#87411=DIRECTION('ref_axis',(0.666102343611793,-0.0042812889172255,-0.745848066565896));
#87412=DIRECTION('',(-0.998646620316722,0.,-0.0520089197156425));
#87413=DIRECTION('center_axis',(-0.113998684179924,-0.987363722714415,-0.110078058998048));
#87414=DIRECTION('ref_axis',(0.807888800879984,-0.0276461771046428,-0.588686142442813));
#87415=DIRECTION('center_axis',(0.110880275037949,-0.987366232725912,0.113196674333434));
#87416=DIRECTION('ref_axis',(0.84938348857533,0.035011289492792,-0.526613614468572));
#87417=DIRECTION('',(0.26547247756443,0.,-0.964118438603786));
#87418=DIRECTION('center_axis',(2.40783168670246E-14,-1.,-1.73734121000225E-14));
#87419=DIRECTION('ref_axis',(1.,2.40783168670246E-14,4.08008794519545E-31));
#87420=DIRECTION('center_axis',(-0.0728831555136991,0.987363722760243,-0.140715758248324));
#87421=DIRECTION('ref_axis',(0.767503369580905,-0.0345726406209256,-0.640111951304187));
#87422=DIRECTION('center_axis',(0.0961353783662722,0.987363722591744,0.12597963460872));
#87423=DIRECTION('ref_axis',(0.81086452814338,-0.0042812878077453,-0.585218239269352));
#87424=DIRECTION('',(-0.964118437085268,0.,-0.265472483079246));
#87425=DIRECTION('center_axis',(-0.0876699255670326,-0.987363722825506,
-0.132010844248598));
#87426=DIRECTION('ref_axis',(0.915550928733872,-0.0276461726499358,-0.401250776986605));
#87427=DIRECTION('center_axis',(0.0839540246621183,-0.98736623247613,0.134386177521815));
#87428=DIRECTION('ref_axis',(0.942731734454702,0.0350112977016713,-0.331709339460428));
#87429=DIRECTION('',(0.466522844039702,0.,-0.884509149748666));
#87430=DIRECTION('center_axis',(-1.6350089538668E-13,-1.,7.07466299821404E-14));
#87431=DIRECTION('ref_axis',(1.,-1.6350089538668E-13,-1.81849133261287E-30));
#87432=DIRECTION('center_axis',(-0.0409294619248677,0.987363722825902,-0.153093624929051));
#87433=DIRECTION('ref_axis',(0.887164714821792,-0.0345726379632342,-0.460155953432563));
#87434=DIRECTION('center_axis',(0.0668058915489451,0.987363722561016,0.143700564455411));
#87435=DIRECTION('ref_axis',(0.91771158853251,-0.00428129039750786,-0.397224257599745));
#87436=DIRECTION('',(-0.88450914743618,0.,-0.466522848424086));
#87437=DIRECTION('center_axis',(-0.0572418275556243,-0.987363722669453,
-0.147770945501514));
#87438=DIRECTION('ref_axis',(0.980402912820427,-0.0276461782575986,-0.195053370545015));
#87439=DIRECTION('center_axis',(0.053102164630045,-0.987366232647523,0.149291937957282));
#87440=DIRECTION('ref_axis',(0.99199889342554,0.0350112918481292,-0.121294702628058));
#87441=DIRECTION('',(0.64575912037299,0.,-0.763541196305152));
#87442=DIRECTION('center_axis',(-2.91477949413467E-14,-1.,5.65745894311796E-15));
#87443=DIRECTION('ref_axis',(1.,-2.91477949413467E-14,2.51222006692366E-32));
#87444=DIRECTION('center_axis',(-0.00706194962947178,0.987363722828334,
-0.158313005498612));
#87445=DIRECTION('ref_axis',(0.9653432251743,-0.0345726379281121,-0.258683571795296));
#87446=DIRECTION('center_axis',(0.0343526394950947,0.987363722496506,0.154702216071917));
#87447=DIRECTION('ref_axis',(0.981647474883865,-0.00428129655811406,-0.190656511963041));
#87448=DIRECTION('',(-0.763541191686731,0.,-0.645759125833779));
#87449=DIRECTION('',(0.794800418951332,0.,-0.606870903928329));
#87450=DIRECTION('',(-0.606870901804627,0.,-0.794800420572888));
#87451=DIRECTION('center_axis',(0.0100961397169233,-0.98736372283294,-0.158148496029187));
#87452=DIRECTION('ref_axis',(0.971690369534208,-0.0276461723068847,0.234634854425451));
#87453=DIRECTION('center_axis',(-0.0144918387531781,-0.987366232640024,
0.15779071345234));
#87454=DIRECTION('ref_axis',(0.951244135720145,0.0350112914715787,0.306445433523697));
#87455=DIRECTION('',(0.906677731515565,0.,-0.421824004975759));
#87456=DIRECTION('center_axis',(2.88293275590696E-14,-1.,7.10427075007399E-15));
#87457=DIRECTION('ref_axis',(1.,2.88293275590696E-14,-2.33857374721434E-31));
#87458=DIRECTION('center_axis',(0.0600646558953371,0.987363722772028,-0.146646227588495));
#87459=DIRECTION('ref_axis',(0.984740195112118,-0.0345726400867478,0.170562248718703));
#87460=DIRECTION('center_axis',(-0.0337801645468462,0.987363722504648,0.154828227287382));
#87461=DIRECTION('ref_axis',(0.970973710277041,-0.00428129541679956,0.239147913351531));
#87462=DIRECTION('',(-0.421824000481472,0.,-0.906677733606493));
#87463=DIRECTION('center_axis',(0.0438573487855876,-0.987363722845839,-0.15228070056808));
#87464=DIRECTION('ref_axis',(0.898533230833495,-0.0276461728542834,0.438033928154466));
#87465=DIRECTION('center_axis',(-0.0480733690119884,-0.987366232709415,
0.150986336127));
#87466=DIRECTION('ref_axis',(0.863127866602312,0.0350112889476249,0.503770280525527));
#87467=DIRECTION('',(0.976159801597288,0.,-0.217053085086444));
#87468=DIRECTION('center_axis',(1.06512422773008E-13,-1.,5.25425203349921E-14));
#87469=DIRECTION('ref_axis',(1.,1.06512422773008E-13,-2.10878361398876E-32));
#87470=DIRECTION('center_axis',(0.0901849798539102,0.987363722846681,-0.130305595486506));
#87471=DIRECTION('ref_axis',(0.925051675281031,-0.0345726381980344,0.37826463057995));
#87472=DIRECTION('center_axis',(-0.0662738964295295,0.987363722501191,0.143946692010062));
#87473=DIRECTION('ref_axis',(0.896863152081214,-0.00428129419318685,0.442287414425258));
#87474=DIRECTION('',(-0.217053076899258,0.,-0.976159803417742));
#87475=DIRECTION('center_axis',(0.0755678353822223,-0.987363722751612,-0.13929243069788));
#87476=DIRECTION('ref_axis',(0.783361677221614,-0.0276461756599869,0.620951021926784));
#87477=DIRECTION('center_axis',(-0.0794070357866266,-0.987366232591193,
0.137122009197124));
#87478=DIRECTION('ref_axis',(0.734652698085276,0.0350112936683274,0.677539388162558));
#87479=DIRECTION('',(0.999997725152046,0.,-0.00213300040646513));
#87480=DIRECTION('center_axis',(9.27271328152013E-14,-1.,7.42111278501564E-14));
#87481=DIRECTION('ref_axis',(1.,9.27271328152013E-14,1.68823144866391E-30));
#87482=DIRECTION('center_axis',(0.116088355864864,0.987363722833873,-0.107872018912356));
#87483=DIRECTION('ref_axis',(0.822108766551035,-0.0345726372684886,0.568279780312688));
#87484=DIRECTION('center_axis',(-0.0956687346786959,0.987363722549271,0.126334368240095));
#87485=DIRECTION('ref_axis',(0.780816270242319,-0.00428129210391877,0.624746046536347));
#87486=DIRECTION('',(-0.00213299544913877,0.,-0.99999772516262));
#87487=DIRECTION('center_axis',(0.103744855571448,-0.98736372273247,-0.11979100122437));
#87488=DIRECTION('ref_axis',(0.631561003133862,-0.0276461768120529,0.774833135731963));
#87489=DIRECTION('center_axis',(-0.107027725080779,-0.987366232739294,0.116846003398692));
#87490=DIRECTION('ref_axis',(0.571825985200744,0.0350112887521891,0.819627508267694));
#87491=DIRECTION('',(0.977076865850012,0.,0.212886820213741));
#87492=DIRECTION('center_axis',(5.59545188505727E-14,-1.,6.930727908743E-14));
#87493=DIRECTION('ref_axis',(1.90179785867072E-30,-6.930727908743E-14,-1.));
#87494=DIRECTION('center_axis',(0.136563569902686,0.987363722841023,-0.0803944661836259));
#87495=DIRECTION('ref_axis',(0.68072496630421,-0.0345726372125825,0.731722797927125));
#87496=DIRECTION('center_axis',(-0.120590206989186,0.987363722543446,0.10281479165691));
#87497=DIRECTION('ref_axis',(0.628259286757571,-0.00428129314207606,0.777992248760809));
#87498=DIRECTION('',(0.212886825057003,0.,-0.977076864794756));
#87499=DIRECTION('center_axis',(0.127070884961093,-0.987363722842759,-0.0946882728181883));
#87500=DIRECTION('ref_axis',(0.450229235832201,-0.0276461724272758,0.892484915475928));
#87501=DIRECTION('center_axis',(-0.129643916496959,-0.987366232921069,0.0911064048384507));
#87502=DIRECTION('ref_axis',(0.382261324293031,0.0350112812986391,0.923390757010035));
#87503=DIRECTION('',(0.90846897872148,0.,0.417952287588848));
#87504=DIRECTION('center_axis',(-3.97473170466724E-14,-1.,-7.97154810525488E-14));
#87505=DIRECTION('ref_axis',(1.34542241016887E-30,7.97154810525487E-14,
-1.));
#87506=DIRECTION('center_axis',(0.150653221823406,0.987363722937457,-0.0491577601331854));
#87507=DIRECTION('ref_axis',(0.507511223892755,-0.0345726343239725,0.860951270734168));
#87508=DIRECTION('center_axis',(-0.139873017737147,0.987363722559245,0.0744877055832257));
#87509=DIRECTION('ref_axis',(0.446325598059899,-0.00428128909263173,0.894860397537057));
#87510=DIRECTION('',(0.417952293183605,0.,-0.908468976147544));
#87511=DIRECTION('center_axis',(0.144455217576619,-0.98736372279966,-0.0651580310789709));
#87512=DIRECTION('ref_axis',(0.247845252571248,-0.0276461738326995,0.968405090780871));
#87513=DIRECTION('center_axis',(-0.146198094728699,-0.987366232569038,0.061106790785668));
#87514=DIRECTION('ref_axis',(0.174822551263119,0.035011294342318,0.983977278618937));
#87515=DIRECTION('',(0.797382090536838,0.,0.603474773036207));
#87516=DIRECTION('center_axis',(-7.22719159625212E-15,-1.,-2.8798758529663E-14));
#87517=DIRECTION('ref_axis',(1.69754332887121E-32,2.8798758529663E-14,-1.));
#87518=DIRECTION('center_axis',(0.157698499589171,0.987363722825349,-0.0156224862231097));
#87519=DIRECTION('ref_axis',(0.310566820979779,-0.03457263809742,0.949922619165108));
#87520=DIRECTION('center_axis',(-0.152615518808298,0.987363722561227,0.0426776614742487));
#87521=DIRECTION('ref_axis',(0.243522219297542,-0.00428129052954995,0.969885869192763));
#87522=DIRECTION('',(0.60347477560539,0.,-0.797382088592429));
#87523=DIRECTION('center_axis',(0.155084985266925,-0.98736372273477,-0.0325810738327332));
#87524=DIRECTION('ref_axis',(0.0338722990281305,-0.0276461769946432,0.9990437208932));
#87525=DIRECTION('center_axis',(-0.155916218266008,-0.987366232783829,0.0282498715023055));
#87526=DIRECTION('ref_axis',(-0.0407907327075091,0.0350112867431234,0.998554117675039));
#87527=DIRECTION('',(0.649010505773103,0.,0.760779444646174));
#87528=DIRECTION('center_axis',(0.,-1.,0.));
#87529=DIRECTION('ref_axis',(0.0292115385192369,0.,0.999573251951721));
#87530=DIRECTION('center_axis',(0.157369968982369,0.987363722822651,0.0186432753636022));
#87531=DIRECTION('ref_axis',(0.0991006546873935,-0.0345726382874032,0.994476642723387));
#87532=DIRECTION('center_axis',(-0.158221888564979,0.987363722509714,0.00887206011545954));
#87533=DIRECTION('ref_axis',(0.0293320137080374,-0.00428129435385591,0.999560555189373));
#87534=DIRECTION('center_axis',(-0.16378581394621,-0.986495109396061,0.00126739403137102));
#87535=DIRECTION('ref_axis',(0.0279022377807928,-0.00334831589290775,0.999605048960591));
#87536=DIRECTION('center_axis',(0.162023731906375,-0.986495109491454,-0.0239939419140432));
#87537=DIRECTION('ref_axis',(0.13673669353806,-0.00163604997374152,0.990606077096624));
#87538=DIRECTION('center_axis',(-0.159684138304561,-0.986495109470319,0.0364468786739426));
#87539=DIRECTION('ref_axis',(0.242135436420398,-0.00334830841955299,0.970236682083414));
#87540=DIRECTION('center_axis',(0.153077721675863,-0.986495109421554,-0.0582632835830904));
#87541=DIRECTION('ref_axis',(0.346490890519673,-0.00163604293581091,0.938051910157639));
#87542=DIRECTION('center_axis',(-0.148115812598509,-0.986495109422795,0.0699221362888171));
#87543=DIRECTION('ref_axis',(0.445046649327853,-0.00334831284885684,0.895501127147876));
#87544=DIRECTION('center_axis',(0.13697396453894,-0.986495109434819,-0.089808307520348));
#87545=DIRECTION('ref_axis',(0.540043558052671,-0.00163604532087848,0.841635478554415));
#87546=DIRECTION('center_axis',(-0.129621748464855,-0.986495109530296,0.100127924165659));
#87547=DIRECTION('ref_axis',(0.627147978031225,-0.00334830330694471,0.778892933923726));
#87548=DIRECTION('center_axis',(0.114465459146429,-0.986495109423811,-0.117153991589281));
#87549=DIRECTION('ref_axis',(0.708344388266892,-0.00163604390614199,0.705865108197834));
#87550=DIRECTION('center_axis',(-0.105066725885366,-0.986495109424266,0.125651829249456));
#87551=DIRECTION('ref_axis',(0.779924561865009,-0.00334830996305795,0.625864575303687));
#87552=DIRECTION('center_axis',(0.0866046722159151,-0.986495109483246,-0.13902168793398));
#87553=DIRECTION('ref_axis',(0.843523823647868,-0.00163604705472412,0.537089268454058));
#87554=DIRECTION('center_axis',(-0.0755988969195904,-0.98649510943077,0.145300398670181));
#87555=DIRECTION('ref_axis',(0.896232743138345,-0.00334831229899437,0.443571481197186));
#87556=DIRECTION('center_axis',(0.0546943551485009,-0.986495109420496,-0.154388881090361));
#87557=DIRECTION('ref_axis',(0.939261021775134,-0.00163604133811556,0.343199732433856));
#87558=DIRECTION('center_axis',(-0.0425961438623839,-0.986495109459446,
0.158154884656308));
#87559=DIRECTION('ref_axis',(0.970634076275854,-0.00334831006889112,0.240537478975321));
#87560=DIRECTION('center_axis',(0.0202265784150031,-0.986495109504033,-0.162537024859717));
#87561=DIRECTION('ref_axis',(0.991079418779179,-0.00163604856804703,0.133262556696951));
#87562=DIRECTION('center_axis',(-0.00760164204240845,-0.986495109429919,
0.163614223431558));
#87563=DIRECTION('ref_axis',(0.99964963868433,-0.00334830736092119,0.0262562129048713));
#87564=DIRECTION('center_axis',(-0.0151869653104653,-0.986495109510341,
-0.163085115804104));
#87565=DIRECTION('ref_axis',(0.996556043201398,-0.00163605039412049,-0.0829058266823295));
#87566=DIRECTION('center_axis',(0.0277482981921578,-0.986495109405202,0.161423142910355));
#87567=DIRECTION('ref_axis',(0.981922695164601,-0.0033483111612951,-0.189252766249411));
#87568=DIRECTION('center_axis',(-0.0498903778715741,-0.98649510947419,-0.15600752923926));
#87569=DIRECTION('ref_axis',(0.955434815240343,-0.00163604664715935,-0.295197623936948));
#87570=DIRECTION('center_axis',(0.0618007641807002,-0.986495109440824,0.151684094736456));
#87571=DIRECTION('ref_axis',(0.918282137943364,-0.00334830913939569,-0.395912495332078));
#87572=DIRECTION('center_axis',(-0.0822609769858708,-0.98649510948161,-0.141635202665852));
#87573=DIRECTION('ref_axis',(0.869638516258114,-0.00163604780339735,-0.49368631172838));
#87574=DIRECTION('center_axis',(0.0929634947864884,-0.986495109470967,0.134852466150781));
#87575=DIRECTION('ref_axis',(0.81170372863756,-0.003348307097733,-0.584059796386861));
#87576=DIRECTION('center_axis',(-0.110785141534113,-0.986495109446713,-0.120640173462175));
#87577=DIRECTION('ref_axis',(0.743178886612869,-0.00163604553725314,-0.66909077549153));
#87578=DIRECTION('center_axis',(0.119779353350238,-0.986495109452289,0.111715287842424));
#87579=DIRECTION('ref_axis',(0.667170953063073,-0.0033483085449882,-0.744897112505344));
#87580=DIRECTION('center_axis',(-0.134129119919762,-0.986495109493058,-0.0940041389292526));
#87581=DIRECTION('ref_axis',(0.581969039393171,-0.00163605002861843,-0.813209296877559));
#87582=DIRECTION('center_axis',(0.140994461083604,-0.986495109424135,0.0833544301522559));
#87583=DIRECTION('ref_axis',(0.491442007146395,-0.00334831305064004,-0.870903865195027));
#87584=DIRECTION('center_axis',(-0.151201364943228,-0.986495109443453,-0.0629725835856714));
#87585=DIRECTION('ref_axis',(0.393546966780992,-0.00163604463201623,-0.919303055741382));
#87586=DIRECTION('center_axis',(0.155616827764946,-0.986495109435589,0.0510960074373685));
#87587=DIRECTION('ref_axis',(0.292733778957593,-0.00334831188603403,-0.956188121378174));
#87588=DIRECTION('center_axis',(-0.161203605678199,-0.986495109504632,-0.0289964901288311));
#87589=DIRECTION('ref_axis',(0.186723073336949,-0.00163604993960994,-0.982411226128956));
#87590=DIRECTION('center_axis',(0.16296272405839,-0.986495109424208,0.0164483935260796));
#87591=DIRECTION('ref_axis',(0.0803376455401133,-0.00334831203061902,-0.996762083706848));
#87592=DIRECTION('center_axis',(-0.163668143673876,-0.986495109448053,0.00633543853423027));
#87593=DIRECTION('ref_axis',(-0.028831781957428,-0.0016360466685548,-0.99958293888024));
#87594=DIRECTION('center_axis',(0.162688663305374,-0.986495109493919,-0.0189683361550779));
#87595=DIRECTION('ref_axis',(-0.135814987330012,-0.00334830488654736,-0.990728559228478));
#87596=DIRECTION('center_axis',(-0.158479742471285,-0.986495109454043,0.0413711282114918));
#87597=DIRECTION('ref_axis',(-0.24303849268562,-0.00163604274440781,-0.970015265053721));
#87598=DIRECTION('center_axis',(0.154807463282918,-0.98649510940734,-0.0534981161098913));
#87599=DIRECTION('ref_axis',(-0.345617063849709,-0.00334831002481114,-0.938369668092423));
#87600=DIRECTION('center_axis',(-0.145881002803882,-0.986495109476937,0.0744723572812044));
#87601=DIRECTION('ref_axis',(-0.445880998647102,-0.00163604585829139,-0.895090754281046));
#87602=DIRECTION('center_axis',(0.139687636995712,-0.98649510943774,-0.08552638847733));
#87603=DIRECTION('ref_axis',(-0.539258470200199,-0.0033483099529629,-0.842133653963431));
#87604=DIRECTION('center_axis',(-0.12646103108995,-0.98649510948253,0.104091337693001));
#87605=DIRECTION('ref_axis',(-0.627874600291905,-0.0016360454288523,-0.778312796800641));
#87606=DIRECTION('center_axis',(0.118036173957979,-0.986495109402125,-0.113555540433086));
#87607=DIRECTION('ref_axis',(-0.707684749028207,-0.00334831214599302,-0.706520406498395));
#87608=DIRECTION('center_axis',(-0.101127883902599,-0.986495109422555,0.128843122372763));
#87609=DIRECTION('ref_axis',(-0.780509485663125,-0.00163604296041615,-0.625141796837578));
#87610=DIRECTION('center_axis',(0.0908654643575122,-0.986495109472117,-0.136274966060128));
#87611=DIRECTION('ref_axis',(-0.843020475033029,-0.0033483062137657,-0.537871051015562));
#87612=DIRECTION('center_axis',(-0.071066104503773,-0.986495109454203,0.147570348693763));
#87613=DIRECTION('ref_axis',(-0.89664861531436,-0.00163604600655692,-0.442739860424047));
#87614=DIRECTION('center_axis',(0.0594459877428719,-0.986495109509029,-0.152622322928339));
#87615=DIRECTION('ref_axis',(-0.938937501589155,-0.00334830299426047,-0.34407144167538));
#87616=DIRECTION('center_axis',(-0.0376813513430268,-0.986495109508868,
0.159397348397173));
#87617=DIRECTION('ref_axis',(-0.970861451591853,-0.00163605045407286,-0.239635901216558));
#87618=DIRECTION('center_axis',(0.0252468968154617,-0.986495109386897,-0.161833226986684));
#87619=DIRECTION('ref_axis',(-0.990950853825989,-0.00334831436270505,-0.134183434493504));
#87620=DIRECTION('center_axis',(-0.00253466500971984,-0.986495109498837,
0.163771103703207));
#87621=DIRECTION('ref_axis',(-0.999677885568108,-0.00163604943518171,-0.0253268325757907));
#87622=DIRECTION('center_axis',(-0.010132729717057,-0.986495109483762,-0.163476991509819));
#87623=DIRECTION('ref_axis',(-0.996628445590177,-0.00334830604890707,0.081978840484062));
#87624=DIRECTION('center_axis',(0.0327305358517654,-0.986495109457993,0.160487105520406));
#87625=DIRECTION('ref_axis',(-0.981750492616112,-0.00163604488853,0.190166489174997));
#87626=DIRECTION('center_axis',(-0.0450385505003737,-0.986495109440284,
-0.157476753901098));
#87627=DIRECTION('ref_axis',(-0.955704798411601,-0.00334830901293553,0.294307878113712));
#87628=DIRECTION('center_axis',(0.0664652997818561,-0.986495109455715,0.149698907627493));
#87629=DIRECTION('ref_axis',(-0.917917538204367,-0.00163604722328872,0.396767836910097));
#87630=DIRECTION('center_axis',(-0.0778384232825467,-0.986495109488177,
-0.144113076494802));
#87631=DIRECTION('ref_axis',(-0.870093457590691,-0.0033483064689008,0.492875404033988));
#87632=DIRECTION('center_axis',(0.0970922171638184,-0.986495109489498,0.131910956025336));
#87633=DIRECTION('ref_axis',(-0.811163778570785,-0.00163604589998996,0.584816764199334));
#87634=DIRECTION('center_axis',(-0.106998645562323,-0.986495109310941,-0.12401084288651));
#87635=DIRECTION('ref_axis',(-0.743797514851689,-0.00334832064433674,0.66839662300861));
#87636=DIRECTION('center_axis',(0.123179209311741,-0.986495109425282,0.107954997444934));
#87637=DIRECTION('ref_axis',(-0.666480903457418,-0.00163604240632611,0.745520307363809));
#87638=DIRECTION('center_axis',(-0.13115574995207,-0.986495109501473,-0.0981099800437549));
#87639=DIRECTION('ref_axis',(-0.582722423500651,-0.00334830642559605,0.812664362448365));
#87640=DIRECTION('center_axis',(0.143506484117382,-0.986495109477908,0.0789511747375405));
#87641=DIRECTION('ref_axis',(-0.49063412094358,-0.00163604904476048,0.871364150461472));
#87642=DIRECTION('center_axis',(-0.149180147807827,-0.986495109495363,-0.0676216122387367));
#87643=DIRECTION('ref_axis',(-0.394399880085478,-0.00334830475442072,0.918932817698787));
#87644=DIRECTION('center_axis',(0.157123550617762,-0.986495109493207,0.046255689242015));
#87645=DIRECTION('ref_axis',(-0.291845832604245,-0.00163604775031448,0.956463973884691));
#87646=DIRECTION('center_axis',(-0.160229045095317,-0.986495109390512,-0.0339713446369772));
#87647=DIRECTION('ref_axis',(-0.187635640680993,-0.00334831465490897,0.982232994322225));
#87648=DIRECTION('center_axis',(0.163393695261222,-0.986495109401722,0.0113973451016927));
#87649=DIRECTION('ref_axis',(-0.0794111591883371,-0.00163604091525733,0.996840604693894));
#87650=DIRECTION('center_axis',(0.156388912663533,0.986495110500922,0.048681669586124));
#87651=DIRECTION('ref_axis',(-0.0847582830594673,-0.0357022416614575,0.995761710146136));
#87652=DIRECTION('center_axis',(-0.160735557249259,0.986495110220615,-0.0314877459750204));
#87653=DIRECTION('ref_axis',(-0.18718085442266,0.000856146315673481,0.982325096264515));
#87654=DIRECTION('center_axis',(0.142267507527056,0.986495108892049,0.0811625309739932));
#87655=DIRECTION('ref_axis',(-0.296836013366402,-0.0357022594544976,0.954260829039202));
#87656=DIRECTION('center_axis',(-0.150208717742484,0.986495110197419,-0.0653049666621294));
#87657=DIRECTION('ref_axis',(-0.393975526808956,0.000856139022975812,0.919120531432945));
#87658=DIRECTION('center_axis',(0.121493832547411,0.986495110620511,0.109848283440242));
#87659=DIRECTION('ref_axis',(-0.495034021429636,-0.0357022382722387,0.868139774350626));
#87660=DIRECTION('center_axis',(-0.132658279393524,0.986495110257214,-0.09606861270445));
#87661=DIRECTION('ref_axis',(-0.582348345137894,0.000856146012755316,0.812938910330389));
#87662=DIRECTION('center_axis',(0.0950392389665278,0.986495110605003,0.133397675426094));
#87663=DIRECTION('ref_axis',(-0.670084790738196,-0.0357022400622654,0.741425467107709));
#87664=DIRECTION('center_axis',(-0.108904892632645,0.986495110251071,-0.122340188864495));
#87665=DIRECTION('ref_axis',(-0.743491199728451,0.00085614329103587,0.668745170408739));
#87666=DIRECTION('center_axis',(0.0641407206135473,0.986495110682393,0.150709537053595));
#87667=DIRECTION('ref_axis',(-0.813803139234317,-0.0357022364465081,0.580042930208694));
#87668=DIRECTION('center_axis',(-0.0800592318971177,0.986495110224998,-0.142891276466454));
#87669=DIRECTION('ref_axis',(-0.869869231963275,0.000856144207940989,0.493281650075002));
#87670=DIRECTION('center_axis',(0.0302430480138401,0.986495110576137,0.160974391926818));
#87671=DIRECTION('ref_axis',(-0.919468959214345,-0.0357022389103626,0.391538226969062));
#87672=DIRECTION('center_axis',(-0.0474700944979826,0.986495110139844,-0.156760925611356));
#87673=DIRECTION('ref_axis',(-0.955573145865708,0.000856140779035256,0.294752828524647));
#87674=DIRECTION('center_axis',(-0.00506877555079224,0.986495108775113,
0.16371227161454));
#87675=DIRECTION('ref_axis',(-0.982141430286934,-0.0357022625894564,0.184725632655374));
#87676=DIRECTION('center_axis',(-0.0126613009637376,0.98649511023473,-0.16330060912585));
#87677=DIRECTION('ref_axis',(-0.996595522149375,0.000856144484601801,0.0824416899901725));
#87678=DIRECTION('center_axis',(-0.0401435441044833,0.986495110627201,0.158795127681416));
#87679=DIRECTION('ref_axis',(-0.998890061000584,-0.0357022375529674,-0.0307245222576411));
#87680=DIRECTION('center_axis',(0.0227395142084494,0.986495110181865,-0.162204537793593));
#87681=DIRECTION('ref_axis',(-0.991018199204409,0.000856141725757606,-0.13372432788014));
#87682=DIRECTION('center_axis',(-0.0733412699600103,0.986495110625005,0.146452909952692));
#87683=DIRECTION('ref_axis',(-0.968931701865205,-0.0357022384448084,-0.244738038095078));
#87684=DIRECTION('center_axis',(0.0570770554642903,0.986495110139408,-0.153523963636179));
#87685=DIRECTION('ref_axis',(-0.939101966597582,0.000856138904126028,-0.343637546491547));
#87686=DIRECTION('center_axis',(-0.103109656079224,0.986495108998291,0.127262715457723));
#87687=DIRECTION('ref_axis',(-0.893667172076722,-0.0357022550788138,-0.447307874438492));
#87688=DIRECTION('center_axis',(0.0887457420158007,0.98649511016544,-0.137664777244365));
#87689=DIRECTION('ref_axis',(-0.843274368614031,0.000856141453340625,-0.537482656706633));
#87690=DIRECTION('center_axis',(-0.128056731448259,0.986495108989023,0.102121855993337));
#87691=DIRECTION('ref_axis',(-0.776615760027788,-0.0357022549333386,-0.62896208969153));
#87692=DIRECTION('center_axis',(0.116264778148262,0.986495110253181,-0.115368534742798));
#87693=DIRECTION('ref_axis',(-0.708016200426445,0.000856148759243582,-0.706195671852358));
#87694=DIRECTION('center_axis',(-0.14701601859467,0.986495108895636,0.0722058889673023));
#87695=DIRECTION('ref_axis',(-0.623250656744172,-0.0357022582606523,-0.781206738080931));
#87696=DIRECTION('center_axis',(0.138347393324671,0.986495110212549,-0.0876777981418294));
#87697=DIRECTION('ref_axis',(-0.539651979497943,0.000856141284190815,-0.841887764518557));
#87698=DIRECTION('center_axis',(-0.159100984330672,0.986495110516033,0.038913670001308));
#87699=DIRECTION('ref_axis',(-0.440743048472606,-0.0357022410037261,-0.89692302635755));
#87700=DIRECTION('center_axis',(0.153961042610626,0.986495110180795,-0.0558873415688195));
#87701=DIRECTION('ref_axis',(-0.346054235065791,0.000856139963462675,-0.938214119173972));
#87702=DIRECTION('center_axis',(-0.163746580379322,0.98649511053951,0.00380188055029804));
#87703=DIRECTION('ref_axis',(-0.237626784347645,-0.0357022419978828,-0.970700191241829));
#87704=DIRECTION('center_axis',(0.162375645555585,0.986495110193823,-0.0214836517865166));
#87705=DIRECTION('ref_axis',(-0.136275375117657,0.000856141339044354,-0.990670625969373));
#87706=DIRECTION('center_axis',(-0.160735568247923,0.986495110466998,-0.0314876821110047));
#87707=DIRECTION('ref_axis',(-0.0233993533168982,-0.0357022441336381,-0.999088494593033));
#87708=DIRECTION('center_axis',(0.163197743665279,0.986495110172426,0.0139245850371073));
#87709=DIRECTION('ref_axis',(0.0798755669367271,0.000856138430815477,-0.996804474725873));
#87710=DIRECTION('center_axis',(-0.150208740918371,0.986495110672989,-0.0653049061710207));
#87711=DIRECTION('ref_axis',(0.191922203698308,-0.0357022365974855,-0.980760530419899));
#87712=DIRECTION('center_axis',(0.156388896590614,0.986495110143671,0.0486817284594198));
#87713=DIRECTION('ref_axis',(0.292291616845161,0.000856140246125589,-0.956328854393676));
#87714=DIRECTION('center_axis',(-0.132658318227324,0.986495110593608,-0.0960685556256756));
#87715=DIRECTION('ref_axis',(0.398269690649453,-0.0357022399347559,-0.916573294163446));
#87716=DIRECTION('center_axis',(0.142267476719927,0.986495110210636,0.0811625689480725));
#87717=DIRECTION('ref_axis',(0.491040435894112,0.000856143201521635,-0.871136359782864));
#87718=DIRECTION('center_axis',(-0.108904939865473,0.98649511054227,-0.122340144470624));
#87719=DIRECTION('ref_axis',(0.585994532833131,-0.0357022411327852,-0.809528107892356));
#87720=DIRECTION('center_axis',(0.121493790101187,0.986495110177345,0.109848334366241));
#87721=DIRECTION('ref_axis',(0.666828750295423,0.000856141722682205,-0.745210496974375));
#87722=DIRECTION('center_axis',(-0.0800592794798436,0.986495108881712,-0.142891259080559));
#87723=DIRECTION('ref_axis',(0.746318920951353,-0.0357022584185192,-0.66463028592882));
#87724=DIRECTION('center_axis',(0.0950391876824411,0.986495110247087,0.133397714610294));
#87725=DIRECTION('ref_axis',(0.81143689427034,0.000856141536668781,-0.584439418279238));
#87726=DIRECTION('center_axis',(-0.0474701529820085,0.986495110541533,-0.156760905373482));
#87727=DIRECTION('ref_axis',(0.871746264002991,-0.0357022413027112,-0.488655094276924));
#87728=DIRECTION('center_axis',(0.0641406633761717,0.986495110174397,0.150709564738503));
#87729=DIRECTION('ref_axis',(0.918103148850275,0.00085613707607792,-0.396340604910116));
#87730=DIRECTION('center_axis',(-0.0126613729171963,0.986495110734072,-0.163300600530505));
#87731=DIRECTION('ref_axis',(0.956411720781313,-0.0357022349766519,-0.289830934804756));
#87732=DIRECTION('center_axis',(0.0302429834584108,0.986495110181741,0.160974406472113));
#87733=DIRECTION('ref_axis',(0.981839921951651,0.000856142423214422,-0.189709342632688));
#87734=DIRECTION('center_axis',(0.022739465422101,0.986495108959912,-0.162204552064631));
#87735=DIRECTION('ref_axis',(0.996356429529177,-0.0357022555345247,-0.0774545949935659));
#87736=DIRECTION('center_axis',(-0.00506882451442394,0.98649511023803,0.163712261283324));
#87737=DIRECTION('ref_axis',(0.999666951069067,0.000856147178261841,0.0257925173700458));
#87738=DIRECTION('center_axis',(0.0570769958324413,0.986495110611179,-0.153523982774619));
#87739=DIRECTION('ref_axis',(0.989712619250393,-0.0357022389867386,0.138543427949004));
#87740=DIRECTION('center_axis',(-0.040143616149589,0.986495110223746,0.158795111974751));
#87741=DIRECTION('ref_axis',(0.970750664504711,0.000856148292627332,0.240088347017847));
#87742=DIRECTION('center_axis',(0.0887456881072519,0.98649511049776,-0.137664809615175));
#87743=DIRECTION('ref_axis',(0.936790945359738,-0.0357022412121723,0.348063319906647));
#87744=DIRECTION('center_axis',(-0.0733413333034938,0.986495110181623,0.146452881217863));
#87745=DIRECTION('ref_axis',(0.896443156372571,0.000856145515749334,0.443157911367537));
#87746=DIRECTION('center_axis',(0.116264744835295,0.986495108930328,-0.115368579626017));
#87747=DIRECTION('ref_axis',(0.840065968072642,-0.0357022576022493,0.541308154463128));
#87748=DIRECTION('center_axis',(-0.103109690306789,0.986495110153459,0.127262678771715));
#87749=DIRECTION('ref_axis',(0.780218961813407,0.000856140399447746,0.6255059061675));
#87750=DIRECTION('center_axis',(0.138347353699895,0.986495110711692,-0.087677855049969));
#87751=DIRECTION('ref_axis',(0.704060443534308,-0.0357022349542924,0.709242019531797));
#87752=DIRECTION('center_axis',(-0.128056758497583,0.986495110176505,0.102121810603498));
#87753=DIRECTION('ref_axis',(0.627512595764402,0.000856142745096334,0.778605939597575));
#87754=DIRECTION('center_axis',(0.153961016969757,0.986495110699521,-0.0558874030491539));
#87755=DIRECTION('ref_axis',(0.535133832406667,-0.0357022359846592,0.844012518721997));
#87756=DIRECTION('center_axis',(-0.147016033672443,0.986495110214052,0.0722058402553995));
#87757=DIRECTION('ref_axis',(0.44546443861938,0.000856144275045226,0.895299224249916));
#87758=DIRECTION('center_axis',(0.162375647399458,0.98649510885926,-0.021483699131286));
#87759=DIRECTION('ref_axis',(0.341184955381354,-0.0357022593273061,0.939317930681805));
#87760=DIRECTION('center_axis',(-0.159101001719445,0.986495110234289,0.0389136060486129));
#87761=DIRECTION('ref_axis',(0.242586858202287,0.000856144391280358,0.970129312640498));
#87762=DIRECTION('center_axis',(0.163197746490851,0.986495110577267,0.0139245232397132));
#87763=DIRECTION('ref_axis',(0.131282652802152,-0.0357022392364338,0.990701880076309));
#87764=DIRECTION('center_axis',(-0.16374658378085,0.986495110232372,0.00380181374105046));
#87765=DIRECTION('ref_axis',(0.0283661888251914,0.000856146182459187,0.999597232061618));
#87766=DIRECTION('center_axis',(0.158420667740754,0.98736372234608,0.00397137601677981));
#87767=DIRECTION('ref_axis',(0.100692121386749,-0.0201568010854275,0.994713426098511));
#87768=DIRECTION('',(-0.603992234724004,0.,0.796990200939199));
#87769=DIRECTION('center_axis',(-0.155915203883767,0.987363722011716,0.028343070635579));
#87770=DIRECTION('ref_axis',(0.241038780754158,0.0102046916675105,0.970461833582609));
#87771=DIRECTION('',(-0.796990199392668,0.,-0.603992236764708));
#87772=DIRECTION('center_axis',(5.40637229578749E-15,-1.,2.16025825271405E-14));
#87773=DIRECTION('ref_axis',(2.85199720979946E-32,-2.16025825271405E-14,
-1.));
#87774=DIRECTION('center_axis',(-0.158340230226139,-0.987363723437772,0.00642254863998973));
#87775=DIRECTION('ref_axis',(0.165682556882615,-0.020156456391398,0.985973127225373));
#87776=DIRECTION('center_axis',(0.149874468456674,-0.987363722435678,-0.0514832334142992));
#87777=DIRECTION('ref_axis',(0.245294997189495,-0.0133103743988677,0.969357105656717));
#87778=DIRECTION('center_axis',(0.155570608715075,0.987363722361946,-0.0301772342600132));
#87779=DIRECTION('ref_axis',(0.312171979328333,-0.0201568001148959,0.949811749101557));
#87780=DIRECTION('',(-0.418541898467443,0.,0.908197489110859));
#87781=DIRECTION('center_axis',(-0.146177069397483,0.987363722011113,0.0611975885041637));
#87782=DIRECTION('ref_axis',(0.444024037449279,0.0102046886099544,0.895956761511187));
#87783=DIRECTION('',(-0.908197487535576,0.,-0.418541901885662));
#87784=DIRECTION('center_axis',(9.9238909863824E-15,-1.,1.99353159073878E-14));
#87785=DIRECTION('ref_axis',(-1.38974827776255E-31,-1.99353159073878E-14,
-1.));
#87786=DIRECTION('center_axis',(-0.153257664657612,-0.987363723478468,0.0403108643225515));
#87787=DIRECTION('ref_axis',(0.373764067895711,-0.0201564538811349,0.927304771322238));
#87788=DIRECTION('center_axis',(0.13530311636008,-0.987363722522325,-0.0824981584649473));
#87789=DIRECTION('ref_axis',(0.447943259549841,-0.013310367689315,0.893962902102676));
#87790=DIRECTION('center_axis',(0.145446240991836,0.987363722371625,-0.0629147894043416));
#87791=DIRECTION('ref_axis',(0.509055019458456,-0.0201567997961947,0.8604979317733));
#87792=DIRECTION('',(-0.21352100493591,0.,0.976938473216793));
#87793=DIRECTION('center_axis',(-0.129603856677957,0.987363722010123,0.091190574033264));
#87794=DIRECTION('ref_axis',(0.626247222002202,0.0102046859892758,0.779557747263399));
#87795=DIRECTION('',(-0.976938472070386,0.,-0.21352101018115));
#87796=DIRECTION('center_axis',(-1.86365060963677E-14,-1.,-2.31145281227288E-14));
#87797=DIRECTION('ref_axis',(2.57068877191084E-31,2.31145281227288E-14,
-1.));
#87798=DIRECTION('center_axis',(-0.141008943747592,-0.987363723371414,0.0723142831902936));
#87799=DIRECTION('ref_axis',(0.564368787726565,-0.0201564581084856,0.82527667399277));
#87800=DIRECTION('center_axis',(0.11440513999799,-0.987363722521747,-0.109655567072713));
#87801=DIRECTION('ref_axis',(0.629646193568477,-0.0133103666202319,0.776767986637686));
#87802=DIRECTION('center_axis',(0.128520967516312,0.987363722411292,-0.0927105203026545));
#87803=DIRECTION('ref_axis',(0.682135215609266,-0.0201567981133334,0.73094818634122));
#87804=DIRECTION('',(0.00148388924556568,0.,0.999998899035747));
#87805=DIRECTION('center_axis',(-0.10697051813911,0.987363721991061,0.116919582384686));
#87806=DIRECTION('ref_axis',(0.779187780646539,0.0102046930062637,0.626707480992344));
#87807=DIRECTION('',(-0.999998899039541,0.,0.00148388668928533));
#87808=DIRECTION('center_axis',(-2.89621690381482E-14,-1.,-2.32097817301061E-14));
#87809=DIRECTION('ref_axis',(1.,-2.89621690381482E-14,1.79017293909041E-31));
#87810=DIRECTION('center_axis',(-0.122166803468733,-0.987363723230526,0.100936366977346));
#87811=DIRECTION('ref_axis',(0.728584246530449,-0.0201564625201907,0.684659559727556));
#87812=DIRECTION('center_axis',(0.0881577081516817,-0.987363722547253,-0.131685602444131));
#87813=DIRECTION('ref_axis',(0.781907570454382,-0.0133103640089616,0.623252264717966));
#87814=DIRECTION('center_axis',(0.105586199074021,0.987363722361599,-0.118171207700302));
#87815=DIRECTION('ref_axis',(0.823319527157923,-0.0201568003226023,0.567220115652829));
#87816=DIRECTION('',(0.216419402668491,0.,0.976300487631043));
#87817=DIRECTION('center_axis',(-0.0793353484309201,0.987363722023703,0.137181569173284));
#87818=DIRECTION('ref_axis',(0.895694387222186,0.0102046883173652,0.444553066612996));
#87819=DIRECTION('',(-0.976300488927256,0.,0.21641939682108));
#87820=DIRECTION('center_axis',(-1.33097866516519E-14,-1.,-6.57645588484366E-15));
#87821=DIRECTION('ref_axis',(1.,-1.33097866516519E-14,-6.73429246899876E-32));
#87822=DIRECTION('center_axis',(-0.0976122735306192,-0.987363723326527,
0.124838783697059));
#87823=DIRECTION('ref_axis',(0.858731920403179,-0.0201564599673544,0.512028520692209));
#87824=DIRECTION('center_axis',(0.0577881148582087,-0.987363722518273,-0.147558168991057));
#87825=DIRECTION('ref_axis',(0.897607820319684,-0.0133103672525045,0.440593957090368));
#87826=DIRECTION('center_axis',(0.0777143295770213,0.987363722455775,-0.138106345099239));
#87827=DIRECTION('ref_axis',(0.926006332830839,-0.0201567935764935,0.376969461932788));
#87828=DIRECTION('',(0.421235379219816,0.,0.906951352219918));
#87829=DIRECTION('center_axis',(-0.0479905531030168,0.987363722018253,0.151029094068421));
#87830=DIRECTION('ref_axis',(0.970319318195053,0.0102046915939821,0.241611847819925));
#87831=DIRECTION('',(-0.90695135278839,0.,0.421235377995853));
#87832=DIRECTION('center_axis',(-5.76494193762726E-14,-1.,-1.42459652129957E-14));
#87833=DIRECTION('ref_axis',(1.,-5.76494193762726E-14,1.74390848177407E-32));
#87834=DIRECTION('center_axis',(-0.0684934961056325,-0.987363723561827,
0.14290387813265));
#87835=DIRECTION('ref_axis',(0.948726241396025,-0.0201564508034618,0.315455601277865));
#87836=DIRECTION('center_axis',(0.0247164153401507,-0.987363722501066,-0.156531077749984));
#87837=DIRECTION('ref_axis',(0.971336925194111,-0.0133103682563698,0.237333966914409));
#87838=DIRECTION('center_axis',(0.0462086345200734,0.987363722388363,-0.151583778179547));
#87839=DIRECTION('ref_axis',(0.985394110347962,-0.0201567982226793,0.169092136945984));
#87840=DIRECTION('',(0.606354862831809,0.,0.795194177745422));
#87841=DIRECTION('',(-0.795194177911868,0.,0.606354862613527));
#87842=DIRECTION('',(0.763121866258984,0.,0.646254607130507));
#87843=DIRECTION('center_axis',(0.019860431055013,0.987363722013889,0.157221002824649));
#87844=DIRECTION('ref_axis',(0.982088143785789,0.0102046850143543,-0.188145534730805));
#87845=DIRECTION('',(-0.646254610502266,0.,0.763121863403588));
#87846=DIRECTION('center_axis',(7.28786518901112E-15,-1.,-1.40963438107777E-15));
#87847=DIRECTION('ref_axis',(1.,7.28786518901112E-15,2.85675081165747E-33));
#87848=DIRECTION('center_axis',(-0.00215923198134159,-0.98736372357585,
0.158455719630701));
#87849=DIRECTION('ref_axis',(0.993496985649308,-0.0201564503692403,-0.112060059852969));
#87850=DIRECTION('center_axis',(-0.0432936835167879,-0.987363722495348,
-0.15244191178176));
#87851=DIRECTION('ref_axis',(0.981215463559103,-0.013310369158375,-0.192455314671647));
#87852=DIRECTION('center_axis',(-0.0217105580192843,0.987363722442619,-0.156976212448723));
#87853=DIRECTION('ref_axis',(0.965319418559905,-0.0201567957597029,-0.260292381248219));
#87854=DIRECTION('',(0.884206138072509,0.,0.467096890799863));
#87855=DIRECTION('center_axis',(0.0531939704811207,0.987363722010318,0.14927585860542));
#87856=DIRECTION('ref_axis',(0.918681740755121,0.0102046879671231,-0.394866716179819));
#87857=DIRECTION('',(-0.467096893063886,0.,0.884206136876501));
#87858=DIRECTION('center_axis',(6.8144492270499E-15,-1.,-2.94335350051688E-15));
#87859=DIRECTION('ref_axis',(1.,6.8144492270499E-15,-2.58910475522156E-32));
#87860=DIRECTION('center_axis',(0.0319545399416091,-0.987363723398425,0.155215286276574));
#87861=DIRECTION('ref_axis',(0.946179978578477,-0.0201564559808906,-0.323012639720991));
#87862=DIRECTION('center_axis',(-0.075052005512317,-0.987363722501073,-0.139571042689389));
#87863=DIRECTION('ref_axis',(0.916902987768194,-0.0133103685324798,-0.398888136087411));
#87864=DIRECTION('center_axis',(-0.0549482178462372,0.98736372235751,-0.148639069991186));
#87865=DIRECTION('ref_axis',(0.886795619052634,-0.0201568012751914,-0.461722030437587));
#87866=DIRECTION('',(0.96394591401818,0.,0.266098242849622));
#87867=DIRECTION('center_axis',(0.0840402245882483,0.987363722020711,0.134350739069664));
#87868=DIRECTION('ref_axis',(0.812318799598595,0.0102046851148157,-0.583124371142559));
#87869=DIRECTION('',(-0.266098244580434,0.,0.963945913540387));
#87870=DIRECTION('center_axis',(-1.20447943868174E-14,-1.,8.67888936384583E-15));
#87871=DIRECTION('ref_axis',(1.,-1.20447943868174E-14,-1.00100324375465E-31));
#87872=DIRECTION('center_axis',(0.0645741589563264,-0.987363723387579,0.144717157701843));
#87873=DIRECTION('ref_axis',(0.85462064542993,-0.020156456556257,-0.51886151299169));
#87874=DIRECTION('center_axis',(-0.103300975920256,-0.987363722552581,-0.120173989536141));
#87875=DIRECTION('ref_axis',(0.809717148348452,-0.0133103638859008,-0.586669390614233));
#87876=DIRECTION('center_axis',(-0.0856165659527258,0.987363722399913,-0.133351727859263));
#87877=DIRECTION('ref_axis',(0.766806244018913,-0.0201567998990961,-0.641562068354602));
#87878=DIRECTION('',(0.99861265071478,0.,0.0526571346770876));
#87879=DIRECTION('center_axis',(0.110956844469907,0.987363721975615,0.113143533583412));
#87880=DIRECTION('ref_axis',(0.667972736265682,0.0102046905761982,-0.744115775868233));
#87881=DIRECTION('',(-0.0526571372340356,0.,0.998612650579951));
#87882=DIRECTION('center_axis',(0.,-1.,0.));
#87883=DIRECTION('ref_axis',(0.,0.,-1.));
#87884=DIRECTION('center_axis',(0.0941743618905338,-0.987363723370125,0.127452215889697));
#87885=DIRECTION('ref_axis',(0.72310020247839,-0.0201564567588206,-0.69044899480457));
#87886=DIRECTION('center_axis',(-0.126719716985301,-0.9873637224691,-0.0951577263238632));
#87887=DIRECTION('ref_axis',(0.664669831879971,-0.0133103712189968,-0.747018640066406));
#87888=DIRECTION('center_axis',(-0.112281578563455,0.987363722364124,-0.111829007303832));
#87889=DIRECTION('ref_axis',(0.61096185800018,-0.0201567995340252,-0.791403381027345));
#87890=DIRECTION('',(0.986585369800577,0.,-0.1632461579807));
#87891=DIRECTION('center_axis',(0.132685249336737,0.987363721998344,0.0866458602013091));
#87892=DIRECTION('ref_axis',(0.492393009084558,0.0102046921590675,-0.870313155629968));
#87893=DIRECTION('',(0.16324615825273,0.,0.986585369755565));
#87894=DIRECTION('center_axis',(-2.91495530570904E-14,-1.,5.1736898213001E-14));
#87895=DIRECTION('ref_axis',(-3.85548631941165E-31,-5.1736898213001E-14,
-1.));
#87896=DIRECTION('center_axis',(0.11937107525839,-0.987363723316579,0.104227751918948));
#87897=DIRECTION('ref_axis',(0.557768397564044,-0.0201564591618209,-0.829751849550753));
#87898=DIRECTION('center_axis',(-0.144213177987697,-0.9873637224976,-0.0656919994395904));
#87899=DIRECTION('ref_axis',(0.488543295503504,-0.0133103699190332,-0.872438125296685));
#87900=DIRECTION('center_axis',(-0.133696428325244,0.987363722375555,-0.0850772871556274));
#87901=DIRECTION('ref_axis',(0.426549576840701,-0.0201567997556429,-0.904239548969536));
#87902=DIRECTION('',(0.928426452468147,0.,-0.37151624777042));
#87903=DIRECTION('center_axis',(0.148209440985322,0.987363721996551,0.056096720830506));
#87904=DIRECTION('ref_axis',(0.293789531228519,0.0102046913623145,-0.955815659850123));
#87905=DIRECTION('',(0.371516244401546,0.,0.928426453816225));
#87906=DIRECTION('center_axis',(-4.33653723296519E-15,-1.,1.41984026416763E-14));
#87907=DIRECTION('ref_axis',(-1.11977916956078E-32,-1.41984026416763E-14,
-1.));
#87908=DIRECTION('center_axis',(0.138986131053651,-0.987363723276318,0.0761297138617028));
#87909=DIRECTION('ref_axis',(0.366355960441036,-0.0201564609952252,-0.930256430953032));
#87910=DIRECTION('center_axis',(-0.154963392508389,-0.987363722477634,-0.0331545851640646));
#87911=DIRECTION('ref_axis',(0.289573017145001,-0.0133103715252556,-0.957063373947306));
#87912=DIRECTION('center_axis',(-0.14885978163699,0.987363722346439,-0.0543474489297465));
#87913=DIRECTION('ref_axis',(0.222192310197494,-0.0201568014481594,-0.974794481234111));
#87914=DIRECTION('',(0.826855347492317,0.,-0.562414646256087));
#87915=DIRECTION('center_axis',(0.156803523203429,0.987363721998679,0.0229245630690647));
#87916=DIRECTION('ref_axis',(0.0814487825518928,0.0102046924843558,-0.996625285687712));
#87917=DIRECTION('',(0.562414644138879,0.,0.82685534893241));
#87918=DIRECTION('center_axis',(1.1829145367693E-15,-1.,-1.47986791925367E-14));
#87919=DIRECTION('ref_axis',(5.07998996178402E-33,1.47986791925367E-14,
-1.));
#87920=DIRECTION('center_axis',(0.152102351271975,-0.987363723473821,0.0444719271614001));
#87921=DIRECTION('ref_axis',(0.157813128528872,-0.0201564541640345,-0.987263254567627));
#87922=DIRECTION('center_axis',(-0.158467690465378,-0.987363722444021,0.000933102381670069));
#87923=DIRECTION('ref_axis',(0.0770626253115131,-0.0133103745061621,-0.996937403105432));
#87924=DIRECTION('center_axis',(-0.157062618092258,0.987363722440241,-0.0210763755649886));
#87925=DIRECTION('ref_axis',(0.00744557762538648,-0.0201567941043528,-0.999769106856808));
#87926=DIRECTION('',(0.686621405562476,0.,-0.727015161756211));
#87927=DIRECTION('center_axis',(0.158065647204977,0.987363722018725,-0.0113195236208035));
#87928=DIRECTION('ref_axis',(-0.13470042036027,0.0102046916006389,-0.990833821094184));
#87929=DIRECTION('',(0.727015160077817,0.,0.686621407339609));
#87930=DIRECTION('center_axis',(4.05203985556794E-15,-1.,2.94139719068973E-14));
#87931=DIRECTION('ref_axis',(4.21776386687562E-32,-2.94139719068973E-14,
-1.));
#87932=DIRECTION('center_axis',(0.158106432646324,-0.987363723454409,0.0107346896601449));
#87933=DIRECTION('ref_axis',(-0.0581088698147696,-0.020156454815659,-0.998106746083862));
#87934=DIRECTION('center_axis',(-0.154562215242167,-0.987363722455789,0.0349771525096206));
#87935=DIRECTION('ref_axis',(-0.139051128634763,-0.0133103707271488,-0.990195747141193));
#87936=DIRECTION('center_axis',(-0.1579213804655,0.987363722325964,0.0131801906847718));
#87937=DIRECTION('ref_axis',(-0.207649299429248,-0.0201568019413548,-0.977995639960649));
#87938=DIRECTION('',(0.514281808963848,0.,-0.857621257297691));
#87939=DIRECTION('center_axis',(0.151936795015725,0.987363722024644,-0.0450343285726719));
#87940=DIRECTION('ref_axis',(-0.344551184645105,0.0102046842600743,-0.93871206745136));
#87941=DIRECTION('',(0.85762125598085,0.,0.514281811159825));
#87942=DIRECTION('center_axis',(2.57010997481761E-15,-1.,6.9638051943949E-15));
#87943=DIRECTION('ref_axis',(-1.02824123169305E-32,-6.9638051943949E-15,
-1.));
#87944=DIRECTION('center_axis',(0.156717633007204,-0.987363723457172,-0.0235044911752826));
#87945=DIRECTION('ref_axis',(-0.271313764309302,-0.0201564546398896,-0.962279875417057));
#87946=DIRECTION('center_axis',(-0.143429583031234,-0.98736372249374,0.067385712245179));
#87947=DIRECTION('ref_axis',(-0.348663004676317,-0.0133103695970175,-0.937153639074871));
#87948=DIRECTION('center_axis',(-0.151395913459791,0.987363722414849,0.0468204767892139));
#87949=DIRECTION('ref_axis',(-0.413034727711651,-0.0201567986262182,-0.910492184026477));
#87950=DIRECTION('',(0.317894965895107,0.,-0.948125936075239));
#87951=DIRECTION('center_axis',(0.138703549433781,0.987363722008433,-0.0766433678547938));
#87952=DIRECTION('ref_axis',(-0.538291114974621,0.0102046874629256,-0.842697181609838));
#87953=DIRECTION('',(0.948125934970735,0.,0.317894969189305));
#87954=DIRECTION('center_axis',(-8.01406900089253E-15,-1.,-1.24969952536102E-14));
#87955=DIRECTION('ref_axis',(5.5988101841633E-32,1.24969952536102E-14,-1.));
#87956=DIRECTION('center_axis',(0.148000890389814,-0.98736372348648,-0.0566446289310448));
#87957=DIRECTION('ref_axis',(-0.471832327136548,-0.0201564532152196,-0.881457867661689));
#87958=DIRECTION('center_axis',(-0.125590341172455,-0.987363722487913,0.096643394595795));
#87959=DIRECTION('ref_axis',(-0.541971788445821,-0.0133103722979742,-0.840291267667425));
#87960=DIRECTION('center_axis',(-0.137791343910941,0.987363722360094,0.0782714846571654));
#87961=DIRECTION('ref_axis',(-0.59910710905729,-0.0201568003086184,-0.800415126842525));
#87962=DIRECTION('',(0.106643708884049,0.,-0.994297299279976));
#87963=DIRECTION('center_axis',(0.118984681183102,0.987363722010516,-0.104668649085082));
#87964=DIRECTION('ref_axis',(-0.706861150377732,0.0102046904694457,-0.707278713364889));
#87965=DIRECTION('',(0.99429729897422,0.,0.106643711734782));
#87966=DIRECTION('center_axis',(3.67961618320588E-14,-1.,3.6687120789681E-14));
#87967=DIRECTION('ref_axis',(1.,3.67961618320588E-14,3.26072068933872E-31));
#87968=DIRECTION('center_axis',(0.132363795311791,-0.987363723319243,-0.0871361208903633));
#87969=DIRECTION('ref_axis',(-0.650288534780861,-0.020156459527977,-0.759419869816335));
#87970=DIRECTION('center_axis',(-0.101878638104898,-0.987363722508935,0.12138213448111));
#87971=DIRECTION('ref_axis',(-0.70993857336524,-0.0133103689258311,-0.704137810465527));
#87972=DIRECTION('center_axis',(-0.117743803763562,0.987363722339622,0.106062606430982));
#87973=DIRECTION('ref_axis',(-0.757165912618984,-0.0201568014598007,-0.652911543873112));
#87974=DIRECTION('',(-0.109594089288496,0.,-0.993976426075098));
#87975=DIRECTION('center_axis',(0.0937022149624435,0.987363721983078,-0.127799747350516));
#87976=DIRECTION('ref_axis',(-0.842379146931304,0.0102046844862637,-0.538788675855223));
#87977=DIRECTION('',(0.993976426077082,0.,-0.109594089270505));
#87978=DIRECTION('center_axis',(-0.0921906923785673,0.987363722375303,0.128894359752262));
#87979=DIRECTION('ref_axis',(-0.879820474071797,-0.0201567989720614,-0.4748785495885));
#87980=DIRECTION('',(-0.32070739268036,0.,-0.947178319156517));
#87981=DIRECTION('center_axis',(1.87810864945458E-14,-1.,1.19654184080002E-14));
#87982=DIRECTION('ref_axis',(1.,1.87810864945458E-14,1.40607568508052E-31));
#87983=DIRECTION('center_axis',(0.1105375112111,-0.987363723357273,-0.113553231628687));
#87984=DIRECTION('ref_axis',(-0.798337974541286,-0.0201564572799021,-0.60187224195442));
#87985=DIRECTION('center_axis',(-0.0734032001647778,-0.987363722506507,
0.140445183910534));
#87986=DIRECTION('ref_axis',(-0.844709418820668,-0.0133103702887437,-0.535059652560746));
#87987=DIRECTION('',(0.947178320273384,0.,-0.320707389381802));
#87988=DIRECTION('center_axis',(0.0640383463728579,0.98736372199852,-0.144955064330502));
#87989=DIRECTION('ref_axis',(-0.938508429326151,0.0102046901058309,-0.345105480083415));
#87990=DIRECTION('center_axis',(2.0914206087111E-14,-1.,7.64829502003661E-15));
#87991=DIRECTION('ref_axis',(1.,2.0914206087111E-14,-8.25113485215167E-32));
#87992=DIRECTION('center_axis',(-0.0623268462666147,0.987363722417612,0.145699155413112));
#87993=DIRECTION('ref_axis',(-0.961335611757529,-0.0201567975226239,-0.274640756408094));
#87994=DIRECTION('center_axis',(0.083542615329035,-0.987363723423162,-0.134660718444295));
#87995=DIRECTION('ref_axis',(-0.909058017628497,-0.0201564551633859,-0.416181736625472));
#87996=DIRECTION('center_axis',(-0.0414955103318477,-0.987363722492924,
0.152941172112732));
#87997=DIRECTION('ref_axis',(-0.939982590838262,-0.0133103712526337,-0.340962700215295));
#87998=DIRECTION('',(-0.516824771977019,0.,-0.856091207215039));
#87999=DIRECTION('center_axis',(0.031380114436834,0.987363721969213,-0.155332446568753));
#88000=DIRECTION('ref_axis',(-0.990754100555664,0.0102046929717233,-0.135285536823009));
#88001=DIRECTION('',(0.856091208538387,0.,-0.516824769784967));
#88002=DIRECTION('center_axis',(0.,-1.,0.));
#88003=DIRECTION('ref_axis',(0.,0.,-1.));
#88004=DIRECTION('center_axis',(0.0526413608956559,-0.987363723435698,-0.149471618597803));
#88005=DIRECTION('ref_axis',(-0.977271517149688,-0.0201564542919456,-0.211031038281868));
#88006=DIRECTION('center_axis',(-0.00764753659104346,-0.987363722466829,
0.158285800817808));
#88007=DIRECTION('ref_axis',(-0.991303222019907,-0.0133103718993134,-0.130922710072981));
#88008=DIRECTION('center_axis',(-0.0295486682057246,0.987363722391953,0.15569121976391));
#88009=DIRECTION('ref_axis',(-0.997899763805172,-0.0201567984337628,-0.0615610662227575));
#88010=DIRECTION('',(-0.688775998780597,0.,-0.724974222647806));
#88011=DIRECTION('center_axis',(-0.00274542668702897,0.98736372204418,-0.158446656712502));
#88012=DIRECTION('ref_axis',(-0.996673211614824,0.0102046860210861,0.0808602104412514));
#88013=DIRECTION('',(0.72497422441144,0.,-0.688775996924277));
#88014=DIRECTION('center_axis',(-4.43853102088631E-14,-1.,3.68048528203422E-15));
#88015=DIRECTION('ref_axis',(1.,-4.43853102088631E-14,1.95112896246476E-32));
#88016=DIRECTION('center_axis',(0.0192786622826518,-0.987363723284348,-0.157293391859486));
#88017=DIRECTION('ref_axis',(-0.999788887210023,-0.0201564613367866,0.00398723936106009));
#88018=DIRECTION('center_axis',(0.0265580251024745,-0.987363722489466,0.156229161216469));
#88019=DIRECTION('ref_axis',(-0.996271616158001,-0.0133103700314487,0.08523908075261));
#88020=DIRECTION('center_axis',(0.00461116960966125,0.987363722328054,0.158403336282166));
#88021=DIRECTION('ref_axis',(-0.987803231645009,-0.0201568018434885,0.154397146641767));
#88022=DIRECTION('',(-0.828520826199668,0.,-0.559958248937739));
#88023=DIRECTION('center_axis',(-0.0367425811626304,0.987363721979082,-0.154152078315933));
#88024=DIRECTION('ref_axis',(-0.955988990855962,0.0102046928250184,0.293225022135811));
#88025=DIRECTION('',(0.559958251059167,0.,-0.828520824765895));
#88026=DIRECTION('center_axis',(2.83709405267036E-14,-1.,-8.75731150790327E-15));
#88027=DIRECTION('ref_axis',(1.,2.83709405267036E-14,7.1912366624173E-32));
#88028=DIRECTION('center_axis',(-0.0149854919521789,-0.98736372325921,-0.157760302429548));
#88029=DIRECTION('ref_axis',(-0.975557240018475,-0.0201564612391877,0.218819077134168));
#88030=DIRECTION('center_axis',(0.0595217627739908,-0.987363722497261,0.146867420664453));
#88031=DIRECTION('ref_axis',(-0.954655456726566,-0.0133103678476456,0.297415186313596));
#88032=DIRECTION('center_axis',(0.0385553986902689,0.987363722351512,0.153708688811013));
#88033=DIRECTION('ref_axis',(-0.931518118380999,-0.0201568010621421,0.363135922897837));
#88034=DIRECTION('',(-0.929524940202268,0.,-0.368759251466278));
#88035=DIRECTION('center_axis',(-0.0690217051008174,0.987363722050075,-0.142649516663741));
#88036=DIRECTION('ref_axis',(-0.870603787481898,0.0102046870362355,0.491878958265819));
#88037=DIRECTION('',(0.368759251362441,0.,-0.929524940243462));
#88038=DIRECTION('center_axis',(-1.29125402862554E-14,-1.,7.32574199636004E-15));
#88039=DIRECTION('ref_axis',(1.,-1.29125402862554E-14,-8.16791645553628E-32));
#88040=DIRECTION('center_axis',(-0.0485489464021499,-0.98736372345918,-0.150850513423275));
#88041=DIRECTION('ref_axis',(-0.905709621322346,-0.0201564548701381,0.423419176669174));
#88042=DIRECTION('center_axis',(0.0897023316329448,-0.987363722499683,0.130638322062027));
#88043=DIRECTION('ref_axis',(-0.868400668737379,-0.0133103683712337,0.495684488995061));
#88044=DIRECTION('center_axis',(0.070696815366875,0.987363722280158,0.141826796558527));
#88045=DIRECTION('ref_axis',(-0.831676253499289,-0.020156805758294,0.554894866210716));
#88046=DIRECTION('',(-0.987065502661801,0.,-0.160317477072854));
#88047=DIRECTION('center_axis',(-0.0980734470899598,0.987363722027219,-0.124476822744034));
#88048=DIRECTION('ref_axis',(-0.744510117580016,0.0102046851999408,0.667533182112291));
#88049=DIRECTION('',(0.160317479600262,0.,-0.987065502251304));
#88050=DIRECTION('center_axis',(5.51791714416026E-15,-1.,-4.96514234470038E-15));
#88051=DIRECTION('ref_axis',(1.,5.51791714416026E-15,-2.12802080022765E-32));
#88052=DIRECTION('center_axis',(-0.0798423016345343,-0.987363723490078,
-0.136887122862264));
#88053=DIRECTION('ref_axis',(-0.793512025280663,-0.020156453595699,0.60822066975188));
#88054=DIRECTION('center_axis',(0.115688518554701,-0.987363722502104,0.10830072096439));
#88055=DIRECTION('ref_axis',(-0.741540431297166,-0.0133103684642173,0.6707761346701));
#88056=DIRECTION('center_axis',(0.0995325357866225,0.987363722369425,0.123313235577846));
#88057=DIRECTION('ref_axis',(-0.692946129975743,-0.0201568006358742,0.720707544250625));
#88058=DIRECTION('',(-0.998451978423991,0.,0.0556205607776269));
#88059=DIRECTION('center_axis',(-0.122539379018189,0.987363722035633,-0.100483734991179));
#88060=DIRECTION('ref_axis',(-0.583603983803612,0.0102046893186796,0.811974294177138));
#88061=DIRECTION('',(-0.0556205582211081,0.,-0.998451978566407));
#88062=DIRECTION('center_axis',(-1.72862098727961E-14,-1.,2.41409965901936E-14));
#88063=DIRECTION('ref_axis',(9.88397516767577E-33,-2.41409965901936E-14,
-1.));
#88064=DIRECTION('center_axis',(-0.107402317354723,-0.987363723483623,-0.116523043967242));
#88065=DIRECTION('ref_axis',(-0.644210689681965,-0.0201564546481271,0.764582438089906));
#88066=DIRECTION('center_axis',(0.136265238378703,-0.987363722512312,0.0808990993536073));
#88067=DIRECTION('ref_axis',(-0.580006587686311,-0.0133103675608265,0.814503033975858));
#88068=DIRECTION('center_axis',(0.123714219117736,0.987363722312337,0.0990336904776107));
#88069=DIRECTION('ref_axis',(-0.521814617623308,-0.0201568038489919,0.852820736200307));
#88070=DIRECTION('',(-0.963151949602078,0.,0.268957844239047));
#88071=DIRECTION('center_axis',(-0.141275510311441,0.987363722055667,-0.0717921343506458));
#88072=DIRECTION('ref_axis',(-0.395409175669361,0.0102046865097965,0.918448391674629));
#88073=DIRECTION('',(-0.268957842517579,0.,-0.963151950082794));
#88074=DIRECTION('center_axis',(-2.92311680908922E-15,-1.,6.8231544174374E-15));
#88075=DIRECTION('ref_axis',(2.66748257699467E-34,-6.8231544174374E-15,
-1.));
#88076=DIRECTION('center_axis',(-0.129940323516781,-0.987363723620263,-0.0907104712978803));
#88077=DIRECTION('ref_axis',(-0.464786779218364,-0.020156448623246,0.885193180860945));
#88078=DIRECTION('center_axis',(0.15047034847597,-0.987363722496393,0.0497147234487595));
#88079=DIRECTION('ref_axis',(-0.391352279647315,-0.0133103692467653,0.920144677366209));
#88080=DIRECTION('center_axis',(0.142111168500603,0.987363722413081,0.0701234301070469));
#88081=DIRECTION('ref_axis',(-0.326283630981388,-0.0201567959017054,0.945056980151238));
#88082=DIRECTION('',(-0.882816006173181,0.,0.469718957723056));
#88083=DIRECTION('center_axis',(-0.153405753362529,0.987363721980081,-0.0397436202794466));
#88084=DIRECTION('ref_axis',(-0.188725472417248,0.0102046916293933,0.981976863439071));
#88085=DIRECTION('',(-0.469718957703103,0.,-0.882816006183797));
#88086=DIRECTION('center_axis',(-5.55199781974273E-15,-1.,2.91680662988243E-14));
#88087=DIRECTION('ref_axis',(2.33192543151121E-32,-2.91680662988243E-14,
-1.));
#88088=DIRECTION('center_axis',(-0.146402458494853,-0.98736372329281,-0.0606563934966637));
#88089=DIRECTION('ref_axis',(-0.263629954398167,-0.0201564602306307,0.964413274615707));
#88090=DIRECTION('center_axis',(0.157639630785437,-0.987363722515614,0.0162057479290574));
#88091=DIRECTION('ref_axis',(-0.184398776981366,-0.013310365432533,0.982761377558067));
#88092=DIRECTION('center_axis',(0.153863152643811,0.987363722405411,0.0379342844434553));
#88093=DIRECTION('ref_axis',(-0.115495988358612,-0.0201567971821641,0.993103408613838));
#88094=DIRECTION('',(-0.761200566737353,0.,0.648516535794372));
#88095=DIRECTION('center_axis',(4.24038427100572E-16,-1.,1.48398242449089E-14));
#88096=DIRECTION('ref_axis',(0.0285626985677906,1.48458813213445E-14,0.999592002894444));
#88097=DIRECTION('center_axis',(-0.156018981952462,-0.987363723488661,-0.027766072987104));
#88098=DIRECTION('ref_axis',(-0.0501460873759626,-0.020156453209744,0.998538475630702));
#88099=DIRECTION('center_axis',(0.157437859804754,-0.987363722525233,-0.0180610005596111));
#88100=DIRECTION('ref_axis',(0.0311770128597521,-0.0133103713432087,0.999425248772438));
#88101=DIRECTION('center_axis',(-0.15836291534669,0.987363722037061,-0.00583673264922174));
#88102=DIRECTION('ref_axis',(0.0267828210981455,0.0102046897763596,0.999589188017054));
#88103=DIRECTION('',(-0.648516533598721,0.,-0.761200568607971));
#88104=DIRECTION('center_axis',(-0.152772347587519,-0.987363722802381,-0.0421128092914994));
#88105=DIRECTION('ref_axis',(-0.157501995156474,-0.0177427248486509,0.98735926452162));
#88106=DIRECTION('',(0.562367402337263,0.,0.826887480125585));
#88107=DIRECTION('',(0.826887478900179,0.,-0.562367404139061));
#88108=DIRECTION('center_axis',(0.154431764554222,-0.987363722245923,0.0355487002483153));
#88109=DIRECTION('ref_axis',(-0.290069428666578,-0.0109157762395627,0.956943348575104));
#88110=DIRECTION('center_axis',(-0.140147600738479,-0.987363722297262,-0.073969790445442));
#88111=DIRECTION('ref_axis',(-0.366072744817863,-0.017742741678619,0.930417078851867));
#88112=DIRECTION('',(0.371463198744195,1.74545579967425E-14,0.928447678643622));
#88113=DIRECTION('center_axis',(-6.93975744812286E-14,-1.,2.27170476996506E-13));
#88114=DIRECTION('ref_axis',(-2.59199074825716E-30,-2.27170476996506E-13,
-1.));
#88115=DIRECTION('center_axis',(0.149682997529586,0.98736372254829,0.0520372909185504));
#88116=DIRECTION('ref_axis',(-0.221888126663152,-0.0177430369618895,0.974910685081093));
#88117=DIRECTION('center_axis',(-0.147323592067659,0.987363722382119,-0.0583835502860794));
#88118=DIRECTION('ref_axis',(-0.294137870802051,0.0126220186732162,0.955679652187201));
#88119=DIRECTION('',(0.928447676446041,0.,-0.371463204236903));
#88120=DIRECTION('center_axis',(0.14317931371119,-0.987363722302444,0.0679158597549498));
#88121=DIRECTION('ref_axis',(-0.489002301735146,-0.0109157720263509,0.872214190906567));
#88122=DIRECTION('center_axis',(-0.120969709374198,-0.987363722292978,-0.102368009229828));
#88123=DIRECTION('ref_axis',(-0.557526335016047,-0.0177427418820099,0.829969626476827));
#88124=DIRECTION('',(0.163189789191805,1.74545580137922E-14,0.986594695254102));
#88125=DIRECTION('center_axis',(1.45762543762546E-14,-1.,-2.58676162557461E-14));
#88126=DIRECTION('ref_axis',(5.47887179583638E-31,2.58676162557461E-14,
-1.));
#88127=DIRECTION('center_axis',(0.134997009526047,0.987363722493814,0.0829981139676269));
#88128=DIRECTION('ref_axis',(-0.426277486400253,-0.0177430437136482,0.904418425834004));
#88129=DIRECTION('center_axis',(-0.131328509014908,0.987363722362473,-0.0886887956984518));
#88130=DIRECTION('ref_axis',(-0.492703966323166,0.0126220221773717,0.87010544540623));
#88131=DIRECTION('',(0.986594694898509,0.,-0.16318979134161));
#88132=DIRECTION('center_axis',(0.125231962048202,-0.987363722236187,0.0971073410894351));
#88133=DIRECTION('ref_axis',(-0.665069967527274,-0.0109157769681648,0.746701268317158));
#88134=DIRECTION('center_axis',(-0.0961354101537728,-0.98736372234748,-0.125979612266014));
#88135=DIRECTION('ref_axis',(-0.72291061702561,-0.0177427394115162,0.690713714204247));
#88136=DIRECTION('',(-0.0527141905833193,1.74545580647872E-14,0.998609640505811));
#88137=DIRECTION('center_axis',(0.,-1.,0.));
#88138=DIRECTION('ref_axis',(0.,0.,-1.));
#88139=DIRECTION('center_axis',(0.113998717626461,0.987363722533795,0.110078025980343));
#88140=DIRECTION('ref_axis',(-0.610734581675629,-0.0177430374931817,0.791636567729163));
#88141=DIRECTION('center_axis',(-0.109192650142314,0.987363722346366,-0.114847050241731));
#88142=DIRECTION('ref_axis',(-0.668231773767008,0.0126220244917432,0.743846073476179));
#88143=DIRECTION('',(0.998609640477331,0.,0.0527141911228425));
#88144=DIRECTION('center_axis',(0.10142890137495,-0.987363722244127,0.121758194640415));
#88145=DIRECTION('ref_axis',(-0.810039701366378,-0.0109157780792778,0.586273424264817));
#88146=DIRECTION('center_axis',(-0.0668059229653221,-0.98736372227003,-0.143700551849403));
#88147=DIRECTION('ref_axis',(-0.854492399176007,-0.0177427420873099,0.519160798648795));
#88148=DIRECTION('',(-0.266153317126965,1.74545580075932E-14,0.963930709015079));
#88149=DIRECTION('center_axis',(-7.22717411294479E-14,-1.,5.20692070645034E-14));
#88150=DIRECTION('ref_axis',(1.,-7.22717411294479E-14,-4.37574147480012E-31));
#88151=DIRECTION('center_axis',(0.0876699694622647,0.987363722548048,0.132010817172483));
#88152=DIRECTION('ref_axis',(-0.766634408653477,-0.0177430370136917,0.641838662053062));
#88153=DIRECTION('center_axis',(-0.0819510665657728,0.987363722349466,-0.135635181560458));
#88154=DIRECTION('ref_axis',(-0.812513804304486,0.0126220234218375,0.582805286814893));
#88155=DIRECTION('',(0.963930709595031,0.,0.266153315026547));
#88156=DIRECTION('center_axis',(0.072883141041351,-0.987363722228438,0.140715769475741));
#88157=DIRECTION('ref_axis',(-0.917132878973961,-0.0109157821110874,0.398432087068595));
#88158=DIRECTION('center_axis',(-0.034352670340833,-0.987363722390964,-0.154702209896024));
#88159=DIRECTION('ref_axis',(-0.946119067924401,-0.0177427377607601,0.323332498469633));
#88160=DIRECTION('',(-0.467147409756163,0.,0.884179448730917));
#88161=DIRECTION('center_axis',(-1.90809286004832E-13,-1.,8.24029964450493E-14));
#88162=DIRECTION('ref_axis',(1.,-1.90809286004832E-13,-8.4845030837726E-31));
#88163=DIRECTION('center_axis',(0.0572418717109346,0.987363722545232,0.147770929227133));
#88164=DIRECTION('ref_axis',(-0.886687261996754,-0.0177430360388344,0.462029094413786));
#88165=DIRECTION('center_axis',(-0.0508775416265985,0.987363722375924,-0.150081163021854));
#88166=DIRECTION('ref_axis',(-0.918803591807643,0.0126220233357556,0.394513173681547));
#88167=DIRECTION('',(0.884179450376195,0.,0.467147406642111));
#88168=DIRECTION('center_axis',(0.0409294380513989,-0.987363722261476,0.153093634951816));
#88169=DIRECTION('ref_axis',(-0.981341943275492,-0.0109157773140059,0.191960506807813));
#88170=DIRECTION('center_axis',(-0.000293123762934843,-0.98736372243561,
-0.15847016658209));
#88171=DIRECTION('ref_axis',(-0.99350625910852,-0.0177427362610183,0.112385534754992));
#88172=DIRECTION('',(-0.646298209424309,0.,0.763084939240012));
#88173=DIRECTION('center_axis',(-5.83035654598321E-14,-1.,1.12737439807136E-14));
#88174=DIRECTION('ref_axis',(1.,-5.83035654598321E-14,1.9003774831539E-31));
#88175=DIRECTION('center_axis',(0.0241372029392072,0.987363722544784,0.156621437985924));
#88176=DIRECTION('ref_axis',(-0.96527960424997,-0.017743040055254,0.260615560066199));
#88177=DIRECTION('center_axis',(-0.0174250414748936,0.987363722392953,-0.157509516004368));
#88178=DIRECTION('ref_axis',(-0.982131145014957,0.0126220211409558,0.187774062569692));
#88179=DIRECTION('',(0.763084941849124,0.,0.646298206343728));
#88180=DIRECTION('center_axis',(0.0070619211713651,-0.987363722269307,0.158313010254586));
#88181=DIRECTION('ref_axis',(-0.999664548667799,-0.0109157740318901,-0.0234869328370264));
#88182=DIRECTION('center_axis',(0.0337801346917581,-0.987363722339333,-0.154828234855351));
#88183=DIRECTION('ref_axis',(-0.994438202640106,-0.0177427401627641,-0.103816454868353));
#88184=DIRECTION('',(-0.795228820662645,0.,0.606309428252191));
#88185=DIRECTION('center_axis',(-1.48409955798332E-13,-1.,-3.80843256108542E-15));
#88186=DIRECTION('ref_axis',(-0.999670904433375,1.48458812936906E-13,-0.0256531251382206));
#88187=DIRECTION('center_axis',(-0.0100960892824427,0.987363722538594,0.158148501086578));
#88188=DIRECTION('ref_axis',(-0.998736545245237,-0.0177430383254438,0.0470159311573217));
#88189=DIRECTION('center_axis',(0.0168422419368752,0.987363722326255,-0.157572899702271));
#88190=DIRECTION('ref_axis',(-0.999535337432634,0.0126220267804277,-0.0277451556741776));
#88191=DIRECTION('',(0.606309431371119,0.,0.795228818284669));
#88192=DIRECTION('center_axis',(-0.0271357980096675,-0.987363722266527,
0.156129844739459));
#88193=DIRECTION('ref_axis',(-0.971243950925299,-0.0109157760761481,-0.237836148689955));
#88194=DIRECTION('center_axis',(0.0662738680381684,-0.987363722346358,-0.143946706143641));
#88195=DIRECTION('ref_axis',(-0.948871320917237,-0.017742740453389,-0.315164102495797));
#88196=DIRECTION('',(-0.906975416896829,0.,0.421183562291816));
#88197=DIRECTION('center_axis',(-5.76486051496427E-14,-1.,-1.4249258802016E-14));
#88198=DIRECTION('ref_axis',(1.,-5.76486051496427E-14,-7.94905549468724E-31));
#88199=DIRECTION('center_axis',(-0.0438573035860945,0.987363722504216,0.152280715800702));
#88200=DIRECTION('ref_axis',(-0.98549367499417,-0.0177430405640933,-0.168782111190805));
#88201=DIRECTION('center_axis',(0.0503219900885229,0.987363722369066,-0.150268350170727));
#88202=DIRECTION('ref_axis',(-0.970202368722082,0.0126220214997916,-0.241967039696155));
#88203=DIRECTION('',(0.421183564268127,0.,0.906975415979064));
#88204=DIRECTION('center_axis',(-0.0600646816443866,-0.98736372228547,0.146646220317949));
#88205=DIRECTION('ref_axis',(-0.897409065200425,-0.0109157738880786,-0.441064412049447));
#88206=DIRECTION('center_axis',(0.0956687123460396,-0.987363722218188,-0.126334387739427));
#88207=DIRECTION('ref_axis',(-0.858936270142699,-0.017742744429567,-0.511775027578971));
#88208=DIRECTION('',(-0.976312851284768,0.,0.216363620824314));
#88209=DIRECTION('center_axis',(-5.32376433741381E-14,-1.,-2.63088650808751E-14));
#88210=DIRECTION('ref_axis',(1.,-5.32376433741381E-14,-1.03806303605968E-30));
#88211=DIRECTION('center_axis',(-0.0755677974580308,0.987363722503259,0.139292453032636));
#88212=DIRECTION('ref_axis',(-0.926170215653369,-0.0177430413683588,-0.376688088635137));
#88213=DIRECTION('center_axis',(0.0814487424077611,0.987363722364132,-0.13593741986458));
#88214=DIRECTION('ref_axis',(-0.895503815254515,0.0126220203453105,-0.444874815500957));
#88215=DIRECTION('',(0.216363620211501,0.,0.976312851420575));
#88216=DIRECTION('center_axis',(-0.0901850061830041,-0.987363722271896,
0.130305581619351));
#88217=DIRECTION('ref_axis',(-0.781612328340454,-0.0109157730780283,-0.623668994005893));
#88218=DIRECTION('center_axis',(0.120590189003312,-0.987363722259253,-0.102814815481514));
#88219=DIRECTION('ref_axis',(-0.728838316062047,-0.0177427435776927,-0.684455918295822));
#88220=DIRECTION('',(-0.999998982187443,0.,0.0014267529843288));
#88221=DIRECTION('center_axis',(2.31686742770819E-14,-1.,1.85691490357775E-14));
#88222=DIRECTION('ref_axis',(1.,2.31686742770819E-14,-7.24715462217508E-31));
#88223=DIRECTION('center_axis',(-0.103744820256812,0.987363722562306,0.119791033211119));
#88224=DIRECTION('ref_axis',(-0.823540068225522,-0.0177430367518507,-0.5669805469978));
#88225=DIRECTION('center_axis',(0.108767043471548,0.98736372236086,-0.11525020616105));
#88226=DIRECTION('ref_axis',(-0.778932498628811,0.0126220208625128,-0.626980739073556));
#88227=DIRECTION('',(0.00142675803820793,0.,0.999998982180232));
#88228=DIRECTION('center_axis',(-0.116088374672241,-0.987363722232209,0.107872004179562));
#88229=DIRECTION('ref_axis',(-0.629268269566731,-0.0109157796553593,-0.777111504657477));
#88230=DIRECTION('center_axis',(0.139873000841585,-0.987363722359222,-0.0744877399610901));
#88231=DIRECTION('ref_axis',(-0.564660688619854,-0.0177427383955641,-0.825132414804786));
#88232=DIRECTION('',(-0.976926272040803,0.,-0.213576822236072));
#88233=DIRECTION('center_axis',(3.72703708254283E-14,-1.,4.62311855372118E-14));
#88234=DIRECTION('ref_axis',(-1.04756410853878E-30,-4.62311855372118E-14,
-1.));
#88235=DIRECTION('center_axis',(-0.127070855555912,0.987363722556134,0.0946883152684742));
#88236=DIRECTION('ref_axis',(-0.682402100079866,-0.0177430371157247,-0.730761629014892));
#88237=DIRECTION('center_axis',(0.130999521498712,0.987363722324349,-0.0891740164224692));
#88238=DIRECTION('ref_axis',(-0.625939163365759,0.0126220266765779,-0.779769740505201));
#88239=DIRECTION('',(-0.213576822851012,0.,0.976926271906364));
#88240=DIRECTION('center_axis',(-0.13656358601598,-0.987363722260568,0.0803944459413213));
#88241=DIRECTION('ref_axis',(-0.447500324708907,-0.0109157777619702,-0.894217146548462));
#88242=DIRECTION('center_axis',(0.15261550972507,-0.987363722385411,-0.0426776980234713));
#88243=DIRECTION('ref_axis',(-0.374080159221782,-0.0177427380813195,-0.927226633419243));
#88244=DIRECTION('',(-0.908173574914686,0.,-0.418593786177817));
#88245=DIRECTION('center_axis',(-3.96910079242655E-14,-1.,-7.97435311668676E-14));
#88246=DIRECTION('ref_axis',(-2.13334119177811E-30,7.97435311668676E-14,
-1.));
#88247=DIRECTION('center_axis',(-0.144455199096664,0.987363722535034,0.065158076058957));
#88248=DIRECTION('ref_axis',(-0.509355770290959,-0.0177430388022161,-0.860373107346671));
#88249=DIRECTION('center_axis',(0.147106601607187,0.987363722352517,-0.0589281557981135));
#88250=DIRECTION('ref_axis',(-0.443677609396436,0.0126220232229998,-0.896097574737272));
#88251=DIRECTION('',(-0.418593784198901,0.,0.908173575826804));
#88252=DIRECTION('center_axis',(-0.15065323545887,-0.987363722271498,0.0491577317209224));
#88253=DIRECTION('ref_axis',(-0.244807760987597,-0.0109157752669287,-0.969510188709));
#88254=DIRECTION('center_axis',(0.158221887782401,-0.987363722345595,-0.00887209233635914));
#88255=DIRECTION('ref_axis',(-0.166008055151417,-0.0177427396082325,-0.98596476651858));
#88256=DIRECTION('',(-0.796955690039799,0.,-0.604037770435913));
#88257=DIRECTION('center_axis',(-2.16205522115258E-14,-1.,-8.64115651514208E-14));
#88258=DIRECTION('ref_axis',(4.82917687363763E-31,8.64115651514208E-14,
-1.));
#88259=DIRECTION('center_axis',(-0.155084977231928,0.987363722540378,0.0325811179700883));
#88260=DIRECTION('ref_axis',(-0.312492527935681,-0.0177430392379542,-0.949754496984862));
#88261=DIRECTION('center_axis',(0.156335143187237,0.987363722338763,-0.0259268743578526));
#88262=DIRECTION('ref_axis',(-0.24067018291622,0.0126220262462275,-0.970524882477782));
#88263=DIRECTION('',(-0.604037768699346,0.,0.796955691355997));
#88264=DIRECTION('',(-0.648473045044079,0.,-0.761237617207177));
#88265=DIRECTION('',(-0.761237617213291,0.,0.648473045036901));
#88266=DIRECTION('center_axis',(-0.157369969703018,-0.987363722263388,-0.0186432988995479));
#88267=DIRECTION('ref_axis',(0.184905254470325,-0.0109157789351342,-0.98269572739455));
#88268=DIRECTION('center_axis',(0.147323590960846,-0.987363722315772,0.0583835542010283));
#88269=DIRECTION('ref_axis',(0.263331029590432,-0.0177427404521949,-0.964542359886848));
#88270=DIRECTION('',(-0.469668516573739,0.,-0.882842842492039));
#88271=DIRECTION('center_axis',(2.77683211871253E-14,-1.,-1.45838744591726E-13));
#88272=DIRECTION('ref_axis',(-1.75617357726029E-31,1.45838744591726E-13,
-1.));
#88273=DIRECTION('center_axis',(-0.154431769535767,0.987363722528783,-0.0355486707508934));
#88274=DIRECTION('ref_axis',(0.115181024600642,-0.0177430401713234,-0.993186043044013));
#88275=DIRECTION('center_axis',(0.152772346306646,0.987363722381786,0.0421128237992417));
#88276=DIRECTION('ref_axis',(0.189086477475989,0.0126220211157706,-0.981879314691309));
#88277=DIRECTION('',(-0.882842840276596,0.,0.46966852073814));
#88278=DIRECTION('center_axis',(-0.149682990353858,-0.98736372222389,-0.0520373177144283));
#88279=DIRECTION('ref_axis',(0.39183280570531,-0.0109157821600972,-0.919971683299512));
#88280=DIRECTION('center_axis',(0.131328508972608,-0.987363722350935,0.0886887958895417));
#88281=DIRECTION('ref_axis',(0.464522591751889,-0.017742740090601,-0.885383508388419));
#88282=DIRECTION('',(-0.268902815661671,0.,-0.963167314504196));
#88283=DIRECTION('center_axis',(-1.16940264748932E-14,-1.,2.72919495009907E-14));
#88284=DIRECTION('ref_axis',(1.20821244774943E-32,-2.72919495009907E-14,
-1.));
#88285=DIRECTION('center_axis',(-0.143179326462339,0.987363722500805,-0.0679158299893592));
#88286=DIRECTION('ref_axis',(0.325993798533084,-0.0177430420158487,-0.945205389202788));
#88287=DIRECTION('center_axis',(0.140147601725461,0.987363722386407,0.0739697873855303));
#88288=DIRECTION('ref_axis',(0.395740769282578,0.0126220205100963,-0.918275518635816));
#88289=DIRECTION('',(-0.963167313918257,0.,0.268902817760414));
#88290=DIRECTION('center_axis',(-0.134996993412494,-0.987363722305443,-0.0829981424173244));
#88291=DIRECTION('ref_axis',(0.58043869111259,-0.0109157701802117,-0.814230785355649));
#88292=DIRECTION('center_axis',(0.10919265044991,-0.987363722260612,0.114847050686525));
#88293=DIRECTION('ref_axis',(0.643993593304886,-0.0177427429237519,-0.764825108672436));
#88294=DIRECTION('',(-0.0555635134513151,0.,-0.998455154712992));
#88295=DIRECTION('center_axis',(8.64379451953179E-14,-1.,-1.2070004440453E-13));
#88296=DIRECTION('ref_axis',(3.17309577792907E-30,1.2070004440453E-13,-1.));
#88297=DIRECTION('center_axis',(-0.125231977120001,0.987363722511643,-0.0971073188517023));
#88298=DIRECTION('ref_axis',(0.52156346317154,-0.0177430425746461,-0.853027982146368));
#88299=DIRECTION('center_axis',(0.120969709501029,0.987363722336303,0.102368008662062));
#88300=DIRECTION('ref_axis',(0.5838906615892,0.012622023301845,-0.811734180527526));
#88301=DIRECTION('',(-0.99845515443243,0.,0.0555635184929094));
#88302=DIRECTION('center_axis',(-0.113998700166117,-0.987363722223595,-0.11007804684497));
#88303=DIRECTION('ref_axis',(0.741903905967849,-0.0109157819403093,-0.670417362554313));
#88304=DIRECTION('center_axis',(0.0819510669257577,-0.987363722306909,0.135635181652755));
#88305=DIRECTION('ref_axis',(0.793352172628083,-0.0177427411803675,-0.608504334677828));
#88306=DIRECTION('',(0.160373871797992,0.,-0.987056341474245));
#88307=DIRECTION('center_axis',(8.82912126861344E-14,-1.,-7.94372331205514E-14));
#88308=DIRECTION('ref_axis',(1.,8.82912126861344E-14,4.09990452814717E-30));
#88309=DIRECTION('center_axis',(-0.101428922427798,0.987363722514867,-0.121758174907153));
#88310=DIRECTION('ref_axis',(0.692745400016714,-0.017743039406182,-0.720963934818042));
#88311=DIRECTION('center_axis',(0.0961354074716145,0.98736372232858,0.125979614460904));
#88312=DIRECTION('ref_axis',(0.744738477174182,0.0126220251617332,-0.6672370531506));
#88313=DIRECTION('',(-0.987056341368623,0.,-0.160373872448067));
#88314=DIRECTION('center_axis',(-0.0876699454717902,-0.987363722241175,
-0.132010835400075));
#88315=DIRECTION('ref_axis',(0.868678520543038,-0.0109157792923925,-0.495255967868736));
#88316=DIRECTION('center_axis',(0.0508775419888311,-0.987363722325599,0.150081163230142));
#88317=DIRECTION('ref_axis',(0.905614485029377,-0.0177427407083583,-0.423730574371417));
#88318=DIRECTION('',(0.36881235729421,0.,-0.929503870409956));
#88319=DIRECTION('center_axis',(-1.2912958762935E-13,-1.,7.32500423227334E-14));
#88320=DIRECTION('ref_axis',(1.,-1.2912958762935E-13,-3.62494059594665E-30));
#88321=DIRECTION('center_axis',(-0.0728831642249594,0.987363722545768,-0.140715755241269));
#88322=DIRECTION('ref_axis',(0.831535330186537,-0.0177430374288357,-0.555188417813597));
#88323=DIRECTION('center_axis',(0.0668059227393821,0.987363722362798,0.143700551317036));
#88324=DIRECTION('ref_axis',(0.870763148538878,0.0126220240826978,-0.491540663276922));
#88325=DIRECTION('',(-0.929503871604648,0.,-0.368812354283272));
#88326=DIRECTION('center_axis',(-0.0572418399771415,-0.987363722286597,
-0.147770943247942));
#88327=DIRECTION('ref_axis',(0.954834693482862,-0.010915775899325,-0.296936952833434));
#88328=DIRECTION('center_axis',(0.017425041224431,-0.987363722356895,0.157509516258108));
#88329=DIRECTION('ref_axis',(0.975531269058269,-0.0177427395283381,-0.219143647600366));
#88330=DIRECTION('',(0.560005585107136,0.,-0.828488831939704));
#88331=DIRECTION('center_axis',(-1.13485762705073E-13,-1.,3.50227621756936E-14));
#88332=DIRECTION('ref_axis',(1.,-1.13485762705073E-13,1.22045136905081E-30));
#88333=DIRECTION('center_axis',(-0.0409294637811914,0.987363722509901,-0.153093626470785));
#88334=DIRECTION('ref_axis',(0.931443595764125,-0.0177430419875243,-0.363452902548632));
#88335=DIRECTION('center_axis',(0.0343526699419355,0.987363722367053,0.154702210137208));
#88336=DIRECTION('ref_axis',(0.956071902701323,0.0126220207023251,-0.292860378778798));
#88337=DIRECTION('',(-0.828488832258417,0.,-0.560005584635622));
#88338=DIRECTION('center_axis',(-0.0241371697553315,-0.987363722282063,
-0.156621444756176));
#88339=DIRECTION('ref_axis',(0.996343856436258,-0.0109157726890224,-0.0847334977935284));
#88340=DIRECTION('center_axis',(-0.0168422380496672,-0.987363722328066,
0.157572900106406));
#88341=DIRECTION('ref_axis',(0.999833296486313,-0.0177427405920249,-0.0043098020368813));
#88342=DIRECTION('',(0.725013574350737,0.,-0.688734576602023));
#88343=DIRECTION('center_axis',(-1.77542081017899E-13,-1.,1.47117976467656E-14));
#88344=DIRECTION('ref_axis',(1.,-1.77542081017899E-13,3.24326134236472E-31));
#88345=DIRECTION('center_axis',(-0.00706195171111479,0.987363722497818,
-0.158313007467113));
#88346=DIRECTION('ref_axis',(0.987798592454597,-0.0177430417900404,-0.154722736573373));
#88347=DIRECTION('center_axis',(0.000293118801652807,0.987363722357134,
0.158470167080217));
#88348=DIRECTION('ref_axis',(0.996675797480111,0.0126220232240424,-0.0804862674443004));
#88349=DIRECTION('',(-0.68873457818185,0.,-0.725013572849964));
#88350=DIRECTION('center_axis',(0.0100961238614255,-0.9873637222979,-0.158148500381796));
#88351=DIRECTION('ref_axis',(0.991265088020046,-0.0109157736626055,0.131432002031304));
#88352=DIRECTION('center_axis',(-0.0503219922735293,-0.987363722301029,
0.150268349886061));
#88353=DIRECTION('ref_axis',(0.977384229993961,-0.0177427415408041,0.210725561054484));
#88354=DIRECTION('',(0.856120735019485,0.,-0.51677585766916));
#88355=DIRECTION('center_axis',(-5.88512824280692E-14,-1.,-7.93281843200647E-15));
#88356=DIRECTION('ref_axis',(1.,-5.88512824280692E-14,1.0842198170146E-31));
#88357=DIRECTION('center_axis',(0.0271357676639449,0.987363722543269,-0.156129848263511));
#88358=DIRECTION('ref_axis',(0.997965225106375,-0.0177430396859387,0.0612420935393733));
#88359=DIRECTION('center_axis',(-0.033780134470556,0.987363722380125,0.154828234643471));
#88360=DIRECTION('ref_axis',(0.990676239571682,0.0126220219592833,0.135651291589024));
#88361=DIRECTION('',(-0.516775860806531,0.,-0.85612073312569));
#88362=DIRECTION('center_axis',(0.0438573361251434,-0.987363722295469,-0.152280707782841));
#88363=DIRECTION('ref_axis',(0.939835865763662,-0.0109157723346735,0.341451887296887));
#88364=DIRECTION('center_axis',(-0.0814487486910026,-0.98736372219626,0.135937417319212));
#88365=DIRECTION('ref_axis',(0.909233762600149,-0.0177427448865258,0.41590763391872));
#88366=DIRECTION('',(0.947196641515208,0.,-0.32065327427349));
#88367=DIRECTION('center_axis',(-5.5770050700255E-14,-1.,-2.03986396420233E-14));
#88368=DIRECTION('ref_axis',(1.,-5.5770050700255E-14,-5.63063762659705E-31));
#88369=DIRECTION('center_axis',(0.0600646471800081,0.987363722582821,-0.146646232432119));
#88370=DIRECTION('ref_axis',(0.961468112966299,-0.0177430359170283,0.274343311246094));
#88371=DIRECTION('center_axis',(-0.0662738702393048,0.987363722336531,0.143946705197631));
#88372=DIRECTION('ref_axis',(0.938353761907754,0.0126220250365005,0.345445946564067));
#88373=DIRECTION('',(-0.32065327633744,0.,-0.947196640816502));
#88374=DIRECTION('center_axis',(0.0755678252582836,-0.987363722276059,-0.139292439561156));
#88375=DIRECTION('ref_axis',(0.844460963137086,-0.0109157740894685,0.535505861418541));
#88376=DIRECTION('center_axis',(-0.108767043096074,-0.987363722378186,0.115250206366968));
#88377=DIRECTION('ref_axis',(0.79856853679574,-0.0177427385073159,0.601642325032217));
#88378=DIRECTION('',(0.993982686191135,0.,-0.109537297539496));
#88379=DIRECTION('center_axis',(-5.00810733926824E-14,-1.,-3.1910643155052E-14));
#88380=DIRECTION('ref_axis',(1.,-5.00810733926824E-14,-1.71968141652445E-31));
#88381=DIRECTION('center_axis',(0.0901849763727487,0.987363722522623,-0.130305600351315));
#88382=DIRECTION('ref_axis',(0.88001382101897,-0.0177430385210899,0.474616539323728));
#88383=DIRECTION('center_axis',(-0.095668707141692,0.98736372237429,0.126334390460485));
#88384=DIRECTION('ref_axis',(0.842154904786648,0.0126220207242787,0.539087934326699));
#88385=DIRECTION('',(-0.109537302858737,0.,-0.993982685604952));
#88386=DIRECTION('center_axis',(0.103744844987445,-0.987363722267051,-0.119791014226798));
#88387=DIRECTION('ref_axis',(0.709600004588852,-0.0109157788340079,0.704520176616645));
#88388=DIRECTION('center_axis',(-0.130999520459926,-0.987363722265585,0.0891740185991351));
#88389=DIRECTION('ref_axis',(0.650563131571766,-0.0177427423106625,0.759244892597134));
#88390=DIRECTION('',(0.994291204618493,1.7454558011431E-14,0.106700517422864));
#88391=DIRECTION('center_axis',(4.20503607033623E-14,-1.,4.19305404221689E-14));
#88392=DIRECTION('ref_axis',(1.,4.20503607033623E-14,1.91185012013183E-30));
#88393=DIRECTION('center_axis',(0.116088354229398,0.987363722546353,-0.107872023304093));
#88394=DIRECTION('ref_axis',(0.757411060199225,-0.017743038907888,0.652697227248744));
#88395=DIRECTION('center_axis',(-0.120590188318903,0.987363722333388,0.102814815572313));
#88396=DIRECTION('ref_axis',(0.706577820236583,0.0126220248222844,0.70752276884854));
#88397=DIRECTION('',(0.106700515256271,0.,-0.994291204850996));
#88398=DIRECTION('center_axis',(0.12707087651531,-0.9873637222525,-0.0946882903072925));
#88399=DIRECTION('ref_axis',(0.541558938450353,-0.0109157767576206,0.840591911692174));
#88400=DIRECTION('center_axis',(-0.147106602631027,-0.98736372225952,0.0589281548004195));
#88401=DIRECTION('ref_axis',(0.472138117688431,-0.0177427424578752,0.881346012026887));
#88402=DIRECTION('',(0.948107771776315,0.,0.317949136022339));
#88403=DIRECTION('center_axis',(-4.80801298667729E-14,-1.,-7.49847183820041E-14));
#88404=DIRECTION('ref_axis',(2.14746148769039E-30,7.49847183820041E-14,
-1.));
#88405=DIRECTION('center_axis',(0.136563571728994,0.987363722495015,-0.0803944673308284));
#88406=DIRECTION('ref_axis',(0.599392599870526,-0.0177430430396784,0.800258518007864));
#88407=DIRECTION('center_axis',(-0.139873001359505,0.987363722361872,0.0744877389534123));
#88408=DIRECTION('ref_axis',(0.537961943656821,0.012622022091116,0.842874623971624));
#88409=DIRECTION('',(0.317949136540617,0.,-0.948107771602509));
#88410=DIRECTION('center_axis',(0.144455213172839,-0.987363722247192,-0.0651580492138836));
#88411=DIRECTION('ref_axis',(0.348195179853326,-0.0109157773107122,0.937358502672597));
#88412=DIRECTION('center_axis',(-0.15633514206494,-0.98736372237218,0.0259268798525389));
#88413=DIRECTION('ref_axis',(0.271636452700257,-0.0177427388279761,0.962236370536524));
#88414=DIRECTION('',(0.857591872604232,1.74545580696915E-14,0.514330807985645));
#88415=DIRECTION('center_axis',(0.,-1.,0.));
#88416=DIRECTION('ref_axis',(0.,0.,-1.));
#88417=DIRECTION('center_axis',(0.150653225068599,0.987363722493285,-0.0491577591091539));
#88418=DIRECTION('ref_axis',(0.413347208971823,-0.0177430422692839,0.910400609229934));
#88419=DIRECTION('center_axis',(-0.15261550883066,0.987363722410109,0.0426777006504942));
#88420=DIRECTION('ref_axis',(0.344191563648143,0.0126220174954829,0.938814599475205));
#88421=DIRECTION('',(0.514330808231272,0.,-0.85759187245692));
#88422=DIRECTION('center_axis',(0.155084985394089,-0.987363722264602,-0.0325810874757932));
#88423=DIRECTION('ref_axis',(0.138550198822444,-0.0109157754770187,0.990295253069506));
#88424=DIRECTION('center_axis',(-0.158253626581311,-0.98736372226607,-0.00828671386947175));
#88425=DIRECTION('ref_axis',(0.0584333675298601,-0.0177427423121442,0.998133626652446));
#88426=DIRECTION('',(0.726975930476597,0.,0.686662942430772));
#88427=DIRECTION('center_axis',(2.4302156024229E-14,-1.,1.76485219614137E-13));
#88428=DIRECTION('ref_axis',(1.46250166471626E-31,-1.76485219614137E-13,
-1.));
#88429=DIRECTION('center_axis',(0.157698501290677,0.987363722511173,-0.0156224889039468));
#88430=DIRECTION('ref_axis',(0.207974160398467,-0.0177430411066726,0.97797338056761));
#88431=DIRECTION('center_axis',(-0.158221887463882,0.987363722382384,0.00887209392241986));
#88432=DIRECTION('ref_axis',(0.13432716864759,0.0126220202709485,0.990856647738411));
#88433=DIRECTION('center_axis',(-1.18376001797387E-14,-1.,1.47986115205468E-13));
#88434=DIRECTION('ref_axis',(5.1637282516317E-31,-1.47986115205468E-13,
-1.));
#88435=DIRECTION('center_axis',(0.158463155145865,-0.987363722292628,0.00151932934686073));
#88436=DIRECTION('ref_axis',(-0.0775732331348036,-0.0109157737333195,0.996926897713577));
#88437=DIRECTION('center_axis',(0.157369971174573,0.987363722509919,0.018643273421546));
#88438=DIRECTION('ref_axis',(-0.00712352888697095,-0.0177430419567505,0.999817203191822));
#88439=DIRECTION('center_axis',(-0.156429985687579,0.987363722414907,-0.0253483576738535));
#88440=DIRECTION('ref_axis',(-0.0818182158823528,0.0126220183822201,0.996567340525359));
#88441=DIRECTION('',(0.686662939327361,0.,-0.726975933407915));
#88442=DIRECTION('center_axis',(0.162023728744164,-0.986495108954454,-0.0239939853458685));
#88443=DIRECTION('ref_axis',(0.0324773729665821,-0.0189711050413171,0.99929240836639));
#88444=DIRECTION('center_axis',(0.153077706971466,-0.986495108938772,-0.058263330390891));
#88445=DIRECTION('ref_axis',(0.246536396631873,-0.018971104116629,0.968947832622772));
#88446=DIRECTION('center_axis',(0.13697394371636,-0.986495108875294,-0.0898083454246302));
#88447=DIRECTION('ref_axis',(0.44906765042969,-0.0189711014311051,0.893296335293081));
#88448=DIRECTION('center_axis',(0.114465436194755,-0.986495109078521,-0.117154016921752));
#88449=DIRECTION('ref_axis',(0.630601004724684,-0.0189710906652105,0.775875293174871));
#88450=DIRECTION('center_axis',(0.0866046342375456,-0.986495108953145,-0.139021715354488));
#88451=DIRECTION('ref_axis',(0.782648160233291,-0.0189711058178337,0.622175179854913));
#88452=DIRECTION('center_axis',(0.0546943161535251,-0.986495108922816,-0.154388898084867));
#88453=DIRECTION('ref_axis',(0.898099551017545,-0.0189710967552618,0.439382855776128));
#88454=DIRECTION('center_axis',(0.0202265331475369,-0.986495108893428,-0.162537034198902));
#88455=DIRECTION('ref_axis',(0.971556809872428,-0.0189711067873972,0.236045466590173));
#88456=DIRECTION('center_axis',(-0.0151870056510711,-0.986495108979521,
-0.163085115258372));
#88457=DIRECTION('ref_axis',(0.999585149477771,-0.0189711027994199,0.0216708606676361));
#88458=DIRECTION('center_axis',(-0.0498904087762942,-0.986495109002119,
-0.156007522341176));
#88459=DIRECTION('ref_axis',(0.980873999808598,-0.018971090818931,-0.1937170467786));
#88460=DIRECTION('center_axis',(-0.0822610132790794,-0.986495109022473,
-0.141635184784849));
#88461=DIRECTION('ref_axis',(0.916298269164019,-0.018971100014056,-0.400046971356214));
#88462=DIRECTION('center_axis',(-0.110785172696402,-0.986495108908185,-0.120640149249146));
#88463=DIRECTION('ref_axis',(0.808877454441714,-0.0189710978365288,-0.587671133494551));
#88464=DIRECTION('center_axis',(-0.134129138216128,-0.986495109061941,-0.0940041173474185));
#88465=DIRECTION('ref_axis',(0.663634428213268,-0.0189710911115877,-0.747816450335298));
#88466=DIRECTION('center_axis',(-0.151201382438819,-0.986495108951864,-0.062972549278554));
#88467=DIRECTION('ref_axis',(0.487360592554928,-0.018971096011209,-0.872994702355428));
#88468=DIRECTION('center_axis',(-0.16120361374351,-0.986495109028429,-0.0289964614913726));
#88469=DIRECTION('ref_axis',(0.288298316451173,-0.0189710924938625,-0.957352692784122));
#88470=DIRECTION('center_axis',(-0.163668145749564,-0.986495108828605,0.00633548136598124));
#88471=DIRECTION('ref_axis',(0.0757555315809696,-0.0189711024502777,-0.996945934695912));
#88472=DIRECTION('center_axis',(-0.158479734362203,-0.986495108855783,0.0413711735403188));
#88473=DIRECTION('ref_axis',(-0.140329497611904,-0.0189711012108083,-0.98992309267884));
#88474=DIRECTION('center_axis',(-0.145880991273112,-0.986495109095868,0.0744723849161958));
#88475=DIRECTION('ref_axis',(-0.349852873668116,-0.01897108864457,-0.936612547738819));
#88476=DIRECTION('center_axis',(-0.126461011979806,-0.986495109024855,0.104091365247475));
#88477=DIRECTION('ref_axis',(-0.543017521318959,-0.0189710911169627,-0.839507039423998));
#88478=DIRECTION('center_axis',(-0.101127849063559,-0.986495108878455,0.128843153883565));
#88479=DIRECTION('ref_axis',(-0.710791271527493,-0.0189711022124235,-0.703147115190823));
#88480=DIRECTION('center_axis',(-0.0710660688100426,-0.986495108919276,
0.147570369458886));
#88481=DIRECTION('ref_axis',(-0.845329211087288,-0.0189710997746033,-0.533908814551591));
#88482=DIRECTION('center_axis',(-0.0376813248201236,-0.986495109040278,
0.159397357567215));
#88483=DIRECTION('ref_axis',(-0.940340495999881,-0.0189710911884959,-0.339705533192815));
#88484=DIRECTION('center_axis',(-0.00253463197808244,-0.986495108968311,
0.163771107410113));
#88485=DIRECTION('ref_axis',(-0.991382506037285,-0.0189710951273427,-0.129617993630908));
#88486=DIRECTION('center_axis',(0.0327305710932476,-0.986495108991966,0.160487101197692));
#88487=DIRECTION('ref_axis',(-0.996068571300047,-0.0189710930823987,0.0865303351174733));
#88488=DIRECTION('center_axis',(0.0664653398970494,-0.986495109036314,0.149698892580411));
#88489=DIRECTION('ref_axis',(-0.954179575331009,-0.0189711015572081,0.298632609282444));
#88490=DIRECTION('center_axis',(0.0970922492532798,-0.986495108967022,0.131910936313417));
#88491=DIRECTION('ref_axis',(-0.86767420750609,-0.018971096596724,0.496771141596003));
#88492=DIRECTION('center_axis',(0.123179242181962,-0.986495108881639,0.107954964907041));
#88493=DIRECTION('ref_axis',(-0.740597354552622,-0.0189711014686376,0.67168121585967));
#88494=DIRECTION('center_axis',(0.143506499163671,-0.986495109075195,0.0789511524203817));
#88495=DIRECTION('ref_axis',(-0.578890995779445,-0.018971089074444,0.815184220151993));
#88496=DIRECTION('center_axis',(0.157123563074936,-0.986495109019346,0.0462556570329008));
#88497=DIRECTION('ref_axis',(-0.390116332765927,-0.0189710950778334,0.920570119252636));
#88498=DIRECTION('center_axis',(0.163393702153687,-0.986495108818127,0.0113972968033836));
#88499=DIRECTION('ref_axis',(-0.183100264679772,-0.0189711023189716,0.982911181313449));
#88500=DIRECTION('center_axis',(-0.160735574475915,0.986495108729145,-0.03148770476503));
#88501=DIRECTION('ref_axis',(-0.0827414017722213,0.0183223861287446,0.996402604673089));
#88502=DIRECTION('center_axis',(0.156388933187229,0.986495109513922,0.0486816236548836));
#88503=DIRECTION('ref_axis',(-0.189986493512465,-0.0183223028001626,0.981615721911043));
#88504=DIRECTION('center_axis',(-0.150208708155227,0.986495107965014,-0.0653050224365125));
#88505=DIRECTION('ref_axis',(-0.295004101909852,0.0183224712765873,0.955320295452096));
#88506=DIRECTION('center_axis',(0.142267533730559,0.986495109449251,0.0811624782700377));
#88507=DIRECTION('ref_axis',(-0.39656307898551,-0.018322309651865,0.917824611434316));
#88508=DIRECTION('center_axis',(-0.132658262707296,0.986495107927723,-0.0960686596666776));
#88509=DIRECTION('ref_axis',(-0.493472694787282,0.0183224713738039,0.869568275952));
#88510=DIRECTION('center_axis',(0.121493864981184,0.986495109445291,0.109848258122087));
#88511=DIRECTION('ref_axis',(-0.584596816960018,-0.0183223081336044,0.811117041261539));
#88512=DIRECTION('center_axis',(-0.108904868035384,0.986495107974999,-0.122340229113693));
#88513=DIRECTION('ref_axis',(-0.668867050422418,0.0183224663674009,0.743156212438158));
#88514=DIRECTION('center_axis',(0.0950392813517184,0.986495109507679,0.133397653343611));
#88515=DIRECTION('ref_axis',(-0.745295455580775,-0.0183223031322053,0.666482540730495));
#88516=DIRECTION('center_axis',(-0.0800591980640834,0.986495108016897,-0.142891310666767));
#88517=DIRECTION('ref_axis',(-0.812985930735701,0.0183224676300055,0.581994985893997));
#88518=DIRECTION('center_axis',(0.0641407625183083,0.98649510951366,0.150709526869412));
#88519=DIRECTION('ref_axis',(-0.871144905238391,-0.0183223048337039,0.490684060493894));
#88520=DIRECTION('center_axis',(-0.0474700514394284,0.986495108004734,-0.156760952086502));
#88521=DIRECTION('ref_axis',(-0.919090489904261,0.0183224666752224,0.393620322877872));
#88522=DIRECTION('center_axis',(0.030243094789543,0.986495109526178,0.160974389573263));
#88523=DIRECTION('ref_axis',(-0.956260590131882,-0.0183223037027041,0.291941735535794));
#88524=DIRECTION('center_axis',(-0.0126612612175189,0.98649510803266,-0.16330062551017));
#88525=DIRECTION('ref_axis',(-0.982219398720206,0.0183224629032323,0.186840413537536));
#88526=DIRECTION('center_axis',(-0.00506870820519181,0.986495109499761,
0.163712269333076));
#88527=DIRECTION('ref_axis',(-0.996662592361594,-0.0183223045077197,0.0795485395503481));
#88528=DIRECTION('center_axis',(0.0227395578527785,0.986495108067057,-0.162204544536908));
#88529=DIRECTION('ref_axis',(-0.99942082101588,0.0183224615593546,-0.0286759467559414));
#88530=DIRECTION('center_axis',(-0.0401435017313524,0.986495109510236,0.158795145332385));
#88531=DIRECTION('ref_axis',(-0.99046175944326,-0.0183223030114974,-0.13656425701082));
#88532=DIRECTION('center_axis',(0.05707710669577,0.986495108026889,-0.153523958163722));
#88533=DIRECTION('ref_axis',(-0.969890436299754,0.0183224663519494,-0.242851454187645));
#88534=DIRECTION('center_axis',(-0.0733412334055878,0.986495109495549,0.146452935866481));
#88535=DIRECTION('ref_axis',(-0.937948035034169,-0.0183223051985068,-0.346291462077474));
#88536=DIRECTION('center_axis',(0.0887457784509185,0.986495108087939,-0.137664768643635));
#88537=DIRECTION('ref_axis',(-0.895009054991074,0.01832245519328,-0.445671492379392));
#88538=DIRECTION('center_axis',(-0.103109611601752,0.986495109457591,0.127262747933526));
#88539=DIRECTION('ref_axis',(-0.841576901967371,-0.0183223090775577,-0.539826463842844));
#88540=DIRECTION('center_axis',(0.116264815017321,0.986495107985349,-0.115368516979126));
#88541=DIRECTION('ref_axis',(-0.77827804080034,0.018322464811729,-0.627652434466088));
#88542=DIRECTION('center_axis',(-0.12805669118874,0.9864951095139,0.102121901406854));
#88543=DIRECTION('ref_axis',(-0.705854571165698,-0.0183223035697561,-0.708119776278269));
#88544=DIRECTION('center_axis',(0.138347433593088,0.986495107922349,-0.0876777603698864));
#88545=DIRECTION('ref_axis',(-0.625155611021741,0.0183224723337327,-0.780285043439648));
#88546=DIRECTION('center_axis',(-0.147015987202331,0.986495109509443,0.072205944498196));
#88547=DIRECTION('ref_axis',(-0.537127260541591,-0.0183223033714437,-0.843302199203969));
#88548=DIRECTION('center_axis',(0.153961071525636,0.986495108040822,-0.0558872996861048));
#88549=DIRECTION('ref_axis',(-0.442801601435135,0.0183224663569708,-0.896432389526995));
#88550=DIRECTION('center_axis',(-0.159100978613269,0.986495109517672,0.038913718686559));
#88551=DIRECTION('ref_axis',(-0.343284481816298,-0.0183223033521734,-0.939052744921172));
#88552=DIRECTION('center_axis',(0.162375666691975,0.986495107908977,-0.0214835969519158));
#88553=DIRECTION('ref_axis',(-0.239742676781274,0.0183224754522504,-0.970663554391042));
#88554=DIRECTION('center_axis',(-0.163746585579862,0.986495109490697,0.00380192870451849));
#88555=DIRECTION('ref_axis',(-0.133390098075001,-0.0183223046117274,-0.990894229920256));
#88556=DIRECTION('center_axis',(0.163197752322382,0.986495107979212,0.0139246389541917));
#88557=DIRECTION('ref_axis',(-0.0254736615879604,0.0183224693088499,-0.999507568597521));
#88558=DIRECTION('center_axis',(-0.16073558406174,0.986495109510974,-0.0314876313377507));
#88559=DIRECTION('ref_axis',(0.0827414566412087,-0.018322302109249,-0.996402601661752));
#88560=DIRECTION('center_axis',(0.156388895407881,0.986495108044351,0.0486817747998856));
#88561=DIRECTION('ref_axis',(0.189986480495769,0.0183224625414125,-0.981615721448699));
#88562=DIRECTION('center_axis',(-0.150208763039716,0.986495109468233,-0.0653048734884087));
#88563=DIRECTION('ref_axis',(0.295004112724699,-0.0183223089330748,-0.955320295226096));
#88564=DIRECTION('center_axis',(0.142267467124047,0.986495108042642,0.0811626121194061));
#88565=DIRECTION('ref_axis',(0.396563065841762,0.0183224630960468,-0.917824614050133));
#88566=DIRECTION('center_axis',(-0.132658350585122,0.986495109509682,-0.096068522074175));
#88567=DIRECTION('ref_axis',(0.493472703917656,-0.0183223047110463,-0.869568274282286));
#88568=DIRECTION('center_axis',(0.121493764696758,0.986495107991744,0.109848382091712));
#88569=DIRECTION('ref_axis',(0.584596805976639,0.0183224713431901,-0.81111704549084));
#88570=DIRECTION('center_axis',(-0.108904979399665,0.98649510950515,-0.122340117640862));
#88571=DIRECTION('ref_axis',(0.668867060361115,-0.0183223051419811,-0.743156207467962));
#88572=DIRECTION('center_axis',(0.0950391544766888,0.986495107995122,0.133397754921323));
#88573=DIRECTION('ref_axis',(0.745295445944788,0.0183224694080519,-0.66648254693484));
#88574=DIRECTION('center_axis',(-0.080059332910558,0.986495109481381,-0.142891225004316));
#88575=DIRECTION('ref_axis',(0.812985939220982,-0.0183223042755116,-0.581994979183681));
#88576=DIRECTION('center_axis',(0.0641406167314776,0.98649510794872,0.150709599158611));
#88577=DIRECTION('ref_axis',(0.871144897914193,0.0183224710739945,-0.490684067289547));
#88578=DIRECTION('center_axis',(-0.0474702014876177,0.986495109526955,-0.15676089706979));
#88579=DIRECTION('ref_axis',(0.919090496426534,-0.0183223033730333,-0.393620315250032));
#88580=DIRECTION('center_axis',(0.0302429388491882,0.986495108017902,0.160974428113639));
#88581=DIRECTION('ref_axis',(0.956260584933476,0.0183224675571459,-0.291941742279695));
#88582=DIRECTION('center_axis',(-0.0126614162704048,0.986495109510479,-0.163300604560837));
#88583=DIRECTION('ref_axis',(0.982219403911675,-0.0183223025459124,-0.186840401971333));
#88584=DIRECTION('center_axis',(-0.00506887179982308,0.986495107936615,
0.163712273687112));
#88585=DIRECTION('ref_axis',(0.996662588632331,0.018322471519566,-0.0795485478064573));
#88586=DIRECTION('center_axis',(0.0227394049424628,0.986495109493483,-0.162204557298197));
#88587=DIRECTION('ref_axis',(0.999420823519324,-0.0183223041105813,0.0286759601066141));
#88588=DIRECTION('center_axis',(-0.0401436445413463,0.986495108156152,0.158795117641948));
#88589=DIRECTION('ref_axis',(0.990461758653599,0.0183224525292182,0.136564242677704));
#88590=DIRECTION('center_axis',(0.0570769529460997,0.9864951095419,-0.153524005589694));
#88591=DIRECTION('ref_axis',(0.969890437076523,-0.0183223020859195,0.242851463478775));
#88592=DIRECTION('center_axis',(-0.0733413793153341,0.986495108018749,0.14645287274479));
#88593=DIRECTION('ref_axis',(0.937948035288988,0.0183224675093107,0.34629145279937));
#88594=DIRECTION('center_axis',(0.0887456490514789,0.986495109536923,-0.137664841677775));
#88595=DIRECTION('ref_axis',(0.895009051824839,-0.018322302725518,0.445671505006139));
#88596=DIRECTION('center_axis',(-0.103109737085043,0.986495108050338,0.12726265717407));
#88597=DIRECTION('ref_axis',(0.841576906157068,0.0183224677937832,0.539826451924174));
#88598=DIRECTION('center_axis',(0.116264699940127,0.986495109476491,-0.115368620199771));
#88599=DIRECTION('ref_axis',(0.778278035980726,-0.0183223065149454,0.627652445063314));
#88600=DIRECTION('center_axis',(-0.128056799605045,0.986495107974527,0.102121780327414));
#88601=DIRECTION('ref_axis',(0.705854575921104,0.0183224696374283,0.708119767241124));
#88602=DIRECTION('center_axis',(0.138347337245002,0.986495109509675,-0.0876778945385417));
#88603=DIRECTION('ref_axis',(0.625155606942879,-0.0183223039101845,0.78028505066245));
#88604=DIRECTION('center_axis',(-0.147016064077881,0.986495108038024,0.0722058080772992));
#88605=DIRECTION('ref_axis',(0.537127269546356,0.0183224638920168,0.843302189980912));
#88606=DIRECTION('center_axis',(0.153961009504263,0.98649510950004,-0.0558874447880148));
#88607=DIRECTION('ref_axis',(0.4428015927046,-0.0183223048421035,0.896432397140768));
#88608=DIRECTION('center_axis',(-0.159101026864052,0.986495107934884,0.0389135615351019));
#88609=DIRECTION('ref_axis',(0.34328448898429,0.0183224711543863,0.939052739026724));
#88610=DIRECTION('center_axis',(0.162375635431742,0.986495109483945,-0.0214837608997327));
#88611=DIRECTION('ref_axis',(0.239742670287193,-0.0183223053354739,0.970663559206155));
#88612=DIRECTION('center_axis',(-0.16374659742247,0.986495108103312,0.00380177863617757));
#88613=DIRECTION('ref_axis',(0.133390110991654,0.0183224591380823,0.99089422532416));
#88614=DIRECTION('center_axis',(0.163197756721024,0.986495109467979,0.0139244819288294));
#88615=DIRECTION('ref_axis',(0.0254736527193002,-0.0183223088757047,0.999507571764516));
#88616=DIRECTION('center_axis',(-0.155915195591883,0.987363722014138,0.0283431161648219));
#88617=DIRECTION('ref_axis',(0.137699079904333,-0.00668761038376333,0.99045153301959));
#88618=DIRECTION('',(-0.727555834386232,0.,-0.686048473397146));
#88619=DIRECTION('center_axis',(5.09401252609433E-15,-1.,3.67634634867259E-14));
#88620=DIRECTION('ref_axis',(-6.45625538871542E-32,-3.67634634867259E-14,
-1.));
#88621=DIRECTION('center_axis',(-0.152615513946062,-0.987363722125795,0.0426776889355044));
#88622=DIRECTION('ref_axis',(0.0672126608260175,0.032713973952949,0.997202213261128));
#88623=DIRECTION('center_axis',(0.149874467494489,-0.987363722004544,-0.0514832444837739));
#88624=DIRECTION('ref_axis',(0.141986603508105,-0.0300375739723024,0.989412729134859));
#88625=DIRECTION('',(-0.513606044697416,0.,0.858026124806393));
#88626=DIRECTION('center_axis',(-0.14617705138698,0.987363722010122,0.0611976315401775));
#88627=DIRECTION('ref_axis',(0.347397555335768,-0.00668761392715165,0.937694094236864));
#88628=DIRECTION('',(-0.858026123626375,0.,-0.513606046668745));
#88629=DIRECTION('center_axis',(-5.15119010035186E-15,-1.,-1.39235567883145E-14));
#88630=DIRECTION('ref_axis',(-6.20982939421556E-32,1.39235567883145E-14,
-1.));
#88631=DIRECTION('center_axis',(-0.139873004476777,-0.987363722032271,0.0744877374688009));
#88632=DIRECTION('ref_axis',(0.280010267064326,0.0327139789846414,0.959439443590661));
#88633=DIRECTION('center_axis',(0.135303109889243,-0.987363721994079,-0.082498175399821));
#88634=DIRECTION('ref_axis',(0.351361525093086,-0.0300375743814345,0.935757886854041));
#88635=DIRECTION('',(-0.317147963824608,0.,0.948376069416508));
#88636=DIRECTION('center_axis',(-0.129603829678582,0.987363721969541,0.0911906128452898));
#88637=DIRECTION('ref_axis',(0.540852105342674,-0.00668761734633794,0.841091122245756));
#88638=DIRECTION('',(-0.948376068001928,0.,-0.317147968054664));
#88639=DIRECTION('center_axis',(-4.01195563274949E-15,-1.,-6.24533907804427E-15));
#88640=DIRECTION('ref_axis',(1.34225804296661E-33,6.24533907804427E-15,
-1.));
#88641=DIRECTION('center_axis',(-0.120590190541021,-0.987363722095157,0.102814815253828));
#88642=DIRECTION('ref_axis',(0.479714901796952,0.0327139771544658,0.876814352467315));
#88643=DIRECTION('center_axis',(0.11440513091871,-0.987363722064315,-0.109655580664077));
#88644=DIRECTION('ref_axis',(0.544307172996746,-0.0300375714644054,0.838348045697496));
#88645=DIRECTION('',(-0.105860401342829,0.,0.994381001139671));
#88646=DIRECTION('center_axis',(-0.106970483025467,0.987363722064335,0.116919613891604));
#88647=DIRECTION('ref_axis',(0.709017011728858,-0.00668761002897997,0.705159664864051));
#88648=DIRECTION('',(-0.994381001052798,0.,-0.105860402158854));
#88649=DIRECTION('center_axis',(-2.10428865491674E-14,-1.,-2.0947498637656E-14));
#88650=DIRECTION('ref_axis',(1.,-2.10428865491674E-14,1.06656828981155E-31));
#88651=DIRECTION('center_axis',(-0.0956687124477457,-0.987363722032615,
0.126334389112749));
#88652=DIRECTION('ref_axis',(0.656988601142513,0.0327139780022003,0.753190396654177));
#88653=DIRECTION('center_axis',(0.0881576982976218,-0.987363722201013,-0.131685611637061));
#88654=DIRECTION('ref_axis',(0.711801621142929,-0.0300375659622816,0.701737982988921));
#88655=DIRECTION('',(0.110377077686696,0.,0.993889782984685));
#88656=DIRECTION('center_axis',(-0.0793353121724068,0.987363722060234,0.1371815898795));
#88657=DIRECTION('ref_axis',(0.844029071912828,-0.00668760940451682,0.536255724115299));
#88658=DIRECTION('',(-0.993889783075357,0.,0.110377076870243));
#88659=DIRECTION('center_axis',(-2.50540085574457E-14,-1.,-1.59341591747121E-14));
#88660=DIRECTION('ref_axis',(1.,-2.50540085574457E-14,2.03091541231879E-31));
#88661=DIRECTION('center_axis',(-0.0662738725216956,-0.987363722042481,
0.143946706163761));
#88662=DIRECTION('ref_axis',(0.803542242785219,0.0327139775453649,0.594348096432437));
#88663=DIRECTION('center_axis',(0.0577880969639443,-0.987363721938116,-0.147558179881013));
#88664=DIRECTION('ref_axis',(0.84601301874443,-0.0300375766578798,0.532315429142777));
#88665=DIRECTION('',(0.321453447978035,0.,0.946925382901437));
#88666=DIRECTION('center_axis',(-0.0479905089208821,0.987363722033518,0.151029108007807));
#88667=DIRECTION('ref_axis',(0.939575270352825,-0.00668761048465775,0.342277062052691));
#88668=DIRECTION('',(-0.946925383165727,0.,0.321453447199499));
#88669=DIRECTION('center_axis',(-1.39468164794721E-14,-1.,-5.08787806647015E-15));
#88670=DIRECTION('ref_axis',(1.,-1.39468164794721E-14,-5.70074136491531E-32));
#88671=DIRECTION('center_axis',(-0.0337801382797952,-0.987363722000072,
0.154828236236041));
#88672=DIRECTION('ref_axis',(0.912523143460641,0.0327139788577966,0.407714738801532));
#88673=DIRECTION('center_axis',(0.0247164010991849,-0.987363722070208,-0.156531082716402));
#88674=DIRECTION('ref_axis',(0.940665786847186,-0.0300375716952866,0.338002399017841));
#88675=DIRECTION('',(0.517499010316405,0.,0.855683805106501));
#88676=DIRECTION('center_axis',(-0.0144017231991955,0.987363722024748,0.157814672316391));
#88677=DIRECTION('ref_axis',(0.991187973412547,-0.0066876108997449,0.132293904707591));
#88678=DIRECTION('',(-0.855683805531977,0.,0.517499009612883));
#88679=DIRECTION('center_axis',(-2.20717365751389E-14,-1.,-2.95615954106558E-15));
#88680=DIRECTION('ref_axis',(1.,-2.20717365751389E-14,-3.49902049063999E-32));
#88681=DIRECTION('center_axis',(0.00029311340816282,-0.987363722109961,
0.158470168630232));
#88682=DIRECTION('ref_axis',(0.978835476575937,0.0327139753810231,0.202017092373709));
#88683=DIRECTION('center_axis',(-0.0095110066128146,-0.987363722136431,
-0.158184768426366));
#88684=DIRECTION('ref_axis',(0.991334067966758,-0.0300375680597071,0.127884753561701));
#88685=DIRECTION('',(0.689346896451424,0.,0.724431402102911));
#88686=DIRECTION('center_axis',(0.0198604748347696,0.98736372197993,0.157220997507575));
#88687=DIRECTION('ref_axis',(0.996453828388622,-0.00668761527781448,-0.0838751673116389));
#88688=DIRECTION('',(-0.724431404105314,0.,0.689346894347108));
#88689=DIRECTION('center_axis',(7.3970661933122E-15,-1.,-6.19241585272321E-16));
#88690=DIRECTION('ref_axis',(1.,7.3970661933122E-15,-2.73744258678365E-33));
#88691=DIRECTION('center_axis',(0.0343526630103307,-0.987363722117046,0.154702213272049));
#88692=DIRECTION('ref_axis',(0.999378550340755,0.0327139758686177,-0.0131266485318631));
#88693=DIRECTION('center_axis',(-0.0432936985350912,-0.987363722000109,
-0.152441910724197));
#88694=DIRECTION('ref_axis',(0.995648669933615,-0.030037572720232,-0.088212642430092));
#88695=DIRECTION('',(0.828961684948636,0.,0.559305395009845));
#88696=DIRECTION('center_axis',(0.0531940151561749,0.987363721983716,0.149275842861553));
#88697=DIRECTION('ref_axis',(0.955126609739221,-0.00668761530697499,-0.296122331426671));
#88698=DIRECTION('',(-0.559305393715893,0.,0.828961685821673));
#88699=DIRECTION('center_axis',(-2.12730247814828E-14,-1.,6.58474391108148E-15));
#88700=DIRECTION('ref_axis',(1.,-2.12730247814828E-14,-4.11537089026276E-32));
#88701=DIRECTION('center_axis',(0.066805920029825,-0.987363722085958,0.143700554478858));
#88702=DIRECTION('ref_axis',(0.973191793942822,0.0327139762673729,-0.22765660095664));
#88703=DIRECTION('center_axis',(-0.0750520182188506,-0.987363722081671,
-0.139571038823626));
#88704=DIRECTION('ref_axis',(0.95340784703351,-0.0300375703472505,-0.300185312069997));
#88705=DIRECTION('',(0.929815148606726,0.,0.368026886818684));
#88706=DIRECTION('center_axis',(0.0840402591504759,0.987363722035372,0.134350717342248));
#88707=DIRECTION('ref_axis',(0.869138731961614,-0.00668761158347473,-0.494523144509402));
#88708=DIRECTION('',(-0.368026888566917,0.,0.929815147914764));
#88709=DIRECTION('center_axis',(6.45338266227362E-15,-1.,-3.66795591991993E-15));
#88710=DIRECTION('ref_axis',(1.,6.45338266227362E-15,2.19847859555268E-32));
#88711=DIRECTION('center_axis',(0.0961354053430143,-0.987363722113789,0.125979617768667));
#88712=DIRECTION('ref_axis',(0.901499670081164,0.0327139749884623,-0.431541586274148));
#88713=DIRECTION('center_axis',(-0.103300989414795,-0.987363722147405,-0.120173981265271));
#88714=DIRECTION('ref_axis',(0.86658673311804,-0.0300375681323686,-0.498121650286851));
#88715=DIRECTION('',(0.987191489212963,0.,0.15953984964733));
#88716=DIRECTION('center_axis',(0.110956879962712,0.98736372196159,0.113143498898947));
#88717=DIRECTION('ref_axis',(0.742510893754301,-0.00668761482372817,-0.669800603511342));
#88718=DIRECTION('',(-0.159539850458518,0.,0.987191489081867));
#88719=DIRECTION('center_axis',(1.65420121889355E-14,-1.,-1.49084629836801E-14));
#88720=DIRECTION('ref_axis',(1.,1.65420121889355E-14,6.43307823203382E-32));
#88721=DIRECTION('center_axis',(0.120969707670699,-0.987363722086591,0.102368013233525));
#88722=DIRECTION('ref_axis',(0.787654424115901,0.0327139760771574,-0.615248164515646));
#88723=DIRECTION('center_axis',(-0.126719727503591,-0.987363722008549,-0.0951577170955746));
#88724=DIRECTION('ref_axis',(0.739244985382749,-0.0300375738261793,-0.672766375308023));
#88725=DIRECTION('',(0.998407852567291,0.,-0.0564070911496949));
#88726=DIRECTION('center_axis',(0.132685278204196,0.98736372199092,0.0866458160796747));
#88727=DIRECTION('ref_axis',(0.58116407064798,-0.00668761625283787,-0.813758931611029));
#88728=DIRECTION('',(0.0564070903287917,0.,0.99840785261367));
#88729=DIRECTION('center_axis',(-3.02175773341056E-14,-1.,4.22705617652681E-14));
#88730=DIRECTION('ref_axis',(-3.42385489395757E-32,-4.22705617652681E-14,
-1.));
#88731=DIRECTION('center_axis',(0.140147600521612,-0.987363722064494,0.0739697939633669));
#88732=DIRECTION('ref_axis',(0.636979333125905,0.0327139770656922,-0.770186422157014));
#88733=DIRECTION('center_axis',(-0.144213188971448,-0.987363721901816,-0.0656919842817939));
#88734=DIRECTION('ref_axis',(0.577336963336558,-0.0300375769362138,-0.815953292007038));
#88735=DIRECTION('',(0.962939774722175,0.,-0.269716499788217));
#88736=DIRECTION('center_axis',(0.148209458094694,0.987363721996652,0.0560966756251662));
#88737=DIRECTION('ref_axis',(0.392642662313079,-0.00668761280541487,-0.919666795946587));
#88738=DIRECTION('',(0.269716499743162,0.,0.962939774734794));
#88739=DIRECTION('center_axis',(2.91774084025479E-15,-1.,-6.82545505654051E-15));
#88740=DIRECTION('ref_axis',(-6.44641099708178E-33,6.82545505654051E-15,
-1.));
#88741=DIRECTION('center_axis',(0.152772347138366,-0.987363722035567,0.042112828899362));
#88742=DIRECTION('ref_axis',(0.456519795472252,0.0327139780841959,-0.889111619528099));
#88743=DIRECTION('center_axis',(-0.154963396046347,-0.987363722152358,-0.0331545783146796));
#88744=DIRECTION('ref_axis',(0.388433310595543,-0.0300375678177878,-0.92098713766229));
#88745=DIRECTION('',(0.882445701968546,0.,-0.470414267510287));
#88746=DIRECTION('center_axis',(0.156803530198347,0.987363722024449,0.022924514114007));
#88747=DIRECTION('ref_axis',(0.18576171983432,-0.00668761285105647,-0.982572063147813));
#88748=DIRECTION('',(0.470414265591377,0.,0.882445702991479));
#88749=DIRECTION('center_axis',(2.76450920575637E-15,-1.,-1.45862154872855E-14));
#88750=DIRECTION('ref_axis',(3.9736416322651E-32,1.45862154872855E-14,-1.));
#88751=DIRECTION('center_axis',(0.158253627833745,-0.987363722044687,0.00828671632925747));
#88752=DIRECTION('ref_axis',(0.254713900192221,0.0327139774057854,-0.966462945348222));
#88753=DIRECTION('center_axis',(-0.158467693352313,-0.987363721969011,0.000933114730172718));
#88754=DIRECTION('ref_axis',(0.181366942943162,-0.0300375755843955,-0.982956650143059));
#88755=DIRECTION('',(0.760689450324145,0.,-0.649115983600427));
#88756=DIRECTION('',(0.649115982975009,0.,0.760689450857831));
#88757=DIRECTION('',(0.603364203507011,0.,-0.797465759720347));
#88758=DIRECTION('center_axis',(0.15193678307463,0.987363721986491,-0.0450343696959965));
#88759=DIRECTION('ref_axis',(-0.243978531110299,-0.00668761449916178,-0.969757573917096));
#88760=DIRECTION('',(0.797465757841021,0.,0.603364205990914));
#88761=DIRECTION('center_axis',(3.61559231045529E-15,-1.,1.43988779150332E-14));
#88762=DIRECTION('ref_axis',(2.43352655744764E-33,-1.43988779150332E-14,
-1.));
#88763=DIRECTION('center_axis',(0.147106605238035,-0.987363722139964,-0.0589281502955677));
#88764=DIRECTION('ref_axis',(-0.174635182534135,0.0327139741043342,-0.984089604111115));
#88765=DIRECTION('center_axis',(-0.14342958100638,-0.98736372219215,0.0673857209740856));
#88766=DIRECTION('ref_axis',(-0.248128604798918,-0.0300375668343596,-0.968261297408511));
#88767=DIRECTION('',(0.417826320448815,0.,-0.908526920867073));
#88768=DIRECTION('center_axis',(0.138703528025338,0.9873637219984,-0.0766434067274603));
#88769=DIRECTION('ref_axis',(-0.446743660603705,-0.0066876128263548,-0.894637008817032));
#88770=DIRECTION('',(0.908526921025422,0.,0.417826320104499));
#88771=DIRECTION('center_axis',(-3.31319745013849E-15,-1.,-6.64249734523797E-15));
#88772=DIRECTION('ref_axis',(-2.41067561919743E-32,6.64249734523797E-15,
-1.));
#88773=DIRECTION('center_axis',(0.130999522255125,-0.987363722009175,-0.0891740188009809));
#88774=DIRECTION('ref_axis',(-0.382102486511712,0.032713978423544,-0.923540732949701));
#88775=DIRECTION('center_axis',(-0.125590338476149,-0.987363722138999,0.0966434016644088));
#88776=DIRECTION('ref_axis',(-0.450475053156877,-0.0300375682025106,-0.8922835709458));
#88777=DIRECTION('',(0.212751341222145,0.,-0.977106374356538));
#88778=DIRECTION('center_axis',(0.118984649782232,0.987363722013483,-0.104668684752799));
#88779=DIRECTION('ref_axis',(-0.628619553791156,-0.00668761262270496,-0.777684211250824));
#88780=DIRECTION('',(0.97710637405149,0.,0.212751342623141));
#88781=DIRECTION('center_axis',(0.,-1.,0.));
#88782=DIRECTION('ref_axis',(0.,0.,-1.));
#88783=DIRECTION('center_axis',(0.108767048291564,-0.987363722066022,-0.115250204138089));
#88784=DIRECTION('ref_axis',(-0.571703099871005,0.0327139779658703,-0.819808124650843));
#88785=DIRECTION('center_axis',(-0.101878629407447,-0.987363722040434,0.121382145592017));
#88786=DIRECTION('ref_axis',(-0.631757788857494,-0.0300375715922423,-0.774583656237808));
#88787=DIRECTION('',(-0.00227165580984505,0.,-0.999997419786612));
#88788=DIRECTION('center_axis',(0.0937021788006043,0.9873637219845,-0.127799773853223));
#88789=DIRECTION('ref_axis',(-0.781101895149244,-0.00668761622474827,-0.624367764369277));
#88790=DIRECTION('',(0.99999741978848,0.,-0.00227165498764559));
#88791=DIRECTION('',(-0.217188431596517,0.,-0.976129696905409));
#88792=DIRECTION('center_axis',(4.0572621615691E-14,-1.,3.24617426702296E-14));
#88793=DIRECTION('ref_axis',(1.,4.0572621615691E-14,-2.92296430474148E-31));
#88794=DIRECTION('center_axis',(0.0814487487035971,-0.987363722049272,-0.135937418379291));
#88795=DIRECTION('ref_axis',(-0.734571511907989,0.032713977419385,-0.677742199936388));
#88796=DIRECTION('center_axis',(-0.0734031935085418,-0.987363722173652,
0.140445189729441));
#88797=DIRECTION('ref_axis',(-0.783500232034526,-0.0300375676236387,-0.620665071462136));
#88798=DIRECTION('',(0.97612969721957,0.,-0.217188430184553));
#88799=DIRECTION('center_axis',(0.0640383051982778,0.987363722029317,-0.144955082310855));
#88800=DIRECTION('ref_axis',(-0.897060779917043,-0.00668761072181317,-0.441856575143406));
#88801=DIRECTION('center_axis',(1.33149632604712E-14,-1.,6.56596881425884E-15));
#88802=DIRECTION('ref_axis',(1.,1.33149632604712E-14,8.86106816052588E-32));
#88803=DIRECTION('center_axis',(0.0503219999089623,-0.987363722182468,-0.150268348108123));
#88804=DIRECTION('ref_axis',(-0.863092177279706,0.0327139724496799,-0.503985802900377));
#88805=DIRECTION('center_axis',(-0.0414955038933948,-0.987363722188286,
0.152941175826287));
#88806=DIRECTION('ref_axis',(-0.898607075736631,-0.0300375670188769,-0.437724877067374));
#88807=DIRECTION('',(-0.42194971744984,0.,-0.906619234267617));
#88808=DIRECTION('center_axis',(0.0313800657302326,0.987363722003927,-0.155332456187748));
#88809=DIRECTION('ref_axis',(-0.971074099998923,-0.00668761233512322,-0.238684662583368));
#88810=DIRECTION('',(0.906619235714275,0.,-0.421949714341488));
#88811=DIRECTION('center_axis',(7.20757801078152E-15,-1.,1.77506829913838E-15));
#88812=DIRECTION('ref_axis',(1.,7.20757801078152E-15,-1.50447430979086E-32));
#88813=DIRECTION('center_axis',(0.0168422433773957,-0.987363722095952,-0.157572900991399));
#88814=DIRECTION('ref_axis',(-0.951255611113478,0.0327139760516595,-0.306663591083151));
#88815=DIRECTION('center_axis',(-0.00764752809376302,-0.987363722126041,
0.158285803354138));
#88816=DIRECTION('ref_axis',(-0.97169605093596,-0.0300375693087569,-0.234317154782747));
#88817=DIRECTION('',(-0.606981102892634,0.,-0.794716264292635));
#88818=DIRECTION('center_axis',(-0.00274546710291745,0.98736372205532,-0.158446655942785));
#88819=DIRECTION('ref_axis',(-0.999681074168654,-0.00668761021136266,-0.0243521214407966));
#88820=DIRECTION('',(0.794716264791645,0.,-0.606981102239283));
#88821=DIRECTION('center_axis',(5.9365248500426E-14,-1.,1.4732157731511E-15));
#88822=DIRECTION('ref_axis',(-0.999692221970019,-5.9383525444618E-14,-0.0248084931554796));
#88823=DIRECTION('center_axis',(-0.0174250350984094,-0.987363722096869,
-0.157509518565821));
#88824=DIRECTION('ref_axis',(-0.99493939068009,0.0327139763908477,-0.0950021295647155));
#88825=DIRECTION('center_axis',(0.0265580391453566,-0.98736372202936,0.15622916173712));
#88826=DIRECTION('ref_axis',(-0.999349599106874,-0.0300375724690615,-0.0199530199492971));
#88827=DIRECTION('',(-0.763630725504658,0.,-0.645653246770455));
#88828=DIRECTION('center_axis',(-0.0367426341140373,0.987363721963562,-0.154152065794214));
#88829=DIRECTION('ref_axis',(-0.981544072352426,-0.00668761746811693,0.191119098476359));
#88830=DIRECTION('',(0.645653245721824,0.,-0.76363072639128));
#88831=DIRECTION('center_axis',(2.18602574241031E-14,-1.,-4.24612529797942E-15));
#88832=DIRECTION('ref_axis',(1.,2.18602574241031E-14,1.16412908801297E-32));
#88833=DIRECTION('center_axis',(-0.0508775382972576,-0.987363722076295,
-0.150081166121724));
#88834=DIRECTION('ref_axis',(-0.992100910024825,0.0327139764061875,0.121101527965626));
#88835=DIRECTION('center_axis',(0.0595217788630251,-0.987363722020241,0.14686741735088));
#88836=DIRECTION('ref_axis',(-0.980274670496925,-0.0300375728765124,0.1953440928153));
#88837=DIRECTION('',(-0.884573827309064,0.,-0.466400197298193));
#88838=DIRECTION('center_axis',(-0.0690217385068017,0.987363722098133,-0.142649500167436));
#88839=DIRECTION('ref_axis',(-0.917511161069893,-0.00668760596951243,0.397653800734475));
#88840=DIRECTION('',(0.466400199211432,0.,-0.884573826300291));
#88841=DIRECTION('center_axis',(-4.08727706304602E-14,-1.,1.7692324809619E-14));
#88842=DIRECTION('ref_axis',(1.,-4.08727706304603E-14,-1.5709522500068E-31));
#88843=DIRECTION('center_axis',(-0.0819510664810077,-0.987363722021505,
-0.135635183999088));
#88844=DIRECTION('ref_axis',(-0.942872892860092,0.0327139788905535,0.331542611883886));
#88845=DIRECTION('center_axis',(0.0897023381954629,-0.987363722254225,0.130638319411068));
#88846=DIRECTION('ref_axis',(-0.915363188590782,-0.0300375642560458,0.401507132821424));
#88847=DIRECTION('',(-0.964155239073704,0.,-0.265338792804085));
#88848=DIRECTION('center_axis',(-0.0980734823229331,0.987363721984803,-0.124476795320935));
#88849=DIRECTION('ref_axis',(-0.810576446806066,-0.00668761541326269,0.585594654759875));
#88850=DIRECTION('',(0.265338796269035,0.,-0.964155238120138));
#88851=DIRECTION('center_axis',(-3.61138611426735E-14,-1.,2.60651256016803E-14));
#88852=DIRECTION('ref_axis',(1.,-3.61138611426735E-14,7.03962851519167E-32));
#88853=DIRECTION('center_axis',(-0.10919264797883,-0.987363722125025,-0.114847054201611));
#88854=DIRECTION('ref_axis',(-0.849557187882663,0.0327139749465049,0.526481130108288));
#88855=DIRECTION('center_axis',(0.115688529444972,-0.98736372208904,0.108300713097081));
#88856=DIRECTION('ref_axis',(-0.807650340411127,-0.0300375706146091,0.588896147028798));
#88857=DIRECTION('',(-0.998653822462692,0.,-0.0518704432278601));
#88858=DIRECTION('center_axis',(-0.122539409041195,0.987363721996483,-0.100483698762969));
#88859=DIRECTION('ref_axis',(-0.665740079912513,-0.00668761365265042,0.746153752132705));
#88860=DIRECTION('',(0.0518704469159844,0.,-0.998653822271129));
#88861=DIRECTION('center_axis',(-9.88876920374125E-15,-1.,1.10730500259122E-14));
#88862=DIRECTION('ref_axis',(2.65179613550382E-33,-1.10730500259122E-14,
-1.));
#88863=DIRECTION('center_axis',(-0.131328506916138,-0.987363722072865,-0.0886888020304502));
#88864=DIRECTION('ref_axis',(-0.716517133417842,0.0327139757254959,0.69680197567954));
#88865=DIRECTION('center_axis',(0.13626524791609,-0.987363722104922,0.0808990882611246));
#88866=DIRECTION('ref_axis',(-0.662172659358769,-0.0300375706213195,0.748749032419344));
#88867=DIRECTION('',(-0.986456463077436,0.,0.164023310699287));
#88868=DIRECTION('center_axis',(-0.141275529117461,0.987363722015998,-0.0717920978889472));
#88869=DIRECTION('ref_axis',(-0.489774445357342,-0.00668761016490139,0.871823530621416));
#88870=DIRECTION('',(-0.164023306625657,0.,-0.98645646375478));
#88871=DIRECTION('center_axis',(3.63859842182505E-15,-1.,-6.46998067506677E-15));
#88872=DIRECTION('ref_axis',(2.29970405697103E-32,6.46998067506677E-15,
-1.));
#88873=DIRECTION('center_axis',(-0.147323591451942,-0.987363722036411,-0.058383557686263));
#88874=DIRECTION('ref_axis',(-0.549973531153307,0.0327139780733239,0.834541137793327));
#88875=DIRECTION('center_axis',(0.150470353914617,-0.987363722120249,0.0497147144581797));
#88876=DIRECTION('ref_axis',(-0.485732522241045,-0.0300375683489521,0.873591243846362));
#88877=DIRECTION('',(-0.928133496571451,0.,0.372247515159002));
#88878=DIRECTION('center_axis',(-0.153405764587397,0.987363722018912,-0.039743575988041));
#88879=DIRECTION('ref_axis',(-0.290907503589963,-0.00668761014234149,0.95672780884933));
#88880=DIRECTION('',(-0.372247514395924,0.,-0.9281334968775));
#88881=DIRECTION('center_axis',(1.08133770958267E-14,-1.,-3.55045361378079E-14));
#88882=DIRECTION('ref_axis',(-5.72023480965401E-33,3.55045361378079E-14,
-1.));
#88883=DIRECTION('center_axis',(-0.156429986999111,-0.987363722017236,-0.0253483650701108));
#88884=DIRECTION('ref_axis',(-0.357713779802522,0.0327139782837103,0.933258081863878));
#88885=DIRECTION('center_axis',(0.157639635047916,-0.987363722095111,0.0162057320861793));
#88886=DIRECTION('ref_axis',(-0.286580070934241,-0.0300375700506857,0.957585300288583));
#88887=DIRECTION('',(-0.82641203914066,0.,0.563065841232956));
#88888=DIRECTION('center_axis',(-0.158362916897451,0.987363722042217,-0.00583668970149514));
#88889=DIRECTION('ref_axis',(-0.0784380504043121,-0.00668760906902361,0.996896558391948));
#88890=DIRECTION('',(-0.563065840553765,0.,-0.826412039603419));
#88891=DIRECTION('center_axis',(1.17125623364526E-15,-1.,-1.47996064969821E-14));
#88892=DIRECTION('ref_axis',(3.94381262549887E-33,1.47996064969821E-14,
-1.));
#88893=DIRECTION('center_axis',(-0.15822188942635,-0.98736372216291,0.00887208334943327));
#88894=DIRECTION('ref_axis',(-0.14872773252229,0.0327139731913081,0.988336914992462));
#88895=DIRECTION('center_axis',(0.157437861539007,-0.987363721967107,-0.0180610159538643));
#88896=DIRECTION('ref_axis',(-0.0740274533496773,-0.0300375752097382,0.996803732048632));
#88897=DIRECTION('',(-0.686048471277773,0.,0.727555836384694));
#88898=DIRECTION('',(0.761237618626307,0.,-0.648473043378173));
#88899=DIRECTION('center_axis',(0.154431769357297,-0.987363722514828,0.0355486719138206));
#88900=DIRECTION('ref_axis',(-0.188052377251641,0.00594770337842175,0.982140992034509));
#88901=DIRECTION('center_axis',(9.79631271996063E-14,-1.,-5.15165042619057E-13));
#88902=DIRECTION('ref_axis',(-2.51994924462431E-30,5.15165042619057E-13,
-1.));
#88903=DIRECTION('center_axis',(-0.179949042279907,0.983673454101297,0.00220859207834743));
#88904=DIRECTION('ref_axis',(-0.00321947738172968,-0.00283418610278911,
0.999990801134952));
#88905=DIRECTION('center_axis',(0.,1.,-4.27898457407613E-15));
#88906=DIRECTION('ref_axis',(0.,-4.27898457407613E-15,-1.));
#88907=DIRECTION('center_axis',(0.15853152106945,0.98256963623183,0.0970807230229386));
#88908=DIRECTION('ref_axis',(-0.347991529212697,-0.0364113180679517,0.936790324198944));
#88909=DIRECTION('center_axis',(-0.1527723673653,-0.987363723844037,-0.0421127131213217));
#88910=DIRECTION('ref_axis',(-0.260766127816424,-0.000828290449268767,0.965401647252873));
#88911=DIRECTION('',(0.469668518497478,0.,0.882842841468619));
#88912=DIRECTION('center_axis',(5.55366423743563E-15,-1.,-2.91677489184056E-14));
#88913=DIRECTION('ref_axis',(-1.35478984408908E-31,2.91677489184056E-14,
-1.));
#88914=DIRECTION('center_axis',(-0.14732530161365,0.987363878712072,-0.0583765922189797));
#88915=DIRECTION('ref_axis',(-0.215660138228666,0.0255338646749638,0.976134584232089));
#88916=DIRECTION('center_axis',(0.157369919791754,0.987363724405155,0.0186436067733055));
#88917=DIRECTION('ref_axis',(-0.160618010575024,0.00696334191558068,0.986992080286508));
#88918=DIRECTION('',(0.882842841300013,0.,-0.469668518814407));
#88919=DIRECTION('center_axis',(0.143179326239305,-0.987363722493451,0.0679158305664762));
#88920=DIRECTION('ref_axis',(-0.394787099410106,0.0059477047491631,0.918753378740765));
#88921=DIRECTION('center_axis',(-2.06418061594693E-13,-1.,4.8206159791424E-13));
#88922=DIRECTION('ref_axis',(-8.43588309106855E-30,-4.8206159791424E-13,
-1.));
#88923=DIRECTION('center_axis',(-0.176216739608827,0.983673453678242,-0.0365266643748751));
#88924=DIRECTION('ref_axis',(-0.218112650942901,-0.00283429096832737,0.975919483509458));
#88925=DIRECTION('center_axis',(0.,1.,-4.27898457407613E-15));
#88926=DIRECTION('ref_axis',(0.,-4.27898457407613E-15,-1.));
#88927=DIRECTION('center_axis',(0.133955657112767,0.982569636300036,0.12889061932003));
#88928=DIRECTION('ref_axis',(-0.541237908795975,-0.0364113167100376,0.840080794982007));
#88929=DIRECTION('center_axis',(-0.140147645931868,-0.98736372384866,-0.0739696841108766));
#88930=DIRECTION('ref_axis',(-0.462202379579607,-0.000828289852944301,0.886774082981042));
#88931=DIRECTION('',(0.268902817760427,0.,0.963167313918253));
#88932=DIRECTION('center_axis',(3.50820794247826E-14,-1.,-8.18758485032203E-14));
#88933=DIRECTION('ref_axis',(1.0873911167328E-31,8.18758485032203E-14,-1.));
#88934=DIRECTION('center_axis',(-0.131331675171813,0.987363878709653,-0.0886823664320867));
#88935=DIRECTION('ref_axis',(-0.42045820551751,0.0255338665054303,0.906952545106015));
#88936=DIRECTION('center_axis',(0.149682873117739,0.987363724365384,0.052037614304822));
#88937=DIRECTION('ref_axis',(-0.369036976815383,0.00696333868578459,0.929388627893256));
#88938=DIRECTION('',(0.9631673145042,0.,-0.268902815661658));
#88939=DIRECTION('center_axis',(0.125231976535853,-0.987363722499094,0.0971073197326294));
#88940=DIRECTION('ref_axis',(-0.583062014846573,0.0059477057068179,0.812405878634491));
#88941=DIRECTION('center_axis',(1.52610558579865E-13,-1.,-2.13208742943039E-13));
#88942=DIRECTION('ref_axis',(4.34777305341731E-30,2.13208742943039E-13,
-1.));
#88943=DIRECTION('center_axis',(-0.164244673331451,0.983673454241399,-0.0735542160792886));
#88944=DIRECTION('ref_axis',(-0.422807164527357,-0.00283414450632821,0.906215244436582));
#88945=DIRECTION('center_axis',(0.,1.,-4.27898457407613E-15));
#88946=DIRECTION('ref_axis',(0.,-4.27898457407613E-15,-1.));
#88947=DIRECTION('center_axis',(0.10311615443596,0.982569635229474,0.154673755431737));
#88948=DIRECTION('ref_axis',(-0.709176608070518,-0.036411345534319,0.70409001731453));
#88949=DIRECTION('center_axis',(-0.120969775086762,-0.987363723798551,-0.102367917054697));
#88950=DIRECTION('ref_axis',(-0.642026559594874,-0.000828292162798994,0.76668194885941));
#88951=DIRECTION('',(0.0555635156269576,0.,0.998455154591919));
#88952=DIRECTION('center_axis',(8.64379451955931E-14,-1.,-1.2070004440492E-13));
#88953=DIRECTION('ref_axis',(3.17309574127229E-30,1.2070004440492E-13,-1.));
#88954=DIRECTION('center_axis',(-0.109197112976554,0.987363878298483,-0.114841466156457));
#88955=DIRECTION('ref_axis',(-0.605596116332949,0.0255338871524541,0.795362410784753));
#88956=DIRECTION('center_axis',(0.134996817658912,0.987363724450577,0.08299840276205));
#88957=DIRECTION('ref_axis',(-0.560200179129411,0.00696333125741769,0.82832799742685));
#88958=DIRECTION('',(0.998455154553505,1.49610497004341E-14,-0.055563516317241));
#88959=DIRECTION('center_axis',(0.10142892175727,-0.987363722503769,0.121758175555722));
#88960=DIRECTION('ref_axis',(-0.74407359701472,0.00594770268880726,0.668071184125092));
#88961=DIRECTION('center_axis',(-7.79504734952084E-13,-1.,7.01669120585349E-13));
#88962=DIRECTION('ref_axis',(1.,-7.79504734952084E-13,-1.59279744026798E-30));
#88963=DIRECTION('center_axis',(-0.14459285205623,0.983673453495816,-0.107142167337888));
#88964=DIRECTION('ref_axis',(-0.607731631042885,-0.00283432086000192,0.794137413332994));
#88965=DIRECTION('center_axis',(0.,1.,-4.27898457407613E-15));
#88966=DIRECTION('ref_axis',(0.,-4.27898457407613E-15,-1.));
#88967=DIRECTION('center_axis',(0.0674551032578653,0.982569636602003,0.173224473652768));
#88968=DIRECTION('ref_axis',(-0.843954992283683,-0.036411307495574,0.535176781714146));
#88969=DIRECTION('center_axis',(-0.0961354912201982,-0.987363723790838,
-0.125979539091637));
#88970=DIRECTION('ref_axis',(-0.791830292288917,-0.000828293965008936,0.610740617727981));
#88971=DIRECTION('',(-0.160373869647189,0.,0.987056341823701));
#88972=DIRECTION('center_axis',(1.10364015858298E-13,-1.,-9.92965414012673E-14));
#88973=DIRECTION('ref_axis',(1.,1.10364015858298E-13,3.53523353257534E-30));
#88974=DIRECTION('center_axis',(-0.0819566430429945,0.98736387872903,-0.135630673677782));
#88975=DIRECTION('ref_axis',(-0.762417021447238,0.025533864141092,0.646582018919137));
#88976=DIRECTION('center_axis',(0.113998471850588,0.987363724368407,0.110078264053714));
#88977=DIRECTION('ref_axis',(-0.725169043306024,0.00696334205636933,0.688535671187798));
#88978=DIRECTION('',(0.987056341019167,0.,0.160373874598871));
#88979=DIRECTION('center_axis',(0.0728831631304263,-0.987363722530532,0.140715755915086));
#88980=DIRECTION('ref_axis',(-0.870293126478398,0.00594770050821674,0.492498222192852));
#88981=DIRECTION('center_axis',(1.8242369488553E-12,-1.,-1.03538802890571E-12));
#88982=DIRECTION('ref_axis',(1.,1.8242369488553E-12,4.32938170593567E-29));
#88983=DIRECTION('center_axis',(-0.118179854965378,0.983673454033135,-0.135720513228048));
#88984=DIRECTION('ref_axis',(-0.764239288201414,-0.00283419611140209,0.644926567681778));
#88985=DIRECTION('center_axis',(0.,1.,-4.27898457407613E-15));
#88986=DIRECTION('ref_axis',(0.,-4.27898457407613E-15,-1.));
#88987=DIRECTION('center_axis',(0.0286398862805303,0.982569636100756,0.183675439639233));
#88988=DIRECTION('ref_axis',(-0.939270981848649,-0.0364113211302585,0.341239268476863));
#88989=DIRECTION('center_axis',(-0.0668060207260926,-0.987363723825072,
-0.143700495716029));
#88990=DIRECTION('ref_axis',(-0.904608919750942,-0.000828292839112309,0.426241734509898));
#88991=DIRECTION('',(-0.368812355268781,0.,0.929503871213614));
#88992=DIRECTION('center_axis',(0.,-1.,0.));
#88993=DIRECTION('ref_axis',(0.,0.,-1.));
#88994=DIRECTION('center_axis',(-0.0508839561738066,0.987363878729922,-0.150077959685978));
#88995=DIRECTION('ref_axis',(-0.883588156432343,0.0255338646246355,0.467568167832054));
#88996=DIRECTION('center_axis',(0.0876696764382493,0.987363724373119,0.132010998122337));
#88997=DIRECTION('ref_axis',(-0.856229809932433,0.00696333997322604,0.516548182147114));
#88998=DIRECTION('',(0.929503870800998,-1.49610497208486E-14,0.36881235630868));
#88999=DIRECTION('center_axis',(0.040929462489895,-0.987363722493695,0.153093626920526));
#89000=DIRECTION('ref_axis',(-0.955818717023452,0.0059477052689164,0.293896588938483));
#89001=DIRECTION('center_axis',(1.25260320433439E-12,-1.,-3.86890133542238E-13));
#89002=DIRECTION('ref_axis',(1.,1.25260320433439E-12,9.01406401442751E-30));
#89003=DIRECTION('center_axis',(-0.0862408680956417,0.983673454504075,-0.157952675109125));
#89004=DIRECTION('ref_axis',(-0.885011957399521,-0.00283407536007535,0.465559666720305));
#89005=DIRECTION('center_axis',(0.,1.,-4.27898457407613E-15));
#89006=DIRECTION('ref_axis',(0.,-4.27898457407613E-15,-1.));
#89007=DIRECTION('center_axis',(-0.0115145015438457,0.982569635704634,0.185537940177905));
#89008=DIRECTION('ref_axis',(-0.990667703801824,-0.0364113341316314,0.131345785584377));
#89009=DIRECTION('center_axis',(-0.0343527775896078,-0.987363723829323,
-0.15470217690056));
#89010=DIRECTION('ref_axis',(-0.975089038524001,-0.000828289881604484,0.221812264958932));
#89011=DIRECTION('',(-0.560005583301831,0.,0.828488833159975));
#89012=DIRECTION('center_axis',(-2.55342966086297E-13,-1.,7.88012148952781E-14));
#89013=DIRECTION('ref_axis',(1.,-2.55342966086297E-13,-6.56380829255718E-31));
#89014=DIRECTION('center_axis',(-0.0174319786951678,0.987363878487336,-0.157507769894744));
#89015=DIRECTION('ref_axis',(-0.963443691424393,0.025533878586369,0.26669134687664));
#89016=DIRECTION('center_axis',(0.0572415384935087,0.987363724423093,0.147771045757462));
#89017=DIRECTION('ref_axis',(-0.94725422437822,0.00696333293275186,0.320407469313818));
#89018=DIRECTION('',(0.828488831038156,0.,0.560005586440912));
#89019=DIRECTION('center_axis',(0.00706195074453439,-0.98736372248627,0.158313007582248));
#89020=DIRECTION('ref_axis',(-0.996651285552064,0.00594770480154678,0.081552681225151));
#89021=DIRECTION('center_axis',(-5.22595194025683E-13,-1.,4.34288782212213E-14));
#89022=DIRECTION('ref_axis',(1.,-5.22595194025683E-13,8.12900788325336E-31));
#89023=DIRECTION('center_axis',(-0.0502692615742574,0.983673455286747,-0.172799116621036));
#89024=DIRECTION('ref_axis',(-0.964402445769318,-0.00283388505453427,0.26442369729216));
#89025=DIRECTION('center_axis',(0.,1.,-4.27898457407613E-15));
#89026=DIRECTION('ref_axis',(0.,-4.27898457407613E-15,-1.));
#89027=DIRECTION('center_axis',(-0.0511301072340958,0.982569648595428,0.178724922138149));
#89028=DIRECTION('ref_axis',(-0.995741923384931,-0.0364109742150284,-0.0846892140144853));
#89029=DIRECTION('center_axis',(-0.000293231080172163,-0.987363723819408,
-0.158470157761663));
#89030=DIRECTION('ref_axis',(-0.99997507892601,-0.000828292153617314,0.00701109542287292));
#89031=DIRECTION('',(-0.725013572849968,0.,0.688734578181845));
#89032=DIRECTION('center_axis',(8.87710405090975E-14,-1.,-7.35589882339766E-15));
#89033=DIRECTION('ref_axis',(1.,8.87710405090975E-14,-3.44266811200455E-31));
#89034=DIRECTION('center_axis',(0.0168351068554852,0.987363878107483,-0.157572686039542));
#89035=DIRECTION('ref_axis',(-0.998249669190184,0.0255338992760699,0.0533443338082583));
#89036=DIRECTION('center_axis',(0.0241368608849463,0.987363724418675,0.156621478886847));
#89037=DIRECTION('ref_axis',(-0.99398608115497,0.00696333673097982,0.109284868173762));
#89038=DIRECTION('',(0.688734576602033,0.,0.725013574350727));
#89039=DIRECTION('center_axis',(-0.0271357688700418,-0.987363722528924,
0.156129848144604));
#89040=DIRECTION('ref_axis',(-0.990881548149455,0.00594770300098519,-0.134604540658744));
#89041=DIRECTION('center_axis',(-2.33870895678053E-12,-1.,-3.14680407007958E-13));
#89042=DIRECTION('ref_axis',(1.,-2.33870895678053E-12,1.39936086943571E-29));
#89043=DIRECTION('center_axis',(-0.0119474158641637,0.983673454794409,-0.179565569046522));
#89044=DIRECTION('ref_axis',(-0.998698529282127,-0.00283400570072031,0.0509236293031502));
#89045=DIRECTION('center_axis',(0.,1.,-1.15648231693495E-15));
#89046=DIRECTION('ref_axis',(0.,-1.15648231693495E-15,-1.));
#89047=DIRECTION('center_axis',(-0.0883556907948313,0.982569633847177,0.163554842623486));
#89048=DIRECTION('ref_axis',(-0.954256320475309,-0.0364113920932505,-0.29676435998744));
#89049=DIRECTION('center_axis',(0.0337800228186421,-0.987363723842413,-0.1548282496782));
#89050=DIRECTION('ref_axis',(-0.978103395941278,-0.000828291187283654,-0.20811790115665));
#89051=DIRECTION('',(-0.856120733893417,0.,0.51677585953467));
#89052=DIRECTION('center_axis',(2.94256412139621E-14,-1.,3.96640921599374E-15));
#89053=DIRECTION('ref_axis',(1.,2.94256412139621E-14,-2.02248610404404E-31));
#89054=DIRECTION('center_axis',(0.0503150650657662,0.987363876577224,-0.15026965581189));
#89055=DIRECTION('ref_axis',(-0.986378597171141,0.0255339838968591,-0.162497011384971));
#89056=DIRECTION('center_axis',(-0.0100964402476896,0.987363724433846,0.158148466848242));
#89057=DIRECTION('ref_axis',(-0.994240255523169,0.00696332969227714,-0.106947773875007));
#89058=DIRECTION('',(0.516775858941039,0.,0.856120734251748));
#89059=DIRECTION('center_axis',(-0.060064648265057,-0.987363722569294,0.14664623207877));
#89060=DIRECTION('ref_axis',(-0.938779290848018,0.00594769916006849,-0.3444678039376));
#89061=DIRECTION('center_axis',(2.46264932681847E-13,-1.,9.00085221191213E-14));
#89062=DIRECTION('ref_axis',(1.,2.46264932681847E-13,-2.27872523730751E-30));
#89063=DIRECTION('center_axis',(0.026932910420601,0.98367345360326,-0.177935817115363));
#89064=DIRECTION('ref_axis',(-0.986296594519741,-0.00283429344636968,-0.164957553386989));
#89065=DIRECTION('center_axis',(0.,1.,6.24500451401115E-15));
#89066=DIRECTION('ref_axis',(0.,6.24500451401115E-15,-1.));
#89067=DIRECTION('center_axis',(-0.121449392028066,0.982569635669132,0.140737188536086));
#89068=DIRECTION('ref_axis',(-0.868150771829313,-0.036411333705666,-0.494963081603004));
#89069=DIRECTION('center_axis',(0.066273764426829,-0.987363723798804,-0.143946743884176));
#89070=DIRECTION('ref_axis',(-0.910496684258415,-0.000828293773487352,-0.413515540075408));
#89071=DIRECTION('',(-0.947196640816497,0.,0.320653276337453));
#89072=DIRECTION('center_axis',(-1.39425126750654E-13,-1.,-5.09965991050609E-14));
#89073=DIRECTION('ref_axis',(1.,-1.39425126750654E-13,2.37851799223888E-30));
#89074=DIRECTION('center_axis',(0.0814421546484781,0.987363878604472,-0.135940231989459));
#89075=DIRECTION('ref_axis',(-0.928385569322247,0.0255338686512898,-0.370740146498738));
#89076=DIRECTION('center_axis',(-0.0438576377861118,0.987363724437607,0.152280607013892));
#89077=DIRECTION('ref_axis',(-0.948004858277966,0.00696332974445473,-0.318179667358307));
#89078=DIRECTION('',(0.320653274273476,0.,0.947196641515213));
#89079=DIRECTION('center_axis',(-0.0901849776072001,-0.98736372250566,0.13030559962548));
#89080=DIRECTION('ref_axis',(-0.842780756740556,0.00594770166763986,-0.538224136315614));
#89081=DIRECTION('center_axis',(1.76926578827669E-12,-1.,1.12675082955071E-12));
#89082=DIRECTION('ref_axis',(1.,1.76926578827669E-12,-4.04402725272487E-29));
#89083=DIRECTION('center_axis',(0.0645545535556254,0.983673455265295,-0.167985841729802));
#89084=DIRECTION('ref_axis',(-0.927776503494073,-0.00283389108700792,-0.373125620435824));
#89085=DIRECTION('center_axis',(-7.60100351384829E-30,1.,-4.27898457407613E-15));
#89086=DIRECTION('ref_axis',(-1.77635683940025E-15,-4.27898457407613E-15,
-1.));
#89087=DIRECTION('center_axis',(-0.148864294762263,0.982569636291619,0.111338814358196));
#89088=DIRECTION('ref_axis',(-0.741451459750958,-0.0364113156534541,-0.670017872094139));
#89089=DIRECTION('center_axis',(0.0956686121200815,-0.987363723836582,-0.126334450988536));
#89090=DIRECTION('ref_axis',(-0.800316162506508,-0.000828290255901962,-0.599577646319564));
#89091=DIRECTION('',(-0.993982685952451,0.,0.109537299705404));
#89092=DIRECTION('center_axis',(0.,-1.,0.));
#89093=DIRECTION('ref_axis',(0.,0.,-1.));
#89094=DIRECTION('center_axis',(0.108761234480361,0.987363878205077,-0.115254353020345));
#89095=DIRECTION('ref_axis',(-0.826982255347822,0.0255338944294636,-0.561647905342034));
#89096=DIRECTION('center_axis',(-0.0755680941385575,0.987363724415618,0.139292278523919));
#89097=DIRECTION('ref_axis',(-0.857441809996997,0.00696333571685899,-0.514533822430332));
#89098=DIRECTION('',(0.109537300692827,0.,0.993982685843636));
#89099=DIRECTION('center_axis',(-0.116088355286957,-0.987363722529239,0.107872022322625));
#89100=DIRECTION('ref_axis',(-0.707374732400917,0.00594770236913799,-0.706813704449241));
#89101=DIRECTION('center_axis',(1.11426240627337E-12,-1.,1.11056089515527E-12));
#89102=DIRECTION('ref_axis',(1.,1.11426240627337E-12,3.64970774101204E-29));
#89103=DIRECTION('center_axis',(0.0991569279023106,0.983673453428792,-0.150181359257569));
#89104=DIRECTION('ref_axis',(-0.825874670625604,-0.00283432932651998,-0.563846605910082));
#89105=DIRECTION('center_axis',(0.,1.,-4.27898457407613E-15));
#89106=DIRECTION('ref_axis',(0.,-4.27898457407613E-15,-1.));
#89107=DIRECTION('center_axis',(-0.169318486318183,0.982569636205712,0.0767343482248568));
#89108=DIRECTION('ref_axis',(-0.580082699670365,-0.0364113198382961,-0.813743373140927));
#89109=DIRECTION('center_axis',(0.120590108538849,-0.987363723795561,-0.102814895103539));
#89110=DIRECTION('ref_axis',(-0.652713741417794,-0.000828293707041192,-0.75760417481289));
#89111=DIRECTION('',(-0.994291204850995,0.,-0.106700515256288));
#89112=DIRECTION('center_axis',(-1.47176262462041E-13,-1.,-1.46756891477855E-13));
#89113=DIRECTION('ref_axis',(1.,-1.47176262462041E-13,6.44798894018817E-30));
#89114=DIRECTION('center_axis',(0.130994717001781,0.987363878694593,-0.0891793427133922));
#89115=DIRECTION('ref_axis',(-0.686910176005267,0.0255338649006621,-0.726293626464978));
#89116=DIRECTION('center_axis',(-0.103745077874136,0.987363724403459,0.119790794926074));
#89117=DIRECTION('ref_axis',(-0.726785732907313,0.00696333438935478,-0.686828952808894));
#89118=DIRECTION('',(-0.106700517422838,0.,0.994291204618495));
#89119=DIRECTION('center_axis',(-0.136563572302587,-0.987363722483103,0.0803944665027728));
#89120=DIRECTION('ref_axis',(-0.538892649528834,0.00594770583704457,-0.842353451396187));
#89121=DIRECTION('center_axis',(-4.24736902889226E-13,-1.,-6.62065039069767E-13));
#89122=DIRECTION('ref_axis',(1.77844195838957E-29,6.62065039069767E-13,
-1.));
#89123=DIRECTION('center_axis',(0.129123319223923,0.983673453902652,-0.125354315920209));
#89124=DIRECTION('ref_axis',(-0.685355812260115,-0.00283422476887034,-0.728202841089787));
#89125=DIRECTION('center_axis',(0.,1.,-4.27898457407613E-15));
#89126=DIRECTION('ref_axis',(0.,-4.27898457407613E-15,-1.));
#89127=DIRECTION('center_axis',(-0.181855534063347,0.982569635880059,0.038541865251469));
#89128=DIRECTION('ref_axis',(-0.391589916338328,-0.0364113275118482,-0.919419138723448));
#89129=DIRECTION('center_axis',(0.139872940537657,-0.987363723824141,-0.0744878337815988));
#89130=DIRECTION('ref_axis',(-0.474591153553507,-0.000828290669261229,-0.88020597072692));
#89131=DIRECTION('',(-0.948107772469134,0.,-0.317949133956387));
#89132=DIRECTION('center_axis',(4.80801298666205E-14,-1.,7.49847183817704E-14));
#89133=DIRECTION('ref_axis',(2.14746147750984E-30,-7.49847183817705E-14,
-1.));
#89134=DIRECTION('center_axis',(0.147103062861328,0.987363878429286,-0.0589343742640444));
#89135=DIRECTION('ref_axis',(-0.514718935115872,0.0255338794681674,-0.856978668831663));
#89136=DIRECTION('center_axis',(-0.127071055085179,0.987363724395657,0.0946880283197176));
#89137=DIRECTION('ref_axis',(-0.562145965376946,0.0069633349371206,-0.827008721584588));
#89138=DIRECTION('',(-0.317949138606538,-1.49610497417568E-14,0.9481077709097));
#89139=DIRECTION('center_axis',(-0.150653225448128,-0.987363722481458,0.049157758183571));
#89140=DIRECTION('ref_axis',(-0.345212548031876,0.00594770514329176,-0.938505685376955));
#89141=DIRECTION('center_axis',(-1.8165491871178E-13,-1.,-4.91928138225692E-13));
#89142=DIRECTION('ref_axis',(5.43771059840649E-30,4.91928138225691E-13,
-1.));
#89143=DIRECTION('center_axis',(0.153052046561606,0.983673454582958,-0.0946657582874232));
#89144=DIRECTION('ref_axis',(-0.512790461815737,-0.00283405764388026,-0.858509120736684));
#89145=DIRECTION('center_axis',(0.,1.,-4.27898457407613E-15));
#89146=DIRECTION('ref_axis',(0.,-4.27898457407613E-15,-1.));
#89147=DIRECTION('center_axis',(-0.185889211649551,0.982569636439812,-0.00145276937064705));
#89148=DIRECTION('ref_axis',(-0.184786826538217,-0.0364113103312805,-0.982103887181949));
#89149=DIRECTION('center_axis',(0.152615469816189,-0.987363723872379,-0.0426778063359844));
#89150=DIRECTION('ref_axis',(-0.274277213979071,-0.000828286521980904,-0.961650312657005));
#89151=DIRECTION('',(-0.85759187372498,0.,-0.514330806116917));
#89152=DIRECTION('center_axis',(3.08365452100123E-14,-1.,8.35674239769942E-14));
#89153=DIRECTION('ref_axis',(-1.42611513161612E-30,-8.35674239769942E-14,
-1.));
#89154=DIRECTION('center_axis',(0.156333027251661,0.987363878204671,-0.0259336963613628));
#89155=DIRECTION('ref_axis',(-0.318460008541339,0.0255338945707047,-0.947592340190602));
#89156=DIRECTION('center_axis',(-0.144455329569359,0.987363724393657,0.0651577586362149));
#89157=DIRECTION('ref_axis',(-0.371220879538658,0.00696333928487479,-0.928518481507261));
#89158=DIRECTION('',(-0.514330810099968,0.,0.857591871336191));
#89159=DIRECTION('center_axis',(-0.157698501364659,-0.987363722506079,0.0156224884790626));
#89160=DIRECTION('ref_axis',(-0.135390689940926,0.00594770349990451,-0.990774437447998));
#89161=DIRECTION('center_axis',(1.07486897960175E-13,-1.,7.79216493293677E-13));
#89162=DIRECTION('ref_axis',(-6.24504444031443E-30,-7.79216493293677E-13,
-1.));
#89163=DIRECTION('center_axis',(0.169824166749787,0.983673455248736,-0.059550699632786));
#89164=DIRECTION('ref_axis',(-0.316247594399455,-0.00283389191344847,-0.948672455641662));
#89165=DIRECTION('center_axis',(0.,1.,-6.93889390918615E-16));
#89166=DIRECTION('ref_axis',(0.,-6.93889390918615E-16,-1.));
#89167=DIRECTION('center_axis',(-0.181230923707162,0.982569636964586,-0.0413794732630985));
#89168=DIRECTION('ref_axis',(0.0306566983224309,-0.0364112919812353,-0.998866549977636));
#89169=DIRECTION('center_axis',(0.158221872134797,-0.987363723844001,-0.00887220463401044));
#89170=DIRECTION('ref_axis',(-0.0611383729137627,-0.000828289971577882,
-0.998128956244222));
#89171=DIRECTION('',(-0.726975931972861,0.,-0.686662940846665));
#89172=DIRECTION('center_axis',(8.10071867472569E-15,-1.,5.8828406537924E-14));
#89173=DIRECTION('ref_axis',(-2.96027912643716E-31,-5.8828406537924E-14,
-1.));
#89174=DIRECTION('center_axis',(0.158253025172948,0.987363878522611,0.00827957803249001));
#89175=DIRECTION('ref_axis',(-0.107310253376575,0.0255338744852763,-0.993897646024995));
#89176=DIRECTION('center_axis',(-0.155085035730741,0.987363724409335,0.0325807828776812));
#89177=DIRECTION('ref_axis',(-0.162937899276276,0.00696334414091573,-0.986611753841302));
#89178=DIRECTION('',(-0.686662940911435,-1.49610497356062E-14,0.726975931911682));
#89179=DIRECTION('center_axis',(-0.157369971134395,-0.987363722499165,-0.0186432743302372));
#89180=DIRECTION('ref_axis',(0.0807618870172637,0.00594770483092212,-0.996715677820237));
#89181=DIRECTION('center_axis',(-1.45914037233135E-13,-1.,1.82957882068821E-12));
#89182=DIRECTION('ref_axis',(-5.57821049776919E-30,-1.82957882068821E-12,
-1.));
#89183=DIRECTION('center_axis',(0.178655370734987,0.983673453557913,-0.021651680604346));
#89184=DIRECTION('ref_axis',(-0.104917442185756,-0.0028343060231339,-0.994476896179376));
#89185=DIRECTION('center_axis',(-1.17815554464648E-28,1.,-4.27898457407613E-15));
#89186=DIRECTION('ref_axis',(-2.75335310107039E-14,-4.27898457407613E-15,
-1.));
#89187=DIRECTION('center_axis',(-0.168098470378799,0.982569635535979,-0.0793713775803403));
#89188=DIRECTION('ref_axis',(0.244666740213606,-0.0364113367971972,-0.968923320384998));
#89189=DIRECTION('center_axis',(0.156429994655349,-0.987363723877192,0.0253482453730552));
#89190=DIRECTION('ref_axis',(0.154859228584172,-0.000828287352707057,-0.987936198983708));
#89191=DIRECTION('',(-0.56236740413906,0.,-0.82688747890018));
#89192=DIRECTION('center_axis',(-7.1025601078218E-15,-1.,8.87916691229752E-14));
#89193=DIRECTION('ref_axis',(1.85894219214295E-31,-8.87916691229752E-14,
-1.));
#89194=DIRECTION('center_axis',(0.152773294212726,0.987363878745721,0.0421057184192046));
#89195=DIRECTION('ref_axis',(0.108857216014725,0.0255338639803358,-0.993729403968584));
#89196=DIRECTION('center_axis',(-0.158463138768053,0.987363724435778,-0.00151964472347802));
#89197=DIRECTION('ref_axis',(0.0529638481076019,0.00696333330908011,-0.998572152016499));
#89198=DIRECTION('',(-0.826887480125574,0.,0.562367402337279));
#89199=DIRECTION('center_axis',(-0.149682997251398,-0.987363722535522,-0.0520372919610015));
#89200=DIRECTION('ref_axis',(0.293138125971869,0.00594769977683875,-0.956051601101669));
#89201=DIRECTION('center_axis',(-1.53087973129973E-13,-1.,5.01553352378593E-13));
#89202=DIRECTION('ref_axis',(-1.5439867913458E-30,-5.01553352378593E-13,
-1.));
#89203=DIRECTION('center_axis',(0.179132969840175,0.983673453912093,0.017260219723152));
#89204=DIRECTION('ref_axis',(0.111318599148628,-0.00283423072957411,-0.993780728641766));
#89205=DIRECTION('center_axis',(5.42341871852767E-29,1.,1.3877787795361E-15));
#89206=DIRECTION('ref_axis',(-3.90798504668055E-14,1.3877787795361E-15,
-1.));
#89207=DIRECTION('center_axis',(-0.147105795085869,0.982569626528976,-0.113652162649302));
#89208=DIRECTION('ref_axis',(0.447236418309252,-0.0364116177255003,-0.893674314407953));
#89209=DIRECTION('center_axis',(0.147323624967262,-0.987363723844384,0.0583834425385917));
#89210=DIRECTION('ref_axis',(0.36361578510832,-0.000828287599040628,-0.931548643260089));
#89211=DIRECTION('',(-0.371463200767281,0.,-0.928447677834204));
#89212=DIRECTION('center_axis',(-7.80722712912228E-14,-1.,2.55566786620522E-13));
#89213=DIRECTION('ref_axis',(1.23397180528547E-30,-2.55566786620522E-13,
-1.));
#89214=DIRECTION('center_axis',(0.140149924152897,0.987363872412991,0.0739633842760113));
#89215=DIRECTION('ref_axis',(0.319934693632977,0.025534215437582,-0.947095452239087));
#89216=DIRECTION('center_axis',(-0.154431681661387,0.987363724384509,-0.0355490009534356));
#89217=DIRECTION('ref_axis',(0.266389055963699,0.0069633360032921,-0.96384043431186));
#89218=DIRECTION('',(-0.928447677255466,0.,0.3714632022138));
#89219=DIRECTION('center_axis',(-0.134997009578242,-0.987363722498697,-0.0829981138246456));
#89220=DIRECTION('ref_axis',(0.491807553744111,0.00594770547493303,-0.870683613535833));
#89221=DIRECTION('center_axis',(3.85992086760888E-13,-1.,-6.85377023961864E-13));
#89222=DIRECTION('ref_axis',(1.33719385355037E-30,6.85377023961864E-13,
-1.));
#89223=DIRECTION('center_axis',(0.171234423252512,0.983673454841072,0.0553652105063214));
#89224=DIRECTION('ref_axis',(0.322349575412552,-0.00283399345383913,-0.946616458610588));
#89225=DIRECTION('center_axis',(-1.06414049193876E-28,1.,-4.27898457407613E-15));
#89226=DIRECTION('ref_axis',(-2.48689957516035E-14,-4.27898457407613E-15,
-1.));
#89227=DIRECTION('center_axis',(-0.119234878010352,0.982569636402058,-0.142618208818457));
#89228=DIRECTION('ref_axis',(0.628893860402292,-0.0364113135319287,-0.776638093705931));
#89229=DIRECTION('center_axis',(0.131328564306877,-0.98736372382475,0.0886886975438091));
#89230=DIRECTION('ref_axis',(0.555370071831342,-0.00082829114203254,-0.831602908393083));
#89231=DIRECTION('',(-0.163189791341605,0.,-0.98659469489851));
#89232=DIRECTION('center_axis',(5.83050175047892E-14,-1.,-1.03470465022567E-13));
#89233=DIRECTION('ref_axis',(2.02332272046579E-30,1.03470465022567E-13,
-1.));
#89234=DIRECTION('center_axis',(0.120973533980727,0.987363878077678,0.102361986809662));
#89235=DIRECTION('ref_axis',(0.516052284274361,0.0255339002001935,-0.856176418640329));
#89236=DIRECTION('center_axis',(-0.143179166359676,0.987363724446293,-0.0679161392313565));
#89237=DIRECTION('ref_axis',(0.467358252587167,0.0069633313518086,-0.884040596214424));
#89238=DIRECTION('',(-0.986594695254103,0.,0.163189789191801));
#89239=DIRECTION('center_axis',(-0.113998716707124,-0.98736372251679,-0.110078027084955));
#89240=DIRECTION('ref_axis',(0.667480605241743,0.00594770079844067,-0.74460342900186));
#89241=DIRECTION('center_axis',(-8.73839331637463E-13,-1.,9.77293987086083E-13));
#89242=DIRECTION('ref_axis',(-4.44913230794167E-30,-9.77293987086083E-13,
-1.));
#89243=DIRECTION('center_axis',(0.155329156822049,0.983673454978525,0.0908811697303888));
#89244=DIRECTION('ref_axis',(0.518307778400948,-0.0028339603480268,-0.855189461767286));
#89245=DIRECTION('center_axis',(1.52533651582418E-28,1.,-6.36065274470406E-15));
#89246=DIRECTION('ref_axis',(2.39808173319034E-14,-6.36065274470406E-15,
-1.));
#89247=DIRECTION('center_axis',(-0.0857885343236945,0.982569636375351,-0.164915848394877));
#89248=DIRECTION('ref_axis',(0.781144903269328,-0.0364113132365839,-0.623287137974738));
#89249=DIRECTION('center_axis',(0.109192725242245,-0.987363723808637,0.114846966267784));
#89250=DIRECTION('ref_axis',(0.721155873171584,-0.000828293443733472,-0.692772343934212));
#89251=DIRECTION('',(0.0527141884073562,0.,-0.998609640620675));
#89252=DIRECTION('center_axis',(3.95924850534664E-14,-1.,-4.42587639328991E-14));
#89253=DIRECTION('ref_axis',(1.36628995448307E-30,4.42587639328991E-14,
-1.));
#89254=DIRECTION('center_axis',(0.0961404457214033,0.987363878266434,0.12597454739413));
#89255=DIRECTION('ref_axis',(0.68803988955902,0.0255338903723136,-0.725223504044143));
#89256=DIRECTION('center_axis',(-0.125231756383122,0.987363724377778,-0.0971075845443635));
#89257=DIRECTION('ref_axis',(0.646474270713916,0.00696333327397,-0.762904010537778));
#89258=DIRECTION('',(-0.998609640362467,0.,-0.0527141932988016));
#89259=DIRECTION('center_axis',(-0.0876699683262286,-0.987363722531034,
-0.132010818054195));
#89260=DIRECTION('ref_axis',(0.811943006995923,0.00594770035885419,-0.58370641443354));
#89261=DIRECTION('center_axis',(-1.4888983012459E-12,-1.,1.0732340937512E-12));
#89262=DIRECTION('ref_axis',(1.,-1.4888983012459E-12,-4.69499685681978E-29));
#89263=DIRECTION('center_axis',(0.132160981848279,0.983673454392736,0.122147492810783));
#89264=DIRECTION('ref_axis',(0.690030470301091,-0.00283410202124129,-0.723774770161125));
#89265=DIRECTION('center_axis',(-2.4703261420007E-28,1.,-4.27898457407613E-15));
#89266=DIRECTION('ref_axis',(-5.77315972805081E-14,-4.27898457407613E-15,
-1.));
#89267=DIRECTION('center_axis',(-0.048330800738981,0.982569635885247,-0.179502212622192));
#89268=DIRECTION('ref_axis',(0.896870480711448,-0.0364113271556149,-0.440791964630915));
#89269=DIRECTION('center_axis',(0.0819511579642553,-0.987363723811783,0.135635115692239));
#89270=DIRECTION('ref_axis',(0.853221223833652,-0.000828292888265932,-0.52154851848193));
#89271=DIRECTION('',(0.266153315026551,0.,-0.96393070959503));
#89272=DIRECTION('center_axis',(0.,-1.,0.));
#89273=DIRECTION('ref_axis',(0.,0.,-1.));
#89274=DIRECTION('center_axis',(0.0668119404962166,0.987363878416488,0.143696681261193));
#89275=DIRECTION('ref_axis',(0.827855514450642,0.0255338802774692,-0.560359945170637));
#89276=DIRECTION('center_axis',(-0.101428648131142,0.987363724383358,-0.121758388253595));
#89277=DIRECTION('ref_axis',(0.795361873886099,0.00696333474618824,-0.606094878329793));
#89278=DIRECTION('',(-0.963930709015073,0.,-0.266153317126987));
#89279=DIRECTION('center_axis',(-0.0572418717027848,-0.987363722547846,
-0.147770929212829));
#89280=DIRECTION('ref_axis',(0.918439855202016,0.00594769809152563,-0.395515938065601));
#89281=DIRECTION('center_axis',(2.40686042267118E-13,-1.,-1.04010479394898E-13));
#89282=DIRECTION('ref_axis',(1.,2.40686042267118E-13,2.52683201209334E-30));
#89283=DIRECTION('center_axis',(0.102812939313603,0.983673454849758,0.147702517695669));
#89284=DIRECTION('ref_axis',(0.829488134170337,-0.00283399370384824,-0.558517147230324));
#89285=DIRECTION('center_axis',(3.80050175692414E-28,1.,-4.27898457407613E-15));
#89286=DIRECTION('ref_axis',(8.88178419700125E-14,-4.27898457407613E-15,
-1.));
#89287=DIRECTION('center_axis',(-0.00861320750497983,0.982569636773598,
-0.185695238353267));
#89288=DIRECTION('ref_axis',(0.970659390064181,-0.0364113029242347,-0.237685854647665));
#89289=DIRECTION('center_axis',(0.0508776450489319,-0.987363723838188,0.150081118341584));
#89290=DIRECTION('ref_axis',(0.945390901075399,-0.000828292330195558,-0.325937659830314));
#89291=DIRECTION('',(0.467147407829532,0.,-0.884179449748833));
#89292=DIRECTION('center_axis',(1.63550816575494E-13,-1.,-7.06311398100092E-14));
#89293=DIRECTION('ref_axis',(1.,1.63550816575494E-13,1.71046772606188E-30));
#89294=DIRECTION('center_axis',(0.0343593611981407,0.987363878193159,0.154699729597115));
#89295=DIRECTION('ref_axis',(0.928961537110486,0.0255338952362097,-0.369294574511176));
#89296=DIRECTION('center_axis',(-0.0728828540416005,0.987363724372173,-0.140715903083703));
#89297=DIRECTION('ref_axis',(0.907059237206504,0.00696334084921954,-0.420945426489672));
#89298=DIRECTION('',(-0.884179449358273,0.,-0.467147408568753));
#89299=DIRECTION('center_axis',(-0.0241372016724106,-0.987363722529379,
-0.156621438278268));
#89300=DIRECTION('ref_axis',(0.981991477421219,0.00594770310859909,-0.188831573365852));
#89301=DIRECTION('center_axis',(0.,-1.,0.));
#89302=DIRECTION('ref_axis',(0.,0.,-1.));
#89303=DIRECTION('center_axis',(0.0686577849377437,0.983673453837433,0.166350968686623));
#89304=DIRECTION('ref_axis',(0.930159821925432,-0.00283423621027203,-0.367143940138951));
#89305=DIRECTION('center_axis',(1.82424084332359E-28,1.,-4.27898457407613E-15));
#89306=DIRECTION('ref_axis',(4.2632564145606E-14,-4.27898457407613E-15,
-1.));
#89307=DIRECTION('center_axis',(0.031507168033603,0.982569636191183,-0.183205372185503));
#89308=DIRECTION('ref_axis',(0.999061345195437,-0.0364113191898648,-0.0234658128164505));
#89309=DIRECTION('center_axis',(0.0174251520844417,-0.987363723855214,0.15750949460143));
#89310=DIRECTION('ref_axis',(0.993355149241018,-0.00082829030093904,-0.115086321565737));
#89311=DIRECTION('',(0.646298207761542,0.,-0.763084940648299));
#89312=DIRECTION('center_axis',(5.83035654598128E-14,-1.,-1.12737439807098E-14));
#89313=DIRECTION('ref_axis',(1.,5.83035654598128E-14,1.90037748068761E-31));
#89314=DIRECTION('center_axis',(0.000300225257138507,0.98736387884835,0.158469178739384));
#89315=DIRECTION('ref_axis',(0.98663034989482,0.0255338596358639,-0.160961407419668));
#89316=DIRECTION('center_axis',(-0.0409291257697323,0.987363724396822,-0.153093704667965));
#89317=DIRECTION('ref_axis',(0.976343520524065,0.0069633328823719,-0.21611303043973));
#89318=DIRECTION('',(-0.763084940440831,0.,-0.646298208006501));
#89319=DIRECTION('',(0.795228819341496,0.,-0.606309429984995));
#89320=DIRECTION('',(-0.606309429638273,0.,-0.795228819605849));
#89321=DIRECTION('center_axis',(0.0438573042826761,-0.987363722495775,-0.152280715654819));
#89322=DIRECTION('ref_axis',(0.970519647114226,0.00594770341361158,0.240948623962417));
#89323=DIRECTION('center_axis',(-5.09105898905421E-13,-1.,-1.25709930644235E-13));
#89324=DIRECTION('ref_axis',(1.,-5.09105898905421E-13,-1.1652925221308E-30));
#89325=DIRECTION('center_axis',(-0.00753699341927212,0.983673454470314,
0.179804695991614));
#89326=DIRECTION('ref_axis',(0.998349928692214,-0.00283408599568885,0.0573531850625539));
#89327=DIRECTION('center_axis',(2.50833115956993E-28,1.,-4.27898457407613E-15));
#89328=DIRECTION('ref_axis',(5.86197757002083E-14,-4.27898457407613E-15,
-1.));
#89329=DIRECTION('center_axis',(0.105521068239957,0.982569636245178,-0.153043177196886));
#89330=DIRECTION('ref_axis',(0.916576558659195,-0.0364113166791358,0.398197976054825));
#89331=DIRECTION('center_axis',(-0.0503218807322454,-0.987363723831604,
0.150268377182156));
#89332=DIRECTION('ref_axis',(0.949868207862548,-0.000828290154810337,0.312649486849749));
#89333=DIRECTION('',(0.906975415979067,0.,-0.421183564268121));
#89334=DIRECTION('center_axis',(0.,-1.,0.));
#89335=DIRECTION('ref_axis',(0.,0.,-1.));
#89336=DIRECTION('center_axis',(-0.0662670360058364,0.987363878238492,0.14394878217215));
#89337=DIRECTION('ref_axis',(0.963027392457796,0.025533892898744,0.268190718872546));
#89338=DIRECTION('center_axis',(0.0271361056266256,0.987363724411646,-0.156129777708749));
#89339=DIRECTION('ref_axis',(0.976848887222061,0.00696333644544283,0.213817126251775));
#89340=DIRECTION('',(-0.421183562291818,0.,-0.906975416896828));
#89341=DIRECTION('center_axis',(0.0755677988040467,-0.987363722485756,-0.139292452426475));
#89342=DIRECTION('ref_axis',(0.896032605267977,0.0059477050242739,0.443948414910591));
#89343=DIRECTION('center_axis',(-1.41053807967382E-12,-1.,-6.9664085453623E-13));
#89344=DIRECTION('ref_axis',(1.,-1.41053807967382E-12,-2.42403792294253E-29));
#89345=DIRECTION('center_axis',(-0.0460132468312074,0.983673453550403,0.173980797492924));
#89346=DIRECTION('ref_axis',(0.962679834130023,-0.00283432164793642,0.270627980039365));
#89347=DIRECTION('center_axis',(1.5582057203389E-28,1.,-4.27898457407613E-15));
#89348=DIRECTION('ref_axis',(3.64153152077052E-14,-4.27898457407613E-15,
-1.));
#89349=DIRECTION('center_axis',(0.135953811406594,0.982569635914727,-0.126781196328247));
#89350=DIRECTION('ref_axis',(0.809546713012962,-0.0364113265778112,0.585925195521368));
#89351=DIRECTION('center_axis',(-0.0814486413983933,-0.987363723826403,
0.135937469764647));
#89352=DIRECTION('ref_axis',(0.860450419908865,-0.000828289274779208,0.509533501170958));
#89353=DIRECTION('',(0.976312850813305,0.,-0.216363622951729));
#89354=DIRECTION('center_axis',(-1.33094108435448E-13,-1.,-6.57721627022386E-14));
#89355=DIRECTION('ref_axis',(1.,-1.33094108435448E-13,1.11854033061799E-30));
#89356=DIRECTION('center_axis',(-0.0956624610075087,0.98736387863115,0.126337899018621));
#89357=DIRECTION('ref_axis',(0.882859272566599,0.0255338678676378,0.468942988469701));
#89358=DIRECTION('center_axis',(0.0600649648957384,0.987363724432964,-0.146646089841971));
#89359=DIRECTION('ref_axis',(0.908046341563117,0.00696333706420843,0.418811835447339));
#89360=DIRECTION('',(-0.21636361808406,0.,-0.976312851892043));
#89361=DIRECTION('center_axis',(0.103744821263164,-0.987363722547432,-0.119791032462169));
#89362=DIRECTION('ref_axis',(0.779648074778519,0.00594769971540888,0.626189671235676));
#89363=DIRECTION('center_axis',(4.09267768806296E-13,-1.,3.27859260674821E-13));
#89364=DIRECTION('ref_axis',(1.,4.09267768806296E-13,2.71155125619176E-30));
#89365=DIRECTION('center_axis',(0.16002949161871,0.982569636160366,-0.0945910773167529));
#89366=DIRECTION('ref_axis',(0.664663364509743,-0.0364113192768025,0.746255202800699));
#89367=DIRECTION('center_axis',(-0.0823382876057148,0.983673453893709,0.160021693838619));
#89368=DIRECTION('ref_axis',(0.881995891203354,-0.00283423637138487,0.471248570294481));
#89369=DIRECTION('center_axis',(-1.56128720824992E-28,1.,-4.39463280580791E-15));
#89370=DIRECTION('ref_axis',(-3.5527136788005E-14,-4.39463280580791E-15,
-1.));
#89371=DIRECTION('center_axis',(-0.108766955552993,-0.987363723823093,0.115250276606735));
#89372=DIRECTION('ref_axis',(0.73079892771557,-0.000828290184863653,0.682592294993976));
#89373=DIRECTION('',(0.999998982184334,0.,-0.00142675516336331));
#89374=DIRECTION('center_axis',(2.31686742770906E-14,-1.,1.85691490357841E-14));
#89375=DIRECTION('ref_axis',(1.,2.31686742770906E-14,-7.24715462277955E-31));
#89376=DIRECTION('center_axis',(-0.120584843313759,0.987363878562272,0.102819584094973));
#89377=DIRECTION('ref_axis',(0.761409632159749,0.0255338730448354,0.647768008921162));
#89378=DIRECTION('center_axis',(0.0901852594295258,0.987363724414169,-0.130305390113422));
#89379=DIRECTION('ref_axis',(0.796784555967793,0.00696333089617327,0.604223372101773));
#89380=DIRECTION('',(-0.00142675585914351,0.,-0.999998982183341));
#89381=DIRECTION('center_axis',(0.127070856507359,-0.987363722538901,-0.0946883141713354));
#89382=DIRECTION('ref_axis',(0.626808067237821,0.0059477006431547,0.779150994161367));
#89383=DIRECTION('center_axis',(-1.15226743321196E-12,-1.,-1.42861098163512E-12));
#89384=DIRECTION('ref_axis',(-2.34737927052863E-29,1.42861098163512E-12,
-1.));
#89385=DIRECTION('center_axis',(-0.114813363762878,0.983673454762913,0.13858003426269));
#89386=DIRECTION('ref_axis',(0.76007077865168,-0.00283402119491597,0.649834117112741));
#89387=DIRECTION('center_axis',(0.,1.,-4.27898457407613E-15));
#89388=DIRECTION('ref_axis',(0.,-4.27898457407613E-15,-1.));
#89389=DIRECTION('center_axis',(0.17662236999008,0.982569636655051,-0.0579779918818218));
#89390=DIRECTION('ref_axis',(0.488701096710683,-0.0364113059965099,0.871691146490203));
#89391=DIRECTION('center_axis',(-0.130999450776611,-0.987363723786601,0.0891741041249308));
#89392=DIRECTION('ref_axis',(0.566976085211815,-0.000828295465522612,0.82373383609301));
#89393=DIRECTION('',(0.976926272506191,0.,0.213576820107329));
#89394=DIRECTION('center_axis',(3.72703708255265E-14,-1.,4.6231185537332E-14));
#89395=DIRECTION('ref_axis',(-1.04756410394469E-30,-4.6231185537332E-14,
-1.));
#89396=DIRECTION('center_axis',(-0.139868816840048,0.987363878289649,0.0744935294142248));
#89397=DIRECTION('ref_axis',(0.60435732197669,0.0255338886823933,0.796304117722568));
#89398=DIRECTION('center_axis',(0.116088579768143,0.987363724373446,-0.107871763862534));
#89399=DIRECTION('ref_axis',(0.648266013062696,0.00696333901246309,0.761382090817478));
#89400=DIRECTION('',(0.213576824979769,0.,-0.976926271440973));
#89401=DIRECTION('center_axis',(0.144455199395496,-0.987363722528263,-0.065158075499038));
#89402=DIRECTION('ref_axis',(0.444659211184389,0.00594770136013063,0.895680082818306));
#89403=DIRECTION('center_axis',(-1.16888399219326E-13,-1.,-2.34702002391639E-13));
#89404=DIRECTION('ref_axis',(-3.88788071104734E-30,2.34702002391639E-13,
-1.));
#89405=DIRECTION('center_axis',(-0.14191956762245,0.983673453820766,0.110658811552366));
#89406=DIRECTION('ref_axis',(0.602605669735964,-0.00283423879207645,0.798034068127759));
#89407=DIRECTION('center_axis',(0.,1.,-1.61907524309175E-15));
#89408=DIRECTION('ref_axis',(0.,-1.61907524309175E-15,-1.));
#89409=DIRECTION('center_axis',(0.184956653255885,0.982569629181649,-0.018653692026481));
#89410=DIRECTION('ref_axis',(0.289887718521787,-0.0364115390294351,0.956367769467239));
#89411=DIRECTION('center_axis',(-0.14710655139176,-0.987363723814766,0.0589282566538495));
#89412=DIRECTION('ref_axis',(0.376642076271981,-0.000828292363707701,0.926358494489737));
#89413=DIRECTION('',(0.90817357582681,0.,0.418593784198889));
#89414=DIRECTION('center_axis',(6.61516798739843E-14,-1.,1.32905885278519E-13));
#89415=DIRECTION('ref_axis',(1.72437707524548E-30,-1.32905885278519E-13,
-1.));
#89416=DIRECTION('center_axis',(-0.152612751853645,0.987363874356831,0.042684043701661));
#89417=DIRECTION('ref_axis',(0.419045901386645,0.0255341087752613,0.9076059397228));
#89418=DIRECTION('center_axis',(0.136563732792872,0.987363724405006,-0.0803941702784063));
#89419=DIRECTION('ref_axis',(0.469435287154992,0.00696333778263528,0.882939422101332));
#89420=DIRECTION('',(0.418593786177838,0.,-0.908173574914676));
#89421=DIRECTION('center_axis',(0.155084977486587,-0.987363722529484,-0.0325811170880482));
#89422=DIRECTION('ref_axis',(0.241718583101083,0.00594770221519151,0.970328166870345));
#89423=DIRECTION('center_axis',(3.18508154599476E-13,-1.,1.27171196046668E-12));
#89424=DIRECTION('ref_axis',(-1.33343971397308E-29,-1.27171196046668E-12,
-1.));
#89425=DIRECTION('center_axis',(-0.162389976522538,0.983673454176114,0.0775630780348588));
#89426=DIRECTION('ref_axis',(0.416963315730168,-0.00283415624667476,0.908918896763443));
#89427=DIRECTION('center_axis',(0.,1.,-4.27898457407613E-15));
#89428=DIRECTION('ref_axis',(0.,-4.27898457407613E-15,-1.));
#89429=DIRECTION('center_axis',(0.184642449885204,0.982569635942888,0.021542428448301));
#89430=DIRECTION('ref_axis',(0.0775194882547595,-0.036411326478108,0.996325721962865));
#89431=DIRECTION('center_axis',(-0.156335115827123,-0.987363723801012,0.0259269836486918));
#89432=DIRECTION('ref_axis',(0.168696700721925,-0.000828295499094795,0.985667660569273));
#89433=DIRECTION('',(0.796955691356011,0.,0.604037768699328));
#89434=DIRECTION('center_axis',(3.60342536859394E-14,-1.,1.44019275252605E-13));
#89435=DIRECTION('ref_axis',(1.34143802813749E-30,-1.44019275252605E-13,
-1.));
#89436=DIRECTION('center_axis',(-0.158220517681057,0.987363878676579,0.00887912549075674));
#89437=DIRECTION('ref_axis',(0.214140432742777,0.0255338675260978,0.97646909663025));
#89438=DIRECTION('center_axis',(0.150653321523514,0.987363724405075,-0.0491574251041693));
#89439=DIRECTION('ref_axis',(0.268654254564643,0.00696333221351926,0.963211505074976));
#89440=DIRECTION('',(0.604037770435926,0.,-0.796955690039789));
#89441=DIRECTION('center_axis',(0.158463153889849,-0.98736372254709,0.0015192949799761));
#89442=DIRECTION('ref_axis',(0.0274754649281728,0.00594770014627042,0.999604783747032));
#89443=DIRECTION('center_axis',(3.01449049754687E-14,-1.,1.04835990607084E-12));
#89444=DIRECTION('ref_axis',(-1.4108466334676E-30,-1.04835990607084E-12,
-1.));
#89445=DIRECTION('center_axis',(-0.175267182846845,0.983673454681373,0.0408405334458729));
#89446=DIRECTION('ref_axis',(0.211824227594113,-0.00283403766675145,0.977303670736307));
#89447=DIRECTION('center_axis',(0.,1.,-4.27898457407613E-15));
#89448=DIRECTION('ref_axis',(0.,-4.27898457407613E-15,-1.));
#89449=DIRECTION('center_axis',(0.175694629832079,0.982569636637783,0.0607314268370501));
#89450=DIRECTION('ref_axis',(-0.138473451533026,-0.0364113059094351,0.989696579777105));
#89451=DIRECTION('center_axis',(-0.158253622888124,-0.987363723835983,-0.00828659734288716));
#89452=DIRECTION('ref_axis',(-0.04713674460817,-0.000828289383721378,0.998888102464155));
#89453=DIRECTION('',(0.64847304670282,0.,0.76123761579415));
#89454=DIRECTION('center_axis',(3.38552468895019E-15,-1.,1.18718787206932E-13));
#89455=DIRECTION('ref_axis',(0.0285055878552679,1.187670502004E-13,0.99959363316351));
#89456=DIRECTION('center_axis',(-0.156430158416636,0.987363878238024,-0.0253412211330566));
#89457=DIRECTION('ref_axis',(-0.000778046602915284,0.0255338905306592,0.999673654288164));
#89458=DIRECTION('center_axis',(0.157698523550761,0.98736372441666,-0.015622143770062));
#89459=DIRECTION('ref_axis',(0.0553112685315642,0.00696333467226083,0.998444878570505));
#89460=DIRECTION('center_axis',(-0.15910099913347,-0.986495109064463,0.0389136462776974));
#89461=DIRECTION('ref_axis',(0.0348288484460351,0.0337827392776246,0.998822145250506));
#89462=DIRECTION('center_axis',(0.153085996405273,-0.986495981700291,-0.0582267618349548));
#89463=DIRECTION('ref_axis',(0.142839315879286,-0.0362134380952001,0.989083169779196));
#89464=DIRECTION('center_axis',(-0.147016025755211,-0.986495109314144,0.0722058686702008));
#89465=DIRECTION('ref_axis',(0.248731805575957,0.0337827286644027,0.967983066039335));
#89466=DIRECTION('center_axis',(0.136989899164217,-0.986495981735127,-0.0897744147707253));
#89467=DIRECTION('ref_axis',(0.352123454896517,-0.0362134363722373,0.935252724956123));
#89468=DIRECTION('center_axis',(-0.12805674336805,-0.986495109232666,0.102121838692806));
#89469=DIRECTION('ref_axis',(0.451004340964367,0.0337827324183721,0.891882173508164));
#89470=DIRECTION('center_axis',(0.114488302547269,-0.986495981577749,-0.117124322456091));
#89471=DIRECTION('ref_axis',(0.544942693575336,-0.036213442345283,0.837690902011215));
#89472=DIRECTION('center_axis',(-0.10310967042645,-0.986495109194319,0.127262702313903));
#89473=DIRECTION('ref_axis',(0.632188414504733,0.0337827335010053,0.774077861382944));
#89474=DIRECTION('center_axis',(0.086633361464682,-0.986495981838967,-0.13899762047209));
#89475=DIRECTION('ref_axis',(0.712281020862011,-0.0362134416118077,0.700959580836441));
#89476=DIRECTION('center_axis',(-0.073341303578005,-0.986495109199416,0.146452902719994));
#89477=DIRECTION('ref_axis',(0.783812058775744,0.0337827346231783,0.62007852999367));
#89478=DIRECTION('center_axis',(0.0547275474985977,-0.986495981988411,-0.154371542278719));
#89479=DIRECTION('ref_axis',(0.846313876508417,-0.0362134352149882,0.531452170509469));
#89480=DIRECTION('center_axis',(-0.040143577861672,-0.986495109147448,0.158795128340351));
#89481=DIRECTION('ref_axis',(0.898785522715291,0.0337827367069714,0.437085015595352));
#89482=DIRECTION('center_axis',(0.0202627271776249,-0.986495981683972,-0.1625272285148));
#89483=DIRECTION('ref_axis',(0.9407740341983,-0.0362134386515169,0.337094650564627));
#89484=DIRECTION('center_axis',(-0.00506879005578622,-0.986495109267344,
0.163712268199367));
#89485=DIRECTION('ref_axis',(0.971732775009283,0.0337827312287656,0.23365389156503));
#89486=DIRECTION('center_axis',(-0.0151495567526714,-0.986495981610252,
-0.163083319800101));
#89487=DIRECTION('ref_axis',(0.991244645617973,-0.0362134411919114,0.126974955053111));
#89488=DIRECTION('center_axis',(0.0302430200186485,-0.986495109092999,0.160974406275479));
#89489=DIRECTION('ref_axis',(0.999242882453265,0.0337827374707905,0.0192973706880221));
#89490=DIRECTION('center_axis',(-0.0498534591473214,-0.986495981670541,
-0.156013815923214));
#89491=DIRECTION('ref_axis',(0.99536575872004,-0.0362134386964945,-0.0890819466864886));
#89492=DIRECTION('center_axis',(0.0641406912897081,-0.986495109175036,0.150709559400234));
#89493=DIRECTION('ref_axis',(0.980029503274231,0.0337827344540997,-0.195961474695582));
#89494=DIRECTION('center_axis',(-0.0822262684116405,-0.986495981776016,
-0.141649280700155));
#89495=DIRECTION('ref_axis',(0.952944675122492,-0.0362134351371844,-0.300973476026134));
#89496=DIRECTION('center_axis',(0.0950392159144675,-0.98649510921924,0.133397702097462));
#89497=DIRECTION('ref_axis',(0.914991035274494,0.0337827328184258,-0.402057374426374));
#89498=DIRECTION('center_axis',(-0.110754276086024,-0.986495981633421,-0.120661379694472));
#89499=DIRECTION('ref_axis',(0.865964958740324,-0.0362134402304153,-0.498791817275051));
#89500=DIRECTION('center_axis',(0.121493814933346,-0.986495109215181,0.109848315542248));
#89501=DIRECTION('ref_axis',(0.807168602240863,0.0337827331963323,-0.589353522509468));
#89502=DIRECTION('center_axis',(-0.134103531952518,-0.986495981849886,-0.0940314868110145));
#89503=DIRECTION('ref_axis',(0.738493679513785,-0.0362134399459039,-0.673287213665516));
#89504=DIRECTION('center_axis',(0.142267496094858,-0.986495109287407,0.0811625462077628));
#89505=DIRECTION('ref_axis',(0.661603860893941,0.0337827300359943,-0.74909215614739));
#89506=DIRECTION('center_axis',(-0.151182255928033,-0.986495981692509,-0.0630047902706147));
#89507=DIRECTION('ref_axis',(0.576491261957089,-0.0362134382866778,-0.816300442101179));
#89508=DIRECTION('center_axis',(0.156388911180492,-0.986495109171287,0.0486817012943271));
#89509=DIRECTION('ref_axis',(0.48510326018357,0.0337827340495557,-0.873804070624192));
#89510=DIRECTION('center_axis',(-0.161191868028005,-0.986495981537598,-0.0290320528349762));
#89511=DIRECTION('ref_axis',(0.387532750534317,-0.0362134429097134,-0.92114437186357));
#89512=DIRECTION('center_axis',(0.163197752494024,-0.986495109143777,0.0139245544383681));
#89513=DIRECTION('ref_axis',(0.285919770480985,0.0337827368528131,-0.957657878127066));
#89514=DIRECTION('center_axis',(-0.16366432424346,-0.986495981676962,0.00629818268533493));
#89515=DIRECTION('ref_axis',(0.180453638313151,-0.0362134381069366,-0.982916614632198));
#89516=DIRECTION('center_axis',(0.16237564746021,-0.98649510913597,-0.021483685966046));
#89517=DIRECTION('ref_axis',(0.0733669880836664,0.0337827359901104,-0.996732668175652));
#89518=DIRECTION('center_axis',(-0.158484018513546,-0.9864959819173,0.0413339271884475));
#89519=DIRECTION('ref_axis',(-0.0350632868139038,-0.0362134385253087,-0.998728768379073));
#89520=DIRECTION('center_axis',(0.153961037350102,-0.986495109136799,-0.0558873744888276));
#89521=DIRECTION('ref_axis',(-0.142616351467159,0.0337827368293704,-0.989201346029469));
#89522=DIRECTION('center_axis',(-0.145893179781864,-0.986495981719679,0.0744369407220874));
#89523=DIRECTION('ref_axis',(-0.248940685134136,-0.0362134373496924,-0.967841475780134));
#89524=DIRECTION('center_axis',(0.138347381237093,-0.986495109182415,-0.087677828805308));
#89525=DIRECTION('ref_axis',(-0.351931111039965,0.0337827344076185,-0.935416067821224));
#89526=DIRECTION('center_axis',(-0.126480538531204,-0.986495981840687,0.104059363754717));
#89527=DIRECTION('ref_axis',(-0.451177899420923,-0.0362134328151596,-0.89169899089203));
#89528=DIRECTION('center_axis',(0.116264754633397,-0.986495109150601,-0.115368567868286));
#89529=DIRECTION('ref_axis',(-0.544789961245158,0.0337827349730038,-0.837891774004402));
#89530=DIRECTION('center_axis',(-0.101153799865448,-0.986495981532177,0.128816098348177));
#89531=DIRECTION('ref_axis',(-0.63231853649629,-0.0362134428581971,-0.773861651045939));
#89532=DIRECTION('center_axis',(0.0887457169003776,-0.986495109151898,-0.137664800698008));
#89533=DIRECTION('ref_axis',(-0.712175035857152,0.0337827361605426,-0.701188594487511));
#89534=DIRECTION('center_axis',(-0.0710972307886002,-0.986495981675317,
0.147549523593419));
#89535=DIRECTION('ref_axis',(-0.783892659372715,-0.0362134382290662,-0.61983940296919));
#89536=DIRECTION('center_axis',(0.0570770288023917,-0.986495109144716,-0.15352397994009));
#89537=DIRECTION('ref_axis',(-0.84625960139423,0.0337827355307125,-0.531698611835822));
#89538=DIRECTION('center_axis',(-0.037716230030684,-0.986495981658015,0.159383701064012));
#89539=DIRECTION('ref_axis',(-0.89881283339374,-0.0362134394467856,-0.436834153117806));
#89540=DIRECTION('center_axis',(0.0227394843068792,-0.98649510919204,-0.162204548005417));
#89541=DIRECTION('ref_axis',(-0.940774006315102,0.033782733441347,-0.337346996374748));
#89542=DIRECTION('center_axis',(-0.00257165909992377,-0.986495981600037,
0.163765273658531));
#89543=DIRECTION('ref_axis',(-0.971705519356601,-0.036213441281663,-0.233403021236782));
#89544=DIRECTION('center_axis',(-0.0126613353093978,-0.986495109225122,
-0.163300612561919));
#89545=DIRECTION('ref_axis',(-0.991298865155135,0.0337827334408555,-0.127221408824948));
#89546=DIRECTION('center_axis',(0.0326931560685295,-0.986495981648445,0.160489363316543));
#89547=DIRECTION('ref_axis',(-0.999162334596164,-0.0362134394397524,-0.0190582246887204));
#89548=DIRECTION('center_axis',(-0.0474701296012096,-0.986495109081729,
-0.156760921640161));
#89549=DIRECTION('ref_axis',(-0.99547169045246,0.0337827378314939,0.0888529129085293));
#89550=DIRECTION('center_axis',(0.0664292714792586,-0.986495981820537,0.149709150497458));
#89551=DIRECTION('ref_axis',(-0.979899429874397,-0.0362134335515134,0.196177711685712));
#89552=DIRECTION('center_axis',(-0.0800592635377692,-0.986495109206595,
-0.142891265769669));
#89553=DIRECTION('ref_axis',(-0.953097367008042,0.0337827328533723,0.300772565177237));
#89554=DIRECTION('center_axis',(0.0970592346613633,-0.986495982026382,0.131928702005114));
#89555=DIRECTION('ref_axis',(-0.914817516009326,-0.0362134347011463,0.402240599081785));
#89556=DIRECTION('center_axis',(-0.108904925617401,-0.986495109062015,-0.122340169090091));
#89557=DIRECTION('ref_axis',(-0.866157268702823,0.0337827385282152,0.498628431249964));
#89558=DIRECTION('center_axis',(0.123150817142994,-0.986495981721548,0.107979416021075));
#89559=DIRECTION('ref_axis',(-0.806959753962968,-0.0362134370030227,0.589495158983052));
#89560=DIRECTION('center_axis',(-0.132658304626744,-0.986495109226923,-0.0960685884403372));
#89561=DIRECTION('ref_axis',(-0.73871662136084,0.0337827326810044,0.673168983463906));
#89562=DIRECTION('center_axis',(0.14348400268928,-0.986495981690008,0.0789811311752993));
#89563=DIRECTION('ref_axis',(-0.661369448832978,-0.0362134378285858,0.749185583864905));
#89564=DIRECTION('center_axis',(-0.150208734751247,-0.986495109188334,-0.0653049427832723));
#89565=DIRECTION('ref_axis',(-0.576734403862306,0.0337827341053085,0.816232904432283));
#89566=DIRECTION('center_axis',(0.157108035070394,-0.98649598169556,0.0462897765692665));
#89567=DIRECTION('ref_axis',(-0.484854242613642,-0.0362134380174296,0.873844923499879));
#89568=DIRECTION('center_axis',(-0.160735569747072,-0.986495109243657,-0.03148771278498));
#89569=DIRECTION('ref_axis',(-0.387784725587891,0.0337827325626061,0.921130682140883));
#89570=DIRECTION('center_axis',(0.163385869707142,-0.986495981745934,0.0114339660295916));
#89571=DIRECTION('ref_axis',(-0.285667791249065,-0.036213435650009,0.957644245072931));
#89572=DIRECTION('center_axis',(-0.163746589113287,-0.986495109212928,0.00380184859480349));
#89573=DIRECTION('ref_axis',(-0.180702665110739,0.0337827324230032,0.982957412003141));
#89574=DIRECTION('center_axis',(0.162023961952625,-0.986495981990144,-0.0239564870228622));
#89575=DIRECTION('ref_axis',(-0.0731238305327095,-0.0362134362190338,0.996665185729608));
#89576=DIRECTION('center_axis',(0.16319774342888,0.986495109427954,0.0139246405501089));
#89577=DIRECTION('ref_axis',(-0.0798755533746233,-0.000856196801981241,
0.996804475762491));
#89578=DIRECTION('center_axis',(0.973816438935882,-0.151617915519108,0.169391708627898));
#89579=DIRECTION('ref_axis',(0.169168347992191,-0.0144665692539132,-0.985480993429916));
#89580=DIRECTION('center_axis',(-0.150208759619426,0.98649511125754,-0.0653048543262073));
#89581=DIRECTION('ref_axis',(-0.191922264154987,0.0357021715627206,0.980760520956737));
#89582=DIRECTION('center_axis',(0.156388881046733,0.986495109575236,0.0486817899126005));
#89583=DIRECTION('ref_axis',(-0.292291612279632,-0.000856205215915049,0.956328855730915));
#89584=DIRECTION('center_axis',(0.914635050695517,-0.151616585406996,0.374773444988745));
#89585=DIRECTION('ref_axis',(0.377062722092037,-0.0144669911495919,-0.926074732284399));
#89586=DIRECTION('center_axis',(-0.132658347021188,0.98649511115752,-0.0960685100744156));
#89587=DIRECTION('ref_axis',(-0.398269746671797,0.0357021763042036,0.916573272299125));
#89588=DIRECTION('center_axis',(0.142267445830776,0.986495109679402,0.0811626295496392));
#89589=DIRECTION('ref_axis',(-0.491040433772505,-0.000856212491145792,0.871136360910667));
#89590=DIRECTION('center_axis',(0.81268611159476,-0.151618552778232,0.562630516835359));
#89591=DIRECTION('ref_axis',(0.567325574073311,-0.0144672535242214,-0.823366498940693));
#89592=DIRECTION('center_axis',(-0.108904975984984,0.986495111019657,-0.122340108468259));
#89593=DIRECTION('ref_axis',(-0.585994582538218,0.0357021804983287,0.809528074586376));
#89594=DIRECTION('center_axis',(0.121493750910025,0.986495109592467,0.109848382964701));
#89595=DIRECTION('ref_axis',(-0.666828746114267,-0.000856205849967259,0.745210500642078));
#89596=DIRECTION('center_axis',(0.672736999254258,-0.151616243451158,0.724180533124259));
#89597=DIRECTION('ref_axis',(0.731061415364102,-0.0144684889231733,-0.682158243953788));
#89598=DIRECTION('center_axis',(-0.0800593355874687,0.98649511117952,-0.142891211780848));
#89599=DIRECTION('ref_axis',(-0.746318960904179,0.0357021749296351,0.664630245550261));
#89600=DIRECTION('center_axis',(0.0950391340827275,0.98649510969273,0.133397756896935));
#89601=DIRECTION('ref_axis',(-0.811436892359336,-0.000856211206739125,0.584439420830417));
#89602=DIRECTION('center_axis',(0.501331437055608,-0.151617256389218,0.851867946212772));
#89603=DIRECTION('ref_axis',(0.860613852619957,-0.0144631736525661,-0.509052662586622));
#89604=DIRECTION('center_axis',(-0.0474702053501761,0.986495111159743,-0.156760885625015));
#89605=DIRECTION('ref_axis',(-0.871746295781278,0.0357021754480533,0.48865504239688));
#89606=DIRECTION('center_axis',(0.0641406006060916,0.986495109654567,0.150709594855518));
#89607=DIRECTION('ref_axis',(-0.918103148144516,-0.000856207867161581,0.396340606392049));
#89608=DIRECTION('center_axis',(0.306484138460259,-0.151617050064071,0.939723226807841));
#89609=DIRECTION('ref_axis',(0.949924348094148,-0.0144650718554515,-0.312144989698896));
#89610=DIRECTION('center_axis',(-0.0126614270578941,0.986495111308531,-0.163300592862446));
#89611=DIRECTION('ref_axis',(-0.95641174064724,0.0357021704228837,0.28983087720119));
#89612=DIRECTION('center_axis',(0.0302429216759704,0.986495109620983,0.160974421515921));
#89613=DIRECTION('ref_axis',(-0.981839921055421,-0.000856207544026785,0.189709346977227));
#89614=DIRECTION('center_axis',(0.0973058256837251,-0.15161590629393,0.983638243078561));
#89615=DIRECTION('ref_axis',(0.994817503161179,-0.0144686949397451,-0.100641901168938));
#89616=DIRECTION('center_axis',(0.0227393955501278,0.986495111215857,-0.162204548139775));
#89617=DIRECTION('ref_axis',(-0.996356436764088,0.0357021755039037,0.077454538815092));
#89618=DIRECTION('center_axis',(-0.00506888908118924,0.986495109651181,
0.163712262820435));
#89619=DIRECTION('ref_axis',(-0.999666951145614,-0.000856213425135731,-0.0257925122042029));
#89620=DIRECTION('center_axis',(-0.11642200968098,-0.151617410714182,0.98155900303047));
#89621=DIRECTION('ref_axis',(0.993194280741403,-0.0144667153514315,0.115567447187813));
#89622=DIRECTION('center_axis',(0.05707694568674,0.986495111122913,-0.153523998129494));
#89623=DIRECTION('ref_axis',(-0.989712613066804,0.035702176775246,-0.138543488154395));
#89624=DIRECTION('center_axis',(-0.0401436782549925,0.986495109645519,0.158795099866574));
#89625=DIRECTION('ref_axis',(-0.970750665684117,-0.000856213207028468,-0.240088342017658));
#89626=DIRECTION('center_axis',(-0.324706330221997,-0.151617247467825,0.933583423901712));
#89627=DIRECTION('ref_axis',(0.945130314425094,-0.0144655603581925,0.326373155020824));
#89628=DIRECTION('center_axis',(0.0887456442119272,0.986495110966998,-0.13766483454979));
#89629=DIRECTION('ref_axis',(-0.936790926669358,0.0357021811528901,-0.348063376371161));
#89630=DIRECTION('center_axis',(-0.0733413910929646,0.986495109609041,0.146452856134646));
#89631=DIRECTION('ref_axis',(-0.896443158535087,-0.000856210127143939,-0.443157906868258));
#89632=DIRECTION('center_axis',(-0.517807853003868,-0.151616633390584,0.841954525996998));
#89633=DIRECTION('ref_axis',(0.852873205617176,-0.0144678116141435,0.52191759652974));
#89634=DIRECTION('center_axis',(0.11626469073227,0.986495110956794,-0.11536861682135));
#89635=DIRECTION('ref_axis',(-0.840065938070627,0.0357021814785561,-0.541308206044569));
#89636=DIRECTION('center_axis',(-0.103109741182452,0.986495109566161,0.12726264210418));
#89637=DIRECTION('ref_axis',(-0.780218965265864,-0.000856204815038207,-0.625505901772941));
#89638=DIRECTION('center_axis',(-0.686697081643996,-0.151616832959728,0.710956717406117));
#89639=DIRECTION('ref_axis',(0.720736642217765,-0.0144674666221049,0.69305799539014));
#89640=DIRECTION('center_axis',(0.138347322440688,0.986495111252765,-0.0876778982862104));
#89641=DIRECTION('ref_axis',(-0.704060402225739,0.0357021718200587,-0.709242063716656));
#89642=DIRECTION('center_axis',(-0.128056801010502,0.986495109612048,0.102121762746588));
#89643=DIRECTION('ref_axis',(-0.627512599215102,-0.000856208303257674,-0.778605936744415));
#89644=DIRECTION('center_axis',(-0.823477034226635,-0.151617428283846,0.546715400864012));
#89645=DIRECTION('ref_axis',(0.554899244324145,-0.0144667771566563,0.831791765411989));
#89646=DIRECTION('center_axis',(0.153960995333326,0.986495111267986,-0.0558874526198495));
#89647=DIRECTION('ref_axis',(-0.535133782798231,0.0357021721389029,-0.844012552876212));
#89648=DIRECTION('center_axis',(-0.147016065904781,0.986495109664312,0.0722057821388122));
#89649=DIRECTION('ref_axis',(-0.445464441648733,-0.000856212141019005,-0.895299222677732));
#89650=DIRECTION('center_axis',(-0.921752483970463,-0.151616266908719,0.356910165031687));
#89651=DIRECTION('ref_axis',(0.363115154710566,-0.014466659431284,0.931631955325933));
#89652=DIRECTION('center_axis',(0.162375622483093,0.986495111326117,-0.0214837741772698));
#89653=DIRECTION('ref_axis',(-0.341184903466239,0.0357021701338604,-0.939317952928861));
#89654=DIRECTION('center_axis',(-0.159101021164541,0.986495109713174,0.0389135397566582));
#89655=DIRECTION('ref_axis',(-0.24258685993834,-0.000856214665175483,-0.970129312144367));
#89656=DIRECTION('center_axis',(-0.976927465576519,-0.151616791789489,0.150416340367998));
#89657=DIRECTION('ref_axis',(0.154352777054545,-0.0144685980696197,0.987909854129135));
#89658=DIRECTION('center_axis',(0.163197748067908,0.986495111005709,0.0139244744028963));
#89659=DIRECTION('ref_axis',(-0.131282594828393,0.0357021809331137,-0.990701889859782));
#89660=DIRECTION('center_axis',(-0.163746588668221,0.986495109665289,0.0038017503851117));
#89661=DIRECTION('ref_axis',(-0.0283661934961215,-0.00085621129693069,-0.999597231873296));
#89662=DIRECTION('center_axis',(-0.986422439235276,-0.151617296518004,-0.0631107500327789));
#89663=DIRECTION('ref_axis',(0.061627591074778,0.0144662562400417,-0.997994372453431));
#89664=DIRECTION('center_axis',(0.156388925054473,0.986495110977037,0.0486816201323364));
#89665=DIRECTION('ref_axis',(0.0847583428158461,0.0357021810443611,-0.995761707233105));
#89666=DIRECTION('center_axis',(-0.160735548481539,0.986495109636285,-0.0314878090383231));
#89667=DIRECTION('ref_axis',(0.18718084923227,-0.000856211651976638,-0.982325097196592));
#89668=DIRECTION('center_axis',(-0.949793410970233,-0.15161801438972,-0.273686781175212));
#89669=DIRECTION('ref_axis',(0.274726623805539,0.0144617426827047,-0.961413615553155));
#89670=DIRECTION('center_axis',(0.142267532453734,0.986495111258958,0.081162458511939));
#89671=DIRECTION('ref_axis',(0.296836072343588,0.0357021720284353,-0.954260813964445));
#89672=DIRECTION('center_axis',(-0.150208694038284,0.98649510964934,-0.0653050294636678));
#89673=DIRECTION('ref_axis',(0.393975523838057,-0.000856207535000212,-0.919120532642583));
#89674=DIRECTION('center_axis',(-0.86875330672716,-0.151616186464143,-0.471466037008706));
#89675=DIRECTION('ref_axis',(0.474978502938863,0.0144685084660171,-0.879878448428375));
#89676=DIRECTION('center_axis',(0.121493865171389,0.986495111116108,0.1098482429069));
#89677=DIRECTION('ref_axis',(0.495034075137913,0.0357021764711176,-0.86813974626645));
#89678=DIRECTION('center_axis',(-0.132658243309647,0.986495109701154,-0.0960686682415635));
#89679=DIRECTION('ref_axis',(0.5823483421027,-0.000856213693593766,-0.812938912433368));
#89680=DIRECTION('center_axis',(-0.747091071425321,-0.15161663426736,-0.647199603839499));
#89681=DIRECTION('ref_axis',(0.653021700873013,0.0144674351368952,-0.75720099809065));
#89682=DIRECTION('center_axis',(0.0950392811829329,0.986495111174896,0.133397641134548));
#89683=DIRECTION('ref_axis',(0.67008483719993,0.0357021758568535,-0.741425428208279));
#89684=DIRECTION('center_axis',(-0.108904843685435,0.986495109715039,-0.122340236758661));
#89685=DIRECTION('ref_axis',(0.743491198027751,-0.000856213060135157,-0.668745172210204));
#89686=DIRECTION('center_axis',(-0.590495723145099,-0.15161685077541,-0.792670884736089));
#89687=DIRECTION('ref_axis',(0.800530337746882,0.0144663375264769,-0.599117604002281));
#89688=DIRECTION('center_axis',(0.064140767632109,0.986495111200935,0.150709513648669));
#89689=DIRECTION('ref_axis',(0.813803175955572,0.0357021742051885,-0.5800428825196));
#89690=DIRECTION('center_axis',(-0.080059177130819,0.986495109654734,-0.14289131108794));
#89691=DIRECTION('ref_axis',(0.869869229684662,-0.000856210562327918,-0.493281653978015));
#89692=DIRECTION('center_axis',(-0.406289357632402,-0.151615763752866,-0.901078031058512));
#89693=DIRECTION('ref_axis',(0.910606840740203,0.0144689391276382,-0.413020376492091));
#89694=DIRECTION('center_axis',(0.0302430998549555,0.986495111138554,0.160974378740519));
#89695=DIRECTION('ref_axis',(0.919468984642088,0.0357021757538406,-0.3915381730147));
#89696=DIRECTION('center_axis',(-0.0474700325199218,0.986495109610278,-0.156760947711994));
#89697=DIRECTION('ref_axis',(0.955573144978911,-0.0008562078867857,-0.294752831204668));
#89698=DIRECTION('center_axis',(-0.203085546924405,-0.151616938372349,-0.967351313964586));
#89699=DIRECTION('ref_axis',(0.978104545608466,0.0144676709904371,-0.20761065569033));
#89700=DIRECTION('center_axis',(-0.00506870252952517,0.986495111106572,
0.1637122598265));
#89701=DIRECTION('ref_axis',(0.982141444060542,0.035702178222545,-0.184725575730159));
#89702=DIRECTION('center_axis',(-0.0126612356724127,0.986495109661314,-0.16330061765211));
#89703=DIRECTION('ref_axis',(0.996595521728744,-0.000856211888700642,-0.0824416943749574));
#89704=DIRECTION('center_axis',(0.00961444697794412,-0.151616752732667,
-0.988392595429625));
#89705=DIRECTION('ref_axis',(0.99986717095386,0.0144667495042641,0.00750690398936496));
#89706=DIRECTION('center_axis',(-0.0401434933614616,0.986495111113504,0.158795137488191));
#89707=DIRECTION('ref_axis',(0.998890061332806,0.0357021761084332,0.0307245828558428));
#89708=DIRECTION('center_axis',(0.0227395785448257,0.986495109616514,-0.162204532212591));
#89709=DIRECTION('ref_axis',(0.991018199734975,-0.000856207842489773,0.133724323524857));
#89710=DIRECTION('center_axis',(0.221864784232945,-0.151617150572385,-0.963217658252578));
#89711=DIRECTION('ref_axis',(0.974877146343857,0.0144698250946434,0.222272746188522));
#89712=DIRECTION('center_axis',(-0.0733412205126192,0.986495111186581,0.146452930932413));
#89713=DIRECTION('ref_axis',(0.968931689381041,0.0357021750131451,0.244738096773943));
#89714=DIRECTION('center_axis',(0.0570771171246619,0.986495109600125,-0.153523944177369));
#89715=DIRECTION('ref_axis',(0.939101967721057,-0.000856204949422194,0.343637543256733));
#89716=DIRECTION('center_axis',(0.423741222458399,-0.15161624686651,-0.893003857816737));
#89717=DIRECTION('ref_axis',(0.904302870344119,0.0144688320150039,0.426646190171093));
#89718=DIRECTION('center_axis',(-0.103109596719155,0.986495111163184,0.127262746770411));
#89719=DIRECTION('ref_axis',(0.893667149003531,0.0357021778745687,0.447307926698055));
#89720=DIRECTION('center_axis',(0.0887457984091327,0.986495109631058,-0.137664744719671));
#89721=DIRECTION('ref_axis',(0.843274370259044,-0.000856207903572526,0.537482654019867));
#89722=DIRECTION('center_axis',(0.605803742148127,-0.151616591887001,-0.781034080603335));
#89723=DIRECTION('ref_axis',(0.791444387993897,0.014467573311151,0.611069938743063));
#89724=DIRECTION('center_axis',(-0.12805668263688,0.986495111047565,0.102121897315367));
#89725=DIRECTION('ref_axis',(0.776615725781708,0.0357021808280826,0.628962136183625));
#89726=DIRECTION('center_axis',(0.116264825596677,0.986495109676501,-0.115368491856844));
#89727=DIRECTION('ref_axis',(0.70801620387057,-0.000856214333401109,0.706195668319852));
#89728=DIRECTION('center_axis',(0.759539707374844,-0.151616246287053,-0.632544027544929));
#89729=DIRECTION('ref_axis',(0.641578860804063,0.0144678318516811,0.766920626408543));
#89730=DIRECTION('center_axis',(-0.147015974594736,0.986495111199057,0.0722059470841616));
#89731=DIRECTION('ref_axis',(0.623250614101209,0.0357021752331852,0.781206775896167));
#89732=DIRECTION('center_axis',(0.138347432562809,0.986495109665889,-0.0876777423783469));
#89733=DIRECTION('ref_axis',(0.539651981929142,-0.000856210824512759,0.841887762889432));
#89734=DIRECTION('center_axis',(0.877760395337333,-0.151616069138643,-0.454476903655395));
#89735=DIRECTION('ref_axis',(0.461713547141786,0.0144657771560889,0.88691112388842));
#89736=DIRECTION('center_axis',(-0.159100969104174,0.986495111013716,0.0389137196390765));
#89737=DIRECTION('ref_axis',(0.440742995292145,0.0357021793475845,0.89692305494437));
#89738=DIRECTION('center_axis',(0.153961068617493,0.986495109630638,-0.0558872796349529));
#89739=DIRECTION('ref_axis',(0.346054238115806,-0.000856208532924168,0.938214117986421));
#89740=DIRECTION('center_axis',(0.954937805615096,-0.151616804017654,-0.255159033048994));
#89741=DIRECTION('ref_axis',(0.260259650356053,0.0144675620557106,0.965430268867052));
#89742=DIRECTION('center_axis',(-0.163746575713377,0.986495111104787,0.00380193483594564));
#89743=DIRECTION('ref_axis',(0.237626725609359,0.0357021776226121,0.970700207988634));
#89744=DIRECTION('center_axis',(0.162375657399043,0.986495109627207,-0.0214835882904524));
#89745=DIRECTION('ref_axis',(0.136275379499101,-0.000856207475975685,0.990670625309509));
#89746=DIRECTION('center_axis',(0.987463458080041,-0.151617315741383,-0.0439102325658274));
#89747=DIRECTION('ref_axis',(-0.0466361827048427,-0.0144684783683654,-0.998807153356655));
#89748=DIRECTION('center_axis',(-0.160735575477852,0.986495110602581,-0.0314876409564998));
#89749=DIRECTION('ref_axis',(0.0233992914794688,0.0357021926497558,0.999088497881073));
#89750=DIRECTION('center_axis',(0.155084985271922,0.987363722734215,-0.0325810738257533));
#89751=DIRECTION('ref_axis',(0.107082710721225,0.0159846151395328,0.994121614865825));
#89752=DIRECTION('',(-0.603474775605395,0.,0.797382088592425));
#89753=DIRECTION('center_axis',(-0.146198072099652,0.987366228112447,0.0611069169353534));
#89754=DIRECTION('ref_axis',(0.247230525195829,-0.0233430562761571,0.968675471525465));
#89755=DIRECTION('',(-0.797382090536838,0.,-0.603474773036207));
#89756=DIRECTION('center_axis',(1.80679789905059E-15,-1.,7.19968963237278E-15));
#89757=DIRECTION('ref_axis',(1.06096449896609E-33,-7.19968963237278E-15,
-1.));
#89758=DIRECTION('center_axis',(-0.152615518807593,-0.987363722561521,0.042677661469956));
#89759=DIRECTION('ref_axis',(0.172020652255709,0.0159849136234662,0.984963642848796));
#89760=DIRECTION('center_axis',(0.157698499589188,-0.987363722825346,-0.0156224862231631));
#89761=DIRECTION('ref_axis',(0.239264796343388,0.0228559962932019,0.970685304650381));
#89762=DIRECTION('center_axis',(0.144455217640186,0.987363722794169,-0.0651580310212521));
#89763=DIRECTION('ref_axis',(0.318285939670239,0.0159846116596834,0.947859985862006));
#89764=DIRECTION('',(-0.417952293183597,0.,0.908468976147547));
#89765=DIRECTION('center_axis',(-0.129643867607601,0.987366228493109,0.0911065223956936));
#89766=DIRECTION('ref_axis',(0.449687003600112,-0.0233430424028127,0.892881123758663));
#89767=DIRECTION('',(-0.908468978721806,0.,-0.41795228758814));
#89768=DIRECTION('center_axis',(-3.31227642057055E-15,-1.,-6.64295675440539E-15));
#89769=DIRECTION('ref_axis',(-2.25783646485001E-32,6.64295675440539E-15,
-1.));
#89770=DIRECTION('center_axis',(-0.139873017737398,-0.987363722559547,0.074487705578756));
#89771=DIRECTION('ref_axis',(0.379736972377725,0.0159849124034919,0.924956385125727));
#89772=DIRECTION('center_axis',(0.150653221823371,-0.987363722937459,-0.0491577601332619));
#89773=DIRECTION('ref_axis',(0.442339566449922,0.0228559928591386,0.896556362725355));
#89774=DIRECTION('center_axis',(0.127070885021152,0.987363722838332,-0.0946882727837558));
#89775=DIRECTION('ref_axis',(0.514606469984781,0.0159846100172811,0.857277477420466));
#89776=DIRECTION('',(-0.212886825056998,0.,0.977076864794757));
#89777=DIRECTION('center_axis',(-0.107027651167834,0.987366228258172,0.116846108966996));
#89778=DIRECTION('ref_axis',(0.631116620567509,-0.0233430513871423,0.775336645074502));
#89779=DIRECTION('',(-0.977076865850031,0.,-0.212886820213656));
#89780=DIRECTION('center_axis',(-4.66287657085733E-15,-1.,-5.77560659059213E-15));
#89781=DIRECTION('ref_axis',(-3.17308563966652E-32,5.77560659059213E-15,
-1.));
#89782=DIRECTION('center_axis',(-0.120590206990325,-0.987363722543746,0.102814791652694));
#89783=DIRECTION('ref_axis',(0.569697214377223,0.0159849163266524,0.821699194584528));
#89784=DIRECTION('center_axis',(0.136563569902727,-0.987363722841019,-0.0803944661836044));
#89785=DIRECTION('ref_axis',(0.624731028720287,0.0228559958350036,0.780505442138928));
#89786=DIRECTION('center_axis',(0.103744859203304,0.987363722854479,-0.119790997073363));
#89787=DIRECTION('ref_axis',(0.686864572632723,0.0159846093646422,0.726609627740733));
#89788=DIRECTION('',(0.00213299544959006,0.,0.999997725162619));
#89789=DIRECTION('center_axis',(-0.0794069421389742,0.987366228166386,0.137122095289646));
#89790=DIRECTION('ref_axis',(0.783035924871884,-0.0233430546583344,0.621538286961673));
#89791=DIRECTION('',(-0.999997725152042,0.,0.00213300040793875));
#89792=DIRECTION('center_axis',(0.,-1.,0.));
#89793=DIRECTION('ref_axis',(0.,0.,-1.));
#89794=DIRECTION('center_axis',(-0.0956687346801696,-0.987363722549481,
0.126334368237338));
#89795=DIRECTION('ref_axis',(0.733019047310366,0.0159849154507234,0.680020263490902));
#89796=DIRECTION('center_axis',(0.116088355865392,-0.987363722833826,-0.107872018912213));
#89797=DIRECTION('ref_axis',(0.777910762482154,0.0228559958636816,0.627958954922623));
#89798=DIRECTION('center_axis',(0.0755678354376402,0.987363722748056,-0.139292430693023));
#89799=DIRECTION('ref_axis',(0.827005651956269,0.0159846135455113,0.561966319063863));
#89800=DIRECTION('',(0.217053076899228,0.,0.976159803417749));
#89801=DIRECTION('center_axis',(-0.0480732588543953,0.987366228278341,0.15098640017737));
#89802=DIRECTION('ref_axis',(0.898341339026026,-0.0233430501545939,0.438677490425948));
#89803=DIRECTION('',(-0.976159801597278,-3.11688536720188E-15,0.217053085086487));
#89804=DIRECTION('center_axis',(-2.66281056931374E-14,-1.,-1.31356300836969E-14));
#89805=DIRECTION('ref_axis',(1.,-2.66281056931374E-14,-1.31798834488888E-33));
#89806=DIRECTION('center_axis',(-0.0662738964320985,-0.987363722501457,
0.143946692007056));
#89807=DIRECTION('ref_axis',(0.862065724724343,0.0159849174326958,0.506544340280457));
#89808=DIRECTION('center_axis',(0.0901849798542257,-0.987363722846656,-0.130305595486476));
#89809=DIRECTION('ref_axis',(0.894716254152115,0.0228559966907545,0.44604980436189));
#89810=DIRECTION('center_axis',(0.0438573488328245,0.98736372284281,-0.152280700574112));
#89811=DIRECTION('ref_axis',(0.928476866871779,0.0159846104613722,0.371046088663339));
#89812=DIRECTION('',(0.421824000481475,0.,0.906677733606492));
#89813=DIRECTION('center_axis',(-0.0144917194007374,0.987366228279528,0.157790751699423));
#89814=DIRECTION('ref_axis',(0.971641310970371,-0.0233430506088162,0.2353046212977));
#89815=DIRECTION('',(-0.90667773151446,0.,0.421824004978135));
#89816=DIRECTION('center_axis',(-1.44146637799513E-14,-1.,-3.55213537512284E-15));
#89817=DIRECTION('ref_axis',(1.,-1.44146637799513E-14,4.42351985979486E-32));
#89818=DIRECTION('center_axis',(-0.0337801645495731,-0.987363722504886,
0.154828227285267));
#89819=DIRECTION('ref_axis',(0.950803166929402,0.0159849187336526,0.309382966774351));
#89820=DIRECTION('center_axis',(0.0600646558957432,-0.987363722771998,-0.146646227588527));
#89821=DIRECTION('ref_axis',(0.96968580795722,0.0228559986227534,0.243283861308783));
#89822=DIRECTION('center_axis',(0.0100961397987127,0.987363722827371,-0.158148496058732));
#89823=DIRECTION('ref_axis',(0.986533534493181,0.015984610039757,0.162776157843428));
#89824=DIRECTION('',(0.606870901804627,0.,0.794800420572888));
#89825=DIRECTION('',(-0.794800418951332,0.,0.606870903928329));
#89826=DIRECTION('',(0.763541191686738,0.,0.645759125833771));
#89827=DIRECTION('center_axis',(0.0531022914963808,0.987366228202565,0.14929192222915));
#89828=DIRECTION('ref_axis',(0.980639616445277,-0.0233430534609367,-0.194424907131723));
#89829=DIRECTION('',(-0.645759120372939,0.,0.763541196305195));
#89830=DIRECTION('center_axis',(2.91477949412441E-14,-1.,-5.65745894309366E-15));
#89831=DIRECTION('ref_axis',(1.,2.91477949412441E-14,2.51222001147484E-32));
#89832=DIRECTION('center_axis',(0.0343526394915633,-0.987363722496745,0.154702216071179));
#89833=DIRECTION('ref_axis',(0.99283211913855,0.0159849199594086,-0.118443512024708));
#89834=DIRECTION('center_axis',(-0.00706194962898739,-0.987363722828293,
-0.158313005498892));
#89835=DIRECTION('ref_axis',(0.982215246104916,0.0228559963878828,-0.186362050182373));
#89836=DIRECTION('center_axis',(-0.0572418275962692,0.987363722673098,-0.147770945461416));
#89837=DIRECTION('ref_axis',(0.963701520646536,0.0159846159200898,-0.266503041553829));
#89838=DIRECTION('',(0.884509147436183,0.,0.466522848424079));
#89839=DIRECTION('center_axis',(0.0839541446999537,0.987366228048496,0.134386135062308));
#89840=DIRECTION('ref_axis',(0.915917198838005,-0.0233430588070783,-0.400687891604266));
#89841=DIRECTION('',(-0.466522844039702,0.,0.884509149748666));
#89842=DIRECTION('center_axis',(-1.36250746154898E-14,-1.,5.8955524984798E-15));
#89843=DIRECTION('ref_axis',(1.,-1.36250746154898E-14,4.41891060473253E-32));
#89844=DIRECTION('center_axis',(0.0668058915450112,-0.987363722561284,0.1437005644554));
#89845=DIRECTION('ref_axis',(0.944158402242533,0.0159849137173079,-0.329103925847561));
#89846=DIRECTION('center_axis',(-0.0409294619246427,-0.987363722825878,
-0.153093624929265));
#89847=DIRECTION('ref_axis',(0.91918926717849,0.0228559962494711,-0.393152253636317));
#89848=DIRECTION('center_axis',(-0.087669925550576,0.987363722823561,-0.132010844274079));
#89849=DIRECTION('ref_axis',(0.883880438918321,0.0159846103812733,-0.467439688011742));
#89850=DIRECTION('',(0.964118437085268,0.,0.265472483079246));
#89851=DIRECTION('center_axis',(0.110880384200007,0.987366228253681,0.113196606414501));
#89852=DIRECTION('ref_axis',(0.808367512052446,-0.0233430518259719,-0.588215153995193));
#89853=DIRECTION('',(-0.265472477562517,0.,0.964118438604313));
#89854=DIRECTION('center_axis',(2.40783168675084E-14,-1.,-1.73734121004002E-14));
#89855=DIRECTION('ref_axis',(1.,2.40783168675084E-14,-9.42922941613875E-32));
#89856=DIRECTION('center_axis',(0.0961353783624827,-0.987363722591995,0.125979634609644));
#89857=DIRECTION('ref_axis',(0.851336887325996,0.0159849109908428,-0.524375806934968));
#89858=DIRECTION('center_axis',(-0.0728831555135252,-0.987363722760217,
-0.140715758248592));
#89859=DIRECTION('ref_axis',(0.813183020583973,0.022855998889668,-0.581559092740093));
#89860=DIRECTION('center_axis',(-0.113998684177927,0.987363722714032,-0.11007805900355));
#89861=DIRECTION('ref_axis',(0.762730088964751,0.0159846145330615,-0.646519375955627));
#89862=DIRECTION('',(0.998646620316722,0.,0.0520089197156425));
#89863=DIRECTION('center_axis',(0.132621977585668,0.987366228627553,0.0867141374117852));
#89864=DIRECTION('ref_axis',(0.663019460029588,-0.0233430386172312,-0.748238129321266));
#89865=DIRECTION('',(-0.0520089118984696,0.,0.998646620723836));
#89866=DIRECTION('center_axis',(2.47257614362469E-14,-1.,-2.76791971940485E-14));
#89867=DIRECTION('ref_axis',(-2.56103310374099E-31,2.76791971940485E-14,
-1.));
#89868=DIRECTION('center_axis',(0.120969685022707,-0.987363722555055,0.102368035478518));
#89869=DIRECTION('ref_axis',(0.718707806582739,0.015984912252531,-0.695128456716675));
#89870=DIRECTION('center_axis',(-0.101428918117671,-0.987363722837366,-0.12175817588243));
#89871=DIRECTION('ref_axis',(0.669153238850915,0.0228559961940831,-0.742772876708154));
#89872=DIRECTION('center_axis',(-0.134996984321599,0.98736372281309,-0.0829981511646479));
#89873=DIRECTION('ref_axis',(0.605915329882612,0.0159846104207681,-0.795368534229851));
#89874=DIRECTION('',(0.986479197453235,0.,-0.163886524742036));
#89875=DIRECTION('center_axis',(0.148162328874504,0.987366228449234,0.0561769990335785));
#89876=DIRECTION('ref_axis',(0.486669352553433,-0.0233430445479536,-0.873274323197731));
#89877=DIRECTION('',(0.163886529632327,0.,0.986479196640797));
#89878=DIRECTION('center_axis',(3.63949553544791E-15,-1.,-6.46947615618595E-15));
#89879=DIRECTION('ref_axis',(2.4838904804171E-32,6.46947615618595E-15,-1.));
#89880=DIRECTION('center_axis',(0.140147584032476,-0.987363722542777,0.0739698188204495));
#89881=DIRECTION('ref_axis',(0.552472745197975,0.0159849147106998,-0.833377674476047));
#89882=DIRECTION('center_axis',(-0.125231975789276,-0.987363722872431,-0.0971073168994375));
#89883=DIRECTION('ref_axis',(0.493834594623234,0.0228559948635626,-0.869255426587665));
#89884=DIRECTION('center_axis',(-0.149682979297111,0.987363722804785,-0.0520373384966535));
#89885=DIRECTION('ref_axis',(0.420768643212658,0.0159846115427924,-0.907027144622918));
#89886=DIRECTION('',(0.928185103589142,0.,-0.372118816341251));
#89887=DIRECTION('center_axis',(0.15677476827983,0.987366228614418,0.0230130967613378));
#89888=DIRECTION('ref_axis',(0.287563128866355,-0.0233430385249353,-0.957477179607439));
#89889=DIRECTION('',(0.372118820942155,0.,0.928185101744593));
#89890=DIRECTION('center_axis',(-1.73092801110785E-14,-1.,5.68048588195008E-14));
#89891=DIRECTION('ref_axis',(1.26963893944953E-31,-5.68048588195008E-14,
-1.));
#89892=DIRECTION('center_axis',(0.152772335842607,-0.987363722537882,0.04211285809975));
#89893=DIRECTION('ref_axis',(0.360404675471254,0.0159849146053789,-0.932659076192109));
#89894=DIRECTION('center_axis',(-0.143179323934672,-0.987363722859305,-0.0679158301062707));
#89895=DIRECTION('ref_axis',(0.29542479569763,0.0228559960548419,-0.955092557573011));
#89896=DIRECTION('center_axis',(-0.157369964369956,0.987363722781334,-0.018643316485656));
#89897=DIRECTION('ref_axis',(0.215947280176704,0.0159846133760726,-0.976274174768288));
#89898=DIRECTION('',(0.826490105990571,0.,-0.562951245402029));
#89899=DIRECTION('center_axis',(0.158056597898232,0.987366228339418,-0.0112268871744602));
#89900=DIRECTION('ref_axis',(0.0750107703523085,-0.0233430480212223,-0.996909467524626));
#89901=DIRECTION('',(0.562951250126444,0.,0.826490102772607));
#89902=DIRECTION('center_axis',(-5.866541577634E-16,-1.,7.39972205357027E-15));
#89903=DIRECTION('ref_axis',(1.03531391909646E-33,-7.39972205357027E-15,
-1.));
#89904=DIRECTION('center_axis',(0.158253623048332,-0.987363722546709,0.00828674790145633));
#89905=DIRECTION('ref_axis',(0.1514844822469,0.0159849132724407,-0.988330377043052));
#89906=DIRECTION('center_axis',(-0.154431767114578,-0.987363722967648,-0.0355486690796414));
#89907=DIRECTION('ref_axis',(0.0832012598696812,0.0228559917419084,-0.996270622871914));
#89908=DIRECTION('center_axis',(-0.157698504332179,0.987363722731131,0.0156224443002877));
#89909=DIRECTION('ref_axis',(0.0010284646078306,0.0159846134183868,-0.999871708967913));
#89910=DIRECTION('',(0.686149350632658,0.,-0.727460699025302));
#89911=DIRECTION('center_axis',(0.151947872945319,0.987366228211681,-0.0449419102223341));
#89912=DIRECTION('ref_axis',(-0.141049007625289,-0.0233430530033732,-0.98972737626298));
#89913=DIRECTION('',(0.727460703861421,0.,0.686149345505369));
#89914=DIRECTION('center_axis',(-4.07113198674605E-15,-1.,-2.94113358440815E-14));
#89915=DIRECTION('ref_axis',(3.16446087767206E-32,2.94113358440815E-14,
-1.));
#89916=DIRECTION('center_axis',(0.156335146712011,-0.987363722543461,-0.0259268453085564));
#89917=DIRECTION('ref_axis',(-0.0645189579561007,0.0159849158098743,-0.997788447783803));
#89918=DIRECTION('center_axis',(-0.158463151597848,-0.987363722911652,-0.00151929711410159));
#89919=DIRECTION('ref_axis',(-0.132912675267693,0.0228559931629575,-0.990864180566499));
#89920=DIRECTION('center_axis',(-0.150653237015209,0.98736372274595,0.0491577174215569));
#89921=DIRECTION('ref_axis',(-0.213938443152542,0.0159846135185208,-0.976716353232672));
#89922=DIRECTION('',(0.513725012558988,0.,-0.857954900604495));
#89923=DIRECTION('center_axis',(0.13873423522595,0.987366228330945,-0.0765554905137078));
#89924=DIRECTION('ref_axis',(-0.350513489393465,-0.0233430488791305,-0.936266733266885));
#89925=DIRECTION('',(0.85795490315098,0.,0.513725008306187));
#89926=DIRECTION('center_axis',(-2.57462974808217E-15,-1.,-6.96213552645962E-15));
#89927=DIRECTION('ref_axis',(-1.45992716183616E-32,6.96213552645962E-15,
-1.));
#89928=DIRECTION('center_axis',(0.147106613134323,-0.987363722546931,-0.0589281237646008));
#89929=DIRECTION('ref_axis',(-0.277505562222682,0.0159849140967657,-0.960591039650481));
#89930=DIRECTION('center_axis',(-0.155084976578354,-0.987363722815579,0.0325811127411562));
#89931=DIRECTION('ref_axis',(-0.342811757964815,0.0228559970767686,-0.939126030945101));
#89932=DIRECTION('center_axis',(-0.136563593350173,0.987363722837714,0.0803944263947326));
#89933=DIRECTION('ref_axis',(-0.418901823414549,0.0159846099984002,-0.907890827458437));
#89934=DIRECTION('',(0.317279463900984,0.,-0.948332084128078));
#89935=DIRECTION('center_axis',(0.119033538070446,0.987366228337816,-0.104589425624143));
#89936=DIRECTION('ref_axis',(-0.543588350657022,-0.0233430493212615,-0.839027298172332));
#89937=DIRECTION('',(0.94833208570079,0.,0.317279459200228));
#89938=DIRECTION('center_axis',(-2.00554483640518E-14,-1.,-3.12294768742199E-14));
#89939=DIRECTION('ref_axis',(8.93331168178509E-32,3.12294768742199E-14,
-1.));
#89940=DIRECTION('center_axis',(0.130999534218378,-0.987363722518234,-0.0891739955901007));
#89941=DIRECTION('ref_axis',(-0.477516315597614,0.0159849202558936,-0.878477461670186));
#89942=DIRECTION('center_axis',(-0.144455198836582,-0.987363722863686,0.065158071655359));
#89943=DIRECTION('ref_axis',(-0.53668134664747,0.0228559953510044,-0.843475391245751));
#89944=DIRECTION('center_axis',(-0.116088384632717,0.9873637227041,0.107871989141148));
#89945=DIRECTION('ref_axis',(-0.604277824084843,0.0159846144351275,-0.796613333694992));
#89946=DIRECTION('',(0.105998282549184,0.,-0.994366312832763));
#89947=DIRECTION('center_axis',(0.0937668866521125,0.987366224079759,-0.127732965651197));
#89948=DIRECTION('ref_axis',(-0.711245635399542,-0.0233431675720497,-0.702555864435566));
#89949=DIRECTION('',(0.994366313661193,0.,0.105998274777704));
#89950=DIRECTION('center_axis',(-0.0901851111012612,0.987363726530036,0.130305476739748));
#89951=DIRECTION('ref_axis',(-0.761398490165991,0.0159844698817519,-0.648087058886034));
#89952=DIRECTION('',(-0.110239262352301,0.,-0.993905078483866));
#89953=DIRECTION('center_axis',(0.,-1.,0.));
#89954=DIRECTION('ref_axis',(0.,0.,-1.));
#89955=DIRECTION('center_axis',(0.108767068287796,-0.987363722515168,-0.115250181418807));
#89956=DIRECTION('ref_axis',(-0.655198934415205,0.0159849158473419,-0.755287255821606));
#89957=DIRECTION('center_axis',(-0.127070814589076,-0.987363725701319,0.0946883374491268));
#89958=DIRECTION('ref_axis',(-0.705456317279217,0.0228559462351422,-0.708384775480488));
#89959=DIRECTION('',(0.993905077902487,0.,-0.110239267593957));
#89960=DIRECTION('center_axis',(0.0641159492092076,0.987366228179104,-0.144903680106382));
#89961=DIRECTION('ref_axis',(-0.845645844217114,-0.0233430542732531,-0.533233727342448));
#89962=DIRECTION('center_axis',(-1.87888493708443E-14,-1.,-1.19532248295311E-14));
#89963=DIRECTION('ref_axis',(1.,-1.87888493708443E-14,4.76728741383965E-32));
#89964=DIRECTION('center_axis',(-0.0600646941590119,0.98736372279682,0.146646211749191));
#89965=DIRECTION('ref_axis',(-0.882916956320006,0.0159846117320783,-0.469257008930492));
#89966=DIRECTION('center_axis',(0.0814487732550144,-0.987363722548193,-0.135937400045126));
#89967=DIRECTION('ref_axis',(-0.802245181914049,0.0159849145847606,-0.596780655351204));
#89968=DIRECTION('center_axis',(-0.103744825459418,-0.987363722817008,0.119791026606059));
#89969=DIRECTION('ref_axis',(-0.841244922299314,0.0228559975989328,-0.540170884146285));
#89970=DIRECTION('',(-0.321322141912006,0.,-0.946969947314634));
#89971=DIRECTION('center_axis',(0.0314669536807221,0.98736622841628,-0.155298943361071));
#89972=DIRECTION('ref_axis',(-0.940504603145758,-0.0233430461605324,-0.338978161033402));
#89973=DIRECTION('',(0.946969945721879,0.,-0.321322146606022));
#89974=DIRECTION('center_axis',(4.18383330129325E-14,-1.,1.52694357023645E-14));
#89975=DIRECTION('ref_axis',(1.,4.18383330129325E-14,-3.94743002442807E-32));
#89976=DIRECTION('center_axis',(0.0503220214576929,-0.987363722544967,-0.15026833851));
#89977=DIRECTION('ref_axis',(-0.911779336272946,0.0159849164455385,-0.410369253711697));
#89978=DIRECTION('center_axis',(-0.0755677933538741,-0.987363722995076,
0.139292451772985));
#89979=DIRECTION('ref_axis',(-0.937697856654406,0.0228559913020375,-0.346699197125309));
#89980=DIRECTION('center_axis',(-0.0271358127651529,0.987363722766446,0.156129839013432));
#89981=DIRECTION('ref_axis',(-0.963151234653621,0.0159846131294028,-0.268484992743187));
#89982=DIRECTION('',(-0.517380356258675,0.,-0.85575555327304));
#89983=DIRECTION('center_axis',(-0.00265341486369742,0.987366228230536,
-0.158432606301121));
#89984=DIRECTION('ref_axis',(-0.991386412655018,-0.0233430525964717,-0.128872350403382));
#89985=DIRECTION('',(0.855755550708218,0.,-0.517380360500933));
#89986=DIRECTION('center_axis',(-7.35710890037785E-15,-1.,-9.86406654151451E-16));
#89987=DIRECTION('ref_axis',(1.,-7.35710890037785E-15,-1.32634067597866E-32));
#89988=DIRECTION('center_axis',(0.0168422667212721,-0.987363722512522,-0.157572895886017));
#89989=DIRECTION('ref_axis',(-0.97867970097764,0.0159849196179625,-0.204769444105129));
#89990=DIRECTION('center_axis',(-0.0438573043102228,-0.987363722881878,
0.152280713143452));
#89991=DIRECTION('ref_axis',(-0.99030508060059,0.0228559947707262,-0.137016242977614));
#89992=DIRECTION('center_axis',(0.00706190712797093,0.987363722756913,0.15831300783993));
#89993=DIRECTION('ref_axis',(-0.998349631045912,0.0159846127507674,-0.055158919004085));
#89994=DIRECTION('',(-0.689246440251492,0.,-0.724526979898366));
#89995=DIRECTION('center_axis',(-0.0366497041828464,0.987366228300195,-0.154158134380116));
#89996=DIRECTION('ref_axis',(-0.995912095239017,-0.0233430501912213,0.0872593866836232));
#89997=DIRECTION('',(0.72452697791723,0.,-0.689246442334036));
#89998=DIRECTION('center_axis',(1.47943040872764E-14,-1.,-1.23643184723331E-15));
#89999=DIRECTION('ref_axis',(1.,1.47943040872764E-14,-1.07193378809406E-32));
#90000=DIRECTION('center_axis',(-0.0174250066718511,-0.987363722557856,
-0.157509518820862));
#90001=DIRECTION('ref_axis',(-0.999818091054278,0.0159849156030328,0.0104051561133797));
#90002=DIRECTION('center_axis',(-0.0100960932873028,-0.98736372289329,0.15814849861645));
#90003=DIRECTION('ref_axis',(-0.996606740262811,0.0228559949662293,0.0790734390098031));
#90004=DIRECTION('center_axis',(0.0409294185715571,0.987363722834022,0.153093636467149));
#90005=DIRECTION('ref_axis',(-0.986866308739757,0.015984610806164,0.160746324660136));
#90006=DIRECTION('',(-0.828884125374412,0.,-0.559420330969743));
#90007=DIRECTION('center_axis',(-0.0689322896726502,0.987366228486843,-0.142675401818788));
#90008=DIRECTION('ref_axis',(-0.953870035607405,-0.0233430431880731,0.299310971240695));
#90009=DIRECTION('',(0.559420330169213,0.,-0.828884125914696));
#90010=DIRECTION('center_axis',(2.1273937814866E-14,-1.,-6.58179424376849E-15));
#90011=DIRECTION('ref_axis',(1.,2.1273937814866E-14,-3.51258760307531E-32));
#90012=DIRECTION('center_axis',(-0.0508775060489346,-0.987363722578911,
-0.150081173747259));
#90013=DIRECTION('ref_axis',(-0.974206098104539,0.0159849106349481,0.22509322745903));
#90014=DIRECTION('center_axis',(0.0241371969397669,-0.987363722764837,0.156621437523263));
#90015=DIRECTION('ref_axis',(-0.956308175974158,0.02285599868685,0.291465737075571));
#90016=DIRECTION('center_axis',(0.0728831202615189,0.987363722755467,0.140715776540549));
#90017=DIRECTION('ref_axis',(-0.929238214197301,0.0159846130470007,0.36913525085143));
#90018=DIRECTION('',(-0.929764109056227,0.,-0.368155811458791));
#90019=DIRECTION('center_axis',(-0.0979916831930273,0.987366228552848,-0.124521326439782));
#90020=DIRECTION('ref_axis',(-0.867226073189164,-0.0233430412166463,0.497367108288898));
#90021=DIRECTION('',(0.368155805866007,0.,-0.929764111270784));
#90022=DIRECTION('center_axis',(-1.29077824990975E-14,-1.,7.33412221364675E-15));
#90023=DIRECTION('ref_axis',(1.,-1.29077824990975E-14,9.53777731518876E-32));
#90024=DIRECTION('center_axis',(-0.0819510393273368,-0.987363722536242,
-0.135635196658328));
#90025=DIRECTION('ref_axis',(-0.903041310616502,0.0159849165097872,0.429256186634747));
#90026=DIRECTION('center_axis',(0.0572418606350587,-0.987363722728211,0.147770932294974));
#90027=DIRECTION('ref_axis',(-0.87129370493947,0.0228560001693836,0.490229418730771));
#90028=DIRECTION('center_axis',(0.101428888140416,0.98736372270075,0.121758201962396));
#90029=DIRECTION('ref_axis',(-0.828159973897691,0.0159846158621332,0.5602638215069));
#90030=DIRECTION('',(-0.987169358123944,0.,-0.159676730869468));
#90031=DIRECTION('center_axis',(-0.122469100495229,0.987366228387713,-0.100544768453219));
#90032=DIRECTION('ref_axis',(-0.740031582688813,-0.0233430463661472,0.672166912908869));
#90033=DIRECTION('',(0.159676728323573,0.,-0.987169358535748));
#90034=DIRECTION('center_axis',(-2.20587724970193E-14,-1.,1.98748924161972E-14));
#90035=DIRECTION('ref_axis',(1.,-2.20587724970193E-14,-2.24130318029432E-32));
#90036=DIRECTION('center_axis',(-0.109192625785226,-0.987363722537315,-0.114847071757986));
#90037=DIRECTION('ref_axis',(-0.789651315668535,0.015984914242963,0.613347603060122));
#90038=DIRECTION('center_axis',(0.0876699622063691,-0.987363722805213,0.132010820067767));
#90039=DIRECTION('ref_axis',(-0.745538508437029,0.022855997249937,0.666070518659399));
#90040=DIRECTION('center_axis',(0.125231945564004,0.987363722864882,0.0971073559554355));
#90041=DIRECTION('ref_axis',(-0.688357894533299,0.0159846077203131,0.725195078133954));
#90042=DIRECTION('',(-0.998415664339409,0.,0.056268652033768));
#90043=DIRECTION('center_axis',(-0.14121998947165,0.987366228605458,-0.0718668573339754));
#90044=DIRECTION('ref_axis',(-0.578234039457966,-0.0233430387658572,0.815536938558457));
#90045=DIRECTION('',(-0.056268656982825,0.,-0.99841566406049));
#90046=DIRECTION('center_axis',(3.02234385184713E-14,-1.,-4.22663719263823E-14));
#90047=DIRECTION('ref_axis',(9.23861481743029E-32,4.22663719263823E-14,
-1.));
#90048=DIRECTION('center_axis',(-0.131328487682649,-0.987363722542341,-0.0886888252843569));
#90049=DIRECTION('ref_axis',(-0.639338102878694,0.0159849129887714,0.768759567591984));
#90050=DIRECTION('center_axis',(0.113998714502946,-0.987363722957852,0.110078025411463));
#90051=DIRECTION('ref_axis',(-0.584922758664488,0.022855991758488,0.810766902406025));
#90052=DIRECTION('center_axis',(0.143179307552888,0.987363722692716,0.0679158670640089));
#90053=DIRECTION('ref_axis',(-0.516368963541762,0.015984615356825,0.856217020131404));
#90054=DIRECTION('',(-0.962977163988183,0.,0.269582977276527));
#90055=DIRECTION('center_axis',(-0.153367597967407,0.987366228380772,-0.0398285192649395));
#90056=DIRECTION('ref_axis',(-0.389398912992463,-0.0233430469757092,0.920773364470421));
#90057=DIRECTION('',(-0.269582982049911,0.,-0.962977162651886));
#90058=DIRECTION('center_axis',(1.16747489638502E-14,-1.,-2.7300201939915E-14));
#90059=DIRECTION('ref_axis',(-8.42829456997971E-32,2.7300201939915E-14,
-1.));
#90060=DIRECTION('center_axis',(-0.147323577180954,-0.987363722544773,-0.0583835851000591));
#90061=DIRECTION('ref_axis',(-0.459130151320057,0.0159849151889484,0.888225189147));
#90062=DIRECTION('center_axis',(0.134997007515849,-0.98736372284086,0.0829981131086931));
#90063=DIRECTION('ref_axis',(-0.396956672600795,0.0228559966621038,0.917552725184927));
#90064=DIRECTION('center_axis',(0.154431756929921,0.987363722830919,0.0355487171218024));
#90065=DIRECTION('ref_axis',(-0.32023519511529,0.0159846109873066,0.947203205242179));
#90066=DIRECTION('',(-0.882510921618163,0.,0.470291902146594));
#90067=DIRECTION('center_axis',(-0.158343905549733,0.987366228052689,-0.00592783908880724));
#90068=DIRECTION('ref_axis',(-0.182355925401121,-0.0233430585632933,0.982955450713821));
#90069=DIRECTION('',(-0.47029190652181,0.,-0.882510919286601));
#90070=DIRECTION('center_axis',(6.91632924006171E-15,-1.,-3.64645803905207E-14));
#90071=DIRECTION('ref_axis',(-4.47855630928108E-32,3.64645803905207E-14,
-1.));
#90072=DIRECTION('center_axis',(-0.156429978770521,-0.987363722548624,-0.0253483951519218));
#90073=DIRECTION('ref_axis',(-0.257453783759328,0.0159849151389363,0.966158388524369));
#90074=DIRECTION('center_axis',(0.149682993082578,-0.987363722771226,0.0520372994801409));
#90075=DIRECTION('ref_axis',(-0.190429332313761,0.0228559990774562,0.981434803082052));
#90076=DIRECTION('center_axis',(0.158463151356584,0.987363722873948,0.00151934677967927));
#90077=DIRECTION('ref_axis',(-0.109127584832606,0.0159846093646868,0.993899221496858));
#90078=DIRECTION('',(-0.760779449282708,0.,0.649010500338092));
#90079=DIRECTION('center_axis',(-1.30101311407807E-15,-1.,-4.45186381807587E-14));
#90080=DIRECTION('ref_axis',(0.0292115385231254,-4.4537644533499E-14,0.999573251951608));
#90081=DIRECTION('center_axis',(-0.158221888563446,-0.987363722509994,0.00887206011162575));
#90082=DIRECTION('ref_axis',(-0.043739163848306,0.0159849177378449,0.998915095466459));
#90083=DIRECTION('center_axis',(0.15736996898241,-0.987363722822644,0.0186432753636452));
#90084=DIRECTION('ref_axis',(0.0250022698571692,0.0228559967621556,0.999426080265068));
#90085=DIRECTION('center_axis',(-0.155916223281314,0.987366228337048,0.0282499992418257));
#90086=DIRECTION('ref_axis',(0.0332138191420049,-0.0233430483582581,0.999175632364674));
#90087=DIRECTION('',(-0.649010505774152,0.,-0.760779444645279));
#90088=DIRECTION('',(0.562951245198508,0.,0.826490106129196));
#90089=DIRECTION('',(0.826490103338819,0.,-0.562951249295166));
#90090=DIRECTION('center_axis',(-1.42506245924468E-14,-1.,4.67670932993191E-14));
#90091=DIRECTION('ref_axis',(-3.31795861312863E-31,-4.67670932993191E-14,
-1.));
#90092=DIRECTION('',(0.37211881550646,0.,0.928185103923818));
#90093=DIRECTION('',(0.928185102079726,0.,-0.372118820106224));
#90094=DIRECTION('center_axis',(-1.19854977313491E-14,-1.,2.13051207289039E-14));
#90095=DIRECTION('ref_axis',(5.98310716154639E-31,-2.13051207289039E-14,
-1.));
#90096=DIRECTION('',(0.163886525562536,0.,0.986479197316923));
#90097=DIRECTION('',(0.986479196610463,0.,-0.163886529814916));
#90098=DIRECTION('center_axis',(-9.77115277883001E-14,-1.,1.09382946720462E-13));
#90099=DIRECTION('ref_axis',(2.26219721903079E-31,-1.09382946720462E-13,
-1.));
#90100=DIRECTION('',(-0.0520089175441786,0.,0.998646620429811));
#90101=DIRECTION('',(0.998646620676925,0.,0.0520089127992341));
#90102=DIRECTION('center_axis',(1.98235311947545E-14,-1.,-1.43034240564314E-14));
#90103=DIRECTION('ref_axis',(1.,1.98235311947545E-14,1.54468048409161E-31));
#90104=DIRECTION('',(-0.26547248098734,0.,0.964118437661279));
#90105=DIRECTION('',(0.964118438699595,0.,0.26547247721648));
#90106=DIRECTION('center_axis',(2.2434881337443E-14,-1.,-9.70754468690818E-15));
#90107=DIRECTION('ref_axis',(1.,2.2434881337443E-14,1.17354887193027E-31));
#90108=DIRECTION('',(-0.466522846721843,0.,0.884509148334006));
#90109=DIRECTION('',(0.884509150646384,0.,0.466522842337664));
#90110=DIRECTION('center_axis',(7.19916042948402E-14,-1.,-1.39732541140984E-14));
#90111=DIRECTION('ref_axis',(1.,7.19916042948402E-14,-3.12122083665017E-31));
#90112=DIRECTION('',(-0.645759126094484,0.,0.763541191466242));
#90113=DIRECTION('',(0.763541194667127,0.,0.645759122309779));
#90114=DIRECTION('center_axis',(-1.22187195728407E-13,-1.,-3.04916613055291E-15));
#90115=DIRECTION('ref_axis',(-0.999688772476419,1.22225235586043E-13,-0.0249471077399778));
#90116=DIRECTION('',(-0.794800422092897,0.,0.606870899813917));
#90117=DIRECTION('',(0.606870906241242,0.,0.794800417185304));
#90118=DIRECTION('center_axis',(7.12050275826231E-14,-1.,1.75467080845981E-14));
#90119=DIRECTION('ref_axis',(1.,7.12050275826231E-14,-3.78306478629417E-31));
#90120=DIRECTION('',(-0.90667773424271,0.,0.421823999113974));
#90121=DIRECTION('',(0.421824003608526,0.,0.906677732151658));
#90122=DIRECTION('center_axis',(2.19227566982768E-14,-1.,1.0814483979915E-14));
#90123=DIRECTION('ref_axis',(1.,2.19227566982768E-14,2.75543852127815E-31));
#90124=DIRECTION('',(-0.976159802699631,0.,0.21705308012884));
#90125=DIRECTION('',(0.217053081215155,0.,0.976159802458085));
#90126=DIRECTION('center_axis',(-5.7256261525697E-14,-1.,-4.58231761920508E-14));
#90127=DIRECTION('ref_axis',(1.,-5.7256261525697E-14,2.12756564536858E-30));
#90128=DIRECTION('',(-0.999997725164459,0.,0.00213299458671958));
#90129=DIRECTION('',(0.00213299954307815,0.,0.999997725153887));
#90130=DIRECTION('center_axis',(-1.07489698006143E-13,-1.,-1.33140605152815E-13));
#90131=DIRECTION('ref_axis',(2.95819333941865E-30,1.33140605152815E-13,
-1.));
#90132=DIRECTION('',(-0.977076864643459,0.,-0.212886825751402));
#90133=DIRECTION('',(-0.212886820908111,0.,0.977076865698722));
#90134=DIRECTION('center_axis',(3.27237231887067E-14,-1.,6.56292683412567E-14));
#90135=DIRECTION('ref_axis',(7.14654171068158E-31,-6.56292683412567E-14,
-1.));
#90136=DIRECTION('',(-0.908468975825409,0.,-0.417952293883803));
#90137=DIRECTION('',(-0.417952286130219,0.,0.90846897939254));
#90138=DIRECTION('center_axis',(1.19002053855136E-14,-1.,4.7419683964371E-14));
#90139=DIRECTION('ref_axis',(-4.27944612850522E-31,-4.7419683964371E-14,
-1.));
#90140=DIRECTION('',(-0.797382087238903,0.,-0.603474777393829));
#90141=DIRECTION('',(-0.603474773441189,0.,0.79738209023034));
#90142=DIRECTION('',(-0.649010502445557,0.,-0.760779447484858));
#90143=DIRECTION('',(-0.760779446212336,0.,0.649010503937226));
#90144=DIRECTION('center_axis',(3.18873609751326E-14,-1.,-1.68117970770856E-13));
#90145=DIRECTION('ref_axis',(-2.02423822237375E-31,1.68117970770856E-13,
-1.));
#90146=DIRECTION('',(-0.470291902230301,0.,-0.882510921573555));
#90147=DIRECTION('',(-0.882510919242011,0.,0.470291906605484));
#90148=DIRECTION('center_axis',(2.88352484393563E-14,-1.,-6.74282682904716E-14));
#90149=DIRECTION('ref_axis',(-1.18951982070183E-30,6.74282682904716E-14,
-1.));
#90150=DIRECTION('',(-0.269582977795074,0.,-0.962977163843017));
#90151=DIRECTION('',(-0.962977162506631,0.,0.269582982568776));
#90152=DIRECTION('center_axis',(4.26561810885819E-14,-1.,-5.96531070916475E-14));
#90153=DIRECTION('ref_axis',(9.5407336789931E-31,5.96531070916475E-14,-1.));
#90154=DIRECTION('',(-0.0562686524745445,0.,-0.998415664314567));
#90155=DIRECTION('',(-0.998415664035649,0.,0.0562686574235875));
#90156=DIRECTION('center_axis',(-1.81608525738086E-14,-1.,1.6362877447134E-14));
#90157=DIRECTION('ref_axis',(1.,-1.81608525738086E-14,1.48384009782733E-31));
#90158=DIRECTION('',(0.159676734244938,0.,-0.987169357577955));
#90159=DIRECTION('',(-0.98716935888988,0.,-0.15967672613422));
#90160=DIRECTION('center_axis',(4.25075937781184E-14,-1.,-2.41525519782833E-14));
#90161=DIRECTION('ref_axis',(1.,4.25075937781184E-14,8.40301947026E-31));
#90162=DIRECTION('',(0.368155812360744,0.,-0.929764108699083));
#90163=DIRECTION('',(-0.929764111872095,0.,-0.368155804347418));
#90164=DIRECTION('center_axis',(-1.6347056178951E-13,-1.,5.05750092776146E-14));
#90165=DIRECTION('ref_axis',(1.,-1.6347056178951E-13,-7.14902888199201E-31));
#90166=DIRECTION('',(0.559420334090901,0.,-0.828884123267918));
#90167=DIRECTION('',(-0.828884127273306,0.,-0.559420328156181));
#90168=DIRECTION('',(0.724526980936292,0.,-0.689246439160437));
#90169=DIRECTION('',(-0.689246444718413,0.,-0.724526975648959));
#90170=DIRECTION('center_axis',(0.,-1.,0.));
#90171=DIRECTION('ref_axis',(0.,0.,-1.));
#90172=DIRECTION('',(0.855755553808345,0.,-0.517380355373272));
#90173=DIRECTION('',(-0.517380359614475,0.,-0.85575555124416));
#90174=DIRECTION('center_axis',(-2.29634960358735E-14,-1.,-8.38082210911572E-15));
#90175=DIRECTION('ref_axis',(1.,-2.29634960358735E-14,4.3992465533463E-31));
#90176=DIRECTION('',(0.946969946451846,0.,-0.321322144454732));
#90177=DIRECTION('',(-0.32132214795012,0.,-0.946969945265805));
#90178=DIRECTION('center_axis',(-1.44374952654912E-13,-1.,-9.18494919385524E-14));
#90179=DIRECTION('ref_axis',(1.,-1.44374952654912E-13,8.12637320795991E-31));
#90180=DIRECTION('',(0.99390507839176,0.,-0.11023926318272));
#90181=DIRECTION('',(-0.110239267677687,0.,-0.9939050778932));
#90182=DIRECTION('center_axis',(-1.38576708982774E-13,-1.,-1.37986798379914E-13));
#90183=DIRECTION('ref_axis',(1.,-1.38576708982774E-13,-8.59017661330448E-31));
#90184=DIRECTION('',(0.994366313149823,0.,0.105998279574848));
#90185=DIRECTION('',(0.105998278540145,0.,-0.994366313260121));
#90186=DIRECTION('center_axis',(-2.6418444921436E-14,-1.,-4.11376599337965E-14));
#90187=DIRECTION('ref_axis',(-7.95516692322674E-31,4.11376599337965E-14,
-1.));
#90188=DIRECTION('',(0.948332083835448,0.,0.317279464775641));
#90189=DIRECTION('',(0.31727946007514,0.,-0.948332085408075));
#90190=DIRECTION('center_axis',(3.39148311317661E-14,-1.,9.17101384722506E-14));
#90191=DIRECTION('ref_axis',(7.13691189980589E-32,-9.17101384722506E-14,
-1.));
#90192=DIRECTION('',(0.857954900607374,0.,0.513725012554179));
#90193=DIRECTION('',(0.513725008301434,0.,-0.857954903153826));
#90194=DIRECTION('center_axis',(3.3517380830713E-15,-1.,2.421417305627E-14));
#90195=DIRECTION('ref_axis',(3.95306254274215E-32,-2.421417305627E-14,-1.));
#90196=DIRECTION('',(0.727460699689289,0.,0.686149349928695));
#90197=DIRECTION('center_axis',(7.72782051473817E-15,-1.,-9.74743349916755E-14));
#90198=DIRECTION('ref_axis',(-0.0790325797119564,-9.77801881363366E-14,
0.99687203358509));
#90199=DIRECTION('',(0.686149346322776,0.,-0.727460703090433));
#90200=DIRECTION('center_axis',(0.163197749987252,-0.986495109897446,0.0139245304238548));
#90201=DIRECTION('ref_axis',(0.0254674151392068,0.0183213284312142,0.999507748689645));
#90202=DIRECTION('center_axis',(-0.159101001719421,-0.98649511023429,0.0389136060486979));
#90203=DIRECTION('ref_axis',(0.139799307721241,0.016506827496646,0.990042260818526));
#90204=DIRECTION('center_axis',(0.162375647399524,-0.986495108859253,-0.0214836991311003));
#90205=DIRECTION('ref_axis',(0.239736643839447,0.0183213442783557,0.970665065789653));
#90206=DIRECTION('center_axis',(-0.147016033672384,-0.986495110214053,0.07220584025551));
#90207=DIRECTION('ref_axis',(0.349360698698762,0.0165068277187146,0.936842904036412));
#90208=DIRECTION('center_axis',(0.153961016969689,-0.986495110699525,-0.0558874030492672));
#90209=DIRECTION('ref_axis',(0.44279603111771,0.0183213213359592,0.896435164421225));
#90210=DIRECTION('center_axis',(-0.128056758497475,-0.986495110176503,0.10212181060365));
#90211=DIRECTION('ref_axis',(0.542586372947516,0.0165068288788752,0.839837813206825));
#90212=DIRECTION('center_axis',(0.138347353699881,-0.986495110711692,-0.08767785504999));
#90213=DIRECTION('ref_axis',(0.625150766853485,0.0183213200643359,0.780288951564483));
#90214=DIRECTION('center_axis',(-0.103109690306681,-0.986495110153458,0.127262678771813));
#90215=DIRECTION('ref_axis',(0.710441310111489,0.0165068311346094,0.703562839704432));
#90216=DIRECTION('center_axis',(0.116264744835321,-0.986495108930328,-0.115368579625991));
#90217=DIRECTION('ref_axis',(0.778274147036787,0.0183213421848879,0.627657295404671));
#90218=DIRECTION('center_axis',(-0.0733413333033863,-0.986495110181623,
0.14645288121792));
#90219=DIRECTION('ref_axis',(0.845076800566642,0.0165068261280715,0.53439005027716));
#90220=DIRECTION('center_axis',(0.0887456881072436,-0.98649511049776,-0.137664809615185));
#90221=DIRECTION('ref_axis',(0.895006296275743,0.0183213269098285,0.445677078844134));
#90222=DIRECTION('center_axis',(-0.0401436161497176,-0.986495110223755,
0.158795111974661));
#90223=DIRECTION('ref_axis',(0.940197438546159,0.0165068233288879,0.340229777260648));
#90224=DIRECTION('center_axis',(0.0570769958322964,-0.986495110611188,-0.153523982774612));
#90225=DIRECTION('ref_axis',(0.969888944115819,0.0183213240737779,0.242857499711427));
#90226=DIRECTION('center_axis',(-0.00506882451432805,-0.986495110238031,
0.163712261283321));
#90227=DIRECTION('ref_axis',(0.991355489517604,0.0165068248546079,0.13016073961272));
#90228=DIRECTION('center_axis',(0.0227394654220306,-0.986495108959915,-0.162204552064625));
#90229=DIRECTION('ref_axis',(0.999420662940406,0.018321340512334,0.0286821716331137));
#90230=DIRECTION('center_axis',(0.0302429834585616,-0.98649511018174,0.160974406472092));
#90231=DIRECTION('ref_axis',(0.996158860300694,0.0165068293684157,-0.0859944744075077));
#90232=DIRECTION('center_axis',(-0.0126613729172467,-0.986495110734072,
-0.163300600530499));
#90233=DIRECTION('ref_axis',(0.982220582776599,0.0183213198539688,-0.186834300942859));
#90234=DIRECTION('center_axis',(0.0641406633763457,-0.986495110174397,0.150709564738432));
#90235=DIRECTION('ref_axis',(0.954382949533046,0.0165068348330388,-0.298128680345246));
#90236=DIRECTION('center_axis',(-0.0474701529819279,-0.986495110541529,
-0.156760905373532));
#90237=DIRECTION('ref_axis',(0.919092959171724,0.018321326784228,-0.39361461022913));
#90238=DIRECTION('center_axis',(0.0950391876824385,-0.986495110247086,0.1333977146103));
#90239=DIRECTION('ref_axis',(0.867981153072863,0.0165068300635194,-0.496322720083975));
#90240=DIRECTION('center_axis',(-0.0800592794799243,-0.986495108881716,
-0.14289125908049));
#90241=DIRECTION('ref_axis',(0.812989570484355,0.0183213433664377,-0.581989936906914));
#90242=DIRECTION('center_axis',(0.121493790101314,-0.986495110177343,0.109848334366111));
#90243=DIRECTION('ref_axis',(0.740993521301427,0.0165068299297818,-0.671309262527325));
#90244=DIRECTION('center_axis',(-0.108904939865407,-0.986495110542266,-0.122340144470716));
#90245=DIRECTION('ref_axis',(0.668871694283925,0.0183213263347191,-0.743152060877913));
#90246=DIRECTION('center_axis',(0.142267476719983,-0.986495110210635,0.081162568947983));
#90247=DIRECTION('ref_axis',(0.579357859691649,0.016506829044998,-0.81490612650071));
#90248=DIRECTION('center_axis',(-0.132658318227354,-0.986495110593608,-0.0960685556256334));
#90249=DIRECTION('ref_axis',(0.493478119854653,0.0183213248467722,-0.869565221406983));
#90250=DIRECTION('center_axis',(0.156388896590567,-0.986495110143674,0.0486817284595133));
#90251=DIRECTION('ref_axis',(0.390632064234538,0.0165068316523958,-0.920398889015335));
#90252=DIRECTION('center_axis',(-0.150208740918382,-0.98649511067299,-0.0653049061709711));
#90253=DIRECTION('ref_axis',(0.295010055448863,0.0183213220749732,-0.955318479011834));
#90254=DIRECTION('center_axis',(0.163197743665263,-0.986495110172428,0.013924585037137));
#90255=DIRECTION('ref_axis',(0.183640749222092,0.0165068333459602,-0.98285482126204));
#90256=DIRECTION('center_axis',(-0.160735568247925,-0.986495110467,-0.0314876821109071));
#90257=DIRECTION('ref_axis',(0.0827476521059804,0.0183213293856647,-0.996402105056232));
#90258=DIRECTION('center_axis',(0.162375645555574,-0.986495110193824,-0.0214836517865426));
#90259=DIRECTION('ref_axis',(-0.0319374034875196,0.0165068301898106,-0.999353554461863));
#90260=DIRECTION('center_axis',(-0.163746580379318,-0.98649511053951,0.00380188055031853));
#90261=DIRECTION('ref_axis',(-0.133383942944882,0.0183213273159671,-0.990895076549408));
#90262=DIRECTION('center_axis',(0.153961042610572,-0.986495110180794,-0.0558873415689909));
#90263=DIRECTION('ref_axis',(-0.24602219607511,0.0165068322773698,-0.969123626544388));
#90264=DIRECTION('center_axis',(-0.159100984330676,-0.986495110516032,0.0389136700013237));
#90265=DIRECTION('ref_axis',(-0.343278649941192,0.0183213262598227,-0.939054895891946));
#90266=DIRECTION('center_axis',(0.138347393324552,-0.986495110212549,-0.0876777981420205));
#90267=DIRECTION('ref_axis',(-0.448603267737991,0.0165068303046711,-0.893578554312988));
#90268=DIRECTION('center_axis',(-0.147016018594641,-0.986495108895638,0.0722058889673391));
#90269=DIRECTION('ref_axis',(-0.537122031167507,0.0183213433011018,-0.843305550802398));
#90270=DIRECTION('center_axis',(0.11626477814819,-0.98649511025318,-0.115368534742875));
#90271=DIRECTION('ref_axis',(-0.630208146839801,0.0165068232943342,-0.776250743279176));
#90272=DIRECTION('center_axis',(-0.128056731448253,-0.986495108989023,0.102121855993341));
#90273=DIRECTION('ref_axis',(-0.705850180445786,0.0183213393733161,-0.708124177872934));
#90274=DIRECTION('center_axis',(0.0887457420157033,-0.986495110165441,-0.137664777244423));
#90275=DIRECTION('ref_axis',(-0.782345196015598,0.0165068299203812,-0.622626307537109));
#90276=DIRECTION('center_axis',(-0.103109656079333,-0.986495108998286,0.127262715457674));
#90277=DIRECTION('ref_axis',(-0.841573562645043,0.018321339942445,-0.53983170262559));
#90278=DIRECTION('center_axis',(0.0570770554641016,-0.986495110139405,-0.153523963636272));
#90279=DIRECTION('ref_axis',(-0.897900651127143,0.0165068329766776,-0.439888559945053));
#90280=DIRECTION('center_axis',(-0.0733412699599285,-0.986495110625006,
0.146452909952731));
#90281=DIRECTION('ref_axis',(-0.937945899781614,0.0183213239878117,-0.346297297376391));
#90282=DIRECTION('center_axis',(0.02273951420849,-0.986495110181865,-0.162204537793588));
#90283=DIRECTION('ref_axis',(-0.971471270290504,0.0165068302411123,-0.236582111655858));
#90284=DIRECTION('center_axis',(-0.04014354410436,-0.986495110627204,0.158795127681432));
#90285=DIRECTION('ref_axis',(-0.990460928077634,0.0183213224042447,-0.13657041808881));
#90286=DIRECTION('center_axis',(-0.0126613009638283,-0.986495110234729,
-0.163300609125851));
#90287=DIRECTION('ref_axis',(-0.99961697252754,0.016506827654815,-0.0222133490417421));
#90288=DIRECTION('center_axis',(-0.00506877555090952,-0.98649510877511,
0.163712271614556));
#90289=DIRECTION('ref_axis',(-0.996663104595291,0.0183213468885308,0.0795423420994461));
#90290=DIRECTION('center_axis',(-0.0474700944980979,-0.986495110139843,
-0.156760925611329));
#90291=DIRECTION('ref_axis',(-0.981021696401571,0.0165068314900331,0.193194088169239));
#90292=DIRECTION('center_axis',(0.0302430480139253,-0.986495110576138,0.160974391926792));
#90293=DIRECTION('ref_axis',(-0.956262422213734,0.0183213243394206,0.29193579591474));
#90294=DIRECTION('center_axis',(-0.0800592318971633,-0.986495110224997,
-0.142891276466436));
#90295=DIRECTION('ref_axis',(-0.916554935759703,0.0165068276718343,0.399567984671869));
#90296=DIRECTION('center_axis',(0.0641407206136267,-0.986495110682394,0.150709537053553));
#90297=DIRECTION('ref_axis',(-0.871147972385388,0.0183213211698033,0.490678651868431));
#90298=DIRECTION('center_axis',(-0.108904892632709,-0.986495110251071,-0.122340188864435));
#90299=DIRECTION('ref_axis',(-0.809231086683801,0.0165068288872051,0.58725852309238));
#90300=DIRECTION('center_axis',(0.0950392389666235,-0.986495110605007,0.133397675425997));
#90301=DIRECTION('ref_axis',(-0.74529960925457,0.0183213254219731,0.666477922724952));
#90302=DIRECTION('center_axis',(-0.132658279393603,-0.986495110257214,-0.0960686127043377));
#90303=DIRECTION('ref_axis',(-0.664068490537254,0.0165068261774196,0.747489507996682));
#90304=DIRECTION('center_axis',(0.121493832547443,-0.986495110620513,0.109848283440187));
#90305=DIRECTION('ref_axis',(-0.584601866466365,0.0183213234933828,0.811113424145781));
#90306=DIRECTION('center_axis',(-0.150208717742504,-0.986495110197418,-0.0653049666620904));
#90307=DIRECTION('ref_axis',(-0.487854788014172,0.016506833265213,0.872768715220248));
#90308=DIRECTION('center_axis',(0.142267507527001,-0.986495108892044,0.0811625309741451));
#90309=DIRECTION('ref_axis',(-0.396568793550313,0.0183213435490668,0.917822161615531));
#90310=DIRECTION('center_axis',(-0.160735557249265,-0.986495110220616,-0.0314877459749657));
#90311=DIRECTION('ref_axis',(-0.28882953792318,0.016506825465469,0.957238226741982));
#90312=DIRECTION('center_axis',(0.156388912663549,-0.986495110500926,0.0486816695859882));
#90313=DIRECTION('ref_axis',(-0.189992599186342,0.018321327088903,0.981614558382321));
#90314=DIRECTION('center_axis',(-0.163746587452144,-0.98649510959552,0.00380182086643908));
#90315=DIRECTION('ref_axis',(-0.0762989170803437,0.0165068292334505,0.996948343617173));
#90316=DIRECTION('center_axis',(-0.163664333248049,0.986495979512518,0.00629828771255697));
#90317=DIRECTION('ref_axis',(-0.0757555104791332,-0.0189332063975585,0.996946656711157));
#90318=DIRECTION('center_axis',(0.163197764356552,0.986495107104501,0.0139245598818328));
#90319=DIRECTION('ref_axis',(-0.183634611457542,0.0165058305046527,0.98285598489005));
#90320=DIRECTION('center_axis',(-0.161191922426216,0.98649597748642,-0.0290318884617355));
#90321=DIRECTION('ref_axis',(-0.288298455888899,-0.0189332806778659,0.957353399333208));
#90322=DIRECTION('center_axis',(0.156388923028194,0.986495107029387,0.0486817066377158));
#90323=DIRECTION('ref_axis',(-0.390626320339424,0.0165058307684231,0.920401344745175));
#90324=DIRECTION('center_axis',(-0.1511823468822,0.98649597751628,-0.0630046374117834));
#90325=DIRECTION('ref_axis',(-0.487360881411285,-0.0189332810357842,0.872995362037643));
#90326=DIRECTION('center_axis',(0.142267505986882,0.986495107181025,0.0811625544704576));
#90327=DIRECTION('ref_axis',(-0.5793527766561,0.0165058262039459,0.814909760576098));
#90328=DIRECTION('center_axis',(-0.13410359443023,0.986495979823994,-0.094031418961912));
#90329=DIRECTION('ref_axis',(-0.663634846270329,-0.0189331951519553,0.747817039747755));
#90330=DIRECTION('center_axis',(0.121493822324455,0.986495107119942,0.109848326183918));
#90331=DIRECTION('ref_axis',(-0.740989340052899,0.0165058281422236,0.671313902407293));
#90332=DIRECTION('center_axis',(-0.110754427179715,0.986495977338123,-0.120661276123679));
#90333=DIRECTION('ref_axis',(-0.808877993467493,-0.0189332878563786,0.587671610931606));
#90334=DIRECTION('center_axis',(0.0950392208017098,0.986495107120491,0.133397714136095));
#90335=DIRECTION('ref_axis',(-0.867978066280491,0.0165058276362661,0.496328151639641));
#90336=DIRECTION('center_axis',(-0.0822263620131329,0.986495979699681,-0.141649240825542));
#90337=DIRECTION('ref_axis',(-0.916298899956403,-0.0189331999132928,0.400047322050441));
#90338=DIRECTION('center_axis',(0.0641406948191214,0.986495107043704,0.150709571849138));
#90339=DIRECTION('ref_axis',(-0.954381102941002,0.0165058315162098,0.298134647223489));
#90340=DIRECTION('center_axis',(-0.0498536337343701,0.98649597752984,-0.156013786316864));
#90341=DIRECTION('ref_axis',(-0.980874689975391,-0.0189332811454051,0.193717251247147));
#90342=DIRECTION('center_axis',(0.0302430199761457,0.986495106974469,0.160974419266395));
#90343=DIRECTION('ref_axis',(-0.996158339361333,0.0165058333444339,0.0860006999185329));
#90344=DIRECTION('center_axis',(-0.0151496822461874,0.986495978873035,-0.163083324699898));
#90345=DIRECTION('ref_axis',(-0.999585868728208,-0.0189332301313235,-0.0216708060687373));
#90346=DIRECTION('center_axis',(-0.00506879156494291,0.986495107120187,
0.163712281090948));
#90347=DIRECTION('ref_axis',(-0.991356319237998,0.0165058285717886,-0.130154546328768));
#90348=DIRECTION('center_axis',(0.0202625533420198,0.986495977468237,-0.162527275775636));
#90349=DIRECTION('ref_axis',(-0.971557521471604,-0.0189332835680874,-0.236045574509002));
#90350=DIRECTION('center_axis',(-0.040143584424462,0.98649510707811,0.158795139536779));
#90351=DIRECTION('ref_axis',(-0.94019957963103,0.0165058313262934,-0.340223908615873));
#90352=DIRECTION('center_axis',(0.054727380587086,0.986495977283348,-0.154371631519033));
#90353=DIRECTION('ref_axis',(-0.898100225644532,-0.0189332899024866,-0.43938310758461));
#90354=DIRECTION('center_axis',(-0.0733413127678706,0.986495107140305,0.146452911987861));
#90355=DIRECTION('ref_axis',(-0.845080151221418,0.0165058292689584,-0.534384782354184));
#90356=DIRECTION('center_axis',(0.0866332565622247,0.986495978515498,-0.138997709442183));
#90357=DIRECTION('ref_axis',(-0.782648764505326,-0.0189332432368636,-0.622175573065048));
#90358=DIRECTION('center_axis',(-0.103109680670976,0.986495107096398,0.12726271027601));
#90359=DIRECTION('ref_axis',(-0.71044571539837,0.0165058293165022,-0.70355841482472));
#90360=DIRECTION('center_axis',(0.11448819137911,0.986495977279155,-0.117124467327646));
#90361=DIRECTION('ref_axis',(-0.630601510825,-0.0189332895128348,-0.775875805199164));
#90362=DIRECTION('center_axis',(-0.128056754262896,0.986495107061115,0.102121846008249));
#90363=DIRECTION('ref_axis',(-0.542591628058386,0.0165058298040078,-0.839834437697949));
#90364=DIRECTION('center_axis',(0.136989821620645,0.986495977428063,-0.0897745804256088));
#90365=DIRECTION('ref_axis',(-0.449068033188857,-0.0189332841864589,-0.893296945207923));
#90366=DIRECTION('center_axis',(-0.14701603772493,0.986495107128574,0.0722058741588577));
#90367=DIRECTION('ref_axis',(-0.349366558275532,0.016505826638935,-0.936840736542597));
#90368=DIRECTION('center_axis',(0.153085958069839,0.986495977607133,-0.0582269319712594));
#90369=DIRECTION('ref_axis',(-0.246536634745093,-0.0189332775614308,-0.968948511908319));
#90370=DIRECTION('center_axis',(-0.159101011931081,0.986495106883992,0.0389136492306638));
#90371=DIRECTION('ref_axis',(-0.139805499905608,0.0165058369330538,-0.990041402943979));
#90372=DIRECTION('center_axis',(0.162023962704327,0.98649597747952,-0.0239566676796347));
#90373=DIRECTION('ref_axis',(-0.0324774595201144,-0.0189332820365999,-0.999293122889596));
#90374=DIRECTION('center_axis',(-0.163746601402507,0.986495107191856,0.00380184371816674));
#90375=DIRECTION('ref_axis',(0.0762927159752781,0.016505826028842,-0.996948834793552));
#90376=DIRECTION('center_axis',(0.163385893887828,0.986495979129472,0.0114338462408331));
#90377=DIRECTION('ref_axis',(0.183100325011878,-0.0189332213510897,-0.982911900482345));
#90378=DIRECTION('center_axis',(-0.160735581661557,0.986495107149784,-0.0314877175650721));
#90379=DIRECTION('ref_axis',(0.288823563605248,0.0165058287140023,-0.957240046553021));
#90380=DIRECTION('center_axis',(0.15710806840229,0.986495980083366,0.0462896977983183));
#90381=DIRECTION('ref_axis',(0.390116541163451,-0.0189331856892312,-0.920570811393845));
#90382=DIRECTION('center_axis',(-0.150208745852932,0.986495107055466,-0.0653049494671993));
#90383=DIRECTION('ref_axis',(0.487849340789981,0.016505830189358,-0.872771779023899));
#90384=DIRECTION('center_axis',(0.143484048841015,0.986495980220824,0.0789810656825073));
#90385=DIRECTION('ref_axis',(0.578891344290511,-0.0189331794489455,-0.815184854018694));
#90386=DIRECTION('center_axis',(-0.132658315821449,0.986495107001696,-0.0960685958319888));
#90387=DIRECTION('ref_axis',(0.664063827017501,0.0165058308092504,-0.747493673014138));
#90388=DIRECTION('center_axis',(0.123150951914379,0.986495977546296,0.107979300458746));
#90389=DIRECTION('ref_axis',(0.740597838944811,-0.0189332788902449,-0.671681748970999));
#90390=DIRECTION('center_axis',(-0.10890493398378,0.986495106879436,-0.12234017924181));
#90391=DIRECTION('ref_axis',(0.809227427902569,0.0165058359713355,-0.587263592698441));
#90392=DIRECTION('center_axis',(0.0970593980376401,0.986495977400082,0.131928616403066));
#90393=DIRECTION('ref_axis',(0.867674794371259,-0.0189332842684578,-0.496771559129146));
#90394=DIRECTION('center_axis',(-0.0800592662611623,0.986495107147041,-0.142891278462583));
#90395=DIRECTION('ref_axis',(0.916552454181826,0.0165058269382781,-0.399573718367906));
#90396=DIRECTION('center_axis',(0.0664293728880749,0.986495979621629,0.149709119989594));
#90397=DIRECTION('ref_axis',(0.954180240376983,-0.0189332022433862,-0.298632889559966));
#90398=DIRECTION('center_axis',(-0.047470133162406,0.98649510690294,-0.15676093427286));
#90399=DIRECTION('ref_axis',(0.981020504823173,0.0165058359565571,-0.193200223850445));
#90400=DIRECTION('center_axis',(0.0326931799835002,0.986495981711792,0.16048935805546));
#90401=DIRECTION('ref_axis',(0.996069280944152,-0.0189331239650817,-0.0865304823534663));
#90402=DIRECTION('center_axis',(-0.0126613348343359,0.986495107103492,-0.163300625415466));
#90403=DIRECTION('ref_axis',(0.99961712783561,0.0165058300291245,0.022207100502665));
#90404=DIRECTION('center_axis',(-0.00257148638013054,0.986495977523527,
0.163765300926962));
#90405=DIRECTION('ref_axis',(0.991383225516875,-0.0189332809941951,0.129618019713895));
#90406=DIRECTION('center_axis',(0.0227394880264797,0.986495107075598,-0.162204560355739));
#90407=DIRECTION('ref_axis',(0.971472764423259,0.0165058297100802,0.236576046060061));
#90408=DIRECTION('center_axis',(-0.0377160676873686,0.986495977585325,0.159383764688175));
#90409=DIRECTION('ref_axis',(0.940341194310948,-0.0189332781904157,0.33970570978249));
#90410=DIRECTION('center_axis',(0.0570770334185452,0.986495106966099,-0.153523992222986));
#90411=DIRECTION('ref_axis',(0.897903414895677,0.0165058338156129,0.43988295598799));
#90412=DIRECTION('center_axis',(-0.0710970874986947,0.986495977655359,0.147549619514932));
#90413=DIRECTION('ref_axis',(0.845329852688694,-0.018933275537671,0.533909141362766));
#90414=DIRECTION('center_axis',(0.0887457235084081,0.986495106948599,-0.137664812226802));
#90415=DIRECTION('ref_axis',(0.782349100079219,0.0165058346295532,0.622621428340222));
#90416=DIRECTION('center_axis',(-0.101153678319687,0.986495977432116,0.12881622519175));
#90417=DIRECTION('ref_axis',(0.710791828123047,-0.0189332835167351,0.703147571885711));
#90418=DIRECTION('center_axis',(0.116264764031022,0.986495106987654,-0.115368576892616));
#90419=DIRECTION('ref_axis',(0.630213007616838,0.0165058336096042,0.776246818020784));
#90420=DIRECTION('center_axis',(-0.126480445892826,0.986495977695225,0.104059515652792));
#90421=DIRECTION('ref_axis',(0.543017965192465,-0.0189332758823195,0.839507606006401));
#90422=DIRECTION('center_axis',(0.13834739311538,0.986495107082014,-0.0876778336948641));
#90423=DIRECTION('ref_axis',(0.448608856798898,0.0165058310964719,0.893575766872289));
#90424=DIRECTION('center_axis',(-0.145893125991885,0.986495977858703,0.0744370973165731));
#90425=DIRECTION('ref_axis',(0.349853187284538,-0.0189332677462982,0.936613195892145));
#90426=DIRECTION('center_axis',(0.153961049669868,0.986495106924751,-0.0558873795957304));
#90427=DIRECTION('ref_axis',(0.246028258851622,0.0165058354854542,0.969122104402415));
#90428=DIRECTION('center_axis',(-0.158484009812962,0.986495980522315,0.0413339938418896));
#90429=DIRECTION('ref_axis',(0.140329675865358,-0.0189331681346543,0.989923793640656));
#90430=DIRECTION('center_axis',(0.162375647171994,0.986495113156432,-0.0214835035307127));
#90431=DIRECTION('ref_axis',(0.0319435454120738,0.0165056650919532,0.999353377402798));
#90432=DIRECTION('center_axis',(-0.158253626588392,0.987363722264226,-0.00828671395391741));
#90433=DIRECTION('ref_axis',(0.132153477991923,0.0294968937920318,0.990790286342806));
#90434=DIRECTION('',(-0.726975930476597,0.,-0.686662942430772));
#90435=DIRECTION('center_axis',(-3.03776950303028E-15,-1.,-2.20606524517768E-14));
#90436=DIRECTION('ref_axis',(2.28515888441093E-33,2.20606524517768E-14,
-1.));
#90437=DIRECTION('center_axis',(-0.158221889114687,-0.987363722231891,0.00887208123073));
#90438=DIRECTION('ref_axis',(0.061138418742882,-0.00082842314327428,0.998128953326531));
#90439=DIRECTION('center_axis',(0.157698501290688,-0.987363722511171,-0.0156224889039391));
#90440=DIRECTION('ref_axis',(0.135390691994632,0.00594770339583162,0.990774437167981));
#90441=DIRECTION('center_axis',(0.155084985279889,0.987363722259802,-0.0325810881648317));
#90442=DIRECTION('ref_axis',(0.210647662491098,-0.00082873789506162,0.977561699065863));
#90443=DIRECTION('',(-0.514330808231265,0.,0.857591872456925));
#90444=DIRECTION('center_axis',(-0.156335142091049,0.98736372237026,0.0259268797681987));
#90445=DIRECTION('ref_axis',(0.3420544268796,0.0294968903025397,0.939217068900767));
#90446=DIRECTION('',(-0.857591872604236,0.,-0.514330807985639));
#90447=DIRECTION('center_axis',(-1.54182726050674E-14,-1.,-4.17837119886613E-14));
#90448=DIRECTION('ref_axis',(8.92452105586287E-32,4.17837119886613E-14,
-1.));
#90449=DIRECTION('center_axis',(-0.152615513172356,-0.987363722259592,0.0426776886068243));
#90450=DIRECTION('ref_axis',(0.274277257963118,-0.000828420576119193,0.961650299996616));
#90451=DIRECTION('center_axis',(0.150653225068809,-0.987363722493281,-0.049157759108585));
#90452=DIRECTION('ref_axis',(0.345212550285589,0.00594770451630662,0.93850568455194));
#90453=DIRECTION('center_axis',(0.144455213653567,0.987363722246305,-0.0651580481615592));
#90454=DIRECTION('ref_axis',(0.415869706492917,-0.000828737827710053,0.909423828814216));
#90455=DIRECTION('',(-0.31794913654061,0.,0.948107771602512));
#90456=DIRECTION('center_axis',(-0.147106602674719,0.987363722257596,0.0589281547235814));
#90457=DIRECTION('ref_axis',(0.535961290935937,0.0294968942300542,0.843727105081415));
#90458=DIRECTION('',(-0.948107771776315,0.,-0.317949136022339));
#90459=DIRECTION('center_axis',(-1.20200324666943E-14,-1.,-1.87461795955026E-14));
#90460=DIRECTION('ref_axis',(1.34216343081091E-31,1.87461795955026E-14,
-1.));
#90461=DIRECTION('center_axis',(-0.139873008188513,-0.987363722211362,0.0744877281249787));
#90462=DIRECTION('ref_axis',(0.474591193787211,-0.000828424723521796,0.880205948907475));
#90463=DIRECTION('center_axis',(0.136563571729436,-0.987363722495009,-0.0803944673301516));
#90464=DIRECTION('ref_axis',(0.538892651517533,0.00594770519656905,0.842353450128447));
#90465=DIRECTION('center_axis',(0.127070876965365,0.9873637222521,-0.094688289707496));
#90466=DIRECTION('ref_axis',(0.601646145372297,-0.000828738403524133,0.798762310672778));
#90467=DIRECTION('',(-0.106700515256271,0.,0.994291204850996));
#90468=DIRECTION('center_axis',(-0.130999520502367,0.987363722264207,0.0891740185520412));
#90469=DIRECTION('ref_axis',(0.704807200182574,0.0294968937672872,0.708785400406133));
#90470=DIRECTION('',(-0.994291204618494,0.,-0.106700517422851));
#90471=DIRECTION('center_axis',(-4.20503607035944E-14,-1.,-4.19305404223952E-14));
#90472=DIRECTION('ref_axis',(1.,-4.20503607035944E-14,-5.12746317913781E-31));
#90473=DIRECTION('center_axis',(-0.120590197321097,-0.987363722182784,0.102814806460049));
#90474=DIRECTION('ref_axis',(0.652713776020247,-0.000828427761268574,0.757604144854577));
#90475=DIRECTION('center_axis',(0.116088354225877,-0.987363722546377,-0.107872023307662));
#90476=DIRECTION('ref_axis',(0.707374734234289,0.0059477013187499,0.706813702623252));
#90477=DIRECTION('center_axis',(0.103744844714906,0.987363722262932,-0.119791014496784));
#90478=DIRECTION('ref_axis',(0.759290278625285,-0.000828735251910435,0.650751554729621));
#90479=DIRECTION('',(0.109537302858737,0.,0.993982685604952));
#90480=DIRECTION('center_axis',(-0.108767043158536,0.987363722376516,0.115250206322328));
#90481=DIRECTION('ref_axis',(0.840697110508886,0.0294968901382479,0.540701675468258));
#90482=DIRECTION('',(-0.993982686191135,0.,0.109537297539497));
#90483=DIRECTION('center_axis',(1.87804025222973E-14,-1.,1.19664911831704E-14));
#90484=DIRECTION('ref_axis',(1.,1.87804025222973E-14,1.48804922800187E-31));
#90485=DIRECTION('center_axis',(-0.0956687178831378,-0.987363722223788,
0.126334383502602));
#90486=DIRECTION('ref_axis',(0.800316189860067,-0.000828424311078544,0.599577609622829));
#90487=DIRECTION('center_axis',(0.0901849763702522,-0.98736372252264,-0.130305600352908));
#90488=DIRECTION('ref_axis',(0.842780758136601,0.0059477006296843,0.538224134141081));
#90489=DIRECTION('center_axis',(0.0755678242784833,0.987363722270313,-0.139292440133444));
#90490=DIRECTION('ref_axis',(0.881430841406361,-0.000828739094572826,0.472312380749423));
#90491=DIRECTION('',(0.32065327633744,0.,0.947196640816502));
#90492=DIRECTION('center_axis',(-0.0814487487602662,0.98736372219462,0.135937417289623));
#90493=DIRECTION('ref_axis',(0.937276955390323,0.0294968964833239,0.347335345152346));
#90494=DIRECTION('',(-0.947196641515213,0.,0.320653274273476));
#90495=DIRECTION('center_axis',(4.87987943628401E-14,-1.,1.7848809686811E-14));
#90496=DIRECTION('ref_axis',(1.,4.87987943628401E-14,8.49501243221605E-32));
#90497=DIRECTION('center_axis',(-0.0662738822247424,-0.987363722186029,
0.143946700711793));
#90498=DIRECTION('ref_axis',(0.910496703083341,-0.000828427828625555,0.413515498357315));
#90499=DIRECTION('center_axis',(0.060064647181345,-0.987363722582784,-0.146646232431821));
#90500=DIRECTION('ref_axis',(0.938779291700636,0.0059476984014665,0.344467801627056));
#90501=DIRECTION('center_axis',(0.0438573363386594,0.98736372229545,-0.152280707721466));
#90502=DIRECTION('ref_axis',(0.962356678422975,-0.000828742191178215,0.271788404243224));
#90503=DIRECTION('',(0.516775860806559,0.,0.856120733125673));
#90504=DIRECTION('center_axis',(-0.0503219923558105,0.987363722299207,0.150268349870477));
#90505=DIRECTION('ref_axis',(0.990030773344163,0.029496893116985,0.137727996892442));
#90506=DIRECTION('',(-0.856120735019485,0.,0.51677585766916));
#90507=DIRECTION('center_axis',(-4.41384618210966E-14,-1.,-5.94961382401061E-15));
#90508=DIRECTION('ref_axis',(1.,-4.41384618210967E-14,6.09873644106572E-32));
#90509=DIRECTION('center_axis',(-0.0337801471428057,-0.987363722229621,
0.154828232838452));
#90510=DIRECTION('ref_axis',(0.978103405358154,-0.000828425242064668,0.208117856366055));
#90511=DIRECTION('center_axis',(0.027135767662474,-0.98736372254328,-0.156129848263698));
#90512=DIRECTION('ref_axis',(0.990881548486045,0.0059477021680321,0.134604538217762));
#90513=DIRECTION('center_axis',(0.0100961228227622,0.987363722292352,-0.158148500482742));
#90514=DIRECTION('ref_axis',(0.998283786987473,-0.000828739584164497,0.0585559034483356));
#90515=DIRECTION('',(0.68873457818185,0.,0.725013572849964));
#90516=DIRECTION('center_axis',(-0.0168422378220747,0.98736372233166,0.157572900108212));
#90517=DIRECTION('ref_axis',(0.996491852157853,0.0294968921553463,-0.078319358629834));
#90518=DIRECTION('',(-0.725013574350738,0.,0.688734576602022));
#90519=DIRECTION('center_axis',(-1.47951734182214E-14,-1.,1.22598313723652E-15));
#90520=DIRECTION('ref_axis',(1.,-1.47951734182214E-14,-9.56296692960351E-33));
#90521=DIRECTION('center_axis',(0.000293106042264333,-0.987363722206634,
0.158470168041523));
#90522=DIRECTION('ref_axis',(0.999975078494077,-0.000828426208563937,-0.00701114118961083));
#90523=DIRECTION('center_axis',(-0.00706195171612666,-0.987363722497847,
-0.158313007466707));
#90524=DIRECTION('ref_axis',(0.996651285363972,0.00594770418828643,-0.0815526835685473));
#90525=DIRECTION('center_axis',(-0.0241371713095924,0.987363722274126,-0.156621444566684));
#90526=DIRECTION('ref_axis',(0.987532254978932,-0.000828740157184411,-0.157414607219208));
#90527=DIRECTION('',(0.828488832258417,0.,0.560005584635622));
#90528=DIRECTION('center_axis',(0.0174250411497456,0.98736372235522,0.157509516276869));
#90529=DIRECTION('ref_axis',(0.956358079489829,0.029496890978043,-0.290704587540608));
#90530=DIRECTION('',(-0.560005585107112,0.,0.82848883193972));
#90531=DIRECTION('center_axis',(2.83714406763352E-14,-1.,-8.75569054394514E-15));
#90532=DIRECTION('ref_axis',(1.,2.83714406763352E-14,7.62782111538623E-32));
#90533=DIRECTION('center_axis',(0.0343526576848451,-0.98736372221655,0.154702213819542));
#90534=DIRECTION('ref_axis',(0.975089028263676,-0.000828423936585177,-0.221812309562794));
#90535=DIRECTION('center_axis',(-0.04092946378296,-0.987363722509905,-0.153093626470282));
#90536=DIRECTION('ref_axis',(0.955818716277087,0.00594770429341317,-0.293896591385574));
#90537=DIRECTION('center_axis',(-0.0572418406899089,0.987363722281683,-0.147770943004677));
#90538=DIRECTION('ref_axis',(0.930604812491207,-0.000828737692389969,-0.36602458409517));
#90539=DIRECTION('',(0.929503871604654,0.,0.368812354283258));
#90540=DIRECTION('center_axis',(0.050877542500497,0.987363722335174,0.15008116299369));
#90541=DIRECTION('ref_axis',(0.871506065916983,0.0294968919960261,-0.489496793076807));
#90542=DIRECTION('',(-0.36881235729421,0.,0.929503870409956));
#90543=DIRECTION('center_axis',(-6.45647938148473E-15,-1.,3.6625021161468E-15));
#90544=DIRECTION('ref_axis',(1.,-6.45647938148473E-15,3.32938379193174E-32));
#90545=DIRECTION('center_axis',(0.0668059115608821,-0.987363722212296,0.143700557547979));
#90546=DIRECTION('ref_axis',(0.904608900141983,-0.000828426894375263,-0.426241775865285));
#90547=DIRECTION('center_axis',(-0.0728831642277669,-0.987363722545787,
-0.140715755239683));
#90548=DIRECTION('ref_axis',(0.870293125245226,0.00594769960714374,-0.492498224382871));
#90549=DIRECTION('center_axis',(-0.0876699468935738,0.987363722232711,-0.132010834519156));
#90550=DIRECTION('ref_axis',(0.830163322499443,-0.000828733271870356,-0.557519659902545));
#90551=DIRECTION('',(0.987056341368623,0.,0.160373872448067));
#90552=DIRECTION('center_axis',(0.0819510668802593,0.987363722305636,0.135635181689508));
#90553=DIRECTION('ref_axis',(0.745903397621654,0.0294968927910069,-0.665400672326192));
#90554=DIRECTION('',(-0.160373871797992,0.,0.987056341474245));
#90555=DIRECTION('center_axis',(-3.31092047575097E-14,-1.,2.97889624204003E-14));
#90556=DIRECTION('ref_axis',(1.,-3.31092047575097E-14,1.45918977073932E-31));
#90557=DIRECTION('center_axis',(0.0961353978983388,-0.987363722178085,0.125979622945795));
#90558=DIRECTION('ref_axis',(0.791830264249037,-0.000828428021104229,-0.610740653900094));
#90559=DIRECTION('center_axis',(-0.101428922433329,-0.98736372251491,-0.121758174902198));
#90560=DIRECTION('ref_axis',(0.744073595414287,0.00594770212191701,-0.668071185912642));
#90561=DIRECTION('center_axis',(-0.113998699590731,0.987363722223241,-0.110078047444021));
#90562=DIRECTION('ref_axis',(0.690904319089775,-0.000828733047382951,-0.722945734522744));
#90563=DIRECTION('',(0.99845515443243,0.,-0.0555635184929094));
#90564=DIRECTION('center_axis',(0.109192650405688,0.987363722259072,0.114847050741811));
#90565=DIRECTION('ref_axis',(0.585423114535646,0.0294968943341152,-0.810191156574808));
#90566=DIRECTION('',(0.0555635134513151,0.,0.998455154712992));
#90567=DIRECTION('center_axis',(-2.59313835586931E-14,-1.,3.62100133214983E-14));
#90568=DIRECTION('ref_axis',(-3.14205114703E-31,-3.62100133214983E-14,-1.));
#90569=DIRECTION('center_axis',(0.12096970197302,-0.987363722185803,0.102368019009623));
#90570=DIRECTION('ref_axis',(0.642026524434684,-0.000828426218626936,-0.766681978158037));
#90571=DIRECTION('center_axis',(-0.125231977122196,-0.987363722511663,-0.0971073188486758));
#90572=DIRECTION('ref_axis',(0.583062012892976,0.00594770501934991,-0.812405880041617));
#90573=DIRECTION('center_axis',(-0.134996993587324,0.987363722305787,-0.0829981421288752));
#90574=DIRECTION('ref_axis',(0.519339399190732,-0.000828743577750021,-0.854567669428403));
#90575=DIRECTION('',(0.963167313918254,0.,-0.268902817760423));
#90576=DIRECTION('center_axis',(0.131328508942538,0.987363722349456,0.0886887959505408));
#90577=DIRECTION('ref_axis',(0.397569097381128,0.0294968917635576,-0.917098002496922));
#90578=DIRECTION('',(0.26890281566168,0.,0.963167314504194));
#90579=DIRECTION('center_axis',(1.75410397124104E-14,-1.,-4.09379242516552E-14));
#90580=DIRECTION('ref_axis',(2.71847771329592E-32,4.09379242516552E-14,
-1.));
#90581=DIRECTION('center_axis',(0.140147596603562,-0.987363722235991,0.0739697990975683));
#90582=DIRECTION('ref_axis',(0.462202338885112,-0.000828423573841437,-0.886774104066822));
#90583=DIRECTION('center_axis',(-0.143179326464291,-0.987363722500833,-0.0679158299848488));
#90584=DIRECTION('ref_axis',(0.394787097393298,0.00594770447014546,-0.918753379609191));
#90585=DIRECTION('center_axis',(-0.14968299022118,0.987363722223763,-0.0520373180984657));
#90586=DIRECTION('ref_axis',(0.323490742166045,-0.000828732599108519,-0.946230972297536));
#90587=DIRECTION('',(0.882842840276593,0.,-0.469668520738146));
#90588=DIRECTION('center_axis',(0.147323590943391,0.987363722314182,0.0583835542719632));
#90589=DIRECTION('ref_axis',(0.191125190999067,0.0294968922969366,-0.981122364799821));
#90590=DIRECTION('',(0.469668516573729,0.,0.882842842492045));
#90591=DIRECTION('center_axis',(-5.55366423744242E-15,-1.,2.9167748918442E-14));
#90592=DIRECTION('ref_axis',(2.50888775606184E-32,-2.9167748918442E-14,
-1.));
#90593=DIRECTION('center_axis',(0.152772343819061,-0.987363722231285,0.0421128363520289));
#90594=DIRECTION('ref_axis',(0.260766083603314,-0.000828424504378514,-0.965401659080318));
#90595=DIRECTION('center_axis',(-0.154431769537021,-0.98736372252885,-0.0355486707435878));
#90596=DIRECTION('ref_axis',(0.188052374858954,0.00594770257096927,-0.982140992497531));
#90597=DIRECTION('center_axis',(-0.157369969829508,0.987363722258356,-0.0186432980983465));
#90598=DIRECTION('ref_axis',(0.112516019003451,-0.000828734656997782,-0.993649565322948));
#90599=DIRECTION('',(0.761237617213275,0.,-0.64847304503692));
#90600=DIRECTION('',(0.648473045044079,0.,0.761237617207177));
#90601=DIRECTION('',(0.604037768699326,0.,-0.796955691356012));
#90602=DIRECTION('center_axis',(0.158221887796976,0.987363722343933,-0.00887209226136718));
#90603=DIRECTION('ref_axis',(-0.238502061658727,0.0294968912689423,-0.970693927038799));
#90604=DIRECTION('',(0.796955690039799,0.,0.604037770435913));
#90605=DIRECTION('center_axis',(9.00856342149284E-15,-1.,3.60048188131825E-14));
#90606=DIRECTION('ref_axis',(8.38398771006801E-32,-3.60048188131825E-14,
-1.));
#90607=DIRECTION('center_axis',(0.156335146200545,-0.987363722188261,-0.025926861919585));
#90608=DIRECTION('ref_axis',(-0.168696745814464,-0.000828429555302509,-0.985667652739037));
#90609=DIRECTION('center_axis',(-0.155084977231241,-0.987363722540395,0.0325811179728436));
#90610=DIRECTION('ref_axis',(-0.241718585361551,0.00594770165660325,-0.970328166310664));
#90611=DIRECTION('center_axis',(-0.150653235101027,0.987363722265028,0.0491577329475541));
#90612=DIRECTION('ref_axis',(-0.315105849132713,-0.000828737892779795,-0.949056171696838));
#90613=DIRECTION('',(0.41859378419889,0.,-0.908173575826809));
#90614=DIRECTION('center_axis',(0.15261550975314,0.987363722383874,-0.0426776979586559));
#90615=DIRECTION('ref_axis',(-0.441596517075355,0.0294968897379356,-0.896728749178202));
#90616=DIRECTION('',(0.908173574914674,0.,0.418593786177842));
#90617=DIRECTION('center_axis',(3.30758399370139E-15,-1.,6.64529426392992E-15));
#90618=DIRECTION('ref_axis',(-1.48148693090119E-32,-6.64529426392992E-15,
-1.));
#90619=DIRECTION('center_axis',(0.147106607223193,-0.987363722202016,-0.0589281443001684));
#90620=DIRECTION('ref_axis',(-0.376642118627037,-0.000828426419835203,-0.926358477148994));
#90621=DIRECTION('center_axis',(-0.144455199094643,-0.98736372253506,0.065158076063034));
#90622=DIRECTION('ref_axis',(-0.444659213194536,0.00594770107279819,-0.895680081822279));
#90623=DIRECTION('center_axis',(-0.136563586161633,0.987363722257796,0.0803944457279543));
#90624=DIRECTION('ref_axis',(-0.511757872330982,-0.000828736723875154,-0.859129322804611));
#90625=DIRECTION('',(0.213576822851012,0.,-0.976926271906364));
#90626=DIRECTION('center_axis',(0.139873000884617,0.987363722357622,-0.0744877399014954));
#90627=DIRECTION('ref_axis',(-0.624042411827881,0.02949689083002,-0.780833530063485));
#90628=DIRECTION('',(0.976926272040803,0.,0.213576822236072));
#90629=DIRECTION('center_axis',(-0.116088374656384,0.987363722186289,0.107872004616938));
#90630=DIRECTION('ref_axis',(-0.684480663267202,-0.000828733527300141,-0.729030544500044));
#90631=DIRECTION('',(-0.00142675803820793,0.,-0.999998982180232));
#90632=DIRECTION('center_axis',(5.59055571639679E-14,-1.,6.93467795473339E-14));
#90633=DIRECTION('ref_axis',(-7.40605167681581E-31,-6.93467795473339E-14,
-1.));
#90634=DIRECTION('center_axis',(0.13099952945553,-0.987363722173848,-0.0891740064000336));
#90635=DIRECTION('ref_axis',(-0.566976122848868,-0.000828429521764835,-0.823733810052612));
#90636=DIRECTION('center_axis',(-0.127070855582807,-0.987363722543795,0.0946883153610486));
#90637=DIRECTION('ref_axis',(-0.626808068839661,0.00594769944621863,-0.779150992881863));
#90638=DIRECTION('',(0.999998982187443,0.,-0.00142675298437618));
#90639=DIRECTION('center_axis',(0.120590189058315,0.987363722257648,-0.102814815432416));
#90640=DIRECTION('ref_axis',(-0.777308772805231,0.0294968950432108,-0.628427406231488));
#90641=DIRECTION('center_axis',(5.79216856928677E-15,-1.,4.64228725895709E-15));
#90642=DIRECTION('ref_axis',(1.,5.79216856928677E-15,-4.5294716458435E-32));
#90643=DIRECTION('center_axis',(-0.0901850056978048,0.987363722272389,0.130305581951427));
#90644=DIRECTION('ref_axis',(-0.825197905853612,-0.000828740984372925,-0.564843101545194));
#90645=DIRECTION('center_axis',(0.108767053397027,-0.987363722210359,-0.115250198083277));
#90646=DIRECTION('ref_axis',(-0.730798958875046,-0.000828424236561228,-0.682592261471249));
#90647=DIRECTION('center_axis',(-0.103744820254132,-0.987363722562327,0.119791033213271));
#90648=DIRECTION('ref_axis',(-0.77964807635652,0.00594769884537839,-0.626189669279223));
#90649=DIRECTION('',(-0.216363620211502,0.,-0.976312851420575));
#90650=DIRECTION('center_axis',(0.095668712408137,0.987363722216639,-0.126334387704511));
#90651=DIRECTION('ref_axis',(-0.894229041770426,0.0294968962556897,-0.44663671363383));
#90652=DIRECTION('',(0.976312851284768,0.,-0.216363620824314));
#90653=DIRECTION('center_axis',(1.33094108435812E-14,-1.,6.57721627024115E-15));
#90654=DIRECTION('ref_axis',(1.,1.33094108435812E-14,-6.4878940055379E-32));
#90655=DIRECTION('center_axis',(0.0814487538371677,-0.98736372221363,-0.135937414109653));
#90656=DIRECTION('ref_axis',(-0.860450443134181,-0.000828423328988154,-0.509533461732377));
#90657=DIRECTION('center_axis',(-0.0755677974550038,-0.987363722503276,
0.139292453034161));
#90658=DIRECTION('ref_axis',(-0.896032606438773,0.00594770394761603,-0.443948412561966));
#90659=DIRECTION('center_axis',(-0.0600646822450734,0.987363722285192,0.146646220073785));
#90660=DIRECTION('ref_axis',(-0.927329806319798,-0.000828740673294093,-0.374244229748146));
#90661=DIRECTION('',(-0.421183564268117,0.,-0.906975415979069));
#90662=DIRECTION('center_axis',(0.066273868112041,0.987363722344678,-0.143946706121153));
#90663=DIRECTION('ref_axis',(-0.969336154742115,0.0294968920441755,-0.243961784854727));
#90664=DIRECTION('',(0.906975416896828,0.,-0.421183562291816));
#90665=DIRECTION('center_axis',(2.88243025748643E-14,-1.,7.12462940101803E-15));
#90666=DIRECTION('ref_axis',(1.,2.88243025748643E-14,7.26131034139924E-33));
#90667=DIRECTION('center_axis',(0.0503220024830037,-0.987363722218607,-0.150268347008667));
#90668=DIRECTION('ref_axis',(-0.949868222071152,-0.000828424185777103,-0.31264944332712));
#90669=DIRECTION('center_axis',(-0.0438573035848928,-0.987363722504221,
0.152280715801018));
#90670=DIRECTION('ref_axis',(-0.970519647663539,0.00594770305628532,-0.240948621758651));
#90671=DIRECTION('center_axis',(-0.0271357991671827,0.987363722265874,0.156129844542407));
#90672=DIRECTION('ref_axis',(-0.98610079774319,-0.000828739050910494,-0.166146110041224));
#90673=DIRECTION('',(-0.606309431371119,0.,-0.795228818284669));
#90674=DIRECTION('center_axis',(0.0337801347624371,0.98736372233779,-0.154828234849766));
#90675=DIRECTION('ref_axis',(-0.999118186429611,0.029496891799609,-0.0298794732176964));
#90676=DIRECTION('',(0.795228820662645,0.,-0.606309428252191));
#90677=DIRECTION('center_axis',(2.2261493369811E-14,-1.,5.7126488416311E-16));
#90678=DIRECTION('ref_axis',(-0.999670904435999,-2.2268821940597E-14,-0.025653125035977));
#90679=DIRECTION('center_axis',(0.0168422547261848,-0.987363722175753,-0.157572899278337));
#90680=DIRECTION('ref_axis',(-0.994871219550474,-0.000828429980520805,-0.101146281265901));
#90681=DIRECTION('center_axis',(-0.0100960892783663,-0.987363722538625,
0.158148501086643));
#90682=DIRECTION('ref_axis',(-0.999626268953331,0.00594770075836641,-0.026682340117246));
#90683=DIRECTION('center_axis',(0.00706192035904516,0.987363722268906,0.158313010293318));
#90684=DIRECTION('ref_axis',(-0.998762811448472,-0.000828741003265544,0.0497208171281756));
#90685=DIRECTION('',(-0.763084941849124,0.,-0.646298206343728));
#90686=DIRECTION('center_axis',(-0.000293123686553503,0.987363722433932,
-0.158470166592687));
#90687=DIRECTION('ref_axis',(-0.982182562075402,0.0294968878401235,0.185599968649636));
#90688=DIRECTION('',(0.646298209424309,0.,-0.763084939240012));
#90689=DIRECTION('center_axis',(-2.91517827299545E-14,-1.,5.63687199036495E-15));
#90690=DIRECTION('ref_axis',(1.,-2.91517827299545E-14,4.7509437268998E-32));
#90691=DIRECTION('center_axis',(-0.0174250288915529,-0.987363722242448,
-0.157509518339896));
#90692=DIRECTION('ref_axis',(-0.993355143863366,-0.000828424355271347,0.115086367017463));
#90693=DIRECTION('center_axis',(0.0241372029417864,-0.987363722544807,0.15662143798538));
#90694=DIRECTION('ref_axis',(-0.981991476957315,0.00594770218863757,0.188831575807297));
#90695=DIRECTION('center_axis',(0.0409294387520858,0.987363722256636,0.153093634795702));
#90696=DIRECTION('ref_axis',(-0.964723785918027,-0.000828736195093086,0.26326285358992));
#90697=DIRECTION('',(-0.884179450376195,0.,-0.467147406642111));
#90698=DIRECTION('center_axis',(-0.034352670268466,0.987363722389285,-0.154702209922811));
#90699=DIRECTION('ref_axis',(-0.919321172442398,0.0294968898590875,0.39240096252147));
#90700=DIRECTION('',(0.467147409756163,0.,-0.884179448730917));
#90701=DIRECTION('center_axis',(-1.36292347146493E-14,-1.,5.88592831751186E-15));
#90702=DIRECTION('ref_axis',(1.,-1.36292347146493E-14,6.86030150678352E-32));
#90703=DIRECTION('center_axis',(-0.0508775298392963,-0.987363722225418,
-0.150081168007915));
#90704=DIRECTION('ref_axis',(-0.945390886052626,-0.000828426384568328,0.325937703063571));
#90705=DIRECTION('center_axis',(0.0572418717131348,-0.987363722545251,0.14777092922616));
#90706=DIRECTION('ref_axis',(-0.918439854452641,0.00594769839045913,0.395515939801251));
#90707=DIRECTION('center_axis',(0.0728831399834482,0.987363722227794,0.140715770028199));
#90708=DIRECTION('ref_axis',(-0.885575348115344,-0.000828733305052812,0.46449501182628));
#90709=DIRECTION('',(-0.963930709595031,0.,-0.266153315026547));
#90710=DIRECTION('center_axis',(-0.0668059229005943,0.987363722268358,-0.143700551890982));
#90711=DIRECTION('ref_axis',(-0.813473347210432,0.0294968936793228,0.580853722241259));
#90712=DIRECTION('',(0.266153317126985,0.,-0.963930709015074));
#90713=DIRECTION('center_axis',(-1.80679352823365E-14,-1.,1.30173017661079E-14));
#90714=DIRECTION('ref_axis',(1.,-1.80679352823365E-14,-2.73483845405841E-32));
#90715=DIRECTION('center_axis',(-0.0819510561257991,-0.987363722198956,
-0.135635188963959));
#90716=DIRECTION('ref_axis',(-0.853221199866751,-0.000828426942305628,0.521548557477386));
#90717=DIRECTION('center_axis',(0.0876699694749035,-0.987363722548255,0.132010817162542));
#90718=DIRECTION('ref_axis',(-0.811943005497672,0.00594769930014769,0.583706416528414));
#90719=DIRECTION('center_axis',(0.101428901188324,0.987363722241381,0.12175819481815));
#90720=DIRECTION('ref_axis',(-0.765018391449837,-0.000828736539028817,0.644007898972717));
#90721=DIRECTION('',(-0.998609640477332,0.,-0.0527141911228325));
#90722=DIRECTION('center_axis',(-0.0961354100920676,0.987363722345577,-0.125979612328009));
#90723=DIRECTION('ref_axis',(-0.669588411565198,0.0294968912752532,0.742146409074847));
#90724=DIRECTION('',(0.052714190583305,0.,-0.998609640505812));
#90725=DIRECTION('center_axis',(-1.48471818950882E-14,-1.,1.65970364748812E-14));
#90726=DIRECTION('ref_axis',(-2.24967672759341E-32,-1.65970364748812E-14,
-1.));
#90727=DIRECTION('center_axis',(-0.10919264153557,-0.987363722195851,-0.114847059718733));
#90728=DIRECTION('ref_axis',(-0.721155841383537,-0.000828427497757081,0.692772376864352));
#90729=DIRECTION('center_axis',(0.113998717628287,-0.98736372253384,0.110078025978054));
#90730=DIRECTION('ref_axis',(-0.667480603309877,0.00594769975790412,0.744603430741944));
#90731=DIRECTION('center_axis',(0.125231961938295,0.987363722236169,0.0971073412313598));
#90732=DIRECTION('ref_axis',(-0.608690023979306,-0.000828737862473461,0.793407693371842));
#90733=DIRECTION('',(-0.986594694898508,0.,0.163189791341617));
#90734=DIRECTION('center_axis',(-0.120969709327324,0.987363722291078,-0.102368009303536));
#90735=DIRECTION('ref_axis',(-0.494394267007933,0.0294968931826504,0.868737153598406));
#90736=DIRECTION('',(-0.163189789191804,0.,-0.986594695254102));
#90737=DIRECTION('center_axis',(3.64406359406342E-14,-1.,-6.46690406393619E-14));
#90738=DIRECTION('ref_axis',(2.63573539539379E-31,6.46690406393619E-14,
-1.));
#90739=DIRECTION('center_axis',(-0.131328502646515,-0.987363722211956,-0.0886888068043261));
#90740=DIRECTION('ref_axis',(-0.555370033707088,-0.000828425196019373,0.831602933720103));
#90741=DIRECTION('center_axis',(0.134997009525635,-0.987363722493808,0.0829981139683667));
#90742=DIRECTION('ref_axis',(-0.491807552156378,0.00594770592011851,0.870683614429627));
#90743=DIRECTION('center_axis',(0.143179313670225,0.987363722302484,0.0679158598407304));
#90744=DIRECTION('ref_axis',(-0.423899990380177,-0.000828742487650782,0.905708623863975));
#90745=DIRECTION('',(-0.928447676446041,0.,0.371463204236903));
#90746=DIRECTION('center_axis',(-0.140147600709755,0.98736372229544,-0.0739697905241924));
#90747=DIRECTION('ref_axis',(-0.296082794574062,0.0294968934003906,0.954706715194221));
#90748=DIRECTION('',(-0.37146319874419,0.,-0.928447678643624));
#90749=DIRECTION('center_axis',(-1.08433710126974E-14,-1.,3.54953870307208E-14));
#90750=DIRECTION('ref_axis',(9.3471061085303E-32,-3.54953870307208E-14,
-1.));
#90751=DIRECTION('center_axis',(-0.147323588236072,-0.987363722231606,-0.0583835625000502));
#90752=DIRECTION('ref_axis',(-0.363615742431591,-0.000828421653191901,0.931548659799094));
#90753=DIRECTION('center_axis',(0.149682997529542,-0.987363722548287,0.0520372909187366));
#90754=DIRECTION('ref_axis',(-0.293138123667199,0.00594769907183128,0.956051601812698));
#90755=DIRECTION('center_axis',(0.15443176489187,0.987363722239235,0.0355486989672672));
#90756=DIRECTION('ref_axis',(-0.219288862023536,-0.00082873654431964,0.97565962722056));
#90757=DIRECTION('',(-0.826887478900176,0.,0.562367404139065));
#90758=DIRECTION('center_axis',(-0.152772346096393,0.987363722316901,-0.0421128260832527));
#90759=DIRECTION('ref_axis',(-0.0839268221560271,0.0294968927169789,0.996035251305311));
#90760=DIRECTION('',(-0.562367402337263,0.,-0.826887480125585));
#90761=DIRECTION('center_axis',(3.55128005392468E-15,-1.,-4.43958345616782E-14));
#90762=DIRECTION('ref_axis',(4.64735541056336E-32,4.43958345616782E-14,
-1.));
#90763=DIRECTION('center_axis',(-0.156429984571224,-0.987363722264397,-0.0253483704257581));
#90764=DIRECTION('ref_axis',(-0.154859183348945,-0.000828421406732601,0.987936205961939));
#90765=DIRECTION('center_axis',(0.157369971174602,-0.987363722509918,0.0186432734213431));
#90766=DIRECTION('ref_axis',(-0.0807618847282569,0.00594770427846209,0.996715678009008));
#90767=DIRECTION('center_axis',(0.158463155145726,0.987363722292644,0.00151932935097974));
#90768=DIRECTION('ref_axis',(-0.00442403238197619,-0.000828740020282138,
0.999989870512428));
#90769=DIRECTION('',(-0.686662939327357,0.,0.726975933407919));
#90770=DIRECTION('center_axis',(-0.16366813813436,0.986495111156834,0.00633531556422871));
#90771=DIRECTION('ref_axis',(-0.0335577555675336,-0.011985490160195,0.99936491086434));
#90772=DIRECTION('',(-0.649115980606237,0.,-0.760689452879165));
#90773=DIRECTION('',(-0.760689448176683,0.,0.649115986117006));
#90774=DIRECTION('',(0.47041426357662,-5.87988638135427E-14,0.882445704065506));
#90775=DIRECTION('center_axis',(-0.161203571543763,0.986495111286343,-0.0289966192801806));
#90776=DIRECTION('ref_axis',(-0.247607116033172,-0.0119854840352497,0.96878638732291));
#90777=DIRECTION('',(-0.88244570195255,0.,0.470414267540294));
#90778=DIRECTION('',(0.26971649656114,0.,0.962939775626069));
#90779=DIRECTION('center_axis',(-0.151201311299598,0.986495111047301,-0.0629726872624588));
#90780=DIRECTION('ref_axis',(-0.45007863477848,-0.0119854954962003,0.892908489383795));
#90781=DIRECTION('',(-0.96293977383831,0.,0.269716502943784));
#90782=DIRECTION('',(0.0564070978796147,0.,0.998407852187071));
#90783=DIRECTION('center_axis',(-0.134129035688083,0.986495111227673,-0.0940042409111719));
#90784=DIRECTION('ref_axis',(-0.631504978925667,-0.0119854855253044,0.775279181797638));
#90785=DIRECTION('',(-0.998407852456459,0.,0.0564070931114327));
#90786=DIRECTION('',(-0.159539851947166,0.,0.987191488841287));
#90787=DIRECTION('center_axis',(-0.110785028158436,0.986495111480653,-0.120640260944295));
#90788=DIRECTION('ref_axis',(-0.783402851553951,-0.0119854703909857,0.621398680942151));
#90789=DIRECTION('',(-0.987191489609563,0.,-0.159539847193271));
#90790=DIRECTION('',(-0.368026896765542,0.,0.929815144669695));
#90791=DIRECTION('center_axis',(-0.0822608656811558,0.986495111070506,-0.14163525624426));
#90792=DIRECTION('ref_axis',(-0.898669672447652,-0.0119854910711511,0.438462276400848));
#90793=DIRECTION('',(-0.929815148084192,0.,-0.368026888138859));
#90794=DIRECTION('',(-0.559305396851014,0.,0.828961683706388));
#90795=DIRECTION('center_axis',(-0.0498902987825146,0.986495110498608,-0.156007548053709));
#90796=DIRECTION('ref_axis',(-0.971915701787856,-0.0119855316084904,0.235023861874241));
#90797=DIRECTION('',(-0.828961686239684,0.,-0.559305393096348));
#90798=DIRECTION('',(-0.724431406155912,0.,0.689346892192145));
#90799=DIRECTION('center_axis',(-0.0151868356753008,0.986495111189406,-0.163085117719467));
#90800=DIRECTION('ref_axis',(-0.999716036541778,-0.0119854881813905,0.0205959790797065));
#90801=DIRECTION('',(-0.689346895693392,0.,-0.724431402824231));
#90802=DIRECTION('',(-0.855683806145248,-5.87988641770928E-14,0.51749900859884));
#90803=DIRECTION('center_axis',(0.0202266966104539,0.986495111081771,-0.162537000575233));
#90804=DIRECTION('ref_axis',(-0.980770758190615,-0.0119854951240054,-0.194794937780318));
#90805=DIRECTION('',(-0.517499012391679,0.,-0.855683803851421));
#90806=DIRECTION('',(-0.94692537997107,0.,0.3214534566102));
#90807=DIRECTION('center_axis',(0.0546944451109593,0.98649511090908,-0.154388839708337));
#90808=DIRECTION('ref_axis',(-0.915965732122738,-0.0119855084629822,-0.401077455317225));
#90809=DIRECTION('',(-0.321453447458394,0.,-0.94692538307784));
#90810=DIRECTION('',(-0.993889783294678,0.,0.110377074895372));
#90811=DIRECTION('center_axis',(0.0866047677771553,0.98649511109968,-0.139021616933104));
#90812=DIRECTION('ref_axis',(-0.808331161615902,-0.0119854949252138,-0.588606049129707));
#90813=DIRECTION('',(-0.110377078468133,0.,-0.993889782897902));
#90814=DIRECTION('',(-0.994381001341741,0.,-0.105860399444722));
#90815=DIRECTION('center_axis',(0.114465528291893,0.986495110946573,-0.117153911208147));
#90816=DIRECTION('ref_axis',(-0.662899930242844,-0.0119855040691067,-0.748612069216254));
#90817=DIRECTION('',(0.105860400614547,0.,-0.994381001217203));
#90818=DIRECTION('',(-0.948376065643579,0.,-0.317147975106899));
#90819=DIRECTION('center_axis',(0.136974028313873,0.986495111363286,-0.0898081890687445));
#90820=DIRECTION('ref_axis',(-0.486472225758986,-0.0119854780315482,-0.873613828806214));
#90821=DIRECTION('',(0.317147963438495,0.,-0.948376069545629));
#90822=DIRECTION('',(-0.858026121541977,0.,-0.513606050150923));
#90823=DIRECTION('center_axis',(0.153077755278516,0.986495111131323,-0.0582631663479477));
#90824=DIRECTION('ref_axis',(-0.287297626645643,-0.0119854883113736,-0.957766371195877));
#90825=DIRECTION('',(0.513606042133383,0.,-0.858026126341198));
#90826=DIRECTION('',(-0.727555834536971,0.,-0.686048473237286));
#90827=DIRECTION('center_axis',(0.162023739988641,0.986495111162649,-0.0239938186266064));
#90828=DIRECTION('ref_axis',(-0.0746893088985458,-0.011985493682322,-0.997134822918871));
#90829=DIRECTION('',(0.686048470544795,0.,-0.727555837075855));
#90830=DIRECTION('',(-0.563065839593039,0.,-0.826412040257998));
#90831=DIRECTION('center_axis',(0.163393676940142,0.986495111128934,0.0113974582558265));
#90832=DIRECTION('ref_axis',(0.141411395860443,-0.0119854934156252,-0.989878358723124));
#90833=DIRECTION('',(0.826412038991147,0.,-0.563065841452396));
#90834=DIRECTION('',(-0.372247517812012,0.,-0.928133495507406));
#90835=DIRECTION('center_axis',(0.157123506083844,0.986495111154749,0.0462558050810983));
#90836=DIRECTION('ref_axis',(0.350899859315066,-0.0119854902499051,-0.936336284011325));
#90837=DIRECTION('',(0.92813349665939,0.,-0.372247514939744));
#90838=DIRECTION('',(-0.164023309346219,0.,-0.986456463302418));
#90839=DIRECTION('center_axis',(0.143506410560108,0.986495111275205,0.0789512859824004));
#90840=DIRECTION('ref_axis',(0.543980638303175,-0.0119854820197903,-0.839012165210984));
#90841=DIRECTION('',(0.986456463205108,0.,-0.164023309931453));
#90842=DIRECTION('',(0.0518704518711036,0.,-0.998653822013758));
#90843=DIRECTION('center_axis',(0.123179135122855,0.986495110884298,0.10795506876364));
#90844=DIRECTION('ref_axis',(0.711625489987081,-0.0119855067328437,-0.70245676708891));
#90845=DIRECTION('',(0.998653822433025,0.,0.0518704437990247));
#90846=DIRECTION('',(0.265338806748466,0.,-0.964155235236163));
#90847=DIRECTION('center_axis',(0.0970921231458836,0.986495110928653,0.13191101446388));
#90848=DIRECTION('ref_axis',(0.845995519867885,-0.0119855017409327,-0.533055276787957));
#90849=DIRECTION('',(0.964155239221636,0.,0.265338792266545));
#90850=DIRECTION('',(0.466400207442933,0.,-0.884573821960151));
#90851=DIRECTION('center_axis',(0.0664651877326862,0.986495111037399,0.149698946953442));
#90852=DIRECTION('ref_axis',(0.940807742843184,-0.0119854948486083,-0.338728709913328));
#90853=DIRECTION('',(0.884573827264078,0.,0.466400197383513));
#90854=DIRECTION('',(0.64565324338827,0.,-0.763630728364311));
#90855=DIRECTION('center_axis',(0.0327304299207421,0.98649511092306,0.160487118118879));
#90856=DIRECTION('ref_axis',(0.991628840021233,-0.0119855044504921,-0.12856356918354));
#90857=DIRECTION('',(0.763630725765876,0.,0.645653246461506));
#90858=DIRECTION('',(0.794716263103415,0.,-0.606981104449672));
#90859=DIRECTION('center_axis',(-0.0025347845356527,0.986495111068613,0.16377109239754));
#90860=DIRECTION('ref_axis',(0.996082475343742,-0.011985496666978,0.0876130708440827));
#90861=DIRECTION('',(0.606981103327021,0.,0.794716263960863));
#90862=DIRECTION('',(0.906619240092249,0.,-0.421949704934786));
#90863=DIRECTION('center_axis',(-0.0376814598423203,0.986495110935352,0.159397313919649));
#90864=DIRECTION('ref_axis',(0.953960400957062,-0.0119855033800166,0.299693011454338));
#90865=DIRECTION('',(0.421949718059285,0.,0.906619233983975));
#90866=DIRECTION('',(0.976129695249212,0.,-0.217188439040112));
#90867=DIRECTION('center_axis',(-0.0710662151983521,0.986495111309187,0.147570282985618));
#90868=DIRECTION('ref_axis',(0.867232196854255,-0.0119854844820484,0.497759645713745));
#90869=DIRECTION('',(0.217188431817788,0.,0.976129696856176));
#90870=DIRECTION('',(0.999997419781085,0.,-0.00227165824295009));
#90871=DIRECTION('center_axis',(-0.101127941833338,0.986495110572297,0.128843068100324));
#90872=DIRECTION('ref_axis',(0.739953182791551,-0.0119855304879602,0.67255158488816));
#90873=DIRECTION('',(0.0022716547051695,0.,0.999997419789121));
#90874=DIRECTION('',(0.97710637494025,-5.87988649286476E-14,0.21275133854132));
#90875=DIRECTION('center_axis',(-0.126461110862709,0.986495111429362,0.10409122232609));
#90876=DIRECTION('ref_axis',(0.578074774319208,-0.0119854720937904,0.815895767702276));
#90877=DIRECTION('',(-0.212751343062777,0.,0.977106373955766));
#90878=DIRECTION('',(0.908526924453842,0.,0.417826312649698));
#90879=DIRECTION('center_axis',(-0.145881042620839,0.986495110847264,0.0744722611332655));
#90880=DIRECTION('ref_axis',(0.389166237075605,-0.0119855091973612,0.921089565400506));
#90881=DIRECTION('',(-0.417826321376943,0.,0.908526920440232));
#90882=DIRECTION('',(0.797465763094675,5.87988639674914E-14,0.603364199047166));
#90883=DIRECTION('center_axis',(-0.158479760463402,0.986495111024107,0.0413710218510204));
#90884=DIRECTION('ref_axis',(0.182060721254228,-0.0119855011715295,0.983214239897927));
#90885=DIRECTION('',(-0.603364204891872,0.,0.797465758672558));
#90886=DIRECTION('center_axis',(-0.163746597512067,-0.986495108034302,0.00380179268390596));
#90887=DIRECTION('ref_axis',(0.0283600360616785,-0.000855145953452464,0.999597407499629));
#90888=DIRECTION('center_axis',(0.162375635431753,-0.986495109483943,-0.0214837608997425));
#90889=DIRECTION('ref_axis',(0.136269316546588,0.000855014963594679,0.990671460332505));
#90890=DIRECTION('center_axis',(-0.159101026864079,-0.986495107934883,0.0389135615350055));
#90891=DIRECTION('ref_axis',(0.242580940584724,-0.000855181560874777,0.97013079320756));
#90892=DIRECTION('center_axis',(0.153961009504166,-0.986495109500042,-0.0558874447882335));
#90893=DIRECTION('ref_axis',(0.346048496507044,0.000855014604045322,0.938216236810705));
#90894=DIRECTION('center_axis',(-0.147016064197888,-0.986495108037815,0.0722058078358147));
#90895=DIRECTION('ref_axis',(0.445458974655576,-0.000855174140654233,0.895301943802197));
#90896=DIRECTION('center_axis',(0.138347337083997,-0.986495109514399,-0.0876778947394444));
#90897=DIRECTION('ref_axis',(0.539646833411019,0.000855013109175183,0.841891064296351));
#90898=DIRECTION('center_axis',(-0.128056799604856,-0.986495107974529,0.102121780327624));
#90899=DIRECTION('ref_axis',(0.627507843518583,-0.000855179310340608,0.778609770675275));
#90900=DIRECTION('center_axis',(0.11626469994015,-0.98649510947649,-0.115368620199751));
#90901=DIRECTION('ref_axis',(0.708011881683628,0.000855015934826577,0.706200003074597));
#90902=DIRECTION('center_axis',(-0.103109737085179,-0.986495108050338,0.127262657173965));
#90903=DIRECTION('ref_axis',(0.780215142492183,-0.00085517714781326,0.625510671450094));
#90904=DIRECTION('center_axis',(0.088745649050942,-0.986495109536929,-0.137664841678073));
#90905=DIRECTION('ref_axis',(0.843271084078966,0.000855012026633975,0.537487811685735));
#90906=DIRECTION('center_axis',(-0.0733413800842794,-0.986495108018088,
0.146452872364165));
#90907=DIRECTION('ref_axis',(0.896440450959432,-0.000855178141471557,0.443163385845443));
#90908=DIRECTION('center_axis',(0.0570769521492894,-0.986495109556937,-0.153524005789303));
#90909=DIRECTION('ref_axis',(0.939099866070296,0.000855010557289998,0.343643289624137));
#90910=DIRECTION('center_axis',(-0.0401436454668397,-0.986495108155403,
0.158795117412634));
#90911=DIRECTION('ref_axis',(0.970749199943287,-0.000855162464340449,0.24009427212374));
#90912=DIRECTION('center_axis',(0.0227394040315997,-0.986495109510181,-0.162204557324335));
#90913=DIRECTION('ref_axis',(0.991017381969255,0.000855012561476741,0.133730391416173));
#90914=DIRECTION('center_axis',(-0.00506887156786354,-0.986495107936793,
0.16371227369322));
#90915=DIRECTION('ref_axis',(0.999666794490313,-0.000855181416868911,0.0257986173700359));
#90916=DIRECTION('center_axis',(-0.0126614160523676,-0.986495109506412,
-0.163300604602312));
#90917=DIRECTION('ref_axis',(0.996596027291127,0.000855012433976403,-0.0824355951108559));
#90918=DIRECTION('center_axis',(0.0302429388489829,-0.986495108017901,0.160974428113681));
#90919=DIRECTION('ref_axis',(0.98184108050694,-0.000855177729948001,-0.189703350787523));
#90920=DIRECTION('center_axis',(-0.0474702014878469,-0.98649510952696,-0.156760897069694));
#90921=DIRECTION('ref_axis',(0.955574949598001,0.000855013104886688,-0.294746984129386));
#90922=DIRECTION('center_axis',(0.0641406153199245,-0.986495107947539,0.150709599767088));
#90923=DIRECTION('ref_axis',(0.918105569468972,-0.000855182164299372,-0.396334999682744));
#90924=DIRECTION('center_axis',(-0.0800593341064972,-0.986495109508332,
-0.14289122414819));
#90925=DIRECTION('ref_axis',(0.869872250224507,0.000855012302154065,-0.493276329498301));
#90926=DIRECTION('center_axis',(0.0950391544766352,-0.986495107995121,0.133397754921367));
#90927=DIRECTION('ref_axis',(0.811440461235714,-0.000855179597100089,-0.584434467273644));
#90928=DIRECTION('center_axis',(-0.108904979399598,-0.986495109505147,-0.122340117640953));
#90929=DIRECTION('ref_axis',(0.743495289462457,0.000855014424802706,-0.668740624979125));
#90930=DIRECTION('center_axis',(0.121493764696541,-0.986495107991742,0.109848382091963));
#90931=DIRECTION('ref_axis',(0.666833302232419,-0.000855180911470078,-0.745206424891396));
#90932=DIRECTION('center_axis',(-0.132658350585395,-0.986495109509689,-0.096068522073723));
#90933=DIRECTION('ref_axis',(0.582353317866532,0.000855013809294289,-0.812935349287524));
#90934=DIRECTION('center_axis',(0.142267467271949,-0.986495108042873,0.0811626118573438));
#90935=DIRECTION('ref_axis',(0.491045754943609,-0.000855172111768815,-0.871133362483908));
#90936=DIRECTION('center_axis',(-0.15020876295495,-0.98649510946296,-0.065304873763033));
#90937=DIRECTION('ref_axis',(0.393981151766117,0.000855018383492621,-0.919118121351444));
#90938=DIRECTION('center_axis',(0.156388895407794,-0.986495108044346,0.0486817748002624));
#90939=DIRECTION('ref_axis',(0.292297455320061,-0.000855171931315512,-0.956327070773585));
#90940=DIRECTION('center_axis',(-0.160735584061753,-0.986495109510977,-0.0314876313375955));
#90941=DIRECTION('ref_axis',(0.187186863093603,0.000855011532842735,-0.982323952288885));
#90942=DIRECTION('center_axis',(0.163197752237843,-0.986495107978401,0.0139246400024645));
#90943=DIRECTION('ref_axis',(0.0798816522042827,-0.00085517970948843,-0.996803987907742));
#90944=DIRECTION('center_axis',(-0.163746585445659,-0.986495109509131,0.00380192970154928));
#90945=DIRECTION('ref_axis',(-0.0283600731337881,0.000855012924968857,-0.999597406561634));
#90946=DIRECTION('center_axis',(0.162375666692026,-0.986495107908973,-0.0214835969517151));
#90947=DIRECTION('ref_axis',(-0.136269329215492,-0.000855186051645274,-0.990671458442191));
#90948=DIRECTION('center_axis',(-0.159100978613244,-0.986495109517671,0.038913718686673));
#90949=DIRECTION('ref_axis',(-0.242580928943249,0.000855013151542972,-0.970130796266947));
#90950=DIRECTION('center_axis',(0.153961071525624,-0.986495108040822,-0.0558872996861401));
#90951=DIRECTION('ref_axis',(-0.346048507034067,-0.000855176233634949,-0.938216232780643));
#90952=DIRECTION('center_axis',(-0.147015987202403,-0.986495109509439,0.0722059444980999));
#90953=DIRECTION('ref_axis',(-0.44545896531509,0.000855013599121798,-0.895301948602903));
#90954=DIRECTION('center_axis',(0.138347433851548,-0.98649510792198,-0.0876777599662118));
#90955=DIRECTION('ref_axis',(-0.53964684376128,-0.000855183119961669,-0.841891057489222));
#90956=DIRECTION('center_axis',(-0.128056690864764,-0.986495109522306,0.102121901731897));
#90957=DIRECTION('ref_axis',(-0.627507834604862,0.000855012399275419,-0.778609778042451));
#90958=DIRECTION('center_axis',(0.11626481501738,-0.986495107985349,-0.115368516979069));
#90959=DIRECTION('ref_axis',(-0.708011890947838,-0.000855174620436058,-0.706199993594474));
#90960=DIRECTION('center_axis',(-0.103109611601658,-0.986495109457592,0.127262747933594));
#90961=DIRECTION('ref_axis',(-0.780215135878132,0.000855018570317058,-0.625510679916748));
#90962=DIRECTION('center_axis',(0.0887457784508654,-0.986495108087938,-0.137664768643676));
#90963=DIRECTION('ref_axis',(-0.843271090120732,-0.000855164333534696,-0.53748780196443));
#90964=DIRECTION('center_axis',(-0.0733412334058362,-0.98649510949555,0.146452935866354));
#90965=DIRECTION('ref_axis',(-0.896440445725003,0.000855014316550816,-0.443163396749862));
#90966=DIRECTION('center_axis',(0.0570771080566019,-0.986495108025782,-0.153523957664907));
#90967=DIRECTION('ref_axis',(-0.939099869820112,-0.000855177615941849,-0.343643278961039));
#90968=DIRECTION('center_axis',(-0.0401435003578533,-0.986495109535651,
0.158795145521716));
#90969=DIRECTION('ref_axis',(-0.970749197330676,0.00085501093554261,-0.24009428322671));
#90970=DIRECTION('center_axis',(0.0227395578524956,-0.986495108067061,-0.162204544536924));
#90971=DIRECTION('ref_axis',(-0.991017383362208,-0.000855170717919725,-0.133730380082331));
#90972=DIRECTION('center_axis',(-0.00506870820541044,-0.986495109499761,
0.163712269333069));
#90973=DIRECTION('ref_axis',(-0.999666794273265,0.000855013666306463,-0.0257986313405084));
#90974=DIRECTION('center_axis',(-0.0126612612176662,-0.986495108032662,
-0.163300625510142));
#90975=DIRECTION('ref_axis',(-0.996596026193594,-0.000855172538075693,0.0824356067186258));
#90976=DIRECTION('center_axis',(0.0302430947892424,-0.986495109526178,0.160974389573322));
#90977=DIRECTION('ref_axis',(-0.981841082996727,0.000855013054772608,0.1897033386435));
#90978=DIRECTION('center_axis',(-0.047470051408464,-0.986495108004711,-0.156760952096022));
#90979=DIRECTION('ref_axis',(-0.955574946429071,-0.00085517663212848,0.2947469939287));
#90980=DIRECTION('center_axis',(0.0641407625449427,-0.986495109514227,0.150709526854366));
#90981=DIRECTION('ref_axis',(-0.91810557395525,0.000855014026993956,0.396334989653089));
#90982=DIRECTION('center_axis',(-0.0800591980642029,-0.986495108016899,
-0.142891310666684));
#90983=DIRECTION('ref_axis',(-0.86987224425126,-0.000855177493715284,0.493276339745513));
#90984=DIRECTION('center_axis',(0.0950392813517479,-0.98649510950768,0.13339765334358));
#90985=DIRECTION('ref_axis',(-0.811440468144587,0.00085501312675468,0.584434457924793));
#90986=DIRECTION('center_axis',(-0.108904866952338,-0.986495107973881,-0.122340230086816));
#90987=DIRECTION('ref_axis',(-0.743495281044057,-0.000855177465418444,0.668740634130094));
#90988=DIRECTION('center_axis',(0.12149386579588,-0.986495109470824,0.109848256991724));
#90989=DIRECTION('ref_axis',(-0.666833310280483,0.000855016297068395,0.745206417878634));
#90990=DIRECTION('center_axis',(-0.132658262045057,-0.98649510792685,-0.0960686605901103));
#90991=DIRECTION('ref_axis',(-0.582353307756762,-0.000855182272220577,0.812935356352545));
#90992=DIRECTION('center_axis',(0.14226753416166,-0.986495109469175,0.0811624772722081));
#90993=DIRECTION('ref_axis',(-0.491045764644718,0.000855018131842603,0.871133357166673));
#90994=DIRECTION('center_axis',(-0.150208707700356,-0.986495107964131,-0.0653050234961099));
#90995=DIRECTION('ref_axis',(-0.393981140864148,-0.00085518191775455,0.919118125872443));
#90996=DIRECTION('center_axis',(0.156388933396878,-0.986495109534142,0.0486816225716499));
#90997=DIRECTION('ref_axis',(-0.292297465065824,0.000855011415688201,0.956327067938356));
#90998=DIRECTION('center_axis',(-0.160735562560586,-0.986495108038274,-0.0314877872338775));
#90999=DIRECTION('ref_axis',(-0.187186850714603,-0.000855172938858934,0.982323954507266));
#91000=DIRECTION('center_axis',(0.163197751262729,-0.986495109399359,0.0139245507624154));
#91001=DIRECTION('ref_axis',(-0.0798816770250956,0.000855085481519109,0.996803985999493));
#91002=DIRECTION('center_axis',(0.158463153892069,0.987363722548616,0.00151929375646194));
#91003=DIRECTION('ref_axis',(0.101017485130246,-0.0177430368692817,0.994726420851792));
#91004=DIRECTION('',(-0.604037770435915,0.,0.796955690039797));
#91005=DIRECTION('center_axis',(-0.15633514620055,0.987363722188261,0.0259268619195614));
#91006=DIRECTION('ref_axis',(0.240670182334486,0.0126220391173118,0.970524882454647));
#91007=DIRECTION('',(-0.796955691356011,0.,-0.604037768699328));
#91008=DIRECTION('center_axis',(-7.96270415248623E-15,1.,-3.17928001485767E-14));
#91009=DIRECTION('ref_axis',(3.14577109114985E-32,3.17928001485767E-14,
1.));
#91010=DIRECTION('center_axis',(0.184642396044489,-0.982569664103368,0.0215416054820449));
#91011=DIRECTION('ref_axis',(0.0522415413826683,0.031699892166001,0.998131222931447));
#91012=DIRECTION('center_axis',(1.88381627626997E-28,-1.,-3.78747958921603E-15));
#91013=DIRECTION('ref_axis',(-4.9737991503207E-14,-3.78747958921603E-15,
1.));
#91014=DIRECTION('center_axis',(-0.162390103070865,-0.98367345539406,0.0775627976399995));
#91015=DIRECTION('ref_axis',(0.394106230517453,0.0074048752412329,0.919035062927409));
#91016=DIRECTION('center_axis',(0.155084977674505,0.987363722502644,-0.0325811170069363));
#91017=DIRECTION('ref_axis',(0.312492526540577,-0.0177430400714078,0.949754497428315));
#91018=DIRECTION('',(-0.418593786177838,0.,0.908173574914676));
#91019=DIRECTION('center_axis',(9.0085634535061E-16,-1.,3.60048189652994E-15));
#91020=DIRECTION('ref_axis',(8.38412477077618E-34,-3.60048189652994E-15,
-1.));
#91021=DIRECTION('center_axis',(0.15065330845072,-0.987363724130564,-0.0491574706822454));
#91022=DIRECTION('ref_axis',(0.31510504360133,0.000828877171355419,0.949056439027542));
#91023=DIRECTION('center_axis',(-0.158221887569141,-0.987363722368478,0.0088720935928883));
#91024=DIRECTION('ref_axis',(0.166010951647992,-0.0177432069293348,0.985964270417945));
#91025=DIRECTION('center_axis',(-0.147106607223195,0.987363722202016,0.0589281443001649));
#91026=DIRECTION('ref_axis',(0.443677608797757,0.0126220360875831,0.896097574852487));
#91027=DIRECTION('',(-0.90817357582681,0.,-0.418593784198889));
#91028=DIRECTION('center_axis',(0.,1.,0.));
#91029=DIRECTION('ref_axis',(0.,0.,1.));
#91030=DIRECTION('center_axis',(0.184956602125193,-0.982569635358866,-0.0186538736204669));
#91031=DIRECTION('ref_axis',(0.265588707980032,0.0317007184657399,0.963565100365436));
#91032=DIRECTION('center_axis',(6.63290272699835E-29,-1.,5.33427468744545E-15));
#91033=DIRECTION('ref_axis',(1.24344978758017E-14,5.33427468744545E-15,
1.));
#91034=DIRECTION('center_axis',(-0.141919738091628,-0.983673454952057,0.110658582869502));
#91035=DIRECTION('ref_axis',(0.582457617398201,0.00740498728053316,0.812827343350472));
#91036=DIRECTION('center_axis',(0.144455200230007,0.987363722485691,-0.0651580742940492));
#91037=DIRECTION('ref_axis',(0.509355769148195,-0.0177430407164443,0.860373107983731));
#91038=DIRECTION('',(-0.213576824979769,0.,0.976926271440973));
#91039=DIRECTION('center_axis',(-6.61516801299152E-15,-1.,-1.32905885845373E-14));
#91040=DIRECTION('ref_axis',(3.63699579032327E-32,1.32905885845373E-14,
-1.));
#91041=DIRECTION('center_axis',(0.136563713886832,-0.987363724124565,-0.0803942058379));
#91042=DIRECTION('ref_axis',(0.511757143220611,0.000828875461218203,0.859129756979787));
#91043=DIRECTION('center_axis',(-0.152615509753122,-0.987363722383875,0.042677697958692));
#91044=DIRECTION('ref_axis',(0.374082881170212,-0.0177432067346035,0.927225526304235));
#91045=DIRECTION('center_axis',(-0.130999529455584,0.987363722173848,0.0891740063999588));
#91046=DIRECTION('ref_axis',(0.625939162818685,0.0126220395445972,0.779769740736058));
#91047=DIRECTION('',(-0.976926272506191,0.,-0.213576820107329));
#91048=DIRECTION('center_axis',(4.11524096047451E-14,1.,5.10218223628352E-14));
#91049=DIRECTION('ref_axis',(2.86061668474823E-31,-5.10218223628352E-14,
1.));
#91050=DIRECTION('center_axis',(0.176622045565574,-0.982569659761808,-0.0579785885978333));
#91051=DIRECTION('ref_axis',(0.466517537295754,0.0317000146039319,0.883943717930964));
#91052=DIRECTION('center_axis',(1.81653712354604E-28,-1.,-3.78747958921603E-15));
#91053=DIRECTION('ref_axis',(-4.79616346638068E-14,-3.78747958921603E-15,
1.));
#91054=DIRECTION('center_axis',(-0.114813486257611,-0.983673455401698,0.138579928241639));
#91055=DIRECTION('ref_axis',(0.743573933005707,0.00740488385359206,0.668612723367975));
#91056=DIRECTION('center_axis',(0.127070856773876,0.987363722510942,-0.0946883141052263));
#91057=DIRECTION('ref_axis',(0.682402099044296,-0.0177430385966853,0.730761629945973));
#91058=DIRECTION('',(0.00142675585917094,0.,0.999998982183341));
#91059=DIRECTION('center_axis',(2.32939818588969E-15,-1.,2.88944910854677E-15));
#91060=DIRECTION('ref_axis',(-4.09201826591339E-33,-2.88944910854677E-15,
-1.));
#91061=DIRECTION('center_axis',(0.116088551147125,-0.987363724096045,-0.107871797202751));
#91062=DIRECTION('ref_axis',(0.684480046866591,0.000828873339334421,0.729031123073972));
#91063=DIRECTION('center_axis',(-0.139873024001403,-0.987363721404996,0.0744877091202357));
#91064=DIRECTION('ref_axis',(0.564663102944633,-0.0177432449166011,0.825130751719246));
#91065=DIRECTION('center_axis',(-0.108767053397066,0.987363722210358,0.115250198083242));
#91066=DIRECTION('ref_axis',(0.778932498160699,0.0126220337349359,0.626980739395977));
#91067=DIRECTION('',(-0.999998982184334,0.,0.00142675516336331));
#91068=DIRECTION('center_axis',(-1.2789618240954E-13,1.,-1.02456022673949E-13));
#91069=DIRECTION('ref_axis',(-1.,-1.2789618240954E-13,-2.64322747769899E-31));
#91070=DIRECTION('center_axis',(0.16002890506933,-0.982569666692213,-0.094591752487546));
#91071=DIRECTION('ref_axis',(0.645632421359425,0.031699816815584,0.762990103542257));
#91072=DIRECTION('center_axis',(9.0826856177302E-29,-1.,-3.78747958921603E-15));
#91073=DIRECTION('ref_axis',(-2.39808173319034E-14,-3.78747958921603E-15,
1.));
#91074=DIRECTION('center_axis',(-0.0823386068103901,-0.983673455332332,
0.160021520749787));
#91075=DIRECTION('ref_axis',(0.869921560179819,0.00740490164403627,0.493134511635469));
#91076=DIRECTION('center_axis',(0.10374482146474,0.987363722520539,-0.119791032509259));
#91077=DIRECTION('ref_axis',(0.823540067399997,-0.0177430379354208,0.566980548159839));
#91078=DIRECTION('',(0.21636361808406,0.,0.976312851892043));
#91079=DIRECTION('center_axis',(-5.79216859279781E-15,-1.,-4.64228727930433E-15));
#91080=DIRECTION('ref_axis',(1.,-5.79216859279781E-15,2.18142135758451E-32));
#91081=DIRECTION('center_axis',(0.0901852223248424,-0.987363724138682,-0.13030541788127));
#91082=DIRECTION('ref_axis',(0.825197426429906,0.00082887969264323,0.564843801746921));
#91083=DIRECTION('center_axis',(-0.120590218143034,-0.987363721307667,0.102814790442288));
#91084=DIRECTION('ref_axis',(0.72884031643368,-0.017743249949096,0.68445377508061));
#91085=DIRECTION('center_axis',(-0.0814487538372487,0.987363722213629,0.135937414109611));
#91086=DIRECTION('ref_axis',(0.895503814866252,0.0126220332170288,0.444874815917308));
#91087=DIRECTION('',(-0.976312850813305,0.,0.216363622951729));
#91088=DIRECTION('center_axis',(0.,1.,0.));
#91089=DIRECTION('ref_axis',(0.,0.,1.));
#91090=DIRECTION('center_axis',(0.135953801314679,-0.982569636304925,-0.126781204126226));
#91091=DIRECTION('ref_axis',(0.794558088009599,0.0317006896209387,0.606360050676236));
#91092=DIRECTION('center_axis',(-3.13926580987588E-28,-1.,1.4137996331574E-14));
#91093=DIRECTION('ref_axis',(-2.22044604925032E-14,1.4137996331574E-14,
1.));
#91094=DIRECTION('center_axis',(-0.0460137206069841,-0.983673455505685,
0.17398066113625));
#91095=DIRECTION('ref_axis',(0.955592620402268,0.00740485812587767,0.294597881711432));
#91096=DIRECTION('center_axis',(0.0755677989895925,0.987363722458875,-0.139292452516357));
#91097=DIRECTION('ref_axis',(0.926170215102622,-0.0177430427789482,0.376688089922825));
#91098=DIRECTION('',(0.421183562291818,0.,0.906975416896828));
#91099=DIRECTION('center_axis',(-3.32735272456251E-15,-1.,-1.64430407496874E-15));
#91100=DIRECTION('ref_axis',(1.,-3.32735272456251E-15,-4.05495624528595E-33));
#91101=DIRECTION('center_axis',(0.0600649742539953,-0.987363724111366,-0.146646088174221));
#91102=DIRECTION('ref_axis',(0.927329485697342,0.00082892748148247,0.374245023795285));
#91103=DIRECTION('center_axis',(-0.0956687490241227,-0.987363721208003,
0.126334367859443));
#91104=DIRECTION('ref_axis',(0.858937762698334,-0.017743254060679,0.511772504875085));
#91105=DIRECTION('center_axis',(-0.0503220025106176,0.987363722217997,0.150268347003433));
#91106=DIRECTION('ref_axis',(0.970202368441141,0.0126220344007601,0.24196704014966));
#91107=DIRECTION('',(-0.906975415979067,0.,0.421183564268121));
#91108=DIRECTION('center_axis',(-3.1819119793911E-14,1.,-7.85687094207709E-15));
#91109=DIRECTION('ref_axis',(-1.,-3.1819119793911E-14,-5.25025999428999E-32));
#91110=DIRECTION('center_axis',(0.105520483328886,-0.982569658070307,-0.153043440361353));
#91111=DIRECTION('ref_axis',(0.906331316741022,0.0317000622763659,0.421377088065025));
#91112=DIRECTION('center_axis',(0.,-1.,-3.78747958921603E-15));
#91113=DIRECTION('ref_axis',(0.,-3.78747958921603E-15,1.));
#91114=DIRECTION('center_axis',(-0.00753719114751718,-0.983673455252781,
0.179804683422486));
#91115=DIRECTION('ref_axis',(0.996581232016566,0.00740491377047555,0.0822861789390829));
#91116=DIRECTION('center_axis',(0.0438573044439995,0.987363722468911,-0.152280715782539));
#91117=DIRECTION('ref_axis',(0.985493674732238,-0.0177430411866941,0.16878211265474));
#91118=DIRECTION('',(0.60630942963828,0.,0.795228819605844));
#91119=DIRECTION('center_axis',(-1.08091135104046E-14,-1.,-2.67173603827549E-15));
#91120=DIRECTION('ref_axis',(1.,-1.08091135104046E-14,1.06766753801264E-32));
#91121=DIRECTION('center_axis',(0.0271360641083462,-0.987363724133007,-0.15612978668693));
#91122=DIRECTION('ref_axis',(0.986100656652269,0.000828877203283326,0.166146946744577));
#91123=DIRECTION('center_axis',(-0.0662738681119184,-0.987363722344681,
0.143946706121192));
#91124=DIRECTION('ref_axis',(0.948872239264686,-0.0177432091114833,0.315161311209428));
#91125=DIRECTION('',(-0.795228819341497,0.,0.606309429984995));
#91126=DIRECTION('center_axis',(-1.96585202152636E-13,1.,-4.99806869102813E-15));
#91127=DIRECTION('ref_axis',(0.999676955525532,1.96648728437366E-13,0.0254162269269747));
#91128=DIRECTION('center_axis',(0.0701542349175453,-0.98256963793636,-0.172149034062771));
#91129=DIRECTION('ref_axis',(0.975725371780959,0.0317006430670899,0.216691181389651));
#91130=DIRECTION('center_axis',(0.0312917311449239,-0.983673455209738,0.177221220731855));
#91131=DIRECTION('ref_axis',(0.990970812698885,0.00740492932440456,-0.133873131735283));
#91132=DIRECTION('',(0.763084940440831,0.,0.646298208006501));
#91133=DIRECTION('center_axis',(0.0174250288914855,0.987363722242448,0.157509518339908));
#91134=DIRECTION('ref_axis',(0.98213114496707,0.0126220340066069,-0.187774061955342));
#91135=DIRECTION('',(-0.646298207761542,0.,0.763084940648299));
#91136=DIRECTION('center_axis',(-1.93063591611731E-13,1.,3.73787918254193E-14));
#91137=DIRECTION('ref_axis',(-1.,-1.93063591611731E-13,-9.54092960034444E-32));
#91138=DIRECTION('center_axis',(0.0315066138997435,-0.982569654868572,-0.183205367312284));
#91139=DIRECTION('ref_axis',(0.999495669260652,0.0317001500081216,0.0018728637601358));
#91140=DIRECTION('center_axis',(2.96028271985281E-28,-1.,-3.78747958921603E-15));
#91141=DIRECTION('ref_axis',(-7.8159700933611E-14,-3.78747958921603E-15,
1.));
#91142=DIRECTION('center_axis',(0.068657441857252,-0.983673455295322,0.166351101664464));
#91143=DIRECTION('ref_axis',(0.939023699618817,0.007404896535104,-0.343772685159094));
#91144=DIRECTION('center_axis',(-0.0241372015785544,0.98736372250249,-0.156621438462242));
#91145=DIRECTION('ref_axis',(0.965279604598994,-0.017743041285082,-0.260615558689739));
#91146=DIRECTION('',(0.88417944935828,0.,0.46714740856874));
#91147=DIRECTION('center_axis',(1.82198642830546E-14,-1.,-3.52304500584695E-15));
#91148=DIRECTION('ref_axis',(1.,1.82198642830546E-14,1.85586446763344E-32));
#91149=DIRECTION('center_axis',(-0.040929172955792,-0.987363724123068,-0.153093693818459));
#91150=DIRECTION('ref_axis',(0.964724009230363,0.00082887542359837,-0.263262034824671));
#91151=DIRECTION('center_axis',(0.000293123686674066,-0.987363722433934,
0.158470166592671));
#91152=DIRECTION('ref_axis',(0.993505920544914,-0.0177432049224071,-0.112388453683129));
#91153=DIRECTION('center_axis',(0.0508775298393055,0.987363722225417,0.150081168007913));
#91154=DIRECTION('ref_axis',(0.918803591899418,0.0126220361989575,-0.394513173056262));
#91155=DIRECTION('',(-0.467147407829532,0.,0.884179449748833));
#91156=DIRECTION('center_axis',(-1.50428781314511E-13,1.,6.50065517177513E-14));
#91157=DIRECTION('ref_axis',(-1.,-1.50428781314511E-13,-4.30966703185921E-32));
#91158=DIRECTION('center_axis',(-0.00861387361504059,-0.982569659926227,
-0.185695084947884));
#91159=DIRECTION('ref_axis',(0.976530624481854,0.0317000071570993,-0.213032976309585));
#91160=DIRECTION('center_axis',(0.,-1.,-3.78747958921603E-15));
#91161=DIRECTION('ref_axis',(0.,-3.78747958921603E-15,1.));
#91162=DIRECTION('center_axis',(0.102812836377922,-0.983673455335804,0.147702586110218));
#91163=DIRECTION('ref_axis',(0.843168882821576,0.00740489427710891,-0.537597807456616));
#91164=DIRECTION('center_axis',(-0.057241870175252,0.987363722501593,-0.147770930113592));
#91165=DIRECTION('ref_axis',(0.886687262551847,-0.0177430376327503,-0.462029093287289));
#91166=DIRECTION('',(0.963930709015073,0.,0.266153317126987));
#91167=DIRECTION('center_axis',(-1.02219260794816E-14,-1.,4.41444625500047E-15));
#91168=DIRECTION('ref_axis',(1.,-1.02219260794816E-14,6.68170667667052E-33));
#91169=DIRECTION('center_axis',(-0.0728828940410096,-0.987363724094902,
-0.140715884311807));
#91170=DIRECTION('ref_axis',(0.885575742122918,0.000828871478840528,-0.464494260390282));
#91171=DIRECTION('center_axis',(0.0343526343809698,-0.98736372143583,0.154702223977148));
#91172=DIRECTION('ref_axis',(0.946118111358501,-0.0177432443320615,-0.323335269712409));
#91173=DIRECTION('center_axis',(0.0819510561257198,0.987363722198955,0.135635188964013));
#91174=DIRECTION('ref_axis',(0.812513804514755,0.0126220362890575,-0.582805286243079));
#91175=DIRECTION('',(-0.266153315026551,0.,0.96393070959503));
#91176=DIRECTION('center_axis',(-1.59524822387274E-13,1.,1.14989370356372E-13));
#91177=DIRECTION('ref_axis',(-1.,-1.59524822387274E-13,-4.15996612950641E-31));
#91178=DIRECTION('center_axis',(-0.0483314596884342,-0.982569660846991,
-0.179501898562145));
#91179=DIRECTION('ref_axis',(0.907904086854337,0.0316999857459318,-0.417977607028057));
#91180=DIRECTION('center_axis',(1.34558305447855E-28,-1.,-3.78747958921603E-15));
#91181=DIRECTION('ref_axis',(-3.5527136788005E-14,-3.78747958921603E-15,
1.));
#91182=DIRECTION('center_axis',(0.132160818328594,-0.983673455323674,0.122147662238378));
#91183=DIRECTION('ref_axis',(0.707888425321867,0.00740489260537495,-0.706285455648657));
#91184=DIRECTION('center_axis',(-0.0876699682442016,0.987363722503006,-0.132010818318304));
#91185=DIRECTION('ref_axis',(0.76663440952793,-0.0177430384823854,-0.641838660967984));
#91186=DIRECTION('',(0.998609640362466,0.,0.0527141932988275));
#91187=DIRECTION('center_axis',(-6.02264512002837E-15,-1.,4.33910060592838E-15));
#91188=DIRECTION('ref_axis',(1.,-6.02264512002837E-15,-2.39473183021396E-32));
#91189=DIRECTION('center_axis',(-0.101428677285743,-0.98736372409962,-0.121758366267762));
#91190=DIRECTION('ref_axis',(0.765018938900932,0.000828885390579215,-0.644007248462237));
#91191=DIRECTION('center_axis',(0.0668059229005948,-0.987363722268358,0.143700551890981));
#91192=DIRECTION('ref_axis',(0.854490866293006,-0.0177432107440181,-0.51916330561233));
#91193=DIRECTION('center_axis',(0.109192641535518,0.98736372219585,0.114847059718792));
#91194=DIRECTION('ref_axis',(0.668231774075443,0.0126220373665493,-0.743846072980629));
#91195=DIRECTION('',(-0.0527141884073562,0.,0.998609640620675));
#91196=DIRECTION('center_axis',(1.31075898179972E-13,1.,-1.46594096344531E-13));
#91197=DIRECTION('ref_axis',(9.98802094496757E-32,1.46594096344531E-13,
1.));
#91198=DIRECTION('center_axis',(-0.0857885195141726,-0.982569635728196,
-0.164915859954485));
#91199=DIRECTION('ref_axis',(0.796825030841459,0.0317007065913415,-0.603377937470469));
#91200=DIRECTION('center_axis',(0.,-1.,7.99418401626902E-15));
#91201=DIRECTION('ref_axis',(0.,7.99418401626902E-15,1.));
#91202=DIRECTION('center_axis',(0.155329165193681,-0.983673454911944,0.0908811561427037));
#91203=DIRECTION('ref_axis',(0.539507892095231,0.00740500281159215,-0.841947979569));
#91204=DIRECTION('center_axis',(-0.11399871667095,0.987363722488542,-0.110078027375789));
#91205=DIRECTION('ref_axis',(0.610734582760325,-0.0177430389816003,-0.791636566858978));
#91206=DIRECTION('',(0.986594695254103,0.,-0.163189789191801));
#91207=DIRECTION('center_axis',(-1.2372651633228E-14,-1.,1.38308637850188E-14));
#91208=DIRECTION('ref_axis',(4.39963560667966E-32,-1.38308637850188E-14,
-1.));
#91209=DIRECTION('center_axis',(-0.125231787326932,-0.987363724103911,-0.0971075474232446));
#91210=DIRECTION('ref_axis',(0.60869069698727,0.000828875038098951,-0.793407176906866));
#91211=DIRECTION('center_axis',(0.0961354100921401,-0.987363722345579,0.125979612327939));
#91212=DIRECTION('ref_axis',(0.722908581050635,-0.0177432080803394,-0.690715833038721));
#91213=DIRECTION('center_axis',(0.131328502646465,0.987363722211955,0.08868880680441));
#91214=DIRECTION('ref_axis',(0.492703966766174,0.0126220350460105,-0.870105444968697));
#91215=DIRECTION('',(0.163189791341605,0.,0.98659469489851));
#91216=DIRECTION('center_axis',(0.,1.,0.));
#91217=DIRECTION('ref_axis',(0.,0.,1.));
#91218=DIRECTION('center_axis',(-0.119235357666559,-0.982569661740983,-0.142617633230741));
#91219=DIRECTION('ref_axis',(0.648487187440979,0.0316999532797268,-0.760565237627221));
#91220=DIRECTION('center_axis',(0.,-1.,-3.78747958921603E-15));
#91221=DIRECTION('ref_axis',(0.,-3.78747958921603E-15,1.));
#91222=DIRECTION('center_axis',(0.171234386949594,-0.983673455275735,0.0553653150618104));
#91223=DIRECTION('ref_axis',(0.345900567498622,0.00740490675994489,-0.93824195427406));
#91224=DIRECTION('center_axis',(-0.134997008872396,0.987363722451529,-0.0829981155338303));
#91225=DIRECTION('ref_axis',(0.426277487512531,-0.0177430452325937,-0.904418425279958));
#91226=DIRECTION('',(0.928447677255466,0.,-0.3714632022138));
#91227=DIRECTION('center_axis',(1.27542226361885E-14,-1.,-2.26341643165069E-14));
#91228=DIRECTION('ref_axis',(5.07241172839367E-32,2.26341643165069E-14,
-1.));
#91229=DIRECTION('center_axis',(-0.143179187504052,-0.987363724170279,-0.0679160986679622));
#91230=DIRECTION('ref_axis',(0.423900758702251,0.000828879569203518,-0.90570826413935));
#91231=DIRECTION('center_axis',(0.120969689331929,-0.987363721339821,0.102368042107466));
#91232=DIRECTION('ref_axis',(0.557523896409954,-0.0177432483395472,-0.829971253761372));
#91233=DIRECTION('center_axis',(0.147323588236072,0.987363722231605,0.0583835625000547));
#91234=DIRECTION('ref_axis',(0.294137871286664,0.0126220315474288,-0.955679651868013));
#91235=DIRECTION('',(0.371463200767281,0.,0.928447677834204));
#91236=DIRECTION('center_axis',(-9.56800049051936E-15,1.,3.13470915944282E-14));
#91237=DIRECTION('ref_axis',(6.09885243099091E-33,-3.13470915944282E-14,
1.));
#91238=DIRECTION('center_axis',(-0.147106180063853,-0.982569655018706,-0.113651418044136));
#91239=DIRECTION('ref_axis',(0.469826904776602,0.03170015665596,-0.882189197177128));
#91240=DIRECTION('center_axis',(0.,-1.,-3.78747958921603E-15));
#91241=DIRECTION('ref_axis',(0.,-3.78747958921603E-15,1.));
#91242=DIRECTION('center_axis',(0.179132923581415,-0.983673455474697,0.017260610755237));
#91243=DIRECTION('ref_axis',(0.136119321091654,0.00740486877593419,-0.990664775968116));
#91244=DIRECTION('center_axis',(-0.149682997370563,0.987363722508653,-0.05203729212805));
#91245=DIRECTION('ref_axis',(0.221888128067994,-0.017743037961803,-0.974910684743155));
#91246=DIRECTION('',(0.82688748012557,0.,-0.562367402337284));
#91247=DIRECTION('center_axis',(-6.5060226382221E-15,-1.,2.12972323065662E-14));
#91248=DIRECTION('ref_axis',(-2.27817423217471E-32,-2.12972323065662E-14,
-1.));
#91249=DIRECTION('center_axis',(-0.154431689931071,-0.987363724094681,-0.0355489730782223));
#91250=DIRECTION('ref_axis',(0.219289691904165,0.000828887532608173,-0.975659440568293));
#91251=DIRECTION('center_axis',(0.140147588783667,-0.987363721370841,0.0739698254617974));
#91252=DIRECTION('ref_axis',(0.366070013200346,-0.0177432466485635,-0.930418143972841));
#91253=DIRECTION('center_axis',(0.156429984571215,0.987363722264396,0.0253483704258555));
#91254=DIRECTION('ref_axis',(0.0818182164522016,0.0126220312518529,-0.996567340315574));
#91255=DIRECTION('',(0.56236740413906,0.,0.82688747890018));
#91256=DIRECTION('center_axis',(2.60560789866602E-15,1.,-3.26710515559638E-14));
#91257=DIRECTION('ref_axis',(7.18875342422977E-33,3.26710515559638E-14,
1.));
#91258=DIRECTION('center_axis',(-0.168098486533422,-0.982569637630382,-0.0793713174394452));
#91259=DIRECTION('ref_axis',(0.269198093291677,0.0317006521827105,-0.962562961690983));
#91260=DIRECTION('center_axis',(0.,-1.,-3.78747958921603E-15));
#91261=DIRECTION('ref_axis',(0.,-3.78747958921603E-15,1.));
#91262=DIRECTION('center_axis',(0.178655412465466,-0.98367345523271,-0.0216512601789133));
#91263=DIRECTION('ref_axis',(-0.0800267183951851,0.00740491324750828,-0.996765213880729));
#91264=DIRECTION('center_axis',(-0.15736997128655,0.987363722472243,-0.0186432744716927));
#91265=DIRECTION('ref_axis',(0.00712353035048156,-0.0177430427862771,-0.999817203166674));
#91266=DIRECTION('',(0.68666294091143,0.,-0.726975931911687));
#91267=DIRECTION('center_axis',(-2.95940006317246E-16,-1.,3.69965289557878E-15));
#91268=DIRECTION('ref_axis',(3.22728447839295E-34,-3.69965289557878E-15,
-1.));
#91269=DIRECTION('center_axis',(-0.158463140916245,-0.987363724157911,-0.00151960125661887));
#91270=DIRECTION('ref_axis',(0.00442488112967827,0.000828879242715846,-0.999989866641752));
#91271=DIRECTION('center_axis',(0.152772346096398,-0.987363722316901,0.0421128260832276));
#91272=DIRECTION('ref_axis',(0.157499094830202,-0.017743210008238,-0.987359718454359));
#91273=DIRECTION('center_axis',(0.158221889065703,0.987363722232188,-0.0088720820712651));
#91274=DIRECTION('ref_axis',(-0.134327168570016,0.0126220323727302,-0.990856647594769));
#91275=DIRECTION('',(0.726975931972861,0.,0.686662940846665));
#91276=DIRECTION('center_axis',(-8.9572421130411E-15,1.,-6.49347121175939E-14));
#91277=DIRECTION('ref_axis',(-4.34106576186858E-32,6.49347121175939E-14,
1.));
#91278=DIRECTION('center_axis',(-0.181230912891191,-0.982569629730098,-0.0413796924189044));
#91279=DIRECTION('ref_axis',(0.0559818735015593,0.0317008821641159,-0.99792839618345));
#91280=DIRECTION('center_axis',(0.,-1.,-1.48029736755923E-14));
#91281=DIRECTION('ref_axis',(0.,-1.48029736755923E-14,1.));
#91282=DIRECTION('center_axis',(0.169824197772912,-0.98367345564293,-0.0595506046508672));
#91283=DIRECTION('ref_axis',(-0.292430796806876,0.00740481273193738,-0.956258018438173));
#91284=DIRECTION('center_axis',(-0.157698501543129,0.987363722479201,0.0156224883762656));
#91285=DIRECTION('ref_axis',(-0.207974158912054,-0.0177430414407734,-0.977973380877647));
#91286=DIRECTION('',(0.514330810099969,0.,-0.857591871336191));
#91287=DIRECTION('center_axis',(2.02517967483958E-15,-1.,1.47071016964003E-14));
#91288=DIRECTION('ref_axis',(1.07744368455052E-32,-1.47071016964003E-14,
-1.));
#91289=DIRECTION('center_axis',(-0.155085103499708,-0.987363723836278,0.0325804776613727));
#91290=DIRECTION('ref_axis',(-0.210646778580884,0.00082922245084035,-0.977561889121923));
#91291=DIRECTION('center_axis',(0.158253630647629,-0.987363721274912,0.00828675431046068));
#91292=DIRECTION('ref_axis',(-0.0584362933306146,-0.0177432508835518,-0.998133446323617));
#91293=DIRECTION('center_axis',(0.152615513172385,0.987363722259592,-0.0426776886067419));
#91294=DIRECTION('ref_axis',(-0.344191563026183,0.0126220303639586,-0.938814599530218));
#91295=DIRECTION('',(0.85759187372498,0.,0.514330806116917));
#91296=DIRECTION('center_axis',(-4.54137237097151E-14,1.,-1.2298201840572E-13));
#91297=DIRECTION('ref_axis',(3.20542588349696E-31,1.2298201840572E-13,1.));
#91298=DIRECTION('center_axis',(-0.185889240027947,-0.982569630822743,-0.00145293726336171));
#91299=DIRECTION('ref_axis',(-0.159852068098868,0.0317008511488114,-0.986631832225656));
#91300=DIRECTION('center_axis',(0.,-1.,-1.15792791941926E-14));
#91301=DIRECTION('ref_axis',(0.,-1.15792791941926E-14,1.));
#91302=DIRECTION('center_axis',(0.153051994296784,-0.983673454167874,-0.0946658471003188));
#91303=DIRECTION('ref_axis',(-0.491161130555647,0.00740519063348927,-0.871037259239224));
#91304=DIRECTION('center_axis',(-0.150653226017932,0.987363722442911,0.0491577572115231));
#91305=DIRECTION('ref_axis',(-0.413347207736676,-0.017743044202828,-0.910400609753041));
#91306=DIRECTION('',(0.31794913860653,0.,-0.948107770909703));
#91307=DIRECTION('center_axis',(-1.28485605524992E-15,-1.,-3.48197601383281E-15));
#91308=DIRECTION('ref_axis',(-2.47587532992437E-33,3.48197601383282E-15,
-1.));
#91309=DIRECTION('center_axis',(-0.144455314496109,-0.987363724113352,0.0651577963013036));
#91310=DIRECTION('ref_axis',(-0.415868934776334,0.000828876094051006,-0.909424181585479));
#91311=DIRECTION('center_axis',(0.156335142091041,-0.987363722370261,-0.0259268797682325));
#91312=DIRECTION('ref_axis',(-0.271639278391324,-0.0177432074989289,-0.962235564205923));
#91313=DIRECTION('center_axis',(0.139873008188529,0.987363722211361,-0.0744877281249552));
#91314=DIRECTION('ref_axis',(-0.537961943085501,0.0126220349637511,-0.8428746241435));
#91315=DIRECTION('',(0.948107772469132,0.,0.317949133956394));
#91316=DIRECTION('center_axis',(-5.30921149349349E-14,1.,-8.27581331014178E-14));
#91317=DIRECTION('ref_axis',(-2.7805240325011E-31,8.27581331014178E-14,
1.));
#91318=DIRECTION('center_axis',(-0.181855215515493,-0.982569664512228,0.0385426383391284));
#91319=DIRECTION('ref_axis',(-0.368211691435434,0.0316998820363428,-0.929201413994371));
#91320=DIRECTION('center_axis',(0.,-1.,-3.78747958921603E-15));
#91321=DIRECTION('ref_axis',(0.,-3.78747958921603E-15,1.));
#91322=DIRECTION('center_axis',(0.129123558039704,-0.983673455292137,-0.125354059020023));
#91323=DIRECTION('ref_axis',(-0.666925320249561,0.00740490243755575,-0.74508776974925));
#91324=DIRECTION('center_axis',(-0.136563572509073,0.987363722456192,0.0803944664825342));
#91325=DIRECTION('ref_axis',(-0.599392598698392,-0.0177430439695527,-0.800258518865175));
#91326=DIRECTION('',(0.106700517422838,0.,-0.994291204618495));
#91327=DIRECTION('center_axis',(1.40233712663849E-14,-1.,2.18705429551819E-14));
#91328=DIRECTION('ref_axis',(-2.0037589829547E-32,-2.18705429551819E-14,
-1.));
#91329=DIRECTION('center_axis',(-0.127071029273013,-0.987363724119497,0.0946880658392329));
#91330=DIRECTION('ref_axis',(-0.601645467602814,0.000828876144709256,-0.79876282104097));
#91331=DIRECTION('center_axis',(0.147106623059428,-0.987363721277475,-0.0589281202580531));
#91332=DIRECTION('ref_axis',(-0.472140697430878,-0.0177432505213094,-0.881344619822701));
#91333=DIRECTION('',(0.994291204851001,0.,0.106700515256233));
#91334=DIRECTION('center_axis',(0.120590197321115,0.987363722182783,-0.102814806460033));
#91335=DIRECTION('ref_axis',(-0.706577819713666,0.0126220377017149,-0.707522769140992));
#91336=DIRECTION('center_axis',(0.,1.,0.));
#91337=DIRECTION('ref_axis',(0.,0.,1.));
#91338=DIRECTION('center_axis',(-0.169318498668954,-0.982569635474812,0.0767343303312521));
#91339=DIRECTION('ref_axis',(-0.559353793109933,0.0317007163076125,-0.828322641679626));
#91340=DIRECTION('center_axis',(-2.38609880511614E-28,-1.,1.16804714017285E-14));
#91341=DIRECTION('ref_axis',(-2.04281036531029E-14,1.16804714017285E-14,
1.));
#91342=DIRECTION('center_axis',(0.0991572193433959,-0.983673454833043,-0.150181157636075));
#91343=DIRECTION('ref_axis',(-0.811504822713002,0.00740500677956439,-0.584298800775882));
#91344=DIRECTION('center_axis',(-0.116088355566142,0.987363722501146,0.107872022279315));
#91345=DIRECTION('ref_axis',(-0.757411059269865,-0.017743040388858,-0.652697228286945));
#91346=DIRECTION('',(-0.109537300692827,0.,-0.993982685843636));
#91347=DIRECTION('center_axis',(5.25629510911856E-15,-1.,5.24131757556537E-15));
#91348=DIRECTION('ref_axis',(1.,5.25629510911856E-15,2.9872547149238E-32));
#91349=DIRECTION('center_axis',(-0.103745042602045,-0.987363724129464,0.119790827731908));
#91350=DIRECTION('ref_axis',(-0.75928972628638,0.000828874316998394,-0.650752199015356));
#91351=DIRECTION('center_axis',(0.130999520502375,-0.987363722264207,-0.0891740185520346));
#91352=DIRECTION('ref_axis',(-0.650565357517768,-0.0177432109538035,-0.759242974325629));
#91353=DIRECTION('center_axis',(0.0956687178831353,0.987363722223788,-0.126334383502603));
#91354=DIRECTION('ref_axis',(-0.842154904346286,0.0126220335947149,-0.539087934713282));
#91355=DIRECTION('',(0.993982685952451,0.,-0.109537299705404));
#91356=DIRECTION('center_axis',(8.29343359167699E-14,1.,5.28164464733621E-14));
#91357=DIRECTION('ref_axis',(-1.,8.293433591677E-14,3.76666855861367E-31));
#91358=DIRECTION('center_axis',(-0.148864271522895,-0.982569637327251,0.11133883629063));
#91359=DIRECTION('ref_axis',(-0.724341307884093,0.0317006605829815,-0.688712376693903));
#91360=DIRECTION('center_axis',(-7.06431103601238E-29,-1.,-3.78747958921603E-15));
#91361=DIRECTION('ref_axis',(1.86517468137026E-14,-3.78747958921603E-15,
1.));
#91362=DIRECTION('center_axis',(0.0645545855673779,-0.983673455399648,-0.167985828641407));
#91363=DIRECTION('ref_axis',(-0.918139262285609,0.00740487866414407,-0.396188670738585));
#91364=DIRECTION('center_axis',(-0.0901849778030904,0.987363722478745,0.130305599693841));
#91365=DIRECTION('ref_axis',(-0.880013820330849,-0.0177430398882603,-0.474616540548502));
#91366=DIRECTION('',(-0.320653274273476,0.,-0.947196641515213));
#91367=DIRECTION('center_axis',(6.26013419967124E-15,-1.,3.98883041207536E-15));
#91368=DIRECTION('ref_axis',(1.,6.26013419967124E-15,-2.68710427983303E-33));
#91369=DIRECTION('center_axis',(-0.075568076442598,-0.987363724119251,0.139292290225014));
#91370=DIRECTION('ref_axis',(-0.881430438857171,0.000828899162159362,-0.472313131706323));
#91371=DIRECTION('center_axis',(0.108767073254341,-0.98736372146031,-0.115250185768753));
#91372=DIRECTION('ref_axis',(-0.798570293939769,-0.0177432430057322,-0.601639977864329));
#91373=DIRECTION('center_axis',(0.0662738822247929,0.987363722186029,-0.143946700711773));
#91374=DIRECTION('ref_axis',(-0.938353761552175,0.0126220379022938,-0.345445947059849));
#91375=DIRECTION('',(0.947196640816497,0.,-0.320653276337453));
#91376=DIRECTION('center_axis',(3.07831179698849E-14,1.,1.12510657658258E-14));
#91377=DIRECTION('ref_axis',(-1.,3.07831179698849E-14,3.56206623346533E-32));
#91378=DIRECTION('center_axis',(-0.121449338297179,-0.982569637779582,0.140737220168932));
#91379=DIRECTION('ref_axis',(-0.855459416436917,0.0317006491305122,-0.516898689952018));
#91380=DIRECTION('center_axis',(0.,-1.,-1.46295013157071E-14));
#91381=DIRECTION('ref_axis',(0.,-1.46295013157071E-14,1.));
#91382=DIRECTION('center_axis',(0.0269333624616044,-0.983673455422475,-0.177935738635387));
#91383=DIRECTION('ref_axis',(-0.981842529371897,0.00740486370994217,-0.18955319968292));
#91384=DIRECTION('center_axis',(-0.0600646491167124,0.987363722533973,0.146646231967762));
#91385=DIRECTION('ref_axis',(-0.961468112563275,-0.0177430377158196,-0.274343312542203));
#91386=DIRECTION('',(-0.516775858941057,0.,-0.856120734251737));
#91387=DIRECTION('center_axis',(-2.43993972821388E-14,-1.,-8.92440488461752E-15));
#91388=DIRECTION('ref_axis',(1.,-2.43993972821388E-14,2.12366322857769E-32));
#91389=DIRECTION('center_axis',(-0.0438576345564159,-0.987363724127006,
0.152280609957948));
#91390=DIRECTION('ref_axis',(-0.962356445818495,0.000828922493000271,-0.271789227305084));
#91391=DIRECTION('center_axis',(0.081448785342375,-0.987363721224333,-0.135937402418504));
#91392=DIRECTION('ref_axis',(-0.909234973830211,-0.0177432523881513,-0.415904964335202));
#91393=DIRECTION('center_axis',(0.0337801471428685,0.987363722229621,-0.154828232838441));
#91394=DIRECTION('ref_axis',(-0.990676239327606,0.0126220348238584,-0.135651292174523));
#91395=DIRECTION('',(0.856120733893417,0.,-0.51677585953467));
#91396=DIRECTION('center_axis',(2.27374502308751E-13,1.,3.0593931262345E-14));
#91397=DIRECTION('ref_axis',(-1.,2.27374502308751E-13,1.1524214611489E-31));
#91398=DIRECTION('center_axis',(-0.0883550911670293,-0.982569655107274,
0.163555038831696));
#91399=DIRECTION('ref_axis',(-0.946577232895948,0.0317001444348233,-0.320915320615675));
#91400=DIRECTION('center_axis',(0.,-1.,-3.78747958921603E-15));
#91401=DIRECTION('ref_axis',(0.,-3.78747958921603E-15,1.));
#91402=DIRECTION('center_axis',(-0.0119472795883105,-0.983673455333531,
-0.179565575160247));
#91403=DIRECTION('ref_axis',(-0.999635931190591,0.0074048951126651,0.02594556997045));
#91404=DIRECTION('center_axis',(-0.027135769578797,0.987363722495344,0.15612984823378));
#91405=DIRECTION('ref_axis',(-0.997965224992306,-0.0177430414057831,-0.0612420948999103));
#91406=DIRECTION('',(-0.688734576602034,0.,-0.725013574350727));
#91407=DIRECTION('center_axis',(-1.83910258353765E-14,-1.,-2.47900577328738E-15));
#91408=DIRECTION('ref_axis',(1.,-1.83910258353765E-14,-7.33039533389768E-33));
#91409=DIRECTION('center_axis',(-0.0100963937174092,-0.9873637241587,0.158148471536609));
#91410=DIRECTION('ref_axis',(-0.998283737173725,0.000828878972048249,-0.0585567507133987));
#91411=DIRECTION('center_axis',(0.0503219923558111,-0.987363722299207,-0.150268349870476));
#91412=DIRECTION('ref_axis',(-0.97738484116564,-0.0177432102047794,-0.210722686845167));
#91413=DIRECTION('center_axis',(-0.000293106042224026,0.987363722206634,
-0.158470168041525));
#91414=DIRECTION('ref_axis',(-0.996675797363578,0.0126220360918558,0.0804862668693937));
#91415=DIRECTION('',(0.725013572849968,0.,-0.688734578181845));
#91416=DIRECTION('center_axis',(-1.30648829703912E-13,1.,1.08572221678296E-14));
#91417=DIRECTION('ref_axis',(-1.,-1.30648829703912E-13,-5.11450308930103E-32));
#91418=DIRECTION('center_axis',(-0.0511306135194889,-0.98256963095643,0.178724874271229));
#91419=DIRECTION('ref_axis',(-0.993434052898061,0.0317008474190799,-0.109926515524896));
#91420=DIRECTION('center_axis',(0.,-1.,-5.37764278031254E-15));
#91421=DIRECTION('ref_axis',(0.,-5.37764278031254E-15,1.));
#91422=DIRECTION('center_axis',(-0.0502691671596196,-0.983673455672302,
-0.172799141892518));
#91423=DIRECTION('ref_axis',(-0.970687468112846,0.00740480799607863,0.240231155488238));
#91424=DIRECTION('center_axis',(0.0070619506335549,0.987363722459408,0.158313007754735));
#91425=DIRECTION('ref_axis',(-0.987798592664615,-0.0177430426809696,0.154722735130385));
#91426=DIRECTION('',(-0.828488831038146,0.,-0.560005586440927));
#91427=DIRECTION('center_axis',(1.10963801102532E-14,-1.,-9.19487355021671E-16));
#91428=DIRECTION('ref_axis',(1.,1.10963801102532E-14,-5.37912607381295E-33));
#91429=DIRECTION('center_axis',(0.0241365891185764,-0.987363723876408,0.156621524186918));
#91430=DIRECTION('ref_axis',(-0.98753239609518,0.00082919088419808,0.157413719557698));
#91431=DIRECTION('center_axis',(0.0168422735472509,-0.987363721427545,-0.157572901954963));
#91432=DIRECTION('ref_axis',(-0.999833274907587,-0.0177432441231643,0.00431273411593884));
#91433=DIRECTION('center_axis',(-0.0343526576847958,0.98736372221655,-0.154702213819554));
#91434=DIRECTION('ref_axis',(-0.956071902708856,0.0126220335741101,0.292860378199444));
#91435=DIRECTION('',(0.560005583301831,0.,-0.828488833159975));
#91436=DIRECTION('center_axis',(3.1315081560836E-14,1.,-9.67225379250271E-15));
#91437=DIRECTION('ref_axis',(-1.,3.1315081560836E-14,2.24514060136425E-32));
#91438=DIRECTION('center_axis',(-0.0115144350220054,-0.982569637967496,
0.185537932322604));
#91439=DIRECTION('ref_axis',(-0.993839068512918,0.0317006448509257,0.106202518865662));
#91440=DIRECTION('center_axis',(0.,-1.,-3.33934269153158E-15));
#91441=DIRECTION('ref_axis',(0.,-3.33934269153158E-15,1.));
#91442=DIRECTION('center_axis',(-0.0862406661628375,-0.983673455403097,
-0.157952779763834));
#91443=DIRECTION('ref_axis',(-0.896350737297868,0.00740487292010241,0.44328379578167));
#91444=DIRECTION('center_axis',(0.0409294624178168,0.987363722466824,0.1530936271131));
#91445=DIRECTION('ref_axis',(-0.931443596256056,-0.0177430432852071,0.363452901224581));
#91446=DIRECTION('',(-0.929503870801002,0.,-0.368812356308672));
#91447=DIRECTION('center_axis',(0.,-1.,0.));
#91448=DIRECTION('ref_axis',(0.,0.,-1.));
#91449=DIRECTION('center_axis',(0.0572415509645948,-0.987363724119703,0.147771042953751));
#91450=DIRECTION('ref_axis',(-0.930605124983861,0.000828910731059022,0.366023789200609));
#91451=DIRECTION('center_axis',(-0.0174250074421581,-0.987363721465215,
-0.157509525584966));
#91452=DIRECTION('ref_axis',(-0.97553061766179,-0.0177432425678975,0.219146506583115));
#91453=DIRECTION('center_axis',(-0.0668059115608627,0.987363722212296,-0.143700557547988));
#91454=DIRECTION('ref_axis',(-0.870763148687641,0.0126220369484988,0.491540662683014));
#91455=DIRECTION('',(0.368812355268781,0.,-0.929503871213614));
#91456=DIRECTION('center_axis',(-1.14014813092713E-13,1.,6.47117539700905E-14));
#91457=DIRECTION('ref_axis',(-1.,-1.14014813092713E-13,-1.69361705489593E-31));
#91458=DIRECTION('center_axis',(0.0286403209154908,-0.982569651704975,0.183675288392918));
#91459=DIRECTION('ref_axis',(-0.94777325181453,0.0317002440392639,0.317365652950603));
#91460=DIRECTION('center_axis',(-2.01837458171782E-29,-1.,-3.78747958921603E-15));
#91461=DIRECTION('ref_axis',(5.32907051820075E-15,-3.78747958921603E-15,
1.));
#91462=DIRECTION('center_axis',(-0.118179585967429,-0.983673455420277,-0.13572073740626));
#91463=DIRECTION('ref_axis',(-0.780101643914051,0.00740487350271539,0.625608977725706));
#91464=DIRECTION('center_axis',(0.0728831627478859,0.987363722498741,0.140715756336291));
#91465=DIRECTION('ref_axis',(-0.831535330925473,-0.0177430390696153,0.555188416654417));
#91466=DIRECTION('',(-0.987056341019165,0.,-0.160373874598885));
#91467=DIRECTION('center_axis',(1.61411985227139E-14,-1.,-9.15625532613643E-15));
#91468=DIRECTION('ref_axis',(1.,1.61411985227139E-14,-5.66390648337493E-32));
#91469=DIRECTION('center_axis',(0.0876697142084478,-0.987363724095884,0.132010975112361));
#91470=DIRECTION('ref_axis',(-0.830163795586117,0.000828872077927888,0.557518955255452));
#91471=DIRECTION('center_axis',(-0.0508775087218593,-0.987363721389257,
-0.150081180667713));
#91472=DIRECTION('ref_axis',(-0.905613234397984,-0.0177432462315155,0.423733226094427));
#91473=DIRECTION('center_axis',(-0.0961353978983087,0.987363722178085,-0.125979622945822));
#91474=DIRECTION('ref_axis',(-0.744738477439971,0.0126220380236425,0.667237052610632));
#91475=DIRECTION('',(0.160373869647189,0.,-0.987056341823701));
#91476=DIRECTION('center_axis',(1.46157135101623E-13,1.,-1.31562957702813E-13));
#91477=DIRECTION('ref_axis',(-1.,1.46157135101623E-13,5.63522651253288E-32));
#91478=DIRECTION('center_axis',(0.0674550899212748,-0.982569636071288,0.173224481856493));
#91479=DIRECTION('ref_axis',(-0.85739063654192,0.0317006985960046,0.513688974067739));
#91480=DIRECTION('center_axis',(0.,-1.,-9.12175427525787E-15));
#91481=DIRECTION('ref_axis',(0.,-9.12175427525787E-15,1.));
#91482=DIRECTION('center_axis',(-0.144592641615338,-0.983673454856816,-0.107142438840795));
#91483=DIRECTION('ref_axis',(-0.627375861967964,0.00740500910540536,0.778681381349332));
#91484=DIRECTION('center_axis',(0.101428920968401,0.987363722463645,0.121758176538255));
#91485=DIRECTION('ref_axis',(-0.692745400955484,-0.0177430414082981,0.720963933866743));
#91486=DIRECTION('',(-0.998455154553505,3.11688535425711E-16,0.055563516317241));
#91487=DIRECTION('center_axis',(1.37955020419649E-14,-1.,-1.24120677249046E-14));
#91488=DIRECTION('ref_axis',(1.,1.37955020419649E-14,5.52387648803174E-32));
#91489=DIRECTION('center_axis',(0.11399850328062,-0.987363724090544,0.110078233996695));
#91490=DIRECTION('ref_axis',(-0.690904932361026,0.000828870840717851,0.722945148273599));
#91491=DIRECTION('center_axis',(-0.0819510668801886,-0.987363722305634,
-0.135635181689564));
#91492=DIRECTION('ref_axis',(-0.793350377678185,-0.0177432098191626,0.608506661215138));
#91493=DIRECTION('center_axis',(-0.120969701972986,0.987363722185803,-0.102368019009666));
#91494=DIRECTION('ref_axis',(-0.583890661941005,0.0126220361724893,0.811734180074336));
#91495=DIRECTION('',(-0.0555635156269576,0.,-0.998455154591919));
#91496=DIRECTION('center_axis',(-1.90763212459409E-14,1.,2.66510948801363E-14));
#91497=DIRECTION('ref_axis',(-6.7895573354269E-32,-2.66510948801363E-14,
1.));
#91498=DIRECTION('center_axis',(0.10311612646859,-0.982569634025935,0.154673781722226));
#91499=DIRECTION('ref_axis',(-0.726917383075444,0.0317007582126674,0.68599284260952));
#91500=DIRECTION('center_axis',(0.,-1.,-4.5247370677682E-15));
#91501=DIRECTION('ref_axis',(0.,-4.5247370677682E-15,1.));
#91502=DIRECTION('center_axis',(-0.164244541101588,-0.983673455463523,-0.0735544950005185));
#91503=DIRECTION('ref_axis',(-0.445314682867744,0.00740486179507685,0.895343510192706));
#91504=DIRECTION('center_axis',(0.125231976596983,0.987363722472282,0.0971073199264145));
#91505=DIRECTION('ref_axis',(-0.521563464398509,-0.0177430435487255,0.853027981375906));
#91506=DIRECTION('',(-0.963167314504198,3.11688536629873E-16,0.268902815661666));
#91507=DIRECTION('center_axis',(-4.32189727882296E-15,-1.,6.03500224482245E-15));
#91508=DIRECTION('ref_axis',(-2.95538501758547E-32,-6.03500224482245E-15,
-1.));
#91509=DIRECTION('center_axis',(0.134996780744609,-0.98736372407516,0.0829984672691258));
#91510=DIRECTION('ref_axis',(-0.519340140134093,0.000828997761539845,0.854567218893992));
#91511=DIRECTION('center_axis',(-0.109192627375346,-0.987363721318639,-0.114847080723355));
#91512=DIRECTION('ref_axis',(-0.643991344872343,-0.0177432487589253,0.76482699014417));
#91513=DIRECTION('center_axis',(-0.140147596738918,0.987363722235712,-0.0739697988448428));
#91514=DIRECTION('ref_axis',(-0.395740769540629,0.0126220331102005,0.918275518351413));
#91515=DIRECTION('',(-0.268902817760427,0.,-0.963167313918253));
#91516=DIRECTION('center_axis',(-1.29011271314033E-14,1.,3.01288458702476E-14));
#91517=DIRECTION('ref_axis',(3.29010680199035E-32,-3.01288458702476E-14,
1.));
#91518=DIRECTION('center_axis',(0.133955574882366,-0.982569631427832,0.128890741923958));
#91519=DIRECTION('ref_axis',(-0.562454294716541,0.0317008349676485,0.826220444807118));
#91520=DIRECTION('center_axis',(0.,-1.,7.19910242023359E-15));
#91521=DIRECTION('ref_axis',(0.,7.19910242023359E-15,1.));
#91522=DIRECTION('center_axis',(-0.176216709575444,-0.983673454206282,-0.036526795045364));
#91523=DIRECTION('ref_axis',(-0.24243108626749,0.00740519116528956,0.970140366934069));
#91524=DIRECTION('center_axis',(0.143179326339322,0.987363722466588,0.0679158307461498));
#91525=DIRECTION('ref_axis',(-0.325993799946702,-0.0177430425423517,0.94520538870536));
#91526=DIRECTION('',(-0.882842841300016,0.,0.469668518814402));
#91527=DIRECTION('center_axis',(1.31557798442278E-14,-1.,-3.07034433151806E-14));
#91528=DIRECTION('ref_axis',(1.5289773705897E-32,3.07034433151806E-14,-1.));
#91529=DIRECTION('center_axis',(0.149682890516781,-0.987363724091402,0.0520375694561118));
#91530=DIRECTION('ref_axis',(-0.323491544844115,0.000828869996302542,0.946230697762917));
#91531=DIRECTION('center_axis',(-0.13132850894257,-0.987363722349457,-0.0886887959504751));
#91532=DIRECTION('ref_axis',(-0.464519985807728,-0.0177432087395852,0.885384866218534));
#91533=DIRECTION('center_axis',(-0.152772343819054,0.987363722231284,-0.0421128363520662));
#91534=DIRECTION('ref_axis',(-0.189086478016743,0.01262203398202,0.981879314421778));
#91535=DIRECTION('',(-0.469668518497478,0.,-0.882842841468619));
#91536=DIRECTION('center_axis',(3.67361741914096E-14,1.,-1.93186898753132E-13));
#91537=DIRECTION('ref_axis',(-1.78965190703203E-31,1.93186898753132E-13,
1.));
#91538=DIRECTION('center_axis',(0.158531736849135,-0.982569656573641,0.0970801647730095));
#91539=DIRECTION('ref_axis',(-0.371691321544402,0.0317001055356064,0.927814994919573));
#91540=DIRECTION('center_axis',(0.,-1.,-3.78747958921603E-15));
#91541=DIRECTION('ref_axis',(0.,-3.78747958921603E-15,1.));
#91542=DIRECTION('center_axis',(-0.179949039173256,-0.983673455413316,0.00220826081986253));
#91543=DIRECTION('ref_axis',(-0.0282116802862476,0.00740488220223463,0.999574543901053));
#91544=DIRECTION('center_axis',(0.154431769493381,0.987363722487946,0.035548672069278));
#91545=DIRECTION('ref_axis',(-0.11518102602311,-0.017743041274024,0.993186042859349));
#91546=DIRECTION('',(-0.761237618626322,0.,0.648473043378155));
#91547=DIRECTION('center_axis',(-1.38841606632461E-15,-1.,7.29193725991163E-15));
#91548=DIRECTION('ref_axis',(-8.46747865150748E-33,-7.29193725991163E-15,
-1.));
#91549=DIRECTION('center_axis',(0.157369926272718,-0.987363724124777,0.0186435669165276));
#91550=DIRECTION('ref_axis',(-0.112516862267976,0.000828873940512268,0.993649469719257));
#91551=DIRECTION('center_axis',(-0.147323582410273,-0.987363721358974,-0.0583835919583681));
#91552=DIRECTION('ref_axis',(-0.263328199075575,-0.017743247115542,0.96454312332493));
#91553=DIRECTION('center_axis',(-7.5362264330552E-15,1.,-2.62089983140031E-13));
#91554=DIRECTION('ref_axis',(-2.13409324614581E-32,2.62089983140031E-13,
1.));
#91555=DIRECTION('center_axis',(0.175694642098467,-0.982569639383468,0.0607313469283601));
#91556=DIRECTION('ref_axis',(-0.163548662564118,0.0317006050560886,0.986025814374333));
#91557=DIRECTION('center_axis',(-3.36395763619637E-30,-1.,-3.78747958921603E-15));
#91558=DIRECTION('ref_axis',(8.88178419700125E-16,-3.78747958921603E-15,
1.));
#91559=DIRECTION('center_axis',(-0.17526714169692,-0.983673452813486,0.040840755029578));
#91560=DIRECTION('ref_axis',(0.187326942949257,0.00740528131793076,0.982269707490712));
#91561=DIRECTION('center_axis',(-4.23190585545145E-16,-1.,-1.48398484630621E-14));
#91562=DIRECTION('ref_axis',(0.0285055883760776,-1.48458813372039E-14,0.999593633148658));
#91563=DIRECTION('center_axis',(0.157698522826405,-0.987363724124184,-0.0156221695673659));
#91564=DIRECTION('ref_axis',(0.103718979496377,0.000828895785446709,0.994606297096498));
#91565=DIRECTION('center_axis',(-0.158253626383321,0.987363722223235,-0.00828672275433531));
#91566=DIRECTION('ref_axis',(0.0264092846868512,0.0126220326853917,0.999571525191278));
#91567=DIRECTION('center_axis',(-0.156429985617351,-0.987363722284086,-0.0253483632029913));
#91568=DIRECTION('ref_axis',(-0.0498234664665366,-0.0177432101527035,0.998600420930582));
#91569=DIRECTION('',(-0.64847304670282,0.,-0.76123761579415));
#91570=DIRECTION('center_axis',(0.,1.,0.));
#91571=DIRECTION('ref_axis',(1.,0.,0.));
#91572=DIRECTION('center_axis',(0.987464241017343,0.151612438471943,-0.0439094660936956));
#91573=DIRECTION('ref_axis',(0.0466366821965845,-0.0144775320618018,0.998806998843668));
#91574=DIRECTION('center_axis',(0.162375657399389,-0.986495109627198,-0.0214835882882429));
#91575=DIRECTION('ref_axis',(0.0319374621849617,-0.0165067558142742,0.999353553814501));
#91576=DIRECTION('center_axis',(-0.163746575713113,-0.986495111104823,0.00380193483800228));
#91577=DIRECTION('ref_axis',(0.133383938187138,-0.018321271348547,0.990895078224664));
#91578=DIRECTION('center_axis',(-0.954918750289514,-0.151717240595822,0.255170647315678));
#91579=DIRECTION('ref_axis',(0.265259226515505,-0.0501190367766773,0.962873628728596));
#91580=DIRECTION('center_axis',(0.15396106861831,-0.986495109630634,-0.055887279632775));
#91581=DIRECTION('ref_axis',(0.246022253877083,-0.0165067551769565,0.969123613183978));
#91582=DIRECTION('center_axis',(-0.159100969103341,-0.986495111013762,0.0389137196413171));
#91583=DIRECTION('ref_axis',(0.343278644332733,-0.0183212726723349,0.939054898987672));
#91584=DIRECTION('center_axis',(-0.877738926131253,-0.151718219821126,0.454484278417046));
#91585=DIRECTION('ref_axis',(0.466046492607051,-0.050113017262808,0.883339884885475));
#91586=DIRECTION('center_axis',(0.138347432677136,-0.986495109670028,-0.0876777421513839));
#91587=DIRECTION('ref_axis',(0.448603321542154,-0.0165067518838875,0.893578528750322));
#91588=DIRECTION('center_axis',(-0.147015974375736,-0.986495111209942,0.0722059473813417));
#91589=DIRECTION('ref_axis',(0.537122028018301,-0.01832126851174,0.843305554433047));
#91590=DIRECTION('center_axis',(-0.759517343082594,-0.151717542940859,0.632546593320007));
#91591=DIRECTION('ref_axis',(0.645042837663815,-0.0501177349543966,0.76250111489863));
#91592=DIRECTION('center_axis',(0.116264825694713,-0.986495109676388,-0.115368491759009));
#91593=DIRECTION('ref_axis',(0.63020819332302,-0.0165067493985915,0.77625070711261));
#91594=DIRECTION('center_axis',(-0.128056682568447,-0.986495111049509,0.1021218973824));
#91595=DIRECTION('ref_axis',(0.705850176713648,-0.0183212736053562,0.708124183294703));
#91596=DIRECTION('center_axis',(-0.605781406098869,-0.151717652691486,0.781031780330776));
#91597=DIRECTION('ref_axis',(0.793877240007919,-0.0501164462036934,0.606009298292791));
#91598=DIRECTION('center_axis',(0.088745798476136,-0.98649510963067,-0.13766474467926));
#91599=DIRECTION('ref_axis',(0.782345232961454,-0.0165067550744596,0.622626263098017));
#91600=DIRECTION('center_axis',(-0.103109596717397,-0.986495111163224,0.127262746771532));
#91601=DIRECTION('ref_axis',(0.84157356154396,-0.0183212714890313,0.539831706665364));
#91602=DIRECTION('center_axis',(-0.423719721590489,-0.151718143346513,0.89299675392174));
#91603=DIRECTION('ref_axis',(0.905590981485017,-0.0501174226749332,0.421180742909058));
#91604=DIRECTION('center_axis',(0.0570771178683077,-0.986495109613493,-0.153523943814994));
#91605=DIRECTION('ref_axis',(0.897900677527084,-0.0165067578719576,0.439888508875784));
#91606=DIRECTION('center_axis',(-0.0733412197425735,-0.986495111214254,
0.146452931131635));
#91607=DIRECTION('ref_axis',(0.937945899306877,-0.0183212681314,0.346297301617368));
#91608=DIRECTION('center_axis',(-0.221845691935971,-0.151717064722958,0.963206323298025));
#91609=DIRECTION('ref_axis',(0.97496017035715,-0.0501146364887038,0.216659154957188));
#91610=DIRECTION('center_axis',(0.0227395794411443,-0.986495109631334,-0.162204531996806));
#91611=DIRECTION('ref_axis',(0.971471285321496,-0.0165067549892282,0.236582055184933));
#91612=DIRECTION('center_axis',(-0.0401434924859694,-0.986495111144129,
0.158795137519262));
#91613=DIRECTION('ref_axis',(0.990460928248932,-0.0183212682441811,0.136570424112209));
#91614=DIRECTION('center_axis',(-0.00959814429645489,-0.151717275059204,
0.98837732879436));
#91615=DIRECTION('ref_axis',(0.998741475234698,-0.0501142782739623,0.0020061802260189));
#91616=DIRECTION('center_axis',(-0.0126612359133152,-0.986495109657588,
-0.163300617655936));
#91617=DIRECTION('ref_axis',(0.999616975098312,-0.0165067521155393,0.0222132894884525));
#91618=DIRECTION('center_axis',(-0.00506870264982865,-0.986495111101261,
0.163712259854776));
#91619=DIRECTION('ref_axis',(0.996663106113405,-0.0183212719598163,-0.0795423403361688));
#91620=DIRECTION('center_axis',(0.203098203142765,-0.151717556225375,0.96733288118061));
#91621=DIRECTION('ref_axis',(0.975822735790439,-0.0501139682928271,-0.212740636683284));
#91622=DIRECTION('center_axis',(-0.0474700324896744,-0.986495109609932,
-0.15676094772333));
#91623=DIRECTION('ref_axis',(0.981021686439629,-0.0165067559608459,-0.193194145208377));
#91624=DIRECTION('center_axis',(0.0302430998611894,-0.986495111138674,0.160974378738608));
#91625=DIRECTION('ref_axis',(0.956262424554126,-0.0183212694076787,-0.291935791695976));
#91626=DIRECTION('center_axis',(0.406297869111721,-0.151717737149366,0.901057029154954));
#91627=DIRECTION('ref_axis',(0.907275678259906,-0.0501130613714625,-0.417539848060047));
#91628=DIRECTION('center_axis',(-0.0800591757629436,-0.986495109678747,
-0.14289131168855));
#91629=DIRECTION('ref_axis',(0.916554913499942,-0.0165067516025223,-0.399568038875291));
#91630=DIRECTION('center_axis',(0.0641407687737649,-0.986495111249863,0.150709512842522));
#91631=DIRECTION('ref_axis',(0.871147975542361,-0.0183212658419171,-0.490678648329429));
#91632=DIRECTION('center_axis',(0.59049944203833,-0.151716819930788,0.792648986312674));
#91633=DIRECTION('ref_axis',(0.796304714906656,-0.0501187538296143,-0.602815818913203));
#91634=DIRECTION('center_axis',(-0.108904843684088,-0.986495109715032,-0.12234023675991));
#91635=DIRECTION('ref_axis',(0.809231052919238,-0.0165067504602018,-0.587258571823746));
#91636=DIRECTION('center_axis',(0.0950392811868488,-0.98649511117499,0.133397641131062));
#91637=DIRECTION('ref_axis',(0.745299613138979,-0.0183212695901069,-0.666477919915952));
#91638=DIRECTION('center_axis',(0.747089985754375,-0.151717860052369,0.647177135046238));
#91639=DIRECTION('ref_axis',(0.648100772001506,-0.050112252039179,-0.759904040999003));
#91640=DIRECTION('center_axis',(-0.132658243305986,-0.986495109701146,-0.096068668246692));
#91641=DIRECTION('ref_axis',(0.664068447290981,-0.0165067500876924,-0.747489548096887));
#91642=DIRECTION('center_axis',(0.121493865175172,-0.986495111116229,0.109848242901632));
#91643=DIRECTION('ref_axis',(0.584601872230696,-0.0183212697798802,-0.811113421204469));
#91644=DIRECTION('center_axis',(0.868747407713005,-0.15171756058632,0.471444295120506));
#91645=DIRECTION('ref_axis',(0.469591427508971,-0.050113881662551,-0.881460430237681));
#91646=DIRECTION('center_axis',(-0.150208694183325,-0.986495109644507,-0.0653050292030545));
#91647=DIRECTION('ref_axis',(0.487854736953721,-0.0165067565324189,-0.872768745212955));
#91648=DIRECTION('center_axis',(0.142267532383275,-0.986495111250233,0.0811624587414861));
#91649=DIRECTION('ref_axis',(0.396568795870637,-0.0183212660190013,-0.917822162160608));
#91650=DIRECTION('center_axis',(0.949783202322275,-0.15171717529495,0.273667256548837));
#91651=DIRECTION('ref_axis',(0.269124975424485,-0.0501127201189362,-0.961800635727099));
#91652=DIRECTION('center_axis',(-0.160735548480359,-0.986495109636274,-0.0314878090446884));
#91653=DIRECTION('ref_axis',(0.288829481865451,-0.0165067519944678,-0.957238244923346));
#91654=DIRECTION('center_axis',(0.156388925054862,-0.986495110977077,0.0486816201302798));
#91655=DIRECTION('ref_axis',(0.189992605884798,-0.0183212744051801,-0.98161455806914));
#91656=DIRECTION('center_axis',(0.986408331523745,-0.15171604175971,0.0630939472002521));
#91657=DIRECTION('ref_axis',(0.0560742479695429,-0.0501144507194969,-0.99716810044432));
#91658=DIRECTION('center_axis',(-0.163746588592943,-0.986495109681682,0.00380174937369959));
#91659=DIRECTION('ref_axis',(0.0762988819238041,-0.0165067512497135,-0.99694834759899));
#91660=DIRECTION('center_axis',(0.163197747944136,-0.986495111039129,0.0139244734858598));
#91661=DIRECTION('ref_axis',(-0.0254674285246704,-0.0183212728921532,-0.999507749366633));
#91662=DIRECTION('center_axis',(0.97690981282241,-0.151717025902171,-0.150429922763672));
#91663=DIRECTION('ref_axis',(0.159598986590751,0.0501170508921964,0.985908943406578));
#91664=DIRECTION('center_axis',(-0.159101021139896,-0.986495109712914,0.0389135398640145));
#91665=DIRECTION('ref_axis',(-0.139799366336145,-0.0165067486026133,-0.990042253857169));
#91666=DIRECTION('center_axis',(0.162375622482608,-0.986495111326154,-0.0214837741792473));
#91667=DIRECTION('ref_axis',(-0.239736640226715,-0.0183212636861886,-0.97066506820311));
#91668=DIRECTION('center_axis',(0.921732155192996,-0.15171733944031,-0.356919715057081));
#91669=DIRECTION('ref_axis',(0.367808905001473,0.050116359261509,0.928549923232989));
#91670=DIRECTION('center_axis',(-0.147016065905711,-0.986495109664305,0.0722057821370199));
#91671=DIRECTION('ref_axis',(-0.3493607543486,-0.016506751405448,-0.936842884628482));
#91672=DIRECTION('center_axis',(0.153960995330712,-0.986495111268092,-0.0558874526251794));
#91673=DIRECTION('ref_axis',(-0.44279602738596,-0.0183212658114637,-0.896435167399337));
#91674=DIRECTION('center_axis',(0.823455469926704,-0.151716935206564,-0.546720276393073));
#91675=DIRECTION('ref_axis',(0.558820565354594,0.050117521772302,0.827772800802355));
#91676=DIRECTION('center_axis',(-0.128056801261591,-0.986495109619452,0.102121762360211));
#91677=DIRECTION('ref_axis',(-0.542586422548281,-0.016506754690969,-0.839837782619852));
#91678=DIRECTION('center_axis',(0.138347322118367,-0.98649511126866,-0.0876778986159592));
#91679=DIRECTION('ref_axis',(-0.625150763581123,-0.0183212647737682,-0.780288955484459));
#91680=DIRECTION('center_axis',(0.68667463949011,-0.151717825667281,-0.710956848800207));
#91681=DIRECTION('ref_axis',(0.723702229126702,0.0501140848303044,0.688290390793496));
#91682=DIRECTION('center_axis',(-0.103109741187975,-0.986495109566151,0.12726264209978));
#91683=DIRECTION('ref_axis',(-0.71044135220098,-0.0165067586843161,-0.703562798903254));
#91684=DIRECTION('center_axis',(0.116264690677343,-0.986495110958096,-0.115368616865576));
#91685=DIRECTION('ref_axis',(-0.778274144616829,-0.0183212748608229,-0.627657300370527));
#91686=DIRECTION('center_axis',(0.517785944433882,-0.151717455051538,-0.841949837923494));
#91687=DIRECTION('ref_axis',(0.854744488964346,0.0501132715862331,0.51662415603222));
#91688=DIRECTION('center_axis',(-0.0733413911618107,-0.986495109608882,
0.146452856101237));
#91689=DIRECTION('ref_axis',(-0.845076832735351,-0.016506753357528,-0.534390001653831));
#91690=DIRECTION('center_axis',(0.0887456442096499,-0.986495110967044,-0.137664834550924));
#91691=DIRECTION('ref_axis',(-0.895006294111261,-0.0183212747084494,-0.445677085336778));
#91692=DIRECTION('center_axis',(0.324686099978472,-0.151717310764794,-0.933574203850486));
#91693=DIRECTION('ref_axis',(0.945819951730904,0.0501143506520829,0.320800827253406));
#91694=DIRECTION('center_axis',(-0.0401436795793762,-0.986495109668196,
0.158795099390891));
#91695=DIRECTION('ref_axis',(-0.940197459534588,-0.0165067489361094,-0.340229722870104));
#91696=DIRECTION('center_axis',(0.0570769443776299,-0.986495111169136,-0.153523998319181));
#91697=DIRECTION('ref_axis',(-0.96988894388744,-0.0183212688445451,-0.242857504790015));
#91698=DIRECTION('center_axis',(0.116404160762717,-0.15171785945768,-0.981545598777106));
#91699=DIRECTION('ref_axis',(0.99266997303653,0.0501125960185313,0.109977508391213));
#91700=DIRECTION('center_axis',(-0.00506888908992799,-0.986495109651168,
0.163712262820244));
#91701=DIRECTION('ref_axis',(-0.991355498490221,-0.0165067503541939,-0.130160680721753));
#91702=DIRECTION('center_axis',(0.0227393958052857,-0.986495111211627,-0.162204548129732));
#91703=DIRECTION('ref_axis',(-0.999420664067506,-0.0183212690319746,-0.0286821780191654));
#91704=DIRECTION('center_axis',(-0.0973205419698992,-0.151717505250181,
-0.983621121525634));
#91705=DIRECTION('ref_axis',(0.993103478144611,0.0501177905127186,-0.105989097416662));
#91706=DIRECTION('center_axis',(0.030242922023399,-0.986495109621249,0.160974421449018));
#91707=DIRECTION('ref_axis',(-0.996158856524345,-0.0165067564987743,0.0859945321401235));
#91708=DIRECTION('center_axis',(-0.0126614273468348,-0.986495111313728,
-0.163300592808647));
#91709=DIRECTION('ref_axis',(-0.98222058466164,-0.018321263438133,0.186834296565104));
#91710=DIRECTION('center_axis',(-0.306494682242744,-0.15171728831044,-0.939703609753972));
#91711=DIRECTION('ref_axis',(0.947101109183711,0.0501142032663003,-0.316998510428627));
#91712=DIRECTION('center_axis',(0.0641406002607645,-0.986495109654418,0.150709595003457));
#91713=DIRECTION('ref_axis',(-0.954382933050281,-0.0165067548247208,0.298128737540512));
#91714=DIRECTION('center_axis',(-0.0474702053972094,-0.986495111161419,
-0.156760885600221));
#91715=DIRECTION('ref_axis',(-0.919092961586165,-0.0183212694610228,0.393614607259574));
#91716=DIRECTION('center_axis',(-0.501337540466072,-0.151717802549987,-0.851846452659652));
#91717=DIRECTION('ref_axis',(0.856813384458168,0.0501114100958997,-0.513185805329357));
#91718=DIRECTION('center_axis',(0.0950391340828693,-0.986495109692731,0.133397756896831));
#91719=DIRECTION('ref_axis',(-0.867981124429243,-0.0165067517519525,0.496322772781127));
#91720=DIRECTION('center_axis',(-0.0800593355866944,-0.986495111179507,
-0.142891211781377));
#91721=DIRECTION('ref_axis',(-0.812989574428096,-0.018321268404428,0.581989933757686));
#91722=DIRECTION('center_axis',(-0.672738355704087,-0.151718004685065,-0.724157960543792));
#91723=DIRECTION('ref_axis',(0.726461248877051,0.0501149835492891,-0.685377663995442));
#91724=DIRECTION('center_axis',(0.12149374987299,-0.986495109615189,0.109848383907616));
#91725=DIRECTION('ref_axis',(-0.740993483164264,-0.0165067564236307,0.671309306430696));
#91726=DIRECTION('center_axis',(-0.108904976768055,-0.986495111066147,-0.12234010739631));
#91727=DIRECTION('ref_axis',(-0.668871699073879,-0.0183212724760737,0.743152057894534));
#91728=DIRECTION('center_axis',(-0.812682678127263,-0.151717508345289,-0.562608800440765));
#91729=DIRECTION('ref_axis',(0.562140841754344,0.0501169055115351,-0.825521634976132));
#91730=DIRECTION('center_axis',(0.142267445198958,-0.986495109697153,0.0811626304413822));
#91731=DIRECTION('ref_axis',(-0.579357812530632,-0.0165067500527332,0.814906161629925));
#91732=DIRECTION('center_axis',(-0.132658347439609,-0.986495111193847,-0.0960685091236052));
#91733=DIRECTION('ref_axis',(-0.49347812376278,-0.0183212686064254,0.869565220374077));
#91734=DIRECTION('center_axis',(-0.914626796186742,-0.151718440025845,-0.374752369776762));
#91735=DIRECTION('ref_axis',(0.371535595523368,0.0501154652021563,-0.927065122527359));
#91736=DIRECTION('center_axis',(0.156388880614704,-0.986495109593218,0.0486817909360894));
#91737=DIRECTION('ref_axis',(-0.390632011378624,-0.0165067574930132,0.920398912778235));
#91738=DIRECTION('center_axis',(-0.150208759826364,-0.98649511129442,-0.0653048532931189));
#91739=DIRECTION('ref_axis',(-0.295010059307927,-0.0183212646087627,0.955318478922223));
#91740=DIRECTION('center_axis',(-0.973804122239227,-0.151717542567578,-0.169373311909354));
#91741=DIRECTION('ref_axis',(0.163558175448119,0.0501137165392175,-0.985260036060892));
#91742=DIRECTION('center_axis',(0.163197741587199,-0.986495109592965,0.0139246504444709));
#91743=DIRECTION('ref_axis',(-0.183640690842074,-0.0165067579730875,0.982854833435876));
#91744=DIRECTION('center_axis',(-0.160735575288252,-0.986495110973083,-0.0314876303166706));
#91745=DIRECTION('ref_axis',(-0.0827476582594976,-0.0183212754840253,0.996402105536318));
#91746=DIRECTION('',(-0.727460699689282,0.,-0.686149349928702));
#91747=DIRECTION('center_axis',(-1.25690178608446E-15,1.,-9.080314930603E-15));
#91748=DIRECTION('ref_axis',(-5.55903758767046E-33,9.080314930603E-15,1.));
#91749=DIRECTION('',(-0.513725008301344,0.,0.85795490315388));
#91750=DIRECTION('',(-0.857954900607409,0.,-0.51372501255412));
#91751=DIRECTION('center_axis',(1.05983846877379E-15,1.,2.86594181608156E-15));
#91752=DIRECTION('ref_axis',(-3.99900629564538E-33,-2.86594181608156E-15,
1.));
#91753=DIRECTION('',(-0.317279460074916,0.,0.94833208540815));
#91754=DIRECTION('',(-0.948332083835433,0.,-0.317279464775685));
#91755=DIRECTION('center_axis',(-3.30230561415707E-15,1.,-5.14220749173894E-15));
#91756=DIRECTION('ref_axis',(1.24299482632711E-32,5.14220749173894E-15,
1.));
#91757=DIRECTION('',(-0.105998278540163,0.,0.994366313260119));
#91758=DIRECTION('',(-0.994366313149823,0.,-0.105998279574853));
#91759=DIRECTION('center_axis',(4.33052217016942E-15,1.,4.31208746369059E-15));
#91760=DIRECTION('ref_axis',(-1.,4.33052217016942E-15,8.38946777378104E-34));
#91761=DIRECTION('',(0.110239267677841,0.,0.993905077893183));
#91762=DIRECTION('',(-0.993905078391756,0.,0.110239263182761));
#91763=DIRECTION('center_axis',(5.15624828916998E-15,1.,3.28033898500044E-15));
#91764=DIRECTION('ref_axis',(-1.,5.15624828916998E-15,-1.49357535274459E-32));
#91765=DIRECTION('',(0.321322147950303,0.,0.946969945265743));
#91766=DIRECTION('',(-0.946969946451846,0.,0.321322144454732));
#91767=DIRECTION('center_axis',(-5.74087398687763E-15,1.,-2.09520551914698E-15));
#91768=DIRECTION('ref_axis',(-1.,-5.74087398687763E-15,3.57632832502997E-33));
#91769=DIRECTION('',(0.517380359614974,0.,0.855755551243859));
#91770=DIRECTION('',(-0.855755553808469,0.,0.517380355373066));
#91771=DIRECTION('center_axis',(1.81711884491992E-14,1.,2.43630771816283E-15));
#91772=DIRECTION('ref_axis',(-1.,1.81711884491992E-14,1.11444476857717E-32));
#91773=DIRECTION('',(0.689246444718554,0.,0.724526975648825));
#91774=DIRECTION('',(-0.724526980936391,0.,0.689246439160332));
#91775=DIRECTION('center_axis',(3.0450150389411E-15,1.,-2.54486696300814E-16));
#91776=DIRECTION('ref_axis',(0.996525810855685,-3.05563087855382E-15,-0.0832845021502743));
#91777=DIRECTION('',(0.828884127273459,0.,0.559420328155955));
#91778=DIRECTION('',(-0.559420334090901,0.,0.828884123267918));
#91779=DIRECTION('center_axis',(-2.91911716366775E-15,1.,9.03125162278983E-16));
#91780=DIRECTION('ref_axis',(-1.,-2.91911716366775E-15,2.14129740204536E-33));
#91781=DIRECTION('',(0.929764111872082,0.,0.36815580434745));
#91782=DIRECTION('',(-0.36815581236092,0.,0.929764108699013));
#91783=DIRECTION('center_axis',(-7.97017386303574E-15,1.,4.52860351294214E-15));
#91784=DIRECTION('ref_axis',(-1.,-7.97017386303574E-15,-2.95419996546644E-32));
#91785=DIRECTION('',(0.987169358889856,0.,0.15967672613437));
#91786=DIRECTION('',(-0.159676734244941,0.,0.987169357577954));
#91787=DIRECTION('center_axis',(9.08042628672507E-15,1.,-8.18143872634072E-15));
#91788=DIRECTION('ref_axis',(-1.,9.08042628672507E-15,-3.70960009999131E-32));
#91789=DIRECTION('',(0.998415664035658,0.,-0.0562686574234377));
#91790=DIRECTION('',(0.0562686524743697,0.,0.998415664314577));
#91791=DIRECTION('center_axis',(0.,1.,0.));
#91792=DIRECTION('ref_axis',(0.,0.,1.));
#91793=DIRECTION('',(0.962977162506725,0.,-0.269582982568442));
#91794=DIRECTION('',(0.269582977795087,0.,0.962977163843013));
#91795=DIRECTION('center_axis',(-1.20146868912725E-15,1.,2.80951118861022E-15));
#91796=DIRECTION('ref_axis',(8.0043662084072E-33,-2.80951118861022E-15,
1.));
#91797=DIRECTION('',(0.882510919242445,0.,-0.47029190660467));
#91798=DIRECTION('',(0.470291902230154,0.,0.882510921573633));
#91799=DIRECTION('center_axis',(1.70825147914177E-15,1.,-9.00631986261566E-15));
#91800=DIRECTION('ref_axis',(7.81898694697755E-33,9.00631986261566E-15,
1.));
#91801=DIRECTION('',(0.76077944621245,0.,-0.649010503937092));
#91802=DIRECTION('',(0.649010502445546,0.,0.760779447484867));
#91803=DIRECTION('center_axis',(-8.92596786684004E-17,1.,-3.05432689493444E-15));
#91804=DIRECTION('ref_axis',(-0.0292115384811887,-3.05563087943486E-15,
-0.999573251952833));
#91805=DIRECTION('',(0.60347477344143,0.,-0.797382090230157));
#91806=DIRECTION('',(0.797382087238821,0.,0.603474777393936));
#91807=DIRECTION('center_axis',(7.43762836885792E-16,1.,2.96373024743229E-15));
#91808=DIRECTION('ref_axis',(1.6716588985035E-33,-2.96373024743229E-15,
1.));
#91809=DIRECTION('',(0.417952286130124,0.,-0.908468979392584));
#91810=DIRECTION('',(0.908468975825409,0.,0.417952293883803));
#91811=DIRECTION('center_axis',(-6.81744233180193E-15,1.,-1.36727642357042E-14));
#91812=DIRECTION('ref_axis',(2.6826757076957E-33,1.36727642357042E-14,1.));
#91813=DIRECTION('',(0.212886820908125,8.54029260079142E-16,-0.977076865698719));
#91814=DIRECTION('',(0.977076864643463,0.,0.212886825751384));
#91815=DIRECTION('center_axis',(1.9194588930583E-15,1.,2.37751080585885E-15));
#91816=DIRECTION('ref_axis',(-9.07626131178252E-33,-2.37751080585885E-15,
1.));
#91817=DIRECTION('',(-0.00213299954342001,0.,-0.999997725153886));
#91818=DIRECTION('',(0.999997725164459,0.,-0.00213299458654189));
#91819=DIRECTION('center_axis',(-7.15703269032E-15,1.,-5.72789702230434E-15));
#91820=DIRECTION('ref_axis',(-1.,-7.15703269032E-15,-3.32432154402052E-32));
#91821=DIRECTION('',(-0.217053081214603,0.,-0.976159802458208));
#91822=DIRECTION('',(0.976159802699633,0.,-0.217053080128833));
#91823=DIRECTION('center_axis',(1.09613783869135E-14,1.,5.40724200926739E-15));
#91824=DIRECTION('ref_axis',(-1.,1.09613783869135E-14,1.13030402369742E-32));
#91825=DIRECTION('',(-0.421824003608544,0.,-0.90667773215165));
#91826=DIRECTION('',(0.90667773424259,0.,-0.421823999114232));
#91827=DIRECTION('center_axis',(5.9337522978211E-15,1.,1.46222567279051E-15));
#91828=DIRECTION('ref_axis',(-1.,5.9337522978211E-15,2.62712725445791E-33));
#91829=DIRECTION('',(-0.606870906241449,0.,-0.794800417185146));
#91830=DIRECTION('',(0.794800422093049,0.,-0.606870899813718));
#91831=DIRECTION('',(-0.763541194667019,0.,-0.645759122309907));
#91832=DIRECTION('',(0.645759126094686,0.,-0.763541191466071));
#91833=DIRECTION('center_axis',(-2.99965019018643E-15,1.,5.82218923504121E-16));
#91834=DIRECTION('ref_axis',(-1.,-2.99965019018643E-15,-2.3362086080716E-33));
#91835=DIRECTION('',(-0.884509150646489,0.,-0.466522842337465));
#91836=DIRECTION('',(0.466522846721858,0.,-0.884509148333998));
#91837=DIRECTION('center_axis',(0.,1.,0.));
#91838=DIRECTION('ref_axis',(0.,0.,1.));
#91839=DIRECTION('',(-0.964118438699621,0.,-0.265472477216386));
#91840=DIRECTION('',(0.265472480987239,0.,-0.964118437661307));
#91841=DIRECTION('center_axis',(1.48676483391871E-14,1.,-1.07275680003584E-14));
#91842=DIRECTION('ref_axis',(-1.,1.48676483391871E-14,7.22009769445324E-32));
#91843=DIRECTION('',(-0.99864662067696,0.,-0.0520089127985631));
#91844=DIRECTION('',(0.0520089175439887,0.,-0.998646620429821));
#91845=DIRECTION('center_axis',(0.,1.,0.));
#91846=DIRECTION('ref_axis',(0.,0.,1.));
#91847=DIRECTION('',(-0.986479196610341,0.,0.16388652981565));
#91848=DIRECTION('',(-0.163886525562761,0.,-0.986479197316885));
#91849=DIRECTION('center_axis',(-1.49818721583241E-15,1.,2.66314009076519E-15));
#91850=DIRECTION('ref_axis',(-9.34860545733725E-33,-2.66314009076519E-15,
1.));
#91851=DIRECTION('',(-0.928185102079373,0.,0.372118820107106));
#91852=DIRECTION('',(-0.372118815506532,0.,-0.928185103923789));
#91853=DIRECTION('center_axis',(0.,1.,0.));
#91854=DIRECTION('ref_axis',(0.,0.,1.));
#91855=DIRECTION('',(-0.826490103338909,0.,0.562951249295035));
#91856=DIRECTION('',(-0.562951245198655,0.,-0.826490106129096));
#91857=DIRECTION('',(-0.686149346322776,0.,0.727460703090433));
#91858=DIRECTION('center_axis',(-0.15848403150235,-0.986495984567242,0.0413338141413225));
#91859=DIRECTION('ref_axis',(0.0350633407380601,0.0362133149627294,0.99872877096622));
#91860=DIRECTION('center_axis',(-0.938019368552222,0.33683080843185,0.0816374345018055));
#91861=DIRECTION('ref_axis',(0.111380041292018,0.0699109451028969,0.991315765110496));
#91862=DIRECTION('center_axis',(0.153961047147948,-0.986495109309872,-0.0558873444422921));
#91863=DIRECTION('ref_axis',(0.14261632231053,-0.0337827101182837,0.989201351145298));
#91864=DIRECTION('center_axis',(-0.145893126005734,-0.986495977860338,0.0744370972677616));
#91865=DIRECTION('ref_axis',(0.24894077710909,0.0362135888321499,0.967841446455058));
#91866=DIRECTION('center_axis',(0.138347359563849,-0.986495107011068,-0.087677887434251));
#91867=DIRECTION('ref_axis',(0.351931117601902,-0.0337827964682365,0.935416063111096));
#91868=DIRECTION('center_axis',(-0.126480595970886,-0.986495984693773,0.104059266891101));
#91869=DIRECTION('ref_axis',(0.451177953046194,0.0362133096746333,0.891698968759893));
#91870=DIRECTION('center_axis',(-0.817045250682722,0.336828066332674,0.467957169052254));
#91871=DIRECTION('ref_axis',(0.517325436789001,0.0698987637591658,0.852929396419194));
#91872=DIRECTION('center_axis',(0.116264722410286,-0.986495107075066,-0.115368618089205));
#91873=DIRECTION('ref_axis',(0.544789966623712,-0.0337827941729723,0.837891768120443));
#91874=DIRECTION('center_axis',(-0.101153885558881,-0.986495984771876,0.128816006246538));
#91875=DIRECTION('ref_axis',(0.632318582174376,0.0362133068361477,0.773861620087841));
#91876=DIRECTION('center_axis',(-0.697347637158444,0.336818240845437,0.63266084562214));
#91877=DIRECTION('ref_axis',(0.688594792234753,0.0699401336332757,0.721765605868371));
#91878=DIRECTION('center_axis',(0.0887457649462112,-0.986495111389322,-0.137664753692004));
#91879=DIRECTION('ref_axis',(0.712175030652464,-0.0337826696403138,0.701188602978639));
#91880=DIRECTION('center_axis',(-0.0710973252204614,-0.986495984603397,
0.147549458514326));
#91881=DIRECTION('ref_axis',(0.783892697096572,0.0362133134291354,0.619839362552222));
#91882=DIRECTION('center_axis',(-0.545039958943152,0.336830199657565,0.7677739639724));
#91883=DIRECTION('ref_axis',(0.827653466131635,0.0699408221214351,0.556864455142603));
#91884=DIRECTION('center_axis',(0.0570769811588049,-0.986495107182151,-0.15352401026378));
#91885=DIRECTION('ref_axis',(0.846259603654513,-0.0337827915677679,0.531698604677872));
#91886=DIRECTION('center_axis',(-0.0377163388188591,-0.986495984668493,
0.159383656687384));
#91887=DIRECTION('ref_axis',(0.898812861906938,0.0362133117090608,0.436834105039571));
#91888=DIRECTION('center_axis',(-0.367248269483428,0.336821700094295,0.866994723690413));
#91889=DIRECTION('ref_axis',(0.928010666644119,0.0699038870008591,0.36593667372499));
#91890=DIRECTION('center_axis',(0.0227394276772378,-0.986495107102228,-0.162204568654139));
#91891=DIRECTION('ref_axis',(0.940774007298495,-0.0337827931227811,0.337346987655669));
#91892=DIRECTION('center_axis',(-0.00257177596363353,-0.986495984633055,
0.163765253552922));
#91893=DIRECTION('ref_axis',(0.971705536836301,0.0362133124927908,0.233402968447226));
#91894=DIRECTION('center_axis',(-0.17228471282127,0.336828211432767,0.925669883765857));
#91895=DIRECTION('ref_axis',(0.984979646001483,0.0699121935542017,0.157884078219537));
#91896=DIRECTION('center_axis',(-0.012661393005518,-0.986495107143346,-0.163300620664463));
#91897=DIRECTION('ref_axis',(0.991298864141802,-0.033782791285507,0.127221401360515));
#91898=DIRECTION('center_axis',(0.0326933264329512,-0.986495977672573,0.160489353050549));
#91899=DIRECTION('ref_axis',(0.999162330746507,0.0362135961898777,0.0190581286648048));
#91900=DIRECTION('center_axis',(-0.0474700622167946,-0.986495111334321,
-0.15676092786986));
#91901=DIRECTION('ref_axis',(0.995471693573044,-0.0337826708549142,-0.0888529034118977));
#91902=DIRECTION('center_axis',(0.0664291596833768,-0.986495984759072,0.149709180740495));
#91903=DIRECTION('ref_axis',(0.979899423791816,0.0362133078390561,-0.196177765273798));
#91904=DIRECTION('center_axis',(0.232319120060856,0.33682143884262,0.912457749591803));
#91905=DIRECTION('ref_axis',(0.960238518096396,0.0699024925997113,-0.270288049851236));
#91906=DIRECTION('center_axis',(-0.0800592438663563,-0.986495109214833,
-0.142891276734311));
#91907=DIRECTION('ref_axis',(0.953097375335365,-0.0337827147074441,-0.300772540827507));
#91908=DIRECTION('center_axis',(0.0970591332333997,-0.986495984709624,0.131928756561151));
#91909=DIRECTION('ref_axis',(0.914817498304034,0.0362133096668296,-0.402240650605732));
#91910=DIRECTION('center_axis',(0.423036348843129,0.336829845929339,0.84118125421855));
#91911=DIRECTION('ref_axis',(0.879683708655244,0.0699088058937639,-0.470392741849896));
#91912=DIRECTION('center_axis',(-0.108904901561428,-0.9864951092803,-0.122340188744111));
#91913=DIRECTION('ref_axis',(0.866157283339105,-0.033782712011013,-0.498628407622152));
#91914=DIRECTION('center_axis',(0.123150730753704,-0.986495984587636,0.10797948836376));
#91915=DIRECTION('ref_axis',(0.80695972441348,0.0362133140582691,-0.589495206985975));
#91916=DIRECTION('center_axis',(0.593975878583261,0.336827700107494,0.730574948996706));
#91917=DIRECTION('ref_axis',(0.757987105710624,0.0699415758510974,-0.64850884615701));
#91918=DIRECTION('center_axis',(-0.132658256173775,-0.98649511141531,-0.096068632875815));
#91919=DIRECTION('ref_axis',(0.738716629391971,-0.0337826676212503,-0.673168977915766));
#91920=DIRECTION('center_axis',(0.14348393489496,-0.986495984508783,0.0789812191290125));
#91921=DIRECTION('ref_axis',(0.661369408704425,0.0362133163355927,-0.749185625162374));
#91922=DIRECTION('center_axis',(0.737147022152457,0.336812593121351,0.585808454058694));
#91923=DIRECTION('ref_axis',(0.600863234638785,0.0699142232257434,-0.796288499634496));
#91924=DIRECTION('center_axis',(-0.150208723144297,-0.98649510928717,-0.0653049679875403));
#91925=DIRECTION('ref_axis',(0.576734425562987,-0.033782710717192,-0.816232890067002));
#91926=DIRECTION('center_axis',(0.157108107777897,-0.9864959776017,0.0462896170443781));
#91927=DIRECTION('ref_axis',(0.484854153870186,0.0362135990806186,-0.873844966064607));
#91928=DIRECTION('center_axis',(-0.160735593006857,-0.98649510717186,-0.0314876589589351));
#91929=DIRECTION('ref_axis',(0.387784716648915,-0.0337827905276527,-0.921130683778195));
#91930=DIRECTION('center_axis',(0.163385845130553,-0.986495984561036,0.0114340743362717));
#91931=DIRECTION('ref_axis',(0.285667736486251,0.0362133139781328,-0.957644266009849));
#91932=DIRECTION('center_axis',(0.914985932287573,0.336825827252756,0.222146586314842));
#91933=DIRECTION('ref_axis',(-0.210968968536098,-0.069936861305119,0.974987656201659));
#91934=DIRECTION('center_axis',(-0.163746599808111,-0.986495107226504,0.0038019033984307));
#91935=DIRECTION('ref_axis',(0.180702658065741,-0.0337827878854193,-0.982957411392103));
#91936=DIRECTION('center_axis',(0.162023962635347,-0.986495984640472,-0.0239563732682202));
#91937=DIRECTION('ref_axis',(0.0731237773961302,0.0362133127214665,-0.996665194115385));
#91938=DIRECTION('center_axis',(0.941351387233131,0.336819278548466,0.0202568347070788));
#91939=DIRECTION('ref_axis',(0.00353863569141246,-0.0698840097142687,0.997548847547677));
#91940=DIRECTION('center_axis',(-0.159101001700983,-0.986495111312731,0.0389135787846211));
#91941=DIRECTION('ref_axis',(-0.034828839057642,-0.0337826723898334,-0.998822147840194));
#91942=DIRECTION('center_axis',(0.153085958589943,-0.986495977708609,-0.0582269288846109));
#91943=DIRECTION('ref_axis',(-0.142839410301014,0.0362135954076269,-0.989083150383481));
#91944=DIRECTION('center_axis',(-0.147016009206128,-0.986495107099126,0.0722059326273673));
#91945=DIRECTION('ref_axis',(-0.2487318162409,-0.0337827937137362,-0.967983061028652));
#91946=DIRECTION('center_axis',(0.136989946942366,-0.986495984715003,-0.0897743091196212));
#91947=DIRECTION('ref_axis',(-0.352123510109114,0.0362133099323452,-0.935252709064337));
#91948=DIRECTION('center_axis',(0.862847394774504,0.336841301078536,-0.376871743725329));
#91949=DIRECTION('ref_axis',(0.422071567400847,-0.0698917385670996,0.90386433543528));
#91950=DIRECTION('center_axis',(-0.128056773935998,-0.98649511147343,0.102121778716044));
#91951=DIRECTION('ref_axis',(-0.451004333228506,-0.0337826658124416,-0.891882179942909));
#91952=DIRECTION('center_axis',(0.114488192993927,-0.986495977375508,-0.117124464937633));
#91953=DIRECTION('ref_axis',(-0.544942774640645,0.0362136074895554,-0.837690842136613));
#91954=DIRECTION('center_axis',(-0.10310962985091,-0.986495106995456,0.127262752233448));
#91955=DIRECTION('ref_axis',(-0.632188419435967,-0.0337827973549945,-0.774077854568857));
#91956=DIRECTION('center_axis',(0.0866334501130605,-0.98649598453504,-0.138997546085356));
#91957=DIRECTION('ref_axis',(-0.712281062451427,0.0362133159577758,-0.700959545066909));
#91958=DIRECTION('center_axis',(0.624856068326553,0.336828197978433,-0.704344843753458));
#91959=DIRECTION('ref_axis',(0.762585940723454,-0.0698942588923449,0.643099895494327));
#91960=DIRECTION('center_axis',(-0.0733412580463798,-0.986495107141828,
0.146452939381247));
#91961=DIRECTION('ref_axis',(-0.783812062389502,-0.0337827924995709,-0.6200785222725));
#91962=DIRECTION('center_axis',(0.0547276501215202,-0.986495984686042,-0.154371488658016));
#91963=DIRECTION('ref_axis',(-0.846313909511036,0.0362133094747293,-0.531452126522261));
#91964=DIRECTION('center_axis',(0.458834021409677,0.336824951473368,-0.822204532255805));
#91965=DIRECTION('ref_axis',(0.88300882564239,-0.0699331565184644,0.464117191512026));
#91966=DIRECTION('center_axis',(-0.0401436056662108,-0.986495109253376,
0.158795120653264));
#91967=DIRECTION('ref_axis',(-0.898785511585147,-0.0337827124044028,-0.437085040360829));
#91968=DIRECTION('center_axis',(0.0202625544542091,-0.98649597750738,-0.162527275399387));
#91969=DIRECTION('ref_axis',(-0.940774062452267,0.0362136030624955,-0.337094554050181));
#91970=DIRECTION('center_axis',(-0.00506873401270936,-0.986495107235941,
0.163712282175342));
#91971=DIRECTION('ref_axis',(-0.971732775235418,-0.0337827882866994,-0.233653882374867));
#91972=DIRECTION('center_axis',(-0.0151497303550186,-0.986495977559997,
-0.163083328173411));
#91973=DIRECTION('ref_axis',(-0.99124465228558,0.0362136008272741,-0.126974857473291));
#91974=DIRECTION('center_axis',(0.0302430763953997,-0.986495107146461,0.160974407612619));
#91975=DIRECTION('ref_axis',(-0.999242880739712,-0.0337827931806898,-0.0192973618899598));
#91976=DIRECTION('center_axis',(-0.0498533426929182,-0.986495984676177,
-0.156013834130575));
#91977=DIRECTION('ref_axis',(-0.995365758355286,0.0362133105381907,0.0890820028606839));
#91978=DIRECTION('center_axis',(-0.132302540794811,0.3368243442411,-0.932226044919252));
#91979=DIRECTION('ref_axis',(0.983828622997496,-0.0699356922579925,-0.164894631565877));
#91980=DIRECTION('center_axis',(0.0641407497217067,-0.986495107067512,0.150709548327221));
#91981=DIRECTION('ref_axis',(-0.980029499961363,-0.0337827935857002,0.195961481069693));
#91982=DIRECTION('center_axis',(-0.0822261691028225,-0.986495984453687,
-0.141649319699833));
#91983=DIRECTION('ref_axis',(-0.952944661855718,0.0362133180488912,0.300973532119657));
#91984=DIRECTION('center_axis',(-0.329609608358645,0.336827084253146,-0.881989241085845));
#91985=DIRECTION('ref_axis',(0.925374513598419,-0.0699627075030704,-0.372541580419325));
#91986=DIRECTION('center_axis',(0.0950392721431884,-0.986495107089222,0.133397677789074));
#91987=DIRECTION('ref_axis',(-0.914991029827499,-0.0337827934393961,0.402057381728833));
#91988=DIRECTION('center_axis',(-0.110754182085875,-0.986495984521845,-0.120661442361528));
#91989=DIRECTION('ref_axis',(-0.865964932744586,0.0362133163850253,0.498791871398344));
#91990=DIRECTION('center_axis',(-0.511503841068363,0.336830860392663,-0.790511727970844));
#91991=DIRECTION('ref_axis',(0.823675742451526,-0.0698814821935577,-0.562738704678609));
#91992=DIRECTION('center_axis',(0.121493796088995,-0.986495109316191,0.109848335477251));
#91993=DIRECTION('ref_axis',(-0.807168618800916,-0.0337827102832155,0.589353501142516));
#91994=DIRECTION('center_axis',(-0.134103453923623,-0.98649598450797,-0.0940315702060031));
#91995=DIRECTION('ref_axis',(-0.73849364637247,0.0362133159122535,0.673287256687762));
#91996=DIRECTION('center_axis',(-0.669485258183011,0.336821850718734,-0.662072903805944));
#91997=DIRECTION('ref_axis',(0.683427665385484,-0.069939876813133,-0.726660195564));
#91998=DIRECTION('center_axis',(0.142267537250305,-0.986495107164757,0.0811624998674068));
#91999=DIRECTION('ref_axis',(-0.661603853930092,-0.0337827916166257,0.749092159520734));
#92000=DIRECTION('center_axis',(-0.151182194028678,-0.986495984697426,-0.0630048917508035));
#92001=DIRECTION('ref_axis',(-0.576491219554483,0.0362133092547474,0.816300477771148));
#92002=DIRECTION('center_axis',(-0.79615852923434,0.336823429075849,-0.502674421423052));
#92003=DIRECTION('ref_axis',(0.511233079746866,-0.0699576495711029,-0.856590138537108));
#92004=DIRECTION('center_axis',(0.156388938553649,-0.986495107211372,0.0486816530747087));
#92005=DIRECTION('ref_axis',(-0.485103252326991,-0.0337827889325442,0.873804072864));
#92006=DIRECTION('center_axis',(-0.161191827682753,-0.986495984704173,-0.0290321692409841));
#92007=DIRECTION('ref_axis',(-0.387532702915014,0.0362133097251902,0.921144397133333));
#92008=DIRECTION('center_axis',(-0.885603712736837,0.336826499306086,-0.319771751960576));
#92009=DIRECTION('ref_axis',(-0.315168257278309,0.069878409286689,0.946459707288015));
#92010=DIRECTION('center_axis',(0.163197749307222,-0.986495109254072,0.0139245839741768));
#92011=DIRECTION('ref_axis',(-0.285919796784119,-0.0337827117026771,0.957657871161169));
#92012=DIRECTION('center_axis',(-0.163664310470787,-0.986495984716146,0.00629806454745587));
#92013=DIRECTION('ref_axis',(-0.180453584359339,0.0362133089092276,0.982916629297578));
#92014=DIRECTION('center_axis',(-0.933640852264392,0.336824940607712,-0.121916850220263));
#92015=DIRECTION('ref_axis',(-0.10432265313841,0.0699226078440237,0.992082462779407));
#92016=DIRECTION('center_axis',(0.16237565034875,-0.986495109299984,-0.0214836566029404));
#92017=DIRECTION('ref_axis',(-0.0733670170758494,-0.0337827112753311,0.996732666879279));
#92018=DIRECTION('center_axis',(0.,-1.,0.));
#92019=DIRECTION('ref_axis',(0.,0.,-1.));
#92020=DIRECTION('',(-0.603364206226571,0.,0.797465757662723));
#92021=DIRECTION('center_axis',(0.158479767859181,0.986495111177158,-0.0413709898705178));
#92022=DIRECTION('ref_axis',(0.182060716416353,0.0119854687619504,0.983214241188827));
#92023=DIRECTION('',(0.797465759836418,0.,0.6033642033536));
#92024=DIRECTION('',(-0.417826324587941,0.,0.908526918963512));
#92025=DIRECTION('center_axis',(0.145881046725855,0.986495110670749,-0.0744722554302954));
#92026=DIRECTION('ref_axis',(0.389166237111431,0.0119855022556315,0.921089565475698));
#92027=DIRECTION('',(0.908526921826082,0.,0.417826318363533));
#92028=DIRECTION('',(-0.212751349470685,0.,0.977106372560533));
#92029=DIRECTION('center_axis',(0.126461096607096,0.986495110752455,-0.104091246060526));
#92030=DIRECTION('ref_axis',(0.578074777275499,0.0119854994431879,0.815895765205936));
#92031=DIRECTION('',(0.977106374521695,0.,0.212751340463627));
#92032=DIRECTION('',(0.00227165745136495,0.,0.999997419782883));
#92033=DIRECTION('center_axis',(0.101127974199879,0.986495110894289,-0.128843040230716));
#92034=DIRECTION('ref_axis',(0.73995317920339,0.0119854881880012,0.672551589589744));
#92035=DIRECTION('',(0.999997419791011,0.,-0.00227165387351802));
#92036=DIRECTION('',(0.217188425318953,0.,0.976129698302164));
#92037=DIRECTION('center_axis',(0.0710662092121789,0.986495110852024,-0.147570288924515));
#92038=DIRECTION('ref_axis',(0.867232196839401,0.011985492721948,0.497759645541218));
#92039=DIRECTION('',(0.976129697249629,0.,-0.217188430049455));
#92040=DIRECTION('',(0.421949715333494,0.,0.906619235252586));
#92041=DIRECTION('center_axis',(0.037681493016981,0.986495111222342,-0.159397304301016));
#92042=DIRECTION('ref_axis',(0.953960399933603,0.0119854691604863,0.299693016080662));
#92043=DIRECTION('',(0.906619236073577,0.,-0.421949713569477));
#92044=DIRECTION('',(0.606981095233153,0.,0.794716270142724));
#92045=DIRECTION('center_axis',(0.00253481763562235,0.986495111223513,-0.163771090952169));
#92046=DIRECTION('ref_axis',(0.99608247502221,0.0119854644543318,0.0876130789063035));
#92047=DIRECTION('',(0.794716264459817,0.,-0.606981102673744));
#92048=DIRECTION('',(0.763630727833486,0.,0.64565324401609));
#92049=DIRECTION('center_axis',(-0.0327304306477485,0.986495110640403,-0.160487119708069));
#92050=DIRECTION('ref_axis',(0.991628840187903,0.0119855052037018,-0.128563567827769));
#92051=DIRECTION('',(0.645653244432689,0.,-0.763630727481249));
#92052=DIRECTION('',(0.884573824525916,0.,0.466400202576708));
#92053=DIRECTION('center_axis',(-0.0664651799120975,0.986495110908589,-0.149698951274562));
#92054=DIRECTION('ref_axis',(0.940807743855523,0.0119854863573399,-0.338728707402042));
#92055=DIRECTION('',(0.466400198110657,0.,-0.884573826880685));
#92056=DIRECTION('',(0.964155238486549,0.,0.265338794937613));
#92057=DIRECTION('center_axis',(-0.0970921104723414,0.986495110838536,-0.131911024466085));
#92058=DIRECTION('ref_axis',(0.845995521661184,0.0119854859784489,-0.53305527429628));
#92059=DIRECTION('',(0.265338798459341,0.,-0.964155237517358));
#92060=DIRECTION('',(0.998653822673426,0.,0.0518704391706294));
#92061=DIRECTION('center_axis',(-0.123179135387685,0.986495110642582,-0.107955070670268));
#92062=DIRECTION('ref_axis',(0.711625490067636,0.0119855055860069,-0.702456767026872));
#92063=DIRECTION('',(0.0518704491632369,0.,-0.998653822154406));
#92064=DIRECTION('',(0.986456463072521,0.,-0.164023310728849));
#92065=DIRECTION('center_axis',(-0.143506400745292,0.98649511126427,-0.0789513039590035));
#92066=DIRECTION('ref_axis',(0.543980643219903,0.0119854622664827,-0.839012162305362));
#92067=DIRECTION('',(-0.164023304687571,0.,-0.986456464077036));
#92068=DIRECTION('',(0.928133495813481,0.,-0.372247517048868));
#92069=DIRECTION('center_axis',(-0.15712350469364,0.986495110979502,-0.0462558135408789));
#92070=DIRECTION('ref_axis',(0.350899859893009,0.0119854818250457,-0.936336283902577));
#92071=DIRECTION('',(-0.372247514176791,0.,-0.928133496965388));
#92072=DIRECTION('',(0.82641204072096,0.,-0.563065838913549));
#92073=DIRECTION('center_axis',(-0.16339367973884,0.986495110748462,-0.0113974510651309));
#92074=DIRECTION('ref_axis',(0.141411393691066,0.0119855006749099,-0.989878358945139));
#92075=DIRECTION('',(-0.563065840773055,0.,-0.826412039454008));
#92076=DIRECTION('',(0.686048466658641,0.,-0.727555840740302));
#92077=DIRECTION('center_axis',(-0.162023741836773,0.986495110751063,0.0239938230688417));
#92078=DIRECTION('ref_axis',(-0.0746893108236778,0.0119854977166643,-0.997134822726179));
#92079=DIRECTION('',(-0.727555834238047,0.,-0.686048473554296));
#92080=DIRECTION('',(0.513606044881543,0.,-0.858026124696176));
#92081=DIRECTION('center_axis',(-0.153077758419838,0.986495110978776,0.0582631606774879));
#92082=DIRECTION('ref_axis',(-0.287297624221738,0.011985482316554,-0.957766371997986));
#92083=DIRECTION('',(-0.858026124717308,0.,-0.513606044846241));
#92084=DIRECTION('',(0.317147963692256,0.,-0.948376069460768));
#92085=DIRECTION('center_axis',(-0.136974036913601,0.986495111296262,0.0898081766888047));
#92086=DIRECTION('ref_axis',(-0.486472223026737,0.0119854633644171,-0.873613830528893));
#92087=DIRECTION('',(-0.948376067456526,0.,-0.317147969685596));
#92088=DIRECTION('',(0.105860400263,0.,-0.994381001254628));
#92089=DIRECTION('center_axis',(-0.114465547034228,0.986495111103593,0.117153891573711));
#92090=DIRECTION('ref_axis',(-0.662899926125668,0.0119854775341654,-0.748612073286867));
#92091=DIRECTION('',(-0.994381001079128,0.,-0.105860401911536));
#92092=DIRECTION('',(-0.110377074078133,0.,-0.993889783385437));
#92093=DIRECTION('center_axis',(-0.086604781679156,0.986495111014318,0.139021608878454));
#92094=DIRECTION('ref_axis',(-0.808331159221251,0.0119854794471593,-0.588606052733447));
#92095=DIRECTION('',(-0.993889782988621,0.,0.110377077651255));
#92096=DIRECTION('',(-0.321453455831505,0.,-0.946925380235414));
#92097=DIRECTION('center_axis',(-0.0546944690174662,0.986495110963998,0.154388830888208));
#92098=DIRECTION('ref_axis',(-0.91596573079673,0.0119854833439481,-0.40107745909615));
#92099=DIRECTION('',(-0.946925383812815,0.,0.321453445293331));
#92100=DIRECTION('',(-0.517499007895215,0.,-0.855683806570785));
#92101=DIRECTION('center_axis',(-0.020226705941467,0.986495110930022,0.162537000335067));
#92102=DIRECTION('ref_axis',(-0.98077075817357,0.0119854859094575,-0.194794938433099));
#92103=DIRECTION('',(-0.855683806294095,0.,0.517499008352721));
#92104=DIRECTION('',(-0.689346898711863,0.,-0.724431399951946));
#92105=DIRECTION('center_axis',(0.0151868177319126,0.986495111230557,0.163085119141475));
#92106=DIRECTION('ref_axis',(-0.999716036804243,0.0119854703633428,0.0205959767087327));
#92107=DIRECTION('',(-0.724431405665859,0.,0.689346892707139));
#92108=DIRECTION('',(-0.828961683246508,0.,-0.559305397532615));
#92109=DIRECTION('center_axis',(0.049890258038083,0.986495110880213,0.156007558670503));
#92110=DIRECTION('ref_axis',(-0.971915703710593,0.0119854899509415,0.235023856047377));
#92111=DIRECTION('',(-0.559305393777797,0.,0.828961685779906));
#92112=DIRECTION('',(-0.929815150843002,0.,-0.368026881168761));
#92113=DIRECTION('center_axis',(0.0822608615150763,0.986495110907273,0.141635259800816));
#92114=DIRECTION('ref_axis',(-0.898669673512321,0.0119854860796758,0.438462274355152));
#92115=DIRECTION('',(-0.368026888901989,0.,0.92981514778214));
#92116=DIRECTION('',(-0.987191490845447,0.,-0.159539839545941));
#92117=DIRECTION('center_axis',(0.110785037875841,0.986495110984941,0.120640256074234));
#92118=DIRECTION('ref_axis',(-0.783402848266655,0.0119854803289976,0.621398684894791));
#92119=DIRECTION('',(-0.159539852444422,0.,0.987191488760925));
#92120=DIRECTION('',(-0.998407852997013,0.,0.0564070835436024));
#92121=DIRECTION('center_axis',(0.134129057425302,0.986495110447697,0.0940042180808219));
#92122=DIRECTION('ref_axis',(-0.631504974824666,0.0119855165618774,0.775279184658303));
#92123=DIRECTION('',(0.0564070922907477,0.,0.998407852502825));
#92124=DIRECTION('',(-0.962939775847857,0.,0.269716495769317));
#92125=DIRECTION('center_axis',(0.151201316773429,0.986495110675738,0.0629726799401554));
#92126=DIRECTION('ref_axis',(-0.450078631102011,0.0119855039511957,0.892908491123461));
#92127=DIRECTION('',(0.269716499111255,0.,0.96293977491179));
#92128=DIRECTION('',(-0.882445701452064,0.,0.470414268479151));
#92129=DIRECTION('center_axis',(0.161203577483734,0.986495110702338,0.0289966061260205));
#92130=DIRECTION('ref_axis',(-0.247607114474751,0.0119854981900649,0.968786387546101));
#92131=DIRECTION('',(0.47041426492384,0.,0.88244570334733));
#92132=DIRECTION('',(-0.76068944558395,0.,0.649115989155392));
#92133=DIRECTION('center_axis',(0.163668139206856,0.986495111098837,-0.00633529688789426));
#92134=DIRECTION('ref_axis',(-0.0335577583546433,0.0119854717406174,0.999364910991659));
#92135=DIRECTION('',(0.649115980606205,0.,0.760689452879193));
#92136=DIRECTION('center_axis',(0.,1.,0.));
#92137=DIRECTION('ref_axis',(1.,0.,0.));
#92138=DIRECTION('center_axis',(0.,-1.,0.));
#92139=DIRECTION('ref_axis',(0.,0.,-1.));
#92436=CARTESIAN_POINT('',(0.,0.,0.));
#92437=CARTESIAN_POINT('Origin',(2.53163762382963E-15,0.,-3.4647252052902E-15));
#92438=CARTESIAN_POINT('',(-1.76317673760922E-10,0.574924266631643,-7.32492426663165));
#92439=CARTESIAN_POINT('',(1.9876441650041E-12,0.520900163746503,-7.27090016374651));
#92440=CARTESIAN_POINT('',(1.70500103440517E-15,0.,-6.75000000000001));
#92441=CARTESIAN_POINT('',(0.583996965696794,0.655900535579078,-7.3828389043069));
#92442=CARTESIAN_POINT('Ctrl Pts',(-3.52635867725153E-10,0.574924266631643,
-7.32492426663165));
#92443=CARTESIAN_POINT('Ctrl Pts',(0.0689301492338497,0.584602182770183,
-7.33460218277351));
#92444=CARTESIAN_POINT('Ctrl Pts',(0.138003016537344,0.594255597212115,
-7.3432826012457));
#92445=CARTESIAN_POINT('Ctrl Pts',(0.332487077960733,0.621315844934006,
-7.36487180976007));
#92446=CARTESIAN_POINT('Ctrl Pts',(0.458124127164828,0.63865680389821,-7.37549809589609));
#92447=CARTESIAN_POINT('Ctrl Pts',(0.583996965696794,0.655900535579078,
-7.3828389043069));
#92448=CARTESIAN_POINT('',(1.30876848074398,0.552026825468249,-7.18378179160119));
#92449=CARTESIAN_POINT('Ctrl Pts',(1.30876848039644,0.55202682497196,-7.18378179076529));
#92450=CARTESIAN_POINT('Ctrl Pts',(1.27769795963077,0.556534160327731,-7.19402386159478));
#92451=CARTESIAN_POINT('Ctrl Pts',(1.2491031004971,0.56067537123005,-7.20323933174539));
#92452=CARTESIAN_POINT('Ctrl Pts',(1.18971706977311,0.569263221052948,-7.22199063171888));
#92453=CARTESIAN_POINT('Ctrl Pts',(1.15980716658276,0.573581754023551,-7.23122799238887));
#92454=CARTESIAN_POINT('Ctrl Pts',(1.06974174972982,0.586565893247897,-7.25842391824879));
#92455=CARTESIAN_POINT('Ctrl Pts',(1.00941728088563,0.595235853584047,-7.27581144677397));
#92456=CARTESIAN_POINT('Ctrl Pts',(0.82802600490288,0.621229052863817,-7.325626142571));
#92457=CARTESIAN_POINT('Ctrl Pts',(0.706365167342942,0.638561214288606,
-7.35576585694803));
#92458=CARTESIAN_POINT('Ctrl Pts',(0.583996965783454,0.655900535821569,
-7.38283890454329));
#92459=CARTESIAN_POINT('',(1.03955650170316,0.499999998541226,-7.17508343307688));
#92460=CARTESIAN_POINT('Origin',(1.50272086180022,0.00294824858821298,-0.139203625378671));
#92461=CARTESIAN_POINT('',(1.35874712529518,0.544769999507073,-7.16711068668613));
#92462=CARTESIAN_POINT('Origin',(1.03656721497925,0.376341643908494,0.158100836374117));
#92463=CARTESIAN_POINT('',(1.66354985423409,0.499999999722904,-7.05656445327241));
#92464=CARTESIAN_POINT('Ctrl Pts',(1.66354985413997,0.499999999773013,-7.05656445301109));
#92465=CARTESIAN_POINT('Ctrl Pts',(1.61318185067642,0.507497225034372,-7.07614119873178));
#92466=CARTESIAN_POINT('Ctrl Pts',(1.56258951116536,0.514976130334334,-7.0951432142536));
#92467=CARTESIAN_POINT('Ctrl Pts',(1.46066238276572,0.529942096572695,-7.13210508637025));
#92468=CARTESIAN_POINT('Ctrl Pts',(1.40948218992217,0.537396680916625,-7.14998763782684));
#92469=CARTESIAN_POINT('Ctrl Pts',(1.35874712542329,0.544769999785901,-7.16711068694564));
#92470=CARTESIAN_POINT('',(1.4106405155084,0.552026825393108,-7.1644740979145));
#92471=CARTESIAN_POINT('Ctrl Pts',(1.41064051525833,0.552026824820363,-7.16447409806159));
#92472=CARTESIAN_POINT('Ctrl Pts',(1.43304694537867,0.54747794893926,-7.15542619891083));
#92473=CARTESIAN_POINT('Ctrl Pts',(1.45540955657652,0.542929077085632,-7.14626901081486));
#92474=CARTESIAN_POINT('Ctrl Pts',(1.4777268899251,0.538380664762857,-7.13700328942627));
#92475=CARTESIAN_POINT('Ctrl Pts',(1.50004426513297,0.533832243908898,-7.12773755065851));
#92476=CARTESIAN_POINT('Ctrl Pts',(1.52231439379302,0.529279732452209,-7.11835902210837));
#92477=CARTESIAN_POINT('Ctrl Pts',(1.54452808931809,0.524710849011714,-7.10885721603945));
#92478=CARTESIAN_POINT('Ctrl Pts',(1.58437756039739,0.516514662640066,-7.09181178810887));
#92479=CARTESIAN_POINT('Ctrl Pts',(1.62405513566634,0.508277071672323,-7.07437909996789));
#92480=CARTESIAN_POINT('Ctrl Pts',(1.66354985423409,0.499999999722904,-7.05656445327241));
#92481=CARTESIAN_POINT('',(2.15743557081923,0.655900535694669,-7.08469014864916));
#92482=CARTESIAN_POINT('Ctrl Pts',(2.15743557081923,0.655900535694667,-7.08469014864917));
#92483=CARTESIAN_POINT('Ctrl Pts',(2.03373840194332,0.638769108056856,-7.10445036682175));
#92484=CARTESIAN_POINT('Ctrl Pts',(1.90957099987732,0.621541657207324,-7.12099361629952));
#92485=CARTESIAN_POINT('Ctrl Pts',(1.66051231613118,0.586905785277197,-7.14760586946283));
#92486=CARTESIAN_POINT('Ctrl Pts',(1.53566986647824,0.569504150491215,-7.15766947092575));
#92487=CARTESIAN_POINT('Ctrl Pts',(1.41064051535414,0.552026827020548,-7.16447409926013));
#92488=CARTESIAN_POINT('',(2.82247093371176,0.552026825486419,-6.73448243022672));
#92489=CARTESIAN_POINT('Ctrl Pts',(2.82247093304854,0.552026825253083,-6.73448242917092));
#92490=CARTESIAN_POINT('Ctrl Pts',(2.79433186951501,0.556533631550359,-6.75116233153416));
#92491=CARTESIAN_POINT('Ctrl Pts',(2.76838058449236,0.560675802469198,-6.7663129162634));
#92492=CARTESIAN_POINT('Ctrl Pts',(2.71441665085727,0.569263221115838,-6.79739050203923));
#92493=CARTESIAN_POINT('Ctrl Pts',(2.68719178408473,0.573581754079392,-6.8128416433915));
#92494=CARTESIAN_POINT('Ctrl Pts',(2.60507836686489,0.586565893274957,-6.85876314585948));
#92495=CARTESIAN_POINT('Ctrl Pts',(2.54990205531152,0.595235853588861,-6.88871214120141));
#92496=CARTESIAN_POINT('Ctrl Pts',(2.38346029380532,0.621229052810113,-6.9763559594211));
#92497=CARTESIAN_POINT('Ctrl Pts',(2.27112296677513,0.638561214198741,-7.03194450776666));
#92498=CARTESIAN_POINT('Ctrl Pts',(2.1574355708213,0.655900535698362,-7.0846901486524));
#92499=CARTESIAN_POINT('',(2.55768309344323,0.499999998717349,-6.78386005050966));
#92500=CARTESIAN_POINT('Origin',(1.49751296178958,0.0029484005309216,0.187090266587314));
#92501=CARTESIAN_POINT('',(2.86769731163377,0.544769999483455,-6.70745715410932));
#92502=CARTESIAN_POINT('Origin',(0.978346013513691,0.376341857620247,0.377235070553447));
#92503=CARTESIAN_POINT('',(3.14160975116893,0.499999999552296,-6.53397185227299));
#92504=CARTESIAN_POINT('Ctrl Pts',(3.14160975112423,0.499999999567421,-6.53397185220206));
#92505=CARTESIAN_POINT('Ctrl Pts',(3.09662781122098,0.507497213775332,-6.56391849238582));
#92506=CARTESIAN_POINT('Ctrl Pts',(3.05130323285072,0.514976107913629,-6.5933520693833));
#92507=CARTESIAN_POINT('Ctrl Pts',(2.95970745311632,0.529941643027644,-6.65135944187097));
#92508=CARTESIAN_POINT('Ctrl Pts',(2.91356238951158,0.537397143986615,-6.67982962830261));
#92509=CARTESIAN_POINT('Ctrl Pts',(2.86769731188293,0.544769999867499,-6.70745715442048));
#92510=CARTESIAN_POINT('',(2.91781067495167,0.552026825837718,-6.69372666237931));
#92511=CARTESIAN_POINT('Ctrl Pts',(2.91781067507541,0.552026824628134,-6.69372666219399));
#92512=CARTESIAN_POINT('Ctrl Pts',(2.93774822535267,0.547477948549068,-6.68007357702528));
#92513=CARTESIAN_POINT('Ctrl Pts',(2.9576194865856,0.542929076717278,-6.66632317844806));
#92514=CARTESIAN_POINT('Ctrl Pts',(2.97742319707285,0.538380664394361,-6.65247651740689));
#92515=CARTESIAN_POINT('Ctrl Pts',(2.99722694470494,0.533832243540209,-6.63862983039422));
#92516=CARTESIAN_POINT('Ctrl Pts',(3.016960303858,0.529279732005685,-6.62468314711241));
#92517=CARTESIAN_POINT('Ctrl Pts',(3.03661204825892,0.524710848528471,-6.61062819995699));
#92518=CARTESIAN_POINT('Ctrl Pts',(3.07186559686841,0.516514662354408,-6.58541482690274));
#92519=CARTESIAN_POINT('Ctrl Pts',(3.10686801904124,0.508277071627687,-6.55986020013196));
#92520=CARTESIAN_POINT('Ctrl Pts',(3.14160975116893,0.499999999552296,-6.53397185227299));
#92521=CARTESIAN_POINT('',(3.62999488593847,0.655900535633648,-6.45526915564017));
#92522=CARTESIAN_POINT('Ctrl Pts',(3.62999488593847,0.655900535633648,-6.45526915564018));
#92523=CARTESIAN_POINT('Ctrl Pts',(3.51343755102735,0.638769108032714,-6.50115862572389));
#92524=CARTESIAN_POINT('Ctrl Pts',(3.39572942354314,0.621541657210048,-6.54400742428145));
#92525=CARTESIAN_POINT('Ctrl Pts',(3.15821444122951,0.586905785296612,-6.62353775264504));
#92526=CARTESIAN_POINT('Ctrl Pts',(3.03845411560859,0.569504150524582,-6.66020350902869));
#92527=CARTESIAN_POINT('Ctrl Pts',(2.91781067511717,0.552026827043759,-6.6937266636037));
#92528=CARTESIAN_POINT('',(4.20419778449755,0.552026825475761,-5.97028615389083));
#92529=CARTESIAN_POINT('Ctrl Pts',(4.20419778376074,0.552026825178374,-5.97028615316268));
#92530=CARTESIAN_POINT('Ctrl Pts',(4.18030228195419,0.556533631466163,-5.99262515546922));
#92531=CARTESIAN_POINT('Ctrl Pts',(4.15821465144795,0.560675802389299,-6.01300028710299));
#92532=CARTESIAN_POINT('Ctrl Pts',(4.11219312688654,0.569263221052653,-6.05495194678946));
#92533=CARTESIAN_POINT('Ctrl Pts',(4.08892630099689,0.57358175402933,-6.07589439067761));
#92534=CARTESIAN_POINT('Ctrl Pts',(4.01860441540169,0.586565893251218,-6.13839423144815));
#92535=CARTESIAN_POINT('Ctrl Pts',(3.97115624405401,0.595235853575711,-6.17950431192812));
#92536=CARTESIAN_POINT('Ctrl Pts',(3.82744662849934,0.621229052835717,-6.30087912525721));
#92537=CARTESIAN_POINT('Ctrl Pts',(3.72968558033533,0.638561214242502,-6.37931724897332));
#92538=CARTESIAN_POINT('Ctrl Pts',(3.62999488602545,0.655900535752202,-6.45526915572728));
#92539=CARTESIAN_POINT('',(3.95621526506587,0.499999998663635,-6.07543091191077));
#92540=CARTESIAN_POINT('Origin',(1.42228368115469,0.00294854809307285,0.50463567534438));
#92541=CARTESIAN_POINT('',(4.24255715901931,0.544769999394389,-5.93417037980192));
#92542=CARTESIAN_POINT('Origin',(0.874379082447689,0.376342413060157,0.578729547218476));
#92543=CARTESIAN_POINT('',(4.47277146634557,0.499999999622954,-5.70585799046131));
#92544=CARTESIAN_POINT('Ctrl Pts',(4.472771466155,0.499999999667942,-5.70585799041082));
#92545=CARTESIAN_POINT('Ctrl Pts',(4.43527881819098,0.507497214479082,-5.74477428551586));
#92546=CARTESIAN_POINT('Ctrl Pts',(4.39734124892664,0.514976109242423,-5.78326316956504));
#92547=CARTESIAN_POINT('Ctrl Pts',(4.32035680324058,0.529941643282175,-5.85960474175593));
#92548=CARTESIAN_POINT('Ctrl Pts',(4.28141083079792,0.53739714477637,-5.89732913864258));
#92549=CARTESIAN_POINT('Ctrl Pts',(4.24255715940239,0.544769999868629,-5.93417038011102));
#92550=CARTESIAN_POINT('',(4.28854724969871,0.552026825667153,-5.90998800741621));
#92551=CARTESIAN_POINT('Ctrl Pts',(4.28854724980574,0.552026824741665,-5.9099880073423));
#92552=CARTESIAN_POINT('Ctrl Pts',(4.3050836615186,0.547477948841813,-5.89236814036842));
#92553=CARTESIAN_POINT('Ctrl Pts',(4.32153441435246,0.542929076963385,-5.87466748472589));
#92554=CARTESIAN_POINT('Ctrl Pts',(4.33789850212508,0.53838066456022,-5.85688733857809));
#92555=CARTESIAN_POINT('Ctrl Pts',(4.35426262059039,0.533832243625994,-5.83910715908161));
#92556=CARTESIAN_POINT('Ctrl Pts',(4.37053650011405,0.529279732161267,-5.82124445270268));
#92557=CARTESIAN_POINT('Ctrl Pts',(4.3867073994258,0.524710848714242,-5.80329355833596));
#92558=CARTESIAN_POINT('Ctrl Pts',(4.41571660990344,0.516514662527723,-5.77109118894962));
#92559=CARTESIAN_POINT('Ctrl Pts',(4.44440720567689,0.508277071788115,-5.73860952892666));
#92560=CARTESIAN_POINT('Ctrl Pts',(4.47277146634557,0.499999999622954,-5.70585799046131));
#92561=CARTESIAN_POINT('',(4.93281967474729,0.655900535551958,-5.52400695138184));
#92562=CARTESIAN_POINT('Ctrl Pts',(4.93281967474729,0.655900535551957,-5.52400695138184));
#92563=CARTESIAN_POINT('Ctrl Pts',(4.82885226510583,0.638769107953755,-5.5938799327855));
#92564=CARTESIAN_POINT('Ctrl Pts',(4.72310731328421,0.621541657142716,-5.66103071826921));
#92565=CARTESIAN_POINT('Ctrl Pts',(4.50824196910535,0.586905785269717,-5.78976037198936));
#92566=CARTESIAN_POINT('Ctrl Pts',(4.39916362665628,0.569504150421789,-5.85131383354925));
#92567=CARTESIAN_POINT('Ctrl Pts',(4.28854725022243,0.55202682693946,-5.90998800878253));
#92568=CARTESIAN_POINT('',(5.38934101926066,0.552026825436104,-4.9269259328291));
#92569=CARTESIAN_POINT('Ctrl Pts',(5.38934101841487,0.552026825142794,-4.92692593229653));
#92570=CARTESIAN_POINT('Ctrl Pts',(5.37080640526157,0.556533631450834,-4.95387948778111));
#92571=CARTESIAN_POINT('Ctrl Pts',(5.35361522227531,0.560675802385154,-4.97852644785407));
#92572=CARTESIAN_POINT('Ctrl Pts',(5.31768802211116,0.569263221065196,-5.02939056849044));
#92573=CARTESIAN_POINT('Ctrl Pts',(5.29946716807536,0.573581754044685,-5.05484506947216));
#92574=CARTESIAN_POINT('Ctrl Pts',(5.24422498739726,0.586565893277644,-5.13100082538544));
#92575=CARTESIAN_POINT('Ctrl Pts',(5.20672358004069,0.595235853610458,-5.18134972930647));
#92576=CARTESIAN_POINT('Ctrl Pts',(5.09246581254656,0.621229052890819,-5.33078018623515));
#92577=CARTESIAN_POINT('Ctrl Pts',(5.01385224139044,0.638561214308336,-5.42840020573969));
#92578=CARTESIAN_POINT('Ctrl Pts',(4.93281967498493,0.655900535823712,-5.52400695153397));
#92579=CARTESIAN_POINT('',(5.16975920818102,0.499999998549721,-5.08292137660211));
#92580=CARTESIAN_POINT('Origin',(1.28054877109914,0.00294807119520506,0.798587994577735));
#92581=CARTESIAN_POINT('',(5.41903974963537,0.544769999481502,-4.8834083934489));
#92582=CARTESIAN_POINT('Origin',(0.729525470119463,0.376341730165788,0.753166654253201));
#92583=CARTESIAN_POINT('',(5.5947913592018,0.499999999550736,-4.61094454995047));
#92584=CARTESIAN_POINT('Ctrl Pts',(5.59479135904148,0.499999999587741,-4.61094454996122));
#92585=CARTESIAN_POINT('Ctrl Pts',(5.56654112187797,0.507497214329946,-4.65701081411809));
#92586=CARTESIAN_POINT('Ctrl Pts',(5.53776448467522,0.514976108986996,-4.7027553047835));
#92587=CARTESIAN_POINT('Ctrl Pts',(5.47899107359703,0.529941643074257,-4.79386143408856));
#92588=CARTESIAN_POINT('Ctrl Pts',(5.4490652670489,0.537397144438014,-4.83907608766772));
#92589=CARTESIAN_POINT('Ctrl Pts',(5.41903974987221,0.544769999736433,-4.88340839356691));
#92590=CARTESIAN_POINT('',(5.45875612184271,0.552026825349422,-4.84990488204123));
#92591=CARTESIAN_POINT('Ctrl Pts',(5.45875612172105,0.552026824787737,-4.84990488225974));
#92592=CARTESIAN_POINT('Ctrl Pts',(5.47111817039548,0.547477948904059,-4.82914211851112));
#92593=CARTESIAN_POINT('Ctrl Pts',(5.48337919604398,0.542929077052408,-4.80831886881669));
#92594=CARTESIAN_POINT('Ctrl Pts',(5.49553849473922,0.538380664711329,-4.78743661749974));
#92595=CARTESIAN_POINT('Ctrl Pts',(5.50769781624091,0.533832243839075,-4.76655432701525));
#92596=CARTESIAN_POINT('Ctrl Pts',(5.51975126758095,0.529279732320647,-4.74561083774347));
#92597=CARTESIAN_POINT('Ctrl Pts',(5.53168518856306,0.52471084886393,-4.72460335998809));
#92598=CARTESIAN_POINT('Ctrl Pts',(5.55309362269106,0.516514662491629,-4.68691774061822));
#92599=CARTESIAN_POINT('Ctrl Pts',(5.57413085193685,0.508277071597412,-4.64902785301941));
#92600=CARTESIAN_POINT('Ctrl Pts',(5.5947913592018,0.499999999550736,-4.61094454995047));
#92601=CARTESIAN_POINT('',(6.00499129856053,0.655900535637417,-4.33444832106312));
#92602=CARTESIAN_POINT('Ctrl Pts',(6.00499129856054,0.655900535637417,-4.33444832106312));
#92603=CARTESIAN_POINT('Ctrl Pts',(5.91847521462983,0.638769108018161,-4.42503763096437));
#92604=CARTESIAN_POINT('Ctrl Pts',(5.82963795480512,0.621541657186257,-4.51335050739163));
#92605=CARTESIAN_POINT('Ctrl Pts',(5.64746911313381,0.586905785286544,-4.68526023114174));
#92606=CARTESIAN_POINT('Ctrl Pts',(5.55417313630222,0.569504150412454,-4.76882322639795));
#92607=CARTESIAN_POINT('Ctrl Pts',(5.45875612252139,0.552026826918684,-4.84990488317817));
#92608=CARTESIAN_POINT('',(6.32248465789244,0.552026825409836,-3.65318813103928));
#92609=CARTESIAN_POINT('Ctrl Pts',(6.32248465691362,0.552026825139949,-3.65318813068195));
#92610=CARTESIAN_POINT('Ctrl Pts',(6.31017759038344,0.556533631445669,-3.68349592099771));
#92611=CARTESIAN_POINT('Ctrl Pts',(6.29868669552113,0.560675802386554,-3.71126224509254));
#92612=CARTESIAN_POINT('Ctrl Pts',(6.27453373572314,0.569263221059156,-3.76866047689442));
#92613=CARTESIAN_POINT('Ctrl Pts',(6.26221084042521,0.573581754029174,-3.7974368107589));
#92614=CARTESIAN_POINT('Ctrl Pts',(6.22463142764196,0.586565893240533,-3.88368752321914));
#92615=CARTESIAN_POINT('Ctrl Pts',(6.19883030841442,0.595235853563861,-3.94092099173871));
#92616=CARTESIAN_POINT('Ctrl Pts',(6.11936695523834,0.621229052814039,-4.11141988999875));
#92617=CARTESIAN_POINT('Ctrl Pts',(6.06357674434361,0.638561214214636,-4.22365720154951));
#92618=CARTESIAN_POINT('Ctrl Pts',(6.00499129862453,0.655900535703095,-4.33444832108668));
#92619=CARTESIAN_POINT('',(6.14157095730116,0.499999998704437,-3.85274008577389));
#92620=CARTESIAN_POINT('Origin',(1.07893795822326,0.00294795557416398,1.05519716394546));
#92621=CARTESIAN_POINT('',(6.34213406351935,0.544769999517614,-3.60430365899014));
#92622=CARTESIAN_POINT('Origin',(0.550561489189073,0.376341714602447,0.892384071056311));
#92623=CARTESIAN_POINT('',(6.45520502561422,0.499999999749251,-3.30042846896563));
#92624=CARTESIAN_POINT('Ctrl Pts',(6.45520502526096,0.499999999833995,-3.30042846906863));
#92625=CARTESIAN_POINT('Ctrl Pts',(6.43751814586516,0.507497215429968,-3.35149070156539));
#92626=CARTESIAN_POINT('Ctrl Pts',(6.41924800134489,0.514976110955304,-3.40235184376848));
#92627=CARTESIAN_POINT('Ctrl Pts',(6.38143380907499,0.529941643395797,-3.50396249680085));
#92628=CARTESIAN_POINT('Ctrl Pts',(6.36192746817965,0.537397143637598,-3.55455321319428));
#92629=CARTESIAN_POINT('Ctrl Pts',(6.34213406386358,0.54476999985951,-3.60430365907642));
#92630=CARTESIAN_POINT('',(6.37371962476082,0.55202682565524,-3.56304559389542));
#92631=CARTESIAN_POINT('Ctrl Pts',(6.37371962481441,0.552026824684896,-3.56304559376603));
#92632=CARTESIAN_POINT('Ctrl Pts',(6.38132927556718,0.547477948641283,-3.54011077625578));
#92633=CARTESIAN_POINT('Ctrl Pts',(6.38882726203103,0.54292907673752,-3.51713860448545));
#92634=CARTESIAN_POINT('Ctrl Pts',(6.39621321628672,0.53838066437267,-3.4941306788099));
#92635=CARTESIAN_POINT('Ctrl Pts',(6.40359918439574,0.533832243476672,-3.47112270997995));
#92636=CARTESIAN_POINT('Ctrl Pts',(6.41086860168613,0.529279732017064,-3.44807773212331));
#92637=CARTESIAN_POINT('Ctrl Pts',(6.4180075274815,0.524710848564556,-3.42499595728427));
#92638=CARTESIAN_POINT('Ctrl Pts',(6.43081414986407,0.516514662364648,-3.38358922709044));
#92639=CARTESIAN_POINT('Ctrl Pts',(6.44321433424654,0.508277071581048,-3.3420628024185));
#92640=CARTESIAN_POINT('Ctrl Pts',(6.45520502561422,0.499999999749251,-3.30042846896563));
#92641=CARTESIAN_POINT('',(6.79637620244565,0.655900535687991,-2.94221570577926));
#92642=CARTESIAN_POINT('Ctrl Pts',(6.79637620244565,0.655900535687989,-2.94221570577926));
#92643=CARTESIAN_POINT('Ctrl Pts',(6.73135684041582,0.638769108082005,-3.04928548835663));
#92644=CARTESIAN_POINT('Ctrl Pts',(6.66358120439581,0.621541657260411,-3.1546310434227));
#92645=CARTESIAN_POINT('Ctrl Pts',(6.52262687807457,0.586905785341988,-3.36168252926548));
#92646=CARTESIAN_POINT('Ctrl Pts',(6.44947568356735,0.569504150535565,-3.46334774481967));
#92647=CARTESIAN_POINT('Ctrl Pts',(6.37371962594718,0.552026827017802,-3.56304559503574));
#92648=CARTESIAN_POINT('',(6.95999594072217,0.552026825409201,-2.20863131313051));
#92649=CARTESIAN_POINT('Ctrl Pts',(6.95999593957526,0.552026825171655,-2.20863131296794));
#92650=CARTESIAN_POINT('Ctrl Pts',(6.95449188441449,0.556533631512047,-2.24087617970752));
#92651=CARTESIAN_POINT('Ctrl Pts',(6.94923857920949,0.560675802451137,-2.27046354526051));
#92652=CARTESIAN_POINT('Ctrl Pts',(6.93798922534277,0.56926322113458,-2.33171201072628));
#92653=CARTESIAN_POINT('Ctrl Pts',(6.93214049364807,0.573581754106621,-2.36246462811705));
#92654=CARTESIAN_POINT('Ctrl Pts',(6.91398102027849,0.586565893322721,-2.45477730974309));
#92655=CARTESIAN_POINT('Ctrl Pts',(6.90108662080075,0.595235853647109,-2.51621916952215));
#92656=CARTESIAN_POINT('Ctrl Pts',(6.86013329986852,0.621229052897615,-2.69981417027227));
#92657=CARTESIAN_POINT('Ctrl Pts',(6.82977513736429,0.638561214294452,-2.82142068202551));
#92658=CARTESIAN_POINT('Ctrl Pts',(6.79637620254562,0.655900535785162,-2.94221570579295));
#92659=CARTESIAN_POINT('',(6.82620967333585,0.499999998625506,-2.44240895193039));
#92660=CARTESIAN_POINT('Origin',(0.826874931113843,0.0029480911267165,1.26246803930745));
#92661=CARTESIAN_POINT('',(6.96867723761365,0.544769999414902,-2.15666569090553));
#92662=CARTESIAN_POINT('Origin',(0.34585306664821,0.37634159742266,0.989875282359732));
#92663=CARTESIAN_POINT('',(7.01378048014667,0.499999999730478,-1.83558801947582));
#92664=CARTESIAN_POINT('Ctrl Pts',(7.01378047986532,0.499999999781752,-1.83558801943565));
#92665=CARTESIAN_POINT('Ctrl Pts',(7.0074839724311,0.507497224995949,-1.88925867030701));
#92666=CARTESIAN_POINT('Ctrl Pts',(7.00057460313458,0.514976130331124,-1.94285831627193));
#92667=CARTESIAN_POINT('Ctrl Pts',(6.98548733490655,0.529942096784993,-2.0502254160513));
#92668=CARTESIAN_POINT('Ctrl Pts',(6.97731355020339,0.537396681043757,-2.10382007041908));
#92669=CARTESIAN_POINT('Ctrl Pts',(6.96867723809537,0.544769999879199,-2.15666569091947));
#92670=CARTESIAN_POINT('',(6.99065508180253,0.552026825728037,-2.10958225482661));
#92671=CARTESIAN_POINT('Ctrl Pts',(6.99065508186297,0.552026824743019,-2.10958225470308));
#92672=CARTESIAN_POINT('Ctrl Pts',(6.99315651518471,0.54747794885825,-2.08554779102925));
#92673=CARTESIAN_POINT('Ctrl Pts',(6.99554086502014,0.542929076980459,-2.06150085049816));
#92674=CARTESIAN_POINT('Ctrl Pts',(6.99780811579523,0.538380664575027,-2.03744307558802));
#92675=CARTESIAN_POINT('Ctrl Pts',(7.00007537082278,0.533832243638573,-2.01338525555501));
#92676=CARTESIAN_POINT('Ctrl Pts',(7.00222084418056,0.529279732233542,-1.98931634671837));
#92677=CARTESIAN_POINT('Ctrl Pts',(7.00423096656736,0.524710848805729,-1.9652395530089));
#92678=CARTESIAN_POINT('Ctrl Pts',(7.00783695425831,0.516514662588317,-1.92204784372608));
#92679=CARTESIAN_POINT('Ctrl Pts',(7.01102027544683,0.508277071769268,-1.8788266105124));
#92680=CARTESIAN_POINT('Ctrl Pts',(7.01378048014667,0.499999999730478,-1.83558801947582));
#92681=CARTESIAN_POINT('',(7.26997010890117,0.655900535569512,-1.41240835399411));
#92682=CARTESIAN_POINT('Ctrl Pts',(7.26997010890117,0.655900535569511,-1.41240835399411));
#92683=CARTESIAN_POINT('Ctrl Pts',(7.22948770171035,0.638769107957234,-1.53095214539221));
#92684=CARTESIAN_POINT('Ctrl Pts',(7.18594280275067,0.621541657141611,-1.64840453819461));
#92685=CARTESIAN_POINT('Ctrl Pts',(7.09279385932106,0.586905785257705,-1.88091628896775));
#92686=CARTESIAN_POINT('Ctrl Pts',(7.04320791534452,0.56950415051741,-1.99592997258257));
#92687=CARTESIAN_POINT('Ctrl Pts',(6.99065508302971,0.55202682705447,-2.10958225559804));
#92688=CARTESIAN_POINT('',(7.27206554910829,0.552026825471009,-0.660801348883197));
#92689=CARTESIAN_POINT('Ctrl Pts',(7.27206554792705,0.552026825214658,-0.660801348974819));
#92690=CARTESIAN_POINT('Ctrl Pts',(7.27362186768549,0.556533631496471,-0.693475557498244));
#92691=CARTESIAN_POINT('Ctrl Pts',(7.27485179082325,0.560675802417086,-0.723500492177397));
#92692=CARTESIAN_POINT('Ctrl Pts',(7.27703205016235,0.569263221067812,-0.785735281041659));
#92693=CARTESIAN_POINT('Ctrl Pts',(7.27793096225669,0.573581754037214,-0.817026223809206));
#92694=CARTESIAN_POINT('Ctrl Pts',(7.28004054507349,0.586565893251948,-0.911084436407912));
#92695=CARTESIAN_POINT('Ctrl Pts',(7.28065579312523,0.595235853581284,-0.973861734512161));
#92696=CARTESIAN_POINT('Ctrl Pts',(7.28012743618024,0.621229052846323,-1.16196813994222));
#92697=CARTESIAN_POINT('Ctrl Pts',(7.27662083598705,0.638561214260605,-1.28725766680698));
#92698=CARTESIAN_POINT('Ctrl Pts',(7.26997010909109,0.655900535753017,-1.41240835397878));
#92699=CARTESIAN_POINT('',(7.19166241188204,0.499999998583707,-0.917873489931604));
#92700=CARTESIAN_POINT('Origin',(0.536150814127319,0.00294833248163803,
1.41070552616189));
#92701=CARTESIAN_POINT('',(7.2693728092005,0.544769999340984,-0.608184432669663));
#92702=CARTESIAN_POINT('Origin',(0.124973750232958,0.376341620246457,1.04108062069729));
#92703=CARTESIAN_POINT('',(7.24439935455547,0.499999999619592,-0.284917513379212));
#92704=CARTESIAN_POINT('Ctrl Pts',(7.24439935438015,0.499999999673154,-0.284917513532033));
#92705=CARTESIAN_POINT('Ctrl Pts',(7.24978765199808,0.507497214783673,-0.338686864437686));
#92706=CARTESIAN_POINT('Ctrl Pts',(7.25456215704695,0.514976109782808,-0.39251861742014));
#92707=CARTESIAN_POINT('Ctrl Pts',(7.2629083902048,0.529942106270729,-0.500619067978217));
#92708=CARTESIAN_POINT('Ctrl Pts',(7.26644697143727,0.537396701243088,-0.554717907480788));
#92709=CARTESIAN_POINT('Ctrl Pts',(7.26937280977078,0.544769999900244,-0.60818443256133));
#92710=CARTESIAN_POINT('',(7.28071527694886,0.552026825363792,-0.557477194078559));
#92711=CARTESIAN_POINT('Ctrl Pts',(7.28071527697879,0.552026824732173,-0.557477194257984));
#92712=CARTESIAN_POINT('Ctrl Pts',(7.2779915286716,0.547477948852738,-0.533466909036562));
#92713=CARTESIAN_POINT('Ctrl Pts',(7.27515075242188,0.542929077057373,-0.509469607951223));
#92714=CARTESIAN_POINT('Ctrl Pts',(7.27219328578453,0.538380664766051,-0.485486898614203));
#92715=CARTESIAN_POINT('Ctrl Pts',(7.26923581360006,0.533832243943573,-0.461504144294403));
#92716=CARTESIAN_POINT('Ctrl Pts',(7.26615702303958,0.529279732525729,-0.437536739919708));
#92717=CARTESIAN_POINT('Ctrl Pts',(7.26294435094913,0.524710849108655,-0.413590731466844));
#92718=CARTESIAN_POINT('Ctrl Pts',(7.25718109175257,0.516514662684973,-0.37063363856986));
#92719=CARTESIAN_POINT('Ctrl Pts',(7.25099870095614,0.508277071644545,-0.327738572807507));
#92720=CARTESIAN_POINT('Ctrl Pts',(7.24439935455547,0.499999999619592,-0.284917513379212));
#92721=CARTESIAN_POINT('',(7.40362829346862,0.655900535690581,0.183441643835477));
#92722=CARTESIAN_POINT('Ctrl Pts',(7.40362829346862,0.655900535690581,0.183441643835477));
#92723=CARTESIAN_POINT('Ctrl Pts',(7.38957575348522,0.638769108062214,0.0589668192730024));
#92724=CARTESIAN_POINT('Ctrl Pts',(7.37229770263256,0.621541657222824,-0.0651004681833282));
#92725=CARTESIAN_POINT('Ctrl Pts',(7.33130968310938,0.586905785298123,-0.312200493074654));
#92726=CARTESIAN_POINT('Ctrl Pts',(7.30760757306436,0.569504150497685,-0.435184733230779));
#92727=CARTESIAN_POINT('Ctrl Pts',(7.28071527804253,0.552026827009743,-0.55747719455429));
#92728=CARTESIAN_POINT('',(7.24410145461844,0.552026825475149,0.917926951901574));
#92729=CARTESIAN_POINT('Ctrl Pts',(7.24410145346206,0.55202682523426,0.917926951554292));
#92730=CARTESIAN_POINT('Ctrl Pts',(7.25264537636084,0.556533631539689,0.886351210476089));
#92731=CARTESIAN_POINT('Ctrl Pts',(7.26030101799742,0.560675802457701,0.857292639234557));
#92732=CARTESIAN_POINT('Ctrl Pts',(7.27580894404161,0.569263221108155,0.796981556471936));
#92733=CARTESIAN_POINT('Ctrl Pts',(7.28341346780423,0.573581754072734,0.766615418115779));
#92734=CARTESIAN_POINT('Ctrl Pts',(7.30569346508482,0.586565893267273,0.675209732313252));
#92735=CARTESIAN_POINT('Ctrl Pts',(7.31978959236433,0.59523585357835,0.61403239277492));
#92736=CARTESIAN_POINT('Ctrl Pts',(7.35971090483336,0.621229052790785,0.430210229646323));
#92737=CARTESIAN_POINT('Ctrl Pts',(7.38321983171316,0.638561214167953,0.307096087032365));
#92738=CARTESIAN_POINT('Ctrl Pts',(7.40362829342209,0.655900535643713,0.183441643821226));
#92739=CARTESIAN_POINT('',(7.2208410099847,0.499999998929002,0.649580717715866));
#92740=CARTESIAN_POINT('Origin',(0.22035445450171,0.00294810763189539,1.4929807488716));
#92741=CARTESIAN_POINT('',(7.23016058784143,0.544769999493435,0.968734855124911));
#92742=CARTESIAN_POINT('Origin',(-0.101750885626912,0.376341834536014,1.04360639317965));
#92743=CARTESIAN_POINT('',(7.13627816756703,0.499999999904053,1.27907541649017));
#92744=CARTESIAN_POINT('Ctrl Pts',(7.13627816725196,0.500000000026025,1.27907541606446));
#92745=CARTESIAN_POINT('Ctrl Pts',(7.15309931318004,0.507497216258348,1.22772147873973));
#92746=CARTESIAN_POINT('Ctrl Pts',(7.16933443097523,0.51497611249203,1.17617465097858));
#92747=CARTESIAN_POINT('Ctrl Pts',(7.20072392982272,0.529942106403902,1.07239574048342));
#92748=CARTESIAN_POINT('Ctrl Pts',(7.21580943246971,0.53739670147069,1.02032239166843));
#92749=CARTESIAN_POINT('Ctrl Pts',(7.23016058818354,0.544769999851955,0.968734855271326));
#92750=CARTESIAN_POINT('',(7.2303373171918,0.552026825426371,1.02069488145051));
#92751=CARTESIAN_POINT('Ctrl Pts',(7.23033731739115,0.552026824912483,1.02069488110041));
#92752=CARTESIAN_POINT('Ctrl Pts',(7.2225157476636,0.547477949056865,1.04355829362695));
#92753=CARTESIAN_POINT('Ctrl Pts',(7.2145826766603,0.542929077162653,1.06638386853634));
#92754=CARTESIAN_POINT('Ctrl Pts',(7.20653878020542,0.538380664759786,1.08917010785261));
#92755=CARTESIAN_POINT('Ctrl Pts',(7.19849486866308,0.533832243825735,1.11195638990767));
#92756=CARTESIAN_POINT('Ctrl Pts',(7.19033577487136,0.529279732284339,1.13470160101827));
#92757=CARTESIAN_POINT('Ctrl Pts',(7.18205052914418,0.524710848777189,1.15739713587703));
#92758=CARTESIAN_POINT('Ctrl Pts',(7.16718750679986,0.516514662461003,1.19811098466673));
#92759=CARTESIAN_POINT('Ctrl Pts',(7.15192848598662,0.508277071585678,1.23867415561305));
#92760=CARTESIAN_POINT('Ctrl Pts',(7.13627816756703,0.499999999904053,1.27907541649017));
#92761=CARTESIAN_POINT('',(7.19110104737666,0.655900535702375,1.77071411332688));
#92762=CARTESIAN_POINT('Ctrl Pts',(7.19110104737667,0.655900535702375,1.77071411332688));
#92763=CARTESIAN_POINT('Ctrl Pts',(7.20413545578322,0.638769108080208,1.64612856036365));
#92764=CARTESIAN_POINT('Ctrl Pts',(7.2139321555394,0.621541657239082,1.52124762701307));
#92765=CARTESIAN_POINT('Ctrl Pts',(7.22702161423002,0.586905785309721,1.27111345093031));
#92766=CARTESIAN_POINT('Ctrl Pts',(7.23031162257484,0.569504150532731,1.14590926119869));
#92767=CARTESIAN_POINT('Ctrl Pts',(7.2303373187043,0.552026827039748,1.02069488122563));
#92768=CARTESIAN_POINT('',(6.87741122726476,0.552026825413561,2.45373400825514));
#92769=CARTESIAN_POINT('Ctrl Pts',(6.8774112262582,0.552026825174671,2.45373400769281));
#92770=CARTESIAN_POINT('Ctrl Pts',(6.89254324801281,0.5565336315074,2.42473318065509));
#92771=CARTESIAN_POINT('Ctrl Pts',(6.90626663890515,0.560675802448533,2.39799971923227));
#92772=CARTESIAN_POINT('Ctrl Pts',(6.93437709832155,0.569263221131459,2.34243242168606));
#92773=CARTESIAN_POINT('Ctrl Pts',(6.94833165467528,0.573581754104273,2.31441097460743));
#92774=CARTESIAN_POINT('Ctrl Pts',(6.98974027851822,0.586565893323153,2.22993184381712));
#92775=CARTESIAN_POINT('Ctrl Pts',(7.01665816578896,0.595235853649897,2.17321504719998));
#92776=CARTESIAN_POINT('Ctrl Pts',(7.09516247148734,0.621229052902576,2.00227244630821));
#92777=CARTESIAN_POINT('Ctrl Pts',(7.14458767415175,0.638561214298158,1.88709036835596));
#92778=CARTESIAN_POINT('Ctrl Pts',(7.19110104743979,0.65590053577218,1.77071411336251));
#92779=CARTESIAN_POINT('',(6.91238110673581,0.499999998645691,2.18666125139118));
#92780=CARTESIAN_POINT('Origin',(-0.105743174771213,0.00294783977492552,
1.5054455554018));
#92781=CARTESIAN_POINT('',(6.85287409290266,0.544769999392285,2.50035717665643));
#92782=CARTESIAN_POINT('Origin',(-0.323715934329361,0.376341767018527,0.997334149364529));
#92783=CARTESIAN_POINT('',(6.69447254313508,0.499999999636659,2.78326020476335));
#92784=CARTESIAN_POINT('Ctrl Pts',(6.69447254303287,0.499999999694329,2.78326020453475));
#92785=CARTESIAN_POINT('Ctrl Pts',(6.72193999413843,0.507497214796774,2.73672295029177));
#92786=CARTESIAN_POINT('Ctrl Pts',(6.74887658417363,0.514976109836711,2.68987133664889));
#92787=CARTESIAN_POINT('Ctrl Pts',(6.80184162063874,0.529942106161782,2.59526651846583));
#92788=CARTESIAN_POINT('Ctrl Pts',(6.82776866093176,0.53739670052164,2.54765355736703));
#92789=CARTESIAN_POINT('Ctrl Pts',(6.85287409329062,0.544769999851891,2.50035717693401));
#92790=CARTESIAN_POINT('',(6.84187682086182,0.552026825706407,2.55114039807484));
#92791=CARTESIAN_POINT('Ctrl Pts',(6.84187682083898,0.552026824711191,2.55114039821205));
#92792=CARTESIAN_POINT('Ctrl Pts',(6.82932315673046,0.547477948795513,2.57178787122331));
#92793=CARTESIAN_POINT('Ctrl Pts',(6.81666873272011,0.542929076939321,2.5923744209764));
#92794=CARTESIAN_POINT('Ctrl Pts',(6.80391453028886,0.538380664576819,2.61289873058665));
#92795=CARTESIAN_POINT('Ctrl Pts',(6.79116030393554,0.533832243683208,2.63342307869278));
#92796=CARTESIAN_POINT('Ctrl Pts',(6.77830241727891,0.529279732193272,2.65388255530014));
#92797=CARTESIAN_POINT('Ctrl Pts',(6.76533200698369,0.524710848747534,2.67426639813));
#92798=CARTESIAN_POINT('Ctrl Pts',(6.74206420002228,0.516514662534077,2.71083326913107));
#92799=CARTESIAN_POINT('Ctrl Pts',(6.71844204411595,0.508277071780336,2.74716785710491));
#92800=CARTESIAN_POINT('Ctrl Pts',(6.69447254313508,0.499999999636659,2.78326020476335));
#92801=CARTESIAN_POINT('',(6.64232590877187,0.655900535624813,3.27518995864757));
#92802=CARTESIAN_POINT('Ctrl Pts',(6.64232590877187,0.655900535624812,3.27518995864757));
#92803=CARTESIAN_POINT('Ctrl Pts',(6.68183779107667,0.638769108022223,3.15631915930124));
#92804=CARTESIAN_POINT('Ctrl Pts',(6.71825115862536,0.621541657210669,3.0364638737519));
#92805=CARTESIAN_POINT('Ctrl Pts',(6.78480604698142,0.586905785313935,2.79499154249107));
#92806=CARTESIAN_POINT('Ctrl Pts',(6.81493433654931,0.569504150542412,2.67342181166954));
#92807=CARTESIAN_POINT('Ctrl Pts',(6.84187682229732,0.552026827040526,2.55114039820044));
#92808=CARTESIAN_POINT('',(6.1891408947314,0.552026825513628,3.8748071900381));
#92809=CARTESIAN_POINT('Ctrl Pts',(6.18914089379959,0.552026825263855,3.8748071892122));
#92810=CARTESIAN_POINT('Ctrl Pts',(6.21015345762421,0.556533631536028,3.84973732301981));
#92811=CARTESIAN_POINT('Ctrl Pts',(6.22930290716358,0.560675802450135,3.82657899851928));
#92812=CARTESIAN_POINT('Ctrl Pts',(6.26870148598491,0.569263221090252,3.77835375142444));
#92813=CARTESIAN_POINT('Ctrl Pts',(6.28835357540481,0.573581754057455,3.75398724728214));
#92814=CARTESIAN_POINT('Ctrl Pts',(6.3469546046639,0.586565893266171,3.68038482155418));
#92815=CARTESIAN_POINT('Ctrl Pts',(6.3854356014944,0.595235853590531,3.63078058208177));
#92816=CARTESIAN_POINT('Ctrl Pts',(6.49885212650631,0.621229052846318,3.48071062903566));
#92817=CARTESIAN_POINT('Ctrl Pts',(6.5718825375239,0.638561214261876,3.37884640143506));
#92818=CARTESIAN_POINT('Ctrl Pts',(6.64232590890062,0.655900535791303,3.27518995876292));
#92819=CARTESIAN_POINT('',(6.28070594613547,0.499999998589842,3.62149593535559));
#92820=CARTESIAN_POINT('Origin',(-0.426897292137384,0.00294846562083999,
1.44751727326905));
#92821=CARTESIAN_POINT('',(6.15515482210084,0.544769999370239,3.91506557539984));
#92822=CARTESIAN_POINT('Origin',(-0.53054502599663,0.376341896131434,0.904427643646886));
#92823=CARTESIAN_POINT('',(5.93964082487683,0.499999999760686,4.15730283636664));
#92824=CARTESIAN_POINT('Ctrl Pts',(5.93964082464481,0.499999999816603,4.15730283616115));
#92825=CARTESIAN_POINT('Ctrl Pts',(5.97647028641283,0.507497225167955,4.11775823300134));
#92826=CARTESIAN_POINT('Ctrl Pts',(6.01284887255721,0.514976130663546,4.07779249736097));
#92827=CARTESIAN_POINT('Ctrl Pts',(6.08491270977972,0.529942096794905,3.9967855680827));
#92828=CARTESIAN_POINT('Ctrl Pts',(6.12046892415114,0.537396680762836,3.95585937707875));
#92829=CARTESIAN_POINT('Ctrl Pts',(6.15515482248417,0.544769999922148,3.91506557582553));
#92830=CARTESIAN_POINT('',(6.13349776832425,0.552026825402507,3.962297425611));
#92831=CARTESIAN_POINT('Ctrl Pts',(6.13349776847326,0.552026824802072,3.96229742541378));
#92832=CARTESIAN_POINT('Ctrl Pts',(6.11679900578816,0.547477948809804,3.97976350511362));
#92833=CARTESIAN_POINT('Ctrl Pts',(6.10001493530689,0.542929076865411,3.99714842583357));
#92834=CARTESIAN_POINT('Ctrl Pts',(6.08314679897251,0.538380664438636,4.01445111215885));
#92835=CARTESIAN_POINT('Ctrl Pts',(6.06627863099977,0.533832243480725,4.03175383093755));
#92836=CARTESIAN_POINT('Ctrl Pts',(6.04932317173958,0.529279731995422,4.04897091103435));
#92837=CARTESIAN_POINT('Ctrl Pts',(6.03227407857486,0.524710848504994,4.06608993632827));
#92838=CARTESIAN_POINT('Ctrl Pts',(6.00168946366319,0.516514662304296,4.09680000349837));
#92839=CARTESIAN_POINT('Ctrl Pts',(5.97080871823432,0.508277071501415,4.12720704368692));
#92840=CARTESIAN_POINT('Ctrl Pts',(5.93964082487683,0.499999999760686,4.15730283636664));
#92841=CARTESIAN_POINT('',(5.7829629925841,0.65590053576872,4.62652156291335));
#92842=CARTESIAN_POINT('Ctrl Pts',(5.7829629925841,0.65590053576872,4.62652156291335));
#92843=CARTESIAN_POINT('Ctrl Pts',(5.84710481719915,0.638769108144735,4.51892378339903));
#92844=CARTESIAN_POINT('Ctrl Pts',(5.90843220401921,0.621541657296678,4.40969844533471));
#92845=CARTESIAN_POINT('Ctrl Pts',(6.02534048954105,0.586905785338163,4.18817893639138));
#92846=CARTESIAN_POINT('Ctrl Pts',(6.08089829496035,0.569504150567409,4.07592813004998));
#92847=CARTESIAN_POINT('Ctrl Pts',(6.13349776971531,0.552026827065365,3.96229742599917));
#92848=CARTESIAN_POINT('',(5.21147321258346,0.552026825488821,5.11469869387848));
#92849=CARTESIAN_POINT('Ctrl Pts',(5.21147321185043,0.552026825253602,5.11469869287415));
#92850=CARTESIAN_POINT('Ctrl Pts',(5.23738379394425,0.556533631561209,5.09473202620163));
#92851=CARTESIAN_POINT('Ctrl Pts',(5.26106389523096,0.56067580248612,5.07623169604516));
#92852=CARTESIAN_POINT('Ctrl Pts',(5.30990835981114,0.569263221146577,5.03760345824506));
#92853=CARTESIAN_POINT('Ctrl Pts',(5.33433907239866,0.573581754115852,5.01803124777013));
#92854=CARTESIAN_POINT('Ctrl Pts',(5.40739238788304,0.58656589331835,4.95874709504346));
#92855=CARTESIAN_POINT('Ctrl Pts',(5.45563716547813,0.595235853632867,4.91857485205941));
#92856=CARTESIAN_POINT('Ctrl Pts',(5.59866267879059,0.62122905286391,4.79639465167396));
#92857=CARTESIAN_POINT('Ctrl Pts',(5.69188347709121,0.638561214252059,4.71261133285237));
#92858=CARTESIAN_POINT('Ctrl Pts',(5.78296299256075,0.655900535730205,4.62652156288089));
#92859=CARTESIAN_POINT('',(5.35535195535873,0.499999998694155,4.88699349605534));
#92860=CARTESIAN_POINT('Origin',(-0.728090752506269,0.0029480239586694,
1.32190450536879));
#92861=CARTESIAN_POINT('',(5.16962735214908,0.544769999440516,5.14670986015818));
#92862=CARTESIAN_POINT('Origin',(-0.712566664853689,0.376341596677865,0.769230974754304));
#92863=CARTESIAN_POINT('',(4.90707810144185,0.499999999671717,5.3369546096604));
#92864=CARTESIAN_POINT('Ctrl Pts',(4.90707810144553,0.499999999737817,5.33695460937341));
#92865=CARTESIAN_POINT('Ctrl Pts',(4.95154737164714,0.507497215012864,5.30625182412512));
#92866=CARTESIAN_POINT('Ctrl Pts',(4.99566684143965,0.514976110205956,5.27504083117598));
#92867=CARTESIAN_POINT('Ctrl Pts',(5.08346013591554,0.529942106054155,5.21141926724436));
#92868=CARTESIAN_POINT('Ctrl Pts',(5.12698304405488,0.537396700469416,5.17909339564586));
#92869=CARTESIAN_POINT('Ctrl Pts',(5.16962735231623,0.54476999976665,5.14670986045255));
#92870=CARTESIAN_POINT('',(5.13832317726269,0.55202682536752,5.18818182882492));
#92871=CARTESIAN_POINT('Ctrl Pts',(5.13832317758696,0.552026824841263,5.18818182871674));
#92872=CARTESIAN_POINT('Ctrl Pts',(5.11826013240217,0.547477949078305,5.20164982047142));
#92873=CARTESIAN_POINT('Ctrl Pts',(5.0981312204291,0.542929077204698,5.21502021216858));
#92874=CARTESIAN_POINT('Ctrl Pts',(5.07793788597092,0.53838066482091,5.22829222036761));
#92875=CARTESIAN_POINT('Ctrl Pts',(5.05774451363797,0.533832243906083,5.24156425345972));
#92876=CARTESIAN_POINT('Ctrl Pts',(5.0374843006292,0.529279732469265,5.25473388501665));
#92877=CARTESIAN_POINT('Ctrl Pts',(5.01715372172125,0.524710849052911,5.26778762574449));
#92878=CARTESIAN_POINT('Ctrl Pts',(4.98068240076011,0.516514662694109,5.29120492094222));
#92879=CARTESIAN_POINT('Ctrl Pts',(4.9439870145053,0.508277071784162,5.31426261449142));
#92880=CARTESIAN_POINT('Ctrl Pts',(4.90707810144185,0.499999999671717,5.3369546096604));
#92881=CARTESIAN_POINT('',(4.65319515451439,0.655900535591315,5.76152215973136));
#92882=CARTESIAN_POINT('Ctrl Pts',(4.65319515451439,0.655900535591315,5.76152215973136));
#92883=CARTESIAN_POINT('Ctrl Pts',(4.73896772095617,0.638769107997606,5.67022855280486));
#92884=CARTESIAN_POINT('Ctrl Pts',(4.82234152657392,0.621541657168761,5.57674041779526));
#92885=CARTESIAN_POINT('Ctrl Pts',(4.9841367074677,0.586905785274489,5.38553173775688));
#92886=CARTESIAN_POINT('Ctrl Pts',(5.06252620792821,0.569504150405887,5.28784857825658));
#92887=CARTESIAN_POINT('Ctrl Pts',(5.13832317842015,0.552026826925386,5.18818182943199));
#92888=CARTESIAN_POINT('',(3.99012283422776,0.552026825492826,6.11543257150016));
#92889=CARTESIAN_POINT('Ctrl Pts',(3.99012283383667,0.552026825050405,6.11543257052606));
#92890=CARTESIAN_POINT('Ctrl Pts',(4.01972335837119,0.556534160395578,6.10150108746967));
#92891=CARTESIAN_POINT('Ctrl Pts',(4.04682057104575,0.560675371296844,6.08852680808817));
#92892=CARTESIAN_POINT('Ctrl Pts',(4.10282982036569,0.569263221096838,6.06130042618763));
#92893=CARTESIAN_POINT('Ctrl Pts',(4.13089680313499,0.573581754058485,6.04743768417028));
#92894=CARTESIAN_POINT('Ctrl Pts',(4.21498651311904,0.586565893258238,6.00524386536356));
#92895=CARTESIAN_POINT('Ctrl Pts',(4.27073919943005,0.595235853580056,5.97638202814542));
#92896=CARTESIAN_POINT('Ctrl Pts',(4.43668598715217,0.621229052810602,5.88780459051503));
#92897=CARTESIAN_POINT('Ctrl Pts',(4.54573827185856,0.638561214197787,5.8260197952161));
#92898=CARTESIAN_POINT('Ctrl Pts',(4.65319515454537,0.655900535666704,5.76152215980325));
#92899=CARTESIAN_POINT('',(4.1795876597685,0.499999998696719,5.92398067050494));
#92900=CARTESIAN_POINT('Origin',(-0.99523750800882,0.00294860086620573,
1.1344822676465));
#92901=CARTESIAN_POINT('',(3.94237385367589,0.544769999466827,6.13769971104598));
#92902=CARTESIAN_POINT('Origin',(-0.861268422572583,0.376342028655932,0.598066782903451));
#92903=CARTESIAN_POINT('',(3.64506586129707,0.499999999748423,6.26705631602722));
#92904=CARTESIAN_POINT('Ctrl Pts',(3.6450658613806,0.499999999832972,6.26705631566973));
#92905=CARTESIAN_POINT('Ctrl Pts',(3.69509565834736,0.507497215478395,6.24663092213573));
#92906=CARTESIAN_POINT('Ctrl Pts',(3.74489308261439,0.514976111013341,6.22563400564159));
#92907=CARTESIAN_POINT('Ctrl Pts',(3.84431057014932,0.529942106213477,6.18237284342222));
#92908=CARTESIAN_POINT('Ctrl Pts',(3.89376504607911,0.537396700953456,6.16015887031076));
#92909=CARTESIAN_POINT('Ctrl Pts',(3.94237385379529,0.544769999856384,6.13769971143229));
#92910=CARTESIAN_POINT('',(3.90288630483179,0.552026825400315,6.17147261660978));
#92911=CARTESIAN_POINT('Ctrl Pts',(3.90288630490168,0.552026824702873,6.17147261644347));
#92912=CARTESIAN_POINT('Ctrl Pts',(3.88039710166864,0.547477948715548,6.18031277249131));
#92913=CARTESIAN_POINT('Ctrl Pts',(3.85786455338572,0.542929076879934,6.18904345089288));
#92914=CARTESIAN_POINT('Ctrl Pts',(3.83529023832017,0.538380664523847,6.19766419700609));
#92915=CARTESIAN_POINT('Ctrl Pts',(3.81271588091332,0.533832243636574,6.20628495928871));
#92916=CARTESIAN_POINT('Ctrl Pts',(3.79009825880634,0.529279732103297,6.21479134522615));
#92917=CARTESIAN_POINT('Ctrl Pts',(3.76743682902675,0.52471084863187,6.22316942325172));
#92918=CARTESIAN_POINT('Ctrl Pts',(3.72678416194743,0.516514662402908,6.23819897875861));
#92919=CARTESIAN_POINT('Ctrl Pts',(3.68598997183275,0.508277071642075,6.25282917252519));
#92920=CARTESIAN_POINT('Ctrl Pts',(3.64506586129707,0.499999999748423,6.26705631602722));
#92921=CARTESIAN_POINT('',(3.30584908284948,0.655900535589578,6.62712038403327));
#92922=CARTESIAN_POINT('Ctrl Pts',(3.30584908284948,0.655900535589577,6.62712038403327));
#92923=CARTESIAN_POINT('Ctrl Pts',(3.40924176110029,0.638769108003684,6.55639973733554));
#92924=CARTESIAN_POINT('Ctrl Pts',(3.51076351889193,0.621541657192441,6.4830202067497));
#92925=CARTESIAN_POINT('Ctrl Pts',(3.70988023275112,0.586905785290167,6.33106306050518));
#92926=CARTESIAN_POINT('Ctrl Pts',(3.80743602116347,0.569504150620629,6.25251510518218));
#92927=CARTESIAN_POINT('Ctrl Pts',(3.90288630586329,0.552026827148797,6.1714726174476));
#92928=CARTESIAN_POINT('',(2.58219874684554,0.552026825517167,6.83021561872381));
#92929=CARTESIAN_POINT('Ctrl Pts',(2.58219874670539,0.552026824982957,6.830215617774));
#92930=CARTESIAN_POINT('Ctrl Pts',(2.61410208447286,0.556534160325457,6.82297308283996));
#92931=CARTESIAN_POINT('Ctrl Pts',(2.64335486588199,0.560675371218705,6.81612723464921));
#92932=CARTESIAN_POINT('Ctrl Pts',(2.70390751748938,0.569263221030049,6.80157772338699));
#92933=CARTESIAN_POINT('Ctrl Pts',(2.73429838960121,0.573581753996881,6.79407265620546));
#92934=CARTESIAN_POINT('Ctrl Pts',(2.82549255285121,0.586565893214642,6.77094210737457));
#92935=CARTESIAN_POINT('Ctrl Pts',(2.88614621429549,0.595235853550835,6.75474022336757));
#92936=CARTESIAN_POINT('Ctrl Pts',(3.06725478939875,0.621229052830664,6.70390733094793));
#92937=CARTESIAN_POINT('Ctrl Pts',(3.18703939713228,0.638561214261602,6.66701004743552));
#92938=CARTESIAN_POINT('Ctrl Pts',(3.3058490828888,0.655900535789811,6.62712038423742));
#92939=CARTESIAN_POINT('',(2.80839049046689,0.499999998797894,6.68396909412142));
#92940=CARTESIAN_POINT('Origin',(-1.21585023743329,0.00294803147734828,
0.894011165756495));
#92941=CARTESIAN_POINT('',(2.53077933515541,0.544769999391056,6.8416975452563));
#92942=CARTESIAN_POINT('Origin',(-0.969699669491749,0.37634162951501,0.398936186856903));
#92943=CARTESIAN_POINT('',(2.21261439168749,0.499999999735722,6.90411743489196));
#92944=CARTESIAN_POINT('Ctrl Pts',(2.21261439184017,0.499999999817213,6.90411743457275));
#92945=CARTESIAN_POINT('Ctrl Pts',(2.26586537544578,0.507497215380639,6.89492450289489));
#92946=CARTESIAN_POINT('Ctrl Pts',(2.31901227965089,0.514976110859343,6.88512345692522));
#92947=CARTESIAN_POINT('Ctrl Pts',(2.42540202165424,0.529941643169758,6.86424618355541));
#92948=CARTESIAN_POINT('Ctrl Pts',(2.47848205947058,0.537397143804212,6.85318147571591));
#92949=CARTESIAN_POINT('Ctrl Pts',(2.53077933520185,0.544769999930024,6.84169754581379));
#92950=CARTESIAN_POINT('',(2.48495480706808,0.55202682538978,6.86619220319719));
#92951=CARTESIAN_POINT('Ctrl Pts',(2.48495480726074,0.552026824761649,6.86619220313449));
#92952=CARTESIAN_POINT('Ctrl Pts',(2.46109101724883,0.547477948836403,6.86999116731842));
#92953=CARTESIAN_POINT('Ctrl Pts',(2.43720842975439,0.54292907699423,6.87367389544388));
#92954=CARTESIAN_POINT('Ctrl Pts',(2.41330868415241,0.53838066468276,6.877240282869));
#92955=CARTESIAN_POINT('Ctrl Pts',(2.38940889372308,0.533832243840099,6.88080667698338));
#92956=CARTESIAN_POINT('Ctrl Pts',(2.36549143763035,0.529279732381481,6.88425206820953));
#92957=CARTESIAN_POINT('Ctrl Pts',(2.34155878047422,0.524710848937538,6.88756273388734));
#92958=CARTESIAN_POINT('Ctrl Pts',(2.29862563898931,0.516514662528013,6.89350178516055));
#92959=CARTESIAN_POINT('Ctrl Pts',(2.2556401341689,0.508277071523872,6.89902038819499));
#92960=CARTESIAN_POINT('Ctrl Pts',(2.21261439168749,0.499999999735722,6.90411743489196));
#92961=CARTESIAN_POINT('',(1.80392518236685,0.655900535538507,7.18284182470367));
#92962=CARTESIAN_POINT('Ctrl Pts',(1.80392518236684,0.655900535538507,7.18284182470367));
#92963=CARTESIAN_POINT('Ctrl Pts',(1.92010344582086,0.638769107941213,7.13600095696403));
#92964=CARTESIAN_POINT('Ctrl Pts',(2.03502611133774,0.621541657127866,7.08616117597769));
#92965=CARTESIAN_POINT('Ctrl Pts',(2.26215388153276,0.58690578524841,6.98056091106265));
#92966=CARTESIAN_POINT('Ctrl Pts',(2.37431435872934,0.56950415051877,6.92482097387188));
#92967=CARTESIAN_POINT('Ctrl Pts',(2.48495480789597,0.552026827062388,6.86619220426093));
#92968=CARTESIAN_POINT('',(1.05353391884569,0.552026825489145,7.22562537467431));
#92969=CARTESIAN_POINT('Ctrl Pts',(1.05353391887314,0.552026825234067,7.22562537350378));
#92970=CARTESIAN_POINT('Ctrl Pts',(1.08624446534929,0.556533631523835,7.22541046479856));
#92971=CARTESIAN_POINT('Ctrl Pts',(1.1162919525488,0.560675802443273,7.22501306695583));
#92972=CARTESIAN_POINT('Ctrl Pts',(1.17855350558121,0.569263221096503,7.22382080521556));
#92973=CARTESIAN_POINT('Ctrl Pts',(1.20984722359606,0.573581754066956,7.22302434149009));
#92974=CARTESIAN_POINT('Ctrl Pts',(1.30388170217393,0.586565893281114,7.22003862145737));
#92975=CARTESIAN_POINT('Ctrl Pts',(1.36660024076868,0.595235853609543,7.21725427280032));
#92976=CARTESIAN_POINT('Ctrl Pts',(1.55440216717859,0.621229052885991,7.20654281528298));
#92977=CARTESIAN_POINT('Ctrl Pts',(1.67931810259728,0.638561214319169,7.19625831961395));
#92978=CARTESIAN_POINT('Ctrl Pts',(1.80392518235829,0.655900535850668,7.18284182502767));
#92979=CARTESIAN_POINT('',(1.30587610362313,0.499999998542182,7.1314225503174));
#92980=CARTESIAN_POINT('Origin',(-1.37960997614413,0.00294866857638937,
0.611738390161336));
#92981=CARTESIAN_POINT('',(1.00084838688029,0.544769999485534,7.22578520659681));
#92982=CARTESIAN_POINT('Origin',(-1.03278788981951,0.376341816128584,0.181153191190526));
#92983=CARTESIAN_POINT('',(0.676703532269247,0.499999999748659,7.21834969580106));
#92984=CARTESIAN_POINT('Ctrl Pts',(0.676703532495311,0.499999999833265,
7.21834969551148));
#92985=CARTESIAN_POINT('Ctrl Pts',(0.730685746631788,0.50749721541619,7.22081907684223));
#92986=CARTESIAN_POINT('Ctrl Pts',(0.784697041277654,0.514976110958078,
7.22267218728766));
#92987=CARTESIAN_POINT('Ctrl Pts',(0.893087446816106,0.529941643242395,
7.22515366262821));
#92988=CARTESIAN_POINT('Ctrl Pts',(0.947305091113319,0.537397144273938,
7.22575828055198));
#92989=CARTESIAN_POINT('Ctrl Pts',(1.00084838683405,0.544769999820073,7.22578520694095));
#92990=CARTESIAN_POINT('',(0.950829584292169,0.552026825382187,7.23985627366907));
#92991=CARTESIAN_POINT('Ctrl Pts',(0.950829584616152,0.552026824852022,
7.23985627373207));
#92992=CARTESIAN_POINT('Ctrl Pts',(0.926707051733455,0.547477948948255,
7.23843641100287));
#92993=CARTESIAN_POINT('Ctrl Pts',(0.902591147829787,0.54292907703239,7.23689898861412));
#92994=CARTESIAN_POINT('Ctrl Pts',(0.878483496783891,0.538380664623052,
7.23524425699157));
#92995=CARTESIAN_POINT('Ctrl Pts',(0.854375800520945,0.533832243682573,
7.23358952226536));
#92996=CARTESIAN_POINT('Ctrl Pts',(0.830276863638705,0.529279732179528,
7.23181281608786));
#92997=CARTESIAN_POINT('Ctrl Pts',(0.80619204309476,0.524710848694838,7.22990126639148));
#92998=CARTESIAN_POINT('Ctrl Pts',(0.762985934765295,0.5165146624528,7.22647210971131));
#92999=CARTESIAN_POINT('Ctrl Pts',(0.719819071259968,0.508277071638636,
7.22262107810339));
#93000=CARTESIAN_POINT('Ctrl Pts',(0.676703532269247,0.499999999748659,
7.21834969580106));
#93001=CARTESIAN_POINT('',(0.21765174455862,0.655900535668849,7.40270156512545));
#93002=CARTESIAN_POINT('Ctrl Pts',(0.21765174455862,0.655900535668849,7.40270156512545));
#93003=CARTESIAN_POINT('Ctrl Pts',(0.341183226867587,0.638769108054916,
7.38193070326879));
#93004=CARTESIAN_POINT('Ctrl Pts',(0.464133144124308,0.621541657205909,
7.35796112462327));
#93005=CARTESIAN_POINT('Ctrl Pts',(0.708651728687176,0.586905785278378,
7.30365549191793));
#93006=CARTESIAN_POINT('Ctrl Pts',(0.83017239566547,0.569504150432432,7.27332991046189));
#93007=CARTESIAN_POINT('Ctrl Pts',(0.95082958488062,0.552026826960472,7.23985627496611));
#93008=CARTESIAN_POINT('',(-0.524392983759562,0.552026825661112,7.28317291910593));
#93009=CARTESIAN_POINT('Ctrl Pts',(-0.524392986242582,0.552026825224637,
7.28317291791701));
#93010=CARTESIAN_POINT('Ctrl Pts',(-0.492420046797248,0.556530947657473,
7.28999077169901));
#93011=CARTESIAN_POINT('Ctrl Pts',(-0.463017453584124,0.560669204314555,
7.29605638370086));
#93012=CARTESIAN_POINT('Ctrl Pts',(-0.40199584998173,0.56925092205502,7.30826883166599));
#93013=CARTESIAN_POINT('Ctrl Pts',(-0.371284572245158,0.57356636754223,
7.31421437802009));
#93014=CARTESIAN_POINT('Ctrl Pts',(-0.27887318750627,0.586541205299183,
7.33150238020033));
#93015=CARTESIAN_POINT('Ctrl Pts',(-0.217066995461581,0.595204946697494,
7.34225972045226));
#93016=CARTESIAN_POINT('Ctrl Pts',(-0.0313101433752705,0.621204274123675,
7.37218433405402));
#93017=CARTESIAN_POINT('Ctrl Pts',(0.092984705121821,0.638548819288446,
7.38900776886407));
#93018=CARTESIAN_POINT('Ctrl Pts',(0.217651744540169,0.655900535742686,
7.40270156519986));
#93019=CARTESIAN_POINT('',(-0.257699600093122,0.499999998735122,7.24541861505891));
#93020=CARTESIAN_POINT('Origin',(-1.47886105903604,0.00294835975049063,
0.30086193846136));
#93021=CARTESIAN_POINT('',(-0.575881118631359,0.544769999479607,7.2720031822402));
#93022=CARTESIAN_POINT('Origin',(-1.04758443315409,0.376341791154719,-0.0451004524651299));
#93023=CARTESIAN_POINT('',(-0.890849230764474,0.499999999848743,7.19505994779791));
#93024=CARTESIAN_POINT('Ctrl Pts',(-0.890849230400919,0.499999999957417,
7.19505994749708));
#93025=CARTESIAN_POINT('Ctrl Pts',(-0.838659931347879,0.507497215999936,
7.20907617723531));
#93026=CARTESIAN_POINT('Ctrl Pts',(-0.786309751644111,0.514976111985247,
7.22249679544923));
#93027=CARTESIAN_POINT('Ctrl Pts',(-0.680986902604104,0.529941643519156,
7.24822098717489));
#93028=CARTESIAN_POINT('Ctrl Pts',(-0.628166811783102,0.537397144461801,
7.26046666019013));
#93029=CARTESIAN_POINT('Ctrl Pts',(-0.57588111875408,0.544769999824209,
7.27200318257616));
#93030=CARTESIAN_POINT('',(-0.627755373541268,0.552026825840142,7.27499271185807));
#93031=CARTESIAN_POINT('Ctrl Pts',(-0.627755373720756,0.552026824602212,
7.27499271173872));
#93032=CARTESIAN_POINT('Ctrl Pts',(-0.651008707501433,0.547477948488361,
7.26842041243539));
#93033=CARTESIAN_POINT('Ctrl Pts',(-0.674230294564099,0.542929076630835,
7.26173472770646));
#93034=CARTESIAN_POINT('Ctrl Pts',(-0.697418603710524,0.538380664303708,
7.2549362505121));
#93035=CARTESIAN_POINT('Ctrl Pts',(-0.720606956350182,0.533832243445335,
7.24813776056616));
#93036=CARTESIAN_POINT('Ctrl Pts',(-0.743760534077517,0.529279731888512,
7.24122203367185));
#93037=CARTESIAN_POINT('Ctrl Pts',(-0.766871338143885,0.52471084838398,
7.23417765045406));
#93038=CARTESIAN_POINT('Ctrl Pts',(-0.808330143625273,0.516514662221979,
7.22154062957309));
#93039=CARTESIAN_POINT('Ctrl Pts',(-0.849659931167968,0.508277071487567,
7.20850003345545));
#93040=CARTESIAN_POINT('Ctrl Pts',(-0.890849230764474,0.499999999848743,
7.19505994779791));
#93041=CARTESIAN_POINT('',(-1.37879884614972,0.655900535669628,7.27641920769329));
#93042=CARTESIAN_POINT('Ctrl Pts',(-1.37879884614972,0.655900535669628,
7.27641920769329));
#93043=CARTESIAN_POINT('Ctrl Pts',(-1.25369034011231,0.638769108073372,
7.28268957415428));
#93044=CARTESIAN_POINT('Ctrl Pts',(-1.12846217290469,0.621541657257245,
7.28571098877648));
#93045=CARTESIAN_POINT('Ctrl Pts',(-0.87798619120963,0.586905785341198,
7.28523925936566));
#93046=CARTESIAN_POINT('Ctrl Pts',(-0.752787506813266,0.569504150568537,
7.28174602444789));
#93047=CARTESIAN_POINT('Ctrl Pts',(-0.627755373309366,0.552026827055009,
7.2749927130075));
#93048=CARTESIAN_POINT('',(-2.07779985949837,0.552026825471116,7.00016739177855));
#93049=CARTESIAN_POINT('Ctrl Pts',(-2.07779985901207,0.552026825063992,
7.00016739084456));
#93050=CARTESIAN_POINT('Ctrl Pts',(-2.0480188374859,0.556534160438074,7.01370873647915));
#93051=CARTESIAN_POINT('Ctrl Pts',(-2.02058797011571,0.560675371355804,
7.02596183329651));
#93052=CARTESIAN_POINT('Ctrl Pts',(-1.96357743496575,0.569263221179983,
7.05102397170068));
#93053=CARTESIAN_POINT('Ctrl Pts',(-1.93484159927572,0.573581754149126,
7.06344101193721));
#93054=CARTESIAN_POINT('Ctrl Pts',(-1.84824454669598,0.586565893347276,
7.10021529850817));
#93055=CARTESIAN_POINT('Ctrl Pts',(-1.79015362512635,0.595235853657326,
7.12402312288938));
#93056=CARTESIAN_POINT('Ctrl Pts',(-1.61521158880238,0.621229052879646,
7.19315764940022));
#93057=CARTESIAN_POINT('Ctrl Pts',(-1.49752260870047,0.638561214263646,
7.23627453375838));
#93058=CARTESIAN_POINT('Ctrl Pts',(-1.37879884618104,0.655900535737622,
7.27641920775656));
#93059=CARTESIAN_POINT('',(-1.80922555565879,0.499999998859462,7.02062695834227));
#93060=CARTESIAN_POINT('Origin',(-1.50896237484285,0.00294800655703135,
-0.0240861790254565));
#93061=CARTESIAN_POINT('',(-2.12568306326361,0.544769999386832,6.97819037132897));
#93062=CARTESIAN_POINT('Origin',(-1.01339705640315,0.376341645026371,-0.269247012856438));
#93063=CARTESIAN_POINT('',(-2.41674687579387,0.499999999814145,6.83533719297713));
#93064=CARTESIAN_POINT('Ctrl Pts',(-2.4167468754063,0.499999999914496,6.83533719277799));
#93065=CARTESIAN_POINT('Ctrl Pts',(-2.36879080914693,0.507497215798708,
6.86024488696298));
#93066=CARTESIAN_POINT('Ctrl Pts',(-2.32054958464766,0.514976111623878,
6.88460547932891));
#93067=CARTESIAN_POINT('Ctrl Pts',(-2.22321906508015,0.52994164330363,6.93236955346637));
#93068=CARTESIAN_POINT('Ctrl Pts',(-2.17426633735912,0.537397144146483,
6.95568368725052));
#93069=CARTESIAN_POINT('Ctrl Pts',(-2.12568306352827,0.544769999861654,
6.97819037174472));
#93070=CARTESIAN_POINT('',(-2.17698718727294,0.552026825671207,6.96995857575535));
#93071=CARTESIAN_POINT('Ctrl Pts',(-2.17698718740211,0.552026824726497,
6.96995857572821));
#93072=CARTESIAN_POINT('Ctrl Pts',(-2.19828402078696,0.547477948713226,
6.95854115432079));
#93073=CARTESIAN_POINT('Ctrl Pts',(-2.21952547527805,0.542929076826028,
6.94701982242141));
#93074=CARTESIAN_POINT('Ctrl Pts',(-2.24071018282034,0.538380664459791,
6.93539548884392));
#93075=CARTESIAN_POINT('Ctrl Pts',(-2.26189493009731,0.533832243562413,
6.92377113346348));
#93076=CARTESIAN_POINT('Ctrl Pts',(-2.28302051311801,0.529279732138545,
6.9120397577923));
#93077=CARTESIAN_POINT('Ctrl Pts',(-2.30407666515051,0.524710848698101,
6.9001919287274));
#93078=CARTESIAN_POINT('Ctrl Pts',(-2.34184960124397,0.516514662521826,
6.87893793657233));
#93079=CARTESIAN_POINT('Ctrl Pts',(-2.37940977898813,0.508277071730129,
6.85731753954631));
#93080=CARTESIAN_POINT('Ctrl Pts',(-2.41674687579387,0.499999999814145,
6.83533719297713));
#93081=CARTESIAN_POINT('',(-2.91077833515283,0.655900535563285,6.80989957534335));
#93082=CARTESIAN_POINT('Ctrl Pts',(-2.91077833515282,0.655900535563285,
6.80989957534335));
#93083=CARTESIAN_POINT('Ctrl Pts',(-2.78994273993378,0.638769107994248,
6.84291797474596));
#93084=CARTESIAN_POINT('Ctrl Pts',(-2.66829185254302,0.621541657190023,
6.87278910459999));
#93085=CARTESIAN_POINT('Ctrl Pts',(-2.42357045251948,0.586905785308089,
6.92617333592512));
#93086=CARTESIAN_POINT('Ctrl Pts',(-2.30054790110173,0.569504150458014,
6.94967578725998));
#93087=CARTESIAN_POINT('Ctrl Pts',(-2.17698718732734,0.552026826956038,
6.96995857719386));
#93088=CARTESIAN_POINT('',(-3.53405111803077,0.552026825436308,6.38984181842886));
#93089=CARTESIAN_POINT('Ctrl Pts',(-3.5340511174011,0.55202682514116,6.38984181765692));
#93090=CARTESIAN_POINT('Ctrl Pts',(-3.50788042103548,0.556533631427338,
6.40946630957861));
#93091=CARTESIAN_POINT('Ctrl Pts',(-3.48371932988497,0.56067580235628,6.42733390841975));
#93092=CARTESIAN_POINT('Ctrl Pts',(-3.43343181318378,0.569263221019227,
6.46406384362574));
#93093=CARTESIAN_POINT('Ctrl Pts',(-3.40803710195941,0.573581753992496,
6.48236793562192));
#93094=CARTESIAN_POINT('Ctrl Pts',(-3.33137002479532,0.586565893218342,
6.53689826642438));
#93095=CARTESIAN_POINT('Ctrl Pts',(-3.27975521506038,0.595235853551728,
6.57263730817139));
#93096=CARTESIAN_POINT('Ctrl Pts',(-3.12376510570602,0.621229052822137,
6.67776287459229));
#93097=CARTESIAN_POINT('Ctrl Pts',(-3.0180964840573,0.638561214233471,6.74517136209263));
#93098=CARTESIAN_POINT('Ctrl Pts',(-2.91077833526805,0.655900535740567,
6.8098995754869));
#93099=CARTESIAN_POINT('',(-3.2761541350426,0.499999998792703,6.46755858744837));
#93100=CARTESIAN_POINT('Origin',(-1.4685061574169,0.00294812732458634,-0.347904248396754));
#93101=CARTESIAN_POINT('',(-3.57609043012587,0.544769999287053,6.35808513454016));
#93102=CARTESIAN_POINT('Origin',(-0.931824239855779,0.376341640093868,-0.480802598575032));
#93103=CARTESIAN_POINT('',(-3.82964012287191,0.499999999696682,6.15600166741686));
#93104=CARTESIAN_POINT('Ctrl Pts',(-3.82964012256917,0.499999999768787,
6.15600166733699));
#93105=CARTESIAN_POINT('Ctrl Pts',(-3.78815966332415,0.507497215154986,
6.1906361677964));
#93106=CARTESIAN_POINT('Ctrl Pts',(-3.74628310205829,0.514976110458603,
6.22479765807499));
#93107=CARTESIAN_POINT('Ctrl Pts',(-3.66149335131078,0.529942106105535,
6.29237031424076));
#93108=CARTESIAN_POINT('Ctrl Pts',(-3.61870214653602,0.53739670052456,6.32565872540602));
#93109=CARTESIAN_POINT('Ctrl Pts',(-3.57609043053771,0.54476999984924,6.35808513495353));
#93110=CARTESIAN_POINT('',(-3.62442550006042,0.552026825406838,6.33901692355712));
#93111=CARTESIAN_POINT('Ctrl Pts',(-3.62442549984507,0.552026824821491,
6.33901692372192));
#93112=CARTESIAN_POINT('Ctrl Pts',(-3.64277001657995,0.547477948894753,
6.32328824595075));
#93113=CARTESIAN_POINT('Ctrl Pts',(-3.66103811189774,0.542929077026949,
6.30746999158048));
#93114=CARTESIAN_POINT('Ctrl Pts',(-3.67922864469353,0.538380664716611,
6.29156334259472));
#93115=CARTESIAN_POINT('Ctrl Pts',(-3.69741921160855,0.533832243875003,
6.27565666377351));
#93116=CARTESIAN_POINT('Ctrl Pts',(-3.71552899113642,0.529279732316413,
6.25965818517536));
#93117=CARTESIAN_POINT('Ctrl Pts',(-3.73354592897964,0.524710848840588,
6.2435609014759));
#93118=CARTESIAN_POINT('Ctrl Pts',(-3.76586677534318,0.516514662443097,
6.21468375055004));
#93119=CARTESIAN_POINT('Ctrl Pts',(-3.79790107138936,0.508277071533348,
6.18549449790963));
#93120=CARTESIAN_POINT('Ctrl Pts',(-3.82964012287191,0.499999999696682,
6.15600166741686));
#93121=CARTESIAN_POINT('',(-4.30665306547384,0.655900535733099,6.02495660721441));
#93122=CARTESIAN_POINT('Ctrl Pts',(-4.30665306547384,0.655900535733099,
6.02495660721441));
#93123=CARTESIAN_POINT('Ctrl Pts',(-4.19574051901911,0.638769108122376,
6.08317913596235));
#93124=CARTESIAN_POINT('Ctrl Pts',(-4.08335517155792,0.621541657284017,
6.13850324028558));
#93125=CARTESIAN_POINT('Ctrl Pts',(-3.85583125313783,0.586905785338359,
6.24324724526053));
#93126=CARTESIAN_POINT('Ctrl Pts',(-3.74073723333524,0.569504150566424,
6.29264643421973));
#93127=CARTESIAN_POINT('Ctrl Pts',(-3.62442550038272,0.552026827061318,
6.33901692498913));
#93128=CARTESIAN_POINT('',(-4.82505407630461,0.552026825514354,5.48073434215193));
#93129=CARTESIAN_POINT('Ctrl Pts',(-4.82505407547324,0.552026825038895,
5.48073434152274));
#93130=CARTESIAN_POINT('Ctrl Pts',(-4.80371141587077,0.55653416040321,5.50552886028028));
#93131=CARTESIAN_POINT('Ctrl Pts',(-4.78396077681986,0.560675371301183,
5.5281673919086));
#93132=CARTESIAN_POINT('Ctrl Pts',(-4.74274273530616,0.569263221112224,
5.5748512749948));
#93133=CARTESIAN_POINT('Ctrl Pts',(-4.72187657706136,0.573581754077447,
5.59818653970657));
#93134=CARTESIAN_POINT('Ctrl Pts',(-4.65872434286268,0.586565893279194,
5.66792313689829));
#93135=CARTESIAN_POINT('Ctrl Pts',(-4.61599909629449,0.595235853596475,
5.71392227800979));
#93136=CARTESIAN_POINT('Ctrl Pts',(-4.48625483849351,0.621229052817995,
5.85012332937484));
#93137=CARTESIAN_POINT('Ctrl Pts',(-4.39754752286322,0.638561214196987,
5.93867147387761));
#93138=CARTESIAN_POINT('Ctrl Pts',(-4.30665306542352,0.655900535670885,
6.02495660717391));
#93139=CARTESIAN_POINT('',(-4.58989338932486,0.499999998946337,5.61207436485739));
#93140=CARTESIAN_POINT('Origin',(-1.35938332557116,0.00294833923909749,
-0.655457300451683));
#93141=CARTESIAN_POINT('',(-4.85928378406155,0.544769999439475,5.44068290297079));
#93142=CARTESIAN_POINT('Origin',(-0.806680331093372,0.376341480826078,-0.669876452008213));
#93143=CARTESIAN_POINT('',(-5.06346365273142,0.499999999752261,5.18881834708339));
#93144=CARTESIAN_POINT('Ctrl Pts',(-5.06346365249666,0.499999999806884,
5.18881834689219));
#93145=CARTESIAN_POINT('Ctrl Pts',(-5.03039833335715,0.507497225171508,
5.2315602412285));
#93146=CARTESIAN_POINT('Ctrl Pts',(-4.99684448589563,0.514976130594258,
5.27392533114672));
#93147=CARTESIAN_POINT('Ctrl Pts',(-4.92856544338408,0.529941633734565,
5.35814269436226));
#93148=CARTESIAN_POINT('Ctrl Pts',(-4.89392655660566,0.537397123185718,
5.39985668623828));
#93149=CARTESIAN_POINT('Ctrl Pts',(-4.85928378438838,0.544769999813635,
5.44068290318055));
#93150=CARTESIAN_POINT('',(-4.90238970435406,0.552026825426173,5.41166988547225));
#93151=CARTESIAN_POINT('Ctrl Pts',(-4.90238970419515,0.552026824885702,
5.41166988580858));
#93152=CARTESIAN_POINT('Ctrl Pts',(-4.91692413516503,0.547477949104674,
5.39236540742167));
#93153=CARTESIAN_POINT('Ctrl Pts',(-4.93136467531652,0.542929077274359,
5.37298987474318));
#93154=CARTESIAN_POINT('Ctrl Pts',(-4.94571046402211,0.538380664934047,
5.35354468768559));
#93155=CARTESIAN_POINT('Ctrl Pts',(-4.96005627963508,0.533832244062601,
5.33409946415606));
#93156=CARTESIAN_POINT('Ctrl Pts',(-4.97430346254159,0.529279732633635,
5.31458195405456));
#93157=CARTESIAN_POINT('Ctrl Pts',(-4.98843873411042,0.524710849218788,
5.29498790704647));
#93158=CARTESIAN_POINT('Ctrl Pts',(-5.01379620343765,0.516514662786328,
5.25983786103679));
#93159=CARTESIAN_POINT('Ctrl Pts',(-5.03880672912297,0.508277071774748,
5.22444460988968));
#93160=CARTESIAN_POINT('Ctrl Pts',(-5.06346365273142,0.499999999752261,
5.18881834708339));
#93161=CARTESIAN_POINT('',(-5.50115348400725,0.655900535618631,4.95829336454301));
#93162=CARTESIAN_POINT('Ctrl Pts',(-5.50115348400725,0.655900535618631,
4.95829336454301));
#93163=CARTESIAN_POINT('Ctrl Pts',(-5.40535013388253,0.638769108037422,
5.03899760190824));
#93164=CARTESIAN_POINT('Ctrl Pts',(-5.30748534043842,0.621541657225329,
5.11718778708195));
#93165=CARTESIAN_POINT('Ctrl Pts',(-5.10779766963579,0.586905785321977,
5.26839385239524));
#93166=CARTESIAN_POINT('Ctrl Pts',(-5.00601384944893,0.569504150565706,
5.34137992789109));
#93167=CARTESIAN_POINT('Ctrl Pts',(-4.90238970497714,0.552026827062365,
5.41166988679766));
#93168=CARTESIAN_POINT('',(-5.89044286688532,0.552026825461704,4.31535382151131));
#93169=CARTESIAN_POINT('Ctrl Pts',(-5.89044286585037,0.552026825217669,
4.31535382099207));
#93170=CARTESIAN_POINT('Ctrl Pts',(-5.87493109527073,0.556533631547463,
4.34415331790915));
#93171=CARTESIAN_POINT('Ctrl Pts',(-5.86050549286374,0.560675802479242,
4.37051449026906));
#93172=CARTESIAN_POINT('Ctrl Pts',(-5.83028827827681,0.56926322115515,4.4249648568579));
#93173=CARTESIAN_POINT('Ctrl Pts',(-5.81492635134257,0.573581754127954,
4.45224016328351));
#93174=CARTESIAN_POINT('Ctrl Pts',(-5.76824188832753,0.586565893336634,
4.53392222111768));
#93175=CARTESIAN_POINT('Ctrl Pts',(-5.73640398994225,0.59523585365148,4.5880305928689));
#93176=CARTESIAN_POINT('Ctrl Pts',(-5.63897228081956,0.621229052877164,
4.7489385194819));
#93177=CARTESIAN_POINT('Ctrl Pts',(-5.5713741265464,0.638561214252923,4.85448590824627));
#93178=CARTESIAN_POINT('Ctrl Pts',(-5.50115348409217,0.655900535709962,
4.9582933645852));
#93179=CARTESIAN_POINT('',(-5.68901432855912,0.499999998629038,4.49417578248358));
#93180=CARTESIAN_POINT('Origin',(-1.18669842542073,0.00294833247686969,
-0.932359553028809));
#93181=CARTESIAN_POINT('',(-5.91526242791687,0.544769999463201,4.26888038646475));
#93182=CARTESIAN_POINT('Origin',(-0.643817013602778,0.376341765642476,-0.827627435534536));
#93183=CARTESIAN_POINT('',(-6.06052525045423,0.499999999933984,3.97901164806514));
#93184=CARTESIAN_POINT('Ctrl Pts',(-6.06052525004562,0.500000000016535,
3.97901164785921));
#93185=CARTESIAN_POINT('Ctrl Pts',(-6.03742122062618,0.507497226262149,
4.02786233269189));
#93186=CARTESIAN_POINT('Ctrl Pts',(-6.0137590823351,0.514976132581203,4.07645004161787));
#93187=CARTESIAN_POINT('Ctrl Pts',(-5.96518059621994,0.529941639804371,
4.17337645202689));
#93188=CARTESIAN_POINT('Ctrl Pts',(-5.9403188393161,0.53739712403384,4.22156149693423));
#93189=CARTESIAN_POINT('Ctrl Pts',(-5.91526242830641,0.544769999863304,
4.26888038660868));
#93190=CARTESIAN_POINT('',(-5.95112361506895,0.552026825675856,4.23127917814192));
#93191=CARTESIAN_POINT('Ctrl Pts',(-5.95112361521097,0.552026824647466,
4.23127917807872));
#93192=CARTESIAN_POINT('Ctrl Pts',(-5.96116834730158,0.547477948689876,
4.2093015533715));
#93193=CARTESIAN_POINT('Ctrl Pts',(-5.97110610902993,0.54292907688231,4.18727472039419));
#93194=CARTESIAN_POINT('Ctrl Pts',(-5.98093636090419,0.538380664555678,
4.16520023027504));
#93195=CARTESIAN_POINT('Ctrl Pts',(-5.99076663121642,0.533832243697881,
4.14312569875219));
#93196=CARTESIAN_POINT('Ctrl Pts',(-6.0004850352215,0.529279732186206,4.12100177376764));
#93197=CARTESIAN_POINT('Ctrl Pts',(-6.01007769116381,0.524710848712617,
4.09882715890195));
#93198=CARTESIAN_POINT('Ctrl Pts',(-6.02728609557759,0.516514662483712,
4.05904779616615));
#93199=CARTESIAN_POINT('Ctrl Pts',(-6.04410338579749,0.508277071670928,
4.01910549692898));
#93200=CARTESIAN_POINT('Ctrl Pts',(-6.06052525045423,0.499999999933984,
3.97901164806514));
#93201=CARTESIAN_POINT('',(-6.43842607969659,0.655900535543649,3.65978583507949));
#93202=CARTESIAN_POINT('Ctrl Pts',(-6.43842607969659,0.655900535543648,
3.65978583507949));
#93203=CARTESIAN_POINT('Ctrl Pts',(-6.36221158414701,0.63876910796355,3.75919814047178));
#93204=CARTESIAN_POINT('Ctrl Pts',(-6.28344339378497,0.621541657163328,
3.85659832020235));
#93205=CARTESIAN_POINT('Ctrl Pts',(-6.12092914436792,0.586905785291491,
4.04719621800423));
#93206=CARTESIAN_POINT('Ctrl Pts',(-6.03721482183592,0.569504150472652,
4.14035643254888));
#93207=CARTESIAN_POINT('Ctrl Pts',(-5.95112361580156,0.552026826978804,
4.23127917908606));
#93208=CARTESIAN_POINT('',(-6.68040109666531,0.552026825412667,2.94819215069797));
#93209=CARTESIAN_POINT('Ctrl Pts',(-6.68040109566058,0.552026825128316,
2.94819215045262));
#93210=CARTESIAN_POINT('Ctrl Pts',(-6.67144302222964,0.556533631437695,
2.97965290314322));
#93211=CARTESIAN_POINT('Ctrl Pts',(-6.66302155520908,0.560675802374939,
3.00849884408019));
#93212=CARTESIAN_POINT('Ctrl Pts',(-6.64521602158031,0.569263221053295,
3.06817199929897));
#93213=CARTESIAN_POINT('Ctrl Pts',(-6.63607663258483,0.573581754029128,
3.09811198443641));
#93214=CARTESIAN_POINT('Ctrl Pts',(-6.60804285427525,0.58656589325219,3.18792014081814));
#93215=CARTESIAN_POINT('Ctrl Pts',(-6.58858100873347,0.595235853578946,
3.24760769601679));
#93216=CARTESIAN_POINT('Ctrl Pts',(-6.52801764659181,0.621229052843535,
3.42569862232371));
#93217=CARTESIAN_POINT('Ctrl Pts',(-6.48468946820172,0.638561214255091,
3.54330997689522));
#93218=CARTESIAN_POINT('Ctrl Pts',(-6.43842607993088,0.655900535776209,
3.65978583513793));
#93219=CARTESIAN_POINT('',(-6.52212328092484,0.499999998610809,3.16613453548233));
#93220=CARTESIAN_POINT('Origin',(-0.958526833969954,0.00294802284599618,
-1.16566486688198));
#93221=CARTESIAN_POINT('',(-6.69464997525716,0.544769999368522,2.89746976731015));
#93222=CARTESIAN_POINT('Origin',(-0.450850612214941,0.3763418800084,-0.946678874814712));
#93223=CARTESIAN_POINT('',(-6.77420342353812,0.499999999786671,2.58315078520083));
#93224=CARTESIAN_POINT('Ctrl Pts',(-6.77420342316194,0.499999999880416,
2.58315078535635));
#93225=CARTESIAN_POINT('Ctrl Pts',(-6.76214102323053,0.507497215697533,
2.63582597812924));
#93226=CARTESIAN_POINT('Ctrl Pts',(-6.74947703553349,0.514976111417823,
2.68836432144651));
#93227=CARTESIAN_POINT('Ctrl Pts',(-6.72286973356319,0.529942106249854,
2.79347100949626));
#93228=CARTESIAN_POINT('Ctrl Pts',(-6.70894923891358,0.53739670136936,2.84586782142646));
#93229=CARTESIAN_POINT('Ctrl Pts',(-6.69464997581791,0.54476999991391,2.89746976738761));
#93230=CARTESIAN_POINT('',(-6.72158959959758,0.552026825343707,2.85303855926069));
#93231=CARTESIAN_POINT('Ctrl Pts',(-6.72158959957876,0.552026824717549,
2.85303855943171));
#93232=CARTESIAN_POINT('Ctrl Pts',(-6.72667495173065,0.547477948832495,
2.82941543926053));
#93233=CARTESIAN_POINT('Ctrl Pts',(-6.73164525610249,0.542929077003787,
2.80576725640421));
#93234=CARTESIAN_POINT('Ctrl Pts',(-6.73650031926673,0.538380664658224,
2.78209564204453));
#93235=CARTESIAN_POINT('Ctrl Pts',(-6.74135539153724,0.533832243781545,
2.75842398328578));
#93236=CARTESIAN_POINT('Ctrl Pts',(-6.74609059481198,0.529279732319472,
2.73472813380816));
#93237=CARTESIAN_POINT('Ctrl Pts',(-6.7506920930816,0.524710848861558,2.71100981166606));
#93238=CARTESIAN_POINT('Ctrl Pts',(-6.75894678762545,0.516514662501874,
2.66846116926658));
#93239=CARTESIAN_POINT('Ctrl Pts',(-6.76678448543499,0.508277071532466,
2.62583747771786));
#93240=CARTESIAN_POINT('Ctrl Pts',(-6.77420342353812,0.499999999786671,
2.58315078520083));
#93241=CARTESIAN_POINT('',(-7.07464502826342,0.655900535710891,2.19015078679768));
#93242=CARTESIAN_POINT('Ctrl Pts',(-7.07464502826342,0.655900535710891,
2.19015078679768));
#93243=CARTESIAN_POINT('Ctrl Pts',(-7.02158309222455,0.638769108081322,
2.30362275157115));
#93244=CARTESIAN_POINT('Ctrl Pts',(-6.96559461778364,0.621541657221281,
2.41567860194491));
#93245=CARTESIAN_POINT('Ctrl Pts',(-6.84785277504007,0.586905785274964,
2.63675618678576));
#93246=CARTESIAN_POINT('Ctrl Pts',(-6.78612233907849,0.569504150426287,
2.7457344722221));
#93247=CARTESIAN_POINT('Ctrl Pts',(-6.7215896004347,0.5520268269623,2.85303856002776));
#93248=CARTESIAN_POINT('',(-7.15799119607484,0.552026825446138,1.44317629208911));
#93249=CARTESIAN_POINT('Ctrl Pts',(-7.15799119488379,0.55202682520204,1.44317629205038));
#93250=CARTESIAN_POINT('Ctrl Pts',(-7.15600568807706,0.556533631500037,
1.47582723080508));
#93251=CARTESIAN_POINT('Ctrl Pts',(-7.15398213489251,0.560675802423479,
1.5058091360986));
#93252=CARTESIAN_POINT('Ctrl Pts',(-7.14942084918708,0.569263221076987,
1.56791482941623));
#93253=CARTESIAN_POINT('Ctrl Pts',(-7.14693134581205,0.573581754042761,
1.59911953277205));
#93254=CARTESIAN_POINT('Ctrl Pts',(-7.13885908057076,0.586565893249146,
1.6928544579728));
#93255=CARTESIAN_POINT('Ctrl Pts',(-7.13268330218066,0.595235853572959,
1.75533027279036));
#93256=CARTESIAN_POINT('Ctrl Pts',(-7.11182016263718,0.621229052815269,
1.94227686467748));
#93257=CARTESIAN_POINT('Ctrl Pts',(-7.09478793767363,0.638561214209733,
2.06645280858534));
#93258=CARTESIAN_POINT('Ctrl Pts',(-7.07464502823531,0.655900535683804,
2.19015078679689));
#93259=CARTESIAN_POINT('',(-7.05026499842311,0.499999998724005,1.69004835618955));
#93260=CARTESIAN_POINT('Origin',(-0.685531569485398,0.00294801892202427,
-1.34446804942707));
#93261=CARTESIAN_POINT('',(-7.16100313078815,0.544769999536036,1.39057668144311));
#93262=CARTESIAN_POINT('Origin',(-0.236801120050296,0.376341888117048,-1.02146591795983));
#93263=CARTESIAN_POINT('',(-7.17112737311027,0.499999999517536,1.0665046612835));
#93264=CARTESIAN_POINT('Ctrl Pts',(-7.17112737305704,0.499999999527143,
1.06650466128172));
#93265=CARTESIAN_POINT('Ctrl Pts',(-7.17067059482892,0.507497213567971,
1.12054138398888));
#93266=CARTESIAN_POINT('Ctrl Pts',(-7.16959687566357,0.514976107571692,
1.17457378031923));
#93267=CARTESIAN_POINT('Ctrl Pts',(-7.16620657274698,0.529941643310162,
1.28293959095106));
#93268=CARTESIAN_POINT('Ctrl Pts',(-7.16387501996956,0.53739714398625,1.33711045128718));
#93269=CARTESIAN_POINT('Ctrl Pts',(-7.16100313111276,0.544769999849767,
1.39057668141728));
#93270=CARTESIAN_POINT('',(-7.17776152484637,0.55202682540428,1.34139302791087));
#93271=CARTESIAN_POINT('Ctrl Pts',(-7.17776152490766,0.552026824855066,
1.34139302824004));
#93272=CARTESIAN_POINT('Ctrl Pts',(-7.17764971205927,0.547477949014844,
1.31722900355443));
#93273=CARTESIAN_POINT('Ctrl Pts',(-7.17742015316916,0.542929077144782,
1.29306523348913));
#93274=CARTESIAN_POINT('Ctrl Pts',(-7.17707301030228,0.53838066479279,1.26890335318175));
#93275=CARTESIAN_POINT('Ctrl Pts',(-7.1767258667843,0.53383224390963,1.24474142755546));
#93276=CARTESIAN_POINT('Ctrl Pts',(-7.17625645642031,0.529279732411963,
1.22058164507269));
#93277=CARTESIAN_POINT('Ctrl Pts',(-7.17565163607013,0.524710848946523,
1.19642865794178));
#93278=CARTESIAN_POINT('Ctrl Pts',(-7.17456664006963,0.516514662615714,
1.15310026393304));
#93279=CARTESIAN_POINT('Ctrl Pts',(-7.1730582631878,0.508277071721035,1.10978821734395));
#93280=CARTESIAN_POINT('Ctrl Pts',(-7.17112737311027,0.499999999517536,
1.0665046612835));
#93281=CARTESIAN_POINT('',(-7.38006143764124,0.655900535683362,0.618106723046989));
#93282=CARTESIAN_POINT('Ctrl Pts',(-7.38006143764124,0.655900535683362,
0.618106723046988));
#93283=CARTESIAN_POINT('Ctrl Pts',(-7.3526331783707,0.63876910802647,0.740332523974201));
#93284=CARTESIAN_POINT('Ctrl Pts',(-7.32204237884272,0.621541657175023,
0.861804437744292));
#93285=CARTESIAN_POINT('Ctrl Pts',(-7.25457842071691,0.586905785258295,
1.10302436718471));
#93286=CARTESIAN_POINT('Ctrl Pts',(-7.21771831817857,0.569504150488276,
1.22272501946576));
#93287=CARTESIAN_POINT('Ctrl Pts',(-7.17776152609422,0.552026827023669,
1.34139302856953));
#93288=CARTESIAN_POINT('',(-7.30088158247247,0.552026825456915,-0.129320885806511));
#93289=CARTESIAN_POINT('Ctrl Pts',(-7.3008815813318,0.552026825209583,-0.1293208855927));
#93290=CARTESIAN_POINT('Ctrl Pts',(-7.30596148125041,0.556533631510786,
-0.0970064823605118));
#93291=CARTESIAN_POINT('Ctrl Pts',(-7.31043046100619,0.560675802446503,
-0.0672905331523253));
#93292=CARTESIAN_POINT('Ctrl Pts',(-7.31932670386724,0.569263221112411,
-0.00565629475601271));
#93293=CARTESIAN_POINT('Ctrl Pts',(-7.32360349251664,0.573581754082038,
0.0253540296392704));
#93294=CARTESIAN_POINT('Ctrl Pts',(-7.33587019047837,0.586565893288676,
0.118632782797426));
#93295=CARTESIAN_POINT('Ctrl Pts',(-7.34326925176093,0.595235853607951,
0.180975557563082));
#93296=CARTESIAN_POINT('Ctrl Pts',(-7.36308187196685,0.621229052849239,
0.368036400349092));
#93297=CARTESIAN_POINT('Ctrl Pts',(-7.37314200827478,0.638561214247294,
0.492970604652602));
#93298=CARTESIAN_POINT('Ctrl Pts',(-7.38006143769083,0.655900535731995,
0.618106723037508));
#93299=CARTESIAN_POINT('',(-7.24874416021239,0.499999998894538,0.134937395088208));
#93300=CARTESIAN_POINT('Origin',(-0.380481977827258,0.00294817441139524,
-1.46040437774116));
#93301=CARTESIAN_POINT('',(-7.2925157382699,0.544769999418317,-0.181338224043539));
#93302=CARTESIAN_POINT('Origin',(-0.0116792896362683,0.376341641496503,
-1.04848995475632));
#93303=CARTESIAN_POINT('',(-7.23273737687419,0.49999999957512,-0.500010032745376));
#93304=CARTESIAN_POINT('Ctrl Pts',(-7.23273737677256,0.499999999597735,
-0.50001003270372));
#93305=CARTESIAN_POINT('Ctrl Pts',(-7.24390757625351,0.507497213911131,
-0.447138462547856));
#93306=CARTESIAN_POINT('Ctrl Pts',(-7.25447432840697,0.514976108202603,
-0.394138493533089));
#93307=CARTESIAN_POINT('Ctrl Pts',(-7.27445873396409,0.529941643242863,
-0.287577405483172));
#93308=CARTESIAN_POINT('Ctrl Pts',(-7.28382682503527,0.537397143705099,
-0.234171816569637));
#93309=CARTESIAN_POINT('Ctrl Pts',(-7.29251573872258,0.544769999874284,
-0.181338224181616));
#93310=CARTESIAN_POINT('',(-7.29830929881042,0.552026825658063,-0.232974550490544));
#93311=CARTESIAN_POINT('Ctrl Pts',(-7.2983092988398,0.552026824668521,-0.232974550626286));
#93312=CARTESIAN_POINT('Ctrl Pts',(-7.29300554884515,0.547477948674746,
-0.256549598283125));
#93313=CARTESIAN_POINT('Ctrl Pts',(-7.2875868606527,0.542929076835482,-0.280099084445121));
#93314=CARTESIAN_POINT('Ctrl Pts',(-7.28205374376109,0.538380664501388,
-0.303621447946045));
#93315=CARTESIAN_POINT('Ctrl Pts',(-7.27652061649133,0.533832243636109,
-0.327143855566465));
#93316=CARTESIAN_POINT('Ctrl Pts',(-7.27086854156995,0.52927973210616,-0.350637886369769));
#93317=CARTESIAN_POINT('Ctrl Pts',(-7.26508568330685,0.524710848643296,
-0.37409617156336));
#93318=CARTESIAN_POINT('Ctrl Pts',(-7.25471173014415,0.516514662450736,
-0.416178329002402));
#93319=CARTESIAN_POINT('Ctrl Pts',(-7.24392780876621,0.508277071726877,
-0.458153506858803));
#93320=CARTESIAN_POINT('Ctrl Pts',(-7.23273737687419,0.49999999957512,-0.500010032745376));
#93321=CARTESIAN_POINT('',(-7.34039437668371,0.655900535573722,-0.98283932438691));
#93322=CARTESIAN_POINT('Ctrl Pts',(-7.34039437668371,0.655900535573721,
-0.98283932438691));
#93323=CARTESIAN_POINT('Ctrl Pts',(-7.3398823091396,0.638769107974336,-0.857574829919374));
#93324=CARTESIAN_POINT('Ctrl Pts',(-7.3361195763012,0.621541657159446,-0.732366744488661));
#93325=CARTESIAN_POINT('Ctrl Pts',(-7.32208804245887,0.586905785274177,
-0.482283646433133));
#93326=CARTESIAN_POINT('Ctrl Pts',(-7.31182181051129,0.569504150452724,
-0.35745769620365));
#93327=CARTESIAN_POINT('Ctrl Pts',(-7.29830930016154,0.552026826973882,
-0.232974550159142));
#93328=CARTESIAN_POINT('',(-7.10239085947497,0.552026825477796,-1.69577116499436));
#93329=CARTESIAN_POINT('Ctrl Pts',(-7.10239085868817,0.552026824950452,
-1.69577116460884));
#93330=CARTESIAN_POINT('Ctrl Pts',(-7.11430003273687,0.556534160312844,
-1.66530070594601));
#93331=CARTESIAN_POINT('Ctrl Pts',(-7.12505008206614,0.560675371213913,
-1.63724669915386));
#93332=CARTESIAN_POINT('Ctrl Pts',(-7.14698897655328,0.569263221046235,
-1.57896293803046));
#93333=CARTESIAN_POINT('Ctrl Pts',(-7.15783207936236,0.573581754020886,
-1.54959700089359));
#93334=CARTESIAN_POINT('Ctrl Pts',(-7.1898641634356,0.586565893249612,-1.46113603045405));
#93335=CARTESIAN_POINT('Ctrl Pts',(-7.21049209255752,0.595235853584485,
-1.4018413744536));
#93336=CARTESIAN_POINT('Ctrl Pts',(-7.27005405652529,0.621229052855129,
-1.22341303761221));
#93337=CARTESIAN_POINT('Ctrl Pts',(-7.30673615337281,0.638561214263141,
-1.10356235732804));
#93338=CARTESIAN_POINT('Ctrl Pts',(-7.3403943768537,0.655900535751893,-0.982839324459895));
#93339=CARTESIAN_POINT('',(-7.10828010110168,0.499999998819424,-1.4264830890482));
#93340=CARTESIAN_POINT('Origin',(-0.0576434912618817,0.00294819472885649,
-1.50805332165096));
#93341=CARTESIAN_POINT('',(-7.08303841516615,0.544769999432261,-1.74477395495737));
#93342=CARTESIAN_POINT('Origin',(0.213987977808648,0.376341652662118,-1.02648755829279));
#93343=CARTESIAN_POINT('',(-6.95615261946262,0.499999999579506,-2.04314481407824));
#93344=CARTESIAN_POINT('Ctrl Pts',(-6.9561526193664,0.499999999623434,-2.04314481391355));
#93345=CARTESIAN_POINT('Ctrl Pts',(-6.97842749214027,0.507497214509123,
-1.99391061084159));
#93346=CARTESIAN_POINT('Ctrl Pts',(-7.00014062758234,0.514976109292713,
-1.94442128735484));
#93347=CARTESIAN_POINT('Ctrl Pts',(-7.04256660156483,0.529942105956751,
-1.8446445168329));
#93348=CARTESIAN_POINT('Ctrl Pts',(-7.06319378908159,0.537396700077726,
-1.79450746095607));
#93349=CARTESIAN_POINT('Ctrl Pts',(-7.08303841565686,0.544769999974806,
-1.74477395523361));
#93350=CARTESIAN_POINT('',(-7.07759624149658,0.55202682539532,-1.79644849796954));
#93351=CARTESIAN_POINT('Ctrl Pts',(-7.07759624155095,0.552026824779479,
-1.79644849775501));
#93352=CARTESIAN_POINT('Ctrl Pts',(-7.06734855208673,0.547477948772125,
-1.81833222393605));
#93353=CARTESIAN_POINT('Ctrl Pts',(-7.05699410635578,0.542929076886224,
-1.84016627842884));
#93354=CARTESIAN_POINT('Ctrl Pts',(-7.04653373779578,0.53838066452945,-1.8619492456006));
#93355=CARTESIAN_POINT('Ctrl Pts',(-7.03607334961583,0.533832243641466,
-1.88373225362949));
#93356=CARTESIAN_POINT('Ctrl Pts',(-7.02550289495077,0.529279732158083,
-1.90546197808978));
#93357=CARTESIAN_POINT('Ctrl Pts',(-7.01481239879411,0.524710848694791,
-1.92712867807061));
#93358=CARTESIAN_POINT('Ctrl Pts',(-6.99563456268909,0.516514662385204,
-1.96599688540912));
#93359=CARTESIAN_POINT('Ctrl Pts',(-6.97607934059764,0.508277071500689,
-2.00467248320679));
#93360=CARTESIAN_POINT('Ctrl Pts',(-6.95615261946262,0.499999999579506,
-2.04314481407824));
#93361=CARTESIAN_POINT('',(-6.95749863316843,0.655900535537742,-2.53782889725405));
#93362=CARTESIAN_POINT('Ctrl Pts',(-6.95749863316843,0.655900535537741,
-2.53782889725405));
#93363=CARTESIAN_POINT('Ctrl Pts',(-6.98392670096081,0.638769107926578,
-2.4153829377179));
#93364=CARTESIAN_POINT('Ctrl Pts',(-7.00716797595779,0.621541657119776,
-2.29229327145058));
#93365=CARTESIAN_POINT('Ctrl Pts',(-7.0472249652761,0.586905785256709,-2.04504061223377));
#93366=CARTESIAN_POINT('Ctrl Pts',(-7.06403264154237,0.56950415053602,-1.92092608751711));
#93367=CARTESIAN_POINT('Ctrl Pts',(-7.07759624290549,0.55202682706362,-1.79644849788882));
#93368=CARTESIAN_POINT('',(-6.57180023450511,0.552026825547467,-3.18292906702191));
#93369=CARTESIAN_POINT('Ctrl Pts',(-6.57180023370417,0.552026825029646,
-3.18292906640069));
#93370=CARTESIAN_POINT('Ctrl Pts',(-6.58998122584121,0.556534160399563,
-3.1557311104335));
#93371=CARTESIAN_POINT('Ctrl Pts',(-6.60651072723157,0.560675371309851,
-3.13064393347764));
#93372=CARTESIAN_POINT('Ctrl Pts',(-6.64046598836063,0.569263221140471,
-3.07843902805526));
#93373=CARTESIAN_POINT('Ctrl Pts',(-6.65736839388578,0.573581754112593,
-3.05209059678148));
#93374=CARTESIAN_POINT('Ctrl Pts',(-6.70766807935086,0.586565893323852,
-2.97258374591643));
#93375=CARTESIAN_POINT('Ctrl Pts',(-6.74056033721591,0.595235853644447,
-2.91910976107274));
#93376=CARTESIAN_POINT('Ctrl Pts',(-6.83708659364138,0.62122905289433,-2.75765704122748));
#93377=CARTESIAN_POINT('Ctrl Pts',(-6.89868023266326,0.638562584594348,
-2.64848530079444));
#93378=CARTESIAN_POINT('Ctrl Pts',(-6.95750328265113,0.655901906252846,
-2.53782015062894));
#93379=CARTESIAN_POINT('',(-6.6354407643065,0.499999998577759,-2.92120280882441));
#93380=CARTESIAN_POINT('Origin',(0.267888816907871,0.002948723900741,-1.48518799392768));
#93381=CARTESIAN_POINT('',(-6.54236608768061,0.544769999554987,-3.2266259964821));
#93382=CARTESIAN_POINT('Origin',(0.429648088530983,0.376341930995795,-0.956488181367567));
#93383=CARTESIAN_POINT('',(-6.35430589758883,0.499999999782203,-3.49074441377444));
#93384=CARTESIAN_POINT('Ctrl Pts',(-6.35430589746526,0.499999999874871,
-3.4907444133915));
#93385=CARTESIAN_POINT('Ctrl Pts',(-6.38664389820455,0.507497215608088,
-3.44744971264936));
#93386=CARTESIAN_POINT('Ctrl Pts',(-6.41848813786028,0.514976111277326,
-3.40378509899666));
#93387=CARTESIAN_POINT('Ctrl Pts',(-6.48136931942955,0.529941643107535,
-3.31546412729002));
#93388=CARTESIAN_POINT('Ctrl Pts',(-6.51229599592233,0.537397144213602,
-3.27092808317226));
#93389=CARTESIAN_POINT('Ctrl Pts',(-6.54236608792216,0.544769999867112,
-3.226625996698));
#93390=CARTESIAN_POINT('',(-6.52594265037054,0.552026825343033,-3.27592250968595));
#93391=CARTESIAN_POINT('Ctrl Pts',(-6.52594265060015,0.552026824772377,
-3.27592250954095));
#93392=CARTESIAN_POINT('Ctrl Pts',(-6.51123019227503,0.547477948958686,
-3.29509165566118));
#93393=CARTESIAN_POINT('Ctrl Pts',(-6.49642415158775,0.542929077147482,
-3.31418934218825));
#93394=CARTESIAN_POINT('Ctrl Pts',(-6.48152564671875,0.538380664815547,
-3.33321436547128));
#93395=CARTESIAN_POINT('Ctrl Pts',(-6.46662711390579,0.533832243952507,
-3.35223942443808));
#93396=CARTESIAN_POINT('Ctrl Pts',(-6.45163254231022,0.529279732515485,
-3.37118878455419));
#93397=CARTESIAN_POINT('Ctrl Pts',(-6.43653428412055,0.524710849087795,
-3.39005078828863));
#93398=CARTESIAN_POINT('Ctrl Pts',(-6.4094492992381,0.516514662679131,-3.42388761102558));
#93399=CARTESIAN_POINT('Ctrl Pts',(-6.38203715678421,0.508277071679413,
-3.45745520047593));
#93400=CARTESIAN_POINT('Ctrl Pts',(-6.35430589758883,0.499999999782203,
-3.49074441377444));
#93401=CARTESIAN_POINT('',(-6.24927798598832,0.655900535655765,-3.97415241251114));
#93402=CARTESIAN_POINT('Ctrl Pts',(-6.24927798598832,0.655900535655764,
-3.97415241251114));
#93403=CARTESIAN_POINT('Ctrl Pts',(-6.30141044213484,0.638769107998681,
-3.86025042465859));
#93404=CARTESIAN_POINT('Ctrl Pts',(-6.35056898884682,0.621541657147841,
-3.74503471332135));
#93405=CARTESIAN_POINT('Ctrl Pts',(-6.44284148098601,0.586905785248514,
-3.51217375248129));
#93406=CARTESIAN_POINT('Ctrl Pts',(-6.48593715743418,0.569504150382786,
-3.39457410907575));
#93407=CARTESIAN_POINT('Ctrl Pts',(-6.52594265148857,0.552026826911856,
-3.27592250983182));
#93408=CARTESIAN_POINT('',(-5.73391953562396,0.55202682544913,-4.52125674256205));
#93409=CARTESIAN_POINT('Ctrl Pts',(-5.73391953482653,0.552026825209883,
-4.52125674168361));
#93410=CARTESIAN_POINT('Ctrl Pts',(-5.75751945158617,0.556533631513851,
-4.49860569374452));
#93411=CARTESIAN_POINT('Ctrl Pts',(-5.77906050160631,0.560675802441731,
-4.47765354396293));
#93412=CARTESIAN_POINT('Ctrl Pts',(-5.82344219070902,0.569263221097661,
-4.43397073094407));
#93413=CARTESIAN_POINT('Ctrl Pts',(-5.84561356122113,0.573581754061752,
-4.41187182893966));
#93414=CARTESIAN_POINT('Ctrl Pts',(-5.91182889066216,0.586565893258212,
-4.34503674964823));
#93415=CARTESIAN_POINT('Ctrl Pts',(-5.95544747185424,0.595235853573338,
-4.29988382003214));
#93416=CARTESIAN_POINT('Ctrl Pts',(-6.08442456016951,0.621229052798543,
-4.16295606704363));
#93417=CARTESIAN_POINT('Ctrl Pts',(-6.16804687114597,0.638562584486272,
-4.06957751305599));
#93418=CARTESIAN_POINT('Ctrl Pts',(-6.24928440687142,0.655901906135767,
-3.97414486969703));
#93419=CARTESIAN_POINT('',(-5.8523355926758,0.499999998656627,-4.27933033369558));
#93420=CARTESIAN_POINT('Origin',(0.580899441097913,0.00294817653332898,
-1.39287596826395));
#93421=CARTESIAN_POINT('',(-5.6957799933929,0.544769999409456,-4.55760459135602));
#93422=CARTESIAN_POINT('Origin',(0.625220773956524,0.376341599776432,-0.841763888523078));
#93423=CARTESIAN_POINT('',(-5.45533889445124,0.499999999895941,-4.7751206845917));
#93424=CARTESIAN_POINT('Ctrl Pts',(-5.45533889440156,0.500000000015963,
-4.77512068407292));
#93425=CARTESIAN_POINT('Ctrl Pts',(-5.49622793426929,0.507497216227668,
-4.73978990121483));
#93426=CARTESIAN_POINT('Ctrl Pts',(-5.53671427714317,0.514976112406574,
-4.70399170969356));
#93427=CARTESIAN_POINT('Ctrl Pts',(-5.61711421180195,0.529942106266039,
-4.63125098296299));
#93428=CARTESIAN_POINT('Ctrl Pts',(-5.65688694612934,0.537396700836268,
-4.59440895204351));
#93429=CARTESIAN_POINT('Ctrl Pts',(-5.69577999365009,0.5447699998331,-4.55760459171267));
#93430=CARTESIAN_POINT('',(-5.6691432330339,0.552026825689722,-4.60221802656881));
#93431=CARTESIAN_POINT('Ctrl Pts',(-5.66914323294736,0.552026824715417,
-4.60221802667545));
#93432=CARTESIAN_POINT('Ctrl Pts',(-5.65065394335861,0.54747794861729,-4.61777626606602));
#93433=CARTESIAN_POINT('Ctrl Pts',(-5.63208862125364,0.542929076718581,
-4.63324459847705));
#93434=CARTESIAN_POINT('Ctrl Pts',(-5.61344861718722,0.53838066432356,-4.6486220894244));
#93435=CARTESIAN_POINT('Ctrl Pts',(-5.59480857815863,0.533832243397299,
-4.66399960921458));
#93436=CARTESIAN_POINT('Ctrl Pts',(-5.57609101865346,0.529279731820936,
-4.6792825543774));
#93437=CARTESIAN_POINT('Ctrl Pts',(-5.55729097574615,0.524710848291274,
-4.69445789598088));
#93438=CARTESIAN_POINT('Ctrl Pts',(-5.52356530743021,0.516514662183872,
-4.72168116031188));
#93439=CARTESIAN_POINT('Ctrl Pts',(-5.48957800753799,0.508277071515041,
-4.74857115672597));
#93440=CARTESIAN_POINT('Ctrl Pts',(-5.45533889445124,0.499999999895941,
-4.7751206845917));
#93441=CARTESIAN_POINT('',(-5.24884804614103,0.655900535635267,-5.2246489769404));
#93442=CARTESIAN_POINT('Ctrl Pts',(-5.24884804614103,0.655900535635267,
-5.2246489769404));
#93443=CARTESIAN_POINT('Ctrl Pts',(-5.32424723478688,0.638769108036499,
-5.12461689150441));
#93444=CARTESIAN_POINT('Ctrl Pts',(-5.39702445404335,0.621541657221802,
-5.02266249409391));
#93445=CARTESIAN_POINT('Ctrl Pts',(-5.53719788981516,0.58690578531704,-4.81508155141789));
#93446=CARTESIAN_POINT('Ctrl Pts',(-5.60456646001111,0.569504150534648,
-4.70949561946656));
#93447=CARTESIAN_POINT('Ctrl Pts',(-5.66914323445625,0.552026827033793,
-4.60221802720604));
#93448=CARTESIAN_POINT('',(-4.62792713082569,0.552026825464003,-5.64817547903717));
#93449=CARTESIAN_POINT('Ctrl Pts',(-4.62792713032582,0.552026825167876,
-5.64817547814032));
#93450=CARTESIAN_POINT('Ctrl Pts',(-4.65584459965789,0.556533631437719,
-5.63112728375854));
#93451=CARTESIAN_POINT('Ctrl Pts',(-4.68138612466351,0.560675802353204,
-5.61529567266897));
#93452=CARTESIAN_POINT('Ctrl Pts',(-4.73412070799516,0.569263221001596,
-5.58217489085802));
#93453=CARTESIAN_POINT('Ctrl Pts',(-4.76052433490904,0.573581753974147,
-5.56535883816861));
#93454=CARTESIAN_POINT('Ctrl Pts',(-4.83955915331318,0.586565893205448,
-5.51432066433269));
#93455=CARTESIAN_POINT('Ctrl Pts',(-4.89186450159291,0.595235853547021,
-5.47960009065209));
#93456=CARTESIAN_POINT('Ctrl Pts',(-5.0472615968587,0.621229052835566,-5.37359989373892));
#93457=CARTESIAN_POINT('Ctrl Pts',(-5.14899450119751,0.638561214261278,
-5.3003866574176));
#93458=CARTESIAN_POINT('Ctrl Pts',(-5.24884804621161,0.655900535773218,
-5.22464897706503));
#93459=CARTESIAN_POINT('',(-4.79558171331894,0.499999998635506,-5.43736112658256));
#93460=CARTESIAN_POINT('Origin',(0.86674356849252,0.0029485729091093,-1.23543653251669));
#93461=CARTESIAN_POINT('',(-4.58286555743328,0.544769999438325,-5.67547466095984));
#93462=CARTESIAN_POINT('Origin',(0.791557319693054,0.376341880383263,-0.687680335770907));
#93463=CARTESIAN_POINT('',(-4.30128630597295,0.499999999668149,-5.8362176204432));
#93464=CARTESIAN_POINT('Ctrl Pts',(-4.3012863060072,0.499999999733392,-5.83621762016198));
#93465=CARTESIAN_POINT('Ctrl Pts',(-4.34881445038693,0.507497215062244,
-5.81050278990619));
#93466=CARTESIAN_POINT('Ctrl Pts',(-4.39604979182165,0.514976110280007,
-5.78424491097689));
#93467=CARTESIAN_POINT('Ctrl Pts',(-4.49020422802782,0.529941643423082,
-5.73049008633081));
#93468=CARTESIAN_POINT('Ctrl Pts',(-4.53697271591002,0.537397143969364,
-5.70305604352401));
#93469=CARTESIAN_POINT('Ctrl Pts',(-4.58286555763755,0.544769999934216,
-5.67547466143228));
#93470=CARTESIAN_POINT('',(-4.54726098010409,0.552026825712293,-5.71331894285122));
#93471=CARTESIAN_POINT('Ctrl Pts',(-4.54726098003085,0.552026824734663,
-5.71331894296981));
#93472=CARTESIAN_POINT('Ctrl Pts',(-4.52585939887053,0.547477948879278,
-5.72453878810256));
#93473=CARTESIAN_POINT('Ctrl Pts',(-4.5044028899783,0.542929077117612,-5.73565448379864));
#93474=CARTESIAN_POINT('Ctrl Pts',(-4.48289297336656,0.538380664817293,
-5.74666540740134));
#93475=CARTESIAN_POINT('Ctrl Pts',(-4.4613830164101,0.533832243985818,-5.75767635165651));
#93476=CARTESIAN_POINT('Ctrl Pts',(-4.43981768212375,0.529279732533536,
-5.76857826781063));
#93477=CARTESIAN_POINT('Ctrl Pts',(-4.41819492443471,0.524710849116548,
-5.77935736461706));
#93478=CARTESIAN_POINT('Ctrl Pts',(-4.37940554536671,0.516514662796208,
-5.79869414293404));
#93479=CARTESIAN_POINT('Ctrl Pts',(-4.34043229426036,0.508277071898963,
-5.81764920186379));
#93480=CARTESIAN_POINT('Ctrl Pts',(-4.30128630597295,0.499999999668149,
-5.8362176204432));
#93481=CARTESIAN_POINT('',(-4.00298780534354,0.655900535589649,-6.23084676214381));
#93482=CARTESIAN_POINT('Ctrl Pts',(-4.00298780534354,0.655900535589649,
-6.23084676214381));
#93483=CARTESIAN_POINT('Ctrl Pts',(-4.09812814433568,0.63876910799483,-6.14936196802781));
#93484=CARTESIAN_POINT('Ctrl Pts',(-4.19112105437463,0.621541657181549,
-6.06543615860511));
#93485=CARTESIAN_POINT('Ctrl Pts',(-4.37264107972524,0.586905785291398,
-5.89284148821998));
#93486=CARTESIAN_POINT('Ctrl Pts',(-4.46113246462634,0.569504150480316,
-5.80420634770189));
#93487=CARTESIAN_POINT('Ctrl Pts',(-4.54726098115828,0.552026826991961,
-5.71331894360413));
#93488=CARTESIAN_POINT('',(-3.30553799692616,0.552026825425635,-6.51099180780492));
#93489=CARTESIAN_POINT('Ctrl Pts',(-3.30553799661828,0.552026825151617,
-6.51099180679462));
#93490=CARTESIAN_POINT('Ctrl Pts',(-3.33646762905524,0.556533631448746,
-6.50034362033982));
#93491=CARTESIAN_POINT('Ctrl Pts',(-3.36481533595166,0.560675802386594,
-6.49037281634335));
#93492=CARTESIAN_POINT('Ctrl Pts',(-3.42343700322561,0.569263221057426,
-6.46936275654394));
#93493=CARTESIAN_POINT('Ctrl Pts',(-3.4528382822726,0.573581754030701,-6.45861585311779));
#93494=CARTESIAN_POINT('Ctrl Pts',(-3.54099700923227,0.586565893258024,
-6.42576107312447));
#93495=CARTESIAN_POINT('Ctrl Pts',(-3.5995433845281,0.595235853593481,-6.40309635090712));
#93496=CARTESIAN_POINT('Ctrl Pts',(-3.7740942910582,0.621229052873939,-6.3329801616529));
#93497=CARTESIAN_POINT('Ctrl Pts',(-3.88918741828664,0.638561214300223,
-6.28334817732656));
#93498=CARTESIAN_POINT('Ctrl Pts',(-4.00298780541949,0.655900535838296,
-6.23084676239056));
#93499=CARTESIAN_POINT('',(-3.51459176321357,0.499999998556402,-6.34114695680857));
#93500=CARTESIAN_POINT('Origin',(1.11206245074807,0.0029480682560324,-1.02022796045556));
#93501=CARTESIAN_POINT('',(-3.25566142038069,0.544769999525692,-6.52796584410679));
#93502=CARTESIAN_POINT('Origin',(0.920882297147526,0.376341845396332,-0.501441043894132));
#93503=CARTESIAN_POINT('',(-2.94611035073431,0.499999999616658,-6.62441950656243));
#93504=CARTESIAN_POINT('Ctrl Pts',(-2.94611035081038,0.499999999669515,
-6.62441950634589));
#93505=CARTESIAN_POINT('Ctrl Pts',(-2.99805524028318,0.507497214728035,
-6.60952302110954));
#93506=CARTESIAN_POINT('Ctrl Pts',(-3.04983091180412,0.514976109662867,
-6.59403323946265));
#93507=CARTESIAN_POINT('Ctrl Pts',(-3.15333976933434,0.529941642974774,
-6.56177559288136));
#93508=CARTESIAN_POINT('Ctrl Pts',(-3.20491234608337,0.537397143866723,
-6.54503678468685));
#93509=CARTESIAN_POINT('Ctrl Pts',(-3.25566142044168,0.544769999834553,
-6.52796584442151));
#93510=CARTESIAN_POINT('',(-3.21275385699847,0.552026825371849,-6.55727141543876));
#93511=CARTESIAN_POINT('Ctrl Pts',(-3.21275385729611,0.552026824836102,
-6.55727141537468));
#93512=CARTESIAN_POINT('Ctrl Pts',(-3.18944069859206,0.547477949075286,
-6.56362823961408));
#93513=CARTESIAN_POINT('Ctrl Pts',(-3.16609628497767,0.542929077270821,
-6.56987154130488));
#93514=CARTESIAN_POINT('Ctrl Pts',(-3.1427222351911,0.538380664940049,-6.57600103934811));
#93515=CARTESIAN_POINT('Ctrl Pts',(-3.11934814156362,0.533832244078171,
-6.58213054888797));
#93516=CARTESIAN_POINT('Ctrl Pts',(-3.09594340312024,0.529279732637972,
-6.5881416748998));
#93517=CARTESIAN_POINT('Ctrl Pts',(-3.0725089863305,0.524710849234664,-6.59402050867988));
#93518=CARTESIAN_POINT('Ctrl Pts',(-3.03046964479739,0.516514662764997,
-6.60456663420605));
#93519=CARTESIAN_POINT('Ctrl Pts',(-2.98833278843496,0.508277071749586,
-6.6147004376975));
#93520=CARTESIAN_POINT('Ctrl Pts',(-2.94611035073431,0.499999999616658,
-6.62441950656243));
#93521=CARTESIAN_POINT('',(-2.56995230272842,0.655900535691932,-6.94569707849852));
#93522=CARTESIAN_POINT('Ctrl Pts',(-2.56994356813194,0.65590189068777,-6.94570175512237));
#93523=CARTESIAN_POINT('Ctrl Pts',(-2.68037640112295,0.638770463049698,
-6.88657439066599));
#93524=CARTESIAN_POINT('Ctrl Pts',(-2.78924549159031,0.621541657200288,
-6.82459677010367));
#93525=CARTESIAN_POINT('Ctrl Pts',(-3.00362443206904,0.586905785275581,
-6.69505870685461));
#93526=CARTESIAN_POINT('Ctrl Pts',(-3.10910087303173,0.569504150420659,
-6.62751883845557));
#93527=CARTESIAN_POINT('Ctrl Pts',(-3.21275385797399,0.552026826943697,
-6.5572714164871));
#93528=CARTESIAN_POINT('',(-1.8285855811266,0.552026825425414,-7.06936139573953));
#93529=CARTESIAN_POINT('Ctrl Pts',(-1.82858558103768,0.552026825163243,
-7.06936139465403));
#93530=CARTESIAN_POINT('Ctrl Pts',(-1.86108114124179,0.556533631476899,
-7.06561111358071));
#93531=CARTESIAN_POINT('Ctrl Pts',(-1.8909095225058,0.560675802405676,-7.06196734049061));
#93532=CARTESIAN_POINT('Ctrl Pts',(-1.9526771894402,0.569263221073273,-7.05405040986236));
#93533=CARTESIAN_POINT('Ctrl Pts',(-1.98370134940776,0.573581754044103,
-7.04987516898144));
#93534=CARTESIAN_POINT('Ctrl Pts',(-2.07686178061951,0.586565893263386,
-7.03674003587851));
#93535=CARTESIAN_POINT('Ctrl Pts',(-2.13891161936245,0.595235853592223,
-7.02719094237657));
#93536=CARTESIAN_POINT('Ctrl Pts',(-2.32445453032465,0.621229052843979,
-6.996237315988));
#93537=CARTESIAN_POINT('Ctrl Pts',(-2.4475262534217,0.638561214240612,-6.97250732017752));
#93538=CARTESIAN_POINT('Ctrl Pts',(-2.56995230273162,0.655900535729553,
-6.94569707853746));
#93539=CARTESIAN_POINT('',(-2.06926340708605,0.499999998689052,-6.94842780378674));
#93540=CARTESIAN_POINT('Origin',(1.30538195718773,0.00294813417282574,-0.757314928844572));
#93541=CARTESIAN_POINT('',(-1.77622617508296,0.544769999508108,-7.0752165988522));
#93542=CARTESIAN_POINT('Origin',(1.00714758409605,0.376341924620739,-0.291755136603755));
#93543=CARTESIAN_POINT('',(-1.45317754992019,0.499999999562998,-7.10287089873148));
#93544=CARTESIAN_POINT('Ctrl Pts',(-1.453177549962,0.499999999591156,-7.10287089861264));
#93545=CARTESIAN_POINT('Ctrl Pts',(-1.50711029708834,0.50749721411147,-7.09948930088892));
#93546=CARTESIAN_POINT('Ctrl Pts',(-1.56100532369139,0.514976108586445,
-7.09549190108463));
#93547=CARTESIAN_POINT('Ctrl Pts',(-1.66903199485859,0.529942106372944,
-7.08623947785291));
#93548=CARTESIAN_POINT('Ctrl Pts',(-1.722990644337,0.537396701470885,-7.0809792252342));
#93549=CARTESIAN_POINT('Ctrl Pts',(-1.7762261750738,0.544769999857778,-7.07521659921502));
#93550=CARTESIAN_POINT('',(-1.72802193438852,0.552026825864411,-7.09461316486523));
#93551=CARTESIAN_POINT('Ctrl Pts',(-1.72802193417285,0.552026824670133,
-7.0946131647742));
#93552=CARTESIAN_POINT('Ctrl Pts',(-1.7038872937459,0.547477948670733,-7.09580972983484));
#93553=CARTESIAN_POINT('Ctrl Pts',(-1.67974653386692,0.542929076807001,
-7.09688870775154));
#93554=CARTESIAN_POINT('Ctrl Pts',(-1.65560129511354,0.538380664413428,
-7.09785017177835));
#93555=CARTESIAN_POINT('Ctrl Pts',(-1.63145601107289,0.533832243488767,
-7.09881163760849));
#93556=CARTESIAN_POINT('Ctrl Pts',(-1.60730624762677,0.529279732034816,
-7.0996508999705));
#93557=CARTESIAN_POINT('Ctrl Pts',(-1.58315593862026,0.524710848592855,
-7.10035458302231));
#93558=CARTESIAN_POINT('Ctrl Pts',(-1.53983234963671,0.516514662436402,
-7.10161693023715));
#93559=CARTESIAN_POINT('Ctrl Pts',(-1.49650216271934,0.508277071708823,
-7.10245563246828));
#93560=CARTESIAN_POINT('Ctrl Pts',(-1.45317754992019,0.499999999562998,
-7.10287089873148));
#93561=CARTESIAN_POINT('',(-1.01674868797125,0.655900535661223,-7.33577431833995));
#93562=CARTESIAN_POINT('Ctrl Pts',(-1.01674868797125,0.655900535661222,
-7.33577431833995));
#93563=CARTESIAN_POINT('Ctrl Pts',(-1.1373102980958,0.638769108040252,-7.30176911356082));
#93564=CARTESIAN_POINT('Ctrl Pts',(-1.25694791022009,0.621541657216736,
-7.26464682128884));
#93565=CARTESIAN_POINT('Ctrl Pts',(-1.49416164478959,0.586905785305847,
-7.18422242117417));
#93566=CARTESIAN_POINT('Ctrl Pts',(-1.61169117978909,0.569504150566262,
-7.14093591456739));
#93567=CARTESIAN_POINT('Ctrl Pts',(-1.72802193502821,0.55202682707541,-7.09461316601479));
#93568=CARTESIAN_POINT('',(-0.266130534258616,0.552026825448126,-7.29717550202562));
#93569=CARTESIAN_POINT('Ctrl Pts',(-0.266130534397895,0.552026825135067,
-7.29717550108625));
#93570=CARTESIAN_POINT('Ctrl Pts',(-0.298672565884604,0.556533631418656,
-7.30049848436175));
#93571=CARTESIAN_POINT('Ctrl Pts',(-0.328586879728604,0.560675802348281,
-7.30335212091617));
#93572=CARTESIAN_POINT('Ctrl Pts',(-0.390612359103792,0.569263221019371,
-7.30889850628478));
#93573=CARTESIAN_POINT('Ctrl Pts',(-0.421808744919157,0.57358175399926,
-7.31149015754806));
#93574=CARTESIAN_POINT('Ctrl Pts',(-0.515614802533565,0.586565893231015,
-7.31868885547649));
#93575=CARTESIAN_POINT('Ctrl Pts',(-0.578266723431897,0.59523585356534,
-7.32270189562898));
#93576=CARTESIAN_POINT('Ctrl Pts',(-0.766125859322722,0.621229052856937,
-7.33235818909006));
#93577=CARTESIAN_POINT('Ctrl Pts',(-0.891421481876299,0.638561214284284,
-7.33563976988323));
#93578=CARTESIAN_POINT('Ctrl Pts',(-1.01674868795464,0.655900535780308,
-7.33577431846248));
#93579=CARTESIAN_POINT('',(-0.527178595390885,0.499999998624239,-7.23080788849307));
#93580=CARTESIAN_POINT('Origin',(1.43766293562731,0.00294815640760344,-0.458991651664984));
#93581=CARTESIAN_POINT('',(-0.213736567552909,0.544769999381455,-7.29163808917903));
#93582=CARTESIAN_POINT('Origin',(1.04631978522547,0.376341808593957,-0.0684270503981665));
#93583=CARTESIAN_POINT('',(-1.6931015459671E-12,0.515079044621721,-7.26507904462173));
#93584=CARTESIAN_POINT('Ctrl Pts',(-0.21373656742832,0.544769999882563,
-7.29163808968401));
#93585=CARTESIAN_POINT('Ctrl Pts',(-0.1531484544219,0.536377426449655,-7.2850179040679));
#93586=CARTESIAN_POINT('Ctrl Pts',(-0.0921392149746007,0.527925589541755,
-7.27759928397786));
#93587=CARTESIAN_POINT('Ctrl Pts',(-0.0206282398277339,0.517957822703902,
-7.26793586550817));
#93588=CARTESIAN_POINT('Ctrl Pts',(-0.0103124763152848,0.516518781586931,
-7.26651878158693));
#93589=CARTESIAN_POINT('Ctrl Pts',(-3.38786891177452E-12,0.515079044621721,
-7.26507904462173));
#93590=CARTESIAN_POINT('',(1.70500103440517E-15,-3.33066907387547E-15,-6.75));
#93591=CARTESIAN_POINT('',(1.70500103440517E-15,0.,-6.75000000000001));
#93592=CARTESIAN_POINT('Origin',(0.,0.,0.));
#93593=CARTESIAN_POINT('',(0.107704216070514,0.499999999886364,-7.24919994256545));
#93594=CARTESIAN_POINT('Ctrl Pts',(-3.38786891177452E-12,0.515079044621721,
-7.26507904462173));
#93595=CARTESIAN_POINT('Ctrl Pts',(0.0359424207011893,0.510061080929743,
-7.26006108092977));
#93596=CARTESIAN_POINT('Ctrl Pts',(0.0718449099581247,0.505034664458654,
-7.25476793811845));
#93597=CARTESIAN_POINT('Ctrl Pts',(0.107704215711866,0.500000000004417,
-7.24919994219928));
#93598=CARTESIAN_POINT('Ctrl Pts',(0.107704215939162,0.499999999815039,
-7.2491999420065));
#93599=CARTESIAN_POINT('Ctrl Pts',(0.089612700297626,0.503531634900662,
-7.25300075962746));
#93600=CARTESIAN_POINT('Ctrl Pts',(0.0715042823655147,0.507055955084127,
-7.25672637957618));
#93601=CARTESIAN_POINT('Ctrl Pts',(0.0356018297225805,0.514022459397225,
-7.2639570313917));
#93602=CARTESIAN_POINT('Ctrl Pts',(0.0178086383737658,0.517464881394668,
-7.26746488139467));
#93603=CARTESIAN_POINT('Ctrl Pts',(3.97374700519909E-12,0.520900163746503,
-7.27090016374651));
#93604=CARTESIAN_POINT('Origin',(-1.99005104861445E-16,1.2,0.));
#93605=CARTESIAN_POINT('',(-3.25,1.2,-3.9801020972289E-16));
#93606=CARTESIAN_POINT('Origin',(-1.99005104861445E-16,1.2,0.));
#93607=CARTESIAN_POINT('',(-3.25,-2.77555756156289E-16,-3.9801020972289E-16));
#93608=CARTESIAN_POINT('',(-3.25,1.2,-3.9801020972289E-16));
#93609=CARTESIAN_POINT('Origin',(-7.89088642168964E-17,0.,0.));
#93610=CARTESIAN_POINT('Origin',(2.53163762382963E-15,0.,-3.4647252052902E-15));
#93611=CARTESIAN_POINT('',(-0.162489628597199,0.552026825816562,-7.30021868724729));
#93612=CARTESIAN_POINT('Ctrl Pts',(3.97374700519909E-12,0.520900163746503,
-7.27090016374651));
#93613=CARTESIAN_POINT('Ctrl Pts',(-0.00482179263778413,0.521830286466864,
-7.27183028646687));
#93614=CARTESIAN_POINT('Ctrl Pts',(-0.00964471767961773,0.522759885796396,
-7.27275508934469));
#93615=CARTESIAN_POINT('Ctrl Pts',(-0.0642175574728398,0.53327019661184,
-7.28315686485796));
#93616=CARTESIAN_POINT('Ctrl Pts',(-0.114535467221313,0.54287200381573,
-7.29212897072435));
#93617=CARTESIAN_POINT('Ctrl Pts',(-0.162489634298702,0.552026826,-7.30021868757157));
#93618=CARTESIAN_POINT('Ctrl Pts',(-0.162489633664295,0.552026826,-7.30021868758569));
#93619=CARTESIAN_POINT('Ctrl Pts',(-0.108422033090161,0.559674024978565,
-7.30907122741516));
#93620=CARTESIAN_POINT('Ctrl Pts',(-0.0542552256312394,0.567306736081167,
-7.31730673607856));
#93621=CARTESIAN_POINT('Ctrl Pts',(-3.52635867725153E-10,0.574924266631643,
-7.32492426663165));
#93622=CARTESIAN_POINT('Origin',(-4.28626379701574E-16,3.7,0.));
#93623=CARTESIAN_POINT('',(-1.28587913910472E-15,3.7,7.));
#93624=CARTESIAN_POINT('Origin',(-4.28626379701574E-16,3.7,0.));
#93625=CARTESIAN_POINT('',(-1.28587913910472E-15,1.2,7.));
#93626=CARTESIAN_POINT('',(-1.28587913910472E-15,3.7,7.));
#93627=CARTESIAN_POINT('Origin',(-4.28626379701574E-16,1.2,0.));
#93628=CARTESIAN_POINT('Origin',(-3.75048082238878E-16,5.2,0.));
#93629=CARTESIAN_POINT('',(6.125,5.2,7.68465866464964E-16));
#93630=CARTESIAN_POINT('',(-6.125,5.2,-7.50096164477754E-16));
#93631=CARTESIAN_POINT('Origin',(0.,5.2,0.));
#93632=CARTESIAN_POINT('',(-6.125,3.7,-7.50096164477754E-16));
#93633=CARTESIAN_POINT('',(-6.125,5.2,-7.50096164477754E-16));
#93634=CARTESIAN_POINT('Origin',(-5.87463201746242E-16,3.7,0.));
#93635=CARTESIAN_POINT('Origin',(0.,5.2,0.));
#93636=CARTESIAN_POINT('Origin',(-3.75048082238878E-16,5.2,0.));
#93637=CARTESIAN_POINT('',(6.425,5.5,-7.86835568452174E-16));
#93638=CARTESIAN_POINT('',(6.125,5.2,-7.50096164477754E-16));
#93639=CARTESIAN_POINT('Origin',(0.,5.5,0.));
#93640=CARTESIAN_POINT('Origin',(-9.54665999398665E-15,5.5,-2.76142397078324E-15));
#93641=CARTESIAN_POINT('',(-0.213736565703542,4.95523000035635,-7.29163808949555));
#93642=CARTESIAN_POINT('',(0.107704216070517,5.00000000011364,-7.24919994256545));
#93643=CARTESIAN_POINT('Ctrl Pts',(-0.213736565699183,4.95523000035695,
-7.29163808949507));
#93644=CARTESIAN_POINT('Ctrl Pts',(-0.152772191073571,4.9636746929782,-7.28497679148068));
#93645=CARTESIAN_POINT('Ctrl Pts',(-0.0913875379650499,4.97217869295328,
-7.27750760769982));
#93646=CARTESIAN_POINT('Ctrl Pts',(0.016083985202725,4.98715979332583,-7.26296732930841));
#93647=CARTESIAN_POINT('Ctrl Pts',(0.0619292881126885,4.99357317727733,
-7.256307570323));
#93648=CARTESIAN_POINT('Ctrl Pts',(0.107704215711865,4.99999999999558,-7.24919994219928));
#93649=CARTESIAN_POINT('',(-0.5271785952156,5.00000000119539,-7.23080788868627));
#93650=CARTESIAN_POINT('Origin',(1.04631978098754,5.12365820970434,-0.0684270868039383));
#93651=CARTESIAN_POINT('',(-0.266130538254917,4.94797317376359,-7.29717550201765));
#93652=CARTESIAN_POINT('Origin',(1.43766416616257,5.4970519860903,-0.458987126402098));
#93653=CARTESIAN_POINT('',(-1.01674868753842,4.84409946427727,-7.33577431846203));
#93654=CARTESIAN_POINT('Ctrl Pts',(-1.01674868753842,4.84409946427728,-7.33577431846203));
#93655=CARTESIAN_POINT('Ctrl Pts',(-0.891421482506232,4.86143878562856,
-7.33563976987693));
#93656=CARTESIAN_POINT('Ctrl Pts',(-0.76612586099832,4.87877094691128,-7.33235818913045));
#93657=CARTESIAN_POINT('Ctrl Pts',(-0.578266726672991,4.90476414598618,
-7.32270189581848));
#93658=CARTESIAN_POINT('Ctrl Pts',(-0.515614806296964,4.91343410624817,
-7.31868885572902));
#93659=CARTESIAN_POINT('Ctrl Pts',(-0.421808749462441,4.92641824537184,
-7.31149015791479));
#93660=CARTESIAN_POINT('Ctrl Pts',(-0.39061236390569,4.93073677831587,-7.30889850669274));
#93661=CARTESIAN_POINT('Ctrl Pts',(-0.328583770897313,4.9393246280689,-7.3033518429423));
#93662=CARTESIAN_POINT('Ctrl Pts',(-0.2986763903816,4.94346583891753,-7.30049887487933));
#93663=CARTESIAN_POINT('Ctrl Pts',(-0.266130538384521,4.94797317431282,
-7.29717550149333));
#93664=CARTESIAN_POINT('',(-1.7280219382183,4.94797317381307,-7.09461316422209));
#93665=CARTESIAN_POINT('Ctrl Pts',(-1.72802193844647,4.94797317343814,-7.09461316465364));
#93666=CARTESIAN_POINT('Ctrl Pts',(-1.61169118369406,4.9304958500154,-7.14093591308127));
#93667=CARTESIAN_POINT('Ctrl Pts',(-1.4941616457248,4.91309421483262,-7.18422242082973));
#93668=CARTESIAN_POINT('Ctrl Pts',(-1.25694791103012,4.87845834289962,-7.26464682104157));
#93669=CARTESIAN_POINT('Ctrl Pts',(-1.1373102982891,4.86123089198667,-7.30176911351439));
#93670=CARTESIAN_POINT('Ctrl Pts',(-1.01674868753842,4.84409946427728,-7.33577431846203));
#93671=CARTESIAN_POINT('',(-1.45317754970485,5.00000000046694,-7.10287089874499));
#93672=CARTESIAN_POINT('Ctrl Pts',(-1.45317754970711,5.00000000048678,-7.10287089858523));
#93673=CARTESIAN_POINT('Ctrl Pts',(-1.49899199588298,4.99124725113094,-7.10243176744319));
#93674=CARTESIAN_POINT('Ctrl Pts',(-1.54480889124354,4.98253937036453,-7.10151921695448));
#93675=CARTESIAN_POINT('Ctrl Pts',(-1.63675210786151,4.96515485125473,-7.09873687841323));
#93676=CARTESIAN_POINT('Ctrl Pts',(-1.68349106311083,4.95636631499385,-7.09682095024594));
#93677=CARTESIAN_POINT('Ctrl Pts',(-1.72802193834098,4.94797317467986,-7.09461316340132));
#93678=CARTESIAN_POINT('',(-1.77622617387013,4.95523000030894,-7.07521659934531));
#93679=CARTESIAN_POINT('Ctrl Pts',(-1.77622617387013,4.95523000030894,-7.07521659934532));
#93680=CARTESIAN_POINT('Ctrl Pts',(-1.72299384371354,4.96260285540458,-7.08097887890016));
#93681=CARTESIAN_POINT('Ctrl Pts',(-1.66902865274438,4.97005835664292,-7.08623976410856));
#93682=CARTESIAN_POINT('Ctrl Pts',(-1.56100532539457,4.9850238911777,-7.09549190093333));
#93683=CARTESIAN_POINT('Ctrl Pts',(-1.50711029785297,4.99250278578221,-7.09948930084237));
#93684=CARTESIAN_POINT('Ctrl Pts',(-1.45317754977974,5.00000000043418,-7.10287089862406));
#93685=CARTESIAN_POINT('',(-2.06926340799607,5.00000000131937,-6.94842780350358));
#93686=CARTESIAN_POINT('Origin',(1.00714768739185,5.12365815569165,-0.291754918966577));
#93687=CARTESIAN_POINT('',(-1.82858558437265,4.94797317379205,-7.06936139493043));
#93688=CARTESIAN_POINT('Origin',(1.3053840183489,5.49705199769362,-0.757310959927074));
#93689=CARTESIAN_POINT('',(-2.56995230260316,4.84409946428864,-6.94569707856559));
#93690=CARTESIAN_POINT('Ctrl Pts',(-2.56995230260316,4.84409946428864,-6.94569707856559));
#93691=CARTESIAN_POINT('Ctrl Pts',(-2.44752625408122,4.86143878566591,-6.97250732003083));
#93692=CARTESIAN_POINT('Ctrl Pts',(-2.32445453178037,4.87877094695098,-6.99623731570619));
#93693=CARTESIAN_POINT('Ctrl Pts',(-2.13891162202374,4.90476414603551,-7.0271909419521));
#93694=CARTESIAN_POINT('Ctrl Pts',(-2.07686178368571,4.91343410630846,-7.03674003541638));
#93695=CARTESIAN_POINT('Ctrl Pts',(-1.98370135308225,4.92641824544418,-7.04987516847821));
#93696=CARTESIAN_POINT('Ctrl Pts',(-1.9526771933166,4.93073677838734,-7.0540504093481));
#93697=CARTESIAN_POINT('Ctrl Pts',(-1.89090642570761,4.93932462813562,-7.06196773743291));
#93698=CARTESIAN_POINT('Ctrl Pts',(-1.86108495939093,4.9434658389819,-7.06561067291908));
#93699=CARTESIAN_POINT('Ctrl Pts',(-1.82858558437693,4.94797317437364,-7.06936139426864));
#93700=CARTESIAN_POINT('',(-3.21275385990511,4.9479731738326,-6.55727141456418));
#93701=CARTESIAN_POINT('Ctrl Pts',(-3.21275386023597,4.9479731734377,-6.55727141495412));
#93702=CARTESIAN_POINT('Ctrl Pts',(-3.10910087559271,4.93049585000559,-6.62751883677731));
#93703=CARTESIAN_POINT('Ctrl Pts',(-3.00362443262307,4.91309421481583,-6.69505870649984));
#93704=CARTESIAN_POINT('Ctrl Pts',(-2.78924549212175,4.87845834288368,-6.82459676980254));
#93705=CARTESIAN_POINT('Ctrl Pts',(-2.68038513592731,4.86123089197814,-6.88656971393363));
#93706=CARTESIAN_POINT('Ctrl Pts',(-2.56995230260316,4.84409946428864,-6.94569707856559));
#93707=CARTESIAN_POINT('',(-2.94611035073431,5.00000000038334,-6.62441950656244));
#93708=CARTESIAN_POINT('Ctrl Pts',(-2.94611035068246,5.00000000041537,-6.62441950630989));
#93709=CARTESIAN_POINT('Ctrl Pts',(-2.99075928957681,4.99124724929563,-6.61414188797));
#93710=CARTESIAN_POINT('Ctrl Pts',(-3.03530883451336,4.9825393695754,-6.60340139544388));
#93711=CARTESIAN_POINT('Ctrl Pts',(-3.12450434638238,4.96515485090219,-6.5809190335638));
#93712=CARTESIAN_POINT('Ctrl Pts',(-3.16973870290945,4.95636631460213,-6.56900040494851));
#93713=CARTESIAN_POINT('Ctrl Pts',(-3.21275385984555,4.94797317473687,-6.55727141369868));
#93714=CARTESIAN_POINT('',(-3.25566141942808,4.95523000031271,-6.52796584476247));
#93715=CARTESIAN_POINT('Ctrl Pts',(-3.25566141942808,4.95523000031271,-6.52796584476247));
#93716=CARTESIAN_POINT('Ctrl Pts',(-3.20491234522498,4.96260285625755,-6.54503678496748));
#93717=CARTESIAN_POINT('Ctrl Pts',(-3.15333976865463,4.97005835712355,-6.56177559309746));
#93718=CARTESIAN_POINT('Ctrl Pts',(-3.04983091146342,4.98502389038635,-6.59403323956458));
#93719=CARTESIAN_POINT('Ctrl Pts',(-2.99805524011227,4.99250278529663,-6.60952302115855));
#93720=CARTESIAN_POINT('Ctrl Pts',(-2.94611035081039,5.00000000033048,-6.62441950634589));
#93721=CARTESIAN_POINT('',(-3.51459176313735,5.00000000126224,-6.34114695705619));
#93722=CARTESIAN_POINT('Origin',(0.920882278249773,5.12365817302287,-0.50144107485158));
#93723=CARTESIAN_POINT('',(-3.30553800089752,4.94797317379562,-6.51099180615017));
#93724=CARTESIAN_POINT('Origin',(1.11206539330992,5.49705207100037,-1.02022445880335));
#93725=CARTESIAN_POINT('',(-4.00298780463037,4.84409946428194,-6.23084676275461));
#93726=CARTESIAN_POINT('Ctrl Pts',(-4.00298780463038,4.84409946428194,-6.23084676275462));
#93727=CARTESIAN_POINT('Ctrl Pts',(-3.88918741840099,4.86143878568141,-6.28334817725779));
#93728=CARTESIAN_POINT('Ctrl Pts',(-3.77409429209713,4.87877094696915,-6.33298016119694));
#93729=CARTESIAN_POINT('Ctrl Pts',(-3.59954338698338,4.90476414604199,-6.40309634994019));
#93730=CARTESIAN_POINT('Ctrl Pts',(-3.54099701216533,4.91343410630816,-6.42576107199865));
#93731=CARTESIAN_POINT('Ctrl Pts',(-3.45283828592698,4.92641824543199,-6.4586158517722));
#93732=CARTESIAN_POINT('Ctrl Pts',(-3.42343700712078,4.93073677837089,-6.4693627551283));
#93733=CARTESIAN_POINT('Ctrl Pts',(-3.36481534024033,4.93932419698624,-6.49037281482567));
#93734=CARTESIAN_POINT('Ctrl Pts',(-3.33646763361339,4.94346636788396,-6.50034361875279));
#93735=CARTESIAN_POINT('Ctrl Pts',(-3.30553800070206,4.94797317425333,-6.51099180538869));
#93736=CARTESIAN_POINT('',(-4.54726098251639,4.94797317384177,-5.71331894151198));
#93737=CARTESIAN_POINT('Ctrl Pts',(-4.54726098289168,4.94797317335979,-5.71331894177495));
#93738=CARTESIAN_POINT('Ctrl Pts',(-4.46113246652684,4.93049584989789,-5.80420634576006));
#93739=CARTESIAN_POINT('Ctrl Pts',(-4.37264108000304,4.91309421476323,-5.89284148794172));
#93740=CARTESIAN_POINT('Ctrl Pts',(-4.19112105443983,4.87845834282927,-6.06543615855723));
#93741=CARTESIAN_POINT('Ctrl Pts',(-4.09812814402033,4.86123089194598,-6.14936196831929));
#93742=CARTESIAN_POINT('Ctrl Pts',(-4.00298780463038,4.84409946428194,-6.23084676275461));
#93743=CARTESIAN_POINT('',(-4.30128630597296,5.00000000033185,-5.83621762044319));
#93744=CARTESIAN_POINT('Ctrl Pts',(-4.30128630584344,5.00000000037138,-5.83621762015252));
#93745=CARTESIAN_POINT('Ctrl Pts',(-4.34268199875195,4.99124724802707,-5.81658208220761));
#93746=CARTESIAN_POINT('Ctrl Pts',(-4.38388110883993,4.98253936886008,-5.79651586247342));
#93747=CARTESIAN_POINT('Ctrl Pts',(-4.46615823557318,4.9651548502495,-5.75538472749207));
#93748=CARTESIAN_POINT('Ctrl Pts',(-4.5077728825359,4.95636631460042,-5.73402070142715));
#93749=CARTESIAN_POINT('Ctrl Pts',(-4.54726098217293,4.94797317484349,-5.71331894045073));
#93750=CARTESIAN_POINT('',(-4.58286555616587,4.95523000030221,-5.67547466231674));
#93751=CARTESIAN_POINT('Ctrl Pts',(-4.58286555616587,4.95523000030221,-5.67547466231674));
#93752=CARTESIAN_POINT('Ctrl Pts',(-4.53696995549485,4.96260329950046,-5.70305770250615));
#93753=CARTESIAN_POINT('Ctrl Pts',(-4.4902071393007,4.97005789384013,-5.73048842422905));
#93754=CARTESIAN_POINT('Ctrl Pts',(-4.39604979132316,4.98502388979892,-5.78424491125399));
#93755=CARTESIAN_POINT('Ctrl Pts',(-4.34881445013615,4.99250278497732,-5.81050279004188));
#93756=CARTESIAN_POINT('Ctrl Pts',(-4.30128630600721,5.00000000026661,-5.83621762016198));
#93757=CARTESIAN_POINT('',(-4.79558171325023,5.00000000122353,-5.43736112682667));
#93758=CARTESIAN_POINT('Origin',(0.791557283173849,5.12365813463513,-0.687680371718459));
#93759=CARTESIAN_POINT('',(-4.62792713406617,4.94797317374629,-5.64817547655208));
#93760=CARTESIAN_POINT('Origin',(0.86674739196922,5.49705157326691,-1.23543359314626));
#93761=CARTESIAN_POINT('',(-5.24884804582745,4.84409946429349,-5.22464897735641));
#93762=CARTESIAN_POINT('Ctrl Pts',(-5.24884804582745,4.84409946429349,-5.22464897735642));
#93763=CARTESIAN_POINT('Ctrl Pts',(-5.14899450165896,4.86143878565774,-5.30038665705747));
#93764=CARTESIAN_POINT('Ctrl Pts',(-5.04726159819795,4.87877094693586,-5.37359989277013));
#93765=CARTESIAN_POINT('Ctrl Pts',(-4.8918645042952,4.90476414600326,-5.47960008883646));
#93766=CARTESIAN_POINT('Ctrl Pts',(-4.83955915647839,4.91343410627102,-5.51432066224534));
#93767=CARTESIAN_POINT('Ctrl Pts',(-4.76052433877805,4.92641824539201,-5.56535883569174));
#93768=CARTESIAN_POINT('Ctrl Pts',(-4.73412071209948,4.93073677832799,-5.58217488825481));
#93769=CARTESIAN_POINT('Ctrl Pts',(-4.68138348157109,4.93932462805598,-5.61529733272974));
#93770=CARTESIAN_POINT('Ctrl Pts',(-4.65584788071166,4.94346583888768,-5.63112528011843));
#93771=CARTESIAN_POINT('Ctrl Pts',(-4.62792713381804,4.94797317426837,-5.64817547600773));
#93772=CARTESIAN_POINT('',(-5.66914323582772,4.94797317380338,-4.60221802398246));
#93773=CARTESIAN_POINT('Ctrl Pts',(-5.6691432362703,4.94797317345716,-4.60221802419248));
#93774=CARTESIAN_POINT('Ctrl Pts',(-5.60456646211845,4.93049585002012,-4.70949561608431));
#93775=CARTESIAN_POINT('Ctrl Pts',(-5.53719789031756,4.91309421481273,-4.81508155063048));
#93776=CARTESIAN_POINT('Ctrl Pts',(-5.39702445448899,4.87845834288268,-5.02266249347739));
#93777=CARTESIAN_POINT('Ctrl Pts',(-5.32424723486628,4.86123089197962,-5.12461689141406));
#93778=CARTESIAN_POINT('Ctrl Pts',(-5.24884804582746,4.84409946429349,-5.22464897735641));
#93779=CARTESIAN_POINT('',(-5.45533889445123,5.00000000010406,-4.77512068459171));
#93780=CARTESIAN_POINT('Ctrl Pts',(-5.45533889410359,5.00000000017678,-4.77512068412071));
#93781=CARTESIAN_POINT('Ctrl Pts',(-5.49154573973822,4.99124724267219,-4.74704534735226));
#93782=CARTESIAN_POINT('Ctrl Pts',(-5.52746798253027,4.98253936613918,-4.71859168193082));
#93783=CARTESIAN_POINT('Ctrl Pts',(-5.59897952991459,4.96515484938229,-4.66073502606677));
#93784=CARTESIAN_POINT('Ctrl Pts',(-5.63502861628044,4.95636631359973,-4.63092455917339));
#93785=CARTESIAN_POINT('Ctrl Pts',(-5.66914323546902,4.9479731746332,-4.60221802331358));
#93786=CARTESIAN_POINT('',(-5.69577999258466,4.95523000036888,-4.55760459272089));
#93787=CARTESIAN_POINT('Ctrl Pts',(-5.69577999258466,4.95523000036888,-4.55760459272089));
#93788=CARTESIAN_POINT('Ctrl Pts',(-5.65688928340724,4.9626028560638,-4.59440674027076));
#93789=CARTESIAN_POINT('Ctrl Pts',(-5.6171117243295,4.97005835676343,-4.63125323347676));
#93790=CARTESIAN_POINT('Ctrl Pts',(-5.53671427677798,4.98502388766089,-4.70399171001648));
#93791=CARTESIAN_POINT('Ctrl Pts',(-5.49622793408486,4.99250278380615,-4.73978990137419));
#93792=CARTESIAN_POINT('Ctrl Pts',(-5.45533889440155,4.99999999998404,-4.77512068407294));
#93793=CARTESIAN_POINT('',(-5.85233559273308,5.00000000113546,-4.27933033396379));
#93794=CARTESIAN_POINT('Origin',(0.625220748686339,5.12365841984548,-0.841763906061353));
#93795=CARTESIAN_POINT('',(-5.73391953761776,4.94797317377359,-4.52125673988802));
#93796=CARTESIAN_POINT('Origin',(0.58090261596229,5.49705193280982,-1.39287448079707));
#93797=CARTESIAN_POINT('',(-6.24927798597133,4.84409946433865,-3.97415241254827));
#93798=CARTESIAN_POINT('Ctrl Pts',(-6.24927798597134,4.84409946433865,-3.97415241254827));
#93799=CARTESIAN_POINT('Ctrl Pts',(-6.16804032445152,4.86143878571084,-4.06958494783095));
#93800=CARTESIAN_POINT('Ctrl Pts',(-6.08442456118427,4.87877094699107,-4.16295606591001));
#93801=CARTESIAN_POINT('Ctrl Pts',(-5.95544747371417,4.90476414605477,-4.29988381808576));
#93802=CARTESIAN_POINT('Ctrl Pts',(-5.911828892812,4.91343410631592,-4.3450367474367));
#93803=CARTESIAN_POINT('Ctrl Pts',(-5.84561356381545,4.92641824543168,-4.41187182634179));
#93804=CARTESIAN_POINT('Ctrl Pts',(-5.82344219345241,4.93073677836905,-4.43397072821995));
#93805=CARTESIAN_POINT('Ctrl Pts',(-5.77905827644861,4.93932462810677,-4.47765573410487));
#93806=CARTESIAN_POINT('Ctrl Pts',(-5.75752222447624,4.94346583895174,-4.498603032325));
#93807=CARTESIAN_POINT('Ctrl Pts',(-5.73391953723181,4.9479731743308,-4.52125673937504));
#93808=CARTESIAN_POINT('',(-6.52594265175988,4.94797317388831,-3.27592250727311));
#93809=CARTESIAN_POINT('Ctrl Pts',(-6.52594265231059,4.94797317344726,-3.27592250739383));
#93810=CARTESIAN_POINT('Ctrl Pts',(-6.48593715840192,4.93049585002046,-3.39457410634552));
#93811=CARTESIAN_POINT('Ctrl Pts',(-6.44284148120856,4.91309421484135,-3.512173751874));
#93812=CARTESIAN_POINT('Ctrl Pts',(-6.35056898909567,4.87845834293924,-3.74503471273904));
#93813=CARTESIAN_POINT('Ctrl Pts',(-6.30141044225873,4.8612308920418,-3.8602504243896));
#93814=CARTESIAN_POINT('Ctrl Pts',(-6.24927798597133,4.84409946433865,-3.97415241254827));
#93815=CARTESIAN_POINT('',(-6.35430589758882,5.0000000002178,-3.49074441377445));
#93816=CARTESIAN_POINT('Ctrl Pts',(-6.35430589724851,5.00000000027394,-3.49074441347699));
#93817=CARTESIAN_POINT('Ctrl Pts',(-6.38363087081989,4.99124724542744,-3.45554207113647));
#93818=CARTESIAN_POINT('Ctrl Pts',(-6.41259657898731,4.9825393675923,-3.42003141116201));
#93819=CARTESIAN_POINT('Ctrl Pts',(-6.4699987557459,4.96515485077748,-3.34815454233767));
#93820=CARTESIAN_POINT('Ctrl Pts',(-6.49879666789651,4.95636631412613,-3.31129153669143));
#93821=CARTESIAN_POINT('Ctrl Pts',(-6.52594265111574,4.94797317489863,-3.27592250653897));
#93822=CARTESIAN_POINT('',(-6.54236608731522,4.9552300002817,-3.22662599759221));
#93823=CARTESIAN_POINT('Ctrl Pts',(-6.54236608731522,4.9552300002817,-3.22662599759221));
#93824=CARTESIAN_POINT('Ctrl Pts',(-6.5122959954036,4.96260285591192,-3.27092808392267));
#93825=CARTESIAN_POINT('Ctrl Pts',(-6.48136931901497,4.9700583569918,-3.31546412787944));
#93826=CARTESIAN_POINT('Ctrl Pts',(-6.41848813764831,4.98502388877246,-3.40378509928733));
#93827=CARTESIAN_POINT('Ctrl Pts',(-6.38664389809692,4.99250278441687,-3.44744971279347));
#93828=CARTESIAN_POINT('Ctrl Pts',(-6.35430589746526,5.00000000012513,-3.49074441339151));
#93829=CARTESIAN_POINT('',(-6.63544076432503,5.00000000130698,-2.92120280906809));
#93830=CARTESIAN_POINT('Origin',(0.429648035935632,5.12365808305802,-0.956488199897906));
#93831=CARTESIAN_POINT('',(-6.5718002370655,4.94797317371172,-3.1829290620009));
#93832=CARTESIAN_POINT('Origin',(0.267892146939279,5.49705138256567,-1.48518724332511));
#93833=CARTESIAN_POINT('',(-6.9574986329725,4.84409946433526,-2.5378288981618));
#93834=CARTESIAN_POINT('Ctrl Pts',(-6.95749863297251,4.84409946433526,-2.5378288981618));
#93835=CARTESIAN_POINT('Ctrl Pts',(-6.89867543702368,4.86143878567583,-2.64849396955423));
#93836=CARTESIAN_POINT('Ctrl Pts',(-6.83708659426749,4.87877094692769,-2.75765704010306));
#93837=CARTESIAN_POINT('Ctrl Pts',(-6.74056033871976,4.90476414595529,-2.91910975859602));
#93838=CARTESIAN_POINT('Ctrl Pts',(-6.70766808115882,4.91343410620189,-2.97258374299614));
#93839=CARTESIAN_POINT('Ctrl Pts',(-6.65736839616571,4.92641824530265,-3.05209059320888));
#93840=CARTESIAN_POINT('Ctrl Pts',(-6.64046599080045,4.93073677823803,-3.07843902426737));
#93841=CARTESIAN_POINT('Ctrl Pts',(-6.60651073008813,4.93932462797207,-3.13064392912216));
#93842=CARTESIAN_POINT('Ctrl Pts',(-6.58998122902561,4.94346583880374,-3.15573110563001));
#93843=CARTESIAN_POINT('Ctrl Pts',(-6.57180023681244,4.94797317419977,-3.18292906175086));
#93844=CARTESIAN_POINT('',(-7.0775962428047,4.94797317380733,-1.79644849492893));
#93845=CARTESIAN_POINT('Ctrl Pts',(-7.0775962432299,4.94797317335439,-1.79644849491167));
#93846=CARTESIAN_POINT('Ctrl Pts',(-7.06403264194361,4.93049584991313,-1.92092608431536));
#93847=CARTESIAN_POINT('Ctrl Pts',(-7.04722496533824,4.91309421480762,-2.04504061177499));
#93848=CARTESIAN_POINT('Ctrl Pts',(-7.0071679759942,4.8784583429011,-2.29229327130114));
#93849=CARTESIAN_POINT('Ctrl Pts',(-6.98392670089476,4.86123089201992,-2.4153829381001));
#93850=CARTESIAN_POINT('Ctrl Pts',(-6.95749863297251,4.84409946433526,-2.5378288981618));
#93851=CARTESIAN_POINT('',(-6.95615261953385,5.0000000003909,-2.0431448139407));
#93852=CARTESIAN_POINT('Ctrl Pts',(-6.95615261934601,5.00000000041751,-2.04314481383768));
#93853=CARTESIAN_POINT('Ctrl Pts',(-6.97722451588073,4.99124725073596,-2.00246150420444));
#93854=CARTESIAN_POINT('Ctrl Pts',(-6.9978792864587,4.98253937018195,-1.9615542801404));
#93855=CARTESIAN_POINT('Ctrl Pts',(-7.03848803841168,4.96515484981917,-1.8790180643763));
#93856=CARTESIAN_POINT('Ctrl Pts',(-7.05868821461483,4.95636631330385,-1.8368261953792));
#93857=CARTESIAN_POINT('Ctrl Pts',(-7.07759624194427,4.94797317474325,-1.79644849433146));
#93858=CARTESIAN_POINT('',(-7.08303841496067,4.95523000028387,-1.74477395697836));
#93859=CARTESIAN_POINT('Ctrl Pts',(-7.08303841496068,4.95523000028387,-1.74477395697837));
#93860=CARTESIAN_POINT('Ctrl Pts',(-7.06319378849081,4.96260330013697,-1.79450746240022));
#93861=CARTESIAN_POINT('Ctrl Pts',(-7.04256660110086,4.97005789420884,-1.84464451794085));
#93862=CARTESIAN_POINT('Ctrl Pts',(-7.00014062676657,4.98502389099315,-1.94442128925669));
#93863=CARTESIAN_POINT('Ctrl Pts',(-6.97842749173757,4.99250278562616,-1.99391061172942));
#93864=CARTESIAN_POINT('Ctrl Pts',(-6.95615261941778,5.00000000035927,-2.0431448138));
#93865=CARTESIAN_POINT('',(-7.10828010096112,5.00000000118293,-1.4264830892052));
#93866=CARTESIAN_POINT('Origin',(0.213987963839789,5.12365837061161,-1.02648756263497));
#93867=CARTESIAN_POINT('',(-7.10239086153082,4.94797317376557,-1.69577115923219));
#93868=CARTESIAN_POINT('Origin',(-0.0576388480719026,5.4970519466876,-1.50805329764877));
#93869=CARTESIAN_POINT('',(-7.34039437668646,4.84409946433426,-0.982839325059756));
#93870=CARTESIAN_POINT('Ctrl Pts',(-7.34039437668647,4.84409946433426,-0.982839325059758));
#93871=CARTESIAN_POINT('Ctrl Pts',(-7.30673615347733,4.86143878567784,-1.10356235691438));
#93872=CARTESIAN_POINT('Ctrl Pts',(-7.27005405695223,4.87877094694078,-1.22341303619949));
#93873=CARTESIAN_POINT('Ctrl Pts',(-7.21049209354376,4.90476414599402,-1.40184137156618));
#93874=CARTESIAN_POINT('Ctrl Pts',(-7.1898641646212,4.91343410625637,-1.46113602707844));
#93875=CARTESIAN_POINT('Ctrl Pts',(-7.15783208086489,4.92641824537678,-1.54959699679477));
#93876=CARTESIAN_POINT('Ctrl Pts',(-7.14698897816429,4.93073677831544,-1.57896293369232));
#93877=CARTESIAN_POINT('Ctrl Pts',(-7.12505118531909,4.93932419693192,-1.63724376826478));
#93878=CARTESIAN_POINT('Ctrl Pts',(-7.11429863727107,4.94346636782592,-1.665304276277));
#93879=CARTESIAN_POINT('Ctrl Pts',(-7.10239086091004,4.94797317420863,-1.69577115892403));
#93880=CARTESIAN_POINT('',(-7.29830929924953,4.94797317385515,-0.232974546960617));
#93881=CARTESIAN_POINT('Ctrl Pts',(-7.29830929980229,4.9479731734908,-0.232974546849461));
#93882=CARTESIAN_POINT('Ctrl Pts',(-7.31182181016524,4.93049585006795,-0.357457692479486));
#93883=CARTESIAN_POINT('Ctrl Pts',(-7.32208804239158,4.9130942148399,-0.48228364561484));
#93884=CARTESIAN_POINT('Ctrl Pts',(-7.3361195762891,4.87845834292249,-0.73236674389168));
#93885=CARTESIAN_POINT('Ctrl Pts',(-7.3398823091514,4.86123089202013,-0.857574829957159));
#93886=CARTESIAN_POINT('Ctrl Pts',(-7.34039437668647,4.84409946433426,-0.982839325059756));
#93887=CARTESIAN_POINT('',(-7.23273737682457,5.00000000045635,-0.500010033007036));
#93888=CARTESIAN_POINT('Ctrl Pts',(-7.23273737668175,5.00000000047483,-0.5000100329652));
#93889=CARTESIAN_POINT('Ctrl Pts',(-7.24457091367181,4.99124725176391,-0.455748046850563));
#93890=CARTESIAN_POINT('Ctrl Pts',(-7.25594894401456,4.98253937067083,-0.411357042952466));
#93891=CARTESIAN_POINT('Ctrl Pts',(-7.27786544000373,4.96515484972087,-0.322020793969775));
#93892=CARTESIAN_POINT('Ctrl Pts',(-7.2885233424811,4.95636631334907,-0.276472907790325));
#93893=CARTESIAN_POINT('Ctrl Pts',(-7.2983092985434,4.94797317475611,-0.232974546627913));
#93894=CARTESIAN_POINT('',(-7.29251573846638,4.95523000034311,-0.18133822573945));
#93895=CARTESIAN_POINT('Ctrl Pts',(-7.29251573846639,4.95523000034311,-0.181338225739452));
#93896=CARTESIAN_POINT('Ctrl Pts',(-7.28382682480052,4.96260285648447,-0.23417181792712));
#93897=CARTESIAN_POINT('Ctrl Pts',(-7.27445873376066,4.97005835691444,-0.287577406606114));
#93898=CARTESIAN_POINT('Ctrl Pts',(-7.25447432879073,4.98502389150509,-0.394138491448891));
#93899=CARTESIAN_POINT('Ctrl Pts',(-7.24390757645083,4.99250278595753,-0.447138461622359));
#93900=CARTESIAN_POINT('Ctrl Pts',(-7.23273737672512,5.00000000043411,-0.500010032928329));
#93901=CARTESIAN_POINT('',(-7.24874416011981,5.00000000111792,0.13493739489825));
#93902=CARTESIAN_POINT('Origin',(-0.0116793057854747,5.12365838142277,-1.04848995574475));
#93903=CARTESIAN_POINT('',(-7.30088158231934,4.94797317377374,-0.129320882509947));
#93904=CARTESIAN_POINT('Origin',(-0.380478934841684,5.49705192399641,-1.4604050333425));
#93905=CARTESIAN_POINT('',(-7.38006143768145,4.84409946429152,0.618106722867779));
#93906=CARTESIAN_POINT('Ctrl Pts',(-7.38006143768146,4.84409946429152,0.618106722867779));
#93907=CARTESIAN_POINT('Ctrl Pts',(-7.37314200830705,4.86143878566475,0.492970605287479));
#93908=CARTESIAN_POINT('Ctrl Pts',(-7.36308187208114,4.87877094695141,0.36803640178613));
#93909=CARTESIAN_POINT('Ctrl Pts',(-7.34326925205903,4.90476414602571,0.180975560198201));
#93910=CARTESIAN_POINT('Ctrl Pts',(-7.33587019084798,4.91343410628931,0.118632785831322));
#93911=CARTESIAN_POINT('Ctrl Pts',(-7.32360349300845,4.92641824541276,0.0253540332676023));
#93912=CARTESIAN_POINT('Ctrl Pts',(-7.31932670440219,4.93073677835475,-0.00565629093040938));
#93913=CARTESIAN_POINT('Ctrl Pts',(-7.31043001499084,4.93932462810217,-0.0672936233185138));
#93914=CARTESIAN_POINT('Ctrl Pts',(-7.30596207811234,4.94346583894984,-0.0970026855058121));
#93915=CARTESIAN_POINT('Ctrl Pts',(-7.30088158184065,4.94797317433898,-0.129320882355863));
#93916=CARTESIAN_POINT('',(-7.17776152475488,4.94797317380236,1.34139303118644));
#93917=CARTESIAN_POINT('Ctrl Pts',(-7.17776152514807,4.94797317339019,1.34139303137954));
#93918=CARTESIAN_POINT('Ctrl Pts',(-7.21771831716903,4.93049584997349,1.2227250226255));
#93919=CARTESIAN_POINT('Ctrl Pts',(-7.25457842050998,4.9130942148394,1.10302436785673));
#93920=CARTESIAN_POINT('Ctrl Pts',(-7.32204237868749,4.87845834291323,0.861804438367264));
#93921=CARTESIAN_POINT('Ctrl Pts',(-7.35263317832365,4.86123089200476,0.740332524198434));
#93922=CARTESIAN_POINT('Ctrl Pts',(-7.38006143768146,4.84409946429152,0.618106722867782));
#93923=CARTESIAN_POINT('',(-7.17112737312078,5.00000000051076,1.06650466102044));
#93924=CARTESIAN_POINT('Ctrl Pts',(-7.17112737304764,5.00000000051987,1.06650466102544));
#93925=CARTESIAN_POINT('Ctrl Pts',(-7.17316922946218,4.99124725346394,1.11227567873281));
#93926=CARTESIAN_POINT('Ctrl Pts',(-7.17473849443647,4.98253937156206,1.15807478980744));
#93927=CARTESIAN_POINT('Ctrl Pts',(-7.17693794222823,4.96515485006557,1.25003380867691));
#93928=CARTESIAN_POINT('Ctrl Pts',(-7.17755521977201,4.95636631307048,1.29680794788393));
#93929=CARTESIAN_POINT('Ctrl Pts',(-7.17776152382245,4.94797317469699,1.34139303135917));
#93930=CARTESIAN_POINT('',(-7.16100313117102,4.95523000029981,1.39057668033257));
#93931=CARTESIAN_POINT('Ctrl Pts',(-7.16100313117103,4.95523000029981,1.39057668033257));
#93932=CARTESIAN_POINT('Ctrl Pts',(-7.16387519267682,4.96260329941632,1.33710723583422));
#93933=CARTESIAN_POINT('Ctrl Pts',(-7.16620646791303,4.97005789390706,1.2829429419715));
#93934=CARTESIAN_POINT('Ctrl Pts',(-7.16959687559227,4.98502389213623,1.17457378243522));
#93935=CARTESIAN_POINT('Ctrl Pts',(-7.17067059482315,4.99250278630537,1.12054138490138));
#93936=CARTESIAN_POINT('Ctrl Pts',(-7.1711273730592,5.00000000050815,1.06650466102737));
#93937=CARTESIAN_POINT('',(-7.05026499821003,5.00000000126723,1.69004835712118));
#93938=CARTESIAN_POINT('Origin',(-0.236800892431308,5.12365819333402,-1.02146601117213));
#93939=CARTESIAN_POINT('',(-7.15799119542332,4.94797317376926,1.44317629552494));
#93940=CARTESIAN_POINT('Origin',(-0.685527333282975,5.49705211802892,-1.34446996642009));
#93941=CARTESIAN_POINT('',(-7.0746450282201,4.8440994643031,2.19015078689032));
#93942=CARTESIAN_POINT('Ctrl Pts',(-7.07464502822011,4.8440994643031,2.19015078689033));
#93943=CARTESIAN_POINT('Ctrl Pts',(-7.09478793753128,4.86143878566637,2.06645280946945));
#93944=CARTESIAN_POINT('Ctrl Pts',(-7.11182016240746,4.87877094695015,1.94227686635824));
#93945=CARTESIAN_POINT('Ctrl Pts',(-7.13268330187995,4.90476414602651,1.75533027567424));
#93946=CARTESIAN_POINT('Ctrl Pts',(-7.13885908025635,4.91343410629485,1.69285446126028));
#93947=CARTESIAN_POINT('Ctrl Pts',(-7.14693134549244,4.92641824541834,1.59911953666473));
#93948=CARTESIAN_POINT('Ctrl Pts',(-7.1494208488683,4.93073677835663,1.56791483350988));
#93949=CARTESIAN_POINT('Ctrl Pts',(-7.15398236358274,4.93932462809247,1.50580602253555));
#93950=CARTESIAN_POINT('Ctrl Pts',(-7.15600545475998,4.94346583893296,1.47583106739905));
#93951=CARTESIAN_POINT('Ctrl Pts',(-7.15799119467072,4.94797317431431,1.4431762955544));
#93952=CARTESIAN_POINT('',(-6.72158959858316,4.94797317388402,2.85303856204128));
#93953=CARTESIAN_POINT('Ctrl Pts',(-6.72158959902029,4.94797317342077,2.85303856237963));
#93954=CARTESIAN_POINT('Ctrl Pts',(-6.78612233751133,4.93049585000813,2.7457344749205));
#93955=CARTESIAN_POINT('Ctrl Pts',(-6.84785277466984,4.91309421482941,2.63675618743939));
#93956=CARTESIAN_POINT('Ctrl Pts',(-6.96559461743177,4.87845834288678,2.41567860264718));
#93957=CARTESIAN_POINT('Ctrl Pts',(-7.02158309203489,4.86123089197945,2.30362275197257));
#93958=CARTESIAN_POINT('Ctrl Pts',(-7.07464502822011,4.8440994643031,2.19015078689033));
#93959=CARTESIAN_POINT('',(-6.77420342353812,5.00000000021333,2.58315078520084));
#93960=CARTESIAN_POINT('Ctrl Pts',(-6.7742034230859,5.00000000027013,2.58315078513325));
#93961=CARTESIAN_POINT('Ctrl Pts',(-6.7663581191946,4.99124724528312,2.62829068126326));
#93962=CARTESIAN_POINT('Ctrl Pts',(-6.75804524388186,4.98253936748107,2.67335635884948));
#93963=CARTESIAN_POINT('Ctrl Pts',(-6.74042480375319,4.96515485062198,2.76363821908636));
#93964=CARTESIAN_POINT('Ctrl Pts',(-6.73097259275404,4.95636631384195,2.80945150006911));
#93965=CARTESIAN_POINT('Ctrl Pts',(-6.72158959756006,4.94797317490626,2.85303856201789));
#93966=CARTESIAN_POINT('',(-6.69464997632219,4.95523000034612,2.89746976556783));
#93967=CARTESIAN_POINT('Ctrl Pts',(-6.6946499763222,4.95523000034612,2.89746976556783));
#93968=CARTESIAN_POINT('Ctrl Pts',(-6.70894923932624,4.96260329885002,2.84586781988646));
#93969=CARTESIAN_POINT('Ctrl Pts',(-6.72286973387921,4.97005789392374,2.79347100827728));
#93970=CARTESIAN_POINT('Ctrl Pts',(-6.74947703568066,4.98502388866908,2.68836432083602));
#93971=CARTESIAN_POINT('Ctrl Pts',(-6.76214102330062,4.99250278434603,2.6358259778232));
#93972=CARTESIAN_POINT('Ctrl Pts',(-6.77420342316194,5.00000000011959,2.58315078535635));
#93973=CARTESIAN_POINT('',(-6.52212328112776,5.00000000126512,3.16613453534081));
#93974=CARTESIAN_POINT('Origin',(-0.450850659841332,5.12365813414324,-0.946678847083811));
#93975=CARTESIAN_POINT('',(-6.68040109545753,4.94797317379139,2.94819215415093));
#93976=CARTESIAN_POINT('Origin',(-0.958523019359824,5.49705207103514,-1.16566772092202));
#93977=CARTESIAN_POINT('',(-6.43842608023093,4.84409946433625,3.65978583438252));
#93978=CARTESIAN_POINT('Ctrl Pts',(-6.43842608023094,4.84409946433625,3.65978583438252));
#93979=CARTESIAN_POINT('Ctrl Pts',(-6.48468946811766,4.86143878571813,3.54330997707003));
#93980=CARTESIAN_POINT('Ctrl Pts',(-6.52801764617062,4.87877094699052,3.42569862344729));
#93981=CARTESIAN_POINT('Ctrl Pts',(-6.58858100787816,4.90476414604654,3.2476076985895));
#93982=CARTESIAN_POINT('Ctrl Pts',(-6.608042853287,4.91343410630369,3.18792014387897));
#93983=CARTESIAN_POINT('Ctrl Pts',(-6.63607663141585,4.92641824542267,3.09811198823373));
#93984=CARTESIAN_POINT('Ctrl Pts',(-6.6452160203545,4.93073677836402,3.06817200334143));
#93985=CARTESIAN_POINT('Ctrl Pts',(-6.66302244782254,4.93932462811458,3.00849585265603));
#93986=CARTESIAN_POINT('Ctrl Pts',(-6.67144196955517,4.94346583896624,2.97965660008473));
#93987=CARTESIAN_POINT('Ctrl Pts',(-6.68040109464971,4.94797317436312,2.94819215400281));
#93988=CARTESIAN_POINT('',(-5.9511236137351,4.94797317388934,4.23127918051304));
#93989=CARTESIAN_POINT('Ctrl Pts',(-5.95112361406283,4.94797317337418,4.23127918092237));
#93990=CARTESIAN_POINT('Ctrl Pts',(-6.03721481998975,4.93049584990762,4.14035643456259));
#93991=CARTESIAN_POINT('Ctrl Pts',(-6.12092914409712,4.91309421476481,4.04719621830559));
#93992=CARTESIAN_POINT('Ctrl Pts',(-6.28344339371998,4.87845834285195,3.85659832029483));
#93993=CARTESIAN_POINT('Ctrl Pts',(-6.36221158439183,4.86123089198366,3.75919814017742));
#93994=CARTESIAN_POINT('Ctrl Pts',(-6.43842608023093,4.84409946433625,3.65978583438252));
#93995=CARTESIAN_POINT('',(-6.06052525045423,5.00000000006602,3.97901164806513));
#93996=CARTESIAN_POINT('Ctrl Pts',(-6.06052524986571,5.00000000014428,3.97901164784023));
#93997=CARTESIAN_POINT('Ctrl Pts',(-6.04315961497363,4.99124724184196,4.02140970579152));
#93998=CARTESIAN_POINT('Ctrl Pts',(-6.02535330478515,4.98253936579715,4.0636347419452));
#93999=CARTESIAN_POINT('Ctrl Pts',(-5.98873689183328,4.96515484996222,4.1480179834896));
#94000=CARTESIAN_POINT('Ctrl Pts',(-5.96965716811944,4.95636631373681,4.19072822695835));
#94001=CARTESIAN_POINT('Ctrl Pts',(-5.95112361260635,4.94797317496797,4.2312791802204));
#94002=CARTESIAN_POINT('',(-5.9152624289547,4.95523000032746,4.26888038538439));
#94003=CARTESIAN_POINT('Ctrl Pts',(-5.9152624289547,4.95523000032746,4.26888038538439));
#94004=CARTESIAN_POINT('Ctrl Pts',(-5.94031885595169,4.96260288086368,4.22156146549675));
#94005=CARTESIAN_POINT('Ctrl Pts',(-5.96518060385663,4.9700583625512,4.17337643669248));
#94006=CARTESIAN_POINT('Ctrl Pts',(-6.01375908058615,4.98502386688622,4.07645004498659));
#94007=CARTESIAN_POINT('Ctrl Pts',(-6.03742121981557,4.99250277347481,4.02786233440585));
#94008=CARTESIAN_POINT('Ctrl Pts',(-6.06052525004563,4.99999999998347,3.97901164785921));
#94009=CARTESIAN_POINT('',(-5.68901432884376,5.00000000114322,4.49417578249345));
#94010=CARTESIAN_POINT('Origin',(-0.643817031139517,5.12365825596667,-0.827627422281949));
#94011=CARTESIAN_POINT('',(-5.89044286473166,4.94797317375056,4.31535382449974));
#94012=CARTESIAN_POINT('Origin',(-1.18669562488869,5.49705179923779,-0.932362816200588));
#94013=CARTESIAN_POINT('',(-5.50115348427103,4.8440994643342,4.9582933643208));
#94014=CARTESIAN_POINT('Ctrl Pts',(-5.50115348427104,4.8440994643342,4.95829336432081));
#94015=CARTESIAN_POINT('Ctrl Pts',(-5.57137412622155,4.86143878566795,4.85448590871698));
#94016=CARTESIAN_POINT('Ctrl Pts',(-5.63897228002819,4.8787709469205,4.74893852071259));
#94017=CARTESIAN_POINT('Ctrl Pts',(-5.73640398850807,4.9047641459615,4.58803059527565));
#94018=CARTESIAN_POINT('Ctrl Pts',(-5.76824188668813,4.91343410621467,4.53392222392337));
#94019=CARTESIAN_POINT('Ctrl Pts',(-5.81492634941089,4.92641824533118,4.45224016669456));
#94020=CARTESIAN_POINT('Ctrl Pts',(-5.83028827625063,4.93073677827342,4.42496486047126));
#94021=CARTESIAN_POINT('Ctrl Pts',(-5.86050700772111,4.93932462802316,4.3705117605863));
#94022=CARTESIAN_POINT('Ctrl Pts',(-5.87492927249967,4.94346583886421,4.3441567020763));
#94023=CARTESIAN_POINT('Ctrl Pts',(-5.89044286410019,4.94797317427384,4.31535382424151));
#94024=CARTESIAN_POINT('',(-4.90238970219432,4.94797317377648,5.41166988820258));
#94025=CARTESIAN_POINT('Ctrl Pts',(-4.90238970237242,4.94797317337695,5.41166988856449));
#94026=CARTESIAN_POINT('Ctrl Pts',(-5.00601384658402,4.93049584992143,5.34137992990052));
#94027=CARTESIAN_POINT('Ctrl Pts',(-5.10779766906465,4.91309421477567,5.2683938528048));
#94028=CARTESIAN_POINT('Ctrl Pts',(-5.30748533998087,4.87845834285546,5.11718778745134));
#94029=CARTESIAN_POINT('Ctrl Pts',(-5.405357821173,4.86122953170664,5.03899135032968));
#94030=CARTESIAN_POINT('Ctrl Pts',(-5.50116106175314,4.84409810933837,4.95828698108094));
#94031=CARTESIAN_POINT('',(-5.06346365273142,5.00000000024774,5.18881834708339));
#94032=CARTESIAN_POINT('Ctrl Pts',(-5.0634636523831,5.00000000029952,5.18881834685435));
#94033=CARTESIAN_POINT('Ctrl Pts',(-5.03738969924476,4.99124724607008,5.22649204615994));
#94034=CARTESIAN_POINT('Ctrl Pts',(-5.01092254989299,4.98253936790085,5.26390206337639));
#94035=CARTESIAN_POINT('Ctrl Pts',(-4.95702230137582,4.96515485070685,5.33844103118426));
#94036=CARTESIAN_POINT('Ctrl Pts',(-4.92920721075983,4.95636631423499,5.37605115707747));
#94037=CARTESIAN_POINT('Ctrl Pts',(-4.90238970136707,4.94797317463228,5.4116698877814));
#94038=CARTESIAN_POINT('',(-4.8592837852266,4.95523000036476,5.44068290219272));
#94039=CARTESIAN_POINT('Ctrl Pts',(-4.8592837852266,4.95523000036476,5.44068290219272));
#94040=CARTESIAN_POINT('Ctrl Pts',(-4.89392864298546,4.9626033208512,5.39985422744277));
#94041=CARTESIAN_POINT('Ctrl Pts',(-4.92856333329916,4.97005790377228,5.3581452969328));
#94042=CARTESIAN_POINT('Ctrl Pts',(-4.99684448344413,4.98502386886887,5.273925334085));
#94043=CARTESIAN_POINT('Ctrl Pts',(-5.03039833218755,4.9925027745633,5.23156024274039));
#94044=CARTESIAN_POINT('Ctrl Pts',(-5.06346365249666,5.00000000019312,5.1888183468922));
#94045=CARTESIAN_POINT('',(-4.58989338860951,5.00000000112623,5.61207436548009));
#94046=CARTESIAN_POINT('Origin',(-0.806680192645151,5.12365860650201,-0.669876686411711));
#94047=CARTESIAN_POINT('',(-4.82505407222897,4.94797317374014,5.48073434620426));
#94048=CARTESIAN_POINT('Origin',(-1.35938120842026,5.49705179230414,-0.655461214805863));
#94049=CARTESIAN_POINT('',(-4.30665306526583,4.84409946429903,6.0249566073236));
#94050=CARTESIAN_POINT('Ctrl Pts',(-4.30665306526583,4.84409946429903,6.02495660732361));
#94051=CARTESIAN_POINT('Ctrl Pts',(-4.39754752209537,4.86143878565606,5.93867147461155));
#94052=CARTESIAN_POINT('Ctrl Pts',(-4.48625483714493,4.87877094691826,5.85012333072359));
#94053=CARTESIAN_POINT('Ctrl Pts',(-4.61599909412046,4.90476414596476,5.71392228032555));
#94054=CARTESIAN_POINT('Ctrl Pts',(-4.65872434042047,4.91343410622358,5.66792313954466));
#94055=CARTESIAN_POINT('Ctrl Pts',(-4.72187657422963,4.92641824533791,5.59818654285872));
#94056=CARTESIAN_POINT('Ctrl Pts',(-4.74274273234744,4.9307367782742,5.57485127831631));
#94057=CARTESIAN_POINT('Ctrl Pts',(-4.78395870432753,4.93932419688864,5.52816973925923));
#94058=CARTESIAN_POINT('Ctrl Pts',(-4.80371391686449,4.94346636778017,5.50552595475308));
#94059=CARTESIAN_POINT('Ctrl Pts',(-4.82505407173893,4.94797317417246,5.48073434586103));
#94060=CARTESIAN_POINT('',(-3.62442549739344,4.94797317379252,6.3390169257249));
#94061=CARTESIAN_POINT('Ctrl Pts',(-3.62442549749584,4.94797317337247,6.33901692614006));
#94062=CARTESIAN_POINT('Ctrl Pts',(-3.74073723005479,4.93049584992828,6.29264643558571));
#94063=CARTESIAN_POINT('Ctrl Pts',(-3.85583125231974,4.91309421478534,6.24324724561167));
#94064=CARTESIAN_POINT('Ctrl Pts',(-4.08335517068789,4.87845834284928,6.1385032407116));
#94065=CARTESIAN_POINT('Ctrl Pts',(-4.19574051848432,4.86123089196007,6.0831791362385));
#94066=CARTESIAN_POINT('Ctrl Pts',(-4.30665306526583,4.84409946429903,6.02495660732361));
#94067=CARTESIAN_POINT('',(-3.82964012287192,5.00000000030332,6.15600166741685));
#94068=CARTESIAN_POINT('Ctrl Pts',(-3.82964012262647,5.00000000034701,6.15600166716498));
#94069=CARTESIAN_POINT('Ctrl Pts',(-3.79607703682092,4.99124724741758,6.18718944279529));
#94070=CARTESIAN_POINT('Ctrl Pts',(-3.76218662411001,4.98253936856204,6.21803518242874));
#94071=CARTESIAN_POINT('Ctrl Pts',(-3.6935228484439,4.96515484867379,6.27924451971109));
#94072=CARTESIAN_POINT('Ctrl Pts',(-3.65827299131585,4.95636631176606,6.30999592123176));
#94073=CARTESIAN_POINT('Ctrl Pts',(-3.62442549665219,4.94797317467946,6.33901692511689));
#94074=CARTESIAN_POINT('',(-3.57609043208675,4.9552300004188,6.35808513377476));
#94075=CARTESIAN_POINT('Ctrl Pts',(-3.57609043208675,4.9552300004188,6.35808513377476));
#94076=CARTESIAN_POINT('Ctrl Pts',(-3.61869958609048,4.9626028564312,6.32566067382102));
#94077=CARTESIAN_POINT('Ctrl Pts',(-3.66149597485689,4.97005835696801,6.29236822343175));
#94078=CARTESIAN_POINT('Ctrl Pts',(-3.74628310255969,4.98502388963094,6.22479765766597));
#94079=CARTESIAN_POINT('Ctrl Pts',(-3.7881596635725,4.9925027848899,6.19063616758905));
#94080=CARTESIAN_POINT('Ctrl Pts',(-3.82964012256919,5.00000000023122,6.15600166733698));
#94081=CARTESIAN_POINT('',(-3.27615413515278,5.00000000120582,6.46755858726378));
#94082=CARTESIAN_POINT('Origin',(-0.931824247626192,5.12365838328379,-0.480802586718734));
#94083=CARTESIAN_POINT('',(-3.53405111422536,4.94797317377853,6.3898418209816));
#94084=CARTESIAN_POINT('Origin',(-1.46850476501289,5.49705202712533,-0.347909162332483));
#94085=CARTESIAN_POINT('',(-2.91077833579864,4.84409946434516,6.80989957516688));
#94086=CARTESIAN_POINT('Ctrl Pts',(-2.91077833579864,4.84409946434516,6.80989957516688));
#94087=CARTESIAN_POINT('Ctrl Pts',(-3.01809648368299,4.8614387857069,6.74517136230629));
#94088=CARTESIAN_POINT('Ctrl Pts',(-3.12376510445404,4.87877094697295,6.6777628753848));
#94089=CARTESIAN_POINT('Ctrl Pts',(-3.27975521253511,4.90476414602561,6.5726373098989));
#94090=CARTESIAN_POINT('Ctrl Pts',(-3.33137002185206,4.91343410628631,6.53689826847531));
#94091=CARTESIAN_POINT('Ctrl Pts',(-3.40803709840257,4.92641824540357,6.48236793817296));
#94092=CARTESIAN_POINT('Ctrl Pts',(-3.43343180942504,4.93073677834079,6.46406384634563));
#94093=CARTESIAN_POINT('Ctrl Pts',(-3.48371932585261,4.93932419695326,6.42733391139021));
#94094=CARTESIAN_POINT('Ctrl Pts',(-3.5078804168098,4.94346636784446,6.4094663127248));
#94095=CARTESIAN_POINT('Ctrl Pts',(-3.53405111372333,4.9479731742255,6.38984182041476));
#94096=CARTESIAN_POINT('',(-2.17698718490753,4.94797317384646,6.96995857709649));
#94097=CARTESIAN_POINT('Ctrl Pts',(-2.1769871849229,4.94797317338406,6.96995857758856));
#94098=CARTESIAN_POINT('Ctrl Pts',(-2.30054789847439,4.93049584991362,6.94967578773418));
#94099=CARTESIAN_POINT('Ctrl Pts',(-2.42357045206225,4.91309421475659,6.92617333601248));
#94100=CARTESIAN_POINT('Ctrl Pts',(-2.66829185230895,4.87845834284315,6.87278910466344));
#94101=CARTESIAN_POINT('Ctrl Pts',(-2.78994274014277,4.8612308919762,6.84291797470086));
#94102=CARTESIAN_POINT('Ctrl Pts',(-2.91077833579864,4.84409946434516,6.80989957516688));
#94103=CARTESIAN_POINT('',(-2.41674687579388,5.00000000018585,6.83533719297713));
#94104=CARTESIAN_POINT('Ctrl Pts',(-2.41674687553562,5.00000000024666,6.83533719256134));
#94105=CARTESIAN_POINT('Ctrl Pts',(-2.37726401472209,4.99124724464907,6.85858075086912));
#94106=CARTESIAN_POINT('Ctrl Pts',(-2.33753502535484,4.98253936723008,6.8814198933422));
#94107=CARTESIAN_POINT('Ctrl Pts',(-2.25731838756175,4.96515485080288,6.92643749957918));
#94108=CARTESIAN_POINT('Ctrl Pts',(-2.21628201016599,4.95636631379398,6.94889227342396));
#94109=CARTESIAN_POINT('Ctrl Pts',(-2.17698718426122,4.94797317482836,6.96995857628212));
#94110=CARTESIAN_POINT('',(-2.12568306502001,4.95523000036473,6.97819037105365));
#94111=CARTESIAN_POINT('Ctrl Pts',(-2.12568306502001,4.95523000036473,6.97819037105365));
#94112=CARTESIAN_POINT('Ctrl Pts',(-2.17426925953366,4.96260329931481,6.95568233351109));
#94113=CARTESIAN_POINT('Ctrl Pts',(-2.22321605556432,4.97005789395287,6.9323710303661));
#94114=CARTESIAN_POINT('Ctrl Pts',(-2.32054958513549,4.98502388845175,6.88460547908258));
#94115=CARTESIAN_POINT('Ctrl Pts',(-2.3687908093894,4.9925027842392,6.86024488683704));
#94116=CARTESIAN_POINT('Ctrl Pts',(-2.4167468754063,5.0000000000855,6.83533719277799));
#94117=CARTESIAN_POINT('',(-1.80922555581647,5.00000000114933,7.02062695820467));
#94118=CARTESIAN_POINT('Origin',(-1.01339706190693,5.12365837744257,-0.269246995538954));
#94119=CARTESIAN_POINT('',(-2.07779985458226,4.94797317377022,7.0001673937011));
#94120=CARTESIAN_POINT('Origin',(-1.50896214363388,5.49705211430466,-0.024090086241163));
#94121=CARTESIAN_POINT('',(-1.37879884640616,4.84409946429526,7.27641920768044));
#94122=CARTESIAN_POINT('Ctrl Pts',(-1.37879884640616,4.84409946429526,7.27641920768044));
#94123=CARTESIAN_POINT('Ctrl Pts',(-1.49752260815187,4.86143878565642,7.23627453393968));
#94124=CARTESIAN_POINT('Ctrl Pts',(-1.61521158749359,4.87877094692771,7.1931576498776));
#94125=CARTESIAN_POINT('Ctrl Pts',(-1.79015362269918,4.90476414598114,7.12402312386852));
#94126=CARTESIAN_POINT('Ctrl Pts',(-1.84824454389819,4.9134341062347,7.10021529966484));
#94127=CARTESIAN_POINT('Ctrl Pts',(-1.93484159592898,4.92641824534835,7.0634410133741));
#94128=CARTESIAN_POINT('Ctrl Pts',(-1.96357743143852,4.93073677828957,7.0510239732327));
#94129=CARTESIAN_POINT('Ctrl Pts',(-2.02058510409539,4.93932419691696,7.02596309323285));
#94130=CARTESIAN_POINT('Ctrl Pts',(-2.04802232781495,4.94346636781934,7.01370714941363));
#94131=CARTESIAN_POINT('Ctrl Pts',(-2.07779985420982,4.9479731742092,7.00016739302812));
#94132=CARTESIAN_POINT('',(-0.627755369881773,4.94797317385797,7.27499271230061));
#94133=CARTESIAN_POINT('Ctrl Pts',(-0.627755369794896,4.94797317343625,
7.27499271281768));
#94134=CARTESIAN_POINT('Ctrl Pts',(-0.752787502800013,4.93049584999059,
7.28174602429238));
#94135=CARTESIAN_POINT('Ctrl Pts',(-0.877986190217805,4.91309421479666,
7.28523925933799));
#94136=CARTESIAN_POINT('Ctrl Pts',(-1.12846217199833,4.87845834286738,7.28571098880058));
#94137=CARTESIAN_POINT('Ctrl Pts',(-1.2536903397881,4.86123089197091,7.28268957417498));
#94138=CARTESIAN_POINT('Ctrl Pts',(-1.37879884640616,4.84409946429526,7.27641920768044));
#94139=CARTESIAN_POINT('',(-0.890849230764476,5.00000000015126,7.19505994779791));
#94140=CARTESIAN_POINT('Ctrl Pts',(-0.890849230588139,5.0000000002171,7.19505994729805));
#94141=CARTESIAN_POINT('Ctrl Pts',(-0.847292775126946,4.99124724379543,
7.20927243748423));
#94142=CARTESIAN_POINT('Ctrl Pts',(-0.803582888665312,4.98253936671115,
7.22303705456792));
#94143=CARTESIAN_POINT('Ctrl Pts',(-0.715564210890097,4.96515484899948,
7.24975797013115));
#94144=CARTESIAN_POINT('Ctrl Pts',(-0.670660129606432,4.95636631231393,
7.26286615515939));
#94145=CARTESIAN_POINT('Ctrl Pts',(-0.627755369455795,4.94797317481926,
7.2749927114588));
#94146=CARTESIAN_POINT('',(-0.575881119919221,4.95523000034009,7.27200318231908));
#94147=CARTESIAN_POINT('Ctrl Pts',(-0.575881119919222,4.95523000034009,
7.27200318231908));
#94148=CARTESIAN_POINT('Ctrl Pts',(-0.628166812764969,4.96260285567682,
7.2604666599647));
#94149=CARTESIAN_POINT('Ctrl Pts',(-0.680986903378122,4.97005835659053,
7.24822098699053));
#94150=CARTESIAN_POINT('Ctrl Pts',(-0.786309752028458,4.98502388806966,
7.2224967953507));
#94151=CARTESIAN_POINT('Ctrl Pts',(-0.838659931539472,4.99250278402759,
7.20907617718386));
#94152=CARTESIAN_POINT('Ctrl Pts',(-0.890849230400931,5.00000000004258,
7.19505994749707));
#94153=CARTESIAN_POINT('',(-0.257699599156794,5.00000000131521,7.24541861504245));
#94154=CARTESIAN_POINT('Origin',(-1.04758446035831,5.12365828658895,-0.0451006802085374));
#94155=CARTESIAN_POINT('',(-0.524392983891646,4.94797317434015,7.28317291923316));
#94156=CARTESIAN_POINT('Origin',(-1.47886142963726,5.4970517149711,0.300859522968813));
#94157=CARTESIAN_POINT('',(-2.18488949210674E-10,4.87444016471971,7.37555983528029));
#94158=CARTESIAN_POINT('Ctrl Pts',(-0.524392986567054,4.94797317482107,
7.28317291784782));
#94159=CARTESIAN_POINT('Ctrl Pts',(-0.492420047419541,4.94346905243022,
7.28999077156774));
#94160=CARTESIAN_POINT('Ctrl Pts',(-0.463017454517293,4.93933079581677,
7.29605638350877));
#94161=CARTESIAN_POINT('Ctrl Pts',(-0.40199585152166,4.93074907816145,7.30826883136319));
#94162=CARTESIAN_POINT('Ctrl Pts',(-0.371284574090945,4.92643363271708,
7.31421437766545));
#94163=CARTESIAN_POINT('Ctrl Pts',(-0.278873190275588,4.91345879508931,
7.33150237970099));
#94164=CARTESIAN_POINT('Ctrl Pts',(-0.217066998849999,4.90479505377733,
7.34225971987183));
#94165=CARTESIAN_POINT('Ctrl Pts',(-0.103503078100512,4.88890015931504,
7.36055436914659));
#94166=CARTESIAN_POINT('Ctrl Pts',(-0.0517890764005938,4.88167113576107,
7.36832886423586));
#94167=CARTESIAN_POINT('Ctrl Pts',(-4.36966868262861E-10,4.87444016471971,
7.37555983528029));
#94168=CARTESIAN_POINT('',(-1.03732965834111E-14,5.50000000000001,6.74999999999999));
#94169=CARTESIAN_POINT('',(-1.03732965834111E-14,5.5,6.75));
#94170=CARTESIAN_POINT('Origin',(0.,5.5,0.));
#94171=CARTESIAN_POINT('',(0.21765174428364,4.84409946429302,7.40270156517168));
#94172=CARTESIAN_POINT('Ctrl Pts',(-4.36966868262861E-10,4.87444016471971,
7.37555983528029));
#94173=CARTESIAN_POINT('Ctrl Pts',(0.07241494809842,4.86432933756015,7.38567066244414));
#94174=CARTESIAN_POINT('Ctrl Pts',(0.144966842395702,4.85421607421616,7.39471764056659));
#94175=CARTESIAN_POINT('Ctrl Pts',(0.217651744283678,4.84409946429301,7.40270156517169));
#94176=CARTESIAN_POINT('',(0.950829587222573,4.94797317382581,7.23985627382323));
#94177=CARTESIAN_POINT('Ctrl Pts',(0.950829587406162,4.94797317340535,7.23985627426545));
#94178=CARTESIAN_POINT('Ctrl Pts',(0.830172398471133,4.93049584997117,7.27332990973079));
#94179=CARTESIAN_POINT('Ctrl Pts',(0.708651729226591,4.91309421479886,7.30365549178332));
#94180=CARTESIAN_POINT('Ctrl Pts',(0.46413314457925,4.8784583428577,7.35796112453704));
#94181=CARTESIAN_POINT('Ctrl Pts',(0.341183226959201,4.86123089195753,7.38193070325828));
#94182=CARTESIAN_POINT('Ctrl Pts',(0.217651744283639,4.84409946429302,7.40270156517168));
#94183=CARTESIAN_POINT('',(0.676703532269286,5.00000000025134,7.21834969580106));
#94184=CARTESIAN_POINT('Ctrl Pts',(0.676703532319703,5.0000000003026,7.21834969539148));
#94185=CARTESIAN_POINT('Ctrl Pts',(0.722296915759018,4.99124724609782,7.22286655391651));
#94186=CARTESIAN_POINT('Ctrl Pts',(0.767943881459432,4.9825393678581,7.22691302904827));
#94187=CARTESIAN_POINT('Ctrl Pts',(0.8596489367427,4.96515485059302,7.23408781029232));
#94188=CARTESIAN_POINT('Ctrl Pts',(0.906321056460437,4.95636631402168,7.23723648333365));
#94189=CARTESIAN_POINT('Ctrl Pts',(0.950829587450824,4.94797317474932,7.23985627290408));
#94190=CARTESIAN_POINT('',(1.00084838567572,4.95523000033943,7.22578520694037));
#94191=CARTESIAN_POINT('Ctrl Pts',(1.00084838567572,4.95523000033943,7.22578520694036));
#94192=CARTESIAN_POINT('Ctrl Pts',(0.947301871009143,4.96260329913093,7.22575827892429));
#94193=CARTESIAN_POINT('Ctrl Pts',(0.89309079863658,4.97005789396946,7.22515373936875));
#94194=CARTESIAN_POINT('Ctrl Pts',(0.78469704089313,4.98502388909517,7.22267218727446));
#94195=CARTESIAN_POINT('Ctrl Pts',(0.730685746439649,4.9925027846105,7.22081907683343));
#94196=CARTESIAN_POINT('Ctrl Pts',(0.676703532495354,5.00000000016673,7.21834969551148));
#94197=CARTESIAN_POINT('',(1.30587610327248,5.00000000125165,7.13142255059264));
#94198=CARTESIAN_POINT('Origin',(-1.03278734186302,5.12365720261328,0.181154547137244));
#94199=CARTESIAN_POINT('',(1.05353392264426,4.94797317373232,7.22562537403499));
#94200=CARTESIAN_POINT('Origin',(-1.37961143582091,5.49705145501706,0.611734678451162));
#94201=CARTESIAN_POINT('',(1.80392518127354,4.84409946430028,7.18284182514446));
#94202=CARTESIAN_POINT('Ctrl Pts',(1.80392518127354,4.84409946430028,7.18284182514446));
#94203=CARTESIAN_POINT('Ctrl Pts',(1.67931810259866,4.86143878568035,7.19625831959543));
#94204=CARTESIAN_POINT('Ctrl Pts',(1.55440216827193,4.87877094696219,7.20654281518377));
#94205=CARTESIAN_POINT('Ctrl Pts',(1.36660024350474,4.90476414601202,7.21725427266271));
#94206=CARTESIAN_POINT('Ctrl Pts',(1.30388170545924,4.91343410626486,7.22003862132074));
#94207=CARTESIAN_POINT('Ctrl Pts',(1.20984722770454,4.92641824536596,7.22302434137574));
#94208=CARTESIAN_POINT('Ctrl Pts',(1.17855350996234,4.930736778299,7.22382080511211));
#94209=CARTESIAN_POINT('Ctrl Pts',(1.11628883152147,4.93932462802435,7.22501312674049));
#94210=CARTESIAN_POINT('Ctrl Pts',(1.08624830934207,4.94346583885495,7.22541043952854));
#94211=CARTESIAN_POINT('Ctrl Pts',(1.05353392271017,4.94797317423728,7.22562537347857));
#94212=CARTESIAN_POINT('',(2.48495480999609,4.94797317381999,6.86619220270977));
#94213=CARTESIAN_POINT('Ctrl Pts',(2.48495481024058,4.94797317330798,6.86619220301851));
#94214=CARTESIAN_POINT('Ctrl Pts',(2.37431436120362,4.93049584986762,6.92482097261293));
#94215=CARTESIAN_POINT('Ctrl Pts',(2.26215388175163,4.91309421478555,6.98056091095388));
#94216=CARTESIAN_POINT('Ctrl Pts',(2.03502611120553,4.8784583428514,7.08616117604617));
#94217=CARTESIAN_POINT('Ctrl Pts',(1.92010344521286,4.86123089196737,7.13600095723115));
#94218=CARTESIAN_POINT('Ctrl Pts',(1.80392518127354,4.84409946430028,7.18284182514446));
#94219=CARTESIAN_POINT('',(2.21261439168749,5.00000000026428,6.90411743489196));
#94220=CARTESIAN_POINT('Ctrl Pts',(2.21261439165011,5.00000000031365,6.90411743449623));
#94221=CARTESIAN_POINT('Ctrl Pts',(2.25811281635062,4.99124724655127,6.8987274617925));
#94222=CARTESIAN_POINT('Ctrl Pts',(2.3035624540921,4.98253936819152,6.89286658436005));
#94223=CARTESIAN_POINT('Ctrl Pts',(2.39466586712529,4.96515484985945,6.88015974650244));
#94224=CARTESIAN_POINT('Ctrl Pts',(2.44092369359696,4.95636631272802,6.87320167850187));
#94225=CARTESIAN_POINT('Ctrl Pts',(2.48495480999432,4.94797317483196,6.86619220148691));
#94226=CARTESIAN_POINT('',(2.53077933337913,4.95523000032694,6.84169754621404));
#94227=CARTESIAN_POINT('Ctrl Pts',(2.53077933337913,4.95523000032694,6.84169754621403));
#94228=CARTESIAN_POINT('Ctrl Pts',(2.47848205792871,4.96260285641261,6.85318147604075));
#94229=CARTESIAN_POINT('Ctrl Pts',(2.42540202043434,4.97005835700181,6.86424618380204));
#94230=CARTESIAN_POINT('Ctrl Pts',(2.31901227904161,4.98502388922639,6.88512345703757));
#94231=CARTESIAN_POINT('Ctrl Pts',(2.26586537514055,4.99250278466233,6.89492450294757));
#94232=CARTESIAN_POINT('Ctrl Pts',(2.21261439184018,5.00000000018279,6.90411743457274));
#94233=CARTESIAN_POINT('',(2.80839049007527,5.00000000117302,6.68396909420632));
#94234=CARTESIAN_POINT('Origin',(-0.969699637310454,5.12365838153926,0.398936247790705));
#94235=CARTESIAN_POINT('',(2.58219875254243,4.94797317374736,6.83021561692927));
#94236=CARTESIAN_POINT('Origin',(-1.2158521634837,5.4970520772469,0.894008300633824));
#94237=CARTESIAN_POINT('',(3.30584908222536,4.84409946430701,6.62712038446017));
#94238=CARTESIAN_POINT('Ctrl Pts',(3.30584908222536,4.84409946430701,6.62712038446016));
#94239=CARTESIAN_POINT('Ctrl Pts',(3.18703939746008,4.86143878569,6.6670100473131));
#94240=CARTESIAN_POINT('Ctrl Pts',(3.06725479073445,4.8787709469758,6.70390733053034));
#94241=CARTESIAN_POINT('Ctrl Pts',(2.88614621716508,4.90476414603823,6.75474022258351));
#94242=CARTESIAN_POINT('Ctrl Pts',(2.82549255623583,4.913434106302,6.77094210648112));
#94243=CARTESIAN_POINT('Ctrl Pts',(2.73429839376083,4.92641824541161,6.79407265516783));
#94244=CARTESIAN_POINT('Ctrl Pts',(2.70390752190762,4.93073677834248,6.80157772230459));
#94245=CARTESIAN_POINT('Ctrl Pts',(2.6433579107688,4.93932419694258,6.81612650304836));
#94246=CARTESIAN_POINT('Ctrl Pts',(2.61409834609453,4.94346636783281,6.82297393148364));
#94247=CARTESIAN_POINT('Ctrl Pts',(2.58219875249933,4.94797317419847,6.83021561645868));
#94248=CARTESIAN_POINT('',(3.90288630848711,4.94797317379406,6.17147261466615));
#94249=CARTESIAN_POINT('Ctrl Pts',(3.90288630880333,4.94797317338954,6.17147261495134));
#94250=CARTESIAN_POINT('Ctrl Pts',(3.80743602447103,4.93049584997553,6.2525151024618));
#94251=CARTESIAN_POINT('Ctrl Pts',(3.70988023341334,4.91309421482796,6.33106305997198));
#94252=CARTESIAN_POINT('Ctrl Pts',(3.51076351938066,4.87845834288964,6.48302020640452));
#94253=CARTESIAN_POINT('Ctrl Pts',(3.40924176104253,4.86123089198511,6.55639973739089));
#94254=CARTESIAN_POINT('Ctrl Pts',(3.30584908222535,4.84409946430701,6.62712038446016));
#94255=CARTESIAN_POINT('',(3.64506586129705,5.00000000025158,6.26705631602723));
#94256=CARTESIAN_POINT('Ctrl Pts',(3.64506586117092,5.00000000030281,6.2670563156346));
#94257=CARTESIAN_POINT('Ctrl Pts',(3.68834187479224,4.99124724618209,6.25201154058592));
#94258=CARTESIAN_POINT('Ctrl Pts',(3.73146900939394,4.98253936797242,6.23651735865113));
#94259=CARTESIAN_POINT('Ctrl Pts',(3.81771087915457,4.96515484992084,6.20452305941057));
#94260=CARTESIAN_POINT('Ctrl Pts',(3.86139143710234,4.95636631419786,6.18778360482291));
#94261=CARTESIAN_POINT('Ctrl Pts',(3.90288630830385,4.94797317467443,6.17147261374693));
#94262=CARTESIAN_POINT('',(3.94237385257086,4.95523000032935,6.13769971199802));
#94263=CARTESIAN_POINT('Ctrl Pts',(3.94237385257086,4.95523000032935,6.13769971199802));
#94264=CARTESIAN_POINT('Ctrl Pts',(3.89376504504097,4.96260329920329,6.16015887077973));
#94265=CARTESIAN_POINT('Ctrl Pts',(3.84431056932647,4.97005789391054,6.18237284378588));
#94266=CARTESIAN_POINT('Ctrl Pts',(3.74489308220244,4.98502388904853,6.22563400581526));
#94267=CARTESIAN_POINT('Ctrl Pts',(3.69509565814041,4.99250278455262,6.24663092222021));
#94268=CARTESIAN_POINT('Ctrl Pts',(3.64506586138057,5.00000000016703,6.26705631566973));
#94269=CARTESIAN_POINT('',(4.17958766035098,5.00000000132489,5.92398067006497));
#94270=CARTESIAN_POINT('Origin',(-0.861267622003431,5.12365714954158,0.598067515194973));
#94271=CARTESIAN_POINT('',(3.99012283826856,4.94797317375666,6.11543256900459));
#94272=CARTESIAN_POINT('Origin',(-0.995240108880086,5.49705150748935,1.1344797623526));
#94273=CARTESIAN_POINT('',(4.65319515431945,4.84409946436975,5.76152215993885));
#94274=CARTESIAN_POINT('Ctrl Pts',(4.65319515431945,4.84409946436975,5.76152215993884));
#94275=CARTESIAN_POINT('Ctrl Pts',(4.54573827233818,4.86143878572445,5.82601979492307));
#94276=CARTESIAN_POINT('Ctrl Pts',(4.43668598835844,4.8787709469975,5.88780458982905));
#94277=CARTESIAN_POINT('Ctrl Pts',(4.27073920175616,4.90476414605707,5.97638202692489));
#94278=CARTESIAN_POINT('Ctrl Pts',(4.21498651582412,4.91343410632183,6.00524386397367));
#94279=CARTESIAN_POINT('Ctrl Pts',(4.13089680641441,4.92641824543627,6.04743768254098));
#94280=CARTESIAN_POINT('Ctrl Pts',(4.10282982383664,4.93073677836966,6.06130042448136));
#94281=CARTESIAN_POINT('Ctrl Pts',(4.0468205750289,4.93932462809372,6.08852680617075));
#94282=CARTESIAN_POINT('Ctrl Pts',(4.01972336279107,4.94346583892761,6.10150108536912));
#94283=CARTESIAN_POINT('Ctrl Pts',(3.99012283811852,4.94797317429759,6.11543256851079));
#94284=CARTESIAN_POINT('',(5.13832317951413,4.94797317385176,5.18818182713878));
#94285=CARTESIAN_POINT('Ctrl Pts',(5.13832317996159,4.94797317343003,5.18818182740512));
#94286=CARTESIAN_POINT('Ctrl Pts',(5.06252620966765,4.93049584998606,5.28784857604244));
#94287=CARTESIAN_POINT('Ctrl Pts',(4.9841367078042,4.91309421480021,5.38553173733754));
#94288=CARTESIAN_POINT('Ctrl Pts',(4.82234152687057,4.87845834289208,5.5767404174663));
#94289=CARTESIAN_POINT('Ctrl Pts',(4.73896772101397,4.86123089201307,5.67022855275052));
#94290=CARTESIAN_POINT('Ctrl Pts',(4.65319515431944,4.84409946436975,5.76152215993884));
#94291=CARTESIAN_POINT('',(4.90707810144186,5.00000000032828,5.3369546096604));
#94292=CARTESIAN_POINT('Ctrl Pts',(4.90707810127956,5.00000000036833,5.3369546093818));
#94293=CARTESIAN_POINT('Ctrl Pts',(4.94610815640319,4.99124724787197,5.31295851374921));
#94294=CARTESIAN_POINT('Ctrl Pts',(4.98489621575647,4.98253936874299,5.28855551546913));
#94295=CARTESIAN_POINT('Ctrl Pts',(5.06224396652565,4.96515485157286,5.2387697744877));
#94296=CARTESIAN_POINT('Ctrl Pts',(5.10130481486224,4.95636631445717,5.21303164702084));
#94297=CARTESIAN_POINT('Ctrl Pts',(5.13832317915037,4.94797317480355,5.18818182627541));
#94298=CARTESIAN_POINT('',(5.1696273514169,4.95523000038885,5.14670986113548));
#94299=CARTESIAN_POINT('Ctrl Pts',(5.1696273514169,4.95523000038884,5.14670986113548));
#94300=CARTESIAN_POINT('Ctrl Pts',(5.12698560699481,4.96260285639141,5.17909144937227));
#94301=CARTESIAN_POINT('Ctrl Pts',(5.083457419883,4.97005835694427,5.21142123548925));
#94302=CARTESIAN_POINT('Ctrl Pts',(4.99566684113432,4.9850238898458,5.27504083139195));
#94303=CARTESIAN_POINT('Ctrl Pts',(4.95154737149327,4.99250278501308,5.30625182423134));
#94304=CARTESIAN_POINT('Ctrl Pts',(4.90707810144554,5.00000000026218,5.33695460937339));
#94305=CARTESIAN_POINT('',(5.3553519559481,5.00000000121457,4.88699349554604));
#94306=CARTESIAN_POINT('Origin',(-0.712566840944546,5.12365847699368,0.769230858395806));
#94307=CARTESIAN_POINT('',(5.21147321561416,4.94797317373827,5.11469869085934));
#94308=CARTESIAN_POINT('Origin',(-0.728094867478207,5.49705211887932,1.3219019862453));
#94309=CARTESIAN_POINT('',(5.78296299265857,4.84409946425117,4.62652156278843));
#94310=CARTESIAN_POINT('Ctrl Pts',(5.78296299265856,4.84409946425117,4.62652156278842));
#94311=CARTESIAN_POINT('Ctrl Pts',(5.69188347782073,4.86143878560935,4.71261133216591));
#94312=CARTESIAN_POINT('Ctrl Pts',(5.59866268018144,4.87877094687763,4.79639465042542));
#94313=CARTESIAN_POINT('Ctrl Pts',(5.45563716790461,4.90476414592899,4.9185748500168));
#94314=CARTESIAN_POINT('Ctrl Pts',(5.40739239066292,4.91343410618348,4.95874709274369));
#94315=CARTESIAN_POINT('Ctrl Pts',(5.33433907571752,4.92641824529631,5.01803124509864));
#94316=CARTESIAN_POINT('Ctrl Pts',(5.30990836331075,4.93073677823582,5.03760345545227));
#94317=CARTESIAN_POINT('Ctrl Pts',(5.26106389895748,4.93932419686102,5.07623169312291));
#94318=CARTESIAN_POINT('Ctrl Pts',(5.23738379781279,4.94346636776206,5.09473202319924));
#94319=CARTESIAN_POINT('Ctrl Pts',(5.21147321523184,4.94797317415825,5.11469869026842));
#94320=CARTESIAN_POINT('',(6.13349777051141,4.9479731738001,3.96229742335492));
#94321=CARTESIAN_POINT('Ctrl Pts',(6.13349777089164,4.9479731733255,3.96229742345793));
#94322=CARTESIAN_POINT('Ctrl Pts',(6.08089829633568,4.93049584987379,4.07592812719467));
#94323=CARTESIAN_POINT('Ctrl Pts',(6.025340489868,4.91309421476424,4.18817893573079));
#94324=CARTESIAN_POINT('Ctrl Pts',(5.90843220440268,4.87845834281139,4.40969844464914));
#94325=CARTESIAN_POINT('Ctrl Pts',(5.84710481743528,4.86123089191899,4.51892378299799));
#94326=CARTESIAN_POINT('Ctrl Pts',(5.78296299265856,4.84409946425117,4.62652156278842));
#94327=CARTESIAN_POINT('',(5.93964082487683,5.00000000023931,4.15730283636664));
#94328=CARTESIAN_POINT('Ctrl Pts',(5.93964082458775,5.00000000029233,4.15730283605268));
#94329=CARTESIAN_POINT('Ctrl Pts',(5.97259993462298,4.99124724583479,4.12547744086007));
#94330=CARTESIAN_POINT('Ctrl Pts',(6.00523522309373,4.9825393678026,4.09330668903726));
#94331=CARTESIAN_POINT('Ctrl Pts',(6.07007216271111,4.9651548509353,4.02805743204809));
#94332=CARTESIAN_POINT('Ctrl Pts',(6.10268685331395,4.95636631401737,3.99452411977945));
#94333=CARTESIAN_POINT('Ctrl Pts',(6.13349776983711,4.94797317475143,3.96229742246247));
#94334=CARTESIAN_POINT('',(6.15515482124631,4.95523000034099,3.91506557728136));
#94335=CARTESIAN_POINT('Ctrl Pts',(6.15515482124631,4.95523000034099,3.91506557728135));
#94336=CARTESIAN_POINT('Ctrl Pts',(6.12047100548719,4.96260287679691,3.95585692921522));
#94337=CARTESIAN_POINT('Ctrl Pts',(6.08491047859624,4.97005836655391,3.99678807609253));
#94338=CARTESIAN_POINT('Ctrl Pts',(6.01284887492248,4.98502386882789,4.07779249461766));
#94339=CARTESIAN_POINT('Ctrl Pts',(5.97647028764588,4.99250277458103,4.11775823167738));
#94340=CARTESIAN_POINT('Ctrl Pts',(5.9396408246448,5.00000000018339,4.15730283616115));
#94341=CARTESIAN_POINT('',(6.28070594613454,5.00000000118451,3.62149593580336));
#94342=CARTESIAN_POINT('Origin',(-0.53054494989452,5.12365811164979,0.904427678178179));
#94343=CARTESIAN_POINT('',(6.18914089681808,4.94797317372704,3.87480718636556));
#94344=CARTESIAN_POINT('Origin',(-0.426900607566502,5.4970516443896,1.44751614087276));
#94345=CARTESIAN_POINT('',(6.64232590857355,4.8440994642892,3.2751899592442));
#94346=CARTESIAN_POINT('Ctrl Pts',(6.64232590857354,4.8440994642892,3.27518995924419));
#94347=CARTESIAN_POINT('Ctrl Pts',(6.57188253777224,4.861438785675,3.37884640105228));
#94348=CARTESIAN_POINT('Ctrl Pts',(6.49885212737317,4.87877094694699,3.48071062781813));
#94349=CARTESIAN_POINT('Ctrl Pts',(6.38543560335193,4.90476414598776,3.63078057965921));
#94350=CARTESIAN_POINT('Ctrl Pts',(6.34695460686237,4.91343410624046,3.6803848187376));
#94351=CARTESIAN_POINT('Ctrl Pts',(6.28835357812894,4.92641824534208,3.75398724388821));
#94352=CARTESIAN_POINT('Ctrl Pts',(6.26870148888606,4.93073677827376,3.778353747841));
#94353=CARTESIAN_POINT('Ctrl Pts',(6.22930291024878,4.939324196881,3.82657899477485));
#94354=CARTESIAN_POINT('Ctrl Pts',(6.21015346081782,4.94346636777425,3.84973731918386));
#94355=CARTESIAN_POINT('Ctrl Pts',(6.18914089648487,4.9479731741602,3.87480718600841));
#94356=CARTESIAN_POINT('',(6.84187682255284,4.94797317381414,2.55114039475589));
#94357=CARTESIAN_POINT('Ctrl Pts',(6.84187682304406,4.94797317344389,2.5511403948112));
#94358=CARTESIAN_POINT('Ctrl Pts',(6.8149343374485,4.93049585000131,2.6734218078687));
#94359=CARTESIAN_POINT('Ctrl Pts',(6.78480604719052,4.91309421480685,2.79499154164727));
#94360=CARTESIAN_POINT('Ctrl Pts',(6.71825115882247,4.87845834287996,3.03646387312177));
#94361=CARTESIAN_POINT('Ctrl Pts',(6.68183779109199,4.86123089197961,3.15631915928958));
#94362=CARTESIAN_POINT('Ctrl Pts',(6.64232590857354,4.8440994642892,3.27518995924419));
#94363=CARTESIAN_POINT('',(6.69447254313508,5.00000000036334,2.78326020476335));
#94364=CARTESIAN_POINT('Ctrl Pts',(6.69447254290451,5.00000000039828,2.78326020460221));
#94365=CARTESIAN_POINT('Ctrl Pts',(6.71981956014049,4.99124724875399,2.74509364678722));
#94366=CARTESIAN_POINT('Ctrl Pts',(6.74477609751374,4.98253936923545,2.70665940034705));
#94367=CARTESIAN_POINT('Ctrl Pts',(6.79407052861097,4.96515485071796,2.62899760210498));
#94368=CARTESIAN_POINT('Ctrl Pts',(6.81871403470949,4.95636631384115,2.58923708620832));
#94369=CARTESIAN_POINT('Ctrl Pts',(6.8418768219553,4.94797317467669,2.55114039420255));
#94370=CARTESIAN_POINT('',(6.85287409254451,4.95523000036724,2.50035717833961));
#94371=CARTESIAN_POINT('Ctrl Pts',(6.8528740925445,4.95523000036724,2.50035717833961));
#94372=CARTESIAN_POINT('Ctrl Pts',(6.82776866029154,4.96260329966329,2.54765355854871));
#94373=CARTESIAN_POINT('Ctrl Pts',(6.80184162012553,4.97005789398453,2.5952665193949));
#94374=CARTESIAN_POINT('Ctrl Pts',(6.74887658391066,4.98502389023629,2.68987133710622));
#94375=CARTESIAN_POINT('Ctrl Pts',(6.72193999400436,4.99250278523982,2.7367229505189));
#94376=CARTESIAN_POINT('Ctrl Pts',(6.69447254303287,5.00000000030567,2.78326020453474));
#94377=CARTESIAN_POINT('',(6.91238110702276,5.00000000129598,2.18666125068283));
#94378=CARTESIAN_POINT('Origin',(-0.323716134246077,5.12365830463126,0.997334119173099));
#94379=CARTESIAN_POINT('',(6.87741122879209,4.94797317381514,2.45373400464787));
#94380=CARTESIAN_POINT('Origin',(-0.10574754861476,5.49705229109587,1.50544504490825));
#94381=CARTESIAN_POINT('',(7.19110104734923,4.84409946426157,1.77071411358907));
#94382=CARTESIAN_POINT('Ctrl Pts',(7.19110104734922,4.84409946426157,1.77071411358906));
#94383=CARTESIAN_POINT('Ctrl Pts',(7.14458767434116,4.86143878562981,1.88709036787101));
#94384=CARTESIAN_POINT('Ctrl Pts',(7.09516247199227,4.87877094691969,2.00227244512627));
#94385=CARTESIAN_POINT('Ctrl Pts',(7.01665816682038,4.90476414601387,2.17321504499532));
#94386=CARTESIAN_POINT('Ctrl Pts',(6.98974027973458,4.91343410628763,2.22993184127428));
#94387=CARTESIAN_POINT('Ctrl Pts',(6.94833165618154,4.92641824542731,2.31441097156495));
#94388=CARTESIAN_POINT('Ctrl Pts',(6.93437709992616,4.93073677837388,2.34243241847897));
#94389=CARTESIAN_POINT('Ctrl Pts',(6.90626664071228,4.93932419700383,2.39799971569474));
#94390=CARTESIAN_POINT('Ctrl Pts',(6.89254324996912,4.94346636790369,2.4247331768729));
#94391=CARTESIAN_POINT('Ctrl Pts',(6.87741122807904,4.94797317428302,2.4537340042031));
#94392=CARTESIAN_POINT('',(7.23033731830119,4.94797317377381,1.02069487829441));
#94393=CARTESIAN_POINT('Ctrl Pts',(7.23033731870489,4.94797317337711,1.02069487823912));
#94394=CARTESIAN_POINT('Ctrl Pts',(7.23031162262742,4.93049584992953,1.14590925787838));
#94395=CARTESIAN_POINT('Ctrl Pts',(7.22702161424753,4.91309421478301,1.27111345026311));
#94396=CARTESIAN_POINT('Ctrl Pts',(7.21393215558699,4.87845834284057,1.52124762643535));
#94397=CARTESIAN_POINT('Ctrl Pts',(7.20413545580418,4.86123089194126,1.64612856020698));
#94398=CARTESIAN_POINT('Ctrl Pts',(7.19110104734922,4.84409946426157,1.77071411358906));
#94399=CARTESIAN_POINT('',(7.13627816756702,5.00000000009595,1.27907541649019));
#94400=CARTESIAN_POINT('Ctrl Pts',(7.1362781670175,5.00000000016985,1.27907541626218));
#94401=CARTESIAN_POINT('Ctrl Pts',(7.15282791462048,4.99124724255673,1.23635228273902));
#94402=CARTESIAN_POINT('Ctrl Pts',(7.16893874895024,4.98253936613945,1.19345170510829));
#94403=CARTESIAN_POINT('Ctrl Pts',(7.20038570823038,4.96515485002847,1.10700876358092));
#94404=CARTESIAN_POINT('Ctrl Pts',(7.21590572580901,4.9563663139889,1.06288020482779));
#94405=CARTESIAN_POINT('Ctrl Pts',(7.23033731750308,4.94797317462113,1.02069487785279));
#94406=CARTESIAN_POINT('',(7.23016058785084,4.95523000031898,0.968734856467267));
#94407=CARTESIAN_POINT('Ctrl Pts',(7.23016058785083,4.95523000031898,0.968734856467265));
#94408=CARTESIAN_POINT('Ctrl Pts',(7.21581029494733,4.96260285540334,1.02031929132061));
#94409=CARTESIAN_POINT('Ctrl Pts',(7.20072295871774,4.97005835660489,1.07239895113449));
#94410=CARTESIAN_POINT('Ctrl Pts',(7.16933443085165,4.98502388756489,1.17617465137087));
#94411=CARTESIAN_POINT('Ctrl Pts',(7.15309931311601,4.99250278377018,1.22772147893514));
#94412=CARTESIAN_POINT('Ctrl Pts',(7.13627816725194,4.99999999997397,1.27907541606446));
#94413=CARTESIAN_POINT('',(7.22084100984491,5.00000000122638,0.649580716950613));
#94414=CARTESIAN_POINT('Origin',(-0.101751095987447,5.12365823908661,1.04360640710232));
#94415=CARTESIAN_POINT('',(7.24410145512007,4.94797317373785,0.917926948134186));
#94416=CARTESIAN_POINT('Origin',(0.220349566562635,5.49705203762993,1.49298124256275));
#94417=CARTESIAN_POINT('',(7.40362829344876,4.84409946433362,0.183441643659611));
#94418=CARTESIAN_POINT('Ctrl Pts',(7.40362829344875,4.84409946433362,0.183441643659609));
#94419=CARTESIAN_POINT('Ctrl Pts',(7.38321983188076,4.86143878569194,0.307096086033609));
#94420=CARTESIAN_POINT('Ctrl Pts',(7.35971090518389,4.87877094695177,0.430210227817895));
#94421=CARTESIAN_POINT('Ctrl Pts',(7.31978959305236,4.90476414598828,0.614032389714094));
#94422=CARTESIAN_POINT('Ctrl Pts',(7.3056934658962,4.91343410624058,0.675209728842564));
#94423=CARTESIAN_POINT('Ctrl Pts',(7.28341346881588,4.92641824534731,0.766615414036037));
#94424=CARTESIAN_POINT('Ctrl Pts',(7.27580894512243,4.93073677828274,0.796981552190475));
#94425=CARTESIAN_POINT('Ctrl Pts',(7.26030024063061,4.93932462801487,0.857295662529265));
#94426=CARTESIAN_POINT('Ctrl Pts',(7.25264638036975,4.94346583884927,0.886347499907857));
#94427=CARTESIAN_POINT('Ctrl Pts',(7.24410145445558,4.94797317424166,0.917926947882475));
#94428=CARTESIAN_POINT('',(7.28071527711384,4.94797317386005,-0.557477196754691));
#94429=CARTESIAN_POINT('Ctrl Pts',(7.28071527752219,4.94797317332841,-0.557477196920467));
#94430=CARTESIAN_POINT('Ctrl Pts',(7.30760757251772,4.93049584988333,-0.435184735912635));
#94431=CARTESIAN_POINT('Ctrl Pts',(7.33130968299057,4.9130942147891,-0.3122004936911));
#94432=CARTESIAN_POINT('Ctrl Pts',(7.37229770253631,4.87845834287167,-0.0651004688633301));
#94433=CARTESIAN_POINT('Ctrl Pts',(7.38957575343373,4.86123089199693,0.0589668188442981));
#94434=CARTESIAN_POINT('Ctrl Pts',(7.40362829344875,4.84409946433362,0.183441643659612));
#94435=CARTESIAN_POINT('',(7.24439935455547,5.00000000038041,-0.28491751337921));
#94436=CARTESIAN_POINT('Ctrl Pts',(7.24439935429826,5.00000000041286,-0.284917513425124));
#94437=CARTESIAN_POINT('Ctrl Pts',(7.25137796208485,4.99124724919002,-0.330199477540848));
#94438=CARTESIAN_POINT('Ctrl Pts',(7.25788978100876,4.98253936940856,-0.375560433736857));
#94439=CARTESIAN_POINT('Ctrl Pts',(7.27001885281739,4.96515485016347,-0.466742571032449));
#94440=CARTESIAN_POINT('Ctrl Pts',(7.27568968574208,4.95636631336266,-0.513175778026053));
#94441=CARTESIAN_POINT('Ctrl Pts',(7.28071527589721,4.94797317493522,-0.557477197096403));
#94442=CARTESIAN_POINT('',(7.26937280966497,4.9552300003664,-0.60818443062782));
#94443=CARTESIAN_POINT('Ctrl Pts',(7.26937280966496,4.95523000036639,-0.60818443062782));
#94444=CARTESIAN_POINT('Ctrl Pts',(7.26644714723044,4.96260285571173,-0.554721120165454));
#94445=CARTESIAN_POINT('Ctrl Pts',(7.26290813196574,4.97005835680198,-0.500615723169021));
#94446=CARTESIAN_POINT('Ctrl Pts',(7.25456215699018,4.98502389030606,-0.39251861678044));
#94447=CARTESIAN_POINT('Ctrl Pts',(7.24978765196605,4.99250278526087,-0.338686864118216));
#94448=CARTESIAN_POINT('Ctrl Pts',(7.24439935438014,5.00000000032684,-0.284917513532059));
#94449=CARTESIAN_POINT('',(7.19166241212645,5.00000000121785,-0.917873489557443));
#94450=CARTESIAN_POINT('Origin',(0.124975105914598,5.12365739689806,1.04108015340628));
#94451=CARTESIAN_POINT('',(7.27206554876221,4.94797317374701,-0.660801352633178));
#94452=CARTESIAN_POINT('Origin',(0.536147021643578,5.49705179128573,1.41070678503679));
#94453=CARTESIAN_POINT('',(7.26997010912512,4.84409946433572,-1.41240835333832));
#94454=CARTESIAN_POINT('Ctrl Pts',(7.26997010912511,4.84409946433571,-1.41240835333831));
#94455=CARTESIAN_POINT('Ctrl Pts',(7.27662083595686,4.86143878568868,-1.28725766717237));
#94456=CARTESIAN_POINT('Ctrl Pts',(7.2801274361364,4.87877094696363,-1.16196814131573));
#94457=CARTESIAN_POINT('Ctrl Pts',(7.28065579313712,4.90476414601994,-0.973861737398919));
#94458=CARTESIAN_POINT('Ctrl Pts',(7.28004054511674,4.91343410627963,-0.9110844398));
#94459=CARTESIAN_POINT('Ctrl Pts',(7.27793096236606,4.92641824539027,-0.817026227957172));
#94460=CARTESIAN_POINT('Ctrl Pts',(7.27703205029688,4.93073677832517,-0.785735285440253));
#94461=CARTESIAN_POINT('Ctrl Pts',(7.27485168155049,4.93932462805329,-0.723497372470726));
#94462=CARTESIAN_POINT('Ctrl Pts',(7.27362205056032,4.9434658388885,-0.693479397176331));
#94463=CARTESIAN_POINT('Ctrl Pts',(7.27206554810619,4.94797317426655,-0.660801352736085));
#94464=CARTESIAN_POINT('',(6.99065508110836,4.94797317379603,-2.10958225861235));
#94465=CARTESIAN_POINT('Ctrl Pts',(6.9906550815225,4.94797317344677,-2.10958225885756));
#94466=CARTESIAN_POINT('Ctrl Pts',(7.04320791370601,4.93049585004491,-1.99592997627474));
#94467=CARTESIAN_POINT('Ctrl Pts',(7.09279385896656,4.91309421486669,-1.88091628978998));
#94468=CARTESIAN_POINT('Ctrl Pts',(7.18594280252527,4.8784583429496,-1.6484045388198));
#94469=CARTESIAN_POINT('Ctrl Pts',(7.22948770172626,4.86123089204045,-1.53095214538267));
#94470=CARTESIAN_POINT('Ctrl Pts',(7.26997010912511,4.84409946433571,-1.41240835333831));
#94471=CARTESIAN_POINT('',(7.01378048014667,5.00000000026952,-1.83558801947581));
#94472=CARTESIAN_POINT('Ctrl Pts',(7.01378047975564,5.00000000031813,-1.83558801946016));
#94473=CARTESIAN_POINT('Ctrl Pts',(7.01086164706033,4.99124724655311,-1.88131152369201));
#94474=CARTESIAN_POINT('Ctrl Pts',(7.00746995880966,4.98253936810556,-1.92701180779298));
#94475=CARTESIAN_POINT('Ctrl Pts',(6.99971399681033,4.96515485196445,-2.01866953306197));
#94476=CARTESIAN_POINT('Ctrl Pts',(6.99527048224866,4.95636631483061,-2.06523621940693));
#94477=CARTESIAN_POINT('Ctrl Pts',(6.99065508034933,4.9479731746186,-2.10958225868904));
#94478=CARTESIAN_POINT('',(6.96867723835465,4.95523000034217,-2.15666568933291));
#94479=CARTESIAN_POINT('Ctrl Pts',(6.96867723835464,4.95523000034216,-2.1566656893329));
#94480=CARTESIAN_POINT('Ctrl Pts',(6.97731355112746,4.9626033197548,-2.10382006469291));
#94481=CARTESIAN_POINT('Ctrl Pts',(6.98548733530497,4.97005790364313,-2.05022541290881));
#94482=CARTESIAN_POINT('Ctrl Pts',(7.00057460256239,4.98502386914664,-1.94285831994863));
#94483=CARTESIAN_POINT('Ctrl Pts',(7.00748397221452,4.99250277474619,-1.88925867215296));
#94484=CARTESIAN_POINT('Ctrl Pts',(7.01378047986531,5.00000000021824,-1.83558801943564));
#94485=CARTESIAN_POINT('',(6.82620967368096,5.00000000114615,-2.44240895163504));
#94486=CARTESIAN_POINT('Origin',(0.345853143282498,5.12365841010391,0.989875246164395));
#94487=CARTESIAN_POINT('',(6.95999593981941,4.94797317380956,-2.20863131600617));
#94488=CARTESIAN_POINT('Origin',(0.826872135186473,5.497052011915,1.26246970665074));
#94489=CARTESIAN_POINT('',(6.79637620263612,4.84409946426182,-2.9422157054656));
#94490=CARTESIAN_POINT('Ctrl Pts',(6.79637620263611,4.84409946426182,-2.94221570546559));
#94491=CARTESIAN_POINT('Ctrl Pts',(6.82977513725051,4.86143878564932,-2.82142068241563));
#94492=CARTESIAN_POINT('Ctrl Pts',(6.86013329958665,4.87877094694303,-2.69981417138956));
#94493=CARTESIAN_POINT('Ctrl Pts',(6.9010866203215,4.90476414603892,-2.51621917174387));
#94494=CARTESIAN_POINT('Ctrl Pts',(6.91398101974245,4.91343410631165,-2.45477731233615));
#94495=CARTESIAN_POINT('Ctrl Pts',(6.93214049304112,4.92641824545061,-2.36246463126814));
#94496=CARTESIAN_POINT('Ctrl Pts',(6.93798922471456,4.93073677839702,-2.33171201406331));
#94497=CARTESIAN_POINT('Ctrl Pts',(6.94923914330869,4.93932462815421,-2.27046047403663));
#94498=CARTESIAN_POINT('Ctrl Pts',(6.95449123775758,4.94346583900203,-2.24087996800498));
#94499=CARTESIAN_POINT('Ctrl Pts',(6.95999593906431,4.94797317440998,-2.2086313159612));
#94500=CARTESIAN_POINT('',(6.37371962360107,4.94797317381679,-3.56304559730339));
#94501=CARTESIAN_POINT('Ctrl Pts',(6.37371962396418,4.94797317343968,-3.56304559764541));
#94502=CARTESIAN_POINT('Ctrl Pts',(6.44947568136037,4.93049584998276,-3.46334774781826));
#94503=CARTESIAN_POINT('Ctrl Pts',(6.52262687755466,4.91309421478169,-3.36168252998804));
#94504=CARTESIAN_POINT('Ctrl Pts',(6.66358120398301,4.87845834284509,-3.15463104407018));
#94505=CARTESIAN_POINT('Ctrl Pts',(6.7313568403172,4.8612308919452,-3.04928548853122));
#94506=CARTESIAN_POINT('Ctrl Pts',(6.79637620263611,4.84409946426182,-2.94221570546559));
#94507=CARTESIAN_POINT('',(6.45520502561423,5.00000000025075,-3.30042846896563));
#94508=CARTESIAN_POINT('Ctrl Pts',(6.45520502521441,5.0000000003021,-3.30042846886068));
#94509=CARTESIAN_POINT('Ctrl Pts',(6.44252523076982,4.99124724615799,-3.34445552223589));
#94510=CARTESIAN_POINT('Ctrl Pts',(6.42938862844364,4.98253936795439,-3.38835824515637));
#94511=CARTESIAN_POINT('Ctrl Pts',(6.4021102929694,4.96515485046747,-3.47620576779447));
#94512=CARTESIAN_POINT('Ctrl Pts',(6.38776020295519,4.95636631289811,-3.5207285295106));
#94513=CARTESIAN_POINT('Ctrl Pts',(6.37371962278214,4.94797317468673,-3.56304559720421));
#94514=CARTESIAN_POINT('',(6.34213406430118,4.9552300003035,-3.6043036579765));
#94515=CARTESIAN_POINT('Ctrl Pts',(6.34213406430117,4.95523000030349,-3.60430365797649));
#94516=CARTESIAN_POINT('Ctrl Pts',(6.36192865855916,4.96260329977038,-3.55455022116892));
#94517=CARTESIAN_POINT('Ctrl Pts',(6.38143263973457,4.97005789381842,-3.50396563895263));
#94518=CARTESIAN_POINT('Ctrl Pts',(6.41924800147741,4.98502388909895,-3.4023518433995));
#94519=CARTESIAN_POINT('Ctrl Pts',(6.4375181459293,4.99250278459722,-3.35149070138016));
#94520=CARTESIAN_POINT('Ctrl Pts',(6.45520502526095,5.000000000166,-3.30042846906862));
#94521=CARTESIAN_POINT('',(6.14157095691406,5.00000000128657,-3.85274008640452));
#94522=CARTESIAN_POINT('Origin',(0.550561349058368,5.12365835348864,0.892384193535622));
#94523=CARTESIAN_POINT('',(6.32248465610192,4.94797317381261,-3.65318813480831));
#94524=CARTESIAN_POINT('Origin',(1.07893432263829,5.49705219109465,1.05520055428565));
#94525=CARTESIAN_POINT('',(6.00499129873184,4.84409946432866,-4.33444832088375));
#94526=CARTESIAN_POINT('Ctrl Pts',(6.00499129873183,4.84409946432866,-4.33444832088374));
#94527=CARTESIAN_POINT('Ctrl Pts',(6.0635767440552,4.86143878570101,-4.22365720208668));
#94528=CARTESIAN_POINT('Ctrl Pts',(6.11936695459161,4.87877094698558,-4.11141989129545));
#94529=CARTESIAN_POINT('Ctrl Pts',(6.19883030728706,4.90476414606178,-3.94092099420311));
#94530=CARTESIAN_POINT('Ctrl Pts',(6.22463142636344,4.91343410632696,-3.88368752607863));
#94531=CARTESIAN_POINT('Ctrl Pts',(6.26221083893537,4.92641824545147,-3.79743681421562));
#94532=CARTESIAN_POINT('Ctrl Pts',(6.27453373416553,4.93073677839264,-3.76866048055067));
#94533=CARTESIAN_POINT('Ctrl Pts',(6.29868669384673,4.93932419701259,-3.71126224911645));
#94534=CARTESIAN_POINT('Ctrl Pts',(6.31017758861645,4.94346636791043,-3.68349592530596));
#94535=CARTESIAN_POINT('Ctrl Pts',(6.32248465533595,4.94797317428232,-3.65318813456712));
#94536=CARTESIAN_POINT('',(5.45875612031797,4.94797317386576,-4.84990488434038));
#94537=CARTESIAN_POINT('Ctrl Pts',(5.45875612062196,4.94797317342923,-4.84990488479222));
#94538=CARTESIAN_POINT('Ctrl Pts',(5.55417313422535,4.93049584997211,-4.76882322821963));
#94539=CARTESIAN_POINT('Ctrl Pts',(5.64746911273217,4.91309421478837,-4.68526023150146));
#94540=CARTESIAN_POINT('Ctrl Pts',(5.82963795448276,4.87845834287648,-4.51335050771509));
#94541=CARTESIAN_POINT('Ctrl Pts',(5.91847521456085,4.86123089199598,-4.42503763104279));
#94542=CARTESIAN_POINT('Ctrl Pts',(6.00499129873183,4.84409946432866,-4.33444832088374));
#94543=CARTESIAN_POINT('',(5.59479135903471,5.00000000038232,-4.61094455025847));
#94544=CARTESIAN_POINT('Ctrl Pts',(5.59479135887404,5.00000000040474,-4.61094455017618));
#94545=CARTESIAN_POINT('Ctrl Pts',(5.57294351023375,4.99124725213808,-4.65121646793442));
#94546=CARTESIAN_POINT('Ctrl Pts',(5.55067623930233,4.9825393709129,-4.69126880256542));
#94547=CARTESIAN_POINT('Ctrl Pts',(5.50515102629905,4.96515484986163,-4.77119847942965));
#94548=CARTESIAN_POINT('Ctrl Pts',(5.48156535851485,4.95636631335134,-4.81159547373595));
#94549=CARTESIAN_POINT('Ctrl Pts',(5.45875611941956,4.9479731748415,-4.84990488401924));
#94550=CARTESIAN_POINT('',(5.4190397503672,4.95523000038511,-4.88340839283606));
#94551=CARTESIAN_POINT('Ctrl Pts',(5.41903975036719,4.95523000038511,-4.88340839283605));
#94552=CARTESIAN_POINT('Ctrl Pts',(5.44906526742851,4.96260285565642,-4.83907608709589));
#94553=CARTESIAN_POINT('Ctrl Pts',(5.47899107385436,4.97005835699077,-4.79386143369335));
#94554=CARTESIAN_POINT('Ctrl Pts',(5.53776448660362,4.98502389150453,-4.70275530179052));
#94555=CARTESIAN_POINT('Ctrl Pts',(5.56654112273603,4.99250278589832,-4.65701081271476));
#94556=CARTESIAN_POINT('Ctrl Pts',(5.59479135889404,5.00000000037313,-4.61094455020163));
#94557=CARTESIAN_POINT('',(5.16975920861961,5.00000000120979,-5.08292137649758));
#94558=CARTESIAN_POINT('Origin',(0.729525520746253,5.12365827876601,0.753166594087148));
#94559=CARTESIAN_POINT('',(5.38934101651039,4.94797317378957,-4.92692593619431));
#94560=CARTESIAN_POINT('Origin',(1.28054633176727,5.49705206174571,0.798591557250787));
#94561=CARTESIAN_POINT('',(4.93281967559905,4.84409946430769,-5.52400695080939));
#94562=CARTESIAN_POINT('Ctrl Pts',(4.93281967559905,4.84409946430769,-5.52400695080939));
#94563=CARTESIAN_POINT('Ctrl Pts',(5.01385224130635,4.86143878567624,-5.42840020581429));
#94564=CARTESIAN_POINT('Ctrl Pts',(5.0924658118048,4.87877094694699,-5.33078018714352));
#94565=CARTESIAN_POINT('Ctrl Pts',(5.20672357837545,4.90476414600742,-5.18134973151522));
#94566=CARTESIAN_POINT('Ctrl Pts',(5.24422498543453,4.91343410626691,-5.13100082803629));
#94567=CARTESIAN_POINT('Ctrl Pts',(5.2994671656839,4.9264182453903,-5.05484507279633));
#94568=CARTESIAN_POINT('Ctrl Pts',(5.31768801958001,4.93073677833341,-5.02939057204024));
#94569=CARTESIAN_POINT('Ctrl Pts',(5.3536152195635,4.93932419696309,-4.97852645172661));
#94570=CARTESIAN_POINT('Ctrl Pts',(5.37080640243511,4.94346636786295,-4.95387949186148));
#94571=CARTESIAN_POINT('Ctrl Pts',(5.38934101594713,4.94797317425716,-4.92692593588516));
#94572=CARTESIAN_POINT('',(4.28854724725375,4.94797317383398,-5.90998800973694));
#94573=CARTESIAN_POINT('Ctrl Pts',(4.28854724746879,4.94797317349561,-5.90998801024313));
#94574=CARTESIAN_POINT('Ctrl Pts',(4.39916362364428,4.93049585005688,-5.85131383520822));
#94575=CARTESIAN_POINT('Ctrl Pts',(4.50824196854606,4.91309421481951,-5.78976037230495));
#94576=CARTESIAN_POINT('Ctrl Pts',(4.72310731303538,4.87845834289832,-5.66103071843775));
#94577=CARTESIAN_POINT('Ctrl Pts',(4.82885226541687,4.86123089199607,-5.59387993259784));
#94578=CARTESIAN_POINT('Ctrl Pts',(4.93281967559905,4.84409946430769,-5.52400695080939));
#94579=CARTESIAN_POINT('',(4.47277146646462,5.00000000040085,-5.70585799033773));
#94580=CARTESIAN_POINT('Ctrl Pts',(4.47277146628161,5.00000000043033,-5.70585799018668));
#94581=CARTESIAN_POINT('Ctrl Pts',(4.4427771279562,4.99124724963524,-5.74049174101125));
#94582=CARTESIAN_POINT('Ctrl Pts',(4.41242038951624,4.9825393696399,-5.77482086437295));
#94583=CARTESIAN_POINT('Ctrl Pts',(4.35077702246364,4.96515485137633,-5.84309524400365));
#94584=CARTESIAN_POINT('Ctrl Pts',(4.31905861476746,4.95636631464917,-5.87747755814629));
#94585=CARTESIAN_POINT('Ctrl Pts',(4.28854724663545,4.94797317468629,-5.9099880093767));
#94586=CARTESIAN_POINT('',(4.24255716059391,4.95523000035748,-5.9341703789812));
#94587=CARTESIAN_POINT('Ctrl Pts',(4.24255716059391,4.95523000035748,-5.93417037898119));
#94588=CARTESIAN_POINT('Ctrl Pts',(4.28141083181686,4.9626028554184,-5.89732913766012));
#94589=CARTESIAN_POINT('Ctrl Pts',(4.32035680406356,4.97005835687664,-5.85960474094954));
#94590=CARTESIAN_POINT('Ctrl Pts',(4.39734124811627,4.9850238906012,-5.78326317035894));
#94591=CARTESIAN_POINT('Ctrl Pts',(4.43527881784727,4.99250278545199,-5.7447742858742));
#94592=CARTESIAN_POINT('Ctrl Pts',(4.47277146625573,5.0000000003522,-5.70585799030624));
#94593=CARTESIAN_POINT('',(3.9562152655006,5.00000000119967,-6.07543091178372));
#94594=CARTESIAN_POINT('Origin',(0.874379005841,5.12365747043237,0.578729661810663));
#94595=CARTESIAN_POINT('',(4.20419778110858,4.94797317373202,-5.97028615646991));
#94596=CARTESIAN_POINT('Origin',(1.42228181186611,5.49705160338535,0.504640299297654));
#94597=CARTESIAN_POINT('',(3.62999488635505,4.84409946430512,-6.45526915547616));
#94598=CARTESIAN_POINT('Ctrl Pts',(3.62999488635505,4.84409946430512,-6.45526915547615));
#94599=CARTESIAN_POINT('Ctrl Pts',(3.7296855797877,4.86143878566297,-6.37931724938182));
#94600=CARTESIAN_POINT('Ctrl Pts',(3.82744662710813,4.87877094691801,-6.30087912636897));
#94601=CARTESIAN_POINT('Ctrl Pts',(3.97115624145015,4.90476414595063,-6.17950431415894));
#94602=CARTESIAN_POINT('Ctrl Pts',(4.01860441240173,4.91343410619924,-6.13839423406338));
#94603=CARTESIAN_POINT('Ctrl Pts',(4.08892629741799,4.92641824530769,-6.07589439388384));
#94604=CARTESIAN_POINT('Ctrl Pts',(4.11219312311801,4.93073677824677,-6.0549519501943));
#94605=CARTESIAN_POINT('Ctrl Pts',(4.15821695793549,4.93932462798877,-6.01299818461731));
#94606=CARTESIAN_POINT('Ctrl Pts',(4.18029947338156,4.94346583882346,-5.99262778107491));
#94607=CARTESIAN_POINT('Ctrl Pts',(4.20419778064507,4.94797317423399,-5.97028615607538));
#94608=CARTESIAN_POINT('',(2.91781067191024,4.94797317384864,-6.69372666398598));
#94609=CARTESIAN_POINT('Ctrl Pts',(2.91781067198254,4.94797317341034,-6.69372666447471));
#94610=CARTESIAN_POINT('Ctrl Pts',(3.03845411208919,4.93049584998617,-6.6602035100653));
#94611=CARTESIAN_POINT('Ctrl Pts',(3.15821444043594,4.9130942148187,-6.62353775288799));
#94612=CARTESIAN_POINT('Ctrl Pts',(3.39572942290471,4.87845834288346,-6.54400742451796));
#94613=CARTESIAN_POINT('Ctrl Pts',(3.51343755092169,4.86123089198299,-6.5011586257738));
#94614=CARTESIAN_POINT('Ctrl Pts',(3.62999488635505,4.84409946430512,-6.45526915547615));
#94615=CARTESIAN_POINT('',(3.14160975151107,5.00000000050473,-6.53397185204522));
#94616=CARTESIAN_POINT('Ctrl Pts',(3.1416097514399,5.00000000051907,-6.5339718519543));
#94617=CARTESIAN_POINT('Ctrl Pts',(3.10487144135448,4.99124725210346,-6.56134798140165));
#94618=CARTESIAN_POINT('Ctrl Pts',(3.06784467500926,4.98253937089912,-6.58834871129871));
#94619=CARTESIAN_POINT('Ctrl Pts',(2.99296550810226,4.96515484931178,-6.6417753822365));
#94620=CARTESIAN_POINT('Ctrl Pts',(2.95459747928808,4.9563663132354,-6.66853533540674));
#94621=CARTESIAN_POINT('Ctrl Pts',(2.9178106712046,4.9479731748178,-6.69372666327845));
#94622=CARTESIAN_POINT('',(2.86769731302197,4.9552300003156,-6.70745715373435));
#94623=CARTESIAN_POINT('Ctrl Pts',(2.86769731302196,4.9552300003156,-6.70745715373435));
#94624=CARTESIAN_POINT('Ctrl Pts',(2.91356514802405,4.96260329944764,-6.67982796665955));
#94625=CARTESIAN_POINT('Ctrl Pts',(2.95970462086193,4.97005789421878,-6.65136123553827));
#94626=CARTESIAN_POINT('Ctrl Pts',(3.05130322991824,4.98502389160803,-6.5933520712326));
#94627=CARTESIAN_POINT('Ctrl Pts',(3.0966278099219,4.99250278600782,-6.56391849325386));
#94628=CARTESIAN_POINT('Ctrl Pts',(3.1416097514151,5.00000000048106,-6.53397185200841));
#94629=CARTESIAN_POINT('',(2.55768309275547,5.00000000129321,-6.78386005075774));
#94630=CARTESIAN_POINT('Origin',(0.978345977284807,5.12365820924026,0.377235247498451));
#94631=CARTESIAN_POINT('',(2.82247093033594,4.94797317374067,-6.73448243143106));
#94632=CARTESIAN_POINT('Origin',(1.49751226228398,5.49705172217515,0.187094326967195));
#94633=CARTESIAN_POINT('',(2.15743557083302,4.84409946430342,-7.08469014864696));
#94634=CARTESIAN_POINT('Ctrl Pts',(2.15743557083301,4.84409946430342,-7.08469014864696));
#94635=CARTESIAN_POINT('Ctrl Pts',(2.27112296602449,4.86143878568678,-7.03194450811468));
#94636=CARTESIAN_POINT('Ctrl Pts',(2.3834602923105,4.87877094695926,-6.97635596016067));
#94637=CARTESIAN_POINT('Ctrl Pts',(2.54990205272904,4.90476414600642,-6.88871214258509));
#94638=CARTESIAN_POINT('Ctrl Pts',(2.60507836392412,4.91343410626223,-6.85876314746769));
#94639=CARTESIAN_POINT('Ctrl Pts',(2.68719178061627,4.92641824537106,-6.81284164534936));
#94640=CARTESIAN_POINT('Ctrl Pts',(2.71441664721448,4.93073677830577,-6.79739050411575));
#94641=CARTESIAN_POINT('Ctrl Pts',(2.76838328981831,4.93932462803495,-6.7663113582995));
#94642=CARTESIAN_POINT('Ctrl Pts',(2.79432856296978,4.94346583886611,-6.75116429152838));
#94643=CARTESIAN_POINT('Ctrl Pts',(2.82247092998867,4.94797317425684,-6.73448243098469));
#94644=CARTESIAN_POINT('',(1.4106405125511,4.94797317381983,-7.1644740989605));
#94645=CARTESIAN_POINT('Ctrl Pts',(1.41064051251384,4.94797317337648,-7.16447409941471));
#94646=CARTESIAN_POINT('Ctrl Pts',(1.53566986328428,4.9304958499545,-7.15766947114909));
#94647=CARTESIAN_POINT('Ctrl Pts',(1.6605123154199,4.91309421482194,-7.14760586952016));
#94648=CARTESIAN_POINT('Ctrl Pts',(1.90957099917454,4.87845834289018,-7.12099361639327));
#94649=CARTESIAN_POINT('Ctrl Pts',(2.03373840160017,4.86123089199066,-7.1044503668768));
#94650=CARTESIAN_POINT('Ctrl Pts',(2.15743557083302,4.84409946430342,-7.08469014864696));
#94651=CARTESIAN_POINT('',(1.66354985423409,5.0000000002771,-7.05656445327241));
#94652=CARTESIAN_POINT('Ctrl Pts',(1.66354985406861,5.0000000003246,-7.05656445292761));
#94653=CARTESIAN_POINT('Ctrl Pts',(1.62178538240259,4.99124724672022,-7.07540290402672));
#94654=CARTESIAN_POINT('Ctrl Pts',(1.57981993525488,4.98253936818981,-7.09381270558874));
#94655=CARTESIAN_POINT('Ctrl Pts',(1.49520626317404,4.96515484998644,-7.12989347614351));
#94656=CARTESIAN_POINT('Ctrl Pts',(1.45198265424955,4.95636631292779,-7.14777980636546));
#94657=CARTESIAN_POINT('Ctrl Pts',(1.41064051201504,4.94797317475814,-7.16447409810473));
#94658=CARTESIAN_POINT('',(1.35874712633804,4.95523000034704,-7.16711068663691));
#94659=CARTESIAN_POINT('Ctrl Pts',(1.35874712633804,4.95523000034704,-7.16711068663691));
#94660=CARTESIAN_POINT('Ctrl Pts',(1.40947914477903,4.96260287653345,-7.14998866555321));
#94661=CARTESIAN_POINT('Ctrl Pts',(1.46066553790084,4.97005836668923,-7.13210394217435));
#94662=CARTESIAN_POINT('Ctrl Pts',(1.5625895074464,4.98502386911349,-7.09514321554628));
#94663=CARTESIAN_POINT('Ctrl Pts',(1.61318184884325,4.99250277469276,-7.07614119944428));
#94664=CARTESIAN_POINT('Ctrl Pts',(1.66354985413998,5.00000000022698,-7.05656445301108));
#94665=CARTESIAN_POINT('',(1.03955650211012,5.00000000120338,-7.17508343327527));
#94666=CARTESIAN_POINT('Origin',(1.036567218847,5.12365836611404,0.158100762754939));
#94667=CARTESIAN_POINT('',(1.30876847510296,4.94797317377319,-7.18378179327604));
#94668=CARTESIAN_POINT('Origin',(1.50272107965398,5.49705188654033,-0.139199236961874));
#94669=CARTESIAN_POINT('',(0.583996966610964,4.84409946429569,-7.38283890436021));
#94670=CARTESIAN_POINT('Ctrl Pts',(0.583996966610964,4.84409946429569,-7.38283890436021));
#94671=CARTESIAN_POINT('Ctrl Pts',(0.706365167153948,4.86143878568503,-7.35576585697531));
#94672=CARTESIAN_POINT('Ctrl Pts',(0.828026003708649,4.87877094696627,-7.32562614285952));
#94673=CARTESIAN_POINT('Ctrl Pts',(1.00941727820285,4.9047641460309,-7.27581144753047));
#94674=CARTESIAN_POINT('Ctrl Pts',(1.06974174655383,4.91343410629532,-7.25842391917415));
#94675=CARTESIAN_POINT('Ctrl Pts',(1.15980716267515,4.92641824541257,-7.23122799358558));
#94676=CARTESIAN_POINT('Ctrl Pts',(1.18971706562288,4.93073677834755,-7.22199063300904));
#94677=CARTESIAN_POINT('Ctrl Pts',(1.24910011444237,4.93932419695411,-7.20324027462032));
#94678=CARTESIAN_POINT('Ctrl Pts',(1.27770160048699,4.94346636784186,-7.19402266140034));
#94679=CARTESIAN_POINT('Ctrl Pts',(1.30876847481697,4.94797317421864,-7.1837817926045));
#94680=CARTESIAN_POINT('',(-0.162489631407365,4.94797317382355,-7.30021868713222));
#94681=CARTESIAN_POINT('Ctrl Pts',(0.583996966611005,4.84409946429568,-7.38283890436021));
#94682=CARTESIAN_POINT('Ctrl Pts',(0.458124049300158,4.8613432067681,-7.37549809137105));
#94683=CARTESIAN_POINT('Ctrl Pts',(0.332486921697074,4.87868417663361,-7.36487179654896));
#94684=CARTESIAN_POINT('Ctrl Pts',(0.0835403843745239,4.91332225950562,
-7.33723683118231));
#94685=CARTESIAN_POINT('Ctrl Pts',(-0.039730334296242,4.93061037670979,
-7.32031818479942));
#94686=CARTESIAN_POINT('Ctrl Pts',(-0.162489633664296,4.947973174,-7.30021868758569));
#94687=CARTESIAN_POINT('Ctrl Pts',(-0.16248963429871,4.947973174,-7.30021868757157));
#94688=CARTESIAN_POINT('Ctrl Pts',(-0.108561113272334,4.95826854665991,
-7.29112111604271));
#94689=CARTESIAN_POINT('Ctrl Pts',(-0.0521079532441121,4.96904363931287,
-7.280985998079));
#94690=CARTESIAN_POINT('Ctrl Pts',(0.0386164317799012,4.98655204091907,
-7.26342789469982));
#94691=CARTESIAN_POINT('Ctrl Pts',(0.0731912356494929,4.99326273977431,
-7.25645071890302));
#94692=CARTESIAN_POINT('Ctrl Pts',(0.107704215939166,5.00000000018496,-7.2491999420065));
#94693=CARTESIAN_POINT('Origin',(1.80433264358217E-13,0.560925700000069,
-1.78199469069718E-12));
#94694=CARTESIAN_POINT('',(0.0337098038873345,0.680081834075993,7.43224893803594));
#94695=CARTESIAN_POINT('',(-0.576449088722096,0.562053379604022,7.28929565008102));
#94696=CARTESIAN_POINT('Origin',(1.46195216787403,0.516179043705186,-0.0906469046179226));
#94697=CARTESIAN_POINT('',(-0.598338399571803,0.767975418683164,7.49397642673713));
#94698=CARTESIAN_POINT('Origin',(-1.04077295590179,0.781987935583024,-0.237140562616648));
#94699=CARTESIAN_POINT('',(-1.20895591280749,0.680609080401461,7.33160125317681));
#94700=CARTESIAN_POINT('Ctrl Pts',(-1.20895590604886,0.680609079137261,
7.33160125103559));
#94701=CARTESIAN_POINT('Ctrl Pts',(-1.10870785777768,0.695136945009207,
7.36285586434991));
#94702=CARTESIAN_POINT('Ctrl Pts',(-1.00781302078567,0.709660812774055,
7.39200030989459));
#94703=CARTESIAN_POINT('Ctrl Pts',(-0.804232337447924,0.738780776769552,
7.44620706154414));
#94704=CARTESIAN_POINT('Ctrl Pts',(-0.701560825553855,0.753373671689897,
7.47123699479757));
#94705=CARTESIAN_POINT('Ctrl Pts',(-0.598394674877222,0.76794900780124,
7.49409641631185));
#94706=CARTESIAN_POINT('Ctrl Pts',(-0.576449088806045,0.562053379332408,
7.28929564980192));
#94707=CARTESIAN_POINT('Ctrl Pts',(-0.681392523124575,0.582224590096564,
7.30123074297468));
#94708=CARTESIAN_POINT('Ctrl Pts',(-0.786632152876032,0.602198953290415,
7.31073322818269));
#94709=CARTESIAN_POINT('Ctrl Pts',(-0.944626918335057,0.63181112165897,
7.32130389112597));
#94710=CARTESIAN_POINT('Ctrl Pts',(-0.997209431170085,0.64160443307101,
7.32421114415442));
#94711=CARTESIAN_POINT('Ctrl Pts',(-1.10694538657959,0.661914308861971,
7.3290041747411));
#94712=CARTESIAN_POINT('Ctrl Pts',(-1.1598156619626,0.671620855129919,7.33059470553222));
#94713=CARTESIAN_POINT('Ctrl Pts',(-1.20895591292573,0.680609080021414,
7.33160125079771));
#94714=CARTESIAN_POINT('Origin',(-1.91686944095437E-13,0.560925699999978,
-1.84856470408779E-14));
#94715=CARTESIAN_POINT('',(-7.41752113576009,0.680609079284826,0.440830472641154));
#94716=CARTESIAN_POINT('',(-7.30981359453413,0.562053379737014,-0.180969162848937));
#94717=CARTESIAN_POINT('Ctrl Pts',(-7.30981359577408,0.562053380753659,
-0.180969163194634));
#94718=CARTESIAN_POINT('Ctrl Pts',(-7.33220244279024,0.581887251281355,
-0.0780125161171526));
#94719=CARTESIAN_POINT('Ctrl Pts',(-7.35239722361586,0.601712674307791,
0.0253974978158168));
#94720=CARTESIAN_POINT('Ctrl Pts',(-7.37931284034215,0.631348476780122,
0.180808155407383));
#94721=CARTESIAN_POINT('Ctrl Pts',(-7.38769933974359,0.641177712391296,
0.232489641937349));
#94722=CARTESIAN_POINT('Ctrl Pts',(-7.40413083467024,0.661766419240893,
0.341043172649691));
#94723=CARTESIAN_POINT('Ctrl Pts',(-7.411386466036,0.67167472079557,0.393456954212761));
#94724=CARTESIAN_POINT('Ctrl Pts',(-7.41752113534007,0.680609080456112,
0.440830481409885));
#94725=CARTESIAN_POINT('',(-7.51537925264731,0.767975418698991,-0.191745179874597));
#94726=CARTESIAN_POINT('Origin',(0.180300736303671,0.781863706247153,-1.05208177488254));
#94727=CARTESIAN_POINT('',(-7.38630038189549,0.680609080418115,-0.810257984958939));
#94728=CARTESIAN_POINT('Ctrl Pts',(-7.38630037943127,0.680609079122411,
-0.810257978393205));
#94729=CARTESIAN_POINT('Ctrl Pts',(-7.41208183476458,0.695136944724126,
-0.708464863768294));
#94730=CARTESIAN_POINT('Ctrl Pts',(-7.43572120077453,0.70966081220104,-0.606140151255856));
#94731=CARTESIAN_POINT('Ctrl Pts',(-7.47882681837764,0.738780776746267,
-0.399923338135681));
#94732=CARTESIAN_POINT('Ctrl Pts',(-7.49826151950297,0.753373671681126,
-0.29604730943592));
#94733=CARTESIAN_POINT('Ctrl Pts',(-7.51550211293464,0.767949007820357,
-0.19179487652695));
#94734=CARTESIAN_POINT('Ctrl Pts',(-7.3098135938762,0.562053378853381,-0.180969163074211));
#94735=CARTESIAN_POINT('Ctrl Pts',(-7.32741270633406,0.582224589722421,
-0.285112536374756));
#94736=CARTESIAN_POINT('Ctrl Pts',(-7.34259881413271,0.602198953022129,
-0.38968336948138));
#94737=CARTESIAN_POINT('Ctrl Pts',(-7.36170779620114,0.631811365835249,
-0.546875435673787));
#94738=CARTESIAN_POINT('Ctrl Pts',(-7.36745767304757,0.641604918980557,
-0.599224737511866));
#94739=CARTESIAN_POINT('Ctrl Pts',(-7.37818459623173,0.661914788918559,
-0.708540272763156));
#94740=CARTESIAN_POINT('Ctrl Pts',(-7.38263500616264,0.671621089600935,
-0.761245578256281));
#94741=CARTESIAN_POINT('Ctrl Pts',(-7.38630037964414,0.680609080075174,
-0.810257985190196));
#94742=CARTESIAN_POINT('Origin',(-1.90342533401555E-12,0.901573518000139,
8.56519716263549E-14));
#94743=CARTESIAN_POINT('',(7.4975175754087,0.900669500589968,0.19295130544917));
#94744=CARTESIAN_POINT('',(7.49067431208828,0.809946052894305,-0.373896494420664));
#94745=CARTESIAN_POINT('Ctrl Pts',(7.49067429618873,0.809946054097563,-0.373896494256488));
#94746=CARTESIAN_POINT('Ctrl Pts',(7.49125842929932,0.811814511300298,-0.362193921634754));
#94747=CARTESIAN_POINT('Ctrl Pts',(7.49181928421141,0.813696729840433,-0.350406919339319));
#94748=CARTESIAN_POINT('Ctrl Pts',(7.49288856452571,0.817476260956881,-0.326742025674024));
#94749=CARTESIAN_POINT('Ctrl Pts',(7.49339363131842,0.819360421133853,-0.31494646269074));
#94750=CARTESIAN_POINT('Ctrl Pts',(7.49482562592852,0.825015714746983,-0.279547522709436));
#94751=CARTESIAN_POINT('Ctrl Pts',(7.49566888951138,0.828788189479575,-0.255941112703458));
#94752=CARTESIAN_POINT('Ctrl Pts',(7.49786506079125,0.840115815423992,-0.185079488469201));
#94753=CARTESIAN_POINT('Ctrl Pts',(7.49888268519632,0.847675760663585,-0.137815748088289));
#94754=CARTESIAN_POINT('Ctrl Pts',(7.50059447826849,0.870367208581086,0.00396235750429899));
#94755=CARTESIAN_POINT('Ctrl Pts',(7.49994903612033,0.885511641104869,0.0984719273944452));
#94756=CARTESIAN_POINT('Ctrl Pts',(7.49751757541842,0.900669500313366,0.192951305493795));
#94757=CARTESIAN_POINT('',(7.46163841178383,0.80994605200789,0.757596327810578));
#94758=CARTESIAN_POINT('Origin',(-0.191501740625454,0.803573279257418,-0.0204809236956735));
#94759=CARTESIAN_POINT('',(7.49028775646232,0.750000000660804,0.381561705761236));
#94760=CARTESIAN_POINT('Origin',(-0.18323094549859,0.946349170784347,-0.0404830745463346));
#94761=CARTESIAN_POINT('',(7.49999996733933,0.750000000076743,-0.000442032240240194));
#94762=CARTESIAN_POINT('Origin',(0.,0.750000001098927,0.));
#94763=CARTESIAN_POINT('Origin',(-0.192837956609714,0.803569462561183,0.00860069228931772));
#94764=CARTESIAN_POINT('Origin',(-1.8385328792773E-14,1.03148891300036,
2.49279763497867E-12));
#94765=CARTESIAN_POINT('',(0.352520299374595,0.940053947031003,-7.49171071504816));
#94766=CARTESIAN_POINT('',(-0.21691191335407,1.03040248142683,-7.49686262514646));
#94767=CARTESIAN_POINT('Ctrl Pts',(-0.216911913327511,1.03040248160653,
-7.49686262520794));
#94768=CARTESIAN_POINT('Ctrl Pts',(-0.122018200336322,1.01543877096837,
-7.49960825066177));
#94769=CARTESIAN_POINT('Ctrl Pts',(-0.0270884842090412,1.00042308922614,
-7.50055169267878));
#94770=CARTESIAN_POINT('Ctrl Pts',(0.162771944844896,0.970299044466182,
-7.49883462807081));
#94771=CARTESIAN_POINT('Ctrl Pts',(0.257687167935843,0.955193108293956,
-7.49617306068821));
#94772=CARTESIAN_POINT('Ctrl Pts',(0.352520283380967,0.940053949645103,
-7.4917107158382));
#94773=CARTESIAN_POINT('',(-0.21323909129465,0.849330497163622,-7.49696798168821));
#94774=CARTESIAN_POINT('Ctrl Pts',(0.352520299950128,0.940053947,-7.49171071505854));
#94775=CARTESIAN_POINT('Ctrl Pts',(0.258300413424799,0.924915272696728,
-7.49614420480774));
#94776=CARTESIAN_POINT('Ctrl Pts',(0.164004206490097,0.909779286371552,
-7.49879990837626));
#94777=CARTESIAN_POINT('Ctrl Pts',(-0.0246342017421915,0.8795298092342,
-7.50055261076486));
#94778=CARTESIAN_POINT('Ctrl Pts',(-0.118951432514705,0.864420318633172,
-7.49964985260826));
#94779=CARTESIAN_POINT('Ctrl Pts',(-0.213239091592113,0.849330499322643,
-7.49696799311674));
#94780=CARTESIAN_POINT('',(-0.778885090560337,0.940053948012018,-7.45944622867757));
#94781=CARTESIAN_POINT('Origin',(-0.0019124445238064,0.80358396694885,0.191459074564228));
#94782=CARTESIAN_POINT('Origin',(0.0190137625473567,0.946429295162185,0.191888929096342));
#94783=CARTESIAN_POINT('Origin',(5.63351448823468E-13,4.93907429999929,
-1.01706634108613E-13));
#94784=CARTESIAN_POINT('',(7.43060586817456,4.81939092007921,0.00690867062542753));
#94785=CARTESIAN_POINT('',(7.28652936255512,4.93794662021698,-0.61042155713763));
#94786=CARTESIAN_POINT('Ctrl Pts',(7.28652936159588,4.93794662121202,-0.610421556668722));
#94787=CARTESIAN_POINT('Ctrl Pts',(7.31511188023545,4.91789697871817,-0.509403982041436));
#94788=CARTESIAN_POINT('Ctrl Pts',(7.34136770815382,4.89804362330483,-0.407718113515646));
#94789=CARTESIAN_POINT('Ctrl Pts',(7.37733075383442,4.86848704273741,-0.253835059088018));
#94790=CARTESIAN_POINT('Ctrl Pts',(7.38878640668564,4.85863343285326,-0.202106738273538));
#94791=CARTESIAN_POINT('Ctrl Pts',(7.4114199687586,4.83820008061128,-0.0939490028819038));
#94792=CARTESIAN_POINT('Ctrl Pts',(7.42160776861126,4.82843422647897,-0.0417175607597513));
#94793=CARTESIAN_POINT('Ctrl Pts',(7.43060586925475,4.81939091904273,0.00690867580317548));
#94794=CARTESIAN_POINT('',(7.49205823556675,4.73201982385041,-0.621930980993225));
#94795=CARTESIAN_POINT('Origin',(-0.147247077923713,4.81289609762555,-1.05774438459138));
#94796=CARTESIAN_POINT('',(7.3263771516294,4.8193909197014,-1.2402214161419));
#94797=CARTESIAN_POINT('Ctrl Pts',(7.32637714974651,4.81939092084888,-1.24022141040838));
#94798=CARTESIAN_POINT('Ctrl Pts',(7.35824914062546,4.80491309543195,-1.13868537527286));
#94799=CARTESIAN_POINT('Ctrl Pts',(7.3879807452778,4.79041128730459,-1.03649293430841));
#94800=CARTESIAN_POINT('Ctrl Pts',(7.44329381503338,4.76128647694134,-0.830331917669992));
#94801=CARTESIAN_POINT('Ctrl Pts',(7.46884404609903,4.74666639456629,-0.72637863675835));
#94802=CARTESIAN_POINT('Ctrl Pts',(7.49219469844694,4.73203683302836,-0.621923452288041));
#94803=CARTESIAN_POINT('Ctrl Pts',(7.28652936366133,4.93794661914144,-0.61042155681656));
#94804=CARTESIAN_POINT('Ctrl Pts',(7.29763906183347,4.91814186442495,-0.715041521521126));
#94805=CARTESIAN_POINT('Ctrl Pts',(7.30652508358286,4.89834552791114,-0.819874369499637));
#94806=CARTESIAN_POINT('Ctrl Pts',(7.31648502147922,4.86872423031979,-0.977205672761118));
#94807=CARTESIAN_POINT('Ctrl Pts',(7.31924110656159,4.85888055797719,-1.02956737186234));
#94808=CARTESIAN_POINT('Ctrl Pts',(7.32384982960819,4.83826147069255,-1.13942245512654));
#94809=CARTESIAN_POINT('Ctrl Pts',(7.32539897638504,4.82833849612749,-1.1923916710017));
#94810=CARTESIAN_POINT('Ctrl Pts',(7.32637714961331,4.81939092000682,-1.24022141624027));
#94811=CARTESIAN_POINT('Origin',(-5.17787725715513E-14,4.89709473199831,
9.39656338849737E-12));
#94812=CARTESIAN_POINT('',(0.40918343007075,4.81939092003514,-7.41933421681296));
#94813=CARTESIAN_POINT('',(-0.215041573947508,4.93794662006386,-7.30889059675964));
#94814=CARTESIAN_POINT('Ctrl Pts',(-0.215041573499948,4.93794662117583,
-7.30889059546253));
#94815=CARTESIAN_POINT('Ctrl Pts',(-0.111912073431109,4.91775746672574,
-7.33212275399106));
#94816=CARTESIAN_POINT('Ctrl Pts',(-0.00823378782372437,4.89776736698642,
-7.35296247351665));
#94817=CARTESIAN_POINT('Ctrl Pts',(0.147742625517286,4.86814634061535,-7.38055596638373));
#94818=CARTESIAN_POINT('Ctrl Pts',(0.199659714009096,4.85836129974299,-7.38912265896429));
#94819=CARTESIAN_POINT('Ctrl Pts',(0.308142139983319,4.83806891418287,-7.40573574428087));
#94820=CARTESIAN_POINT('Ctrl Pts',(0.360483919976071,4.82837106019443,-7.41302625476642));
#94821=CARTESIAN_POINT('Ctrl Pts',(0.409183435372163,4.81939091904092,-7.41933421745164));
#94822=CARTESIAN_POINT('',(-0.215407009827946,4.73201982383798,-7.5147411512686));
#94823=CARTESIAN_POINT('Origin',(-1.06416490854892,4.8128960435549,0.0897660560821278));
#94824=CARTESIAN_POINT('',(-0.841760461628196,4.81939091968843,-7.38277662222671));
#94825=CARTESIAN_POINT('Ctrl Pts',(-0.841760456065915,4.81939092085314,
-7.38277662005998));
#94826=CARTESIAN_POINT('Ctrl Pts',(-0.73864781800586,4.8049130955081,-7.40910481766066));
#94827=CARTESIAN_POINT('Ctrl Pts',(-0.634995615012,4.79041128745961,-7.43326023103532));
#94828=CARTESIAN_POINT('Ctrl Pts',(-0.42614236103085,4.76128647694644,-7.47733084719864));
#94829=CARTESIAN_POINT('Ctrl Pts',(-0.320958274967625,4.74666639456744,
-7.49721568948058));
#94830=CARTESIAN_POINT('Ctrl Pts',(-0.215392104223649,4.73203683301729,
-7.51487700641513));
#94831=CARTESIAN_POINT('Ctrl Pts',(-0.215041573798538,4.93794661921194,
-7.30889059741849));
#94832=CARTESIAN_POINT('Ctrl Pts',(-0.31890663738018,4.91814186444707,-7.32564801301616));
#94833=CARTESIAN_POINT('Ctrl Pts',(-0.423104659537805,4.89834552786635,
-7.34019653868519));
#94834=CARTESIAN_POINT('Ctrl Pts',(-0.5796660027,4.86872423024089,-7.35865961455493));
#94835=CARTESIAN_POINT('Ctrl Pts',(-0.631801697389271,4.85888055789695,
-7.36424646284628));
#94836=CARTESIAN_POINT('Ctrl Pts',(-0.741246156930806,4.83826147071718,
-7.37479586106029));
#94837=CARTESIAN_POINT('Ctrl Pts',(-0.794053819745922,4.82833849616759,
-7.37921043141456));
#94838=CARTESIAN_POINT('Ctrl Pts',(-0.841760461825666,4.81939091997017,
-7.38277662029196));
#94839=CARTESIAN_POINT('Origin',(1.04430353253804E-12,1.16011713400017,
4.97377746627725E-14));
#94840=CARTESIAN_POINT('',(7.49772190572655,1.15903910528887,0.184841071447948));
#94841=CARTESIAN_POINT('',(7.49040836445842,1.06939092095439,-0.379186648426675));
#94842=CARTESIAN_POINT('Ctrl Pts',(7.49040836574509,1.0693909221528,-0.379186648467453));
#94843=CARTESIAN_POINT('Ctrl Pts',(7.49516278556348,1.0844050142568,-0.285268399695008));
#94844=CARTESIAN_POINT('Ctrl Pts',(7.49815066787259,1.09938963374112,-0.191263707148619));
#94845=CARTESIAN_POINT('Ctrl Pts',(7.50058866531781,1.12928008044628,-0.00320582877183695));
#94846=CARTESIAN_POINT('Ctrl Pts',(7.5000395265062,1.14418337209935,0.0908312575294414));
#94847=CARTESIAN_POINT('Ctrl Pts',(7.49772190590341,1.15903910529533,0.184841071561819));
#94848=CARTESIAN_POINT('',(7.46217159729501,1.06939091911158,0.752326401888058));
#94849=CARTESIAN_POINT('Origin',(-0.181513436785086,1.33838400563824,0.0240420059235262));
#94850=CARTESIAN_POINT('',(7.49755829997,0.979367659104793,0.191362310599562));
#94851=CARTESIAN_POINT('Origin',(-0.19191440622657,0.946436322382179,0.000401916073186764));
#94852=CARTESIAN_POINT('Ctrl Pts',(7.4975583002797,0.979367658874596,0.191362310570904));
#94853=CARTESIAN_POINT('Ctrl Pts',(7.49998541853642,0.994471430918934,0.0962680332434526));
#94854=CARTESIAN_POINT('Ctrl Pts',(7.5006033321718,1.00953259012931,0.00112879444476032));
#94855=CARTESIAN_POINT('Ctrl Pts',(7.4982187960069,1.03954821707066,-0.189104195261569));
#94856=CARTESIAN_POINT('Ctrl Pts',(7.4952177633165,1.05450026189394,-0.284182377452428));
#94857=CARTESIAN_POINT('Ctrl Pts',(7.49040836538004,1.069390921,-0.379186655678594));
#94858=CARTESIAN_POINT('Origin',(-4.50160742015981E-13,4.74999999999911,
-7.45388993583784E-14));
#94859=CARTESIAN_POINT('',(7.49028775568068,4.75000000000442,0.381561704655806));
#94860=CARTESIAN_POINT('',(7.4999999819041,4.75000000415214,-0.00044203176353017));
#94861=CARTESIAN_POINT('Origin',(0.,4.75000000067138,0.));
#94862=CARTESIAN_POINT('',(7.46163840082974,4.69005394803158,0.757596337309733));
#94863=CARTESIAN_POINT('Origin',(-0.183233979794819,4.55370521392812,-0.0404746383756041));
#94864=CARTESIAN_POINT('',(7.4975175754792,4.5993304994336,0.192951308991991));
#94865=CARTESIAN_POINT('Origin',(-0.19149502490191,4.69642568282372,-0.0204805842445447));
#94866=CARTESIAN_POINT('',(7.49067431020226,4.69005394712068,-0.373896499429461));
#94867=CARTESIAN_POINT('Ctrl Pts',(7.49751757532976,4.59933049913374,0.192951308940038));
#94868=CARTESIAN_POINT('Ctrl Pts',(7.49994903597294,4.61448835770566,0.0984719348112532));
#94869=CARTESIAN_POINT('Ctrl Pts',(7.50059447821245,4.62963278959406,0.00396236889379918));
#94870=CARTESIAN_POINT('Ctrl Pts',(7.49888268543748,4.65232423742436,-0.137815736135372));
#94871=CARTESIAN_POINT('Ctrl Pts',(7.49786506102374,4.65988418320927,-0.185079479921373));
#94872=CARTESIAN_POINT('Ctrl Pts',(7.49566888963438,4.67121180996999,-0.255941109259036));
#94873=CARTESIAN_POINT('Ctrl Pts',(7.49482562599899,4.67498428497423,-0.279547520964337));
#94874=CARTESIAN_POINT('Ctrl Pts',(7.49339363128608,4.68063957899424,-0.314946463492495));
#94875=CARTESIAN_POINT('Ctrl Pts',(7.4928885644551,4.68252373930679,-0.326742027324636));
#94876=CARTESIAN_POINT('Ctrl Pts',(7.49181928405843,4.68630327068637,-0.350406922637988));
#94877=CARTESIAN_POINT('Ctrl Pts',(7.49125842910013,4.68818548936229,-0.36219392578413));
#94878=CARTESIAN_POINT('Ctrl Pts',(7.49067429593706,4.69005394670754,-0.373896499298968));
#94879=CARTESIAN_POINT('Origin',(-0.192835064026876,4.69643091592117,0.00860058943978748));
#94880=CARTESIAN_POINT('Origin',(4.05578348683377E-12,4.78597145200587,
3.00810833964919E-13));
#94881=CARTESIAN_POINT('',(7.46187241733356,4.78575691081507,0.188108803306894));
#94882=CARTESIAN_POINT('Ctrl Pts',(7.49999998560045,4.75000000137362,-0.000442028262827379));
#94883=CARTESIAN_POINT('Ctrl Pts',(7.49405312262923,4.75594872264478,0.0310883694741082));
#94884=CARTESIAN_POINT('Ctrl Pts',(7.48790160624312,4.76190334823606,0.0625682707651447));
#94885=CARTESIAN_POINT('Ctrl Pts',(7.47519008163412,4.77382403272204,0.125426831226749));
#94886=CARTESIAN_POINT('Ctrl Pts',(7.46863459627975,4.77978626801372,0.156785509594588));
#94887=CARTESIAN_POINT('Ctrl Pts',(7.46187241698066,4.78575691117149,0.188108803162771));
#94888=CARTESIAN_POINT('Origin',(-0.261599883382976,4.80792711944447,1.42878715025716));
#94889=CARTESIAN_POINT('Origin',(-9.65329266569198E-14,1.28891220999942,
-2.21003770839445E-12));
#94890=CARTESIAN_POINT('',(0.346190408762415,1.19797317426376,-7.49200588672075));
#94891=CARTESIAN_POINT('',(-0.215486077596536,1.28783500377754,-7.49690374767466));
#94892=CARTESIAN_POINT('Ctrl Pts',(-0.215486074181298,1.28783500620183,
-7.49690374433565));
#94893=CARTESIAN_POINT('Ctrl Pts',(-0.121879038955992,1.27281874405466,
-7.49959432343662));
#94894=CARTESIAN_POINT('Ctrl Pts',(-0.0282369965533449,1.25781697911053,
-7.50053152780386));
#94895=CARTESIAN_POINT('Ctrl Pts',(0.112248484511282,1.23534090680584,-7.49930625044361));
#94896=CARTESIAN_POINT('Ctrl Pts',(0.15908255975695,1.22785302041325,-7.49845896723859));
#94897=CARTESIAN_POINT('Ctrl Pts',(0.229301947591752,1.21663380888301,-7.4965304222764));
#94898=CARTESIAN_POINT('Ctrl Pts',(0.252694445968612,1.21289755923839,-7.49577836510434));
#94899=CARTESIAN_POINT('Ctrl Pts',(0.287773141688719,1.2072966749925,-7.49448620361555));
#94900=CARTESIAN_POINT('Ctrl Pts',(0.299462014246144,1.20543067036107,-7.49402824540192));
#94901=CARTESIAN_POINT('Ctrl Pts',(0.322912484277998,1.20168768135239,-7.49305452574449));
#94902=CARTESIAN_POINT('Ctrl Pts',(0.334592979913718,1.19982364587847,-7.49254178002325));
#94903=CARTESIAN_POINT('Ctrl Pts',(0.346190411497856,1.19797317338938,-7.49200588620877));
#94904=CARTESIAN_POINT('',(-0.220938354192998,1.1083007626432,-7.49674504312255));
#94905=CARTESIAN_POINT('Ctrl Pts',(0.346190409540422,1.19797317429373,-7.49200588629922));
#94906=CARTESIAN_POINT('Ctrl Pts',(0.334478336782823,1.19613294342686,-7.49254707744697));
#94907=CARTESIAN_POINT('Ctrl Pts',(0.322694364732621,1.19428069285451,-7.49306406841878));
#94908=CARTESIAN_POINT('Ctrl Pts',(0.299045101682687,1.19056192455289,-7.49404506041721));
#94909=CARTESIAN_POINT('Ctrl Pts',(0.28724999051619,1.18870644997233,-7.49450643984025));
#94910=CARTESIAN_POINT('Ctrl Pts',(0.251844369753666,1.18313463689047,-7.49580766695149));
#94911=CARTESIAN_POINT('Ctrl Pts',(0.228231329885431,1.17941569911441,-7.49656378454989));
#94912=CARTESIAN_POINT('Ctrl Pts',(0.157317570547834,1.16823832462178,-7.49849918027799));
#94913=CARTESIAN_POINT('Ctrl Pts',(0.11001033880432,1.16077003178017,-7.49934237919276));
#94914=CARTESIAN_POINT('Ctrl Pts',(-0.031866414243553,1.13833699173946,
-7.50052851618956));
#94915=CARTESIAN_POINT('Ctrl Pts',(-0.12642295644833,1.1233390886692,-7.49953052900198));
#94916=CARTESIAN_POINT('Ctrl Pts',(-0.220938354235387,1.10830076288434,
-7.49674504325897));
#94917=CARTESIAN_POINT('',(-0.785187302803007,1.19797317358555,-7.45878548488081));
#94918=CARTESIAN_POINT('Origin',(0.0417752178770776,1.33917527074983,0.181485827824975));
#94919=CARTESIAN_POINT('Ctrl Pts',(-0.215486081067869,1.28783500479116,
-7.49690374413771));
#94920=CARTESIAN_POINT('Ctrl Pts',(-0.371541670048592,1.26310656824362,
-7.492418184706));
#94921=CARTESIAN_POINT('Ctrl Pts',(-0.52705976664116,1.23856749893779,-7.4830668161156));
#94922=CARTESIAN_POINT('Ctrl Pts',(-0.68159806042696,1.21428571428671,-7.46896405695075));
#94923=CARTESIAN_POINT('Ctrl Pts',(-0.716124358854676,1.20886077964635,
-7.46581327755717));
#94924=CARTESIAN_POINT('Ctrl Pts',(-0.750655784688141,1.20342302038954,
-7.46242062154302));
#94925=CARTESIAN_POINT('Ctrl Pts',(-0.785187302078986,1.1979731744789,-7.45878548428992));
#94926=CARTESIAN_POINT('Origin',(4.64569195380408E-14,4.651755933,1.34441069388203E-13));
#94927=CARTESIAN_POINT('',(0.352520299435009,4.55994605297308,-7.49171071504532));
#94928=CARTESIAN_POINT('',(-0.213239091294667,4.65066950283638,-7.49696798168821));
#94929=CARTESIAN_POINT('Ctrl Pts',(-0.21323909159213,4.65066950067736,-7.49696799311675));
#94930=CARTESIAN_POINT('Ctrl Pts',(-0.118951423809548,4.63557967997365,
-7.49964985285588));
#94931=CARTESIAN_POINT('Ctrl Pts',(-0.0246341842936763,4.62047018797078,
-7.50055261092768));
#94932=CARTESIAN_POINT('Ctrl Pts',(0.164004223867748,4.59022071083884,-7.49879990788983));
#94933=CARTESIAN_POINT('Ctrl Pts',(0.258300407446502,4.57508472826227,-7.49614420490339));
#94934=CARTESIAN_POINT('Ctrl Pts',(0.352520285220108,4.55994605536672,-7.49171071575167));
#94935=CARTESIAN_POINT('',(-0.216911910735758,4.46959751859283,-7.49686262533737));
#94936=CARTESIAN_POINT('Ctrl Pts',(0.352520299950129,4.559946053,-7.49171071505855));
#94937=CARTESIAN_POINT('Ctrl Pts',(0.257687188908902,4.54480689504879,-7.49617305991154));
#94938=CARTESIAN_POINT('Ctrl Pts',(0.162771970224917,4.5297009595704,-7.4988346274642));
#94939=CARTESIAN_POINT('Ctrl Pts',(-0.0270884634955866,4.49957691405067,
-7.50055169286844));
#94940=CARTESIAN_POINT('Ctrl Pts',(-0.122018188701805,4.48456123086711,
-7.49960825096596));
#94941=CARTESIAN_POINT('Ctrl Pts',(-0.216911910766392,4.46959751879733,
-7.49686262528204));
#94942=CARTESIAN_POINT('',(-0.778885090560973,4.55994605198798,-7.45944622867665));
#94943=CARTESIAN_POINT('Origin',(0.019013766933039,4.55357071037472,0.191888962985897));
#94944=CARTESIAN_POINT('Origin',(-0.00191244455506986,4.69641603310801,
0.191459074053018));
#94945=CARTESIAN_POINT('Origin',(-1.0698907038087E-12,1.41887506700011,
-6.74102700742862E-14));
#94946=CARTESIAN_POINT('',(7.4975151551836,1.41778968867681,0.193045310352991));
#94947=CARTESIAN_POINT('',(7.49065292194418,1.32710049349124,-0.374324466840203));
#94948=CARTESIAN_POINT('Ctrl Pts',(7.4906529218194,1.32710049291663,-0.374324464653929));
#94949=CARTESIAN_POINT('Ctrl Pts',(7.49537415365484,1.34215639817109,-0.279847313460021));
#94950=CARTESIAN_POINT('Ctrl Pts',(7.49830730405831,1.3572471693734,-0.185294207848121));
#94951=CARTESIAN_POINT('Ctrl Pts',(7.50059562915091,1.38748517979131,0.00388086647019446));
#94952=CARTESIAN_POINT('Ctrl Pts',(7.49995002764233,1.40262869206186,0.0984794794256389));
#94953=CARTESIAN_POINT('Ctrl Pts',(7.49751515557731,1.41778968810576,0.1930453104547));
#94954=CARTESIAN_POINT('',(7.46168168499786,1.32710049307755,0.757170029230453));
#94955=CARTESIAN_POINT('Origin',(-0.192110746278644,1.33928593621152,-0.0175336555807591));
#94956=CARTESIAN_POINT('',(7.49763545617134,1.23689319392375,0.188315065789256));
#94957=CARTESIAN_POINT('Origin',(-0.180076328767131,1.48200507450974,-0.0430982005950535));
#94958=CARTESIAN_POINT('Ctrl Pts',(7.49763520838133,1.23689161580505,0.188324937383956));
#94959=CARTESIAN_POINT('Ctrl Pts',(7.49999062502235,1.25189323496832,0.0945456360206955));
#94960=CARTESIAN_POINT('Ctrl Pts',(7.50058654174518,1.26691709131601,0.000733325220453728));
#94961=CARTESIAN_POINT('Ctrl Pts',(7.49884066957372,1.28947386856058,-0.139957457048645));
#94962=CARTESIAN_POINT('Ctrl Pts',(7.49781889281453,1.29699561098365,-0.186845521176366));
#94963=CARTESIAN_POINT('Ctrl Pts',(7.49562653093622,1.30828230113851,-0.257163397504894));
#94964=CARTESIAN_POINT('Ctrl Pts',(7.49478566948927,1.31204559065348,-0.280602684308469));
#94965=CARTESIAN_POINT('Ctrl Pts',(7.49335944336427,1.31769120063995,-0.315755915413143));
#94966=CARTESIAN_POINT('Ctrl Pts',(7.49285652500688,1.31957324836617,-0.327473114439529));
#94967=CARTESIAN_POINT('Ctrl Pts',(7.49179152371613,1.32335238839832,-0.350997861002957));
#94968=CARTESIAN_POINT('Ctrl Pts',(7.49123331922751,1.32523416776575,-0.362710060842525));
#94969=CARTESIAN_POINT('Ctrl Pts',(7.49065292159669,1.32710049380022,-0.374324469110649));
#94970=CARTESIAN_POINT('Origin',(2.16840434497101E-15,4.52171036999889,
-3.69170839731314E-14));
#94971=CARTESIAN_POINT('',(7.49755829997,4.52063234089521,0.191362310599587));
#94972=CARTESIAN_POINT('',(7.49040836444859,4.43060907904567,-0.379186648479543));
#94973=CARTESIAN_POINT('Ctrl Pts',(7.49040836538005,4.430609079,-0.379186655678578));
#94974=CARTESIAN_POINT('Ctrl Pts',(7.49521776331607,4.44549973810469,-0.28418237746117));
#94975=CARTESIAN_POINT('Ctrl Pts',(7.49821879600634,4.46045178292658,-0.189104195279084));
#94976=CARTESIAN_POINT('Ctrl Pts',(7.50060333217191,4.49046740986781,0.00112879442655575));
#94977=CARTESIAN_POINT('Ctrl Pts',(7.49998541853666,4.50552856907956,0.096268033234006));
#94978=CARTESIAN_POINT('Ctrl Pts',(7.49755830027969,4.52063234112541,0.191362310570927));
#94979=CARTESIAN_POINT('',(7.4621715972985,4.43060908088843,0.752326401885845));
#94980=CARTESIAN_POINT('Origin',(-0.191914406238891,4.55356367763345,0.000401916168807082));
#94981=CARTESIAN_POINT('',(7.49772190590322,4.34096089502546,0.184841070538928));
#94982=CARTESIAN_POINT('Origin',(-0.181513473722006,4.1616169543297,0.0240418511233536));
#94983=CARTESIAN_POINT('Ctrl Pts',(7.49772190592924,4.3409608948701,0.184841070515018));
#94984=CARTESIAN_POINT('Ctrl Pts',(7.50003951773272,4.35581657174786,0.0908316128767517));
#94985=CARTESIAN_POINT('Ctrl Pts',(7.50058866069735,4.37071997613226,-0.00320618473889875));
#94986=CARTESIAN_POINT('Ctrl Pts',(7.49815066788195,4.4006103662136,-0.191263706864571));
#94987=CARTESIAN_POINT('Ctrl Pts',(7.49516278557001,4.41559498572476,-0.285268399579692));
#94988=CARTESIAN_POINT('Ctrl Pts',(7.4904083657424,4.43060907785576,-0.379186648520938));
#94989=CARTESIAN_POINT('Origin',(1.95927331601629E-14,1.54874775200071,
4.17200995972422E-13));
#94990=CARTESIAN_POINT('',(0.352840825559124,1.45719264094421,-7.49169562594985));
#94991=CARTESIAN_POINT('',(-0.216060229695852,1.5476605353396,-7.49688720083611));
#94992=CARTESIAN_POINT('Ctrl Pts',(-0.21606023090219,1.54766053042136,-7.49688721914786));
#94993=CARTESIAN_POINT('Ctrl Pts',(-0.121254461794605,1.5326678365177,-7.49961952067055));
#94994=CARTESIAN_POINT('Ctrl Pts',(-0.0264122851482628,1.51762759595714,
-7.5005530047104));
#94995=CARTESIAN_POINT('Ctrl Pts',(0.163270940331239,1.48746377141007,-7.49882263926133));
#94996=CARTESIAN_POINT('Ctrl Pts',(0.258096561970816,1.47234261566213,-7.49615785262344));
#94997=CARTESIAN_POINT('Ctrl Pts',(0.352840824503127,1.45719264779623,-7.49169562599575));
#94998=CARTESIAN_POINT('',(-0.213439952126814,1.36645689698012,-7.49696226262636));
#94999=CARTESIAN_POINT('Ctrl Pts',(0.35284082530523,1.45719263430125,-7.49169562595797));
#95000=CARTESIAN_POINT('Ctrl Pts',(0.258534072859532,1.44204301532236,-7.49613724692419));
#95001=CARTESIAN_POINT('Ctrl Pts',(0.164150094801047,1.4269003938282,-7.49879783063957));
#95002=CARTESIAN_POINT('Ctrl Pts',(-0.0246589716878631,1.39664733164099,
-7.50055356277755));
#95003=CARTESIAN_POINT('Ctrl Pts',(-0.119068897208256,1.3815393153964,-7.49964903915524));
#95004=CARTESIAN_POINT('Ctrl Pts',(-0.213439952646206,1.36645690010564,
-7.49696227712133));
#95005=CARTESIAN_POINT('',(-0.778565868050108,1.45719264185526,-7.4594796221293));
#95006=CARTESIAN_POINT('Origin',(0.00109374381087227,1.33929191273629,0.192073141094562));
#95007=CARTESIAN_POINT('Origin',(0.0160466501341866,1.48214300449102,0.192311369972427));
#95008=CARTESIAN_POINT('Origin',(8.81553556769983E-15,4.39277644299907,
-3.33934269125535E-13));
#95009=CARTESIAN_POINT('',(0.346190408897311,4.30202682581797,-7.49200588608201));
#95010=CARTESIAN_POINT('',(-0.22093835419311,4.39169923735679,-7.49674504312255));
#95011=CARTESIAN_POINT('Ctrl Pts',(-0.220938354235514,4.39169923711568,
-7.49674504325896));
#95012=CARTESIAN_POINT('Ctrl Pts',(-0.126423456390729,4.37666099087654,
-7.49953051426805));
#95013=CARTESIAN_POINT('Ctrl Pts',(-0.0318659149821987,4.36166292932587,
-7.50052851196345));
#95014=CARTESIAN_POINT('Ctrl Pts',(0.157228920363726,4.33176393656074,-7.4989476160608));
#95015=CARTESIAN_POINT('Ctrl Pts',(0.251742511016298,4.31686672140778,-7.49637013230712));
#95016=CARTESIAN_POINT('Ctrl Pts',(0.346190410702883,4.30202682552361,-7.49200588624552));
#95017=CARTESIAN_POINT('',(-0.215486073506791,4.21216499623305,-7.49690374429604));
#95018=CARTESIAN_POINT('Ctrl Pts',(0.346190408849771,4.30202682618809,-7.49200588633115));
#95019=CARTESIAN_POINT('Ctrl Pts',(0.252649129683146,4.2871014901393,-7.49632823927246));
#95020=CARTESIAN_POINT('Ctrl Pts',(0.15903942881174,4.27214510978957,-7.49889815186353));
#95021=CARTESIAN_POINT('Ctrl Pts',(-0.0282336964774338,4.24218354883077,
-7.5005314988649));
#95022=CARTESIAN_POINT('Ctrl Pts',(-0.121882317798758,4.22718072995957,
-7.49959422918663));
#95023=CARTESIAN_POINT('Ctrl Pts',(-0.215486073772638,4.21216499386373,
-7.49690374434742));
#95024=CARTESIAN_POINT('',(-0.785187302803463,4.30202682641444,-7.45878548488046));
#95025=CARTESIAN_POINT('Ctrl Pts',(-0.785187302079502,4.30202682552109,
-7.45878548428987));
#95026=CARTESIAN_POINT('Ctrl Pts',(-0.750655784688943,4.29657697961046,
-7.46242062154294));
#95027=CARTESIAN_POINT('Ctrl Pts',(-0.716124358855617,4.29113922035365,
-7.46581327755709));
#95028=CARTESIAN_POINT('Ctrl Pts',(-0.681598060427919,4.28571428571329,
-7.46896405695068));
#95029=CARTESIAN_POINT('Ctrl Pts',(-0.527059766177999,4.26143250098929,
-7.4830668161579));
#95030=CARTESIAN_POINT('Ctrl Pts',(-0.37154166922301,4.23689343090281,-7.49241818475199));
#95031=CARTESIAN_POINT('Ctrl Pts',(-0.215486079999965,4.21216499285671,
-7.49690374416843));
#95032=CARTESIAN_POINT('Origin',(0.0417752178670641,4.16082472928313,0.181485827653811));
#95033=CARTESIAN_POINT('Origin',(-1.196959198424E-13,1.67745375799978,8.90672084696842E-14));
#95034=CARTESIAN_POINT('',(7.49772469075855,1.67637477915458,0.184728058371449));
#95035=CARTESIAN_POINT('',(7.49046336885653,1.58673401543383,-0.378098557106388));
#95036=CARTESIAN_POINT('Ctrl Pts',(7.49046336880353,1.58673401412648,-0.378098559389485));
#95037=CARTESIAN_POINT('Ctrl Pts',(7.49104984295418,1.58859408979895,-0.36647999318996));
#95038=CARTESIAN_POINT('Ctrl Pts',(7.49161452488343,1.59047040833691,-0.354756247142257));
#95039=CARTESIAN_POINT('Ctrl Pts',(7.49269257930982,1.59423866938533,-0.331203385564833));
#95040=CARTESIAN_POINT('Ctrl Pts',(7.49320174293478,1.59611422170125,-0.319476780521802));
#95041=CARTESIAN_POINT('Ctrl Pts',(7.49464630148781,1.60173828677872,-0.284301798040097));
#95042=CARTESIAN_POINT('Ctrl Pts',(7.49549918410855,1.60548553472768,-0.260849964297874));
#95043=CARTESIAN_POINT('Ctrl Pts',(7.49772641398529,1.61671588159084,-0.19052031221021));
#95044=CARTESIAN_POINT('Ctrl Pts',(7.49877119174833,1.6241933649187,-0.143632234283588));
#95045=CARTESIAN_POINT('Ctrl Pts',(7.50058632742757,1.64660512917628,-0.0029156602441874));
#95046=CARTESIAN_POINT('Ctrl Pts',(7.50003602916833,1.66151082526603,0.0909156932702936));
#95047=CARTESIAN_POINT('Ctrl Pts',(7.4977246911644,1.67637478000353,0.18472805824694));
#95048=CARTESIAN_POINT('',(7.46206223280785,1.5867340145509,0.753410392836019));
#95049=CARTESIAN_POINT('Ctrl Pts',(7.46206223337568,1.58673401558742,0.753410394279069));
#95050=CARTESIAN_POINT('Ctrl Pts',(7.46642527039844,1.59355605166272,0.710197223313913));
#95051=CARTESIAN_POINT('Ctrl Pts',(7.47040896742014,1.60035948085492,0.666985156712096));
#95052=CARTESIAN_POINT('Ctrl Pts',(7.47401454883397,1.60714285706879,0.62378403772218));
#95053=CARTESIAN_POINT('Ctrl Pts',(7.48616963301732,1.63001087959054,0.47814503827788));
#95054=CARTESIAN_POINT('Ctrl Pts',(7.494104357436,1.65310706300625,0.331669800426859));
#95055=CARTESIAN_POINT('Ctrl Pts',(7.49772469043156,1.67637477800781,0.18472806265998));
#95056=CARTESIAN_POINT('',(7.49754425839464,1.49654505839769,0.191911677629216));
#95057=CARTESIAN_POINT('Origin',(-0.192404287439453,1.48214578128891,-0.00260234602763698));
#95058=CARTESIAN_POINT('Ctrl Pts',(7.49754425848888,1.4965450582203,0.191911677603393));
#95059=CARTESIAN_POINT('Ctrl Pts',(7.49997612730393,1.51166788439511,0.0969042017717349));
#95060=CARTESIAN_POINT('Ctrl Pts',(7.50060207017734,1.52675096771425,0.00186225802549974));
#95061=CARTESIAN_POINT('Ctrl Pts',(7.49883027565662,1.54931297209943,-0.140733683683761));
#95062=CARTESIAN_POINT('Ctrl Pts',(7.49778716674769,1.55682462514503,-0.188280250890954));
#95063=CARTESIAN_POINT('Ctrl Pts',(7.49554517915627,1.5680672540857,-0.259550299424227));
#95064=CARTESIAN_POINT('Ctrl Pts',(7.49468580826546,1.57180799972993,-0.283281797632825));
#95065=CARTESIAN_POINT('Ctrl Pts',(7.49322802771744,1.57741257213675,-0.318864395530059));
#95066=CARTESIAN_POINT('Ctrl Pts',(7.49271420215881,1.57927897900857,-0.330718414082093));
#95067=CARTESIAN_POINT('Ctrl Pts',(7.4916274518607,1.58301976664233,-0.354486080543136));
#95068=CARTESIAN_POINT('Ctrl Pts',(7.49105747772631,1.58488296741043,-0.366328741600808));
#95069=CARTESIAN_POINT('Ctrl Pts',(7.49046336891913,1.58673401549796,-0.37809855709943));
#95070=CARTESIAN_POINT('Origin',(-1.32718118079324E-13,1.80614392399977,
-8.28330459778925E-13));
#95071=CARTESIAN_POINT('',(0.345447470364996,1.71532338704984,-7.49204017902143));
#95072=CARTESIAN_POINT('',(-0.216253748659272,1.80506741735209,-7.49688163939095));
#95073=CARTESIAN_POINT('Ctrl Pts',(-0.21625374864293,1.80506741777536,-7.49688163946837));
#95074=CARTESIAN_POINT('Ctrl Pts',(-0.122646000119446,1.79006264722948,
-7.49958183236105));
#95075=CARTESIAN_POINT('Ctrl Pts',(-0.0289925193184668,1.7750750069347,
-7.50052867438228));
#95076=CARTESIAN_POINT('Ctrl Pts',(0.15828886644386,1.7451527227798,-7.49891406340871));
#95077=CARTESIAN_POINT('Ctrl Pts',(0.251901963680161,1.73022043511571,-7.49635343127732));
#95078=CARTESIAN_POINT('Ctrl Pts',(0.345447470172254,1.71532338695633,-7.49204017910686));
#95079=CARTESIAN_POINT('',(-0.220230577166923,1.62564958718448,-7.49676586836886));
#95080=CARTESIAN_POINT('Ctrl Pts',(0.345447470364785,1.71532338707357,-7.49204017909798));
#95081=CARTESIAN_POINT('Ctrl Pts',(0.251240613271182,1.70047396625177,-7.49638392522001));
#95082=CARTESIAN_POINT('Ctrl Pts',(0.156967907525142,1.68557177708759,-7.49895005759635));
#95083=CARTESIAN_POINT('Ctrl Pts',(-0.0316419039501056,1.65567252678535,
-7.50052637935151));
#95084=CARTESIAN_POINT('Ctrl Pts',(-0.125958586906449,1.64067867637695,
-7.49953527307687));
#95085=CARTESIAN_POINT('Ctrl Pts',(-0.220230577126277,1.62564958683412,
-7.49676586888631));
#95086=CARTESIAN_POINT('',(-0.785926947266129,1.7153233873478,-7.45870758578964));
#95087=CARTESIAN_POINT('Origin',(0.0444645659943935,1.87485304789864,0.179386017271571));
#95088=CARTESIAN_POINT('Ctrl Pts',(-0.21625375099681,1.80506741660064,-7.49688163879576));
#95089=CARTESIAN_POINT('Ctrl Pts',(-0.333198817477333,1.78658581162692,
-7.4935082618823));
#95090=CARTESIAN_POINT('Ctrl Pts',(-0.44982066598863,1.76822051520783,-7.48740412737111));
#95091=CARTESIAN_POINT('Ctrl Pts',(-0.5659326671137,1.75000000002106,-7.47861753370175));
#95092=CARTESIAN_POINT('Ctrl Pts',(-0.639240188522535,1.73849644467944,
-7.47307010195039));
#95093=CARTESIAN_POINT('Ctrl Pts',(-0.712587645320282,1.72693520694186,
-7.46643537569407));
#95094=CARTESIAN_POINT('Ctrl Pts',(-0.785926945488551,1.71532338729505,
-7.45870758473092));
#95095=CARTESIAN_POINT('Origin',(7.4013735416371E-14,4.134630322,-2.08166817117217E-14));
#95096=CARTESIAN_POINT('',(0.352840846703245,4.04280735915174,-7.49169562495402));
#95097=CARTESIAN_POINT('',(-0.213439952122633,4.13354310263043,-7.49696226262648));
#95098=CARTESIAN_POINT('Ctrl Pts',(-0.213439952646204,4.13354309989436,
-7.49696227712133));
#95099=CARTESIAN_POINT('Ctrl Pts',(-0.119068801382565,4.11846066928871,
-7.49964904188342));
#95100=CARTESIAN_POINT('Ctrl Pts',(-0.0246587799652441,4.10335263767846,
-7.50055356461426));
#95101=CARTESIAN_POINT('Ctrl Pts',(0.164150289677141,4.07309957490726,-7.49879782520741));
#95102=CARTESIAN_POINT('Ctrl Pts',(0.258534175068266,4.05795696825996,-7.4961372422326));
#95103=CARTESIAN_POINT('Ctrl Pts',(0.352840834990003,4.04280736414296,-7.49169562550186));
#95104=CARTESIAN_POINT('',(-0.216060229702239,3.95233946533212,-7.4968872008231));
#95105=CARTESIAN_POINT('Ctrl Pts',(0.352840846647665,4.04280735574477,-7.49169562495281));
#95106=CARTESIAN_POINT('Ctrl Pts',(0.25809657502234,4.02765738641835,-7.49615785228942));
#95107=CARTESIAN_POINT('Ctrl Pts',(0.163270944270159,4.01253622921479,-7.49882263929091));
#95108=CARTESIAN_POINT('Ctrl Pts',(-0.0264122886211297,3.98237240349212,
-7.5005530046766));
#95109=CARTESIAN_POINT('Ctrl Pts',(-0.121254463560225,3.96733216320307,
-7.49961952062042));
#95110=CARTESIAN_POINT('Ctrl Pts',(-0.21606023096172,3.95233946956923,-7.49688721914614));
#95111=CARTESIAN_POINT('',(-0.778565868050654,4.04280735814475,-7.45947962212857));
#95112=CARTESIAN_POINT('Origin',(0.0160466022232138,4.01785667422611,0.192311407730464));
#95113=CARTESIAN_POINT('Origin',(0.00109374380103399,4.16070808729083,0.192073140869918));
#95114=CARTESIAN_POINT('Origin',(1.0321604682062E-12,1.93599222699994,7.12320827322976E-14));
#95115=CARTESIAN_POINT('',(7.49751546373246,1.93490816812523,0.193032549393738));
#95116=CARTESIAN_POINT('',(7.49062612097592,1.84427517280653,-0.374860382219912));
#95117=CARTESIAN_POINT('Ctrl Pts',(7.4906261216132,1.84427517300727,-0.374860382283726));
#95118=CARTESIAN_POINT('Ctrl Pts',(7.49121303530402,1.84614015233912,-0.363132413068011));
#95119=CARTESIAN_POINT('Ctrl Pts',(7.49177591444379,1.84801682086589,-0.351333568492057));
#95120=CARTESIAN_POINT('Ctrl Pts',(7.49284976660165,1.85178766568973,-0.327631235139327));
#95121=CARTESIAN_POINT('Ctrl Pts',(7.49335705074457,1.85366774354606,-0.315816333714424));
#95122=CARTESIAN_POINT('Ctrl Pts',(7.49479553393039,1.85931163604412,-0.280356648675277));
#95123=CARTESIAN_POINT('Ctrl Pts',(7.49564276527711,1.86307720271901,-0.256708875702626));
#95124=CARTESIAN_POINT('Ctrl Pts',(7.4978500074469,1.87438749651835,-0.185712247460573));
#95125=CARTESIAN_POINT('Ctrl Pts',(7.49887334226035,1.8819386651109,-0.138355057832773));
#95126=CARTESIAN_POINT('Ctrl Pts',(7.50059683829672,1.90460873985635,0.0036923073310301));
#95127=CARTESIAN_POINT('Ctrl Pts',(7.49995243135686,1.91974763415408,0.0983798626929981));
#95128=CARTESIAN_POINT('Ctrl Pts',(7.49751548411153,1.93490816308888,0.193032550384539));
#95129=CARTESIAN_POINT('',(7.4617358852843,1.8442751723037,0.75663616261998));
#95130=CARTESIAN_POINT('Origin',(-0.192468731460285,1.87499927803,-0.0145618870896762));
#95131=CARTESIAN_POINT('',(7.49766239512274,1.75423095970248,0.187239441586169));
#95132=CARTESIAN_POINT('Origin',(-0.177845399432686,2.01767772337631,-0.0457629068187224));
#95133=CARTESIAN_POINT('Ctrl Pts',(7.49766239501538,1.75423096138946,0.187239441623221));
#95134=CARTESIAN_POINT('Ctrl Pts',(7.50000203158565,1.76919630156981,0.0935529566687501));
#95135=CARTESIAN_POINT('Ctrl Pts',(7.50058539451906,1.78418803845602,-0.000165562178714458));
#95136=CARTESIAN_POINT('Ctrl Pts',(7.49823961397369,1.814210421049,-0.187579914718305));
#95137=CARTESIAN_POINT('Ctrl Pts',(7.49531020708347,1.82923869541257,-0.281260911311939));
#95138=CARTESIAN_POINT('Ctrl Pts',(7.49062612155154,1.84427517297352,-0.374860382221891));
#95139=CARTESIAN_POINT('Origin',(-2.35922392732846E-13,4.00453392000067,
-1.61275073157219E-14));
#95140=CARTESIAN_POINT('',(7.49754425839464,4.00345494160231,0.191911677629249));
#95141=CARTESIAN_POINT('',(7.49046336898085,3.91326598495459,-0.378098554637036));
#95142=CARTESIAN_POINT('Ctrl Pts',(7.49046336879689,3.91326598412122,-0.378098559520896));
#95143=CARTESIAN_POINT('Ctrl Pts',(7.49105747761129,3.91511703221824,-0.366328743954911));
#95144=CARTESIAN_POINT('Ctrl Pts',(7.49162745175183,3.91698023299548,-0.354486082844943));
#95145=CARTESIAN_POINT('Ctrl Pts',(7.49271420206082,3.92072102064167,-0.330718416303762));
#95146=CARTESIAN_POINT('Ctrl Pts',(7.49322802762509,3.92258742752121,-0.318864397702178));
#95147=CARTESIAN_POINT('Ctrl Pts',(7.49468580818944,3.92819199995176,-0.283281799652642));
#95148=CARTESIAN_POINT('Ctrl Pts',(7.49554517909013,3.93193274561174,-0.259550301343109));
#95149=CARTESIAN_POINT('Ctrl Pts',(7.49778716670837,3.94317537459964,-0.188280252507716));
#95150=CARTESIAN_POINT('Ctrl Pts',(7.49883027563135,3.95068702767696,-0.140733685098229));
#95151=CARTESIAN_POINT('Ctrl Pts',(7.50060207018266,3.97324903215747,0.00186225721714485));
#95152=CARTESIAN_POINT('Ctrl Pts',(7.49997612731427,3.98833211554058,0.0969042013677435));
#95153=CARTESIAN_POINT('Ctrl Pts',(7.49754425848887,4.0034549417797,0.191911677603424));
#95154=CARTESIAN_POINT('',(7.46206223280808,3.91326598544903,0.753410392836296));
#95155=CARTESIAN_POINT('Origin',(-0.192404287971952,4.01785421864167,-0.0026023460724639));
#95156=CARTESIAN_POINT('',(7.49772469113674,3.82362522066483,0.18472805242102));
#95157=CARTESIAN_POINT('Ctrl Pts',(7.49772469126306,3.82362522012807,0.184728050404971));
#95158=CARTESIAN_POINT('Ctrl Pts',(7.49410435803577,3.84689293573233,0.331669792293636));
#95159=CARTESIAN_POINT('Ctrl Pts',(7.48616963408108,3.86998912007418,0.478145035441857));
#95160=CARTESIAN_POINT('Ctrl Pts',(7.47401454883743,3.89285714293126,0.623784037719768));
#95161=CARTESIAN_POINT('Ctrl Pts',(7.47040896720935,3.89964051905595,0.666985156348763));
#95162=CARTESIAN_POINT('Ctrl Pts',(7.46642527039842,3.90644394833732,0.710197223314147));
#95163=CARTESIAN_POINT('Ctrl Pts',(7.46206223337563,3.91326598441267,0.753410394279661));
#95164=CARTESIAN_POINT('Ctrl Pts',(7.49772469130685,3.82362522091266,0.184728052464479));
#95165=CARTESIAN_POINT('Ctrl Pts',(7.50003602919478,3.83848917537128,0.090915689258002));
#95166=CARTESIAN_POINT('Ctrl Pts',(7.50058632740452,3.85339487118032,-0.0029156624840335));
#95167=CARTESIAN_POINT('Ctrl Pts',(7.49877119175063,3.87580663501669,-0.143632233877501));
#95168=CARTESIAN_POINT('Ctrl Pts',(7.49772641401234,3.88328411820511,-0.190520310930482));
#95169=CARTESIAN_POINT('Ctrl Pts',(7.4954991841973,3.89451446485863,-0.260849961708079));
#95170=CARTESIAN_POINT('Ctrl Pts',(7.49464630160125,3.89826171273757,-0.284301795013283));
#95171=CARTESIAN_POINT('Ctrl Pts',(7.49320174309141,3.90388577770994,-0.319476776839918));
#95172=CARTESIAN_POINT('Ctrl Pts',(7.49269257948187,3.9057613299908,-0.331203381664559));
#95173=CARTESIAN_POINT('Ctrl Pts',(7.49161452508621,3.9095295909769,-0.354756242854235));
#95174=CARTESIAN_POINT('Ctrl Pts',(7.491049843174,3.9114059094791,-0.366479988688053));
#95175=CARTESIAN_POINT('Ctrl Pts',(7.49046336904451,3.91326598510923,-0.37809855461549));
#95176=CARTESIAN_POINT('Origin',(4.14511924508249E-14,2.06597317200048,
1.50400525367189E-12));
#95177=CARTESIAN_POINT('',(0.353054365832619,1.97432008473567,-7.49168556575891));
#95178=CARTESIAN_POINT('',(-0.215318823985962,2.06488542583352,-7.49690853987847));
#95179=CARTESIAN_POINT('Ctrl Pts',(-0.21531882455298,2.06488542424203,-7.49690854978191));
#95180=CARTESIAN_POINT('Ctrl Pts',(-0.120597229775604,2.04986689835188,
-7.49962905014707));
#95181=CARTESIAN_POINT('Ctrl Pts',(-0.0258486669508494,2.03480680756073,
-7.5005539179205));
#95182=CARTESIAN_POINT('Ctrl Pts',(0.116255388562765,2.01216376703626,-7.49924848405551));
#95183=CARTESIAN_POINT('Ctrl Pts',(0.163608775699612,2.00460910542996,-7.49836482670986));
#95184=CARTESIAN_POINT('Ctrl Pts',(0.234638059001823,1.9932632677006,-7.49636622501913));
#95185=CARTESIAN_POINT('Ctrl Pts',(0.258323187161593,1.9894775996329,-7.49558741551992));
#95186=CARTESIAN_POINT('Ctrl Pts',(0.29384846706808,1.9837959838051,-7.49425070100337));
#95187=CARTESIAN_POINT('Ctrl Pts',(0.305691842860589,1.98190126977851,-7.49377695059779));
#95188=CARTESIAN_POINT('Ctrl Pts',(0.329478959924526,1.9780946126958,-7.49276895103959));
#95189=CARTESIAN_POINT('Ctrl Pts',(0.341319546987744,1.97619916724463,-7.49223858260928));
#95190=CARTESIAN_POINT('Ctrl Pts',(0.353054369828204,1.97432008410232,-7.49168556547491));
#95191=CARTESIAN_POINT('',(-0.213747920400373,1.88359400911337,-7.49695348562358));
#95192=CARTESIAN_POINT('Ctrl Pts',(0.353054367065202,1.9743200854565,-7.49168556560512));
#95193=CARTESIAN_POINT('Ctrl Pts',(0.341349315939044,1.9724405873732,-7.4922371797086));
#95194=CARTESIAN_POINT('Ctrl Pts',(0.329552974666823,1.97054679727599,-7.49276563402704));
#95195=CARTESIAN_POINT('Ctrl Pts',(0.305841049153146,1.96674083570353,-7.49377080520936));
#95196=CARTESIAN_POINT('Ctrl Pts',(0.294034012727743,1.96484608111116,-7.49424336601566));
#95197=CARTESIAN_POINT('Ctrl Pts',(0.258613729773365,1.95916306904533,-7.49557718010503));
#95198=CARTESIAN_POINT('Ctrl Pts',(0.234997369840539,1.95537543065149,-7.49635475238689));
#95199=CARTESIAN_POINT('Ctrl Pts',(0.164158264868712,1.94401858829907,-7.49835205236256));
#95200=CARTESIAN_POINT('Ctrl Pts',(0.116926694462175,1.93645243803566,-7.49923727598405));
#95201=CARTESIAN_POINT('Ctrl Pts',(-0.0247977080462619,1.91376710880402,
-7.50055422089684));
#95202=CARTESIAN_POINT('Ctrl Pts',(-0.119287039118363,1.89866636706812,
-7.49964670593636));
#95203=CARTESIAN_POINT('Ctrl Pts',(-0.213747921084859,1.88359401243752,
-7.49695350300585));
#95204=CARTESIAN_POINT('',(-0.778353303331698,1.97432008362658,-7.45950173389065));
#95205=CARTESIAN_POINT('Origin',(0.00409925169774547,1.87500219272972,0.192502951085732));
#95206=CARTESIAN_POINT('Origin',(0.0130774175759701,2.01785756222504,0.192617386214208));
#95207=CARTESIAN_POINT('Origin',(-1.68728737038287E-13,3.87542691999814,
-2.61249355482107E-12));
#95208=CARTESIAN_POINT('',(0.345447470705384,3.78467661285328,-7.49204017900575));
#95209=CARTESIAN_POINT('',(-0.22023057716692,3.87435041281552,-7.49676586836886));
#95210=CARTESIAN_POINT('Ctrl Pts',(-0.220230577126272,3.87435041316588,
-7.49676586888631));
#95211=CARTESIAN_POINT('Ctrl Pts',(-0.125958586550348,3.85932132356628,
-7.49953527308733));
#95212=CARTESIAN_POINT('Ctrl Pts',(-0.0316419034223253,3.84432747313072,
-7.5005263793582));
#95213=CARTESIAN_POINT('Ctrl Pts',(0.156967908702848,3.81442822272598,-7.49895005757541));
#95214=CARTESIAN_POINT('Ctrl Pts',(0.251240614743078,3.79952603351569,-7.49638392517439));
#95215=CARTESIAN_POINT('Ctrl Pts',(0.345447472130071,3.78467661264817,-7.4920401790166));
#95216=CARTESIAN_POINT('',(-0.216253753419816,3.69493258269211,-7.49688163925365));
#95217=CARTESIAN_POINT('Ctrl Pts',(0.345447470002635,3.78467661301666,-7.49204017911469));
#95218=CARTESIAN_POINT('Ctrl Pts',(0.251901960340126,3.76977956435237,-7.49635343142922));
#95219=CARTESIAN_POINT('Ctrl Pts',(0.158288859355404,3.75484727608745,-7.49891406345454));
#95220=CARTESIAN_POINT('Ctrl Pts',(-0.0289925200732418,3.72492499294492,
-7.50052867440407));
#95221=CARTESIAN_POINT('Ctrl Pts',(-0.122646002852608,3.70993735233324,
-7.49958183234109));
#95222=CARTESIAN_POINT('Ctrl Pts',(-0.216253753350609,3.69493258147004,
-7.49688163933261));
#95223=CARTESIAN_POINT('',(-0.785926947266576,3.7846766126522,-7.45870758578904));
#95224=CARTESIAN_POINT('Ctrl Pts',(-0.785926945489019,3.78467661270495,
-7.4587075847303));
#95225=CARTESIAN_POINT('Ctrl Pts',(-0.712587645321075,3.77306479305815,
-7.46643537569305));
#95226=CARTESIAN_POINT('Ctrl Pts',(-0.639240188779733,3.76150355535492,
-7.4730701018862));
#95227=CARTESIAN_POINT('Ctrl Pts',(-0.565932667114682,3.74999999997894,
-7.47861753370054));
#95228=CARTESIAN_POINT('Ctrl Pts',(-0.449820668513435,3.73177948519748,
-7.48740412724795));
#95229=CARTESIAN_POINT('Ctrl Pts',(-0.333198823358805,3.71341418928976,
-7.49350826150332));
#95230=CARTESIAN_POINT('Ctrl Pts',(-0.216253759848471,3.69493258476514,
-7.49688163830947));
#95231=CARTESIAN_POINT('Origin',(0.0444645660021557,3.62514695210178,0.179386017273158));
#95232=CARTESIAN_POINT('Origin',(-6.24500451351651E-14,2.19479107900067,
9.90418684565508E-14));
#95233=CARTESIAN_POINT('',(7.4977201549805,2.19371102280125,0.184912079215527));
#95234=CARTESIAN_POINT('',(7.49051254924921,2.10403448601065,-0.37712299467934));
#95235=CARTESIAN_POINT('Ctrl Pts',(7.490512548626,2.104034486,-0.37712300231648));
#95236=CARTESIAN_POINT('Ctrl Pts',(7.49522437558569,2.11903557744126,-0.283535502345184));
#95237=CARTESIAN_POINT('Ctrl Pts',(7.49818204534608,2.13401580726065,-0.18986395636617));
#95238=CARTESIAN_POINT('Ctrl Pts',(7.50058481057828,2.16391559853964,-0.00247117275680855));
#95239=CARTESIAN_POINT('Ctrl Pts',(7.50003045536675,2.17883280263076,0.091235199694861));
#95240=CARTESIAN_POINT('Ctrl Pts',(7.49772015487359,2.19371102268306,0.184912079231655));
#95241=CARTESIAN_POINT('',(7.46196404695618,2.10403448645287,0.754382247112074));
#95242=CARTESIAN_POINT('Ctrl Pts',(7.46196404603328,2.10403448479514,0.7543822497587));
#95243=CARTESIAN_POINT('Ctrl Pts',(7.47026686575195,2.11704095516578,0.672254992309608));
#95244=CARTESIAN_POINT('Ctrl Pts',(7.47720030543364,2.12998516342589,0.590120924256145));
#95245=CARTESIAN_POINT('Ctrl Pts',(7.48277273680961,2.14285714326542,0.508047408556932));
#95246=CARTESIAN_POINT('Ctrl Pts',(7.49006088260498,2.15969232114795,0.400703994567648));
#95247=CARTESIAN_POINT('Ctrl Pts',(7.49505584610473,2.17665108712233,0.292943108994319));
#95248=CARTESIAN_POINT('Ctrl Pts',(7.49772015503783,2.19371102301421,0.184912078878391));
#95249=CARTESIAN_POINT('',(7.49753295098489,2.01370168038256,0.192352916919592));
#95250=CARTESIAN_POINT('Origin',(-0.192711908600478,2.01785800812459,-0.00560467461627225));
#95251=CARTESIAN_POINT('Ctrl Pts',(7.49753295126449,2.0137016812419,0.192352917063813));
#95252=CARTESIAN_POINT('Ctrl Pts',(7.49996803906273,2.02883889136636,0.0974380528380879));
#95253=CARTESIAN_POINT('Ctrl Pts',(7.50060070245807,2.04394235290159,0.00247949131625866));
#95254=CARTESIAN_POINT('Ctrl Pts',(7.49825945640149,2.07406116001761,-0.187395514074732));
#95255=CARTESIAN_POINT('Ctrl Pts',(7.49528675591947,2.08907407473323,-0.282296488362628));
#95256=CARTESIAN_POINT('Ctrl Pts',(7.490512548626,2.104034486,-0.377123002316484));
#95257=CARTESIAN_POINT('Origin',(5.81566045321225E-13,3.74685310400011,
6.96328845278815E-14));
#95258=CARTESIAN_POINT('',(7.49766239511298,3.74576903988833,0.18723944161622));
#95259=CARTESIAN_POINT('',(7.49062612097616,3.65572482719341,-0.374860382220325));
#95260=CARTESIAN_POINT('Ctrl Pts',(7.49062612155167,3.65572482702639,-0.374860382222295));
#95261=CARTESIAN_POINT('Ctrl Pts',(7.49531020708282,3.67076130458482,-0.281260911328065));
#95262=CARTESIAN_POINT('Ctrl Pts',(7.49823961397226,3.68578957894398,-0.187579914762058));
#95263=CARTESIAN_POINT('Ctrl Pts',(7.50058539451876,3.71581196152875,-0.000165562273871897));
#95264=CARTESIAN_POINT('Ctrl Pts',(7.50000203158683,3.73080369841115,0.0935529565497265));
#95265=CARTESIAN_POINT('Ctrl Pts',(7.49766239501894,3.74576903858778,0.187239441480738));
#95266=CARTESIAN_POINT('',(7.4617358794251,3.65572482796968,0.756636166346095));
#95267=CARTESIAN_POINT('Origin',(-0.177843206429112,3.48232181763573,-0.0457629117666998));
#95268=CARTESIAN_POINT('',(7.49751546373715,3.56509183186907,0.19303254812848));
#95269=CARTESIAN_POINT('Origin',(-0.192466710504741,3.62500080527713,-0.0145618519171436));
#95270=CARTESIAN_POINT('Ctrl Pts',(7.49751548414534,3.56509183712149,0.193032549071094));
#95271=CARTESIAN_POINT('Ctrl Pts',(7.49995243849788,3.58025241037405,0.0983795846860867));
#95272=CARTESIAN_POINT('Ctrl Pts',(7.50059684165538,3.59539121607547,0.00369258345655861));
#95273=CARTESIAN_POINT('Ctrl Pts',(7.49887334224948,3.61806133497713,-0.138355058384732));
#95274=CARTESIAN_POINT('Ctrl Pts',(7.49785000743527,3.62561250355198,-0.185712247901861));
#95275=CARTESIAN_POINT('Ctrl Pts',(7.49564276526749,3.63692279732492,-0.25670887597848));
#95276=CARTESIAN_POINT('Ctrl Pts',(7.49479553392196,3.640688363991,-0.280356648895874));
#95277=CARTESIAN_POINT('Ctrl Pts',(7.49335705073873,3.64633225647582,-0.315816333851884));
#95278=CARTESIAN_POINT('Ctrl Pts',(7.49284976659679,3.64821233432779,-0.327631235249468));
#95279=CARTESIAN_POINT('Ctrl Pts',(7.49177591444114,3.65198317914295,-0.351333568547655));
#95280=CARTESIAN_POINT('Ctrl Pts',(7.49121303530262,3.65385984766531,-0.36313241309592));
#95281=CARTESIAN_POINT('Ctrl Pts',(7.49062612161318,3.65572482699279,-0.374860382284109));
#95282=CARTESIAN_POINT('Origin',(7.01313526684356E-14,2.32340998499977,
1.50834206236183E-12));
#95283=CARTESIAN_POINT('',(0.345002061015038,2.23266407489608,-7.49206070239071));
#95284=CARTESIAN_POINT('',(-0.217131941212996,2.32233405333693,-7.4968562557694));
#95285=CARTESIAN_POINT('Ctrl Pts',(-0.217131941025569,2.32233405396696,
-7.49685625580393));
#95286=CARTESIAN_POINT('Ctrl Pts',(-0.123452179549237,2.30733288148859,
-7.49956950889964));
#95287=CARTESIAN_POINT('Ctrl Pts',(-0.0297257413240806,2.29235307873659,
-7.50052672529768));
#95288=CARTESIAN_POINT('Ctrl Pts',(0.110879654202442,2.2699241212905,-7.49932688666955));
#95289=CARTESIAN_POINT('Ctrl Pts',(0.157757857214269,2.26245346441813,-7.4984872311799));
#95290=CARTESIAN_POINT('Ctrl Pts',(0.228038659103193,2.25126411895454,-7.49656900932632));
#95291=CARTESIAN_POINT('Ctrl Pts',(0.251448152483116,2.24753891515717,-7.49582032886621));
#95292=CARTESIAN_POINT('Ctrl Pts',(0.286551146394412,2.24195560118718,-7.49453303715063));
#95293=CARTESIAN_POINT('Ctrl Pts',(0.298247249301271,2.24009572515162,-7.49407670011623));
#95294=CARTESIAN_POINT('Ctrl Pts',(0.321707635570041,2.23636603413695,-7.49310635560389));
#95295=CARTESIAN_POINT('Ctrl Pts',(0.333394495071327,2.23450853328971,-7.49259522007918));
#95296=CARTESIAN_POINT('Ctrl Pts',(0.345002061078998,2.23266407597544,-7.49206070302766));
#95297=CARTESIAN_POINT('',(-0.219224277906958,2.14301213152219,-7.49679536286557));
#95298=CARTESIAN_POINT('Ctrl Pts',(0.345002067217683,2.232664075,-7.49206070274498));
#95299=CARTESIAN_POINT('Ctrl Pts',(0.251036504641597,2.2178090840518,-7.4963877249919));
#95300=CARTESIAN_POINT('Ctrl Pts',(0.15700486422329,2.20290583169153,-7.49894626488442));
#95301=CARTESIAN_POINT('Ctrl Pts',(-0.0311189115788482,2.17301418427561,
-7.50052548339322));
#95302=CARTESIAN_POINT('Ctrl Pts',(-0.125196010903262,2.15802815571166,
-7.49954497514307));
#95303=CARTESIAN_POINT('Ctrl Pts',(-0.219224277787359,2.14301213155917,
-7.49679536308873));
#95304=CARTESIAN_POINT('',(-0.786370364711829,2.23266407449122,-7.45866084596208));
#95305=CARTESIAN_POINT('Origin',(0.0471099633924378,2.41052394526463,0.177110167734925));
#95306=CARTESIAN_POINT('Ctrl Pts',(-0.217131942481557,2.32233405325538,
-7.49685625574591));
#95307=CARTESIAN_POINT('Ctrl Pts',(-0.29496967936998,2.31006874163771,-7.49460183611176));
#95308=CARTESIAN_POINT('Ctrl Pts',(-0.372654673125393,2.2978593648052,-7.49113829054721));
#95309=CARTESIAN_POINT('Ctrl Pts',(-0.450131733931299,2.28571428607735,
-7.4864799085177));
#95310=CARTESIAN_POINT('Ctrl Pts',(-0.562135980734646,2.26815682575238,
-7.47974554609165));
#95311=CARTESIAN_POINT('Ctrl Pts',(-0.674272603922395,2.25046493734972,
-7.47047937137698));
#95312=CARTESIAN_POINT('Ctrl Pts',(-0.786370369442445,2.23266407446841,
-7.45866084752161));
#95313=CARTESIAN_POINT('Origin',(-4.70537863882532E-15,3.61749373599881,
4.70110061989715E-13));
#95314=CARTESIAN_POINT('',(0.353054364847621,3.52567991485733,-7.49168556587659));
#95315=CARTESIAN_POINT('',(-0.213747920400581,3.61640599088661,-7.49695348562358));
#95316=CARTESIAN_POINT('Ctrl Pts',(-0.213747920849145,3.61640598752487,
-7.49695350301259));
#95317=CARTESIAN_POINT('Ctrl Pts',(-0.119290334839949,3.60133415880332,
-7.49964661196808));
#95318=CARTESIAN_POINT('Ctrl Pts',(-0.0247944268889988,3.58623236600729,
-7.50055419025866));
#95319=CARTESIAN_POINT('Ctrl Pts',(0.116926685865832,3.56354756335538,-7.49923727598735));
#95320=CARTESIAN_POINT('Ctrl Pts',(0.164158251379456,3.55598141386297,-7.49835205273171));
#95321=CARTESIAN_POINT('Ctrl Pts',(0.234997367947894,3.54462456965167,-7.49635475244958));
#95322=CARTESIAN_POINT('Ctrl Pts',(0.258613728155951,3.54083693121376,-7.49557718016419));
#95323=CARTESIAN_POINT('Ctrl Pts',(0.294034012069731,3.53515391899408,-7.49424336604505));
#95324=CARTESIAN_POINT('Ctrl Pts',(0.305841049178711,3.53325916429236,-7.49377080520672));
#95325=CARTESIAN_POINT('Ctrl Pts',(0.329549629766121,3.52945373960847,-7.49276577582196));
#95326=CARTESIAN_POINT('Ctrl Pts',(0.341352546817462,3.52755889383967,-7.49223702744892));
#95327=CARTESIAN_POINT('Ctrl Pts',(0.353054366551428,3.52567991462599,-7.49168556562935));
#95328=CARTESIAN_POINT('',(-0.215318825491527,3.43511457396892,-7.49690853966387));
#95329=CARTESIAN_POINT('Ctrl Pts',(0.353054364802041,3.52567991509285,-7.4916855657118));
#95330=CARTESIAN_POINT('Ctrl Pts',(0.341319541914271,3.52380083194171,-7.4922385828405));
#95331=CARTESIAN_POINT('Ctrl Pts',(0.329478954738908,3.52190538647417,-7.49276895126789));
#95332=CARTESIAN_POINT('Ctrl Pts',(0.305691837408766,3.51809872934921,-7.49377695082036));
#95333=CARTESIAN_POINT('Ctrl Pts',(0.293848461509,3.51620401530564,-7.49425070122153));
#95334=CARTESIAN_POINT('Ctrl Pts',(0.258323181276033,3.51052239942619,-7.49558741572346));
#95335=CARTESIAN_POINT('Ctrl Pts',(0.234638052906211,3.50673673132531,-7.49636622521058));
#95336=CARTESIAN_POINT('Ctrl Pts',(0.163608768968816,3.49539089349572,-7.49836482685939));
#95337=CARTESIAN_POINT('Ctrl Pts',(0.11625538140688,3.48783623182252,-7.49924848416912));
#95338=CARTESIAN_POINT('Ctrl Pts',(-0.0258453825439643,3.46519371578282,
-7.50055388765264));
#95339=CARTESIAN_POINT('Ctrl Pts',(-0.120600525541143,3.45013257908954,
-7.49962895551085));
#95340=CARTESIAN_POINT('Ctrl Pts',(-0.215318826251877,3.43511457548861,
-7.49690854973315));
#95341=CARTESIAN_POINT('',(-0.778353303338544,3.52567991637271,-7.45950173388933));
#95342=CARTESIAN_POINT('Origin',(0.0130772088859088,3.48214112196594,0.192617420003678));
#95343=CARTESIAN_POINT('Origin',(0.00409925167992709,3.6249978073121,0.192502950758071));
#95344=CARTESIAN_POINT('Origin',(-1.14925430283463E-13,2.45311202899922,
5.55653613398821E-14));
#95345=CARTESIAN_POINT('',(7.49751856063912,2.45202942596296,0.192913016089072));
#95346=CARTESIAN_POINT('',(7.49059383870815,2.36147458181351,-0.375504899176539));
#95347=CARTESIAN_POINT('Ctrl Pts',(7.49059383965004,2.36147458233101,-0.375504899298271));
#95348=CARTESIAN_POINT('Ctrl Pts',(7.4911823243483,2.36333688481693,-0.363765771889329));
#95349=CARTESIAN_POINT('Ctrl Pts',(7.49174663150587,2.36521061426394,-0.351957688190679));
#95350=CARTESIAN_POINT('Ctrl Pts',(7.49282321345917,2.36897545960216,-0.328238288443623));
#95351=CARTESIAN_POINT('Ctrl Pts',(7.49333186630279,2.37085280695196,-0.316413682529276));
#95352=CARTESIAN_POINT('Ctrl Pts',(7.49477437393667,2.37648893076456,-0.280923509903681));
#95353=CARTESIAN_POINT('Ctrl Pts',(7.49562410848287,2.38024966579896,-0.257254971800962));
#95354=CARTESIAN_POINT('Ctrl Pts',(7.49783844368032,2.39154716307407,-0.186190543045395));
#95355=CARTESIAN_POINT('Ctrl Pts',(7.49886566756327,2.39909119483712,-0.138786406196185));
#95356=CARTESIAN_POINT('Ctrl Pts',(7.50059811512875,2.42174259853615,0.00339777825096544));
#95357=CARTESIAN_POINT('Ctrl Pts',(7.49995628033341,2.43687275373891,0.0981716218080551));
#95358=CARTESIAN_POINT('Ctrl Pts',(7.49751856071574,2.45202942632333,0.192913015950082));
#95359=CARTESIAN_POINT('',(7.46180089043427,2.36147458096339,0.755994147437323));
#95360=CARTESIAN_POINT('Origin',(-0.192710522543249,2.41071411382912,-0.0115878204131166));
#95361=CARTESIAN_POINT('',(7.49768896324805,2.27159573047444,0.186172524012441));
#95362=CARTESIAN_POINT('Ctrl Pts',(7.49768896256665,2.27159573309532,0.186172532960065));
#95363=CARTESIAN_POINT('Ctrl Pts',(7.49694289493809,2.27631121117708,0.216218782605194));
#95364=CARTESIAN_POINT('Ctrl Pts',(7.49601668785442,2.28101755500063,0.246241293301155));
#95365=CARTESIAN_POINT('Ctrl Pts',(7.49491115290311,2.28571428596856,0.276236875889871));
#95366=CARTESIAN_POINT('Ctrl Pts',(7.48932977407838,2.30942609312731,0.42767188314124));
#95367=CARTESIAN_POINT('Ctrl Pts',(7.47913550857591,2.33338323202062,0.579455883520034));
#95368=CARTESIAN_POINT('Ctrl Pts',(7.46427457798021,2.3575225017414,0.731166892692783));
#95369=CARTESIAN_POINT('Ctrl Pts',(7.46346389862386,2.35883932423202,0.739442887421059));
#95370=CARTESIAN_POINT('Ctrl Pts',(7.46263934471632,2.36015668777524,0.747718662273833));
#95371=CARTESIAN_POINT('Ctrl Pts',(7.46180091190877,2.36147458179854,0.755994147902303));
#95372=CARTESIAN_POINT('Ctrl Pts',(7.4976889633641,2.27159572893773,0.186172523881806));
#95373=CARTESIAN_POINT('Ctrl Pts',(7.50001352343751,2.28652496523362,0.0925559791646668));
#95374=CARTESIAN_POINT('Ctrl Pts',(7.5005844224481,2.30148474771429,-0.00109164279741452));
#95375=CARTESIAN_POINT('Ctrl Pts',(7.49821906806474,2.33145198408239,-0.188365088745824));
#95376=CARTESIAN_POINT('Ctrl Pts',(7.49528245577757,2.34645707710048,-0.281976109257676));
#95377=CARTESIAN_POINT('Ctrl Pts',(7.49059383954544,2.361474582,-0.375504901384827));
#95378=CARTESIAN_POINT('Origin',(1.68431523742753E-13,2.58316965299976,
1.28022592527088E-12));
#95379=CARTESIAN_POINT('',(0.353161059393618,2.49144077909165,-7.49168053681783));
#95380=CARTESIAN_POINT('',(-0.214686790752558,2.58208164289175,-7.49692666440967));
#95381=CARTESIAN_POINT('Ctrl Pts',(-0.214686791009888,2.58208164104049,
-7.49692667576293));
#95382=CARTESIAN_POINT('Ctrl Pts',(-0.120052354351971,2.56704149196775,
-7.49963668806582));
#95383=CARTESIAN_POINT('Ctrl Pts',(-0.0253904843322359,2.55196418346729,
-7.50055439644757));
#95384=CARTESIAN_POINT('Ctrl Pts',(0.116586597891132,2.5293015607346,-7.4992430842681));
#95385=CARTESIAN_POINT('Ctrl Pts',(0.16389926048191,2.52174124069315,-7.49835822710871));
#95386=CARTESIAN_POINT('Ctrl Pts',(0.234864949024222,2.51038899728159,-7.4963590470893));
#95387=CARTESIAN_POINT('Ctrl Pts',(0.258527076426483,2.50660176131153,-7.49558031352006));
#95388=CARTESIAN_POINT('Ctrl Pts',(0.294017234894503,2.50091831508106,-7.49424406250517));
#95389=CARTESIAN_POINT('Ctrl Pts',(0.305848454025024,2.49902313294419,-7.49377054115703));
#95390=CARTESIAN_POINT('Ctrl Pts',(0.329609345416721,2.4952159669497,-7.49276319401097));
#95391=CARTESIAN_POINT('Ctrl Pts',(0.341437329052012,2.49332026768562,-7.49223319856089));
#95392=CARTESIAN_POINT('Ctrl Pts',(0.353161059381371,2.49144077728819,-7.49168053684465));
#95393=CARTESIAN_POINT('',(-0.214163364586765,2.40074633135423,-7.49694162681415));
#95394=CARTESIAN_POINT('Ctrl Pts',(0.353161059342393,2.49144078070713,-7.49168053684648));
#95395=CARTESIAN_POINT('Ctrl Pts',(0.341445095676823,2.48956080663179,-7.49223283243877));
#95396=CARTESIAN_POINT('Ctrl Pts',(0.329636241314836,2.4876663623943,-7.49276199369556));
#95397=CARTESIAN_POINT('Ctrl Pts',(0.305898177313054,2.48385907115041,-7.49376849248492));
#95398=CARTESIAN_POINT('Ctrl Pts',(0.294079068303966,2.4819638757106,-7.49424161722381));
#95399=CARTESIAN_POINT('Ctrl Pts',(0.258623899996873,2.47627996468824,-7.49557690117514));
#95400=CARTESIAN_POINT('Ctrl Pts',(0.23498468888381,2.47249207223284,-7.49635522214074));
#95401=CARTESIAN_POINT('Ctrl Pts',(0.164082374314062,2.46113616130948,-7.49835396752701));
#95402=CARTESIAN_POINT('Ctrl Pts',(0.1168103051957,2.45357201211615,-7.49923934606941));
#95403=CARTESIAN_POINT('Ctrl Pts',(-0.0250402834869289,2.43089529097404,
-7.50055449258178));
#95404=CARTESIAN_POINT('Ctrl Pts',(-0.119615788079795,2.41580442945549,
-7.49964256498655));
#95405=CARTESIAN_POINT('Ctrl Pts',(-0.214163365287468,2.40074633459546,
-7.49694164662957));
#95406=CARTESIAN_POINT('',(-0.77824708168631,2.49144077881243,-7.45951282263306));
#95407=CARTESIAN_POINT('Origin',(0.00710118688723879,2.41071461179977,0.192748080607653));
#95408=CARTESIAN_POINT('Origin',(0.0100862188857957,2.55357129378393,0.192647581726705));
#95409=CARTESIAN_POINT('Origin',(-5.2989451611378E-14,3.35806380000116,
-3.57353036051222E-13));
#95410=CARTESIAN_POINT('',(0.345002067680305,3.26733592524982,-7.49206070116328));
#95411=CARTESIAN_POINT('',(-0.219224277907411,3.3569878684778,-7.49679536286556));
#95412=CARTESIAN_POINT('Ctrl Pts',(-0.219224277787808,3.3569878684409,-7.49679536308871));
#95413=CARTESIAN_POINT('Ctrl Pts',(-0.125196017082453,3.34197184527514,
-7.49954497496237));
#95414=CARTESIAN_POINT('Ctrl Pts',(-0.0311189239394535,3.32698581769337,
-7.50052548326445));
#95415=CARTESIAN_POINT('Ctrl Pts',(0.157004851868707,3.29709417026657,-7.49894626522065));
#95416=CARTESIAN_POINT('Ctrl Pts',(0.251036498468413,3.28219091692411,-7.49638772527614));
#95417=CARTESIAN_POINT('Ctrl Pts',(0.345002067217704,3.267335925,-7.49206070274495));
#95418=CARTESIAN_POINT('',(-0.21713193487299,3.17766594634372,-7.49685625595301));
#95419=CARTESIAN_POINT('Ctrl Pts',(0.345002067007358,3.26733592496657,-7.49206070275464));
#95420=CARTESIAN_POINT('Ctrl Pts',(0.333394500515828,3.26549146757557,-7.49259521983764));
#95421=CARTESIAN_POINT('Ctrl Pts',(0.321707640575037,3.26363396665861,-7.49310635538957));
#95422=CARTESIAN_POINT('Ctrl Pts',(0.298247253481625,3.25990427551308,-7.49407669995052));
#95423=CARTESIAN_POINT('Ctrl Pts',(0.286551150129963,3.25804439940689,-7.49453303700846));
#95424=CARTESIAN_POINT('Ctrl Pts',(0.251448154881864,3.25246108522453,-7.4958203287885));
#95425=CARTESIAN_POINT('Ctrl Pts',(0.228038660609242,3.24873588128519,-7.49656900928323));
#95426=CARTESIAN_POINT('Ctrl Pts',(0.157757856048062,3.23754653539625,-7.49848723121556));
#95427=CARTESIAN_POINT('Ctrl Pts',(0.110879651250187,3.23007587823904,-7.49932688672432));
#95428=CARTESIAN_POINT('Ctrl Pts',(-0.0297257424336825,3.20764692108542,
-7.50052672524788));
#95429=CARTESIAN_POINT('Ctrl Pts',(-0.123452177029398,3.19266711891365,
-7.4995695088958));
#95430=CARTESIAN_POINT('Ctrl Pts',(-0.217131934884892,3.17766594701636,
-7.49685625598175));
#95431=CARTESIAN_POINT('',(-0.786370364711874,3.26733592550877,-7.45866084596202));
#95432=CARTESIAN_POINT('Ctrl Pts',(-0.786370365032877,3.26733592483135,
-7.45866084798646));
#95433=CARTESIAN_POINT('Ctrl Pts',(-0.674272603922472,3.24953506265028,
-7.47047937137689));
#95434=CARTESIAN_POINT('Ctrl Pts',(-0.562135980523448,3.23184317427154,
-7.47974554652098));
#95435=CARTESIAN_POINT('Ctrl Pts',(-0.4501317339314,3.21428571392265,-7.48647990851758));
#95436=CARTESIAN_POINT('Ctrl Pts',(-0.372654670650082,3.20214063476731,
-7.49113829040766));
#95437=CARTESIAN_POINT('Ctrl Pts',(-0.294969674111711,3.189931257554,-7.49460183646999));
#95438=CARTESIAN_POINT('Ctrl Pts',(-0.217131934940514,3.17766594555634,
-7.49685625596432));
#95439=CARTESIAN_POINT('Origin',(0.0471099633931913,3.08947605473442,0.177110167732994));
#95440=CARTESIAN_POINT('Origin',(-2.51534904016637E-14,2.71213386199933,
1.21701693861498E-13));
#95441=CARTESIAN_POINT('',(7.49770826960434,2.71105259871213,0.185393371624325));
#95442=CARTESIAN_POINT('',(7.49055600853578,2.6212967969219,-0.376258793102556));
#95443=CARTESIAN_POINT('Ctrl Pts',(7.49055600834388,2.621296797,-0.376258801708933));
#95444=CARTESIAN_POINT('Ctrl Pts',(7.49525383105908,2.63630241371388,-0.282734599734975));
#95445=CARTESIAN_POINT('Ctrl Pts',(7.49819984507317,2.65129140216,-0.18912734946931));
#95446=CARTESIAN_POINT('Ctrl Pts',(7.50058420320881,2.68121760799003,-0.00186233163152409));
#95447=CARTESIAN_POINT('Ctrl Pts',(7.50002300113011,2.69615247103889,0.0917806350178888));
#95448=CARTESIAN_POINT('Ctrl Pts',(7.49770826971422,2.71105259844403,0.185393371669702));
#95449=CARTESIAN_POINT('',(7.4618769614406,2.62129679727526,0.755243144934415));
#95450=CARTESIAN_POINT('Ctrl Pts',(7.4618769610079,2.6212967956465,0.755243148620498));
#95451=CARTESIAN_POINT('Ctrl Pts',(7.47412902591129,2.64052352569905,0.634191540197154));
#95452=CARTESIAN_POINT('Ctrl Pts',(7.48340741224169,2.65962575012096,0.513101823956039));
#95453=CARTESIAN_POINT('Ctrl Pts',(7.48973882790869,2.67857142921234,0.392189105781614));
#95454=CARTESIAN_POINT('Ctrl Pts',(7.49334082608902,2.68934979372956,0.323400789414678));
#95455=CARTESIAN_POINT('Ctrl Pts',(7.49600058062456,2.70017879535254,0.254456008468695));
#95456=CARTESIAN_POINT('Ctrl Pts',(7.4977082697183,2.71105259958609,0.185393367698602));
#95457=CARTESIAN_POINT('',(7.49752438375778,2.53084202102195,0.192686562343836));
#95458=CARTESIAN_POINT('Origin',(-0.192836928120053,2.55357153483116,-0.00860198345926738));
#95459=CARTESIAN_POINT('Ctrl Pts',(7.49752438400009,2.53084202125182,0.192686562386803));
#95460=CARTESIAN_POINT('Ctrl Pts',(7.49996148555515,2.54599092181985,0.0978577995033554));
#95461=CARTESIAN_POINT('Ctrl Pts',(7.50059940836,2.56110926407678,0.0029936701125065));
#95462=CARTESIAN_POINT('Ctrl Pts',(7.49827553106324,2.59126912608015,-0.186706858669859));
#95463=CARTESIAN_POINT('Ctrl Pts',(7.49531483046176,2.60630700020248,-0.281520224309993));
#95464=CARTESIAN_POINT('Ctrl Pts',(7.49055600834388,2.621296797,-0.376258801708936));
#95465=CARTESIAN_POINT('Origin',(-2.92734586571086E-13,3.22948687199989,
-6.29379361127835E-14));
#95466=CARTESIAN_POINT('',(7.49768896323947,3.22840426987216,0.186172524292213));
#95467=CARTESIAN_POINT('',(7.49059383870793,3.1385254181866,-0.375504899172903));
#95468=CARTESIAN_POINT('Ctrl Pts',(7.49059383954544,3.138525418,-0.375504901384827));
#95469=CARTESIAN_POINT('Ctrl Pts',(7.49528245578119,3.15354292291116,-0.281976109185188));
#95470=CARTESIAN_POINT('Ctrl Pts',(7.49821906806929,3.16854801594089,-0.188365088600545));
#95471=CARTESIAN_POINT('Ctrl Pts',(7.50058442244902,3.19851525233201,-0.00109164250782899));
#95472=CARTESIAN_POINT('Ctrl Pts',(7.50001352343393,3.21347503482403,0.092555979525696));
#95473=CARTESIAN_POINT('Ctrl Pts',(7.49768896335334,3.22840427113122,0.186172524314138));
#95474=CARTESIAN_POINT('',(7.4618008792551,3.13852541980614,0.755994151517736));
#95475=CARTESIAN_POINT('Ctrl Pts',(7.46180090019942,3.13852541968788,0.755994148221503));
#95476=CARTESIAN_POINT('Ctrl Pts',(7.4860504720066,3.176642188,0.516646540994622));
#95477=CARTESIAN_POINT('Ctrl Pts',(7.49491115300642,3.214285714,0.276236875994415));
#95478=CARTESIAN_POINT('Ctrl Pts',(7.49657057771863,3.22133557900681,0.231213047961645));
#95479=CARTESIAN_POINT('Ctrl Pts',(7.49768896298581,3.22840426981376,0.186172533427897));
#95480=CARTESIAN_POINT('',(7.49751856071513,3.04797057404127,0.192913013134775));
#95481=CARTESIAN_POINT('Origin',(-0.192706250093664,3.08928601452239,-0.0115877305831265));
#95482=CARTESIAN_POINT('Ctrl Pts',(7.49751856079352,3.04797057416027,0.192913012927193));
#95483=CARTESIAN_POINT('Ctrl Pts',(7.49995628036005,3.06312724666373,0.0981716192870708));
#95484=CARTESIAN_POINT('Ctrl Pts',(7.50059811512331,3.07825740178565,0.00339777623310703));
#95485=CARTESIAN_POINT('Ctrl Pts',(7.49886566753833,3.10090880536359,-0.138786407457143));
#95486=CARTESIAN_POINT('Ctrl Pts',(7.4978384436537,3.10845283708619,-0.186190544052926));
#95487=CARTESIAN_POINT('Ctrl Pts',(7.49562410846093,3.11975033430075,-0.257254972428406));
#95488=CARTESIAN_POINT('Ctrl Pts',(7.49477437391748,3.12351106931505,-0.280923510404845));
#95489=CARTESIAN_POINT('Ctrl Pts',(7.49333186628946,3.12914719309778,-0.316413682842507));
#95490=CARTESIAN_POINT('Ctrl Pts',(7.49282321344814,3.13102454043743,-0.32823828869302));
#95491=CARTESIAN_POINT('Ctrl Pts',(7.49174678273641,3.13478885687642,-0.351954356252219));
#95492=CARTESIAN_POINT('Ctrl Pts',(7.49118216168839,3.13666362993207,-0.363769016638318));
#95493=CARTESIAN_POINT('Ctrl Pts',(7.49059383965076,3.13852541766671,-0.375504899283886));
#95494=CARTESIAN_POINT('Origin',(-2.82179343832881E-14,2.8407150569993,
4.6750797677575E-13));
#95495=CARTESIAN_POINT('',(0.344853648470777,2.75,-7.49206753559307));
#95496=CARTESIAN_POINT('',(-0.21812170991374,2.83963938431667,-7.49682752354381));
#95497=CARTESIAN_POINT('Ctrl Pts',(-0.218121710046857,2.83963938326183,
-7.49682752366668));
#95498=CARTESIAN_POINT('Ctrl Pts',(-0.124301827177169,2.8246344539578,-7.49955723209645));
#95499=CARTESIAN_POINT('Ctrl Pts',(-0.0304342443090152,2.80965517837476,
-7.50052565814021));
#95500=CARTESIAN_POINT('Ctrl Pts',(0.157272188344805,2.77976775476086,-7.49893806965916));
#95501=CARTESIAN_POINT('Ctrl Pts',(0.251096123377212,2.76486196385957,-7.49638311684237));
#95502=CARTESIAN_POINT('Ctrl Pts',(0.344853647954533,2.75000000170506,-7.49206753583365));
#95503=CARTESIAN_POINT('',(-0.218121709913735,2.66036061568333,-7.49682752354381));
#95504=CARTESIAN_POINT('Ctrl Pts',(0.344853648348658,2.74999999835741,-7.49206753581551));
#95505=CARTESIAN_POINT('Ctrl Pts',(0.251096125186365,2.7351380364273,-7.49638311676404));
#95506=CARTESIAN_POINT('Ctrl Pts',(0.157272191176333,2.72023224568898,-7.49893806958205));
#95507=CARTESIAN_POINT('Ctrl Pts',(-0.0304342414766552,2.69034482207722,
-7.50052565816943));
#95508=CARTESIAN_POINT('Ctrl Pts',(-0.124301825761971,2.67536554626854,
-7.49955723213764));
#95509=CARTESIAN_POINT('Ctrl Pts',(-0.218121710046853,2.66036061673817,
-7.49682752366669));
#95510=CARTESIAN_POINT('',(-0.786518123685502,2.75,-7.45864526828673));
#95511=CARTESIAN_POINT('Ctrl Pts',(-0.786518123401192,2.75000000173934,
-7.45864526821688));
#95512=CARTESIAN_POINT('Ctrl Pts',(-0.635720241859938,2.72598918212309,
-7.47454698532651));
#95513=CARTESIAN_POINT('Ctrl Pts',(-0.484816616171727,2.70215892392458,
-7.48583171136412));
#95514=CARTESIAN_POINT('Ctrl Pts',(-0.334222996511701,2.67857142890602,
-7.49254929789627));
#95515=CARTESIAN_POINT('Ctrl Pts',(-0.295567349309514,2.67251679064144,
-7.49427362521657));
#95516=CARTESIAN_POINT('Ctrl Pts',(-0.256864644539784,2.66644617679107,
-7.49570028979618));
#95517=CARTESIAN_POINT('Ctrl Pts',(-0.218121709824728,2.66036061481515,
-7.49682752356268));
#95518=CARTESIAN_POINT('Ctrl Pts',(-0.218121709824731,2.83963938518485,
-7.49682752356268));
#95519=CARTESIAN_POINT('Ctrl Pts',(-0.256864644539786,2.83355382320893,
-7.49570028979618));
#95520=CARTESIAN_POINT('Ctrl Pts',(-0.295567349307819,2.82748320939227,
-7.49427362497814));
#95521=CARTESIAN_POINT('Ctrl Pts',(-0.33422299662364,2.82142857109398,-7.49254929776551));
#95522=CARTESIAN_POINT('Ctrl Pts',(-0.484816616726417,2.7978410759441,-7.48583171165279));
#95523=CARTESIAN_POINT('Ctrl Pts',(-0.635720241859905,2.77401081787673,
-7.4745469853265));
#95524=CARTESIAN_POINT('Ctrl Pts',(-0.786518123401192,2.74999999826065,
-7.45864526821688));
#95525=CARTESIAN_POINT('Origin',(-8.38095573446691E-14,3.100341677,-4.9439619065339E-14));
#95526=CARTESIAN_POINT('',(0.353161049945379,3.00855922064419,-7.49168053798488));
#95527=CARTESIAN_POINT('',(-0.214163364586773,3.09925366864577,-7.49694162681412));
#95528=CARTESIAN_POINT('Ctrl Pts',(-0.214163365287477,3.09925366540454,
-7.49694164662956));
#95529=CARTESIAN_POINT('Ctrl Pts',(-0.119615787895196,3.08419557051511,
-7.49964256499181));
#95530=CARTESIAN_POINT('Ctrl Pts',(-0.0250402831176017,3.06910470896703,
-7.50055449258533));
#95531=CARTESIAN_POINT('Ctrl Pts',(0.11681030494971,3.04642798792313,-7.49923934606818));
#95532=CARTESIAN_POINT('Ctrl Pts',(0.16408237326809,3.03886383885786,-7.49835396754483));
#95533=CARTESIAN_POINT('Ctrl Pts',(0.23498468663855,3.02750792812686,-7.49635522220983));
#95534=CARTESIAN_POINT('Ctrl Pts',(0.25862389735179,3.02372003573565,-7.49557690126512));
#95535=CARTESIAN_POINT('Ctrl Pts',(0.294079065058776,3.01803612480972,-7.49424161735081));
#95536=CARTESIAN_POINT('Ctrl Pts',(0.305898173867865,3.01614092940207,-7.49376849262521));
#95537=CARTESIAN_POINT('Ctrl Pts',(0.329632892545769,3.01233417470685,-7.49276213568984));
#95538=CARTESIAN_POINT('Ctrl Pts',(0.341448322432607,3.01043867559549,-7.49223268032143));
#95539=CARTESIAN_POINT('Ctrl Pts',(0.353161055097876,3.00855921997396,-7.49168053704654));
#95540=CARTESIAN_POINT('',(-0.214686789545212,2.91791835699471,-7.49692666437975));
#95541=CARTESIAN_POINT('Ctrl Pts',(0.353161051407822,3.00855922143352,-7.4916805372205));
#95542=CARTESIAN_POINT('Ctrl Pts',(0.34143732161125,3.00667973111906,-7.49223319889911));
#95543=CARTESIAN_POINT('Ctrl Pts',(0.329609338416344,3.00478403192845,-7.49276319431832));
#95544=CARTESIAN_POINT('Ctrl Pts',(0.305848447833043,3.00097686606387,-7.49377054140901));
#95545=CARTESIAN_POINT('Ctrl Pts',(0.294017229147902,2.99908168399852,-7.49424406272989));
#95546=CARTESIAN_POINT('Ctrl Pts',(0.258527072016622,2.99339823798258,-7.49558031366932));
#95547=CARTESIAN_POINT('Ctrl Pts',(0.234864945505131,2.98961100215531,-7.49635904719672));
#95548=CARTESIAN_POINT('Ctrl Pts',(0.163899259634153,2.97825875917154,-7.49835822711598));
#95549=CARTESIAN_POINT('Ctrl Pts',(0.116586598825047,2.97069843941478,-7.49924308424233));
#95550=CARTESIAN_POINT('Ctrl Pts',(-0.0253904821596797,2.94803581687887,
-7.50055439646177));
#95551=CARTESIAN_POINT('Ctrl Pts',(-0.120062227954501,2.93295693655023,
-7.49963653001752));
#95552=CARTESIAN_POINT('Ctrl Pts',(-0.214696662028744,2.91791679016923,
-7.49692639308361));
#95553=CARTESIAN_POINT('',(-0.778247084124863,3.00855922118781,-7.45951282173075));
#95554=CARTESIAN_POINT('Origin',(0.0100862188859288,2.94642870621689,0.192647581726551));
#95555=CARTESIAN_POINT('Origin',(0.00710118688749452,3.08928538820124,0.192748080609783));
#95556=CARTESIAN_POINT('Origin',(-1.53436291450149E-12,2.97023924200033,
-1.48345962250329E-13));
#95557=CARTESIAN_POINT('',(7.49752438375815,2.96915797897799,0.192686562343938));
#95558=CARTESIAN_POINT('',(7.49055600845813,2.87870320295594,-0.37625879506456));
#95559=CARTESIAN_POINT('Ctrl Pts',(7.49055600834388,2.878703203,-0.376258801708937));
#95560=CARTESIAN_POINT('Ctrl Pts',(7.4953148304482,2.8936929997548,-0.281520224579953));
#95561=CARTESIAN_POINT('Ctrl Pts',(7.49827553104638,2.90873087383415,-0.18670685921018));
#95562=CARTESIAN_POINT('Ctrl Pts',(7.50059940835647,2.93889073574426,0.00299366898818003));
#95563=CARTESIAN_POINT('Ctrl Pts',(7.49996148554706,2.9540090782303,0.0978577998172472));
#95564=CARTESIAN_POINT('Ctrl Pts',(7.49752438400006,2.96915797874819,0.192686562386881));
#95565=CARTESIAN_POINT('',(7.46187696234892,2.87870320365575,0.755243147028956));
#95566=CARTESIAN_POINT('Origin',(-0.192836927089979,2.9464284653058,-0.00860198342095067));
#95567=CARTESIAN_POINT('',(7.49770826960434,2.78894740128786,0.185393371623732));
#95568=CARTESIAN_POINT('Ctrl Pts',(7.4977082697184,2.7889474004133,0.185393367694706));
#95569=CARTESIAN_POINT('Ctrl Pts',(7.49600058062463,2.79982120464723,0.254456008467217));
#95570=CARTESIAN_POINT('Ctrl Pts',(7.49334082631797,2.81065020634723,0.323400789690236));
#95571=CARTESIAN_POINT('Ctrl Pts',(7.48973882790671,2.82142857078767,0.392189105783304));
#95572=CARTESIAN_POINT('Ctrl Pts',(7.48340741183381,2.84037424974404,0.513101823476185));
#95573=CARTESIAN_POINT('Ctrl Pts',(7.47412902590999,2.85947647430091,0.634191540197448));
#95574=CARTESIAN_POINT('Ctrl Pts',(7.46187696100449,2.87870320435315,0.755243148621063));
#95575=CARTESIAN_POINT('Ctrl Pts',(7.49770826971422,2.78894740155606,0.185393371669134));
#95576=CARTESIAN_POINT('Ctrl Pts',(7.50002300113748,2.80384752900865,0.0917806347191898));
#95577=CARTESIAN_POINT('Ctrl Pts',(7.50058420321237,2.81878239210518,-0.0018623322285248));
#95578=CARTESIAN_POINT('Ctrl Pts',(7.49819984505442,2.84870859793545,-0.189127350065385));
#95579=CARTESIAN_POINT('Ctrl Pts',(7.49525383104411,2.86369758633394,-0.282734600033004));
#95580=CARTESIAN_POINT('Ctrl Pts',(7.49055600834388,2.878703203,-0.376258801708931));
#95581=CARTESIAN_POINT('Ctrl Pts',(0.201304349,3.009344995,7.247204741));
#95582=CARTESIAN_POINT('Ctrl Pts',(0.598071101,2.943588707,7.23618382));
#95583=CARTESIAN_POINT('Ctrl Pts',(0.991263374999999,2.878703203,7.181914572));
#95584=CARTESIAN_POINT('Ctrl Pts',(-0.037736949,3.009344995,7.499905061));
#95585=CARTESIAN_POINT('Ctrl Pts',(0.372864527,2.943588707,7.501971067));
#95586=CARTESIAN_POINT('Ctrl Pts',(0.781237513,2.878703203,7.459200222));
#95587=CARTESIAN_POINT('',(0.213503817067261,2.96915797893806,7.49696045860227));
#95588=CARTESIAN_POINT('',(0.781237505398224,2.87870320271434,7.45920022318093));
#95589=CARTESIAN_POINT('Origin',(0.0138847566270039,3.0892087125302,-0.187163919861857));
#95590=CARTESIAN_POINT('',(0.991263371067069,2.8787032034874,7.18191455661634));
#95591=CARTESIAN_POINT('',(0.886250438692909,2.87870320212873,7.32055739764249));
#95592=CARTESIAN_POINT('',(0.20604568399897,3.00855922136916,7.24707150249123));
#95593=CARTESIAN_POINT('Origin',(0.0078833829971733,3.08923052942512,-0.195171233689059));
#95594=CARTESIAN_POINT('Ctrl Pts',(0.213503815207119,2.9691579789368,7.49696045865927));
#95595=CARTESIAN_POINT('Ctrl Pts',(0.212222310116716,2.97541038103787,7.45527257747656));
#95596=CARTESIAN_POINT('Ctrl Pts',(0.210958287707541,2.98181495147342,7.41358339843693));
#95597=CARTESIAN_POINT('Ctrl Pts',(0.20847147405997,2.99493785104416,7.33030086491618));
#95598=CARTESIAN_POINT('Ctrl Pts',(0.207247253797146,3.00166370045464,7.28865974186892));
#95599=CARTESIAN_POINT('Ctrl Pts',(0.206045688483612,3.00855921915399,7.24707150199437));
#95600=CARTESIAN_POINT('Ctrl Pts',(0.961669527891964,2.87421362525411,7.18350692905047));
#95601=CARTESIAN_POINT('Ctrl Pts',(0.975080023200985,2.87645841412705,7.18166062121529));
#95602=CARTESIAN_POINT('Ctrl Pts',(0.988490518509999,2.878703203,7.17981431338));
#95603=CARTESIAN_POINT('Ctrl Pts',(1.37865591428,2.944013165,7.12609777192));
#95604=CARTESIAN_POINT('Ctrl Pts',(1.76070279869,3.00933735,7.03041767896));
#95605=CARTESIAN_POINT('Ctrl Pts',(0.964434538633709,2.87421362525411,7.18561754598276));
#95606=CARTESIAN_POINT('Ctrl Pts',(0.977848956816862,2.87645841412705,7.1837660589914));
#95607=CARTESIAN_POINT('Ctrl Pts',(0.991263375,2.878703203,7.181914572));
#95608=CARTESIAN_POINT('Ctrl Pts',(1.381542903,2.944013165,7.128047348));
#95609=CARTESIAN_POINT('Ctrl Pts',(1.763686919,3.00933735,7.032205092));
#95610=CARTESIAN_POINT('Ctrl Pts',(1.2415009216866,2.87421362525411,7.3971107566939));
#95611=CARTESIAN_POINT('Ctrl Pts',(1.25530842931717,2.87645841412705,7.39474029520778));
#95612=CARTESIAN_POINT('Ctrl Pts',(1.26911593694774,2.878703203,7.39236983372176));
#95613=CARTESIAN_POINT('Ctrl Pts',(1.67083202238253,2.944013165,7.32340354854395));
#95614=CARTESIAN_POINT('Ctrl Pts',(2.06270905602152,3.00933735,7.21131183416782));
#95615=CARTESIAN_POINT('',(1.26854901500601,2.87870320364628,7.39194043595267));
#95616=CARTESIAN_POINT('',(1.82013710546423,2.96915797900293,7.27578867997919));
#95617=CARTESIAN_POINT('Origin',(-0.0433008801937831,2.94642849080139,-0.18810913934697));
#95618=CARTESIAN_POINT('',(1.75913460167935,3.00855922008955,7.033345266035));
#95619=CARTESIAN_POINT('Ctrl Pts',(1.75913460568618,3.00855921928539,7.03334526489348));
#95620=CARTESIAN_POINT('Ctrl Pts',(1.76924832116047,3.00166370059594,7.07370289367572));
#95621=CARTESIAN_POINT('Ctrl Pts',(1.77939553036737,2.99493785113426,7.11410729951582));
#95622=CARTESIAN_POINT('Ctrl Pts',(1.79972748647054,2.98181495154672,7.19490814237825));
#95623=CARTESIAN_POINT('Ctrl Pts',(1.80992389783552,2.97541038112898,7.23535092406372));
#95624=CARTESIAN_POINT('Ctrl Pts',(1.82013710423511,2.9691579790021,7.27578868028949));
#95625=CARTESIAN_POINT('Origin',(-0.0383633275899339,2.9464287300554,-0.19584155044102));
#95626=CARTESIAN_POINT('',(1.12990618766699,2.87870320492457,7.28692750483482));
#95627=CARTESIAN_POINT('Origin',(9.36750677027476E-14,2.970239242,2.02962646689286E-13));
#95628=CARTESIAN_POINT('',(1.8272136544172,2.78894740126616,7.27401472765982));
#95629=CARTESIAN_POINT('Ctrl Pts',(1.8272136579114,2.78894740043443,7.27401472665859));
#95630=CARTESIAN_POINT('Ctrl Pts',(1.76021149589788,2.79982120465073,7.29084549616711));
#95631=CARTESIAN_POINT('Ctrl Pts',(1.69306819303316,2.81065020634441,7.30672737246874));
#95632=CARTESIAN_POINT('Ctrl Pts',(1.62582357463571,2.8214285708981,7.32165949085884));
#95633=CARTESIAN_POINT('Ctrl Pts',(1.50762429158704,2.84037425004919,7.34790643447895));
#95634=CARTESIAN_POINT('Ctrl Pts',(1.3884660660231,2.85947647430085,7.37136117628156));
#95635=CARTESIAN_POINT('Ctrl Pts',(1.26854901542685,2.87870320435315,7.39194043534716));
#95636=CARTESIAN_POINT('',(2.36648016283983,2.87870320271433,7.11686529676572));
#95637=CARTESIAN_POINT('Origin',(-0.0703573075978353,2.9464046053574,-0.177135214929172));
#95638=CARTESIAN_POINT('Origin',(-0.0266746805751597,3.08920866307571,-0.185773302501384));
#95639=CARTESIAN_POINT('Ctrl Pts',(1.754532759,3.009344995,7.034494637));
#95640=CARTESIAN_POINT('Ctrl Pts',(2.139654152,2.943588707,6.938438256));
#95641=CARTESIAN_POINT('Ctrl Pts',(2.511987525,2.878703203,6.800913077));
#95642=CARTESIAN_POINT('Ctrl Pts',(1.575403212,3.009344995,7.332673777));
#95643=CARTESIAN_POINT('Ctrl Pts',(1.976849185,2.943588707,7.2464243));
#95644=CARTESIAN_POINT('Ctrl Pts',(2.36648017,2.878703203,7.116865294));
#95645=CARTESIAN_POINT('',(2.51198751841429,2.8787032034984,6.80091306248545));
#95646=CARTESIAN_POINT('',(2.43923384245511,2.87870320212873,6.95888918726834));
#95647=CARTESIAN_POINT('Origin',(-0.034256928265696,3.08923055943144,-0.192302861328456));
#95648=CARTESIAN_POINT('Ctrl Pts',(2.48342787635727,2.87421362543563,6.80883000765615));
#95649=CARTESIAN_POINT('Ctrl Pts',(2.49612793959364,2.87645841421781,6.80414400555299));
#95650=CARTESIAN_POINT('Ctrl Pts',(2.50882800283,2.878703203,6.79945800345));
#95651=CARTESIAN_POINT('Ctrl Pts',(2.87832407923,2.944013165,6.66312329717));
#95652=CARTESIAN_POINT('Ctrl Pts',(3.23087052879,3.00933735,6.48755136434));
#95653=CARTESIAN_POINT('Ctrl Pts',(2.48658196293872,2.87421362543563,6.81029688395002));
#95654=CARTESIAN_POINT('Ctrl Pts',(2.49928474396936,2.87645841421781,6.80560498047503));
#95655=CARTESIAN_POINT('Ctrl Pts',(2.511987525,2.878703203,6.800913077));
#95656=CARTESIAN_POINT('Ctrl Pts',(2.881562673,2.944013165,6.664406676));
#95657=CARTESIAN_POINT('Ctrl Pts',(3.234169123,3.00933735,6.488655491));
#95658=CARTESIAN_POINT('Ctrl Pts',(2.8026354768333,2.87421362543563,6.95728441748712));
#95659=CARTESIAN_POINT('Ctrl Pts',(2.81561059294661,2.87645841421781,6.95200117027104));
#95660=CARTESIAN_POINT('Ctrl Pts',(2.82858570905992,2.878703203,6.94671792305481));
#95661=CARTESIAN_POINT('Ctrl Pts',(3.20608418331742,2.944013165,6.79300694691974));
#95662=CARTESIAN_POINT('Ctrl Pts',(3.56470294445965,3.00933735,6.59929389665744));
#95663=CARTESIAN_POINT('',(2.82793973365375,2.87870320364628,6.94642043584862));
#95664=CARTESIAN_POINT('',(3.34166280795495,2.96915797895592,6.71440910846434));
#95665=CARTESIAN_POINT('Origin',(-0.0827265550078515,2.94642849629458,-0.174403114624736));
#95666=CARTESIAN_POINT('',(3.22996834025014,3.00855922010428,6.49074762261723));
#95667=CARTESIAN_POINT('Ctrl Pts',(3.22996834425851,3.00855921924352,6.49074762046088));
#95668=CARTESIAN_POINT('Ctrl Pts',(3.24852130392303,3.00166370057168,6.52798756039884));
#95669=CARTESIAN_POINT('Ctrl Pts',(3.26711702995854,2.99493785111864,6.56526598359234));
#95670=CARTESIAN_POINT('Ctrl Pts',(3.30434341445289,2.98181495668542,6.63980694870173));
#95671=CARTESIAN_POINT('Ctrl Pts',(3.32299542485086,2.97541039175451,6.67711223927901));
#95672=CARTESIAN_POINT('Ctrl Pts',(3.34166280629983,2.96915797895513,6.71440910928904));
#95673=CARTESIAN_POINT('Origin',(-0.0795666252702048,2.94642872170379,-0.183016063846523));
#95674=CARTESIAN_POINT('',(2.66996362233808,2.87870320492457,6.87366675883567));
#95675=CARTESIAN_POINT('Origin',(-9.73613550891983E-14,2.97023924200033,
-3.51715184754298E-13));
#95676=CARTESIAN_POINT('',(3.34819256234159,2.78894740128846,6.71115538203976));
#95677=CARTESIAN_POINT('Ctrl Pts',(3.3481925660512,2.78894740039827,6.71115538033786));
#95678=CARTESIAN_POINT('Ctrl Pts',(3.2863749950435,2.79982120464277,6.74199614030772));
#95679=CARTESIAN_POINT('Ctrl Pts',(3.22421559910966,2.81065020634769,6.77194053268262));
#95680=CARTESIAN_POINT('Ctrl Pts',(3.16175308677193,2.82142857082205,6.80097915141608));
#95681=CARTESIAN_POINT('Ctrl Pts',(3.05195955474273,2.84037424983904,6.85202180653093));
#95682=CARTESIAN_POINT('Ctrl Pts',(2.94062925804189,2.8594764743009,6.9005436862566));
#95683=CARTESIAN_POINT('Ctrl Pts',(2.82793973391688,2.87870320435315,6.94642043515864));
#95684=CARTESIAN_POINT('',(3.84106883658366,2.87870320271408,6.44175365830848));
#95685=CARTESIAN_POINT('Origin',(-0.106791214160791,2.94640461889648,-0.15786910551179));
#95686=CARTESIAN_POINT('Origin',(-0.0659866315263863,3.08920870918657,-0.17569542356631));
#95687=CARTESIAN_POINT('Ctrl Pts',(3.225721167,3.009344995,6.492859382));
#95688=CARTESIAN_POINT('Ctrl Pts',(3.581189353,2.943588707,6.31625903));
#95689=CARTESIAN_POINT('Ctrl Pts',(3.91525393,2.878703203,6.101908444));
#95690=CARTESIAN_POINT('Ctrl Pts',(3.114879271,3.009344995,6.822574817));
#95691=CARTESIAN_POINT('Ctrl Pts',(3.488398571,2.943588707,6.652042788));
#95692=CARTESIAN_POINT('Ctrl Pts',(3.841068843,2.878703203,6.441753654));
#95693=CARTESIAN_POINT('',(3.91525392053432,2.87870320349625,6.10190843154593));
#95694=CARTESIAN_POINT('',(3.87816138194936,2.87870320212799,6.27183105181387));
#95695=CARTESIAN_POINT('Origin',(-0.0747953746061175,3.08923058068278,-0.180442555176319));
#95696=CARTESIAN_POINT('Ctrl Pts',(3.88906389553692,2.87421362532651,6.11577976177853));
#95697=CARTESIAN_POINT('Ctrl Pts',(3.90045968671849,2.87645841416325,6.10847317745435));
#95698=CARTESIAN_POINT('Ctrl Pts',(3.9118554779,2.878703203,6.10116659312999));
#95699=CARTESIAN_POINT('Ctrl Pts',(4.24340501024,2.944013165,5.88858858277999));
#95700=CARTESIAN_POINT('Ctrl Pts',(4.5499663445,3.00933735,5.64133435845));
#95701=CARTESIAN_POINT('Ctrl Pts',(3.89245957637044,2.87421362532651,6.11653430794216));
#95702=CARTESIAN_POINT('Ctrl Pts',(3.90385675318525,2.87645841416325,6.10922137597116));
#95703=CARTESIAN_POINT('Ctrl Pts',(3.91525393,2.878703203,6.101908444));
#95704=CARTESIAN_POINT('Ctrl Pts',(4.246843776,2.944013165,5.889145755));
#95705=CARTESIAN_POINT('Ctrl Pts',(4.553425174,3.00933735,5.641703571));
#95706=CARTESIAN_POINT('Ctrl Pts',(4.23272190964473,2.87421362532651,6.19214319192831));
#95707=CARTESIAN_POINT('Ctrl Pts',(4.24425793307692,2.87645841416325,6.1841941974943));
#95708=CARTESIAN_POINT('Ctrl Pts',(4.25579395650913,2.878703203,6.17624520306029));
#95709=CARTESIAN_POINT('Ctrl Pts',(4.59142341067223,2.944013165,5.9449768913485));
#95710=CARTESIAN_POINT('Ctrl Pts',(4.90001528472145,3.00933735,5.6787003118293));
#95711=CARTESIAN_POINT('',(4.25509913271638,2.87870320364628,6.17609353656161));
#95712=CARTESIAN_POINT('',(4.7069360695642,2.96915797893838,5.83907123054069));
#95713=CARTESIAN_POINT('Origin',(-0.11828387119569,2.94642851897792,-0.152541778771623));
#95714=CARTESIAN_POINT('',(4.54977234856429,3.00855922012106,5.64464983369177));
#95715=CARTESIAN_POINT('Ctrl Pts',(4.54977235220724,3.00855921929496,5.64464983057676));
#95716=CARTESIAN_POINT('Ctrl Pts',(4.57589704002969,3.00166370067037,5.67703078343159));
#95717=CARTESIAN_POINT('Ctrl Pts',(4.6020717677554,2.99493785110817,5.70944012703413));
#95718=CARTESIAN_POINT('Ctrl Pts',(4.65445194454172,2.98181495155238,5.77423581901457));
#95719=CARTESIAN_POINT('Ctrl Pts',(4.68068744031158,2.97541038108866,5.80665933175871));
#95720=CARTESIAN_POINT('Ctrl Pts',(4.70693606860236,2.96915797893756,5.83907123131948));
#95721=CARTESIAN_POINT('Origin',(-0.117049403438313,2.9464287394627,-0.161632706015527));
#95722=CARTESIAN_POINT('',(4.08517652503108,2.87870320492457,6.13900099413378));
#95723=CARTESIAN_POINT('Origin',(1.07769695945059E-12,2.97023924199989,
1.36609473733174E-12));
#95724=CARTESIAN_POINT('',(4.71261370775459,2.78894740132767,5.83448986989326));
#95725=CARTESIAN_POINT('Ctrl Pts',(4.71261371106242,2.78894740043244,5.83448986742808));
#95726=CARTESIAN_POINT('Ctrl Pts',(4.6588712522757,2.79982120466691,5.87789853788241));
#95727=CARTESIAN_POINT('Ctrl Pts',(4.60460226762575,2.81065020636038,5.92050527960023));
#95728=CARTESIAN_POINT('Ctrl Pts',(4.5498425389075,2.82142857082138,5.96229258530749));
#95729=CARTESIAN_POINT('Ctrl Pts',(4.45358858163541,2.84037424983719,6.03574425558343));
#95730=CARTESIAN_POINT('Ctrl Pts',(4.35529189432717,2.85947647430089,6.10706444342323));
#95731=CARTESIAN_POINT('Ctrl Pts',(4.25509913278488,2.87870320435315,6.17609353582243));
#95732=CARTESIAN_POINT('',(5.13605340166303,2.87870320271433,5.4654327785827));
#95733=CARTESIAN_POINT('Origin',(-0.138231745003453,2.94640460767842,-0.131221324898843));
#95734=CARTESIAN_POINT('Origin',(-0.102213261567797,3.08920872757977,-0.15740263547115));
#95735=CARTESIAN_POINT('Ctrl Pts',(4.546078438,3.009344995,5.647625239));
#95736=CARTESIAN_POINT('Ctrl Pts',(4.85527212,2.943588707,5.398738552));
#95737=CARTESIAN_POINT('Ctrl Pts',(5.135447414,2.878703203,5.117585355));
#95738=CARTESIAN_POINT('Ctrl Pts',(4.508707036,3.009344995,5.993459841));
#95739=CARTESIAN_POINT('Ctrl Pts',(4.83683431699999,2.943588707,5.746619148));
#95740=CARTESIAN_POINT('Ctrl Pts',(5.136053407,2.878703203,5.465432773));
#95741=CARTESIAN_POINT('',(5.13544740171401,2.87870320347604,5.11758534466438));
#95742=CARTESIAN_POINT('',(5.13575040666388,2.87870320212873,5.2915090677232));
#95743=CARTESIAN_POINT('Origin',(-0.111836554344424,3.08923061262737,-0.160145186282088));
#95744=CARTESIAN_POINT('Ctrl Pts',(5.11285161102639,2.87421362525373,5.13676245265013));
#95745=CARTESIAN_POINT('Ctrl Pts',(5.1224102754232,2.87645841412686,5.12717693379505));
#95746=CARTESIAN_POINT('Ctrl Pts',(5.13196893981999,2.878703203,5.11759141494));
#95747=CARTESIAN_POINT('Ctrl Pts',(5.41006903912,2.944013165,4.83871001114));
#95748=CARTESIAN_POINT('Ctrl Pts',(5.65631079023,3.00933735,4.53133482854));
#95749=CARTESIAN_POINT('Ctrl Pts',(5.11633010784345,2.87421362525373,5.13676938693466));
#95750=CARTESIAN_POINT('Ctrl Pts',(5.12588876092166,2.87645841412686,5.12717737096732));
#95751=CARTESIAN_POINT('Ctrl Pts',(5.135447414,2.878703203,5.117585355));
#95752=CARTESIAN_POINT('Ctrl Pts',(5.413547184,2.944013165,4.838514924));
#95753=CARTESIAN_POINT('Ctrl Pts',(5.65976812400001,3.00933735,4.530951863));
#95754=CARTESIAN_POINT('Ctrl Pts',(5.46489097127091,2.87421362525373,5.13746423310858));
#95755=CARTESIAN_POINT('Ctrl Pts',(5.47444849018795,2.87645841412686,5.12722117757431));
#95756=CARTESIAN_POINT('Ctrl Pts',(5.48400600910502,2.878703203,5.11697812203994));
#95757=CARTESIAN_POINT('Ctrl Pts',(5.76207278177934,2.944013165,4.81896632426267));
#95758=CARTESIAN_POINT('Ctrl Pts',(6.0062083559296,3.00933735,4.49257701135858));
#95759=CARTESIAN_POINT('',(5.4832948306121,2.87870320365809,5.11697936510087));
#95760=CARTESIAN_POINT('',(5.85211823264346,2.9691579789893,4.69070487109329));
#95761=CARTESIAN_POINT('Origin',(-0.14831033925738,2.94642847277019,-0.123547826397968));
#95762=CARTESIAN_POINT('',(5.656834059487,3.00855922008602,4.53461449353195));
#95763=CARTESIAN_POINT('Ctrl Pts',(5.65683406228931,3.00855921918535,4.53461448979404));
#95764=CARTESIAN_POINT('Ctrl Pts',(5.68930891736726,3.00166370050065,4.56062235843146));
#95765=CARTESIAN_POINT('Ctrl Pts',(5.72183874466791,2.9949378510848,4.58664719622671));
#95766=CARTESIAN_POINT('Ctrl Pts',(5.78692346058031,2.98181495152155,4.63866781124971));
#95767=CARTESIAN_POINT('Ctrl Pts',(5.81951568171008,2.97541038109961,4.66469342404267));
#95768=CARTESIAN_POINT('Ctrl Pts',(5.852118231867,2.96915797898848,4.69070487206631));
#95769=CARTESIAN_POINT('Origin',(-0.149059046436379,2.94642874945867,-0.132691610561059));
#95770=CARTESIAN_POINT('',(5.30937111469021,2.87870320492457,5.11728236662172));
#95771=CARTESIAN_POINT('Origin',(-4.69242700251726E-13,2.97023924200033,
-3.59521440396193E-13));
#95772=CARTESIAN_POINT('',(5.85667827404667,2.78894740128657,4.68501009565305));
#95773=CARTESIAN_POINT('Ctrl Pts',(5.85667827417289,2.78894740104823,4.68501009580207));
#95774=CARTESIAN_POINT('Ctrl Pts',(5.81352386782961,2.799821204639,4.73895693236775));
#95775=CARTESIAN_POINT('Ctrl Pts',(5.76968285191742,2.81065020634729,4.79223377956724));
#95776=CARTESIAN_POINT('Ctrl Pts',(5.72518641047971,2.8214285708838,4.84481584443312));
#95777=CARTESIAN_POINT('Ctrl Pts',(5.64697275514493,2.84037424976446,4.93724201088193));
#95778=CARTESIAN_POINT('Ctrl Pts',(5.56630592368743,2.85947647380641,5.02802565260594));
#95779=CARTESIAN_POINT('Ctrl Pts',(5.48329482921344,2.8787032036066,5.11697936380678));
#95780=CARTESIAN_POINT('',(6.19088181798404,2.87870320271433,4.233554336582));
#95781=CARTESIAN_POINT('Origin',(-0.163208569815573,2.94640456450875,-0.0984376413161392));
#95782=CARTESIAN_POINT('Origin',(-0.133660425928305,3.08920869346161,-0.13174977378177));
#95783=CARTESIAN_POINT('Ctrl Pts',(5.653866134,3.009344995,4.538314416));
#95784=CARTESIAN_POINT('Ctrl Pts',(5.902327759,2.943588707,4.22877906));
#95785=CARTESIAN_POINT('Ctrl Pts',(6.115513083,2.878703203,3.893969662));
#95786=CARTESIAN_POINT('Ctrl Pts',(5.691712671,3.009344995,4.884097344));
#95787=CARTESIAN_POINT('Ctrl Pts',(5.959105067,2.943588707,4.572489983));
#95788=CARTESIAN_POINT('Ctrl Pts',(6.19088182200001,2.878703203,4.23355433));
#95789=CARTESIAN_POINT('',(6.11551306924178,2.87870320348678,3.89396965459726));
#95790=CARTESIAN_POINT('',(6.15319744955395,2.87870320212873,4.06376200046081));
#95791=CARTESIAN_POINT('Origin',(-0.143648542792849,3.08923055370613,-0.132359630470066));
#95792=CARTESIAN_POINT('Ctrl Pts',(6.09756806636714,2.87421362525822,3.91755583942908));
#95793=CARTESIAN_POINT('Ctrl Pts',(6.10484265133856,2.87645841412911,3.90613959440954));
#95794=CARTESIAN_POINT('Ctrl Pts',(6.11211723631001,2.878703203,3.89472334939));
#95795=CARTESIAN_POINT('Ctrl Pts',(6.32376425318999,2.944013165,3.56257873745));
#95796=CARTESIAN_POINT('Ctrl Pts',(6.49817243005,3.00933735,3.20945511758));
#95797=CARTESIAN_POINT('Ctrl Pts',(6.10096672854019,2.87421362525822,3.91681483759963));
#95798=CARTESIAN_POINT('Ctrl Pts',(6.10823990577015,2.87645841412911,3.90539224979982));
#95799=CARTESIAN_POINT('Ctrl Pts',(6.115513083,2.878703203,3.893969662));
#95800=CARTESIAN_POINT('Ctrl Pts',(6.32711914299999,2.944013165,3.561640513));
#95801=CARTESIAN_POINT('Ctrl Pts',(6.501466607,3.00933735,3.208337881));
#95802=CARTESIAN_POINT('Ctrl Pts',(6.44152780532348,2.87421362525822,3.84256315617861));
#95803=CARTESIAN_POINT('Ctrl Pts',(6.44865992058245,2.87645841412911,3.83050499356452));
#95804=CARTESIAN_POINT('Ctrl Pts',(6.45579203584133,2.878703203,3.81844683095049));
#95805=CARTESIAN_POINT('Ctrl Pts',(6.66329403417121,2.944013165,3.46762624718633));
#95806=CARTESIAN_POINT('Ctrl Pts',(6.8315577993736,3.00933735,3.09638580299897));
#95807=CARTESIAN_POINT('',(6.45509774771361,2.87870320364628,3.81860093110838));
#95808=CARTESIAN_POINT('',(6.72366185127656,2.96915797897381,3.32300636522837));
#95809=CARTESIAN_POINT('Origin',(-0.171402023084778,2.94642845415883,-0.0887769886318324));
#95810=CARTESIAN_POINT('',(6.49938849676149,3.00855922009366,3.21254561858901));
#95811=CARTESIAN_POINT('Ctrl Pts',(6.49938849887401,3.00855921919985,3.21254561397554));
#95812=CARTESIAN_POINT('Ctrl Pts',(6.53669503270114,3.00166370052502,3.23096429927456));
#95813=CARTESIAN_POINT('Ctrl Pts',(6.57405890158005,2.99493785108369,3.2493877396616));
#95814=CARTESIAN_POINT('Ctrl Pts',(6.64880486723471,2.98181495152726,3.28620085165117));
#95815=CARTESIAN_POINT('Ctrl Pts',(6.68622983778637,2.97541038108343,3.30461163604335));
#95816=CARTESIAN_POINT('Ctrl Pts',(6.72366185073906,2.96915797897302,3.32300636632187));
#95817=CARTESIAN_POINT('Origin',(-0.174099247004787,2.94642876633121,-0.097546256532349));
#95818=CARTESIAN_POINT('',(6.2853054112379,2.87870320492457,3.85628530270651));
#95819=CARTESIAN_POINT('Origin',(-1.57426155444895E-13,2.970239242001,-3.53449908230274E-14));
#95820=CARTESIAN_POINT('',(6.72689107318561,2.78894740126561,3.31646445626045));
#95821=CARTESIAN_POINT('Ctrl Pts',(6.72689107500255,2.78894740038621,3.31646445271653));
#95822=CARTESIAN_POINT('Ctrl Pts',(6.69634256802001,2.79982120463123,3.37842696767838));
#95823=CARTESIAN_POINT('Ctrl Pts',(6.66497947801158,2.81065020634044,3.43988275429206));
#95824=CARTESIAN_POINT('Ctrl Pts',(6.63282692833449,2.82142857086638,3.50080089926231));
#95825=CARTESIAN_POINT('Ctrl Pts',(6.57631075775242,2.84037424996154,3.60787981825588));
#95826=CARTESIAN_POINT('Ctrl Pts',(6.51704567080299,2.85947647430086,3.71388197465343));
#95827=CARTESIAN_POINT('Ctrl Pts',(6.45509774747662,2.87870320435315,3.81860093040627));
#95828=CARTESIAN_POINT('',(6.9562314805007,2.87870320271433,2.80371959930828));
#95829=CARTESIAN_POINT('Origin',(-0.18055420657661,2.94640463077747,-0.0610512711219108));
#95830=CARTESIAN_POINT('Origin',(-0.158857905135916,3.08920872516404,-0.0999365369811978));
#95831=CARTESIAN_POINT('Ctrl Pts',(6.497285334,3.009344995,3.216797055));
#95832=CARTESIAN_POINT('Ctrl Pts',(6.673397112,2.943588707,2.861086559));
#95833=CARTESIAN_POINT('Ctrl Pts',(6.809624158,2.878703203,2.488276275));
#95834=CARTESIAN_POINT('Ctrl Pts',(6.608580148,3.009344995,3.546359884));
#95835=CARTESIAN_POINT('Ctrl Pts',(6.802734686,2.943588707,3.184556269));
#95836=CARTESIAN_POINT('Ctrl Pts',(6.956231483,2.878703203,2.803719592));
#95837=CARTESIAN_POINT('',(6.80962414281031,2.87870320347874,2.48827627106145));
#95838=CARTESIAN_POINT('',(6.88292781858177,2.87870320212873,2.64599793848983));
#95839=CARTESIAN_POINT('Origin',(-0.168743259941024,3.08923062687531,-0.098384840025989));
#95840=CARTESIAN_POINT('Ctrl Pts',(6.79716901704737,2.87421362534792,2.51516866831626));
#95841=CARTESIAN_POINT('Ctrl Pts',(6.80181937093871,2.87645841417397,2.5024555082831));
#95842=CARTESIAN_POINT('Ctrl Pts',(6.80646972483,2.878703203,2.48974234825));
#95843=CARTESIAN_POINT('Ctrl Pts',(6.94176727817,2.944013165,2.11986524042));
#95844=CARTESIAN_POINT('Ctrl Pts',(7.03618674890999,3.00933735,1.73750485288));
#95845=CARTESIAN_POINT('Ctrl Pts',(6.80032892689619,2.87421362534792,2.51371437879972));
#95846=CARTESIAN_POINT('Ctrl Pts',(6.80497654244815,2.87645841417397,2.50099532689983));
#95847=CARTESIAN_POINT('Ctrl Pts',(6.809624158,2.878703203,2.488276275));
#95848=CARTESIAN_POINT('Ctrl Pts',(6.944842042,2.944013165,2.118227749));
#95849=CARTESIAN_POINT('Ctrl Pts',(7.039163737,3.00933735,1.735705586));
#95850=CARTESIAN_POINT('Ctrl Pts',(7.11696595811632,2.87421362534792,2.36798809638245));
#95851=CARTESIAN_POINT('Ctrl Pts',(7.12133917986923,2.87645841417397,2.35467865321177));
#95852=CARTESIAN_POINT('Ctrl Pts',(7.12571240162204,2.878703203,2.34136921004108));
#95853=CARTESIAN_POINT('Ctrl Pts',(7.25294706315576,2.944013165,1.95414382044622));
#95854=CARTESIAN_POINT('Ctrl Pts',(7.33747119382016,3.00933735,1.55541103631185));
#95855=CARTESIAN_POINT('',(7.12506747388459,2.87870320365548,2.34166895685243));
#95856=CARTESIAN_POINT('',(7.28081451506283,2.96915797898314,1.79992777426841));
#95857=CARTESIAN_POINT('Origin',(-0.186479305376558,2.9464284651642,-0.0498551048602675));
#95858=CARTESIAN_POINT('',(7.03803875113726,3.00855922007997,1.74026168046718));
#95859=CARTESIAN_POINT('Ctrl Pts',(7.03803875201502,3.00855921921256,1.74026167631026));
#95860=CARTESIAN_POINT('Ctrl Pts',(7.07843255283472,3.0016637005282,1.7502299408843));
#95861=CARTESIAN_POINT('Ctrl Pts',(7.118883370277,2.99493785110666,1.76019052401283));
#95862=CARTESIAN_POINT('Ctrl Pts',(7.19979551660409,2.98181495661769,1.78007478494072));
#95863=CARTESIAN_POINT('Ctrl Pts',(7.24030324971683,2.97541039162867,1.79000986396595));
#95864=CARTESIAN_POINT('Ctrl Pts',(7.28081451460902,2.9691579789846,1.79992777604475));
#95865=CARTESIAN_POINT('Origin',(-0.190998271341551,2.94642869800802,-0.0578394435499486));
#95866=CARTESIAN_POINT('',(6.96734581257855,2.87870320492449,2.41497262381362));
#95867=CARTESIAN_POINT('Origin',(-1.09547787507935E-12,2.97023924200033,
-1.85181731060524E-13));
#95868=CARTESIAN_POINT('',(7.28256192199601,2.78894740128747,1.79284462519746));
#95869=CARTESIAN_POINT('Ctrl Pts',(7.28256192321671,2.78894740038391,1.79284462117268));
#95870=CARTESIAN_POINT('Ctrl Pts',(7.26604773257175,2.79982120463769,1.8599255130922));
#95871=CARTESIAN_POINT('Ctrl Pts',(7.24862907170715,2.81065020634741,1.92668663488117));
#95872=CARTESIAN_POINT('Ctrl Pts',(7.23032383120981,2.82142857087646,1.99309239523889));
#95873=CARTESIAN_POINT('Ctrl Pts',(7.19814777979972,2.84037424998939,2.10981717482112));
#95874=CARTESIAN_POINT('Ctrl Pts',(7.16305560768842,2.85947647430068,2.22608130136318));
#95875=CARTESIAN_POINT('Ctrl Pts',(7.12506747217466,2.87870320435307,2.34166895820505));
#95876=CARTESIAN_POINT('',(7.39631549110475,2.87870320271433,1.24278604964134));
#95877=CARTESIAN_POINT('Origin',(-0.189457228805128,2.94640462537924,-0.0208101341724251));
#95878=CARTESIAN_POINT('Origin',(-0.17662714545213,3.08920871805869,-0.0634502948560189));
#95879=CARTESIAN_POINT('Ctrl Pts',(7.036898692,3.009344995,1.744865839));
#95880=CARTESIAN_POINT('Ctrl Pts',(7.132425833,2.943588707,1.35961283));
#95881=CARTESIAN_POINT('Ctrl Pts',(7.185324776,2.878703203,0.966233856));
#95882=CARTESIAN_POINT('Ctrl Pts',(7.216437762,3.009344995,2.042798577));
#95883=CARTESIAN_POINT('Ctrl Pts',(7.328275993,2.943588707,1.647716243));
#95884=CARTESIAN_POINT('Ctrl Pts',(7.396315492,2.878703203,1.242786042));
#95885=CARTESIAN_POINT('',(7.18532476004359,2.8787032034815,0.96623385508769));
#95886=CARTESIAN_POINT('',(7.29082013319928,2.87870320212873,1.10450995428553));
#95887=CARTESIAN_POINT('Origin',(-0.185948094727437,3.08923058801028,-0.0598098675866138));
#95888=CARTESIAN_POINT('Ctrl Pts',(7.17894189898616,2.87421362534608,0.995175007239506));
#95889=CARTESIAN_POINT('Ctrl Pts',(7.18075057656315,2.87645841417304,0.981759385199748));
#95890=CARTESIAN_POINT('Ctrl Pts',(7.18255925414001,2.878703203,0.968343763159999));
#95891=CARTESIAN_POINT('Ctrl Pts',(7.23518098069,2.944013165,0.57802920212));
#95892=CARTESIAN_POINT('Ctrl Pts',(7.24519679643001,3.00933735,0.18431079146));
#95893=CARTESIAN_POINT('Ctrl Pts',(7.1817153026374,2.87421362534608,0.993075430992086));
#95894=CARTESIAN_POINT('Ctrl Pts',(7.18352003931876,2.87645841417304,0.979654643496043));
#95895=CARTESIAN_POINT('Ctrl Pts',(7.185324776,2.878703203,0.966233856));
#95896=CARTESIAN_POINT('Ctrl Pts',(7.237831846,2.944013165,0.575769010999999));
#95897=CARTESIAN_POINT('Ctrl Pts',(7.247717395,3.00933735,0.181913626));
#95898=CARTESIAN_POINT('Ctrl Pts',(7.45962269256269,2.87421362534609,0.782688546049605));
#95899=CARTESIAN_POINT('Ctrl Pts',(7.46103253396369,2.87645841417304,0.768750156842104));
#95900=CARTESIAN_POINT('Ctrl Pts',(7.4624423753646,2.878703203,0.754811767634591));
#95901=CARTESIAN_POINT('Ctrl Pts',(7.50346034873261,2.944013165,0.349287800947444));
#95902=CARTESIAN_POINT('Ctrl Pts',(7.50029259058361,3.00933735,-0.0582930225762464));
#95903=CARTESIAN_POINT('',(7.24759813578533,3.00855922012093,0.186605041169535));
#95904=CARTESIAN_POINT('Ctrl Pts',(7.24759813575441,3.00855921921561,0.186605036456814));
#95905=CARTESIAN_POINT('Ctrl Pts',(7.28919043403294,3.00166370056477,0.187656775431321));
#95906=CARTESIAN_POINT('Ctrl Pts',(7.33083676504322,2.9949378511043,0.188688755670289));
#95907=CARTESIAN_POINT('Ctrl Pts',(7.41413179084453,2.98181495154648,0.190714414764441));
#95908=CARTESIAN_POINT('Ctrl Pts',(7.45582826192075,2.97541038110894,0.191709252839048));
#95909=CARTESIAN_POINT('Ctrl Pts',(7.49752438372885,2.96915797897716,0.192686563589115));
#95910=CARTESIAN_POINT('Origin',(-0.198966747437768,2.94642872685435,-0.0154282146167841));
#95911=CARTESIAN_POINT('',(7.32360086760227,2.87870320492457,0.860738509892561));
#95912=CARTESIAN_POINT('Ctrl Pts',(7.247474489,3.009344995,0.191346636));
#95913=CARTESIAN_POINT('Ctrl Pts',(7.25795025,2.943588707,-0.205434883));
#95914=CARTESIAN_POINT('Ctrl Pts',(7.22504759300001,2.878703203,-0.600988585));
#95915=CARTESIAN_POINT('Ctrl Pts',(7.486862767,3.009344995,0.443718279));
#95916=CARTESIAN_POINT('Ctrl Pts',(7.511155258,2.943588707,0.033830836));
#95917=CARTESIAN_POINT('Ctrl Pts',(7.490556008,2.878703203,-0.376258802));
#95918=CARTESIAN_POINT('',(7.22504757715887,2.87870320349508,-0.600988582157999));
#95919=CARTESIAN_POINT('',(7.35780180085423,2.87870320212873,-0.488623688165908));
#95920=CARTESIAN_POINT('Origin',(-0.194458153582505,3.08923057649802,-0.0184381958679822));
#95921=CARTESIAN_POINT('Ctrl Pts',(7.22503543617682,2.87421362527074,-0.571351931454881));
#95922=CARTESIAN_POINT('Ctrl Pts',(7.22391786567334,2.87645841413537,-0.58484271615244));
#95923=CARTESIAN_POINT('Ctrl Pts',(7.22280029517,2.878703203,-0.59833350085));
#95924=CARTESIAN_POINT('Ctrl Pts',(7.19028566172,2.944013165,-0.99083484021));
#95925=CARTESIAN_POINT('Ctrl Pts',(7.11542949334,3.00933735,-1.37750143675));
#95926=CARTESIAN_POINT('Ctrl Pts',(7.22729265236689,2.87421362527074,-0.573998620574956));
#95927=CARTESIAN_POINT('Ctrl Pts',(7.22617012268338,2.87645841413537,-0.587493602787484));
#95928=CARTESIAN_POINT('Ctrl Pts',(7.22504759300001,2.878703203,-0.600988584999999));
#95929=CARTESIAN_POINT('Ctrl Pts',(7.192388677,2.944013165,-0.993612047));
#95930=CARTESIAN_POINT('Ctrl Pts',(7.117375842,3.00933735,-1.380384412));
#95931=CARTESIAN_POINT('Ctrl Pts',(7.45347576121302,2.87421362527074,-0.839208650499396));
#95932=CARTESIAN_POINT('Ctrl Pts',(7.4518562996145,2.87645841413536,-0.853124242393329));
#95933=CARTESIAN_POINT('Ctrl Pts',(7.45023683801584,2.878703203,-0.86703983428725));
#95934=CARTESIAN_POINT('Ctrl Pts',(7.40312016832172,2.944013165,-1.2719005283683));
#95935=CARTESIAN_POINT('Ctrl Pts',(7.31240864069362,3.00933735,-1.66927136382287));
#95936=CARTESIAN_POINT('',(7.44977737784609,2.87870320365574,-0.86649699318621));
#95937=CARTESIAN_POINT('',(7.36365834535818,2.96915797897503,-1.42356445975563));
#95938=CARTESIAN_POINT('Origin',(-0.190177538421263,2.9464284868015,0.0330533512148072));
#95939=CARTESIAN_POINT('',(7.11826788656465,3.00855922009091,-1.37577704263269));
#95940=CARTESIAN_POINT('Ctrl Pts',(7.11826788559849,3.00855921919469,-1.37577704683838));
#95941=CARTESIAN_POINT('Ctrl Pts',(7.15911387198548,3.00166370052759,-1.38369101187184));
#95942=CARTESIAN_POINT('Ctrl Pts',(7.20000837997906,2.99493785110683,-1.3916358889752));
#95943=CARTESIAN_POINT('Ctrl Pts',(7.28179147137155,2.98181495153996,-1.40756355721969));
#95944=CARTESIAN_POINT('Ctrl Pts',(7.32272696298951,2.97541038109973,-1.41555548667772));
#95945=CARTESIAN_POINT('Ctrl Pts',(7.36365834559492,2.96915797897421,-1.4235644585451));
#95946=CARTESIAN_POINT('Origin',(-0.197631358334211,2.94642873841696,0.0277044275786476));
#95947=CARTESIAN_POINT('',(7.33741248569151,2.87870320492457,-0.733742780585012));
#95948=CARTESIAN_POINT('Origin',(-1.99926880606327E-13,2.97023924200056,
6.41847686111419E-14));
#95949=CARTESIAN_POINT('',(7.36227011168011,2.78894740127468,-1.43072666945416));
#95950=CARTESIAN_POINT('Ctrl Pts',(7.36227011098476,2.78894740039408,-1.43072667338475));
#95951=CARTESIAN_POINT('Ctrl Pts',(7.37544877285625,2.79982120463674,-1.36291157598455));
#95952=CARTESIAN_POINT('Ctrl Pts',(7.38767229193052,2.81065020634305,-1.29500691682899));
#95953=CARTESIAN_POINT('Ctrl Pts',(7.39894196063855,2.82142857078376,-1.22705251018671));
#95954=CARTESIAN_POINT('Ctrl Pts',(7.41875122933032,2.84037424973322,-1.10760559749431));
#95955=CARTESIAN_POINT('Ctrl Pts',(7.43572047689678,2.85947647430088,-0.987352312321885));
#95956=CARTESIAN_POINT('Ctrl Pts',(7.44977737688105,2.87870320435315,-0.866496991366489));
#95957=CARTESIAN_POINT('',(7.23454645341812,2.87870320271433,-1.97771019567721));
#95958=CARTESIAN_POINT('Origin',(-0.180684634096219,2.94640460378407,0.0606642555156378));
#95959=CARTESIAN_POINT('Origin',(-0.186944872367999,3.08920871784849,0.016577968539003));
#95960=CARTESIAN_POINT('Ctrl Pts',(7.119166433,3.009344995,-1.371119723));
#95961=CARTESIAN_POINT('Ctrl Pts',(7.044100979,2.943588707,-1.76087669));
#95962=CARTESIAN_POINT('Ctrl Pts',(6.926935215,2.878703203,-2.140109468));
#95963=CARTESIAN_POINT('Ctrl Pts',(7.40721039,3.009344995,-1.176109793));
#95964=CARTESIAN_POINT('Ctrl Pts',(7.342821252,2.943588707,-1.581636462));
#95965=CARTESIAN_POINT('Ctrl Pts',(7.234546451,2.878703203,-1.977710203));
#95966=CARTESIAN_POINT('',(6.92693520013569,2.87870320350798,-2.1401094613818));
#95967=CARTESIAN_POINT('',(7.08074083449266,2.8787032021287,-2.05890983036663));
#95968=CARTESIAN_POINT('Origin',(-0.193875393915119,3.08923059316947,0.0237955986485733));
#95969=CARTESIAN_POINT('Ctrl Pts',(6.93329434686559,2.87421362526316,-2.11116308955185));
#95970=CARTESIAN_POINT('Ctrl Pts',(6.92930278461267,2.87645841413158,-2.12409822259592));
#95971=CARTESIAN_POINT('Ctrl Pts',(6.92531122236,2.878703203,-2.13703335564));
#95972=CARTESIAN_POINT('Ctrl Pts',(6.80918057741999,2.944013165,-2.51336854665));
#95973=CARTESIAN_POINT('Ctrl Pts',(6.65295261534001,3.00933735,-2.87490322868));
#95974=CARTESIAN_POINT('Ctrl Pts',(6.93492983066302,2.87421362526316,-2.11423313530778));
#95975=CARTESIAN_POINT('Ctrl Pts',(6.93093252283145,2.87645841413158,-2.12717130165389));
#95976=CARTESIAN_POINT('Ctrl Pts',(6.926935215,2.878703203,-2.140109468));
#95977=CARTESIAN_POINT('Ctrl Pts',(6.810637408,2.944013165,-2.51653291));
#95978=CARTESIAN_POINT('Ctrl Pts',(6.654233705,3.00933735,-2.878137209));
#95979=CARTESIAN_POINT('Ctrl Pts',(7.0988125865179,2.87421362526317,-2.42186538445608));
#95980=CARTESIAN_POINT('Ctrl Pts',(7.09423954612034,2.87645841413158,-2.4351075011659));
#95981=CARTESIAN_POINT('Ctrl Pts',(7.08966650572267,2.878703203,-2.44834961787577));
#95982=CARTESIAN_POINT('Ctrl Pts',(6.95661831629257,2.944013165,-2.83361620186825));
#95983=CARTESIAN_POINT('Ctrl Pts',(6.782604590907,3.00933735,-3.20219643111895));
#95984=CARTESIAN_POINT('',(7.08933448239759,2.87870320364628,-2.44772069546989));
#95985=CARTESIAN_POINT('',(6.88547582676876,2.96915797900449,-2.97325118946044));
#95986=CARTESIAN_POINT('Origin',(-0.178625803362676,2.94642847631061,0.0731631295020271));
#95987=CARTESIAN_POINT('',(6.65609534290466,3.00855922007134,-2.87382932098887));
#95988=CARTESIAN_POINT('Ctrl Pts',(6.65609534087897,3.00855921916919,-2.87382932529785));
#95989=CARTESIAN_POINT('Ctrl Pts',(6.69428510228388,3.00166370051113,-2.89033894558407));
#95990=CARTESIAN_POINT('Ctrl Pts',(6.73251560584482,2.99493785107109,-2.90688918613176));
#95991=CARTESIAN_POINT('Ctrl Pts',(6.80896267611153,2.98181495152546,-2.94002542125667));
#95992=CARTESIAN_POINT('Ctrl Pts',(6.84722308990285,2.97541038112037,-2.95663042439218));
#95993=CARTESIAN_POINT('Ctrl Pts',(6.88547582727347,2.96915797900365,-2.97325118829854));
#95994=CARTESIAN_POINT('Origin',(-0.187055439915118,2.94642874800422,0.0695416967131169));
#95995=CARTESIAN_POINT('',(7.00813485072502,2.87870320492457,-2.29391507461971));
#95996=CARTESIAN_POINT('Origin',(5.37330596683816E-13,2.97023924200022,
-1.88434337577981E-13));
#95997=CARTESIAN_POINT('',(6.88258038540432,2.78894740126419,-2.97994752197196));
#95998=CARTESIAN_POINT('Ctrl Pts',(6.88258038384381,2.78894740041576,-2.97994752537121));
#95999=CARTESIAN_POINT('Ctrl Pts',(6.91002917723491,2.79982120464213,-2.91655093023161));
#96000=CARTESIAN_POINT('Ctrl Pts',(6.93656441164617,2.81065020634171,-2.8528615397131));
#96001=CARTESIAN_POINT('Ctrl Pts',(6.96217879061306,2.82142857083718,-2.78891851496595));
#96002=CARTESIAN_POINT('Ctrl Pts',(7.00720248597009,2.84037424988088,-2.67652261174883));
#96003=CARTESIAN_POINT('Ctrl Pts',(7.04962590309075,2.85947647430089,-2.56272866850826));
#96004=CARTESIAN_POINT('Ctrl Pts',(7.0893344817164,2.87870320435315,-2.44772069575774));
#96005=CARTESIAN_POINT('',(6.64025754595189,2.87870320271433,-3.4866860663639));
#96006=CARTESIAN_POINT('Origin',(-0.163419285037631,2.94640460318537,0.0980878044349803));
#96007=CARTESIAN_POINT('Origin',(-0.179010304998681,3.08920866068137,0.0563779571333461));
#96008=CARTESIAN_POINT('Ctrl Pts',(6.657974068,3.009344995,-2.869474048));
#96009=CARTESIAN_POINT('Ctrl Pts',(6.500877375,2.943588707,-3.23398186));
#96010=CARTESIAN_POINT('Ctrl Pts',(6.304927044,2.878703203,-3.57916121));
#96011=CARTESIAN_POINT('Ctrl Pts',(6.981205087,3.009344995,-2.740944277));
#96012=CARTESIAN_POINT('Ctrl Pts',(6.831145085,2.943588707,-3.123148198));
#96013=CARTESIAN_POINT('Ctrl Pts',(6.640257542,2.878703203,-3.486686073));
#96014=CARTESIAN_POINT('',(6.30492703114527,2.87870320349741,-3.57916120050747));
#96015=CARTESIAN_POINT('',(6.47259229556122,2.87870320212873,-3.53292363680765));
#96016=CARTESIAN_POINT('Origin',(-0.184227357519026,3.08923058099144,0.0649167702287662));
#96017=CARTESIAN_POINT('Ctrl Pts',(6.31736011824193,2.87421362536507,-3.55225860772393));
#96018=CARTESIAN_POINT('Ctrl Pts',(6.31068120543596,2.87645841418253,-3.56403325637194));
#96019=CARTESIAN_POINT('Ctrl Pts',(6.30400229263001,2.878703203,-3.57580790502));
#96020=CARTESIAN_POINT('Ctrl Pts',(6.1096857769,2.944013165,-3.91837993219));
#96021=CARTESIAN_POINT('Ctrl Pts',(5.87939106768,3.00933735,-4.23787774194));
#96022=CARTESIAN_POINT('Ctrl Pts',(6.31829739625371,2.87421362536507,-3.55560845819292));
#96023=CARTESIAN_POINT('Ctrl Pts',(6.31161222012684,2.87645841418253,-3.56738483409645));
#96024=CARTESIAN_POINT('Ctrl Pts',(6.304927044,2.878703203,-3.57916121));
#96025=CARTESIAN_POINT('Ctrl Pts',(6.110428303,2.944013165,-3.92178349));
#96026=CARTESIAN_POINT('Ctrl Pts',(5.879946996,3.00933735,-4.24131151));
#96027=CARTESIAN_POINT('Ctrl Pts',(6.41221682473787,2.87421362536508,-3.89127838495085));
#96028=CARTESIAN_POINT('Ctrl Pts',(6.40490403598191,2.87645841418253,-3.90322783954293));
#96029=CARTESIAN_POINT('Ctrl Pts',(6.39759124722613,2.878703203,-3.91517729413501));
#96030=CARTESIAN_POINT('Ctrl Pts',(6.18483272311035,2.944013165,-4.26283513137004));
#96031=CARTESIAN_POINT('Ctrl Pts',(5.93565348803107,3.00933735,-4.58539035288206));
#96032=CARTESIAN_POINT('',(6.39740218615542,2.87870320364628,-3.91449170041254));
#96033=CARTESIAN_POINT('',(6.08533611102078,2.96915797896983,-4.38391199843602));
#96034=CARTESIAN_POINT('Origin',(-0.158721867595243,2.94642846403946,0.109851978861961));
#96035=CARTESIAN_POINT('',(5.88269117803425,3.00855922074793,-4.23750453416616));
#96036=CARTESIAN_POINT('Ctrl Pts',(5.88269117488078,3.00855921928978,-4.23750453812649));
#96037=CARTESIAN_POINT('Ctrl Pts',(5.91643900043501,3.00166370065495,-4.2618378423234));
#96038=CARTESIAN_POINT('Ctrl Pts',(5.95021788409653,2.99493785110104,-4.2862195759487));
#96039=CARTESIAN_POINT('Ctrl Pts',(6.01775435318733,2.98181495154895,-4.33501496450934));
#96040=CARTESIAN_POINT('Ctrl Pts',(6.05155067503837,2.97541038110632,-4.35945660995131));
#96041=CARTESIAN_POINT('Ctrl Pts',(6.08533611175129,2.96915797896901,-4.38391199742659));
#96042=CARTESIAN_POINT('Origin',(-0.167732537891877,2.94642877561658,0.10812709419047));
#96043=CARTESIAN_POINT('',(6.35116461858435,2.87870320492457,-3.74682644868655));
#96044=CARTESIAN_POINT('Origin',(5.49039980146659E-13,2.97023924200022,
-4.05925293378573E-13));
#96045=CARTESIAN_POINT('',(6.0810688504322,2.78894740130207,-4.38982934047308));
#96046=CARTESIAN_POINT('Ctrl Pts',(6.08106884814993,2.78894740043738,-4.38982934357451));
#96047=CARTESIAN_POINT('Ctrl Pts',(6.12150429781557,2.79982120466031,-4.33381560487324));
#96048=CARTESIAN_POINT('Ctrl Pts',(6.16111048936085,2.81065020635268,-4.27731952794972));
#96049=CARTESIAN_POINT('Ctrl Pts',(6.19987187858141,2.8214285708836,-4.22037778961493));
#96050=CARTESIAN_POINT('Ctrl Pts',(6.26800474235051,2.84037425000917,-4.1202884024779));
#96051=CARTESIAN_POINT('Ctrl Pts',(6.33389865714034,2.85947647430085,-4.01827467958502));
#96052=CARTESIAN_POINT('Ctrl Pts',(6.39740218542473,2.87870320435315,-3.91449170053438));
#96053=CARTESIAN_POINT('',(5.73547757627587,2.87870320271434,-4.83262837136912));
#96054=CARTESIAN_POINT('Origin',(-0.138512604171944,2.94640460791274,0.130924848640008));
#96055=CARTESIAN_POINT('Origin',(-0.162705727006365,3.08920870108171,0.0935419213033933));
#96056=CARTESIAN_POINT('Ctrl Pts',(5.885462235,3.009344995,-4.233654956));
#96057=CARTESIAN_POINT('Ctrl Pts',(5.653679971,2.943588707,-4.555869632));
#96058=CARTESIAN_POINT('Ctrl Pts',(5.388107493,2.878703203,-4.850855352));
#96059=CARTESIAN_POINT('Ctrl Pts',(6.228766394,3.009344995,-4.177615254));
#96060=CARTESIAN_POINT('Ctrl Pts',(6.000052166,2.943588707,-4.518624994));
#96061=CARTESIAN_POINT('Ctrl Pts',(5.735477571,2.878703203,-4.832628377));
#96062=CARTESIAN_POINT('',(5.38810748217986,2.87870320347741,-4.85085534039044));
#96063=CARTESIAN_POINT('',(5.56179253551006,2.87870320212873,-4.84174186046794));
#96064=CARTESIAN_POINT('Origin',(-0.165965131742308,3.08923060397874,0.103002543905989));
#96065=CARTESIAN_POINT('Ctrl Pts',(5.40603315323794,2.8742136253572,-4.8272544609917));
#96066=CARTESIAN_POINT('Ctrl Pts',(5.39697918824401,2.8764584141786,-4.83731805610593));
#96067=CARTESIAN_POINT('Ctrl Pts',(5.38792522325,2.878703203,-4.84738165122));
#96068=CARTESIAN_POINT('Ctrl Pts',(5.12450885906,2.944013165,-5.14017222832));
#96069=CARTESIAN_POINT('Ctrl Pts',(4.83091572861,3.00933735,-5.40269380138));
#96070=CARTESIAN_POINT('Ctrl Pts',(5.40622839938105,2.8742136253572,-4.83072748088307));
#96071=CARTESIAN_POINT('Ctrl Pts',(5.39716794619055,2.8764584141786,-4.84079141644154));
#96072=CARTESIAN_POINT('Ctrl Pts',(5.388107493,2.878703203,-4.850855352));
#96073=CARTESIAN_POINT('Ctrl Pts',(5.124502361,2.944013165,-5.143655834));
#96074=CARTESIAN_POINT('Ctrl Pts',(4.830720501,3.00933735,-5.406166798));
#96075=CARTESIAN_POINT('Ctrl Pts',(5.42579293193448,2.87421362535721,-5.17873953196392));
#96076=CARTESIAN_POINT('Ctrl Pts',(5.41608233257222,2.8764584141786,-5.18883758156331));
#96077=CARTESIAN_POINT('Ctrl Pts',(5.40637173320981,2.878703203,-5.19893563116283));
#96078=CARTESIAN_POINT('Ctrl Pts',(5.12385122646595,2.944013165,-5.4927286282283));
#96079=CARTESIAN_POINT('Ctrl Pts',(4.81115782554438,3.00933735,-5.75417651719669));
#96080=CARTESIAN_POINT('',(5.40633447466497,2.87870320364628,-5.1982254236792));
#96081=CARTESIAN_POINT('',(5.00065284185713,2.96915797901993,-5.58958595540412));
#96082=CARTESIAN_POINT('Origin',(-0.131396090152665,2.94642848507124,0.141404195005143));
#96083=CARTESIAN_POINT('',(4.83421891288071,3.00855922009732,-5.40303874586003));
#96084=CARTESIAN_POINT('Ctrl Pts',(4.8342189094851,3.00855921915052,-5.40303874868488));
#96085=CARTESIAN_POINT('Ctrl Pts',(4.86194678848687,3.00166370047611,-5.43405793901585));
#96086=CARTESIAN_POINT('Ctrl Pts',(4.88969458781813,2.99493785108942,-5.46513110214075));
#96087=CARTESIAN_POINT('Ctrl Pts',(4.94516250405332,2.98181495662009,-5.5273040023307));
#96088=CARTESIAN_POINT('Ctrl Pts',(4.97291443011225,2.9754103916399,-5.55843939755067));
#96089=CARTESIAN_POINT('Ctrl Pts',(5.00065284321323,2.96915797902156,-5.58958595417019));
#96090=CARTESIAN_POINT('Origin',(-0.140567026918474,2.94642871097474,0.141656766218079));
#96091=CARTESIAN_POINT('',(5.39722098865919,2.87870320492457,-5.02454038223562));
#96092=CARTESIAN_POINT('Origin',(-3.33934269125535E-13,2.97023924200011,
4.43221848112074E-13));
#96093=CARTESIAN_POINT('',(4.99521329427853,2.78894740128863,-5.59444761728865));
#96094=CARTESIAN_POINT('Ctrl Pts',(4.99521329131002,2.78894740039219,-5.59444762017117));
#96095=CARTESIAN_POINT('Ctrl Pts',(5.04674468096817,2.79982120464079,-5.54843587769016));
#96096=CARTESIAN_POINT('Ctrl Pts',(5.09756988842109,2.81065020634783,-5.50177480787537));
#96097=CARTESIAN_POINT('Ctrl Pts',(5.14766584842138,2.82142857087551,-5.45449688854607));
#96098=CARTESIAN_POINT('Ctrl Pts',(5.23572206310051,2.84037424998681,-5.37139408782123));
#96099=CARTESIAN_POINT('Ctrl Pts',(5.32200534986858,2.85947647430085,-5.28593063299671));
#96100=CARTESIAN_POINT('Ctrl Pts',(5.40633447392617,2.87870320435315,-5.19822542366011));
#96101=CARTESIAN_POINT('',(4.56251304938851,2.87870320271433,-5.95260234463916));
#96102=CARTESIAN_POINT('Origin',(-0.107129220033608,2.94640461850637,0.157639935299));
#96103=CARTESIAN_POINT('Origin',(-0.138792725147368,3.08920868830491,0.126331557648913));
#96104=CARTESIAN_POINT('Ctrl Pts',(4.837752729,3.009344995,-5.399874863));
#96105=CARTESIAN_POINT('Ctrl Pts',(4.542122774,2.943588707,-5.664730004));
#96106=CARTESIAN_POINT('Ctrl Pts',(4.219346023,2.878703203,-5.895728889));
#96107=CARTESIAN_POINT('Ctrl Pts',(5.185077507,3.009344995,-5.418945585));
#96108=CARTESIAN_POINT('Ctrl Pts',(4.888403477,2.943588707,-5.702815909));
#96109=CARTESIAN_POINT('Ctrl Pts',(4.562513043,2.878703203,-5.952602349));
#96110=CARTESIAN_POINT('',(4.21934601544481,2.87870320349341,-5.89572887525597));
#96111=CARTESIAN_POINT('',(4.39092953729476,2.87870320212873,-5.92416561581676));
#96112=CARTESIAN_POINT('Origin',(-0.139942396941389,3.08923058268686,0.136271951790612));
#96113=CARTESIAN_POINT('Ctrl Pts',(4.24192608543235,2.87421362529374,-5.87653326056445));
#96114=CARTESIAN_POINT('Ctrl Pts',(4.2309204215162,2.87645841414687,-5.88441523968227));
#96115=CARTESIAN_POINT('Ctrl Pts',(4.2199147576,2.878703203,-5.8922972188));
#96116=CARTESIAN_POINT('Ctrl Pts',(3.89971560339,2.944013165,-6.12161578297));
#96117=CARTESIAN_POINT('Ctrl Pts',(3.55655213791,3.00933735,-6.31488590327));
#96118=CARTESIAN_POINT('Ctrl Pts',(4.2413701702162,2.87421362529374,-5.87996705533547));
#96119=CARTESIAN_POINT('Ctrl Pts',(4.23035809660807,2.87645841414687,-5.88784797216778));
#96120=CARTESIAN_POINT('Ctrl Pts',(4.219346023,2.878703203,-5.895728889));
#96121=CARTESIAN_POINT('Ctrl Pts',(3.898960385,2.944013165,-6.125016547));
#96122=CARTESIAN_POINT('Ctrl Pts',(3.555614883,3.00933735,-6.31823573500001));
#96123=CARTESIAN_POINT('Ctrl Pts',(4.1856649912382,2.87421362529374,-6.22404857479066));
#96124=CARTESIAN_POINT('Ctrl Pts',(4.17401063797508,2.87645841414687,-6.23182304588729));
#96125=CARTESIAN_POINT('Ctrl Pts',(4.16235628471193,2.878703203,-6.2395975169839));
#96126=CARTESIAN_POINT('Ctrl Pts',(3.82328414093741,2.944013165,-6.46578823919032));
#96127=CARTESIAN_POINT('Ctrl Pts',(3.46169776941115,3.00933735,-6.65390378403689));
#96128=CARTESIAN_POINT('',(4.16247256938398,2.87870320365574,-6.2388959060018));
#96129=CARTESIAN_POINT('',(3.6821446043708,2.96915797895617,-6.53389708421412));
#96130=CARTESIAN_POINT('Origin',(-0.0979263322834728,2.94642846350857,0.16634440571257));
#96131=CARTESIAN_POINT('',(3.55970394316431,3.00855922005574,-6.31593287016463));
#96132=CARTESIAN_POINT('Ctrl Pts',(3.55970393905358,3.00855921908199,-6.31593287229377));
#96133=CARTESIAN_POINT('Ctrl Pts',(3.58011534677,3.00166370041136,-6.35218752553784));
#96134=CARTESIAN_POINT('Ctrl Pts',(3.60053460648103,2.99493785103531,-6.38849917192794));
#96135=CARTESIAN_POINT('Ctrl Pts',(3.64134039390338,2.98181495147748,-6.46114249472729));
#96136=CARTESIAN_POINT('Ctrl Pts',(3.66175032427549,2.97541038106563,-6.49751583846894));
#96137=CARTESIAN_POINT('Ctrl Pts',(3.68214460546018,2.96915797895535,-6.53389708360331));
#96138=CARTESIAN_POINT('Origin',(-0.10682872237075,2.94642875408866,0.168562830046286));
#96139=CARTESIAN_POINT('',(4.19090930285252,2.87870320492457,-6.06731239219452));
#96140=CARTESIAN_POINT('Origin',(-7.63278329429795E-14,2.97023924199967,
1.39211558947139E-13));
#96141=CARTESIAN_POINT('',(3.67578711653968,2.78894740127316,-6.5374757419103));
#96142=CARTESIAN_POINT('Ctrl Pts',(3.67578711304387,2.78894740038181,-6.53747574404648));
#96143=CARTESIAN_POINT('Ctrl Pts',(3.73600489189342,2.79982120463246,-6.50361745621602));
#96144=CARTESIAN_POINT('Ctrl Pts',(3.79567258490586,2.81065020634291,-6.46897321361542));
#96145=CARTESIAN_POINT('Ctrl Pts',(3.85476068413728,2.82142857084263,-6.43356977651691));
#96146=CARTESIAN_POINT('Ctrl Pts',(3.95862283830183,2.84037424989596,-6.3713393564955));
#96147=CARTESIAN_POINT('Ctrl Pts',(4.06126098658263,2.85947647430088,-6.30642234553358));
#96148=CARTESIAN_POINT('Ctrl Pts',(4.16247257015051,2.87870320435315,-6.23889590408228));
#96149=CARTESIAN_POINT('',(3.17621048313442,2.87870320271434,-6.79423924909755));
#96150=CARTESIAN_POINT('Origin',(-0.0707368491739291,2.94640461726311,0.176984353505357));
#96151=CARTESIAN_POINT('Origin',(-0.108390380535675,3.08920870998506,0.153214497359081));
#96152=CARTESIAN_POINT('Ctrl Pts',(3.563835282,3.009344995,-6.313602623));
#96153=CARTESIAN_POINT('Ctrl Pts',(3.218180965,2.943588707,-6.508713897));
#96154=CARTESIAN_POINT('Ctrl Pts',(2.853292624,2.878703203,-6.664924696));
#96155=CARTESIAN_POINT('Ctrl Pts',(3.898940158,3.009344995,-6.406892042));
#96156=CARTESIAN_POINT('Ctrl Pts',(3.548178474,2.943588707,-6.620349489));
#96157=CARTESIAN_POINT('Ctrl Pts',(3.176210476,2.878703203,-6.794239252));
#96158=CARTESIAN_POINT('',(2.85329261859847,2.87870320347467,-6.66492468100942));
#96159=CARTESIAN_POINT('',(3.01475155487866,2.87870320212873,-6.72958197181443));
#96160=CARTESIAN_POINT('Origin',(-0.107376206837705,3.08923053390024,0.163169527380586));
#96161=CARTESIAN_POINT('Ctrl Pts',(2.87947126959757,2.87421362535152,-6.65103189674269));
#96162=CARTESIAN_POINT('Ctrl Pts',(2.86702851957879,2.87645841417576,-6.65636370710636));
#96163=CARTESIAN_POINT('Ctrl Pts',(2.85458576956,2.878703203,-6.66169551747));
#96164=CARTESIAN_POINT('Ctrl Pts',(2.49257597954,2.944013165,-6.81681938857999));
#96165=CARTESIAN_POINT('Ctrl Pts',(2.11588812321,3.00933735,-6.93180095857));
#96166=CARTESIAN_POINT('Ctrl Pts',(2.87819018699049,2.87421362535152,-6.65426590596142));
#96167=CARTESIAN_POINT('Ctrl Pts',(2.86574140549524,2.87645841417576,-6.6595953009807));
#96168=CARTESIAN_POINT('Ctrl Pts',(2.853292624,2.878703203,-6.664924696));
#96169=CARTESIAN_POINT('Ctrl Pts',(2.491107354,2.944013165,-6.819978295));
#96170=CARTESIAN_POINT('Ctrl Pts',(2.114252666,3.00933735,-6.934870991));
#96171=CARTESIAN_POINT('Ctrl Pts',(2.74982000782131,2.87421362535152,-6.97832802384403));
#96172=CARTESIAN_POINT('Ctrl Pts',(2.73676684554007,2.87645841417576,-6.98341539060992));
#96173=CARTESIAN_POINT('Ctrl Pts',(2.72371368325884,2.878703203,-6.98850275737577));
#96174=CARTESIAN_POINT('Ctrl Pts',(2.3439445382234,2.944013165,-7.1365147781814));
#96175=CARTESIAN_POINT('Ctrl Pts',(1.9503725743425,3.00933735,-7.24250190481638));
#96176=CARTESIAN_POINT('',(2.72397807488941,2.87870320365573,-6.98784254743535));
#96177=CARTESIAN_POINT('',(2.19146337730603,2.96915797899442,-7.17269044818231));
#96178=CARTESIAN_POINT('Origin',(-0.0598777743908424,2.94642848835606,0.183506743041469));
#96179=CARTESIAN_POINT('',(2.1187411738591,3.00855922009277,-6.93350099308368));
#96180=CARTESIAN_POINT('Ctrl Pts',(2.11874116901794,3.00855921917228,-6.93350099440111));
#96181=CARTESIAN_POINT('Ctrl Pts',(2.13088169066033,3.00166370050573,-6.97329588324973));
#96182=CARTESIAN_POINT('Ctrl Pts',(2.1430176289345,2.99493785108816,-7.01314812101293));
#96183=CARTESIAN_POINT('Ctrl Pts',(2.16725323268625,2.98181495153355,-7.09286512136001));
#96184=CARTESIAN_POINT('Ctrl Pts',(2.17936679654682,2.97541038110711,-7.13277560835332));
#96185=CARTESIAN_POINT('Ctrl Pts',(2.19146337849108,2.9691579789936,-7.17269044782304));
#96186=CARTESIAN_POINT('Origin',(-0.0680950929918261,2.94642876632057,0.18758694096996));
#96187=CARTESIAN_POINT('',(2.78863535708515,2.87870320492457,-6.82638361797163));
#96188=CARTESIAN_POINT('Origin',(4.96889855650107E-13,2.97023924199989,
-1.6831154525665E-12));
#96189=CARTESIAN_POINT('',(2.18448521775634,2.78894740125864,-7.17481876632809));
#96190=CARTESIAN_POINT('Ctrl Pts',(2.18448521418145,2.78894740041504,-7.17481876732048));
#96191=CARTESIAN_POINT('Ctrl Pts',(2.2505736657173,2.7998212046406,-7.15469710993879));
#96192=CARTESIAN_POINT('Ctrl Pts',(2.31629384925405,2.81065020634061,-7.13368962084375));
#96193=CARTESIAN_POINT('Ctrl Pts',(2.38161119431194,2.82142857088646,-7.11181609123042));
#96194=CARTESIAN_POINT('Ctrl Pts',(2.49642281089811,2.84037425001707,-7.07336787714953));
#96195=CARTESIAN_POINT('Ctrl Pts',(2.61061657427729,2.85947647430087,-7.03203275809879));
#96196=CARTESIAN_POINT('Ctrl Pts',(2.7239780760405,2.87870320435315,-6.98784254573441));
#96197=CARTESIAN_POINT('',(1.64139184460424,2.87870320271434,-7.31818507670773));
#96198=CARTESIAN_POINT('Origin',(-0.0310366276400662,2.94640459783726,0.188052768844947));
#96199=CARTESIAN_POINT('Origin',(-0.0729196359696244,3.08920870897142,0.172932995349643));
#96200=CARTESIAN_POINT('Ctrl Pts',(2.123276858,3.009344995,-6.932113342));
#96201=CARTESIAN_POINT('Ctrl Pts',(1.743760591,2.943588707,-7.048357562));
#96202=CARTESIAN_POINT('Ctrl Pts',(1.353822432,2.878703203,-7.122476032));
#96203=CARTESIAN_POINT('Ctrl Pts',(2.430492701,3.009344995,-7.095259349));
#96204=CARTESIAN_POINT('Ctrl Pts',(2.042044589,2.943588707,-7.228322886));
#96205=CARTESIAN_POINT('Ctrl Pts',(1.641391837,2.878703203,-7.318185078));
#96206=CARTESIAN_POINT('',(1.35382243033776,2.87870320349874,-7.12247601598353));
#96207=CARTESIAN_POINT('',(1.49760713973443,2.87870320212873,-7.2203305539143));
#96208=CARTESIAN_POINT('Origin',(-0.0697891869278638,3.08923055983671,0.182437410565597));
#96209=CARTESIAN_POINT('Ctrl Pts',(1.38237557612321,2.87421362542889,-7.11453567379985));
#96210=CARTESIAN_POINT('Ctrl Pts',(1.36907754929659,2.87645841421444,-7.11706800587004));
#96211=CARTESIAN_POINT('Ctrl Pts',(1.35577952247,2.878703203,-7.11960033794));
#96212=CARTESIAN_POINT('Ctrl Pts',(0.968886273399999,2.944013165,-7.19327609412999));
#96213=CARTESIAN_POINT('Ctrl Pts',(0.57628753136,3.00933735,-7.22459270619));
#96214=CARTESIAN_POINT('Ctrl Pts',(1.38042922812558,2.87421362542889,-7.11741867878759));
#96215=CARTESIAN_POINT('Ctrl Pts',(1.36712583006278,2.87645841421444,-7.11994735539385));
#96216=CARTESIAN_POINT('Ctrl Pts',(1.353822432,2.878703203,-7.12247603199999));
#96217=CARTESIAN_POINT('Ctrl Pts',(0.966772911999999,2.944013165,-7.196045436));
#96218=CARTESIAN_POINT('Ctrl Pts',(0.574030344,3.00933735,-7.227239388));
#96219=CARTESIAN_POINT('Ctrl Pts',(1.18539649581848,2.87421362542889,-7.40630861043445));
#96220=CARTESIAN_POINT('Ctrl Pts',(1.17155487598325,2.87645841421444,-7.40847099329545));
#96221=CARTESIAN_POINT('Ctrl Pts',(1.15771325614798,2.878703203,-7.41063337615648));
#96222=CARTESIAN_POINT('Ctrl Pts',(0.755004693420168,2.944013165,-7.47354581735855));
#96223=CARTESIAN_POINT('Ctrl Pts',(0.347850124077315,3.00933735,-7.4924486854024));
#96224=CARTESIAN_POINT('',(1.1581133920687,2.87870320365573,-7.41004543795076));
#96225=CARTESIAN_POINT('',(0.598311757139471,2.96915797894638,-7.47609677821526));
#96226=CARTESIAN_POINT('Origin',(-0.0190293521124379,2.94642847731649,0.192088534679514));
#96227=CARTESIAN_POINT('',(0.578708421721079,3.00855922013913,-7.22686631479652));
#96228=CARTESIAN_POINT('Ctrl Pts',(0.578708417200027,3.0085592193911,-7.22686631503209));
#96229=CARTESIAN_POINT('Ctrl Pts',(0.582010375225272,3.0016637006968,-7.26834067461964));
#96230=CARTESIAN_POINT('Ctrl Pts',(0.585295528807544,2.99493785114926,-7.30987005778705));
#96231=CARTESIAN_POINT('Ctrl Pts',(0.591827716122462,2.98181495671242,-7.39293322468151));
#96232=CARTESIAN_POINT('Ctrl Pts',(0.59507849357419,2.97541039178165,-7.43451464653668));
#96233=CARTESIAN_POINT('Ctrl Pts',(0.598311758986549,2.96915797894511,-7.47609677807154));
#96234=CARTESIAN_POINT('Origin',(-0.0261773973727075,2.94642875462569,0.197839503071079));
#96235=CARTESIAN_POINT('',(1.25596792029945,2.87870320492457,-7.26626073296047));
#96236=CARTESIAN_POINT('Origin',(1.52183021501391E-13,2.97023924199944,
-1.55431223447522E-12));
#96237=CARTESIAN_POINT('',(0.591039218776085,2.78894740131378,-7.47667523986356));
#96238=CARTESIAN_POINT('Ctrl Pts',(0.591039214962054,2.78894740045328,-7.47667524011751));
#96239=CARTESIAN_POINT('Ctrl Pts',(0.659908116785784,2.79982120466984,-7.47123107939932));
#96240=CARTESIAN_POINT('Ctrl Pts',(0.728607788144424,2.81065020635683,-7.46484263043069));
#96241=CARTESIAN_POINT('Ctrl Pts',(0.797100212037056,2.82142857084698,-7.45752179009138));
#96242=CARTESIAN_POINT('Ctrl Pts',(0.917492825796067,2.84037424990796,-7.44465357697846));
#96243=CARTESIAN_POINT('Ctrl Pts',(1.03790263162977,2.85947647430088,-7.42883313360311));
#96244=CARTESIAN_POINT('Ctrl Pts',(1.15811339355452,2.87870320435315,-7.41004543653923));
#96245=CARTESIAN_POINT('',(0.0298235486719519,2.87870320271433,-7.49994070433841));
#96246=CARTESIAN_POINT('Origin',(0.0101147754068714,2.94640462088094,0.190328198298189));
#96247=CARTESIAN_POINT('Origin',(-0.0340393366165772,3.08920866174723,0.184565482605681));
#96248=CARTESIAN_POINT('Ctrl Pts',(0.583436368,3.009344995,-7.226486145));
#96249=CARTESIAN_POINT('Ctrl Pts',(0.18780391,2.943588707,-7.258427861));
#96250=CARTESIAN_POINT('Ctrl Pts',(-0.208950992,2.878703203,-7.246988304));
#96251=CARTESIAN_POINT('Ctrl Pts',(0.848398107,3.009344995,-7.45186021400001));
#96252=CARTESIAN_POINT('Ctrl Pts',(0.440426968,2.943588707,-7.498307938));
#96253=CARTESIAN_POINT('Ctrl Pts',(0.029823541,2.878703203,-7.499940704));
#96254=CARTESIAN_POINT('',(-0.208950990233284,2.87870320350635,-7.24698828830006));
#96255=CARTESIAN_POINT('',(-0.0895637201545536,2.87870320212873,-7.37346450406493));
#96256=CARTESIAN_POINT('Origin',(-0.0289389099765305,3.08923058488446,0.193174565987628));
#96257=CARTESIAN_POINT('Ctrl Pts',(-0.179358461221556,2.8742136252575,-7.24537166885229));
#96258=CARTESIAN_POINT('Ctrl Pts',(-0.192889964610784,2.87645841412874,
-7.24498611376108));
#96259=CARTESIAN_POINT('Ctrl Pts',(-0.206421468,2.878703203,-7.24460055867));
#96260=CARTESIAN_POINT('Ctrl Pts',(-0.60010747717,2.944013165,-7.23338320603999));
#96261=CARTESIAN_POINT('Ctrl Pts',(-0.990259625069999,3.00933735,-7.1795705277));
#96262=CARTESIAN_POINT('Ctrl Pts',(-0.181879065534904,2.8742136252575,-7.24776886349914));
#96263=CARTESIAN_POINT('Ctrl Pts',(-0.195415028767454,2.87645841412874,
-7.24737858374956));
#96264=CARTESIAN_POINT('Ctrl Pts',(-0.208950992,2.878703203,-7.246988304));
#96265=CARTESIAN_POINT('Ctrl Pts',(-0.602766756,2.944013165,-7.235633492));
#96266=CARTESIAN_POINT('Ctrl Pts',(-0.993032999,3.00933735,-7.181670103));
#96267=CARTESIAN_POINT('Ctrl Pts',(-0.434454836637015,2.87421362525749,
-7.48797843674292));
#96268=CARTESIAN_POINT('Ctrl Pts',(-0.448437696021408,2.87645841412875,
-7.48711472518749));
#96269=CARTESIAN_POINT('Ctrl Pts',(-0.462420555405793,2.878703203,-7.48625101363205));
#96270=CARTESIAN_POINT('Ctrl Pts',(-0.869238330894868,2.944013165,-7.46112216094301));
#96271=CARTESIAN_POINT('Ctrl Pts',(-1.27093741073838,3.00933735,-7.39205689301606));
#96272=CARTESIAN_POINT('',(-0.461903382889853,2.87870320364628,-7.48576283800869));
#96273=CARTESIAN_POINT('',(-1.02281625401732,2.96915797896033,-7.42992913193523));
#96274=CARTESIAN_POINT('Origin',(0.0227088631124259,2.9464284729253,0.191688079987331));
#96275=CARTESIAN_POINT('',(-0.988384093003342,3.00855922008486,-7.18231140161262));
#96276=CARTESIAN_POINT('Ctrl Pts',(-0.988384096897368,3.00855921917128,
-7.18231140092207));
#96277=CARTESIAN_POINT('Ctrl Pts',(-0.994075098219697,3.00166370049321,
-7.22352593649195));
#96278=CARTESIAN_POINT('Ctrl Pts',(-0.999794339433125,2.9949378510805,-7.26479059594575));
#96279=CARTESIAN_POINT('Ctrl Pts',(-1.01127100116623,2.98181495151466,-7.34731605168395));
#96280=CARTESIAN_POINT('Ctrl Pts',(-1.01703500703518,2.97541038107445,-7.38862418208822));
#96281=CARTESIAN_POINT('Ctrl Pts',(-1.02281625280334,2.96915797895953,-7.42992913210503));
#96282=CARTESIAN_POINT('Origin',(0.0169642529079538,2.94642871660925,0.198841623721504));
#96283=CARTESIAN_POINT('',(-0.33542718003798,2.87870320492457,-7.36637557104469));
#96284=CARTESIAN_POINT('Origin',(-6.66513285535464E-14,2.97023924199933,
-8.90346824045096E-13));
#96285=CARTESIAN_POINT('',(-1.03004311690319,2.78894740130355,-7.42893068869816));
#96286=CARTESIAN_POINT('Ctrl Pts',(-1.0300431208892,2.78894740042007,-7.42893068822525));
#96287=CARTESIAN_POINT('Ctrl Pts',(-0.961614001997674,2.79982120465479,
-7.43841858722712));
#96288=CARTESIAN_POINT('Ctrl Pts',(-0.893147163133885,2.8106502063526,-7.44694789537783));
#96289=CARTESIAN_POINT('Ctrl Pts',(-0.824682289782256,2.82142857084429,
-7.45452205871353));
#96290=CARTESIAN_POINT('Ctrl Pts',(-0.704338102554433,2.84037424990055,
-7.46783554994457));
#96291=CARTESIAN_POINT('Ctrl Pts',(-0.583342483860824,2.85947647430086,
-7.47826952876738));
#96292=CARTESIAN_POINT('Ctrl Pts',(-0.461903383331452,2.87870320435315,
-7.48576283741235));
#96293=CARTESIAN_POINT('',(-1.58313926454892,2.87870320271433,-7.33100743903185));
#96294=CARTESIAN_POINT('Origin',(0.050793168375533,2.94640459030149,0.183703662817273));
#96295=CARTESIAN_POINT('Origin',(0.00643263499772659,3.0892086783798,0.187568015178932));
#96296=CARTESIAN_POINT('Ctrl Pts',(-0.983684957,3.009344995,-7.182956488));
#96297=CARTESIAN_POINT('Ctrl Pts',(-1.376934274,2.943588707,-7.12910214));
#96298=CARTESIAN_POINT('Ctrl Pts',(-1.7619541,2.878703203,-7.032639458));
#96299=CARTESIAN_POINT('Ctrl Pts',(-0.77336664,3.009344995,-7.460020378));
#96300=CARTESIAN_POINT('Ctrl Pts',(-1.181784528,2.943588707,-7.417680444));
#96301=CARTESIAN_POINT('Ctrl Pts',(-1.583139272,2.878703203,-7.331007437));
#96302=CARTESIAN_POINT('',(-1.76195409466987,2.87870320350153,-7.03263944295868));
#96303=CARTESIAN_POINT('',(-1.67254668079349,2.87870320212873,-7.18182344871253));
#96304=CARTESIAN_POINT('Origin',(0.0132645304981956,3.08923054631695,0.19487939873126));
#96305=CARTESIAN_POINT('Ctrl Pts',(-1.73270589824458,2.87421362540002,-7.03742213803915));
#96306=CARTESIAN_POINT('Ctrl Pts',(-1.74583815922732,2.87645841420001,-7.0341367238745));
#96307=CARTESIAN_POINT('Ctrl Pts',(-1.75897042021,2.878703203,-7.03085130971));
#96308=CARTESIAN_POINT('Ctrl Pts',(-2.14104086967,2.944013165,-6.93526535782));
#96309=CARTESIAN_POINT('Ctrl Pts',(-2.51050334239,3.00933735,-6.79883961102));
#96310=CARTESIAN_POINT('Ctrl Pts',(-1.73568289820881,2.87421362540002,-7.0392214321956));
#96311=CARTESIAN_POINT('Ctrl Pts',(-1.74881849910441,2.87645841420001,-7.03593044509774));
#96312=CARTESIAN_POINT('Ctrl Pts',(-1.7619541,2.878703203,-7.032639458));
#96313=CARTESIAN_POINT('Ctrl Pts',(-2.144121721,2.944013165,-6.936891367));
#96314=CARTESIAN_POINT('Ctrl Pts',(-2.513663223,3.00933735,-6.80029390600001));
#96315=CARTESIAN_POINT('Ctrl Pts',(-2.03399154486928,2.87421362540002,-7.21951871510421));
#96316=CARTESIAN_POINT('Ctrl Pts',(-2.04746181990317,2.87645841420001,-7.21566929529133));
#96317=CARTESIAN_POINT('Ctrl Pts',(-2.06093209493699,2.878703203,-7.21181987547844));
#96318=CARTESIAN_POINT('Ctrl Pts',(-2.45283673674315,2.944013165,-7.0998247239959));
#96319=CARTESIAN_POINT('Ctrl Pts',(-2.83029732434841,3.00933735,-6.94602073587786));
#96320=CARTESIAN_POINT('',(-2.06032207028557,2.87870320364628,-7.21145428992307));
#96321=CARTESIAN_POINT('',(-2.59611851412711,2.96915797894434,-7.03634625720979));
#96322=CARTESIAN_POINT('Origin',(0.0633852977853117,2.94642849123412,0.18232499930925));
#96323=CARTESIAN_POINT('',(-2.50926086557918,3.00855922011313,-6.80191958859531));
#96324=CARTESIAN_POINT('Ctrl Pts',(-2.50926086955055,3.00855921921572,-6.80191958696962));
#96325=CARTESIAN_POINT('Ctrl Pts',(-2.52367872523229,3.00166370051747,-6.84094715263986));
#96326=CARTESIAN_POINT('Ctrl Pts',(-2.53813493563224,2.99493785112607,-6.88001759932214));
#96327=CARTESIAN_POINT('Ctrl Pts',(-2.56708381281762,2.9818149515234,-6.95814651287553));
#96328=CARTESIAN_POINT('Ctrl Pts',(-2.58159308632967,2.97541038107013,-6.99724979130255));
#96329=CARTESIAN_POINT('Ctrl Pts',(-2.59611851297962,2.96915797894355,-7.03634625763599));
#96330=CARTESIAN_POINT('Origin',(0.0593126565460807,2.94642874914839,0.190545812164119));
#96331=CARTESIAN_POINT('',(-1.91113807793474,2.87870320492457,-7.12204687560344));
#96332=CARTESIAN_POINT('Origin',(4.10912623372006E-13,2.97023924199956,
1.22167900795667E-12));
#96333=CARTESIAN_POINT('',(-2.60296178177553,2.78894740129189,-7.03381759525304));
#96334=CARTESIAN_POINT('Ctrl Pts',(-2.60296178585068,2.78894740038344,-7.03381759402443));
#96335=CARTESIAN_POINT('Ctrl Pts',(-2.53817211941089,2.79982120463919,-7.05779390899228));
#96336=CARTESIAN_POINT('Ctrl Pts',(-2.47313954621206,2.81065020634898,-7.0808421530776));
#96337=CARTESIAN_POINT('Ctrl Pts',(-2.40790356477809,2.82142857087124,-7.10295716073517));
#96338=CARTESIAN_POINT('Ctrl Pts',(-2.29323496508005,2.84037424997502,-7.14182983350586));
#96339=CARTESIAN_POINT('Ctrl Pts',(-2.17731115325935,2.85947647430088,-7.17803035289085));
#96340=CARTESIAN_POINT('Ctrl Pts',(-2.06032207062276,2.87870320435315,-7.21145428926619));
#96341=CARTESIAN_POINT('',(-3.12207624415868,2.87870320271433,-6.8192844145898));
#96342=CARTESIAN_POINT('Origin',(0.0890965170584079,2.94640463018758,0.168489748353048));
#96343=CARTESIAN_POINT('Origin',(0.0466038476664976,3.08920870044056,0.181800031890108));
#96344=CARTESIAN_POINT('Ctrl Pts',(-2.504810268,3.009344995,-6.803559768));
#96345=CARTESIAN_POINT('Ctrl Pts',(-2.877288541,2.943588707,-6.666427527));
#96346=CARTESIAN_POINT('Ctrl Pts',(-3.232570193,2.878703203,-6.48945220700001));
#96347=CARTESIAN_POINT('Ctrl Pts',(-2.358969622,3.009344995,-7.11935828));
#96348=CARTESIAN_POINT('Ctrl Pts',(-2.748737092,2.943588707,-6.990210457));
#96349=CARTESIAN_POINT('Ctrl Pts',(-3.122076251,2.878703203,-6.819284411));
#96350=CARTESIAN_POINT('',(-3.23257018454474,2.878703203489,-6.48945219339775));
#96351=CARTESIAN_POINT('',(-3.17732321717587,2.87870320212873,-6.65436831130342));
#96352=CARTESIAN_POINT('Origin',(0.0548477622940036,3.08923055998583,0.187471849778713));
#96353=CARTESIAN_POINT('Ctrl Pts',(-3.20503393312873,2.87421362546291,-6.50041056930446));
#96354=CARTESIAN_POINT('Ctrl Pts',(-3.2171529020443,2.87645841423145,-6.49437891844234));
#96355=CARTESIAN_POINT('Ctrl Pts',(-3.22927187096,2.878703203,-6.48834726758));
#96356=CARTESIAN_POINT('Ctrl Pts',(-3.58186157136,2.944013165,-6.31286220897));
#96357=CARTESIAN_POINT('Ctrl Pts',(-3.91335871321,3.00933735,-6.10020250954));
#96358=CARTESIAN_POINT('Ctrl Pts',(-3.20832812754588,2.87421362546291,-6.50152782997139));
#96359=CARTESIAN_POINT('Ctrl Pts',(-3.22044916027291,2.87645841423145,-6.49549001848572));
#96360=CARTESIAN_POINT('Ctrl Pts',(-3.232570193,2.878703203,-6.489452207));
#96361=CARTESIAN_POINT('Ctrl Pts',(-3.585219938,2.944013165,-6.313787911));
#96362=CARTESIAN_POINT('Ctrl Pts',(-3.916757348,3.00933735,-6.100943523));
#96363=CARTESIAN_POINT('Ctrl Pts',(-3.53842107018125,2.8742136254629,-6.61348232156619));
#96364=CARTESIAN_POINT('Ctrl Pts',(-3.55074890599567,2.87645841423145,-6.6068271881958));
#96365=CARTESIAN_POINT('Ctrl Pts',(-3.56307674181016,2.878703203,-6.60017205482557));
#96366=CARTESIAN_POINT('Ctrl Pts',(-3.92174322298085,2.944013165,-6.40654737458526));
#96367=CARTESIAN_POINT('Ctrl Pts',(-4.25731568083914,3.00933735,-6.17519636984648));
#96368=CARTESIAN_POINT('',(-3.5624023890913,2.87870320364628,-6.59994615371924));
#96369=CARTESIAN_POINT('',(-4.04802915911568,2.96915797899007,-6.31375165200505));
#96370=CARTESIAN_POINT('Origin',(0.101097921122694,2.94642846559488,0.164436471006835));
#96371=CARTESIAN_POINT('',(-3.91280738900488,3.00855922007331,-6.10347757543102));
#96372=CARTESIAN_POINT('Ctrl Pts',(-3.91280739300367,3.00855921915691,-6.10347757268442));
#96373=CARTESIAN_POINT('Ctrl Pts',(-3.93527794006492,3.00166370051067,-6.13849328278278));
#96374=CARTESIAN_POINT('Ctrl Pts',(-3.95779516364713,2.99493785106891,-6.17354262673068));
#96375=CARTESIAN_POINT('Ctrl Pts',(-4.00286262173748,2.98181495656297,-6.2436217500575));
#96376=CARTESIAN_POINT('Ctrl Pts',(-4.02543870508714,2.97541039152408,-6.27869171914441));
#96377=CARTESIAN_POINT('Ctrl Pts',(-4.04802915756938,2.9691579789933,-6.31375165296533));
#96378=CARTESIAN_POINT('Origin',(0.0988877438210358,2.94642876685686,0.173340571503577));
#96379=CARTESIAN_POINT('',(-3.39748628437228,2.87870320492457,-6.54469918351707));
#96380=CARTESIAN_POINT('Origin',(-8.00141203294302E-14,2.970239242,-1.25767452008319E-13));
#96381=CARTESIAN_POINT('',(-4.05416884645276,2.78894740128127,-6.30981100856562));
#96382=CARTESIAN_POINT('Ctrl Pts',(-4.05416885007228,2.78894740038107,-6.30981100648208));
#96383=CARTESIAN_POINT('Ctrl Pts',(-3.9960481289277,2.79982120463475,-6.34715463168828));
#96384=CARTESIAN_POINT('Ctrl Pts',(-3.93749067225874,2.81065020634522,-6.38364410164896));
#96385=CARTESIAN_POINT('Ctrl Pts',(-3.87853394488013,2.82142857080492,-6.41926588030258));
#96386=CARTESIAN_POINT('Ctrl Pts',(-3.77490270966395,2.84037424979169,-6.48188009002636));
#96387=CARTESIAN_POINT('Ctrl Pts',(-3.66947117360319,2.85947647430088,-6.54215445487876));
#96388=CARTESIAN_POINT('Ctrl Pts',(-3.56240238930578,2.87870320435315,-6.59994615301406));
#96389=CARTESIAN_POINT('',(-4.51502840909075,2.87870320271434,-5.98869922997258));
#96390=CARTESIAN_POINT('Origin',(0.123233813057545,2.94640457796691,0.145397461512357));
#96391=CARTESIAN_POINT('Origin',(0.0845957594067731,3.08920869620704,0.1675309736737));
#96392=CARTESIAN_POINT('Ctrl Pts',(-3.908813434,3.009344995,-6.106036156));
#96393=CARTESIAN_POINT('Ctrl Pts',(-4.243103994,2.943588707,-5.892038171));
#96394=CARTESIAN_POINT('Ctrl Pts',(-4.55203489600001,2.878703203,-5.642825383));
#96395=CARTESIAN_POINT('Ctrl Pts',(-3.834269807,3.009344995,-6.445802902));
#96396=CARTESIAN_POINT('Ctrl Pts',(-4.187161766,2.943588707,-6.235885999));
#96397=CARTESIAN_POINT('Ctrl Pts',(-4.515028415,2.878703203,-5.98869922500001));
#96398=CARTESIAN_POINT('',(-4.55203488468433,2.87870320348395,-5.64282537181518));
#96399=CARTESIAN_POINT('',(-4.53353165128382,2.87870320212873,-5.81576230728662));
#96400=CARTESIAN_POINT('Origin',(0.0938663525190531,3.08923056724444,0.171298211864391));
#96401=CARTESIAN_POINT('Ctrl Pts',(-4.52749814143103,2.87421362522429,-5.65944702767209));
#96402=CARTESIAN_POINT('Ctrl Pts',(-4.53803714951051,2.87645841411214,-5.65095117293104));
#96403=CARTESIAN_POINT('Ctrl Pts',(-4.54857615759,2.878703203,-5.64245531819));
#96404=CARTESIAN_POINT('Ctrl Pts',(-4.85519840653001,2.944013165,-5.39527663992));
#96405=CARTESIAN_POINT('Ctrl Pts',(-5.13322978040999,3.00933735,-5.11632672005));
#96406=CARTESIAN_POINT('Ctrl Pts',(-4.53095549742285,2.87421362522429,-5.65983001298227));
#96407=CARTESIAN_POINT('Ctrl Pts',(-4.54149519671143,2.87645841411214,-5.65132769799116));
#96408=CARTESIAN_POINT('Ctrl Pts',(-4.552034896,2.878703203,-5.642825383));
#96409=CARTESIAN_POINT('Ctrl Pts',(-4.858677255,2.944013165,-5.39545875));
#96410=CARTESIAN_POINT('Ctrl Pts',(-5.136708253,3.00933735,-5.116319803));
#96411=CARTESIAN_POINT('Ctrl Pts',(-4.8773979560828,2.87421362522429,-5.69820684568864));
#96412=CARTESIAN_POINT('Ctrl Pts',(-4.88800691759854,2.87645841411214,-5.68905718488251));
#96413=CARTESIAN_POINT('Ctrl Pts',(-4.89861587911412,2.878703203,-5.67990752407634));
#96414=CARTESIAN_POINT('Ctrl Pts',(-5.2072733556336,2.944013165,-5.41370699056625));
#96415=CARTESIAN_POINT('Ctrl Pts',(-5.48526668878461,3.00933735,-5.11562668380304));
#96416=CARTESIAN_POINT('',(-4.89790873033672,2.87870320364628,-5.67983187031397));
#96417=CARTESIAN_POINT('',(-5.3106584585667,2.96915797898921,-5.29593303699521));
#96418=CARTESIAN_POINT('Origin',(0.134083018405543,2.94642846777895,0.138858694066594));
#96419=CARTESIAN_POINT('',(-5.13339538778399,3.00855922013794,-5.11964373418263));
#96420=CARTESIAN_POINT('Ctrl Pts',(-5.13339539093452,3.00855921933033,-5.11964373083109));
#96421=CARTESIAN_POINT('Ctrl Pts',(-5.16286793163712,3.00166370066671,-5.14901028953704));
#96422=CARTESIAN_POINT('Ctrl Pts',(-5.19239328821135,2.99493785113664,-5.17839966207307));
#96423=CARTESIAN_POINT('Ctrl Pts',(-5.2514720567996,2.9818149515647,-5.23715222562473));
#96424=CARTESIAN_POINT('Ctrl Pts',(-5.28105935724491,2.97541038112397,-5.26654911421085));
#96425=CARTESIAN_POINT('Ctrl Pts',(-5.31065845768295,2.96915797898838,-5.29593303788525));
#96426=CARTESIAN_POINT('Origin',(0.13383883078985,2.94642871007955,0.148029969099221));
#96427=CARTESIAN_POINT('',(-4.72497180730675,2.87870320492457,-5.66132863117273));
#96428=CARTESIAN_POINT('Origin',(-1.34007388519208E-13,2.97023924199967,
-2.68882138776405E-14));
#96429=CARTESIAN_POINT('',(-5.3158074822294,2.78894740125489,-5.29076467184895));
#96430=CARTESIAN_POINT('Ctrl Pts',(-5.315807485249,2.78894740036227,-5.29076466905292));
#96431=CARTESIAN_POINT('Ctrl Pts',(-5.26707336984818,2.79982120462009,-5.33972945793396));
#96432=CARTESIAN_POINT('Ctrl Pts',(-5.21772911131924,2.81065020633716,-5.38795394643646));
#96433=CARTESIAN_POINT('Ctrl Pts',(-5.16780838853748,2.82142857088395,-5.43541686148898));
#96434=CARTESIAN_POINT('Ctrl Pts',(-5.08006019774948,2.84037425001013,-5.51884483931084));
#96435=CARTESIAN_POINT('Ctrl Pts',(-4.9900507994269,2.85947647430088,-5.60037468588646));
#96436=CARTESIAN_POINT('Ctrl Pts',(-4.89790873034857,2.87870320435315,-5.67983186957425));
#96437=CARTESIAN_POINT('',(-5.69686286429477,2.87870320271433,-4.87808912509862));
#96438=CARTESIAN_POINT('Origin',(0.151608896763318,2.94640461492605,0.11550657870882));
#96439=CARTESIAN_POINT('Origin',(0.118632343573259,3.08920869426911,0.145428778230158));
#96440=CARTESIAN_POINT('Ctrl Pts',(-5.130044829,3.009344995,-5.123001079));
#96441=CARTESIAN_POINT('Ctrl Pts',(-5.41051662,2.943588707,-4.84214366));
#96442=CARTESIAN_POINT('Ctrl Pts',(-5.658651506,2.878703203,-4.532346316));
#96443=CARTESIAN_POINT('Ctrl Pts',(-5.130283797,3.009344995,-5.470848943));
#96444=CARTESIAN_POINT('Ctrl Pts',(-5.429799409,2.943588707,-5.189978441));
#96445=CARTESIAN_POINT('Ctrl Pts',(-5.696862869,2.878703203,-4.878089119));
#96446=CARTESIAN_POINT('',(-5.65865149264154,2.87870320350527,-4.53234630772529));
#96447=CARTESIAN_POINT('',(-5.67775718408892,2.87870320212873,-4.70521772161613));
#96448=CARTESIAN_POINT('Origin',(0.128495716125747,3.08923059219918,0.147114741849005));
#96449=CARTESIAN_POINT('Ctrl Pts',(-5.63826157005105,2.87421362540045,-4.55385403199581));
#96450=CARTESIAN_POINT('Ctrl Pts',(-5.64672782401047,2.87645841420022,-4.54329123080791));
#96451=CARTESIAN_POINT('Ctrl Pts',(-5.65519407797001,2.878703203,-4.53272842962));
#96452=CARTESIAN_POINT('Ctrl Pts',(-5.90151155978999,2.944013165,-4.22541393114));
#96453=CARTESIAN_POINT('Ctrl Pts',(-6.11307672812999,3.00933735,-3.89321717911));
#96454=CARTESIAN_POINT('Ctrl Pts',(-5.64172042550909,2.87421362540045,-4.55348483398032));
#96455=CARTESIAN_POINT('Ctrl Pts',(-5.65018596575451,2.87645841420022,-4.54291557499019));
#96456=CARTESIAN_POINT('Ctrl Pts',(-5.658651506,2.878703203,-4.532346316));
#96457=CARTESIAN_POINT('Ctrl Pts',(-5.904948223,2.944013165,-4.224843934));
#96458=CARTESIAN_POINT('Ctrl Pts',(-6.116472389,3.00933735,-3.892462655));
#96459=CARTESIAN_POINT('Ctrl Pts',(-5.98831313732949,2.87421362540045,-4.51648954957949));
#96460=CARTESIAN_POINT('Ctrl Pts',(-5.99670716025377,2.87645841420022,-4.50527319005817));
#96461=CARTESIAN_POINT('Ctrl Pts',(-6.00510118317804,2.878703203,-4.49405683053692));
#96462=CARTESIAN_POINT('Ctrl Pts',(-6.24931717279247,2.944013165,-4.16772768358729));
#96463=CARTESIAN_POINT('Ctrl Pts',(-6.45673272182828,3.00933735,-3.81685598088723));
#96464=CARTESIAN_POINT('',(-6.00439430383142,2.87870320364628,-4.49413496160079));
#96465=CARTESIAN_POINT('',(-6.32496727096953,2.96915797898409,-4.03048247922108));
#96466=CARTESIAN_POINT('Origin',(0.160798983820203,2.9464284946586,0.106788522587034));
#96467=CARTESIAN_POINT('',(-6.11395152353537,3.00855922012302,-3.89642104262903));
#96468=CARTESIAN_POINT('Ctrl Pts',(-6.11395152592256,3.00855921933987,-3.89642103863776));
#96469=CARTESIAN_POINT('Ctrl Pts',(-6.1490479569122,3.00166370068712,-3.91876529849187));
#96470=CARTESIAN_POINT('Ctrl Pts',(-6.18420087352747,2.9949378511202,-3.94112048507939));
#96471=CARTESIAN_POINT('Ctrl Pts',(-6.25452847761625,2.98181495155569,-3.9857992574478));
#96472=CARTESIAN_POINT('Ctrl Pts',(-6.2897435054049,2.97541038112154,-4.00814846808177));
#96473=CARTESIAN_POINT('Ctrl Pts',(-6.32496727029219,2.96915797898326,-4.03048248028911));
#96474=CARTESIAN_POINT('Origin',(0.162531914113991,2.94642873184857,0.115797771320268));
#96475=CARTESIAN_POINT('',(-5.8315229001711,2.87870320492457,-4.51324064446962));
#96476=CARTESIAN_POINT('Origin',(-5.30391702779909E-13,2.97023924200056,
-3.57786716920216E-13));
#96477=CARTESIAN_POINT('',(-6.32888486767176,2.78894740126767,-4.02432805943019));
#96478=CARTESIAN_POINT('Ctrl Pts',(-6.32888487003153,2.78894740037185,-4.02432805603769));
#96479=CARTESIAN_POINT('Ctrl Pts',(-6.29181611341766,2.79982120462702,-4.0826244695479));
#96480=CARTESIAN_POINT('Ctrl Pts',(-6.25399233574641,2.81065020634096,-4.14032905322512));
#96481=CARTESIAN_POINT('Ctrl Pts',(-6.21544185532186,2.82142857091001,-4.1974137915234));
#96482=CARTESIAN_POINT('Ctrl Pts',(-6.14767971779934,2.84037425008215,-4.29775453722658));
#96483=CARTESIAN_POINT('Ctrl Pts',(-6.07730119665039,2.85947647430087,-4.39672762094291));
#96484=CARTESIAN_POINT('Ctrl Pts',(-6.00439430370237,2.87870320435315,-4.49413496087379));
#96485=CARTESIAN_POINT('',(-6.61231834271407,2.87870320271434,-3.53938499496242));
#96486=CARTESIAN_POINT('Origin',(0.17289507850705,2.94640462869725,0.0802147943709647));
#96487=CARTESIAN_POINT('Origin',(0.147121763688923,3.08920867755301,0.116526339563724));
#96488=CARTESIAN_POINT('Ctrl Pts',(-6.111401029,3.009344995,-3.900420166));
#96489=CARTESIAN_POINT('Ctrl Pts',(-6.32493950200001,2.943588707,-3.565835892));
#96490=CARTESIAN_POINT('Ctrl Pts',(-6.500675861,2.878703203,-3.209939773));
#96491=CARTESIAN_POINT('Ctrl Pts',(-6.186411418,3.009344995,-4.240084169));
#96492=CARTESIAN_POINT('Ctrl Pts',(-6.418545666,2.943588707,-3.90139326));
#96493=CARTESIAN_POINT('Ctrl Pts',(-6.612318346,2.878703203,-3.539384988));
#96494=CARTESIAN_POINT('',(-6.50067584637424,2.87870320347896,-3.20993976725337));
#96495=CARTESIAN_POINT('',(-6.55649710105352,2.87870320212873,-3.37466238525318));
#96496=CARTESIAN_POINT('Origin',(0.157116902266113,3.08923058993594,0.116052513379786));
#96497=CARTESIAN_POINT('Ctrl Pts',(-6.48538615356865,2.87421362538382,-3.23532788416263));
#96498=CARTESIAN_POINT('Ctrl Pts',(-6.49138378120933,2.87645841419191,-3.22319204100631));
#96499=CARTESIAN_POINT('Ctrl Pts',(-6.49738140885,2.878703203,-3.21105619785));
#96500=CARTESIAN_POINT('Ctrl Pts',(-6.6718765916,2.944013165,-2.85797556393));
#96501=CARTESIAN_POINT('Ctrl Pts',(-6.80708300218001,3.00933735,-2.48806512947));
#96502=CARTESIAN_POINT('Ctrl Pts',(-6.48868477624723,2.87421362538382,-3.23422376610241));
#96503=CARTESIAN_POINT('Ctrl Pts',(-6.4946803186236,2.87645841419191,-3.22208176955118));
#96504=CARTESIAN_POINT('Ctrl Pts',(-6.500675861,2.878703203,-3.209939773));
#96505=CARTESIAN_POINT('Ctrl Pts',(-6.675110375,2.944013165,-2.856680112));
#96506=CARTESIAN_POINT('Ctrl Pts',(-6.81023707400001,3.00933735,-2.486598279));
#96507=CARTESIAN_POINT('Ctrl Pts',(-6.81922145039138,2.87421362538383,-3.12358622217583));
#96508=CARTESIAN_POINT('Ctrl Pts',(-6.82500804000554,2.87645841419191,-3.11082762807001));
#96509=CARTESIAN_POINT('Ctrl Pts',(-6.83079462961964,2.878703203,-3.09806903396426));
#96510=CARTESIAN_POINT('Ctrl Pts',(-6.99914986484071,2.944013165,-2.72687006272138));
#96511=CARTESIAN_POINT('Ctrl Pts',(-7.12628910873856,3.00933735,-2.33961333314017));
#96512=CARTESIAN_POINT('',(-6.83012107408333,2.87870320365575,-3.09829729477548));
#96513=CARTESIAN_POINT('',(-7.04352764417412,2.96915797898783,-2.57657103907726));
#96514=CARTESIAN_POINT('Origin',(0.179995934489753,2.94642846182119,0.0697248336034639));
#96515=CARTESIAN_POINT('',(-6.80862608162002,3.00855922010261,-2.49100603347877));
#96516=CARTESIAN_POINT('Ctrl Pts',(-6.80862608309258,3.00855921927237,-2.49100602904712));
#96517=CARTESIAN_POINT('Ctrl Pts',(-6.84770533459544,3.00166370059657,-2.50528319728228));
#96518=CARTESIAN_POINT('Ctrl Pts',(-6.88684209941936,2.9949378511142,-2.51955889384014));
#96519=CARTESIAN_POINT('Ctrl Pts',(-6.96513006845013,2.98181495661202,-2.54807473423967));
#96520=CARTESIAN_POINT('Ctrl Pts',(-7.00432617261881,2.9754103915964,-2.56233122981507));
#96521=CARTESIAN_POINT('Ctrl Pts',(-7.04352764352837,2.96915797898996,-2.5765710407879));
#96522=CARTESIAN_POINT('Origin',(0.183624911733789,2.94642874499142,0.0781508407550076));
#96523=CARTESIAN_POINT('',(-6.66539846337813,2.87870320492457,-3.15411854132372));
#96524=CARTESIAN_POINT('Origin',(1.43765208071578E-12,2.97023924199989,
4.51895465491958E-13));
#96525=CARTESIAN_POINT('',(-7.04603063111017,2.78894740127532,-2.56971833965995));
#96526=CARTESIAN_POINT('Ctrl Pts',(-7.04603063233613,2.78894740042345,-2.56971833609903));
#96527=CARTESIAN_POINT('Ctrl Pts',(-7.0223605283775,2.79982120464813,-2.63462049873483));
#96528=CARTESIAN_POINT('Ctrl Pts',(-6.99782582942406,2.81065020634501,-2.69910697557628));
#96529=CARTESIAN_POINT('Ctrl Pts',(-6.97244816946066,2.82142857080435,-2.76314431783759));
#96530=CARTESIAN_POINT('Ctrl Pts',(-6.92784056788042,2.84037424979018,-2.87570600714895));
#96531=CARTESIAN_POINT('Ctrl Pts',(-6.88038374407231,2.85947647430088,-2.98749445823547));
#96532=CARTESIAN_POINT('Ctrl Pts',(-6.8301210723039,2.87870320435315,-3.09829729585191));
#96533=CARTESIAN_POINT('',(-7.218589164312,2.87870320271433,-2.0351831555464));
#96534=CARTESIAN_POINT('Origin',(0.186096308467992,2.94640459671127,0.0411719524297086));
#96535=CARTESIAN_POINT('Origin',(0.168731710661435,3.08920867055077,0.082175130974515));
#96536=CARTESIAN_POINT('Ctrl Pts',(-6.806994909,3.009344995,-2.49545994));
#96537=CARTESIAN_POINT('Ctrl Pts',(-6.943615243,2.943588707,-2.122793602));
#96538=CARTESIAN_POINT('Ctrl Pts',(-7.038735838,2.878703203,-1.737440013));
#96539=CARTESIAN_POINT('Ctrl Pts',(-6.953269318,3.009344995,-2.811057772));
#96540=CARTESIAN_POINT('Ctrl Pts',(-7.107167862,2.943588707,-2.430383266));
#96541=CARTESIAN_POINT('Ctrl Pts',(-7.218589166,2.878703203,-2.035183148));
#96542=CARTESIAN_POINT('',(-7.03873582220987,2.87870320348778,-1.73744001092693));
#96543=CARTESIAN_POINT('',(-7.1286625006325,2.87870320212873,-1.88631158566797));
#96544=CARTESIAN_POINT('Origin',(0.178391247383135,3.08923062900728,0.0795637173879721));
#96545=CARTESIAN_POINT('Ctrl Pts',(-7.02926128892046,2.87421362546414,-1.76552139884387));
#96546=CARTESIAN_POINT('Ctrl Pts',(-7.03250984778527,2.87645841423207,-1.75237997256197));
#96547=CARTESIAN_POINT('Ctrl Pts',(-7.03575840664999,2.878703203,-1.73923854628));
#96548=CARTESIAN_POINT('Ctrl Pts',(-7.13027209054,2.944013165,-1.35690143583));
#96549=CARTESIAN_POINT('Ctrl Pts',(-7.18279764011,3.00933735,-0.966573919529999));
#96550=CARTESIAN_POINT('Ctrl Pts',(-7.03224543889102,2.87421362546414,-1.76373398808801));
#96551=CARTESIAN_POINT('Ctrl Pts',(-7.03549063844558,2.87645841423207,-1.750587000544));
#96552=CARTESIAN_POINT('Ctrl Pts',(-7.038735838,2.878703203,-1.737440013));
#96553=CARTESIAN_POINT('Ctrl Pts',(-7.133151786,2.944013165,-1.354941103));
#96554=CARTESIAN_POINT('Ctrl Pts',(-7.185562642,3.00933735,-0.964463331));
#96555=CARTESIAN_POINT('Ctrl Pts',(-7.33127054800838,2.87421362546415,-1.58462747481222));
#96556=CARTESIAN_POINT('Ctrl Pts',(-7.33417912971884,2.87645841423207,-1.57092322405938));
#96557=CARTESIAN_POINT('Ctrl Pts',(-7.33708771142929,2.878703203,-1.55721897330654));
#96558=CARTESIAN_POINT('Ctrl Pts',(-7.42171008824157,2.944013165,-1.1585070282478));
#96559=CARTESIAN_POINT('Ctrl Pts',(-7.46262813804142,3.00933735,-0.752972966339245));
#96560=CARTESIAN_POINT('',(-7.33647897257464,2.87870320365574,-1.55758669204523));
#96561=CARTESIAN_POINT('',(-7.43274049270505,2.96915797897333,-1.00218200151024));
#96562=CARTESIAN_POINT('Origin',(0.190776647659696,2.94642846480955,0.0294009218485594));
#96563=CARTESIAN_POINT('',(-7.18493685125043,3.00855922004598,-0.969114350955477));
#96564=CARTESIAN_POINT('Ctrl Pts',(-7.18493685170426,3.00855921907439,-0.969114346370303));
#96565=CARTESIAN_POINT('Ctrl Pts',(-7.22617162141738,3.00166370041615,-0.97465683841719));
#96566=CARTESIAN_POINT('Ctrl Pts',(-7.26746224275235,2.99493785104705,-0.980185529411084));
#96567=CARTESIAN_POINT('Ctrl Pts',(-7.35004994567778,2.98181495654752,-0.991205086004124));
#96568=CARTESIAN_POINT('Ctrl Pts',(-7.3913943919297,2.97541039153636,-0.996702268783438));
#96569=CARTESIAN_POINT('Ctrl Pts',(-7.43274049243919,2.96915797897599,-1.00218200331461));
#96570=CARTESIAN_POINT('Origin',(0.196132190811885,2.94642874722832,0.0368498301381716));
#96571=CARTESIAN_POINT('',(-7.18760740282466,2.87870320492457,-1.64751336067173));
#96572=CARTESIAN_POINT('Origin',(-9.3198018746854E-13,2.97023924199933,
-5.52129956338243E-14));
#96573=CARTESIAN_POINT('',(-7.43371183306105,2.78894740126599,-0.994951446309474));
#96574=CARTESIAN_POINT('Ctrl Pts',(-7.43371183348005,2.78894740041728,-0.994951442589054));
#96575=CARTESIAN_POINT('Ctrl Pts',(-7.4245471698726,2.79982120464327,-1.06342460138507));
#96576=CARTESIAN_POINT('Ctrl Pts',(-7.41444876488241,2.81065020634229,-1.13167765525743));
#96577=CARTESIAN_POINT('Ctrl Pts',(-7.40343055618149,2.82142857082246,-1.19967328687996));
#96578=CARTESIAN_POINT('Ctrl Pts',(-7.38406329126841,2.84037424984021,-1.31919266278128));
#96579=CARTESIAN_POINT('Ctrl Pts',(-7.36174719434581,2.85947647430085,-1.43856937610525));
#96580=CARTESIAN_POINT('Ctrl Pts',(-7.33647897107824,2.87870320435315,-1.55758669346289));
#96581=CARTESIAN_POINT('',(-7.48732677997331,2.87870320271433,-0.435818413732416));
#96582=CARTESIAN_POINT('Origin',(0.190596323641602,2.9464046004507,0.000204179866555437));
#96583=CARTESIAN_POINT('Origin',(0.182451887430135,3.08920867961731,0.0439815725690257));
#96584=CARTESIAN_POINT('Ctrl Pts',(-7.184301272,3.009344995,-0.973814782));
#96585=CARTESIAN_POINT('Ctrl Pts',(-7.237615252,2.943588707,-0.580491841));
#96586=CARTESIAN_POINT('Ctrl Pts',(-7.24767235,2.878703203,-0.18369949));
#96587=CARTESIAN_POINT('Ctrl Pts',(-7.395000072,3.009344995,-1.250589437));
#96588=CARTESIAN_POINT('Ctrl Pts',(-7.463466788,2.943588707,-0.845731252));
#96589=CARTESIAN_POINT('Ctrl Pts',(-7.48732678,2.878703203,-0.435818406));
#96590=CARTESIAN_POINT('',(-7.24767233445532,2.87870320348066,-0.183699490833677));
#96591=CARTESIAN_POINT('',(-7.36749956477544,2.87870320212873,-0.309758953341122));
#96592=CARTESIAN_POINT('Origin',(0.191324778271704,3.08923051194625,0.0393547283114241));
#96593=CARTESIAN_POINT('Ctrl Pts',(-7.24445597850345,2.87421362531791,-0.213161097600263));
#96594=CARTESIAN_POINT('Ctrl Pts',(-7.24480356966667,2.87645841415895,-0.199628565955134));
#96595=CARTESIAN_POINT('Ctrl Pts',(-7.24515116083001,2.878703203,-0.18609603431));
#96596=CARTESIAN_POINT('Ctrl Pts',(-7.25526398982,2.944013165,0.20761989627));
#96597=CARTESIAN_POINT('Ctrl Pts',(-7.22265264346,3.00933735,0.600113212189999));
#96598=CARTESIAN_POINT('Ctrl Pts',(-7.24698612022989,2.87421362531791,-0.210773971470073));
#96599=CARTESIAN_POINT('Ctrl Pts',(-7.24732923511493,2.87645841415895,-0.197236730735039));
#96600=CARTESIAN_POINT('Ctrl Pts',(-7.24767235000001,2.878703203,-0.18369949));
#96601=CARTESIAN_POINT('Ctrl Pts',(-7.257654946,2.944013165,0.210153447));
#96602=CARTESIAN_POINT('Ctrl Pts',(-7.224899287,3.00933735,0.602768849999999));
#96603=CARTESIAN_POINT('Ctrl Pts',(-7.50051758257425,2.8742136253179,0.0284266915784136));
#96604=CARTESIAN_POINT('Ctrl Pts',(-7.5004121544549,2.87645841415895,0.0424358040815379));
#96605=CARTESIAN_POINT('Ctrl Pts',(-7.50030672633554,2.878703203,0.0564449165846612));
#96606=CARTESIAN_POINT('Ctrl Pts',(-7.49723939708658,2.944013165,0.464026506667312));
#96607=CARTESIAN_POINT('Ctrl Pts',(-7.45002296924085,3.00933735,0.868875578477823));
#96608=CARTESIAN_POINT('',(-7.49979126809725,2.87870320365573,0.0559549340228299));
#96609=CARTESIAN_POINT('',(-7.4744066564856,2.96915797898704,0.61906795124598));
#96610=CARTESIAN_POINT('Origin',(0.192636452580373,2.94642845830759,-0.0122977839134168));
#96611=CARTESIAN_POINT('',(-7.22528795887605,3.00855922068919,0.59809204170826));
#96612=CARTESIAN_POINT('Ctrl Pts',(-7.22528795819246,3.00855921913363,0.598092046812644));
#96613=CARTESIAN_POINT('Ctrl Pts',(-7.2667501538357,3.00166370046621,0.601543391562507));
#96614=CARTESIAN_POINT('Ctrl Pts',(-7.30826392881565,2.99493785104743,0.605020221165689));
#96615=CARTESIAN_POINT('Ctrl Pts',(-7.39128968801793,2.98181495150243,0.612012212856943));
#96616=CARTESIAN_POINT('Ctrl Pts',(-7.43284929343284,2.97541038109254,0.61553138801568));
#96617=CARTESIAN_POINT('Ctrl Pts',(-7.4744066565912,2.96915797898622,0.619067950003641));
#96618=CARTESIAN_POINT('Origin',(0.199468459704489,2.94642872644919,-0.00617432263199562));
#96619=CARTESIAN_POINT('',(-7.37373180839628,2.87870320492457,-0.0638722864739663));
#96620=CARTESIAN_POINT('Origin',(-5.72892427941341E-13,2.97023924200067,
-5.41220171977608E-14));
#96621=CARTESIAN_POINT('',(-7.47380093222391,2.78894740127503,0.62633827058956));
#96622=CARTESIAN_POINT('Ctrl Pts',(-7.47380093190115,2.78894740040347,0.62633827448373));
#96623=CARTESIAN_POINT('Ctrl Pts',(-7.47957023810749,2.79982120463978,0.557495848341243));
#96624=CARTESIAN_POINT('Ctrl Pts',(-7.48438031722103,2.81065020634327,0.488667654540507));
#96625=CARTESIAN_POINT('Ctrl Pts',(-7.48823675894358,2.82142857084232,0.419893134006143));
#96626=CARTESIAN_POINT('Ctrl Pts',(-7.49501542250106,2.84037424989509,0.299004664932385));
#96627=CARTESIAN_POINT('Ctrl Pts',(-7.49888352801377,2.85947647430086,0.177621611978818));
#96628=CARTESIAN_POINT('Ctrl Pts',(-7.49979126694244,2.87870320435315,0.0559549323218407));
#96629=CARTESIAN_POINT('',(-7.40596531758727,2.87870320271433,1.18392471247567));
#96630=CARTESIAN_POINT('Origin',(0.186184211535964,2.94640464720024,-0.0407731753774626));
#96631=CARTESIAN_POINT('Origin',(0.187641356349982,3.08920870438448,0.0037315182555403));
#96632=CARTESIAN_POINT('Ctrl Pts',(-7.225677693,3.009344995,0.593364874));
#96633=CARTESIAN_POINT('Ctrl Pts',(-7.19319241600001,2.943588707,0.988953072));
#96634=CARTESIAN_POINT('Ctrl Pts',(-7.117715759,2.878703203,1.378630618));
#96635=CARTESIAN_POINT('Ctrl Pts',(-7.490948841,3.009344995,0.36835507));
#96636=CARTESIAN_POINT('Ctrl Pts',(-7.470782301,2.943588707,0.778466215));
#96637=CARTESIAN_POINT('Ctrl Pts',(-7.405965316,2.878703203,1.18392472));
#96638=CARTESIAN_POINT('',(-7.11771574350775,2.87870320346112,1.37863061353755));
#96639=CARTESIAN_POINT('',(-7.26184053842887,2.87870320212873,1.28127766373548));
#96640=CARTESIAN_POINT('Origin',(0.195311683314985,3.08923059998896,-0.0026944978714246));
#96641=CARTESIAN_POINT('Ctrl Pts',(-7.12090795932426,2.87421362526545,1.34916638133665));
#96642=CARTESIAN_POINT('Ctrl Pts',(-7.11833832967722,2.87645841413273,1.36245725188334));
#96643=CARTESIAN_POINT('Ctrl Pts',(-7.11576870003,2.878703203,1.37574812243));
#96644=CARTESIAN_POINT('Ctrl Pts',(-7.04100780956999,2.944013165,1.76243315237));
#96645=CARTESIAN_POINT('Ctrl Pts',(-6.92478443736999,3.00933735,2.13873971657));
#96646=CARTESIAN_POINT('Ctrl Pts',(-7.12286578617501,2.87421362526545,1.35204160345241));
#96647=CARTESIAN_POINT('Ctrl Pts',(-7.12029077258757,2.87645841413273,1.36533611072621));
#96648=CARTESIAN_POINT('Ctrl Pts',(-7.117715759,2.878703203,1.378630618));
#96649=CARTESIAN_POINT('Ctrl Pts',(-7.04279822799999,2.944013165,1.765421455));
#96650=CARTESIAN_POINT('Ctrl Pts',(-6.926407672,3.00933735,2.141816229));
#96651=CARTESIAN_POINT('Ctrl Pts',(-7.31904875066755,2.87421362526546,1.64015165671574));
#96652=CARTESIAN_POINT('Ctrl Pts',(-7.31593424229251,2.87645841413272,1.65381058023419));
#96653=CARTESIAN_POINT('Ctrl Pts',(-7.3128197339176,2.878703203,1.66746950375257));
#96654=CARTESIAN_POINT('Ctrl Pts',(-7.22220612362153,2.944013165,2.06486267909898));
#96655=CARTESIAN_POINT('Ctrl Pts',(-7.08906300674669,3.00933735,2.45009646767011));
#96656=CARTESIAN_POINT('',(-7.31242165847653,2.87870320364628,1.66688016618383));
#96657=CARTESIAN_POINT('',(-7.16657787235505,2.9691579789703,2.21137097685948));
#96658=CARTESIAN_POINT('Origin',(0.185489064144846,2.94642850249844,-0.0534214073414038));
#96659=CARTESIAN_POINT('',(-6.92779263185941,3.00855922011726,2.13733231535534));
#96660=CARTESIAN_POINT('Ctrl Pts',(-6.92779263023839,3.00855921928044,2.13733232013128));
#96661=CARTESIAN_POINT('Ctrl Pts',(-6.96754352551728,3.0016637006159,2.14961612077638));
#96662=CARTESIAN_POINT('Ctrl Pts',(-7.00733931618843,2.99493785112561,2.1619358986615));
#96663=CARTESIAN_POINT('Ctrl Pts',(-7.08692087679833,2.98181495663568,2.18661249604047));
#96664=CARTESIAN_POINT('Ctrl Pts',(-7.12675228698315,2.97541039162993,2.19898347034704));
#96665=CARTESIAN_POINT('Ctrl Pts',(-7.16657787288143,2.9691579789718,2.21137097510419));
#96666=CARTESIAN_POINT('Origin',(0.193477601862492,2.94642873647769,-0.0489097679838857));
#96667=CARTESIAN_POINT('',(-7.21506870997276,2.87870320492457,1.52275538478368));
#96668=CARTESIAN_POINT('Origin',(-5.78963960107259E-13,2.97023924200022,
1.82362805412062E-13));
#96669=CARTESIAN_POINT('',(-7.16442340567892,2.78894740128806,2.21834110639615));
#96670=CARTESIAN_POINT('Ctrl Pts',(-7.16442340449826,2.78894740044059,2.218341109943));
#96671=CARTESIAN_POINT('Ctrl Pts',(-7.18485691423675,2.79982120465849,2.15234841177283));
#96672=CARTESIAN_POINT('Ctrl Pts',(-7.20435056352046,2.81065020634985,2.086163407635));
#96673=CARTESIAN_POINT('Ctrl Pts',(-7.22290133274774,2.82142857085343,2.0198258179021));
#96674=CARTESIAN_POINT('Ctrl Pts',(-7.25550896269093,2.8403742499258,1.90322086607327));
#96675=CARTESIAN_POINT('Ctrl Pts',(-7.28538040220174,2.85947647430087,1.78550720985898));
#96676=CARTESIAN_POINT('Ctrl Pts',(-7.31242165780932,2.87870320435315,1.66688016651236));
#96677=CARTESIAN_POINT('',(-6.97830914718863,2.87870320271433,2.74830883498448));
#96678=CARTESIAN_POINT('Origin',(0.173066247482618,2.94640463867172,-0.0798440046925969));
#96679=CARTESIAN_POINT('Origin',(0.184056299537407,3.08920868238395,-0.0366929833980065));
#96680=CARTESIAN_POINT('Ctrl Pts',(-6.929189456,3.009344995,2.132799448));
#96681=CARTESIAN_POINT('Ctrl Pts',(-6.812423898,2.943588707,2.512155639));
#96682=CARTESIAN_POINT('Ctrl Pts',(-6.654942689,2.878703203,2.87649749));
#96683=CARTESIAN_POINT('Ctrl Pts',(-7.236629169,3.009344995,1.970075703));
#96684=CARTESIAN_POINT('Ctrl Pts',(-7.128772338,2.943588707,2.366263468));
#96685=CARTESIAN_POINT('Ctrl Pts',(-6.978309144,2.878703203,2.748308842));
#96686=CARTESIAN_POINT('',(-6.65494267496771,2.8787032034983,2.87649748235107));
#96687=CARTESIAN_POINT('',(-6.81662591853887,2.87870320212873,2.81240316105823));
#96688=CARTESIAN_POINT('Origin',(0.190166153774641,3.08923059048807,-0.0446177339177142));
#96689=CARTESIAN_POINT('Ctrl Pts',(-6.66439419721484,2.87421362532376,2.8484083398753));
#96690=CARTESIAN_POINT('Ctrl Pts',(-6.65902749986735,2.87645841416188,2.86083608265768));
#96691=CARTESIAN_POINT('Ctrl Pts',(-6.65366080252,2.878703203,2.87326382544));
#96692=CARTESIAN_POINT('Ctrl Pts',(-6.49752192928999,2.944013165,3.23483699218));
#96693=CARTESIAN_POINT('Ctrl Pts',(-6.30312100693,3.00933735,3.57736112926));
#96694=CARTESIAN_POINT('Ctrl Pts',(-6.66568816340659,2.87421362532376,2.85163721580676));
#96695=CARTESIAN_POINT('Ctrl Pts',(-6.66031542620323,2.87645841416188,2.8640673529034));
#96696=CARTESIAN_POINT('Ctrl Pts',(-6.65494268900001,2.878703203,2.87649749));
#96697=CARTESIAN_POINT('Ctrl Pts',(-6.498628092,2.944013165,3.238140317));
#96698=CARTESIAN_POINT('Ctrl Pts',(-6.304044932,3.00933735,3.580714662));
#96699=CARTESIAN_POINT('Ctrl Pts',(-6.7953493351026,2.87421362532376,3.17518495546575));
#96700=CARTESIAN_POINT('Ctrl Pts',(-6.7893713774583,2.87645841416188,3.18785501350917));
#96701=CARTESIAN_POINT('Ctrl Pts',(-6.78339341981402,2.878703203,3.20052507155262));
#96702=CARTESIAN_POINT('Ctrl Pts',(-6.60947051893528,2.944013165,3.5691481666538));
#96703=CARTESIAN_POINT('Ctrl Pts',(-6.3966263362901,3.00933735,3.91675356870704));
#96704=CARTESIAN_POINT('',(-6.78313134128405,2.87870320364628,3.19986393784715));
#96705=CARTESIAN_POINT('',(-6.52364787174035,2.96915797895534,3.70027275209121));
#96706=CARTESIAN_POINT('Origin',(0.169668427901872,2.94642847961565,-0.092047134371907));
#96707=CARTESIAN_POINT('',(-6.30636142167441,3.00855922005457,3.57663330547928));
#96708=CARTESIAN_POINT('Ctrl Pts',(-6.30636141925212,3.00855921911747,3.57663330943115));
#96709=CARTESIAN_POINT('Ctrl Pts',(-6.34254230674416,3.00166370044041,3.59717518928132));
#96710=CARTESIAN_POINT('Ctrl Pts',(-6.37875930532485,2.99493785105421,3.61776185602894));
#96711=CARTESIAN_POINT('Ctrl Pts',(-6.45117555386215,2.9818149566436,3.65896921127782));
#96712=CARTESIAN_POINT('Ctrl Pts',(-6.48741633343306,2.97541039173818,3.67961353455249));
#96713=CARTESIAN_POINT('Ctrl Pts',(-6.52364787265427,2.96915797895447,3.70027275048276));
#96714=CARTESIAN_POINT('Origin',(0.178440093734214,2.94642876048637,-0.0893582737752734));
#96715=CARTESIAN_POINT('',(-6.7190370179336,2.87870320492457,3.03818070708917));
#96716=CARTESIAN_POINT('Origin',(-2.69315819645399E-13,2.97023924200022,
1.02565525517129E-13));
#96717=CARTESIAN_POINT('',(-6.52004540366864,2.78894740123955,3.70661677740616));
#96718=CARTESIAN_POINT('Ctrl Pts',(-6.52004540174397,2.78894740037085,3.70661678078457));
#96719=CARTESIAN_POINT('Ctrl Pts',(-6.55418766686882,2.79982120461768,3.64655955570536));
#96720=CARTESIAN_POINT('Ctrl Pts',(-6.58745338504171,2.81065020633199,3.5861124785167));
#96721=CARTESIAN_POINT('Ctrl Pts',(-6.61983106844917,2.82142857082093,3.52531369197218));
#96722=CARTESIAN_POINT('Ctrl Pts',(-6.6767429673408,2.84037424983601,3.41844457607452));
#96723=CARTESIAN_POINT('Ctrl Pts',(-6.73122098611541,2.85947647430085,3.30990447608648));
#96724=CARTESIAN_POINT('Ctrl Pts',(-6.78313134059163,2.87870320435315,3.19986393809974));
#96725=CARTESIAN_POINT('',(-6.22435499666414,2.87870320271433,4.18418509082716));
#96726=CARTESIAN_POINT('Origin',(0.151855941409106,2.94640463093673,-0.115181421971133));
#96727=CARTESIAN_POINT('Origin',(0.171865247837747,3.0892087258185,-0.0754017748086588));
#96728=CARTESIAN_POINT('Ctrl Pts',(-6.308700021,3.009344995,3.572506689));
#96729=CARTESIAN_POINT('Ctrl Pts',(-6.113114009,2.943588707,3.9178926));
#96730=CARTESIAN_POINT('Ctrl Pts',(-5.880991895,2.878703203,4.239862537));
#96731=CARTESIAN_POINT('Ctrl Pts',(-6.643932759,3.009344995,3.479677786));
#96732=CARTESIAN_POINT('Ctrl Pts',(-6.453428903,2.943588707,3.84341687));
#96733=CARTESIAN_POINT('Ctrl Pts',(-6.224354992,2.878703203,4.184185097));
#96734=CARTESIAN_POINT('',(-5.88099188278071,2.87870320349035,4.23986252603742));
#96735=CARTESIAN_POINT('',(-6.05267344655354,2.87870320212873,4.21202381261207));
#96736=CARTESIAN_POINT('Origin',(0.176128705036702,3.08923060890683,-0.0844547233562909));
#96737=CARTESIAN_POINT('Ctrl Pts',(-5.89626076918051,2.87421362531623,4.21446189044749));
#96738=CARTESIAN_POINT('Ctrl Pts',(-5.8883479448953,2.87645841415811,4.22544539823875));
#96739=CARTESIAN_POINT('Ctrl Pts',(-5.88043512061,2.878703203,4.23642890603));
#96740=CARTESIAN_POINT('Ctrl Pts',(-5.65021914495,2.944013165,4.5559834508));
#96741=CARTESIAN_POINT('Ctrl Pts',(-5.38673064420001,3.00933735,4.84870911242));
#96742=CARTESIAN_POINT('Ctrl Pts',(-5.89683037027871,2.87421362531623,4.2178934415251));
#96743=CARTESIAN_POINT('Ctrl Pts',(-5.88891113263942,2.87645841415811,4.22887798926253));
#96744=CARTESIAN_POINT('Ctrl Pts',(-5.880991895,2.878703203,4.239862537));
#96745=CARTESIAN_POINT('Ctrl Pts',(-5.650589329,2.944013165,4.559447338));
#96746=CARTESIAN_POINT('Ctrl Pts',(-5.386912058,3.00933735,4.852182858));
#96747=CARTESIAN_POINT('Ctrl Pts',(-5.95390693554475,2.87421362531623,4.56175013290872));
#96748=CARTESIAN_POINT('Ctrl Pts',(-5.94534505127836,2.87645841415811,4.57283888788507));
#96749=CARTESIAN_POINT('Ctrl Pts',(-5.93678316701207,2.878703203,4.58392764286153));
#96750=CARTESIAN_POINT('Ctrl Pts',(-5.6876834184535,2.944013165,4.90654425277428));
#96751=CARTESIAN_POINT('Ctrl Pts',(-5.40509052821043,3.00933735,5.20026762632871));
#96752=CARTESIAN_POINT('',(-5.93666933994906,2.87870320364628,4.58322562703605));
#96753=CARTESIAN_POINT('',(-5.57567934758532,2.96915797894798,5.0161538860231));
#96754=CARTESIAN_POINT('Origin',(0.145914193178012,2.9464284750525,-0.126368748783031));
#96755=CARTESIAN_POINT('',(-5.3900517594732,3.00855922011665,4.84869489727826));
#96756=CARTESIAN_POINT('Ctrl Pts',(-5.39005175646099,3.00855921928191,4.84869490041694));
#96757=CARTESIAN_POINT('Ctrl Pts',(-5.42097085771323,3.0016637006203,4.87653434368228));
#96758=CARTESIAN_POINT('Ctrl Pts',(-5.45191559860267,2.99493785111403,4.90442529016004));
#96759=CARTESIAN_POINT('Ctrl Pts',(-5.51378045129136,2.98181495260962,4.96023661051122));
#96760=CARTESIAN_POINT('Ctrl Pts',(-5.54473604521456,2.97541038325639,4.98818899810971));
#96761=CARTESIAN_POINT('Ctrl Pts',(-5.57567934830649,2.96915797897617,5.01615388499148));
#96762=CARTESIAN_POINT('Origin',(0.15505878287245,2.9464287453994,-0.125628383698799));
#96763=CARTESIAN_POINT('',(-5.90883062166377,2.87870320492457,4.41154407590484));
#96764=CARTESIAN_POINT('Ctrl Pts',(-5.39322278500001,3.009344995,4.845167489));
#96765=CARTESIAN_POINT('Ctrl Pts',(-5.127961704,2.943588707,5.14043325799999));
#96766=CARTESIAN_POINT('Ctrl Pts',(-4.832052457,2.878703203,5.404976323));
#96767=CARTESIAN_POINT('Ctrl Pts',(-5.740573438,3.009344995,4.826574003));
#96768=CARTESIAN_POINT('Ctrl Pts',(-5.476330305,2.943588707,5.140856372));
#96769=CARTESIAN_POINT('Ctrl Pts',(-5.179356919,2.878703203,5.424413508));
#96770=CARTESIAN_POINT('',(-5.17935691552083,2.8787032027125,5.42441350247272));
#96771=CARTESIAN_POINT('Origin',(0.151636229114196,3.08920894165074,-0.110583258555224));
#96772=CARTESIAN_POINT('',(-4.83205244725023,2.87870320348952,5.40497631046383));
#96773=CARTESIAN_POINT('',(-5.00570469192539,2.87870320212873,5.41469491187111));
#96774=CARTESIAN_POINT('Origin',(0.153855660404065,3.0892305891035,-0.120342688878163));
#96775=CARTESIAN_POINT('Origin',(-8.52182907573606E-13,2.97023924199978,
7.3595643468316E-13));
#96776=CARTESIAN_POINT('',(-5.57079732493957,2.78894740126208,5.02157516776139));
#96777=CARTESIAN_POINT('Ctrl Pts',(-5.57079732239725,2.78894740042159,5.02157517044124));
#96778=CARTESIAN_POINT('Ctrl Pts',(-5.61705188831202,2.79982120464436,4.97026162768222));
#96779=CARTESIAN_POINT('Ctrl Pts',(-5.66253420719846,2.81065020634201,4.91837891565976));
#96780=CARTESIAN_POINT('Ctrl Pts',(-5.70722486025001,2.82142857081912,4.86596181587965));
#96781=CARTESIAN_POINT('Ctrl Pts',(-5.7857798915122,2.84037424983099,4.77382561681668));
#96782=CARTESIAN_POINT('Ctrl Pts',(-5.86231715742168,2.85947647430087,4.6795342873684));
#96783=CARTESIAN_POINT('Ctrl Pts',(-5.93666933920597,2.87870320435315,4.58322562705654));
#96784=CARTESIAN_POINT('Origin',(0.12354331983747,2.94640418831007,-0.145131449832491));
#96785=CARTESIAN_POINT('Ctrl Pts',(-4.85242474194373,2.87421362524044,5.38345188573344));
#96786=CARTESIAN_POINT('Ctrl Pts',(-4.84233578539689,2.87645841412021,5.39247758205179));
#96787=CARTESIAN_POINT('Ctrl Pts',(-4.83224682884999,2.878703203,5.40150327837001));
#96788=CARTESIAN_POINT('Ctrl Pts',(-4.538718393,2.944013165,5.66409718592));
#96789=CARTESIAN_POINT('Ctrl Pts',(-4.21846274216001,3.00933735,5.89333684504));
#96790=CARTESIAN_POINT('Ctrl Pts',(-4.85224334403582,2.87421362524044,5.38692565646078));
#96791=CARTESIAN_POINT('Ctrl Pts',(-4.84214790051791,2.87645841412021,5.39595098973046));
#96792=CARTESIAN_POINT('Ctrl Pts',(-4.832052457,2.878703203,5.404976323));
#96793=CARTESIAN_POINT('Ctrl Pts',(-4.538335289,2.944013165,5.667559668));
#96794=CARTESIAN_POINT('Ctrl Pts',(-4.217893162,3.00933735,5.896768375));
#96795=CARTESIAN_POINT('Ctrl Pts',(-4.83406646628024,2.87421362524044,5.73501294467682));
#96796=CARTESIAN_POINT('Ctrl Pts',(-4.82332099939224,2.87645841412021,5.74400189885382));
#96797=CARTESIAN_POINT('Ctrl Pts',(-4.81257553250423,2.878703203,5.75299085303085));
#96798=CARTESIAN_POINT('Ctrl Pts',(-4.49994656305007,2.944013165,6.01451578350822));
#96799=CARTESIAN_POINT('Ctrl Pts',(-4.16081869483506,3.00933735,6.24062295032004));
#96800=CARTESIAN_POINT('',(-4.81261527617338,2.87870320365809,5.75228078483036));
#96801=CARTESIAN_POINT('',(-4.3669982542543,2.96915797894115,6.09748523951937));
#96802=CARTESIAN_POINT('Origin',(0.115337244766743,2.94642848604879,-0.154781540117167));
#96803=CARTESIAN_POINT('',(-4.22170926802649,3.00855922011897,5.894036904481));
#96804=CARTESIAN_POINT('Ctrl Pts',(-4.22170926388751,3.00855921923334,5.89403690726225));
#96805=CARTESIAN_POINT('Ctrl Pts',(-4.24592083658128,3.00166370058843,5.9278721725509));
#96806=CARTESIAN_POINT('Ctrl Pts',(-4.27014637778941,2.99493785108862,5.9617632487325));
#96807=CARTESIAN_POINT('Ctrl Pts',(-4.318567084774,2.9818149515275,6.02956885146576));
#96808=CARTESIAN_POINT('Ctrl Pts',(-4.34279002162138,2.97541038108071,6.0635222716142));
#96809=CARTESIAN_POINT('Ctrl Pts',(-4.36699825526788,2.96915797894033,6.09748523879675));
#96810=CARTESIAN_POINT('Origin',(0.124427177248334,2.94642874500272,-0.156024291755323));
#96811=CARTESIAN_POINT('',(-4.82233387355899,2.87870320492458,5.57862854666914));
#96812=CARTESIAN_POINT('Origin',(7.22729168178837E-13,2.97023924200044,
-9.77082997843937E-13));
#96813=CARTESIAN_POINT('',(-3.8921778798055,2.87870320271433,6.41100236735067));
#96814=CARTESIAN_POINT('Origin',(0.124320393650231,3.08920869069784,-0.140597308569476));
#96815=CARTESIAN_POINT('',(-4.36106495481666,2.78894740129025,6.1017302840077));
#96816=CARTESIAN_POINT('Ctrl Pts',(-4.36106495490976,2.7889474010463,6.10173028407192));
#96817=CARTESIAN_POINT('Ctrl Pts',(-4.41726900647749,2.7998212046449,6.06155979027827));
#96818=CARTESIAN_POINT('Ctrl Pts',(-4.47284122357436,2.81065020634812,6.02066742140645));
#96819=CARTESIAN_POINT('Ctrl Pts',(-4.52775516105136,2.8214285708076,5.97908297344064));
#96820=CARTESIAN_POINT('Ctrl Pts',(-4.62428017742959,2.84037424955422,5.90598787681786));
#96821=CARTESIAN_POINT('Ctrl Pts',(-4.71929789205897,2.85947647380709,5.8303542776607));
#96822=CARTESIAN_POINT('Ctrl Pts',(-4.81261527495825,2.87870320360758,5.75228078336553));
#96823=CARTESIAN_POINT('Origin',(0.0894574475054982,2.94640462797529,-0.168298699732703));
#96824=CARTESIAN_POINT('Ctrl Pts',(-4.225564445,3.009344995,5.891273642));
#96825=CARTESIAN_POINT('Ctrl Pts',(-3.903031608,2.943588707,6.12261297));
#96826=CARTESIAN_POINT('Ctrl Pts',(-3.557171616,2.878703203,6.317359424));
#96827=CARTESIAN_POINT('Ctrl Pts',(-4.568791283,3.009344995,5.94778498400001));
#96828=CARTESIAN_POINT('Ctrl Pts',(-4.243164588,2.943588707,6.197915143));
#96829=CARTESIAN_POINT('Ctrl Pts',(-3.892177873,2.878703203,6.411002371));
#96830=CARTESIAN_POINT('',(-3.55717160955683,2.8787032034775,6.31735940957115));
#96831=CARTESIAN_POINT('Origin',(0.124388509564735,3.08923057516672,-0.150603615695601));
#96832=CARTESIAN_POINT('',(-3.72467474911375,2.87870320212873,6.36418089479977));
#96833=CARTESIAN_POINT('Ctrl Pts',(-3.58169472559154,2.87421362531487,6.30071765536191));
#96834=CARTESIAN_POINT('Ctrl Pts',(-3.5699013855308,2.87645841415743,6.30736350839607));
#96835=CARTESIAN_POINT('Ctrl Pts',(-3.55810804547,2.878703203,6.31400936143));
#96836=CARTESIAN_POINT('Ctrl Pts',(-3.21499221354,2.944013165,6.50736403287));
#96837=CARTESIAN_POINT('Ctrl Pts',(-2.8529442122,3.00933735,6.6623986972));
#96838=CARTESIAN_POINT('Ctrl Pts',(-3.58077081065103,2.87421362531487,6.30407121606779));
#96839=CARTESIAN_POINT('Ctrl Pts',(-3.56897121332551,2.87645841415743,6.31071532003394));
#96840=CARTESIAN_POINT('Ctrl Pts',(-3.557171616,2.878703203,6.317359424));
#96841=CARTESIAN_POINT('Ctrl Pts',(-3.213873735,2.944013165,6.51066320800001));
#96842=CARTESIAN_POINT('Ctrl Pts',(-2.851650271,3.00933735,6.66562755700001));
#96843=CARTESIAN_POINT('Ctrl Pts',(-3.48819042137566,2.87421362531487,6.6401129250722));
#96844=CARTESIAN_POINT('Ctrl Pts',(-3.47576381827483,2.87645841415743,6.64658176465065));
#96845=CARTESIAN_POINT('Ctrl Pts',(-3.46333721517399,2.878703203,6.65305060422911));
#96846=CARTESIAN_POINT('Ctrl Pts',(-3.10179720708204,2.944013165,6.84125524024739));
#96847=CARTESIAN_POINT('Ctrl Pts',(-2.72199160358739,3.00933735,6.98917368021653));
#96848=CARTESIAN_POINT('',(-3.46352867565415,2.87870320365576,6.65236567872762));
#96849=CARTESIAN_POINT('',(-2.95412117554173,2.96915797898617,6.89370496034624));
#96850=CARTESIAN_POINT('Origin',(0.0793673339405909,2.9464285207357,-0.175957075573957));
#96851=CARTESIAN_POINT('',(-2.8559643433261,3.00855922006514,6.66378029754188));
#96852=CARTESIAN_POINT('Ctrl Pts',(-2.85596433928434,3.00855921920204,6.6637802991163));
#96853=CARTESIAN_POINT('Ctrl Pts',(-2.87233627702716,3.00166370051212,6.70202928740138));
#96854=CARTESIAN_POINT('Ctrl Pts',(-2.88870985871751,2.9949378510811,6.74033578394761));
#96855=CARTESIAN_POINT('Ctrl Pts',(-2.92142231603079,2.98181495151758,6.81696515014832));
#96856=CARTESIAN_POINT('Ctrl Pts',(-2.93777995225721,2.97541038108882,6.85533197352984));
#96857=CARTESIAN_POINT('Ctrl Pts',(-2.95412117667018,2.96915797898535,6.89370495986555));
#96858=CARTESIAN_POINT('Origin',(0.0879774927772421,2.94642876675558,-0.179124625771928));
#96859=CARTESIAN_POINT('',(-3.51035015303056,2.87870320492457,6.48486254679966));
#96860=CARTESIAN_POINT('Origin',(1.82145964977565E-14,2.97023924199967,
1.08853898117545E-13));
#96861=CARTESIAN_POINT('',(-2.94741403486527,2.78894740127924,6.89657527394928));
#96862=CARTESIAN_POINT('Ctrl Pts',(-2.94741403109273,2.78894740037632,6.89657527581036));
#96863=CARTESIAN_POINT('Ctrl Pts',(-3.01093953572611,2.79982120463271,6.86942615381304));
#96864=CARTESIAN_POINT('Ctrl Pts',(-3.07400315581137,2.81065020634479,6.84143620967188));
#96865=CARTESIAN_POINT('Ctrl Pts',(-3.1365726630489,2.82142857082642,6.81262885629397));
#96866=CARTESIAN_POINT('Ctrl Pts',(-3.24655426490462,2.84037424985116,6.76199270720585));
#96867=CARTESIAN_POINT('Ctrl Pts',(-3.35560950750758,2.85947647430088,6.7085533784839));
#96868=CARTESIAN_POINT('Ctrl Pts',(-3.4635286766403,2.87870320435315,6.65236567688422));
#96869=CARTESIAN_POINT('',(-2.42300492243708,2.87870320271434,7.09781988690226));
#96870=CARTESIAN_POINT('Origin',(0.0511867594797774,2.9464046138362,-0.183594736941044));
#96871=CARTESIAN_POINT('Origin',(0.09118953595046,3.08920869532132,-0.164035303891673));
#96872=CARTESIAN_POINT('Ctrl Pts',(-2.860323408,3.009344995,6.661910387));
#96873=CARTESIAN_POINT('Ctrl Pts',(-2.495600093,2.943588707,6.818506104));
#96874=CARTESIAN_POINT('Ctrl Pts',(-2.115961384,2.878703203,6.93434982));
#96875=CARTESIAN_POINT('Ctrl Pts',(-3.183377525,3.009344995,6.79088415));
#96876=CARTESIAN_POINT('Ctrl Pts',(-2.811593211,2.943588707,6.965166291));
#96877=CARTESIAN_POINT('Ctrl Pts',(-2.423004915,2.878703203,7.097819889));
#96878=CARTESIAN_POINT('',(-2.11596138092829,2.8787032035214,6.93434980424421));
#96879=CARTESIAN_POINT('',(-2.26948315458636,2.87870320212873,7.01608485285472));
#96880=CARTESIAN_POINT('Origin',(0.0891050703775054,3.08923060677095,-0.173822507783961));
#96881=CARTESIAN_POINT('Ctrl Pts',(-2.14348864496989,2.87421362536565,6.92336887051515));
#96882=CARTESIAN_POINT('Ctrl Pts',(-2.13054236483491,2.87645841418282,6.92732412760264));
#96883=CARTESIAN_POINT('Ctrl Pts',(-2.1175960847,2.878703203,6.93127938469));
#96884=CARTESIAN_POINT('Ctrl Pts',(-1.74093657126,2.944013165,7.04635376857));
#96885=CARTESIAN_POINT('Ctrl Pts',(-1.35402518099,3.00933735,7.11993419126));
#96886=CARTESIAN_POINT('Ctrl Pts',(-2.14186541422007,2.87421362536565,6.92644541242972));
#96887=CARTESIAN_POINT('Ctrl Pts',(-2.12891339911001,2.87645841418282,6.93039761621492));
#96888=CARTESIAN_POINT('Ctrl Pts',(-2.115961384,2.878703203,6.93434982));
#96889=CARTESIAN_POINT('Ctrl Pts',(-1.739135017,2.944013165,7.049335371));
#96890=CARTESIAN_POINT('Ctrl Pts',(-1.352067382,3.00933735,7.122809403));
#96891=CARTESIAN_POINT('Ctrl Pts',(-1.97921046829331,2.87421362536565,7.23472860556921));
#96892=CARTESIAN_POINT('Ctrl Pts',(-1.96568378315297,2.87645841418282,7.23837485487639));
#96893=CARTESIAN_POINT('Ctrl Pts',(-1.95215709801269,2.878703203,7.24202110418358));
#96894=CARTESIAN_POINT('Ctrl Pts',(-1.55861126165646,2.944013165,7.34810520522359));
#96895=CARTESIAN_POINT('Ctrl Pts',(-1.15588720928481,3.00933735,7.41091841655401));
#96896=CARTESIAN_POINT('',(-1.95249132098841,2.87870320365575,7.24139335021025));
#96897=CARTESIAN_POINT('',(-1.40311267351616,2.96915797892996,7.36758269877179));
#96898=CARTESIAN_POINT('Origin',(0.0396862188766633,2.94642847507453,-0.188904990300104));
#96899=CARTESIAN_POINT('',(-1.35667770072638,3.00855922010768,7.12193272850302));
#96900=CARTESIAN_POINT('Ctrl Pts',(-1.35667769588376,3.00855921925971,7.12193272928015));
#96901=CARTESIAN_POINT('Ctrl Pts',(-1.36444446482813,3.00166370057974,7.16280696003061));
#96902=CARTESIAN_POINT('Ctrl Pts',(-1.37220047685128,2.99493785109333,7.20373770835499));
#96903=CARTESIAN_POINT('Ctrl Pts',(-1.38767508043678,2.98181495662563,7.2856077020983));
#96904=CARTESIAN_POINT('Ctrl Pts',(-1.39540254430737,2.97541039165304,7.32659390134666));
#96905=CARTESIAN_POINT('Ctrl Pts',(-1.40311267532109,2.96915797893043,7.36758269842035));
#96906=CARTESIAN_POINT('Origin',(0.0474141165200966,2.94642877611754,-0.193849341569747));
#96907=CARTESIAN_POINT('',(-2.03422636050977,2.87870320492457,7.08787158219669));
#96908=CARTESIAN_POINT('Origin',(-1.15142270717961E-13,2.97023924199922,
8.89479462307108E-13));
#96909=CARTESIAN_POINT('',(-1.39594530977002,2.78894740124346,7.36894406900654));
#96910=CARTESIAN_POINT('Ctrl Pts',(-1.39594530611969,2.78894740040204,7.36894406960381));
#96911=CARTESIAN_POINT('Ctrl Pts',(-1.46382187831905,2.79982120463159,7.35608578463714));
#96912=CARTESIAN_POINT('Ctrl Pts',(-1.53142811658635,2.81065020633578,7.34230704400092));
#96913=CARTESIAN_POINT('Ctrl Pts',(-1.59872751298941,2.82142857082903,7.32762378513747));
#96914=CARTESIAN_POINT('Ctrl Pts',(-1.71702308128857,2.84037424985837,7.3018142747674));
#96915=CARTESIAN_POINT('Ctrl Pts',(-1.83501654880148,2.85947647430087,7.27306798144716));
#96916=CARTESIAN_POINT('Ctrl Pts',(-1.95249132234644,2.87870320435315,7.24139334862288));
#96917=CARTESIAN_POINT('',(-0.840534948682288,2.87870320271433,7.45275123752289));
#96918=CARTESIAN_POINT('Origin',(0.0105225791164858,2.94640460981423,-0.190305859621067));
#96919=CARTESIAN_POINT('Origin',(0.0537948407192751,3.08920870227923,-0.179803285374214));
#96920=CARTESIAN_POINT('Ctrl Pts',(-1.361336828,3.009344995,7.121043606));
#96921=CARTESIAN_POINT('Ctrl Pts',(-0.971477090999999,2.943588707,7.195573471));
#96922=CARTESIAN_POINT('Ctrl Pts',(-0.575811149,2.878703203,7.227097725));
#96923=CARTESIAN_POINT('Ctrl Pts',(-1.649112573,3.009344995,7.31644912000001));
#96924=CARTESIAN_POINT('Ctrl Pts',(-1.248554861,2.943588707,7.406734004));
#96925=CARTESIAN_POINT('Ctrl Pts',(-0.840534941,2.878703203,7.45275123800001));
#96926=CARTESIAN_POINT('',(-0.575811149137818,2.87870320291937,7.22709770862388));
#96927=CARTESIAN_POINT('',(-0.708173050321132,2.87870320212873,7.33992448098661));
#96928=CARTESIAN_POINT('Origin',(0.0496551467651213,3.0892306107498,-0.188913537216816));
#96929=CARTESIAN_POINT('Origin',(1.01210272801522E-13,2.97023924199933,
1.20823490101785E-12));
#96930=CARTESIAN_POINT('',(0.220796265851409,2.78894740126403,7.49674922941047));
#96931=CARTESIAN_POINT('',(-0.350157643002028,2.87870320365575,7.49182151673046));
#96932=CARTESIAN_POINT('Ctrl Pts',(0.220796270213487,2.78894740034443,7.49674922963154));
#96933=CARTESIAN_POINT('Ctrl Pts',(0.151742463241555,2.79982120461821,7.49878302093711));
#96934=CARTESIAN_POINT('Ctrl Pts',(0.0827547993552023,2.8106502063407,7.49985976246062));
#96935=CARTESIAN_POINT('Ctrl Pts',(0.0138723589321241,2.82142857082974,
7.49998717083208));
#96936=CARTESIAN_POINT('Ctrl Pts',(-0.107205806614306,2.84037424986034,
7.50021112251022));
#96937=CARTESIAN_POINT('Ctrl Pts',(-0.22862025575631,2.85947647430103,7.49750200929462));
#96938=CARTESIAN_POINT('Ctrl Pts',(-0.3501576446624,2.87870320435365,7.49182151547619));
#96939=CARTESIAN_POINT('Origin',(-0.0306335706352003,2.94640463429058,-0.188118757514659));
#96940=CARTESIAN_POINT('Origin',(-0.00185061631441531,2.94642847975205,
-0.193019681328986));
#96941=CARTESIAN_POINT('Ctrl Pts',(-0.605055418118393,2.87421362524808,
7.22229105134406));
#96942=CARTESIAN_POINT('Ctrl Pts',(-0.591561551124188,2.87645841412404,
7.22337076921714));
#96943=CARTESIAN_POINT('Ctrl Pts',(-0.57806768413,2.878703203,7.22445048709));
#96944=CARTESIAN_POINT('Ctrl Pts',(-0.18547667031,2.944013165,7.25586383469));
#96945=CARTESIAN_POINT('Ctrl Pts',(0.20820656273,3.00933735,7.24454947603));
#96946=CARTESIAN_POINT('Ctrl Pts',(-0.602808772038777,2.87421362524808,
7.22494671879012));
#96947=CARTESIAN_POINT('Ctrl Pts',(-0.589309960519383,2.87645841412404,
7.22602222189512));
#96948=CARTESIAN_POINT('Ctrl Pts',(-0.575811149000001,2.878703203,7.227097725));
#96949=CARTESIAN_POINT('Ctrl Pts',(-0.183076279,2.944013165,7.258388448));
#96950=CARTESIAN_POINT('Ctrl Pts',(0.210736675,3.00933735,7.246936598));
#96951=CARTESIAN_POINT('Ctrl Pts',(-0.377684835310627,2.87421362524809,
7.49105641693585));
#96952=CARTESIAN_POINT('Ctrl Pts',(-0.363690560359198,2.87645841412404,
7.49170958152752));
#96953=CARTESIAN_POINT('Ctrl Pts',(-0.349696285407776,2.878703203,7.49236274611927));
#96954=CARTESIAN_POINT('Ctrl Pts',(0.0574536141147641,2.944013165,7.51136593841193));
#96955=CARTESIAN_POINT('Ctrl Pts',(0.464265185679141,3.00933735,7.48613684418653));
#96956=CARTESIAN_POINT('Origin',(0.00463374273094159,2.94642873394642,-0.199509935818043));
#96957=CARTESIAN_POINT('',(-0.46298440445079,2.87870320492457,7.35945961974818));
#96958=CARTESIAN_POINT('Ctrl Pts',(-1.18865511349561,3.01309343441768,7.4057932170506));
#96959=CARTESIAN_POINT('Ctrl Pts',(-1.17466739473715,3.01082632770884,7.40798415865071));
#96960=CARTESIAN_POINT('Ctrl Pts',(-1.16067967597869,3.008559221,7.41017510025082));
#96961=CARTESIAN_POINT('Ctrl Pts',(-0.755006818590786,2.942808424,7.47371695111569));
#96962=CARTESIAN_POINT('Ctrl Pts',(-0.344821887743239,2.877933005,7.49259435614662));
#96963=CARTESIAN_POINT('Ctrl Pts',(-1.38356493866731,3.01309343441768,7.1168108876801));
#96964=CARTESIAN_POINT('Ctrl Pts',(-1.37012131683364,3.01082632770884,7.11937180234004));
#96965=CARTESIAN_POINT('Ctrl Pts',(-1.356677695,3.008559221,7.121932717));
#96966=CARTESIAN_POINT('Ctrl Pts',(-0.966784777,2.942808424,7.196204554));
#96967=CARTESIAN_POINT('Ctrl Pts',(-0.571114157,2.877933005,7.227470416));
#96968=CARTESIAN_POINT('',(-0.597132064613574,2.91791835922337,7.47619110706827));
#96969=CARTESIAN_POINT('Ctrl Pts',(-0.597132067174111,2.91791835924552,
7.4761910949071));
#96970=CARTESIAN_POINT('Ctrl Pts',(-0.593617782586462,2.91168301766321,
7.43463380428372));
#96971=CARTESIAN_POINT('Ctrl Pts',(-0.590083571577411,2.90530192562621,
7.39307657483869));
#96972=CARTESIAN_POINT('Ctrl Pts',(-0.58297921601715,2.89224022492298,7.31005814253514));
#96973=CARTESIAN_POINT('Ctrl Pts',(-0.579405192990811,2.88555248749285,
7.26855156492777));
#96974=CARTESIAN_POINT('Ctrl Pts',(-0.575811147778446,2.87870320302431,
7.22709772429943));
#96975=CARTESIAN_POINT('',(-1.16108395640224,3.00855922016356,7.40958056024041));
#96976=CARTESIAN_POINT('Origin',(0.0421309665231484,3.08925205799903,-0.185224272254657));
#96977=CARTESIAN_POINT('',(-1.25888083740932,3.00855921853322,7.26575663541678));
#96978=CARTESIAN_POINT('Ctrl Pts',(-2.43066974068,2.877925369,7.09788290211));
#96979=CARTESIAN_POINT('Ctrl Pts',(-2.04495695187,2.943232886,7.22997023301));
#96980=CARTESIAN_POINT('Ctrl Pts',(-1.64720201441,3.008559221,7.31948240046));
#96981=CARTESIAN_POINT('Ctrl Pts',(-2.427598248,2.877925369,7.096250189));
#96982=CARTESIAN_POINT('Ctrl Pts',(-2.041974184,2.943232886,7.228170609));
#96983=CARTESIAN_POINT('Ctrl Pts',(-1.644325536,3.008559221,7.317526463));
#96984=CARTESIAN_POINT('Ctrl Pts',(-2.12044898,2.877925369,6.932978878));
#96985=CARTESIAN_POINT('Ctrl Pts',(-1.743697397,2.943232886,7.048208208));
#96986=CARTESIAN_POINT('Ctrl Pts',(-1.356677695,3.008559221,7.121932717));
#96987=CARTESIAN_POINT('',(-1.64432554279485,3.00855922118749,7.31752646662718));
#96988=CARTESIAN_POINT('',(-1.50050161853982,3.00855922150568,7.21972958936822));
#96989=CARTESIAN_POINT('',(-2.1903315442912,2.917918359213,7.17303617034655));
#96990=CARTESIAN_POINT('Origin',(0.0519544797057715,2.94642873241194,-0.185783815546355));
#96991=CARTESIAN_POINT('Ctrl Pts',(-2.11596138347576,2.87870320309923,6.9343498203138));
#96992=CARTESIAN_POINT('Ctrl Pts',(-2.12838275208153,2.88555248752913,6.97406187955045));
#96993=CARTESIAN_POINT('Ctrl Pts',(-2.14079590348602,2.89224022492635,7.01382974697511));
#96994=CARTESIAN_POINT('Ctrl Pts',(-2.16558061665956,2.9053018965811,7.09337985114029));
#96995=CARTESIAN_POINT('Ctrl Pts',(-2.17796571374631,2.91168295872474,7.13320554516882));
#96996=CARTESIAN_POINT('Ctrl Pts',(-2.19033154210413,2.9179183592551,7.17303615867629));
#96997=CARTESIAN_POINT('Ctrl Pts',(-2.75289164401948,3.0130934341647,6.97712417439583));
#96998=CARTESIAN_POINT('Ctrl Pts',(-2.73970193875433,3.01082632758236,6.98227083876427));
#96999=CARTESIAN_POINT('Ctrl Pts',(-2.72651223348926,3.008559221,6.98741750313253));
#97000=CARTESIAN_POINT('Ctrl Pts',(-2.34398340131143,2.942808424,7.13668145337599));
#97001=CARTESIAN_POINT('Ctrl Pts',(-1.94744645126371,2.877933005,7.24329515157678));
#97002=CARTESIAN_POINT('Ctrl Pts',(-2.88112192756206,3.0130934341647,6.65299824119357));
#97003=CARTESIAN_POINT('Ctrl Pts',(-2.86854313178099,3.01082632758236,6.65838926409685));
#97004=CARTESIAN_POINT('Ctrl Pts',(-2.855964336,3.008559221,6.663780287));
#97005=CARTESIAN_POINT('Ctrl Pts',(-2.491153147,2.942808424,6.820131142));
#97006=CARTESIAN_POINT('Ctrl Pts',(-2.111454323,2.877933005,6.935723513));
#97007=CARTESIAN_POINT('',(-2.7267792535095,3.00855922016357,6.98674995484222));
#97008=CARTESIAN_POINT('Origin',(0.0809638181095518,3.08925204475167,-0.171837215531635));
#97009=CARTESIAN_POINT('',(-2.79137180550544,3.00855921853322,6.82526511527211));
#97010=CARTESIAN_POINT('Origin',(-1.18069616583671E-13,3.10034167700022,
4.57099635919889E-13));
#97011=CARTESIAN_POINT('',(-2.19083234810381,3.09925366546078,7.17288321534975));
#97012=CARTESIAN_POINT('Origin',(0.0548153802264575,3.08928542089756,-0.18492601784178));
#97013=CARTESIAN_POINT('Origin',(0.0785761698327736,2.94644891567482,-0.173890755843731));
#97014=CARTESIAN_POINT('Ctrl Pts',(-3.89967704495,2.877925369,6.40941620005));
#97015=CARTESIAN_POINT('Ctrl Pts',(-3.55137687838,2.943232886,6.62133224987));
#97016=CARTESIAN_POINT('Ctrl Pts',(-3.18216370068,3.008559221,6.79425722689));
#97017=CARTESIAN_POINT('Ctrl Pts',(-3.896326377,2.877925369,6.408481939));
#97018=CARTESIAN_POINT('Ctrl Pts',(-3.54807698,2.943232886,6.620215907));
#97019=CARTESIAN_POINT('Ctrl Pts',(-3.178934004,3.008559221,6.792965376));
#97020=CARTESIAN_POINT('Ctrl Pts',(-3.561259582,2.877925369,6.315055834));
#97021=CARTESIAN_POINT('Ctrl Pts',(-3.218087142,2.943232886,6.50858162000001));
#97022=CARTESIAN_POINT('Ctrl Pts',(-2.855964336,3.008559221,6.663780287));
#97023=CARTESIAN_POINT('',(-3.17893401143054,3.00855922118749,6.79296537808149));
#97024=CARTESIAN_POINT('',(-3.0174491728329,3.00855922150568,6.72837283022954));
#97025=CARTESIAN_POINT('',(-3.68111355336686,2.91791835921217,6.5344780342737));
#97026=CARTESIAN_POINT('Origin',(0.0906779232219468,2.94642872914588,-0.170271772116001));
#97027=CARTESIAN_POINT('Ctrl Pts',(-3.55717161529236,2.8787032030457,6.31735942487094));
#97028=CARTESIAN_POINT('Ctrl Pts',(-3.57783949806911,2.88555248749211,6.35347281116653));
#97029=CARTESIAN_POINT('Ctrl Pts',(-3.59851135292373,2.89224022489924,6.38964246730138));
#97030=CARTESIAN_POINT('Ctrl Pts',(-3.6398175358269,2.90530189702292,6.4620047559652));
#97031=CARTESIAN_POINT('Ctrl Pts',(-3.66047442494779,2.91168295963675,6.49823692039235));
#97032=CARTESIAN_POINT('Ctrl Pts',(-3.68111354879359,2.91791835926664,6.53447802340237));
#97033=CARTESIAN_POINT('Ctrl Pts',(-4.1884060227692,3.01309343424243,6.22221256008111));
#97034=CARTESIAN_POINT('Ctrl Pts',(-4.17663106600069,3.01082632762121,6.23007429516647));
#97035=CARTESIAN_POINT('Ctrl Pts',(-4.16485610923219,3.008559221,6.23793603025165));
#97036=CARTESIAN_POINT('Ctrl Pts',(-3.82335792607495,2.942808424,6.4659426633839));
#97037=CARTESIAN_POINT('Ctrl Pts',(-3.45901058280773,2.877933005,6.65530751471446));
#97038=CARTESIAN_POINT('Ctrl Pts',(-4.24396085829933,3.01309343424242,5.87809879068148));
#97039=CARTESIAN_POINT('Ctrl Pts',(-4.23283505814969,3.01082632762121,5.88606784384073));
#97040=CARTESIAN_POINT('Ctrl Pts',(-4.221709258,3.008559221,5.894036897));
#97041=CARTESIAN_POINT('Ctrl Pts',(-3.899037964,2.942808424,6.125155977));
#97042=CARTESIAN_POINT('Ctrl Pts',(-3.553065231,2.877933005,6.31966988600001));
#97043=CARTESIAN_POINT('',(-4.16497338333524,3.00855922016357,6.23722668743309));
#97044=CARTESIAN_POINT('Origin',(0.116010787647586,3.08925205701893,-0.150414833038365));
#97045=CARTESIAN_POINT('',(-4.19334132994663,3.00855921853322,6.0656317843953));
#97046=CARTESIAN_POINT('Origin',(-1.18720137887163E-12,3.10034167699922,
1.91296631313342E-12));
#97047=CARTESIAN_POINT('',(-3.68156976764921,3.09925366549505,6.53422099774608));
#97048=CARTESIAN_POINT('Origin',(0.0932874242518589,3.08928540831311,-0.16881882010959));
#97049=CARTESIAN_POINT('Origin',(0.114120485973642,2.94644892506214,-0.152933755915976));
#97050=CARTESIAN_POINT('Ctrl Pts',(-5.1863397847,2.877925369,5.42125231998));
#97051=CARTESIAN_POINT('Ctrl Pts',(-4.89173836931,2.943232886,5.70308813079));
#97052=CARTESIAN_POINT('Ctrl Pts',(-4.56833094893001,3.008559221,5.95134013681));
#97053=CARTESIAN_POINT('Ctrl Pts',(-5.182866615,2.877925369,5.421060196));
#97054=CARTESIAN_POINT('Ctrl Pts',(-4.88827564,2.943232886,5.70270726800001));
#97055=CARTESIAN_POINT('Ctrl Pts',(-4.564899051,3.008559221,5.950772778));
#97056=CARTESIAN_POINT('Ctrl Pts',(-4.835549645,2.877925369,5.401847798));
#97057=CARTESIAN_POINT('Ctrl Pts',(-4.542002709,2.943232886,5.664620989));
#97058=CARTESIAN_POINT('Ctrl Pts',(-4.221709258,3.008559221,5.894036897));
#97059=CARTESIAN_POINT('',(-4.56489905631851,3.00855922118773,5.95077277945273));
#97060=CARTESIAN_POINT('',(-4.39330415699359,3.00855922150568,5.92240483565023));
#97061=CARTESIAN_POINT('',(-4.9997707835736,2.91791835921264,5.59037496809944));
#97062=CARTESIAN_POINT('Origin',(0.125161223023473,2.94642873590838,-0.146797725607164));
#97063=CARTESIAN_POINT('Ctrl Pts',(-4.83205245536977,2.87870320302285,5.40497632402961));
#97064=CARTESIAN_POINT('Ctrl Pts',(-4.86000044535219,2.88555248748605,5.43580241560536));
#97065=CARTESIAN_POINT('Ctrl Pts',(-4.88796441085964,2.89224022491598,5.46668260764667));
#97066=CARTESIAN_POINT('Ctrl Pts',(-4.94386062906873,2.90530189649512,5.52847349533871));
#97067=CARTESIAN_POINT('Ctrl Pts',(-4.97182341329659,2.91168295853286,5.55941794837993));
#97068=CARTESIAN_POINT('Ctrl Pts',(-4.99977077667311,2.91791835925263,5.59037495841998));
#97069=CARTESIAN_POINT('Ctrl Pts',(-5.42807519061426,3.01309343423535,5.17635720193932));
#97070=CARTESIAN_POINT('Ctrl Pts',(-5.41826556645109,3.01082632761767,5.18656640164015));
#97071=CARTESIAN_POINT('Ctrl Pts',(-5.40845594228794,3.008559221,5.1967756013411));
#97072=CARTESIAN_POINT('Ctrl Pts',(-5.12395648294645,2.942808424,5.49286358054539));
#97073=CARTESIAN_POINT('Ctrl Pts',(-4.80883522363903,2.877933005,5.75612509561966));
#97074=CARTESIAN_POINT('Ctrl Pts',(-5.40835689648362,3.01309343423534,4.82834597343307));
#97075=CARTESIAN_POINT('Ctrl Pts',(-5.39920432224181,3.01082632761767,4.83852043271648));
#97076=CARTESIAN_POINT('Ctrl Pts',(-5.390051748,3.008559221,4.848694892));
#97077=CARTESIAN_POINT('Ctrl Pts',(-5.1246081,2.942808424,5.143775327));
#97078=CARTESIAN_POINT('Ctrl Pts',(-4.828538757,2.877933005,5.408115519));
#97079=CARTESIAN_POINT('',(-5.40841798704712,3.00855922016356,5.19605763176611));
#97080=CARTESIAN_POINT('Origin',(0.145633308193763,3.08925205901162,-0.121959380627193));
#97081=CARTESIAN_POINT('',(-5.39923487480588,3.00855921853322,5.02237625242081));
#97082=CARTESIAN_POINT('Origin',(4.34981911601184E-13,3.10034167700033,
-3.37837396946483E-13));
#97083=CARTESIAN_POINT('',(-5.00016107681818,3.09925366546916,5.59002586821102));
#97084=CARTESIAN_POINT('Origin',(0.127397609977411,3.08928538692933,-0.144818061837442));
#97085=CARTESIAN_POINT('Origin',(0.144328720891362,2.94644890452984,-0.12482579074787));
#97086=CARTESIAN_POINT('Ctrl Pts',(-6.23049503990001,2.877925369,4.17959670742));
#97087=CARTESIAN_POINT('Ctrl Pts',(-6.00336761087,2.943232886,4.51817394899));
#97088=CARTESIAN_POINT('Ctrl Pts',(-5.74088811843,3.008559221,4.83014499667001));
#97089=CARTESIAN_POINT('Ctrl Pts',(-6.22706177,2.877925369,4.180155704));
#97090=CARTESIAN_POINT('Ctrl Pts',(-5.999903964,2.943232886,4.518546375));
#97091=CARTESIAN_POINT('Ctrl Pts',(-5.737414491,3.008559221,4.83032865900001));
#97092=CARTESIAN_POINT('Ctrl Pts',(-5.88373478,2.877925369,4.236055362));
#97093=CARTESIAN_POINT('Ctrl Pts',(-5.653539277,2.943232886,4.555788976));
#97094=CARTESIAN_POINT('Ctrl Pts',(-5.390051748,3.008559221,4.848694892));
#97095=CARTESIAN_POINT('',(-5.73741449864667,3.00855922118759,4.83032865776541));
#97096=CARTESIAN_POINT('',(-5.56373312153765,3.00855922150568,4.83951177315742));
#97097=CARTESIAN_POINT('',(-6.0846442887004,2.91791835921996,4.384872182072));
#97098=CARTESIAN_POINT('Origin',(0.153792080298203,2.94642869722729,-0.116459622361765));
#97099=CARTESIAN_POINT('Ctrl Pts',(-5.88099189403477,2.8787032030517,4.23986253723746));
#97100=CARTESIAN_POINT('Ctrl Pts',(-5.91491317388903,2.88555248749573,4.2639599403647));
#97101=CARTESIAN_POINT('Ctrl Pts',(-5.9488616857871,2.89224022491036,4.28810674482912));
#97102=CARTESIAN_POINT('Ctrl Pts',(-6.01673429743481,2.90530189681822,4.33643696279344));
#97103=CARTESIAN_POINT('Ctrl Pts',(-6.05069547196218,2.91168295920914,4.36064678124216));
#97104=CARTESIAN_POINT('Ctrl Pts',(-6.08464427990727,2.91791835926124,4.3848721740921));
#97105=CARTESIAN_POINT('Ctrl Pts',(-6.41393359534823,3.01309343428173,3.88846113385415));
#97106=CARTESIAN_POINT('Ctrl Pts',(-6.40654799083191,3.01082632764086,3.90054042749791));
#97107=CARTESIAN_POINT('Ctrl Pts',(-6.39916238631558,3.008559221,3.91261972114173));
#97108=CARTESIAN_POINT('Ctrl Pts',(-6.18496452966363,2.942808424,4.26294430224455));
#97109=CARTESIAN_POINT('Ctrl Pts',(-5.93380407381153,2.877933005,4.58779266509604));
#97110=CARTESIAN_POINT('Ctrl Pts',(-6.31986417743961,3.01309343428173,3.55282506371949));
#97111=CARTESIAN_POINT('Ctrl Pts',(-6.31311279321987,3.01082632764086,3.56472918285974));
#97112=CARTESIAN_POINT('Ctrl Pts',(-6.306361409,3.008559221,3.576633302));
#97113=CARTESIAN_POINT('Ctrl Pts',(-6.110557257,2.942808424,3.921877459));
#97114=CARTESIAN_POINT('Ctrl Pts',(-5.87823517799999,2.877933005,4.243683681));
#97115=CARTESIAN_POINT('',(-6.39897097620884,3.00855922016355,3.91192669654753));
#97116=CARTESIAN_POINT('Origin',(0.168446060194178,3.08925205243713,-0.0878011240636639));
#97117=CARTESIAN_POINT('',(-6.35266619768326,3.00855921853322,3.74427998846434));
#97118=CARTESIAN_POINT('Origin',(-8.53050269311595E-13,3.10034167700022,
5.52509427098613E-13));
#97119=CARTESIAN_POINT('',(-6.08495041118462,3.09925366547201,4.38444734227687));
#97120=CARTESIAN_POINT('Origin',(0.155550450068147,3.08928541145801,-0.114045366557798));
#97121=CARTESIAN_POINT('Origin',(0.167788296014985,2.94644889903272,-0.0908810507973845));
#97122=CARTESIAN_POINT('Ctrl Pts',(-6.98331927221,2.877925369,2.7425077969));
#97123=CARTESIAN_POINT('Ctrl Pts',(-6.83428605413999,2.943232886,3.12199497441));
#97124=CARTESIAN_POINT('Ctrl Pts',(-6.64500774098,3.008559221,3.48309764438));
#97125=CARTESIAN_POINT('Ctrl Pts',(-6.980086438,2.877925369,2.743791776));
#97126=CARTESIAN_POINT('Ctrl Pts',(-6.830983446,2.943232886,3.123103275));
#97127=CARTESIAN_POINT('Ctrl Pts',(-6.641654807,3.008559221,3.48402374));
#97128=CARTESIAN_POINT('Ctrl Pts',(-6.656803017,2.877925369,2.872189686));
#97129=CARTESIAN_POINT('Ctrl Pts',(-6.500722632,2.943232886,3.233933334));
#97130=CARTESIAN_POINT('Ctrl Pts',(-6.306361409,3.008559221,3.576633302));
#97131=CARTESIAN_POINT('',(-6.64165481419034,3.00855922118751,3.48402373714726));
#97132=CARTESIAN_POINT('',(-6.4740081094864,3.00855922150568,3.5303285182742));
#97133=CARTESIAN_POINT('',(-6.88500659019446,2.91791835923352,2.97433764536223));
#97134=CARTESIAN_POINT('Origin',(0.175232140451512,2.94642872746011,-0.0806762294130415));
#97135=CARTESIAN_POINT('Ctrl Pts',(-6.65494268860888,2.87870320306324,2.87649749093035));
#97136=CARTESIAN_POINT('Ctrl Pts',(-6.69325113712358,2.88555248753272,2.89273943758659));
#97137=CARTESIAN_POINT('Ctrl Pts',(-6.73159680084652,2.89224022496146,2.90902377651066));
#97138=CARTESIAN_POINT('Ctrl Pts',(-6.80827217211815,2.90530189949898,2.94163346192576));
#97139=CARTESIAN_POINT('Ctrl Pts',(-6.84664376590286,2.91168296458449,2.95797662692451));
#97140=CARTESIAN_POINT('Ctrl Pts',(-6.8850065803265,2.91791835932858,2.97433763934861));
#97141=CARTESIAN_POINT('Ctrl Pts',(-7.09988359430054,3.01309343433985,2.4187449445366));
#97142=CARTESIAN_POINT('Ctrl Pts',(-7.09526735214123,3.01082632766993,2.4321295178125));
#97143=CARTESIAN_POINT('Ctrl Pts',(-7.09065110998202,3.008559221,2.44551409108841));
#97144=CARTESIAN_POINT('Ctrl Pts',(-6.95677051003518,2.942808424,2.83369448509874));
#97145=CARTESIAN_POINT('Ctrl Pts',(-6.78131484154021,2.877933005,3.20494014832406));
#97146=CARTESIAN_POINT('Ctrl Pts',(-6.93586163283426,3.01309343433985,2.11117800370404));
#97147=CARTESIAN_POINT('Ctrl Pts',(-6.9318271259172,3.01082632766993,2.12425515935203));
#97148=CARTESIAN_POINT('Ctrl Pts',(-6.92779261899999,3.008559221,2.137332315));
#97149=CARTESIAN_POINT('Ctrl Pts',(-6.810783548,2.942808424,2.51659696));
#97150=CARTESIAN_POINT('Ctrl Pts',(-6.653071856,2.877933005,2.880821911));
#97151=CARTESIAN_POINT('',(-7.09031519513093,3.00855922016356,2.44487841651762));
#97152=CARTESIAN_POINT('Origin',(0.183382530523761,3.08925209210665,-0.0495374482622934));
#97153=CARTESIAN_POINT('',(-7.00905390970135,3.00855921853322,2.29110535411744));
#97154=CARTESIAN_POINT('Origin',(-7.01261965163624E-13,3.10034167699956,
2.68014777038417E-13));
#97155=CARTESIAN_POINT('',(-6.88521422698715,3.09925366552651,2.97385693108467));
#97156=CARTESIAN_POINT('Origin',(0.176430221718098,3.08928538933908,-0.0779403288848335));
#97157=CARTESIAN_POINT('Origin',(0.183402201308652,2.94644894544234,-0.0526867791533125));
#97158=CARTESIAN_POINT('Ctrl Pts',(-7.40961125679,2.877925369,1.17718227082));
#97159=CARTESIAN_POINT('Ctrl Pts',(-7.34564087914,2.943232886,1.57983498574));
#97160=CARTESIAN_POINT('Ctrl Pts',(-7.23841418707,3.008559221,1.97318451829));
#97161=CARTESIAN_POINT('Ctrl Pts',(-7.406730022,2.877925369,1.179131195));
#97162=CARTESIAN_POINT('Ctrl Pts',(-7.342653736,2.943232886,1.581627338));
#97163=CARTESIAN_POINT('Ctrl Pts',(-7.235338726,3.008559221,1.974809744));
#97164=CARTESIAN_POINT('Ctrl Pts',(-7.118606543,2.877925369,1.374023613));
#97165=CARTESIAN_POINT('Ctrl Pts',(-7.043939422,2.943232886,1.760862564));
#97166=CARTESIAN_POINT('Ctrl Pts',(-6.92779261900001,3.008559221,2.137332315));
#97167=CARTESIAN_POINT('',(-7.23533873110783,3.00855922118775,1.97480974195313));
#97168=CARTESIAN_POINT('',(-7.08156567336568,3.00855922150568,2.05607102651839));
#97169=CARTESIAN_POINT('',(-7.36343363499263,2.91791835920902,1.42472638692165));
#97170=CARTESIAN_POINT('Origin',(0.18847804656132,2.94642872398803,-0.0411202707498361));
#97171=CARTESIAN_POINT('Ctrl Pts',(-7.11771575797658,2.87870320295267,1.37863061942183));
#97172=CARTESIAN_POINT('Ctrl Pts',(-7.15862011480401,2.88555248745624,1.38625765429204));
#97173=CARTESIAN_POINT('Ctrl Pts',(-7.19956992987178,2.89224022491387,1.39391809020301));
#97174=CARTESIAN_POINT('Ctrl Pts',(-7.28146277411364,2.90530189659957,1.40928243761697));
#97175=CARTESIAN_POINT('Ctrl Pts',(-7.32245053844715,2.91168295872708,1.41699474627592));
#97176=CARTESIAN_POINT('Ctrl Pts',(-7.36343362367443,2.91791835925492,1.42472638344372));
#97177=CARTESIAN_POINT('Ctrl Pts',(-7.45385092630109,3.01309343452991,0.835930928663964));
#97178=CARTESIAN_POINT('Ctrl Pts',(-7.45221989688324,3.01082632776496,0.849994934267147));
#97179=CARTESIAN_POINT('Ctrl Pts',(-7.45058886746543,3.008559221,0.864058939870347));
#97180=CARTESIAN_POINT('Ctrl Pts',(-7.40328563243026,2.942808424,1.27194426389399));
#97181=CARTESIAN_POINT('Ctrl Pts',(-7.31173886264471,2.877933005,1.67222819236713));
#97182=CARTESIAN_POINT('Ctrl Pts',(-7.22754590703971,3.01309343452991,0.57081460535899));
#97183=CARTESIAN_POINT('Ctrl Pts',(-7.22641692651976,3.01082632776496,0.584453324679495));
#97184=CARTESIAN_POINT('Ctrl Pts',(-7.225287946,3.008559221,0.598092044));
#97185=CARTESIAN_POINT('Ctrl Pts',(-7.19254517,2.942808424,0.993643183999999));
#97186=CARTESIAN_POINT('Ctrl Pts',(-7.116818287,2.877933005,1.38325611));
#97187=CARTESIAN_POINT('',(-7.45012415486043,3.00855922016356,0.863510338789426));
#97188=CARTESIAN_POINT('Origin',(0.189743965845582,3.08925208532173,-0.00895742294459656));
#97189=CARTESIAN_POINT('',(-7.3377060504996,3.00855921853322,0.730801179443037));
#97190=CARTESIAN_POINT('Origin',(-6.75241113023972E-13,3.10034167700089,
9.92044987824237E-14));
#97191=CARTESIAN_POINT('',(-7.363533078059,3.09925366545442,1.42421227530059));
#97192=CARTESIAN_POINT('Origin',(0.189060473729974,3.08928542070922,-0.0381908852368218));
#97193=CARTESIAN_POINT('Origin',(0.190440410096412,2.94644894857135,-0.0120289264421042));
#97194=CARTESIAN_POINT('Ctrl Pts',(-7.48943805504001,2.877925369,-0.44318699073));
#97195=CARTESIAN_POINT('Ctrl Pts',(-7.51352169964,2.943232886,-0.0361963315300001));
#97196=CARTESIAN_POINT('Ctrl Pts',(-7.49336043001001,3.008559221,0.37100747594));
#97197=CARTESIAN_POINT('Ctrl Pts',(-7.487043143,2.877925369,-0.440664251));
#97198=CARTESIAN_POINT('Ctrl Pts',(-7.510989697,2.943232886,-0.033803736));
#97199=CARTESIAN_POINT('Ctrl Pts',(-7.49070624700001,3.008559221,0.373255838));
#97200=CARTESIAN_POINT('Ctrl Pts',(-7.24755193900001,2.877925369,-0.188390278));
#97201=CARTESIAN_POINT('Ctrl Pts',(-7.257789433,2.943232886,0.205455817));
#97202=CARTESIAN_POINT('Ctrl Pts',(-7.225287946,3.008559221,0.598092044));
#97203=CARTESIAN_POINT('',(-7.4907062523096,3.00855922118742,0.373255832402714));
#97204=CARTESIAN_POINT('',(-7.35799709670449,3.00855922150568,0.485673937902005));
#97205=CARTESIAN_POINT('',(-7.49755470732808,2.91791835920472,-0.191503494391312));
#97206=CARTESIAN_POINT('Origin',(0.192911317041647,2.9464287636347,0.00035828858451639));
#97207=CARTESIAN_POINT('Ctrl Pts',(-7.24767235082839,2.87870320304189,-0.18369948845923));
#97208=CARTESIAN_POINT('Ctrl Pts',(-7.28925997327148,2.88555248749686,-0.185043996982772));
#97209=CARTESIAN_POINT('Ctrl Pts',(-7.33089917141281,2.89224022490725,-0.186365657539663));
#97210=CARTESIAN_POINT('Ctrl Pts',(-7.4141802834907,2.90530189604263,-0.188965060643359));
#97211=CARTESIAN_POINT('Ctrl Pts',(-7.45586769143985,2.91168295765171,-0.190244219085969));
#97212=CARTESIAN_POINT('Ctrl Pts',(-7.49755469545811,2.9179183592416,-0.191503495366743));
#97213=CARTESIAN_POINT('Ctrl Pts',(-7.45928447425713,3.0130934343785,-0.785970285244055));
#97214=CARTESIAN_POINT('Ctrl Pts',(-7.46071492280142,3.01082632768925,-0.771884465656615));
#97215=CARTESIAN_POINT('Ctrl Pts',(-7.46214537134582,3.008559221,-0.757798646069158));
#97216=CARTESIAN_POINT('Ctrl Pts',(-7.5036313465345,2.942808424,-0.349280657629427));
#97217=CARTESIAN_POINT('Ctrl Pts',(-7.50027410223868,2.877933005,0.0613247039030384));
#97218=CARTESIAN_POINT('Ctrl Pts',(-7.18127816733622,3.0130934343785,-0.996239447247901));
#97219=CARTESIAN_POINT('Ctrl Pts',(-7.18310750316813,3.01082632768925,-0.982676896623952));
#97220=CARTESIAN_POINT('Ctrl Pts',(-7.184936839,3.008559221,-0.969114346));
#97221=CARTESIAN_POINT('Ctrl Pts',(-7.237991373,2.942808424,-0.575772243));
#97222=CARTESIAN_POINT('Ctrl Pts',(-7.247790206,2.877933005,-0.178989209));
#97223=CARTESIAN_POINT('',(-7.46157359058,3.00855922016356,-0.75823452133945));
#97224=CARTESIAN_POINT('Origin',(0.187233646271958,3.08925209820063,0.0320413507772142));
#97225=CARTESIAN_POINT('',(-7.32325521222774,3.00855921853322,-0.863674445527309));
#97226=CARTESIAN_POINT('Origin',(1.72604985859692E-12,3.10034167700011,
6.96328845278815E-14));
#97227=CARTESIAN_POINT('',(-7.49754130651673,3.09925366544336,-0.192026963734092));
#97228=CARTESIAN_POINT('Origin',(0.192850144087738,3.08928539902374,0.00334440390494479));
#97229=CARTESIAN_POINT('Origin',(0.188574042439491,2.94644890795088,0.0291913744015247));
#97230=CARTESIAN_POINT('Ctrl Pts',(-7.21906705286,2.877925369,-2.04283331976));
#97231=CARTESIAN_POINT('Ctrl Pts',(-7.3300785955,2.943232886,-1.6505351487));
#97232=CARTESIAN_POINT('Ctrl Pts',(-7.39792546831,3.008559221,-1.24851746249));
#97233=CARTESIAN_POINT('Ctrl Pts',(-7.21727044700001,2.877925369,-2.039854725));
#97234=CARTESIAN_POINT('Ctrl Pts',(-7.328120127,2.943232886,-1.647654185));
#97235=CARTESIAN_POINT('Ctrl Pts',(-7.39581667,3.008559221,-1.245751095));
#97236=CARTESIAN_POINT('Ctrl Pts',(-7.037609861,2.877925369,-1.741995249));
#97237=CARTESIAN_POINT('Ctrl Pts',(-7.132273277,2.943232886,-1.359557815));
#97238=CARTESIAN_POINT('Ctrl Pts',(-7.184936839,3.008559221,-0.969114346));
#97239=CARTESIAN_POINT('',(-7.39581667399582,3.00855922118755,-1.24575110158274));
#97240=CARTESIAN_POINT('',(-7.29037675403373,3.00855922150568,-1.10743272356952));
#97241=CARTESIAN_POINT('',(-7.28109845410024,2.91791835917478,-1.79877888497127));
#97242=CARTESIAN_POINT('Origin',(0.188324448607423,2.94642871267471,0.041820229100854));
#97243=CARTESIAN_POINT('Ctrl Pts',(-7.03873583842746,2.87870320301111,-1.73744001218541));
#97244=CARTESIAN_POINT('Ctrl Pts',(-7.07906213591146,2.88555248744445,-1.74769319633835));
#97245=CARTESIAN_POINT('Ctrl Pts',(-7.11944371485452,2.8922402248462,-1.75793515394807));
#97246=CARTESIAN_POINT('Ctrl Pts',(-7.20021896298775,2.90530189548184,-1.7783767609778));
#97247=CARTESIAN_POINT('Ctrl Pts',(-7.24065675767129,2.91168295656746,-1.78858757293469));
#97248=CARTESIAN_POINT('Ctrl Pts',(-7.2810984424229,2.91791835922825,-1.79877888336987));
#97249=CARTESIAN_POINT('Ctrl Pts',(-7.11593016989708,3.01309343428781,-2.37112040385951));
#97250=CARTESIAN_POINT('Ctrl Pts',(-7.12035521010569,3.01082632764391,-2.35767140730608));
#97251=CARTESIAN_POINT('Ctrl Pts',(-7.12478025031426,3.008559221,-2.34422241075272));
#97252=CARTESIAN_POINT('Ctrl Pts',(-7.25311559847784,2.942808424,-1.95417360356047));
#97253=CARTESIAN_POINT('Ctrl Pts',(-7.33810486053925,2.877933005,-1.55244625908855));
#97254=CARTESIAN_POINT('Ctrl Pts',(-6.79922184224499,3.01309343428781,-2.5167104506348));
#97255=CARTESIAN_POINT('Ctrl Pts',(-6.80392395662256,3.01082632764391,-2.50385823831738));
#97256=CARTESIAN_POINT('Ctrl Pts',(-6.808626071,3.008559221,-2.491006026));
#97257=CARTESIAN_POINT('Ctrl Pts',(-6.944997145,2.942808424,-2.1182652));
#97258=CARTESIAN_POINT('Ctrl Pts',(-7.039863509,2.877933005,-1.732865192));
#97259=CARTESIAN_POINT('',(-7.12412813718847,3.00855922016357,-2.34452517951831));
#97260=CARTESIAN_POINT('Origin',(0.175968387386487,3.08925208219559,0.0715419718021096));
#97261=CARTESIAN_POINT('',(-6.96637709903875,3.00855921853322,-2.417765613795));
#97262=CARTESIAN_POINT('Origin',(2.5804011705155E-13,3.10034167700044,4.06575814682064E-14));
#97263=CARTESIAN_POINT('',(-7.28097283641159,3.09925366542632,-1.79928723503156));
#97264=CARTESIAN_POINT('Origin',(0.187622637445009,3.08928541987947,0.0447233372682446));
#97265=CARTESIAN_POINT('Origin',(0.1778901658128,2.94644891472726,0.0690467906906783));
#97266=CARTESIAN_POINT('Ctrl Pts',(-6.61114049838,2.877925369,-3.54695903503));
#97267=CARTESIAN_POINT('Ctrl Pts',(-6.80388916456,2.943232886,-3.18769677721));
#97268=CARTESIAN_POINT('Ctrl Pts',(-6.95657173252999,3.008559221,-2.80966311266));
#97269=CARTESIAN_POINT('Ctrl Pts',(-6.610026206,2.877925369,-3.543663861));
#97270=CARTESIAN_POINT('Ctrl Pts',(-6.80259580600001,2.943232886,-3.184462156));
#97271=CARTESIAN_POINT('Ctrl Pts',(-6.955106924,3.008559221,-2.806508092));
#97272=CARTESIAN_POINT('Ctrl Pts',(-6.498596968,2.877925369,-3.214146458));
#97273=CARTESIAN_POINT('Ctrl Pts',(-6.67325995,2.943232886,-2.861000035));
#97274=CARTESIAN_POINT('Ctrl Pts',(-6.80862607100001,3.008559221,-2.491006026));
#97275=CARTESIAN_POINT('',(-6.95510692647804,3.00855922118749,-2.8065080993318));
#97276=CARTESIAN_POINT('',(-6.88186649638477,3.00855922150568,-2.64875706189753));
#97277=CARTESIAN_POINT('',(-6.72418612977475,2.91791835923578,-3.32194537401143));
#97278=CARTESIAN_POINT('Origin',(0.174931003159876,2.94642873441672,0.081326479956936));
#97279=CARTESIAN_POINT('Ctrl Pts',(-6.50067586169062,2.87870320298644,-3.2099397714576));
#97280=CARTESIAN_POINT('Ctrl Pts',(-6.5378552213195,2.88555248745678,-3.22862220385387));
#97281=CARTESIAN_POINT('Ctrl Pts',(-6.57509098335056,2.89224022488905,-3.24730555608538));
#97282=CARTESIAN_POINT('Ctrl Pts',(-6.64958341887247,2.90530189713171,-3.28463354502223));
#97283=CARTESIAN_POINT('Ctrl Pts',(-6.68688078783159,2.91168295985056,-3.30329856955462));
#97284=CARTESIAN_POINT('Ctrl Pts',(-6.72418611854397,2.91791835926929,-3.3219453699723));
#97285=CARTESIAN_POINT('Ctrl Pts',(-6.43984287988421,3.01309343442669,-3.84539956829271));
#97286=CARTESIAN_POINT('Ctrl Pts',(-6.44705560205367,3.01082632771334,-3.8332162542701));
#97287=CARTESIAN_POINT('Ctrl Pts',(-6.45426832422315,3.008559221,-3.82103294024745));
#97288=CARTESIAN_POINT('Ctrl Pts',(-6.66345222738474,2.942808424,-3.46769156360501));
#97289=CARTESIAN_POINT('Ctrl Pts',(-6.8328139904108,2.877933005,-3.0936265599123));
#97290=CARTESIAN_POINT('Ctrl Pts',(-6.09924145999368,3.01309343442668,-3.91950287199552));
#97291=CARTESIAN_POINT('Ctrl Pts',(-6.1065964874969,3.01082632771334,-3.90796195249775));
#97292=CARTESIAN_POINT('Ctrl Pts',(-6.113951515,3.008559221,-3.896421033));
#97293=CARTESIAN_POINT('Ctrl Pts',(-6.327262568,2.942808424,-3.56171043));
#97294=CARTESIAN_POINT('Ctrl Pts',(-6.502760619,2.877933005,-3.205714324));
#97295=CARTESIAN_POINT('',(-6.45356637077136,3.00855922016357,-3.82118844541768));
#97296=CARTESIAN_POINT('Origin',(0.156474692526415,3.08925205823525,0.107697219502322));
#97297=CARTESIAN_POINT('',(-6.28375893558174,3.00855921853322,-3.85880474889426));
#97298=CARTESIAN_POINT('Origin',(1.22471477403963E-12,3.10034167700033,
6.61580165650655E-13));
#97299=CARTESIAN_POINT('',(-6.72395416877963,3.09925366545874,-3.32241483495412));
#97300=CARTESIAN_POINT('Origin',(0.1736215916407,3.08928536449683,0.0840108764691233));
#97301=CARTESIAN_POINT('Origin',(0.158887925882241,2.94644891559956,0.105673502394065));
#97302=CARTESIAN_POINT('Ctrl Pts',(-5.69408436183001,2.877925369,-4.88523288661));
#97303=CARTESIAN_POINT('Ctrl Pts',(-5.95955743762001,2.943232886,-4.57580524642));
#97304=CARTESIAN_POINT('Ctrl Pts',(-6.18993643594999,3.008559221,-4.23943203857));
#97305=CARTESIAN_POINT('Ctrl Pts',(-5.693704486,2.877925369,-4.88177521199999));
#97306=CARTESIAN_POINT('Ctrl Pts',(-5.958989665,2.943232886,-4.572368215));
#97307=CARTESIAN_POINT('Ctrl Pts',(-6.18918411,3.008559221,-4.23603589));
#97308=CARTESIAN_POINT('Ctrl Pts',(-5.65571690300001,2.877925369,-4.536007751));
#97309=CARTESIAN_POINT('Ctrl Pts',(-5.902212403,2.943232886,-4.228665073));
#97310=CARTESIAN_POINT('Ctrl Pts',(-6.113951515,3.008559221,-3.896421033));
#97311=CARTESIAN_POINT('',(-6.18918411085223,3.00855922118745,-4.23603589763653));
#97312=CARTESIAN_POINT('',(-6.15156781078797,3.00855922150568,-4.06622846409005));
#97313=CARTESIAN_POINT('',(-5.85285833527549,2.91791835920682,-4.68978138984361));
#97314=CARTESIAN_POINT('Origin',(0.153358491952596,2.94642875212302,0.117030173352469));
#97315=CARTESIAN_POINT('Ctrl Pts',(-5.65865150674991,2.87870320301381,-4.53234631577129));
#97316=CARTESIAN_POINT('Ctrl Pts',(-5.69094546277738,2.88555248747294,-4.55858442652626));
#97317=CARTESIAN_POINT('Ctrl Pts',(-5.72329430486643,2.89224022489121,-4.58483556042797));
#97318=CARTESIAN_POINT('Ctrl Pts',(-5.78802073411798,2.90530189705154,-4.63730451296399));
#97319=CARTESIAN_POINT('Ctrl Pts',(-5.82043368251407,2.91168295970418,-4.66355099107896));
#97320=CARTESIAN_POINT('Ctrl Pts',(-5.85285832531392,2.91791835926746,-4.6897813835981));
#97321=CARTESIAN_POINT('Ctrl Pts',(-5.46263569397422,3.01309343427872,-5.1398721217525));
#97322=CARTESIAN_POINT('Ctrl Pts',(-5.47229883877705,3.01082632763937,-5.1295241692268));
#97323=CARTESIAN_POINT('Ctrl Pts',(-5.48196198357988,3.008559221,-5.11917621670124));
#97324=CARTESIAN_POINT('Ctrl Pts',(-5.76221323479108,2.942808424,-4.81906412049076));
#97325=CARTESIAN_POINT('Ctrl Pts',(-6.00802833361441,2.877933005,-4.49015232226918));
#97326=CARTESIAN_POINT('Ctrl Pts',(-5.11406732750078,3.01309343427873,-5.13902369378443));
#97327=CARTESIAN_POINT('Ctrl Pts',(-5.12373135475034,3.01082632763937,-5.12933370839221));
#97328=CARTESIAN_POINT('Ctrl Pts',(-5.133395382,3.008559221,-5.119643723));
#97329=CARTESIAN_POINT('Ctrl Pts',(-5.413672226,2.942808424,-4.838614039));
#97330=CARTESIAN_POINT('Ctrl Pts',(-5.66159587,2.877933005,-4.528667818));
#97331=CARTESIAN_POINT('',(-5.48124301243205,3.00855922016357,-5.11917718699627));
#97332=CARTESIAN_POINT('Origin',(0.12966488231818,3.08925206018815,0.138816935313775));
#97333=CARTESIAN_POINT('',(-5.30731918799498,3.00855921853322,-5.11941046289062));
#97334=CARTESIAN_POINT('Origin',(1.8995222061946E-13,3.10034167700033,5.3776427755281E-14));
#97335=CARTESIAN_POINT('',(-5.8525308771641,3.09925366548655,-4.69019001010936));
#97336=CARTESIAN_POINT('Origin',(0.151502844515639,3.08928542269922,0.119370499732209));
#97337=CARTESIAN_POINT('Origin',(0.132456427435822,2.94644893686484,0.137359030828437));
#97338=CARTESIAN_POINT('Ctrl Pts',(-4.51077916970999,2.877925369,-5.99507867818));
#97339=CARTESIAN_POINT('Ctrl Pts',(-4.83656342825001,2.943232886,-5.74995414786));
#97340=CARTESIAN_POINT('Ctrl Pts',(-5.13386659043,3.008559221,-5.47096983334));
#97341=CARTESIAN_POINT('Ctrl Pts',(-4.511151473,2.877925369,-5.99162018));
#97342=CARTESIAN_POINT('Ctrl Pts',(-4.83674779000001,2.943232886,-5.746475418));
#97343=CARTESIAN_POINT('Ctrl Pts',(-5.133861925,3.008559221,-5.46749135700001));
#97344=CARTESIAN_POINT('Ctrl Pts',(-4.548381802,2.877925369,-5.645770362));
#97345=CARTESIAN_POINT('Ctrl Pts',(-4.85518396500001,2.943232886,-5.398602432));
#97346=CARTESIAN_POINT('Ctrl Pts',(-5.13339538200001,3.008559221,-5.119643723));
#97347=CARTESIAN_POINT('',(-5.1338619255737,3.00855922118768,-5.46749136247341));
#97348=CARTESIAN_POINT('',(-5.13362865127121,3.00855922150568,-5.29356754216145));
#97349=CARTESIAN_POINT('',(-4.70785739014204,2.91791835921984,-5.83832843962122));
#97350=CARTESIAN_POINT('Origin',(0.124615097880204,2.94642874656054,0.147261696058592));
#97351=CARTESIAN_POINT('Ctrl Pts',(-4.55203489682575,2.87870320305795,-5.6428253826466));
#97352=CARTESIAN_POINT('Ctrl Pts',(-4.57793341989185,2.88555248751722,-5.67539230694019));
#97353=CARTESIAN_POINT('Ctrl Pts',(-4.60388274619806,2.89224022493592,-5.70798374879017));
#97354=CARTESIAN_POINT('Ctrl Pts',(-4.65581663663197,2.90530189785697,-5.77314027923381));
#97355=CARTESIAN_POINT('Ctrl Pts',(-4.6818295747134,2.91168296129037,-5.80574095935479));
#97356=CARTESIAN_POINT('Ctrl Pts',(-4.70785738175949,2.91791835928726,-5.83832843143792));
#97357=CARTESIAN_POINT('Ctrl Pts',(-4.23000173511302,3.01309343431576,-6.19400996767578));
#97358=CARTESIAN_POINT('Ctrl Pts',(-4.24166346495119,3.01082632765788,-6.18598123495631));
#97359=CARTESIAN_POINT('Ctrl Pts',(-4.25332519478933,3.008559221,-6.17795250223672));
#97360=CARTESIAN_POINT('Ctrl Pts',(-4.59153955651358,2.942808424,-5.94510259489902));
#97361=CARTESIAN_POINT('Ctrl Pts',(-4.90231394849256,2.877933005,-5.67672355131862));
#97362=CARTESIAN_POINT('Ctrl Pts',(-3.88976508856774,3.01309343431575,-6.11824948059964));
#97363=CARTESIAN_POINT('Ctrl Pts',(-3.90128623678383,3.01082632765788,-6.11086352179979));
#97364=CARTESIAN_POINT('Ctrl Pts',(-3.912807385,3.008559221,-6.103477563));
#97365=CARTESIAN_POINT('Ctrl Pts',(-4.246944588,2.942808424,-5.889269433));
#97366=CARTESIAN_POINT('Ctrl Pts',(-4.555701191,2.877933005,-5.639865837));
#97367=CARTESIAN_POINT('',(-4.25262282382441,3.00855922016355,-6.17779889244642));
#97368=CARTESIAN_POINT('Origin',(0.0967918109286592,3.08925206385687,0.163445524649569));
#97369=CARTESIAN_POINT('',(-4.08271509389942,3.00855921853322,-6.14063823337773));
#97370=CARTESIAN_POINT('Origin',(-1.58727198051878E-13,3.10034167699978,
-3.5605199344424E-13));
#97371=CARTESIAN_POINT('',(-4.70744974629859,3.0992536654783,-5.83865711346283));
#97372=CARTESIAN_POINT('Origin',(0.122299545909472,3.08928544800128,0.149148174631047));
#97373=CARTESIAN_POINT('Origin',(0.0998316880435851,2.94644890557194,0.162622073715286));
#97374=CARTESIAN_POINT('Ctrl Pts',(-3.11655495708,2.877925369,-6.82460125420999));
#97375=CARTESIAN_POINT('Ctrl Pts',(-3.48741708843,2.943232886,-6.65524158477));
#97376=CARTESIAN_POINT('Ctrl Pts',(-3.83774284877,3.008559221,-6.44669115942001));
#97377=CARTESIAN_POINT('Ctrl Pts',(-3.117662031,2.877925369,-6.821303648));
#97378=CARTESIAN_POINT('Ctrl Pts',(-3.488344964,2.943232886,-6.65188381800001));
#97379=CARTESIAN_POINT('Ctrl Pts',(-3.838486062,3.008559221,-6.44329300500001));
#97380=CARTESIAN_POINT('Ctrl Pts',(-3.228369423,2.877925369,-6.491543027));
#97381=CARTESIAN_POINT('Ctrl Pts',(-3.581132521,2.943232886,-6.316107141));
#97382=CARTESIAN_POINT('Ctrl Pts',(-3.912807385,3.008559221,-6.103477563));
#97383=CARTESIAN_POINT('',(-3.83848606137266,3.0085592211877,-6.4432930104941));
#97384=CARTESIAN_POINT('',(-3.87564672085867,3.00855922150568,-6.27338528563179));
#97385=CARTESIAN_POINT('',(-3.34272226580324,2.91791835921079,-6.71388174049539));
#97386=CARTESIAN_POINT('Origin',(0.0900447143230324,2.94642872540765,0.170607277916067));
#97387=CARTESIAN_POINT('Ctrl Pts',(-3.23257019413014,2.87870320301883,-6.48945220613886));
#97388=CARTESIAN_POINT('Ctrl Pts',(-3.2508622980708,2.88555248747773,-6.52682515079375));
#97389=CARTESIAN_POINT('Ctrl Pts',(-3.26919874694083,2.89224022490049,-6.56423296099061));
#97390=CARTESIAN_POINT('Ctrl Pts',(-3.30591171996773,2.90530189646074,-6.63903041146088));
#97391=CARTESIAN_POINT('Ctrl Pts',(-3.32430830306973,2.911682958487,-6.67646090970598));
#97392=CARTESIAN_POINT('Ctrl Pts',(-3.34272225937116,2.91791835925212,-6.71388173051157));
#97393=CARTESIAN_POINT('Ctrl Pts',(-2.79957759524227,3.01309343436868,-6.95852279143793));
#97394=CARTESIAN_POINT('Ctrl Pts',(-2.81269262067868,3.01082632768435,-6.95318869316753));
#97395=CARTESIAN_POINT('Ctrl Pts',(-2.82580764611506,3.008559221,-6.9478545948972));
#97396=CARTESIAN_POINT('Ctrl Pts',(-3.20617059112771,2.942808424,-6.79315467937377));
#97397=CARTESIAN_POINT('Ctrl Pts',(-3.56737281165495,2.877933005,-6.59785749655774));
#97398=CARTESIAN_POINT('Ctrl Pts',(-2.48358175878518,3.01309343436869,-6.81139272192371));
#97399=CARTESIAN_POINT('Ctrl Pts',(-2.49642131189258,3.01082632768435,-6.80665614896187));
#97400=CARTESIAN_POINT('Ctrl Pts',(-2.509260865,3.008559221,-6.801919576));
#97401=CARTESIAN_POINT('Ctrl Pts',(-2.881634541,2.942808424,-6.664549134));
#97402=CARTESIAN_POINT('Ctrl Pts',(-3.236786987,2.877933005,-6.487349998));
#97403=CARTESIAN_POINT('',(-2.82515471777632,3.00855922016355,-6.94755358741828));
#97404=CARTESIAN_POINT('Origin',(0.0593929041144048,3.08925206325076,0.180431615768841));
#97405=CARTESIAN_POINT('',(-2.66720777989305,3.00855921853322,-6.87473658497311));
#97406=CARTESIAN_POINT('Origin',(-1.32272665043232E-13,3.10034167700067,
-2.12503625807159E-13));
#97407=CARTESIAN_POINT('',(-3.34225349745923,3.09925366545785,-6.71411509886201));
#97408=CARTESIAN_POINT('Origin',(0.0873777332247544,3.08928540246991,0.171951807331283));
#97409=CARTESIAN_POINT('Origin',(0.0625387623973611,2.94644889145861,0.180280994928028));
#97410=CARTESIAN_POINT('Ctrl Pts',(-1.576604098,2.877925369,-7.33501306085001));
#97411=CARTESIAN_POINT('Ctrl Pts',(-1.97520300205,2.943232886,-7.24933732122));
#97412=CARTESIAN_POINT('Ctrl Pts',(-2.36217051692,3.008559221,-7.12097237258));
#97413=CARTESIAN_POINT('Ctrl Pts',(-1.578394177,2.877925369,-7.332030539));
#97414=CARTESIAN_POINT('Ctrl Pts',(-1.976831005,2.943232886,-7.246257523));
#97415=CARTESIAN_POINT('Ctrl Pts',(-2.363626857,3.008559221,-7.117813434));
#97416=CARTESIAN_POINT('Ctrl Pts',(-1.757402077,2.877925369,-7.033778354));
#97417=CARTESIAN_POINT('Ctrl Pts',(-2.1396313,2.943232886,-6.938277701));
#97418=CARTESIAN_POINT('Ctrl Pts',(-2.509260865,3.008559221,-6.801919576));
#97419=CARTESIAN_POINT('',(-2.36362685520607,3.00855922118764,-7.11781343921217));
#97420=CARTESIAN_POINT('',(-2.43644385806964,3.00855922150568,-6.95986650602584));
#97421=CARTESIAN_POINT('',(-1.82128516328855,2.91791835917736,-7.27550139344267));
#97422=CARTESIAN_POINT('Origin',(0.0512640569840399,2.94642876615184,0.185975714800092));
#97423=CARTESIAN_POINT('Ctrl Pts',(-1.76195410109328,2.87870320313799,-7.03263945803826));
#97424=CARTESIAN_POINT('Ctrl Pts',(-1.77178446761464,2.88555248754599,-7.07307090546907));
#97425=CARTESIAN_POINT('Ctrl Pts',(-1.78165064719965,2.89224022492362,-7.11354593614641));
#97426=CARTESIAN_POINT('Ctrl Pts',(-1.80142604852422,2.90530189501338,-7.19448685877411));
#97427=CARTESIAN_POINT('Ctrl Pts',(-1.81134607668391,2.91168295556601,-7.23499696438467));
#97428=CARTESIAN_POINT('Ctrl Pts',(-1.821285159244,2.91791835921545,-7.27550138225621));
#97429=CARTESIAN_POINT('Ctrl Pts',(-1.23824831937288,3.01309343425735,-7.39766282394084));
#97430=CARTESIAN_POINT('Ctrl Pts',(-1.25220339591637,3.01082632762868,-7.39527277675328));
#97431=CARTESIAN_POINT('Ctrl Pts',(-1.26615847245984,3.008559221,-7.39288272956574));
#97432=CARTESIAN_POINT('Ctrl Pts',(-1.67088465221739,2.942808424,-7.32356640122884));
#97433=CARTESIAN_POINT('Ctrl Pts',(-2.06562528681077,2.877933005,-7.21048295867911));
#97434=CARTESIAN_POINT('Ctrl Pts',(-0.961268906319293,3.01309343425735,
-7.18604280915326));
#97435=CARTESIAN_POINT('Ctrl Pts',(-0.974826500659645,3.01082632762868,
-7.18417709907661));
#97436=CARTESIAN_POINT('Ctrl Pts',(-0.988384095,3.008559221,-7.182311389));
#97437=CARTESIAN_POINT('Ctrl Pts',(-1.381582466,2.942808424,-7.128201925));
#97438=CARTESIAN_POINT('Ctrl Pts',(-1.766524221,2.877933005,-7.031492884));
#97439=CARTESIAN_POINT('',(-1.26558551692927,3.00855922016356,-7.39244839919028));
#97440=CARTESIAN_POINT('Origin',(0.0192169037645398,3.08925205889063,0.188981087051618));
#97441=CARTESIAN_POINT('',(-1.12698479404631,3.00855921853322,-7.28737989481257));
#97442=CARTESIAN_POINT('Origin',(-2.46005472936961E-13,3.10034167699967,
-1.12800394025392E-12));
#97443=CARTESIAN_POINT('',(-1.82077718939073,3.09925366550626,-7.27562852432749));
#97444=CARTESIAN_POINT('Origin',(0.0483703533938834,3.08928542389148,0.186715408607567));
#97445=CARTESIAN_POINT('Origin',(0.0223215694314258,2.94644894993203,0.189510086032583));
#97446=CARTESIAN_POINT('Ctrl Pts',(0.03706701598,2.877925369,-7.50244780807));
#97447=CARTESIAN_POINT('Ctrl Pts',(-0.37063061727,2.943232886,-7.50446210275));
#97448=CARTESIAN_POINT('Ctrl Pts',(-0.77614571692,3.008559221,-7.46228483128));
#97449=CARTESIAN_POINT('Ctrl Pts',(0.034677634,2.877925369,-7.49991983));
#97450=CARTESIAN_POINT('Ctrl Pts',(-0.372882624,2.943232886,-7.501804281));
#97451=CARTESIAN_POINT('Ctrl Pts',(-0.778247087,3.008559221,-7.459512817));
#97452=CARTESIAN_POINT('Ctrl Pts',(-0.204260564,2.877925369,-7.247122023));
#97453=CARTESIAN_POINT('Ctrl Pts',(-0.598083297,2.943232886,-7.23602210600001));
#97454=CARTESIAN_POINT('Ctrl Pts',(-0.988384095,3.008559221,-7.182311389));
#97455=CARTESIAN_POINT('',(-0.88331558791762,3.00855922150568,-7.32091210337191));
#97456=CARTESIAN_POINT('Ctrl Pts',(-0.20895099349809,2.87870320312668,-7.24698830408616));
#97457=CARTESIAN_POINT('Ctrl Pts',(-0.20985996526507,2.88555248754736,-7.2885877250765));
#97458=CARTESIAN_POINT('Ctrl Pts',(-0.21079454375944,2.89224022494082,-7.33023740914598));
#97459=CARTESIAN_POINT('Ctrl Pts',(-0.212707701350711,2.9053018958938,-7.41353711031396));
#97460=CARTESIAN_POINT('Ctrl Pts',(-0.213687329218262,2.91168295475788,
-7.45523261427169));
#97461=CARTESIAN_POINT('Ctrl Pts',(-0.214686788680074,2.91791835670407,
-7.49692665869679));
#97462=CARTESIAN_POINT('Ctrl Pts',(0.363928114147479,3.01031422125333,-7.49137659943433));
#97463=CARTESIAN_POINT('Ctrl Pts',(0.358454361386452,3.00943672112667,-7.49163449536675));
#97464=CARTESIAN_POINT('Ctrl Pts',(0.352980608625425,3.008559221,-7.49189239129917));
#97465=CARTESIAN_POINT('Ctrl Pts',(-0.0571658924187911,2.942808424,-7.51121644902179));
#97466=CARTESIAN_POINT('Ctrl Pts',(-0.466970758802433,2.877933005,-7.48565195769581));
#97467=CARTESIAN_POINT('Ctrl Pts',(0.589268653938478,3.01031422125333,-7.2260206670324));
#97468=CARTESIAN_POINT('Ctrl Pts',(0.583988535469239,3.00943672112667,-7.2264434850162));
#97469=CARTESIAN_POINT('Ctrl Pts',(0.578708417,3.008559221,-7.226866303));
#97470=CARTESIAN_POINT('Ctrl Pts',(0.18307087,2.942808424,-7.258547916));
#97471=CARTESIAN_POINT('Ctrl Pts',(-0.213660746,2.877933005,-7.246850977));
#97472=CARTESIAN_POINT('',(0.465934748101219,3.00855921853322,-7.3592734190439));
#97473=CARTESIAN_POINT('Ctrl Pts',(1.64900491812,2.877925369,-7.31907643485));
#97474=CARTESIAN_POINT('Ctrl Pts',(1.25127204218,2.943232886,-7.40868657547001));
#97475=CARTESIAN_POINT('Ctrl Pts',(0.84617079334,3.008559221,-7.45466914569));
#97476=CARTESIAN_POINT('Ctrl Pts',(1.646127958,2.877925369,-7.317121206));
#97477=CARTESIAN_POINT('Ctrl Pts',(1.248501333,2.943232886,-7.406575007));
#97478=CARTESIAN_POINT('Ctrl Pts',(0.843522651,3.008559221,-7.452413672));
#97479=CARTESIAN_POINT('Ctrl Pts',(1.358431946,2.877925369,-7.121598321));
#97480=CARTESIAN_POINT('Ctrl Pts',(0.971430415,2.943232886,-7.19541816));
#97481=CARTESIAN_POINT('Ctrl Pts',(0.578708417,3.008559221,-7.226866303));
#97482=CARTESIAN_POINT('',(0.843522657377817,3.00855922118756,-7.45241367635266));
#97483=CARTESIAN_POINT('',(0.711115537090266,3.00855922150568,-7.33963998720059));
#97484=CARTESIAN_POINT('',(1.4019500970824,2.91791835924909,-7.3678040214789));
#97485=CARTESIAN_POINT('Origin',(-0.0315631804265319,2.94642870889188,0.190312136075106));
#97486=CARTESIAN_POINT('Ctrl Pts',(1.35382243093574,2.87870320305526,-7.12247603196901));
#97487=CARTESIAN_POINT('Ctrl Pts',(1.36187735611562,2.88555248751697,-7.16329828373009));
#97488=CARTESIAN_POINT('Ctrl Pts',(1.36991807837126,2.89224022494186,-7.20417512809119));
#97489=CARTESIAN_POINT('Ctrl Pts',(1.38595662582573,2.9053018985513,-7.28593861717606));
#97490=CARTESIAN_POINT('Ctrl Pts',(1.39396320871808,2.91168296268184,-7.32686992942572));
#97491=CARTESIAN_POINT('Ctrl Pts',(1.40195009630196,2.91791835930475,-7.36780400971366));
#97492=CARTESIAN_POINT('Ctrl Pts',(1.98239425956791,3.01309343443221,-7.23386391540278));
#97493=CARTESIAN_POINT('Ctrl Pts',(1.96872541981646,3.01082632771611,-7.23755435206928));
#97494=CARTESIAN_POINT('Ctrl Pts',(1.95505658006501,3.008559221,-7.24124478873574));
#97495=CARTESIAN_POINT('Ctrl Pts',(1.55863187657184,2.942808424,-7.34827510644113));
#97496=CARTESIAN_POINT('Ctrl Pts',(1.15289247445925,2.877933005,-7.41139064311515));
#97497=CARTESIAN_POINT('Ctrl Pts',(2.14491702942533,3.01309343443221,-6.92550215463664));
#97498=CARTESIAN_POINT('Ctrl Pts',(2.13182909821269,3.01082632771611,-6.92950156831831));
#97499=CARTESIAN_POINT('Ctrl Pts',(2.118741167,3.008559221,-6.933500982));
#97500=CARTESIAN_POINT('Ctrl Pts',(1.739164016,2.942808424,-7.049492274));
#97501=CARTESIAN_POINT('Ctrl Pts',(1.349193269,2.877933005,-7.123354373));
#97502=CARTESIAN_POINT('',(1.95539420948476,3.00855922016357,-7.24061002354905));
#97503=CARTESIAN_POINT('Origin',(-0.0619102307666214,3.08925202244823,0.179583189245777));
#97504=CARTESIAN_POINT('',(2.03706769954263,3.00855921853322,-7.08705549831994));
#97505=CARTESIAN_POINT('Origin',(-1.95102180938767E-13,3.10034167699989,
6.10188982674842E-13));
#97506=CARTESIAN_POINT('',(1.40246450243754,3.09925366544267,-7.36770610985706));
#97507=CARTESIAN_POINT('Origin',(-0.0345000262589518,3.0892854313886,0.189768554694597));
#97508=CARTESIAN_POINT('Origin',(-0.0593146635395822,2.94644893318334,0.181367007252413));
#97509=CARTESIAN_POINT('Ctrl Pts',(3.1838371828,2.877925369,-6.79347318230001));
#97510=CARTESIAN_POINT('Ctrl Pts',(2.81466661134,2.943232886,-6.96648909860001));
#97511=CARTESIAN_POINT('Ctrl Pts',(2.42892129841,3.008559221,-7.09848141564));
#97512=CARTESIAN_POINT('Ctrl Pts',(3.180607168,2.877925369,-6.792182127));
#97513=CARTESIAN_POINT('Ctrl Pts',(2.811506755,2.943232886,-6.96502251800001));
#97514=CARTESIAN_POINT('Ctrl Pts',(2.425850208,3.008559221,-7.096847946));
#97515=CARTESIAN_POINT('Ctrl Pts',(2.857605688,2.877925369,-6.663076597));
#97516=CARTESIAN_POINT('Ctrl Pts',(2.495521121,2.943232886,-6.818364458));
#97517=CARTESIAN_POINT('Ctrl Pts',(2.118741167,3.008559221,-6.933500982));
#97518=CARTESIAN_POINT('',(2.42585021516617,3.00855922118751,-7.09684794887307));
#97519=CARTESIAN_POINT('',(2.27229569045365,3.00855922150568,-7.01517446304328));
#97520=CARTESIAN_POINT('',(2.9530333567116,2.9179183592309,-6.89417102827685));
#97521=CARTESIAN_POINT('Origin',(-0.071736775555461,2.94642872856476,0.179077716464233));
#97522=CARTESIAN_POINT('Ctrl Pts',(2.85329262188022,2.87870320297217,-6.66492469631897));
#97523=CARTESIAN_POINT('Ctrl Pts',(2.86993480505275,2.88555248745112,-6.70306097574357));
#97524=CARTESIAN_POINT('Ctrl Pts',(2.88657485310286,2.89224022489599,-6.7412536246611));
#97525=CARTESIAN_POINT('Ctrl Pts',(2.9198151589043,2.90530189741744,-6.81765770875573));
#97526=CARTESIAN_POINT('Ctrl Pts',(2.93643357145378,2.91168296040963,-6.85591088368492));
#97527=CARTESIAN_POINT('Ctrl Pts',(2.95303335331849,2.91791835927626,-6.89417101691848));
#97528=CARTESIAN_POINT('Ctrl Pts',(3.49111389256556,3.01309343426058,-6.63858403115588));
#97529=CARTESIAN_POINT('Ctrl Pts',(3.47855795797211,3.01082632763029,-6.64512658367306));
#97530=CARTESIAN_POINT('Ctrl Pts',(3.46600202337865,3.008559221,-6.65166913619008));
#97531=CARTESIAN_POINT('Ctrl Pts',(3.10185386397271,2.942808424,-6.84141673635196));
#97532=CARTESIAN_POINT('Ctrl Pts',(2.71916839817603,2.877933005,-6.99027864620438));
#97533=CARTESIAN_POINT('Ctrl Pts',(3.58354830696306,3.01309343426058,-6.30249400563588));
#97534=CARTESIAN_POINT('Ctrl Pts',(3.57162612048153,3.0108263276303,-6.30921343331795));
#97535=CARTESIAN_POINT('Ctrl Pts',(3.559703934,3.008559221,-6.315932861));
#97536=CARTESIAN_POINT('Ctrl Pts',(3.213935785,2.942808424,-6.510810208));
#97537=CARTESIAN_POINT('Ctrl Pts',(2.848960505,2.877933005,-6.666777635));
#97538=CARTESIAN_POINT('',(3.46619530345603,3.00855922016358,-6.65097663113775));
#97539=CARTESIAN_POINT('Origin',(-0.0990680448027226,3.08925207644981,0.162076097716589));
#97540=CARTESIAN_POINT('',(3.51294962880404,3.00855921853322,-6.48345473929143));
#97541=CARTESIAN_POINT('Origin',(3.45643652588379E-13,3.10034167699945,
-8.7213222754734E-13));
#97542=CARTESIAN_POINT('',(2.95351468760115,3.09925366544939,-6.8939648237853));
#97543=CARTESIAN_POINT('Origin',(-0.0744880397876002,3.0892853942158,0.177915339575154));
#97544=CARTESIAN_POINT('Origin',(-0.0969165599810617,2.94644894008946,0.164376056078851));
#97545=CARTESIAN_POINT('Ctrl Pts',(4.56979675856999,2.877925369,-5.95021467344));
#97546=CARTESIAN_POINT('Ctrl Pts',(4.24645049813,2.943232886,-6.19854633505999));
#97547=CARTESIAN_POINT('Ctrl Pts',(3.89809814271,3.008559221,-6.41037658437));
#97548=CARTESIAN_POINT('Ctrl Pts',(4.566364721,2.877925369,-5.94964816));
#97549=CARTESIAN_POINT('Ctrl Pts',(4.243049246,2.943232886,-6.197793318));
#97550=CARTESIAN_POINT('Ctrl Pts',(3.894747705,3.008559221,-6.409441498));
#97551=CARTESIAN_POINT('Ctrl Pts',(4.223160964,2.877925369,-5.892996816));
#97552=CARTESIAN_POINT('Ctrl Pts',(3.902924033,2.943232886,-6.122491612));
#97553=CARTESIAN_POINT('Ctrl Pts',(3.559703934,3.008559221,-6.31593286100001));
#97554=CARTESIAN_POINT('',(3.89474771260811,3.00855922118748,-6.4094414992632));
#97555=CARTESIAN_POINT('',(3.72722582217893,3.00855922150568,-6.3626871779307));
#97556=CARTESIAN_POINT('',(4.36603605880988,2.91791835919084,-6.09817426023959));
#97557=CARTESIAN_POINT('Origin',(-0.108555880427207,2.94642873921719,0.159469471285798));
#97558=CARTESIAN_POINT('Ctrl Pts',(4.21934602252135,2.8787032030072,-5.89572888979621));
#97559=CARTESIAN_POINT('Ctrl Pts',(4.24379729330923,2.88555248746722,-5.92939598666343));
#97560=CARTESIAN_POINT('Ctrl Pts',(4.26825859668524,2.89224022488836,-5.9631185941482));
#97561=CARTESIAN_POINT('Ctrl Pts',(4.31714637918945,2.90530189662508,-6.03059070613479));
#97562=CARTESIAN_POINT('Ctrl Pts',(4.34159956115091,2.91168295883936,-6.06437707132088));
#97563=CARTESIAN_POINT('Ctrl Pts',(4.36603605311106,2.91791835925659,-6.09817425000079));
#97564=CARTESIAN_POINT('Ctrl Pts',(4.8365929217786,3.01309343425874,-5.73289133585869));
#97565=CARTESIAN_POINT('Ctrl Pts',(4.82573699335903,3.01082632762937,-5.74198008190041));
#97566=CARTESIAN_POINT('Ctrl Pts',(4.81488106493935,3.008559221,-5.75106882794202));
#97567=CARTESIAN_POINT('Ctrl Pts',(4.50003661231422,2.942808424,-6.0146613243089));
#97568=CARTESIAN_POINT('Ctrl Pts',(4.15829902992391,2.877933005,-6.2423089886404));
#97569=CARTESIAN_POINT('Ctrl Pts',(4.85461685012897,3.01309343425874,-5.38478824126976));
#97570=CARTESIAN_POINT('Ctrl Pts',(4.84441787606454,3.01082632762937,-5.39391349013488));
#97571=CARTESIAN_POINT('Ctrl Pts',(4.834218902,3.008559221,-5.403038739));
#97572=CARTESIAN_POINT('Ctrl Pts',(4.538427489,2.942808424,-5.66768989300001));
#97573=CARTESIAN_POINT('Ctrl Pts',(4.215513515,2.877933005,-5.898469785));
#97574=CARTESIAN_POINT('',(4.81492095813824,3.00855922016357,-5.75035096374377));
#97575=CARTESIAN_POINT('Origin',(-0.131593479604116,3.08925209839837,0.136990176737752));
#97576=CARTESIAN_POINT('',(4.82456993844337,3.00855921853322,-5.57669484259999));
#97577=CARTESIAN_POINT('Origin',(4.31946145518225E-13,3.10034167700033,
-5.37330596683816E-13));
#97578=CARTESIAN_POINT('',(4.36646180827853,3.09925366547195,-6.09786940478255));
#97579=CARTESIAN_POINT('Origin',(-0.110993050041802,3.08928540862611,0.157742983199022));
#97580=CARTESIAN_POINT('Origin',(-0.129986767072367,2.94644890496931,0.139698935014254));
#97581=CARTESIAN_POINT('Ctrl Pts',(5.74207771809,2.877925369,-4.82873074004));
#97582=CARTESIAN_POINT('Ctrl Pts',(5.47967508015,2.943232886,-5.14076643327));
#97583=CARTESIAN_POINT('Ctrl Pts',(5.18500425127,3.008559221,-5.4225296685));
#97584=CARTESIAN_POINT('Ctrl Pts',(5.738604136,2.877925369,-4.828915258));
#97585=CARTESIAN_POINT('Ctrl Pts',(5.476191471,2.943232886,-5.14076219));
#97586=CARTESIAN_POINT('Ctrl Pts',(5.181531129,3.008559221,-5.42233668900001));
#97587=CARTESIAN_POINT('Ctrl Pts',(5.391245927,2.877925369,-4.847367054));
#97588=CARTESIAN_POINT('Ctrl Pts',(5.127830556,2.943232886,-5.14033786300001));
#97589=CARTESIAN_POINT('Ctrl Pts',(4.83421890200001,3.008559221,-5.403038739));
#97590=CARTESIAN_POINT('',(5.18153113441456,3.00855922118773,-5.42233668988285));
#97591=CARTESIAN_POINT('',(5.00787501777894,3.00855922150568,-5.4126877118915));
#97592=CARTESIAN_POINT('',(5.57488776725939,2.91791835921303,-5.01703364133197));
#97593=CARTESIAN_POINT('Origin',(-0.140299164977526,2.94642873468267,0.132404891235894));
#97594=CARTESIAN_POINT('Ctrl Pts',(5.38810749193988,2.87870320295152,-4.85085535283309));
#97595=CARTESIAN_POINT('Ctrl Pts',(5.41922453632117,2.88555248744538,-4.87847903131057));
#97596=CARTESIAN_POINT('Ctrl Pts',(5.45036331187865,2.89224022489509,-4.9061547658748));
#97597=CARTESIAN_POINT('Ctrl Pts',(5.51261263464246,2.90530189660948,-4.96153998905137));
#97598=CARTESIAN_POINT('Ctrl Pts',(5.54375718430893,2.91168295877134,-4.9892797362151));
#97599=CARTESIAN_POINT('Ctrl Pts',(5.57488775937166,2.91791835925558,-5.01703363246046));
#97600=CARTESIAN_POINT('Ctrl Pts',(5.95591824100316,3.01309343431531,-4.55913501208992));
#97601=CARTESIAN_POINT('Ctrl Pts',(5.94726992978911,3.01082632765766,-4.57034497217893));
#97602=CARTESIAN_POINT('Ctrl Pts',(5.93862161857506,3.008559221,-4.58155493226809));
#97603=CARTESIAN_POINT('Ctrl Pts',(5.68780264933675,2.942808424,-4.90666703394516));
#97604=CARTESIAN_POINT('Ctrl Pts',(5.40299222083258,2.877933005,-5.20245589984858));
#97605=CARTESIAN_POINT('Ctrl Pts',(5.89868890410138,3.01309343431532,-4.21529576255416));
#97606=CARTESIAN_POINT('Ctrl Pts',(5.89069003505073,3.01082632765766,-4.22640014627709));
#97607=CARTESIAN_POINT('Ctrl Pts',(5.882691166,3.008559221,-4.23750453));
#97608=CARTESIAN_POINT('Ctrl Pts',(5.650707367,2.942808424,-4.55955469800001));
#97609=CARTESIAN_POINT('Ctrl Pts',(5.384953798,2.877933005,-4.854356043));
#97610=CARTESIAN_POINT('',(5.93850625965619,3.00855922016355,-4.58084527514519));
#97611=CARTESIAN_POINT('Origin',(-0.157965620748939,3.08925204684029,0.105498622484728));
#97612=CARTESIAN_POINT('',(5.91059871904763,3.00855921853322,-4.40917489237146));
#97613=CARTESIAN_POINT('Origin',(-3.02275565688959E-13,3.100341677,4.0462425077159E-13));
#97614=CARTESIAN_POINT('',(5.57523802806611,3.09925366543908,-5.01664438946001));
#97615=CARTESIAN_POINT('Origin',(-0.142308321067965,3.08928536684624,0.130194957196356));
#97616=CARTESIAN_POINT('Origin',(-0.156978694153445,2.94644889134558,0.10848936492422));
#97617=CARTESIAN_POINT('Ctrl Pts',(6.64586550476001,2.877925369,-3.48146072451));
#97618=CARTESIAN_POINT('Ctrl Pts',(6.45667614448,2.943232886,-3.84261000606));
#97619=CARTESIAN_POINT('Ctrl Pts',(6.22946532249,3.008559221,-4.18113129112));
#97620=CARTESIAN_POINT('Ctrl Pts',(6.642512799,2.877925369,-3.482387646));
#97621=CARTESIAN_POINT('Ctrl Pts',(6.453273068,2.943232886,-3.843354735));
#97622=CARTESIAN_POINT('Ctrl Pts',(6.226031915,3.008559221,-4.181689442));
#97623=CARTESIAN_POINT('Ctrl Pts',(6.307242223,2.877925369,-3.575079795));
#97624=CARTESIAN_POINT('Ctrl Pts',(6.11296542000001,2.943232886,-3.917827629));
#97625=CARTESIAN_POINT('Ctrl Pts',(5.882691166,3.008559221,-4.23750453));
#97626=CARTESIAN_POINT('',(6.22603192246108,3.00855922118754,-4.18168943994305));
#97627=CARTESIAN_POINT('',(6.0543615422724,3.00855922150568,-4.20959698345089));
#97628=CARTESIAN_POINT('',(6.52306391963344,2.91791835919899,-3.70130210519327));
#97629=CARTESIAN_POINT('Origin',(-0.165482309760923,2.94642871606807,0.0991492473473568));
#97630=CARTESIAN_POINT('Ctrl Pts',(6.3049270436911,2.87870320303805,-3.57916121057829));
#97631=CARTESIAN_POINT('Ctrl Pts',(6.34125486302186,2.88555248746677,-3.59944981817011));
#97632=CARTESIAN_POINT('Ctrl Pts',(6.37761509597951,2.89224022486561,-3.61978459314537));
#97633=CARTESIAN_POINT('Ctrl Pts',(6.45031524954148,2.90530189648302,-3.66049317608533));
#97634=CARTESIAN_POINT('Ctrl Pts',(6.48669488220596,2.9116829585802,-3.68088922557261));
#97635=CARTESIAN_POINT('Ctrl Pts',(6.52306391009491,2.91791835925355,-3.7013020982684));
#97636=CARTESIAN_POINT('Ctrl Pts',(6.79675144293879,3.01309343437702,-3.17219860221281));
#97637=CARTESIAN_POINT('Ctrl Pts',(6.79071513441644,3.01082632768851,-3.18500561110874));
#97638=CARTESIAN_POINT('Ctrl Pts',(6.78467882589409,3.008559221,-3.19781262000476));
#97639=CARTESIAN_POINT('Ctrl Pts',(6.60961335663601,2.942808424,-3.56924244567881));
#97640=CARTESIAN_POINT('Ctrl Pts',(6.39504749999349,2.877933005,-3.91934175591123));
#97641=CARTESIAN_POINT('Ctrl Pts',(6.6669448214866,3.01309343437701,-2.8487007390812));
#97642=CARTESIAN_POINT('Ctrl Pts',(6.66152007574329,3.01082632768851,-2.86126502904062));
#97643=CARTESIAN_POINT('Ctrl Pts',(6.65609533,3.008559221,-2.873829319));
#97644=CARTESIAN_POINT('Ctrl Pts',(6.49876645,2.942808424,-3.238219792));
#97645=CARTESIAN_POINT('Ctrl Pts',(6.302599626,2.877933005,-3.583258008));
#97646=CARTESIAN_POINT('',(6.78441360869358,3.00855922016356,-3.1971443530287));
#97647=CARTESIAN_POINT('Origin',(-0.176951505971167,3.08925206221049,0.0690741528171268));
#97648=CARTESIAN_POINT('',(6.72025447322881,3.00855921853322,-3.03548682471005));
#97649=CARTESIAN_POINT('Origin',(-8.14452671971111E-13,3.10034167700089,
4.8095208371457E-13));
#97650=CARTESIAN_POINT('',(6.52332231405112,3.09925366544977,-3.70084665820566));
#97651=CARTESIAN_POINT('Origin',(-0.166969114518551,3.08928541551715,0.0965588810779272));
#97652=CARTESIAN_POINT('Origin',(-0.176630635389806,2.94644889976632,0.0722071675918656));
#97653=CARTESIAN_POINT('Ctrl Pts',(7.23890000664,2.877925369,-1.97140147378));
#97654=CARTESIAN_POINT('Ctrl Pts',(7.13177020874,2.943232886,-2.36477740657));
#97655=CARTESIAN_POINT('Ctrl Pts',(6.98264351939001,3.008559221,-2.74422786226));
#97656=CARTESIAN_POINT('Ctrl Pts',(7.235824946,2.877925369,-1.973027457));
#97657=CARTESIAN_POINT('Ctrl Pts',(7.128606789,2.943232886,-2.366236285));
#97658=CARTESIAN_POINT('Ctrl Pts',(6.979410369,3.008559221,-2.745511045));
#97659=CARTESIAN_POINT('Ctrl Pts',(6.928318882,2.877925369,-2.135625779));
#97660=CARTESIAN_POINT('Ctrl Pts',(6.81226481500001,2.943232886,-2.512124128));
#97661=CARTESIAN_POINT('Ctrl Pts',(6.65609533,3.008559221,-2.873829319));
#97662=CARTESIAN_POINT('',(6.9794103743155,3.0085592211877,-2.74551104348943));
#97663=CARTESIAN_POINT('',(6.81775285068297,3.00855922150568,-2.80967017912947));
#97664=CARTESIAN_POINT('',(7.16622885296103,2.91791835924605,-2.21250179662255));
#97665=CARTESIAN_POINT('Origin',(-0.182927537908617,2.94642874070228,0.0612573726355285));
#97666=CARTESIAN_POINT('Ctrl Pts',(6.92693521466343,2.87870320306878,-2.14010946824917));
#97667=CARTESIAN_POINT('Ctrl Pts',(6.96677516062568,2.88555248753215,-2.15211433211194));
#97668=CARTESIAN_POINT('Ctrl Pts',(7.00665668705788,2.89224022495434,-2.16415731607856));
#97669=CARTESIAN_POINT('Ctrl Pts',(7.08640830760725,2.9053018989249,-2.18828577534183));
#97670=CARTESIAN_POINT('Ctrl Pts',(7.12632196852394,2.91168296343591,-2.20038443586059));
#97671=CARTESIAN_POINT('Ctrl Pts',(7.166228842292,2.91791835931419,-2.21250179176944));
#97672=CARTESIAN_POINT('Ctrl Pts',(7.31977610100223,3.01309343437182,-1.63693371248333));
#97673=CARTESIAN_POINT('Ctrl Pts',(7.31663404636609,3.01082632768591,-1.65073892851269));
#97674=CARTESIAN_POINT('Ctrl Pts',(7.31349199172984,3.008559221,-1.66454414454206));
#97675=CARTESIAN_POINT('Ctrl Pts',(7.22236588909272,2.942808424,-2.06492404828789));
#97676=CARTESIAN_POINT('Ctrl Pts',(7.08807746584068,2.877933005,-2.45296354772446));
#97677=CARTESIAN_POINT('Ctrl Pts',(7.12346180852388,3.01309343437182,-1.34890363637351));
#97678=CARTESIAN_POINT('Ctrl Pts',(7.12086484126195,3.01082632768591,-1.36234034018676));
#97679=CARTESIAN_POINT('Ctrl Pts',(7.118267874,3.008559221,-1.375777044));
#97680=CARTESIAN_POINT('Ctrl Pts',(7.04295043600001,2.942808424,-1.765469329));
#97681=CARTESIAN_POINT('Ctrl Pts',(6.925542901,2.877933005,-2.144610811));
#97682=CARTESIAN_POINT('',(7.31308931751528,3.00855922016356,-1.66394851513886));
#97683=CARTESIAN_POINT('Origin',(-0.187663364952104,3.08925205844719,0.0294198893682893));
#97684=CARTESIAN_POINT('',(7.21567859711876,3.00855921853322,-1.51986276769344));
#97685=CARTESIAN_POINT('Origin',(-1.64972202565394E-12,3.100341677,5.011182441228E-13));
#97686=CARTESIAN_POINT('',(7.16638329838837,3.09925366545765,-2.2120014507076));
#97687=CARTESIAN_POINT('Origin',(-0.183822865913644,3.08928540630914,0.0584079944972435));
#97688=CARTESIAN_POINT('Origin',(-0.188023592722597,2.94644890831842,0.0325486638177702));
#97689=CARTESIAN_POINT('Ctrl Pts',(7.4934515901,2.877925369,-0.36916168223));
#97690=CARTESIAN_POINT('Ctrl Pts',(7.473390625,2.943232886,-0.7763704436));
#97691=CARTESIAN_POINT('Ctrl Pts',(7.40932106577,3.008559221,-1.17900738859));
#97692=CARTESIAN_POINT('Ctrl Pts',(7.490797961,2.877925369,-0.371410698));
#97693=CARTESIAN_POINT('Ctrl Pts',(7.47061478,2.943232886,-0.778475256));
#97694=CARTESIAN_POINT('Ctrl Pts',(7.406439351,3.008559221,-1.180955603));
#97695=CARTESIAN_POINT('Ctrl Pts',(7.225435051,2.877925369,-0.596312275));
#97696=CARTESIAN_POINT('Ctrl Pts',(7.19303028,2.943232886,-0.988956496));
#97697=CARTESIAN_POINT('Ctrl Pts',(7.11826787400001,3.008559221,-1.375777044));
#97698=CARTESIAN_POINT('',(7.40643935690396,3.00855922118749,-1.1809555980013));
#97699=CARTESIAN_POINT('',(7.26235361303831,3.00855922150574,-1.27836632044191));
#97700=CARTESIAN_POINT('',(7.47430889007143,2.91791835920043,-0.620247362827596));
#97701=CARTESIAN_POINT('Origin',(-0.191819194413607,2.94642872304643,0.0205011828756771));
#97702=CARTESIAN_POINT('Ctrl Pts',(7.22504759247685,2.87870320299642,-0.600988586293256));
#97703=CARTESIAN_POINT('Ctrl Pts',(7.26653679368753,2.88555248744925,-0.604148372301362));
#97704=CARTESIAN_POINT('Ctrl Pts',(7.30807479791577,2.89224022487032,-0.607336448616159));
#97705=CARTESIAN_POINT('Ctrl Pts',(7.39114876161084,2.90530189663738,-0.613756555677362));
#97706=CARTESIAN_POINT('Ctrl Pts',(7.43273010190432,2.91168295887499,-0.616992097636169));
#97707=CARTESIAN_POINT('Ctrl Pts',(7.47430887852099,2.91791835925716,-0.620247360538585));
#97708=CARTESIAN_POINT('Ctrl Pts',(7.50053616437872,3.01309343429141,-0.0251276216729472));
#97709=CARTESIAN_POINT('Ctrl Pts',(7.50043528258605,3.0108263276457,-0.0392855280246127));
#97710=CARTESIAN_POINT('Ctrl Pts',(7.50033440079339,3.008559221,-0.0534434343762788));
#97711=CARTESIAN_POINT('Ctrl Pts',(7.49740861947476,2.942808424,-0.464052096406355));
#97712=CARTESIAN_POINT('Ctrl Pts',(7.44967680772641,2.877933005,-0.871887489858721));
#97713=CARTESIAN_POINT('Ctrl Pts',(7.24689363902802,3.01309343429141,0.213966701145049));
#97714=CARTESIAN_POINT('Ctrl Pts',(7.24724588151406,3.0108263276457,0.200285869072528));
#97715=CARTESIAN_POINT('Ctrl Pts',(7.247598124,3.008559221,0.186605037));
#97716=CARTESIAN_POINT('Ctrl Pts',(7.257813887,2.942808424,-0.210167481));
#97717=CARTESIAN_POINT('Ctrl Pts',(7.224655486,2.877933005,-0.605683996000001));
#97718=CARTESIAN_POINT('',(7.49981309817101,3.00855922016355,-0.0529482935119721));
#97719=CARTESIAN_POINT('Origin',(-0.189600522067149,3.08925208754637,-0.0116100011989929));
#97720=CARTESIAN_POINT('',(7.37370560986287,3.00855921853322,0.0668283836308336));
#97721=CARTESIAN_POINT('Origin',(-1.23295471055052E-12,3.10034167699989,
9.98990657991722E-14));
#97722=CARTESIAN_POINT('',(7.47435216511154,3.09925366543305,-0.619725513626576));
#97723=CARTESIAN_POINT('Origin',(-0.19208124950314,3.08928537215579,0.0175259825682194));
#97724=CARTESIAN_POINT('Origin',(-0.190624840073971,2.94644892047951,-0.00863181313441378));
#97725=CARTESIAN_POINT('Ctrl Pts',(7.39761770582,2.877925369,1.25033969985));
#97726=CARTESIAN_POINT('Ctrl Pts',(7.46556360084,2.943232886,0.84833873868));
#97727=CARTESIAN_POINT('Ctrl Pts',(7.48954699437,3.008559221,0.44134215973));
#97728=CARTESIAN_POINT('Ctrl Pts',(7.395509589,2.877925369,1.247572813));
#97729=CARTESIAN_POINT('Ctrl Pts',(7.463305126,2.943232886,0.845686411));
#97730=CARTESIAN_POINT('Ctrl Pts',(7.487151461,3.008559221,0.43882001));
#97731=CARTESIAN_POINT('Ctrl Pts',(7.184697907,2.877925369,0.970884128));
#97732=CARTESIAN_POINT('Ctrl Pts',(7.237457642,2.943232886,0.580453643));
#97733=CARTESIAN_POINT('Ctrl Pts',(7.247598124,3.008559221,0.186605037));
#97734=CARTESIAN_POINT('',(7.48715146569571,3.00855922118754,0.438820016133631));
#97735=CARTESIAN_POINT('',(7.36737479236834,3.00855922150568,0.312712526601943));
#97736=CARTESIAN_POINT('',(7.43289855028286,2.91791835921972,1.00100914803522));
#97737=CARTESIAN_POINT('Origin',(-0.191741974370172,2.94642869754464,-0.0212136133593398));
#97738=CARTESIAN_POINT('Ctrl Pts',(7.18532477592923,2.87870320303117,0.966233854152873));
#97739=CARTESIAN_POINT('Ctrl Pts',(7.22652324323512,2.88555248748559,0.972066894051458));
#97740=CARTESIAN_POINT('Ctrl Pts',(7.26777545414825,2.89224022490859,0.977882796247031));
#97741=CARTESIAN_POINT('Ctrl Pts',(7.35028732932028,2.90530189689843,0.989471234464394));
#97742=CARTESIAN_POINT('Ctrl Pts',(7.39159206841385,2.91168295936306,0.995250096922327));
#97743=CARTESIAN_POINT('Ctrl Pts',(7.4328985384329,2.91791835926312,1.00100914773029));
#97744=CARTESIAN_POINT('Ctrl Pts',(7.33057949306216,3.01309343423581,1.58785340936343));
#97745=CARTESIAN_POINT('Ctrl Pts',(7.33352450114769,3.01082632761791,1.57400482053784));
#97746=CARTESIAN_POINT('Ctrl Pts',(7.33646950923327,3.008559221,1.56015623171219));
#97747=CARTESIAN_POINT('Ctrl Pts',(7.42188085569069,2.942808424,1.15851841485023));
#97748=CARTESIAN_POINT('Ctrl Pts',(7.4629375410039,2.877933005,0.749957057499588));
#97749=CARTESIAN_POINT('Ctrl Pts',(7.03146877652035,3.01309343423581,1.76683219387563));
#97750=CARTESIAN_POINT('Ctrl Pts',(7.03475375826022,3.01082632761791,1.75354693393781));
#97751=CARTESIAN_POINT('Ctrl Pts',(7.03803874,3.008559221,1.740261674));
#97752=CARTESIAN_POINT('Ctrl Pts',(7.133310028,2.942808424,1.354961564));
#97753=CARTESIAN_POINT('Ctrl Pts',(7.185951211,2.877933005,0.961563929));
#97754=CARTESIAN_POINT('',(7.3358539538905,3.00855922016357,1.56052773146292));
#97755=CARTESIAN_POINT('Origin',(-0.182671985471999,3.08925207572926,-0.0520970703534511));
#97756=CARTESIAN_POINT('',(7.18694634311339,3.00855921853322,1.65039471424761));
#97757=CARTESIAN_POINT('Origin',(-1.37476835471162E-12,3.100341677,-2.28576923014256E-13));
#97758=CARTESIAN_POINT('',(7.43282863131925,3.09925366549807,1.0015281002253));
#97759=CARTESIAN_POINT('Origin',(-0.191357879377316,3.08928538259554,-0.0241755478480393));
#97760=CARTESIAN_POINT('Origin',(-0.184312315726758,2.94644892100903,-0.0494086674092373));
#97761=CARTESIAN_POINT('Ctrl Pts',(6.95587943833,2.877925369,2.81137658738));
#97762=CARTESIAN_POINT('Ctrl Pts',(7.10865512091,2.943232886,2.43338054406));
#97763=CARTESIAN_POINT('Ctrl Pts',(7.2195700295,3.008559221,2.04105504014));
#97764=CARTESIAN_POINT('Ctrl Pts',(6.954415407,2.877925369,2.808221206));
#97765=CARTESIAN_POINT('Ctrl Pts',(7.10701962,2.943232886,2.430304721));
#97766=CARTESIAN_POINT('Ctrl Pts',(7.21777269,3.008559221,2.038076888));
#97767=CARTESIAN_POINT('Ctrl Pts',(6.80801227400001,2.877925369,2.492683068));
#97768=CARTESIAN_POINT('Ctrl Pts',(6.943469529,2.943232886,2.122722415));
#97769=CARTESIAN_POINT('Ctrl Pts',(7.03803874,3.008559221,1.740261674));
#97770=CARTESIAN_POINT('',(7.21777269325456,3.00855922118747,2.03807689497795));
#97771=CARTESIAN_POINT('',(7.12790571420459,3.00855922150568,1.88916928400112));
#97772=CARTESIAN_POINT('',(7.04393413548324,2.91791835922453,2.57545958400812));
#97773=CARTESIAN_POINT('Origin',(-0.182698656706801,2.94642872972437,-0.0619364437379809));
#97774=CARTESIAN_POINT('Ctrl Pts',(6.80962415877199,2.87870320302982,2.48827627387171));
#97775=CARTESIAN_POINT('Ctrl Pts',(6.84860549753355,2.88555248748783,2.50282939327934));
#97776=CARTESIAN_POINT('Ctrl Pts',(6.88764300755156,2.89224022490975,2.51737732889852));
#97777=CARTESIAN_POINT('Ctrl Pts',(6.96573463276544,2.90530189749325,2.54643245134944));
#97778=CARTESIAN_POINT('Ctrl Pts',(7.00483140947897,2.9116829605772,2.56095550664469));
#97779=CARTESIAN_POINT('Ctrl Pts',(7.04393412401197,2.9179183592784,2.57545958125269));
#97780=CARTESIAN_POINT('Ctrl Pts',(6.81785307114309,3.0130934344198,3.12658818002624));
#97781=CARTESIAN_POINT('Ctrl Pts',(6.82370626405869,3.01082632770991,3.11369645271363));
#97782=CARTESIAN_POINT('Ctrl Pts',(6.82955945697441,3.008559221,3.10080472540109));
#97783=CARTESIAN_POINT('Ctrl Pts',(6.99931419217042,2.942808424,2.72691789343058));
#97784=CARTESIAN_POINT('Ctrl Pts',(7.12723960983362,2.877933005,2.33673444667371));
#97785=CARTESIAN_POINT('Ctrl Pts',(6.48726024873397,3.0130934344198,3.23708257895296));
#97786=CARTESIAN_POINT('Ctrl Pts',(6.49332436786697,3.01082632770991,3.22481409447648));
#97787=CARTESIAN_POINT('Ctrl Pts',(6.499388487,3.008559221,3.21254561));
#97788=CARTESIAN_POINT('Ctrl Pts',(6.67526052,2.942808424,2.856734113));
#97789=CARTESIAN_POINT('Ctrl Pts',(6.811239844,2.877933005,2.483850194));
#97790=CARTESIAN_POINT('',(6.82887843149303,3.00855922016357,3.10103521348777));
#97791=CARTESIAN_POINT('Origin',(-0.16720171822584,3.08925211066832,-0.0901480920089814));
#97792=CARTESIAN_POINT('',(6.66413345302227,3.00855921853322,3.15679042217479));
#97793=CARTESIAN_POINT('Origin',(3.60822483003176E-13,3.10034167699911,
1.28369537222284E-13));
#97794=CARTESIAN_POINT('',(7.0437542921393,3.09925366545849,2.5759513724016));
#97795=CARTESIAN_POINT('Origin',(-0.181687328973064,3.08928539963458,-0.0647467316431227));
#97796=CARTESIAN_POINT('Origin',(-0.169381881647932,2.94644890184184,-0.0878752678220951));
#97797=CARTESIAN_POINT('Ctrl Pts',(6.18889198036999,2.877925369,4.24095662977));
#97798=CARTESIAN_POINT('Ctrl Pts',(6.41935382777,2.943232886,3.90464017938));
#97799=CARTESIAN_POINT('Ctrl Pts',(6.61201399403,3.008559221,3.54533045445));
#97800=CARTESIAN_POINT('Ctrl Pts',(6.188140491,2.877925369,4.237560296));
#97801=CARTESIAN_POINT('Ctrl Pts',(6.418417775,2.943232886,3.901284683));
#97802=CARTESIAN_POINT('Ctrl Pts',(6.61089889000001,3.008559221,3.542035555));
#97803=CARTESIAN_POINT('Ctrl Pts',(6.11299155399999,2.877925369,3.897926919));
#97804=CARTESIAN_POINT('Ctrl Pts',(6.324812498,2.943232886,3.565735045));
#97805=CARTESIAN_POINT('Ctrl Pts',(6.499388487,3.008559221,3.21254561));
#97806=CARTESIAN_POINT('',(6.61089889168035,3.00855922118749,3.5420355625124));
#97807=CARTESIAN_POINT('',(6.55514368707799,3.0085592215057,3.37729058526005));
#97808=CARTESIAN_POINT('',(6.32560318942504,2.91791835919154,4.0294843921115));
#97809=CARTESIAN_POINT('Origin',(-0.165112878023673,2.94642872513648,-0.0997632859033443));
#97810=CARTESIAN_POINT('Ctrl Pts',(6.11551308427135,2.87870320302233,3.89396966096815));
#97811=CARTESIAN_POINT('Ctrl Pts',(6.15045457056271,2.8855524874798,3.91656237190437));
#97812=CARTESIAN_POINT('Ctrl Pts',(6.1854520291735,2.89224022489624,3.93916209546234));
#97813=CARTESIAN_POINT('Ctrl Pts',(6.25547191867812,2.90530189663992,3.98432531331739));
#97814=CARTESIAN_POINT('Ctrl Pts',(6.29053260184279,2.91168295886177,4.00691347567795));
#97815=CARTESIAN_POINT('Ctrl Pts',(6.32560317889203,2.91791835925685,4.0294843869756));
#97816=CARTESIAN_POINT('Ctrl Pts',(5.98633141818167,3.01309343439026,4.51912716191478));
#97817=CARTESIAN_POINT('Ctrl Pts',(5.99481910694851,3.01082632769513,4.50779509954357));
#97818=CARTESIAN_POINT('Ctrl Pts',(6.00330679571537,3.008559221,4.49646303717236));
#97819=CARTESIAN_POINT('Ctrl Pts',(6.2494673766473,2.942808424,4.16780972140263));
#97820=CARTESIAN_POINT('Ctrl Pts',(6.45827987543194,2.877933005,3.81424873072673));
#97821=CARTESIAN_POINT('Ctrl Pts',(5.63971464235043,3.01309343439026,4.55597057842557));
#97822=CARTESIAN_POINT('Ctrl Pts',(5.64827434717523,3.01082632769513,4.54529253071275));
#97823=CARTESIAN_POINT('Ctrl Pts',(5.65683405200001,3.008559221,4.534614483));
#97824=CARTESIAN_POINT('Ctrl Pts',(5.905083248,2.942808424,4.224928949));
#97825=CARTESIAN_POINT('Ctrl Pts',(6.118042472,2.877933005,3.889994385));
#97826=CARTESIAN_POINT('',(6.00259214409304,3.00855922016357,4.49654173624063));
#97827=CARTESIAN_POINT('Origin',(-0.143913387883455,3.08925206949373,-0.123983845329459));
#97828=CARTESIAN_POINT('',(5.82971308973404,3.00855921853322,4.51557811846257));
#97829=CARTESIAN_POINT('Origin',(2.78856798763272E-13,3.100341677,1.81278603239576E-13));
#97830=CARTESIAN_POINT('',(6.32532183056699,3.09925366549247,4.02992602189084));
#97831=CARTESIAN_POINT('Origin',(-0.163520847236953,3.08928539071856,-0.102290334525119));
#97832=CARTESIAN_POINT('Origin',(-0.14653118572046,2.94644889901171,-0.122232846529689));
#97833=CARTESIAN_POINT('Ctrl Pts',(5.1325188116,2.877925369,5.47223425438));
#97834=CARTESIAN_POINT('Ctrl Pts',(5.42989068484001,2.943232886,5.19332318041001));
#97835=CARTESIAN_POINT('Ctrl Pts',(5.69528753253,3.008559221,4.88383015693));
#97836=CARTESIAN_POINT('Ctrl Pts',(5.132515003,2.877925369,5.468755777));
#97837=CARTESIAN_POINT('Ctrl Pts',(5.429697849,2.943232886,5.18984491));
#97838=CARTESIAN_POINT('Ctrl Pts',(5.694906805,3.008559221,4.880372576));
#97839=CARTESIAN_POINT('Ctrl Pts',(5.132134143,2.877925369,5.120908039));
#97840=CARTESIAN_POINT('Ctrl Pts',(5.410414265,2.943232886,4.842017869));
#97841=CARTESIAN_POINT('Ctrl Pts',(5.656834052,3.008559221,4.534614483));
#97842=CARTESIAN_POINT('',(5.69490680616228,3.0085592211877,4.8803725814005));
#97843=CARTESIAN_POINT('',(5.67587042651797,3.00855922150568,4.70749353188976));
#97844=CARTESIAN_POINT('',(5.31149406848905,2.917918359164,5.29509498865337));
#97845=CARTESIAN_POINT('Origin',(-0.139806310419599,2.94642872523138,-0.132925095633846));
#97846=CARTESIAN_POINT('Ctrl Pts',(5.13544741496531,2.8787032030605,5.1175853537983));
#97847=CARTESIAN_POINT('Ctrl Pts',(5.16471522369949,2.88555248750377,5.14716124648086));
#97848=CARTESIAN_POINT('Ctrl Pts',(5.19403618863513,2.89224022490984,5.17675602021783));
#97849=CARTESIAN_POINT('Ctrl Pts',(5.25271028727322,2.90530189488208,5.23591554579191));
#97850=CARTESIAN_POINT('Ctrl Pts',(5.2820954749823,2.91168295528719,5.26551261105691));
#97851=CARTESIAN_POINT('Ctrl Pts',(5.31149405931312,2.91791835921186,5.29509498119979));
#97852=CARTESIAN_POINT('Ctrl Pts',(4.87489556082486,3.01309343436845,5.70035678014367));
#97853=CARTESIAN_POINT('Ctrl Pts',(4.88562087052289,3.01082632768423,5.69111425733716));
#97854=CARTESIAN_POINT('Ctrl Pts',(4.89634618022078,3.008559221,5.68187173453059));
#97855=CARTESIAN_POINT('Ctrl Pts',(5.20740241132506,2.942808424,5.41381939934602));
#97856=CARTESIAN_POINT('Ctrl Pts',(5.4873381521754,2.877933005,5.11341298321379));
#97857=CARTESIAN_POINT('Ctrl Pts',(4.52846224745558,3.01309343436846,5.66182645664609));
#97858=CARTESIAN_POINT('Ctrl Pts',(4.5391172957278,3.01082632768423,5.65323813932303));
#97859=CARTESIAN_POINT('Ctrl Pts',(4.549772344,3.008559221,5.644649822));
#97860=CARTESIAN_POINT('Ctrl Pts',(4.85879084800001,2.942808424,5.395570803));
#97861=CARTESIAN_POINT('Ctrl Pts',(5.138772234,2.877933005,5.114246761));
#97862=CARTESIAN_POINT('',(4.89563131846189,3.00855922016355,5.68179496485426));
#97863=CARTESIAN_POINT('Origin',(-0.113895955393939,3.08925208356024,-0.152022352616782));
#97864=CARTESIAN_POINT('',(4.72270182137908,3.00855921853322,5.66322240019098));
#97865=CARTESIAN_POINT('Origin',(-3.77302356024956E-14,3.100341677,-3.51281503885303E-14));
#97866=CARTESIAN_POINT('',(5.31112435035528,3.09925366548904,5.29546580931712));
#97867=CARTESIAN_POINT('Origin',(-0.137708370213362,3.08928540048914,-0.135050933526252));
#97868=CARTESIAN_POINT('Origin',(-0.116828942207328,2.94644888520062,-0.150875016634339));
#97869=CARTESIAN_POINT('Ctrl Pts',(3.83615476674,2.877925369,6.44763628624));
#97870=CARTESIAN_POINT('Ctrl Pts',(4.18653188712,2.943232886,6.23917216139));
#97871=CARTESIAN_POINT('Ctrl Pts',(4.51225575563,3.008559221,5.99396738978));
#97872=CARTESIAN_POINT('Ctrl Pts',(3.836898817,2.877925369,6.444238315));
#97873=CARTESIAN_POINT('Ctrl Pts',(4.187091285,2.943232886,6.235733757));
#97874=CARTESIAN_POINT('Ctrl Pts',(4.512627207,3.008559221,5.9905088));
#97875=CARTESIAN_POINT('Ctrl Pts',(3.911303843,2.877925369,6.104441191));
#97876=CARTESIAN_POINT('Ctrl Pts',(4.243031073,2.943232886,5.891893318));
#97877=CARTESIAN_POINT('Ctrl Pts',(4.549772344,3.008559221,5.644649822));
#97878=CARTESIAN_POINT('',(4.51262720696789,3.00855922118776,5.99050880554579));
#97879=CARTESIAN_POINT('',(4.53119977305047,3.0085592215057,5.81757931290789));
#97880=CARTESIAN_POINT('',(4.04902538805296,2.91791835924187,6.31311282809917));
#97881=CARTESIAN_POINT('Origin',(-0.107962680822556,2.94642870747082,-0.15987151407948));
#97882=CARTESIAN_POINT('Ctrl Pts',(3.91525393165377,2.87870320305441,6.10190844352905));
#97883=CARTESIAN_POINT('Ctrl Pts',(3.93747953250698,2.88555248749456,6.1370845819654));
#97884=CARTESIAN_POINT('Ctrl Pts',(3.95975298798327,2.89224022490414,6.17229058701452));
#97885=CARTESIAN_POINT('Ctrl Pts',(4.00433778169506,2.90530189846678,6.24268021169786));
#97886=CARTESIAN_POINT('Ctrl Pts',(4.02667347970861,2.91168296256646,6.27790228240161));
#97887=CARTESIAN_POINT('Ctrl Pts',(4.04902538054254,2.91791835930351,6.31311281906005));
#97888=CARTESIAN_POINT('Ctrl Pts',(3.5355150063926,3.01309343420852,6.61504405096348));
#97889=CARTESIAN_POINT('Ctrl Pts',(3.5479764330658,3.01082632760426,6.60832323795142));
#97890=CARTESIAN_POINT('Ctrl Pts',(3.56043785973906,3.008559221,6.60160242493936));
#97891=CARTESIAN_POINT('Ctrl Pts',(3.9218450974854,2.942808424,6.40668489825574));
#97892=CARTESIAN_POINT('Ctrl Pts',(4.25981459580143,2.877933005,6.17347972710565));
#97893=CARTESIAN_POINT('Ctrl Pts',(3.20546399185573,3.01309343420852,6.50294162320019));
#97894=CARTESIAN_POINT('Ctrl Pts',(3.21771616492783,3.01082632760426,6.4968446166001));
#97895=CARTESIAN_POINT('Ctrl Pts',(3.229968338,3.008559221,6.49074761));
#97896=CARTESIAN_POINT('Ctrl Pts',(3.585306787,2.942808424,6.313921764));
#97897=CARTESIAN_POINT('Ctrl Pts',(3.919218717,2.877933005,6.099362643));
#97898=CARTESIAN_POINT('',(3.55975621426659,3.00855922016355,6.60137377596147));
#97899=CARTESIAN_POINT('Origin',(-0.0785529492724818,3.08925207262269,-0.172952618710034));
#97900=CARTESIAN_POINT('',(3.3948622650675,3.00855921853322,6.54606069746625));
#97901=CARTESIAN_POINT('Origin',(4.56665955050894E-13,3.10034167699978,
6.96057794735694E-13));
#97902=CARTESIAN_POINT('',(4.04858459835594,3.09925366545561,6.31339550070091));
#97903=CARTESIAN_POINT('Origin',(-0.105456859436555,3.08928538134748,-0.161496726582855));
#97904=CARTESIAN_POINT('Origin',(-0.0816639073474729,2.94644894146221,-0.172462423706753));
#97905=CARTESIAN_POINT('Ctrl Pts',(2.36041638985,2.877925369,7.12155401276));
#97906=CARTESIAN_POINT('Ctrl Pts',(2.74741551223,2.943232886,6.9932843864));
#97907=CARTESIAN_POINT('Ctrl Pts',(3.11823591539,3.008559221,6.82383336981));
#97908=CARTESIAN_POINT('Ctrl Pts',(2.361873508,2.877925369,7.118395433));
#97909=CARTESIAN_POINT('Ctrl Pts',(2.748700987,2.943232886,6.990046624));
#97910=CARTESIAN_POINT('Ctrl Pts',(3.119342177,3.008559221,6.820535491));
#97911=CARTESIAN_POINT('Ctrl Pts',(2.507585323,2.877925369,6.802537457));
#97912=CARTESIAN_POINT('Ctrl Pts',(2.877248464,2.943232886,6.666270384));
#97913=CARTESIAN_POINT('Ctrl Pts',(3.229968338,3.008559221,6.49074761));
#97914=CARTESIAN_POINT('',(3.11934217580073,3.00855922118776,6.82053549638459));
#97915=CARTESIAN_POINT('',(3.17465525469764,3.0085592215057,6.65564155183669));
#97916=CARTESIAN_POINT('',(2.5972287809459,2.91791835920175,7.03593652892802));
#97917=CARTESIAN_POINT('Origin',(-0.0710709945505126,2.94642870905485,-0.17934275964715));
#97918=CARTESIAN_POINT('Ctrl Pts',(2.51198752636156,2.87870320303939,6.8009130764396));
#97919=CARTESIAN_POINT('Ctrl Pts',(2.52613167518388,2.88555248749972,6.84004466358328));
#97920=CARTESIAN_POINT('Ctrl Pts',(2.54031613932612,2.89224022492161,6.87921570642526));
#97921=CARTESIAN_POINT('Ctrl Pts',(2.5687268716989,2.90530189613789,6.95754405958114));
#97922=CARTESIAN_POINT('Ctrl Pts',(2.58296866366645,2.91168295781116,6.99674415685239));
#97923=CARTESIAN_POINT('Ctrl Pts',(2.59722877565496,2.91791835924352,7.03593651830473));
#97924=CARTESIAN_POINT('Ctrl Pts',(2.03081769722786,3.01309343440098,7.22041921455049));
#97925=CARTESIAN_POINT('Ctrl Pts',(2.04443255938671,3.0108263277005,7.2165343686569));
#97926=CARTESIAN_POINT('Ctrl Pts',(2.05804742154557,3.008559221,7.21264952276332));
#97927=CARTESIAN_POINT('Ctrl Pts',(2.45290666561806,2.942808424,7.09998093346858));
#97928=CARTESIAN_POINT('Ctrl Pts',(2.83310684306066,2.877933005,6.94488142064696));
#97929=CARTESIAN_POINT('Ctrl Pts',(1.73258180030284,3.01309343440098,7.03998646713984));
#97930=CARTESIAN_POINT('Ctrl Pts',(1.74585820115142,3.0108263277005,7.03666586006987));
#97931=CARTESIAN_POINT('Ctrl Pts',(1.759134602,3.008559221,7.033345253));
#97932=CARTESIAN_POINT('Ctrl Pts',(2.144177766,2.942808424,6.93704076));
#97933=CARTESIAN_POINT('Ctrl Pts',(2.516406889,2.877933005,6.799279107));
#97934=CARTESIAN_POINT('',(2.05743086531991,3.00855922016355,7.21227968582777));
#97935=CARTESIAN_POINT('Origin',(-0.0395366255264623,3.08925206834798,-0.185795359950095));
#97936=CARTESIAN_POINT('',(1.908282721884,3.00855921853322,7.12281247141579));
#97937=CARTESIAN_POINT('Origin',(1.93204827136917E-13,3.10034167700056,
4.70543742858709E-13));
#97938=CARTESIAN_POINT('',(2.59673753012002,3.09925366546135,7.0361178357594));
#97939=CARTESIAN_POINT('Origin',(-0.068274347774625,3.08928543181574,-0.180391257391856));
#97940=CARTESIAN_POINT('Origin',(-0.0426803358656677,2.94644893093892,-0.18598572011913));
#97941=CARTESIAN_POINT('Ctrl Pts',(0.77430756518,2.877925369,7.46247578759));
#97942=CARTESIAN_POINT('Ctrl Pts',(1.17983304171,2.943232886,7.42039840523001));
#97943=CARTESIAN_POINT('Ctrl Pts',(1.57841082871,3.008559221,7.33462448469));
#97944=CARTESIAN_POINT('Ctrl Pts',(0.776409618,2.877925369,7.459704291));
#97945=CARTESIAN_POINT('Ctrl Pts',(1.181784486,2.943232886,7.417512679));
#97946=CARTESIAN_POINT('Ctrl Pts',(1.580200173,3.008559221,7.331641522));
#97947=CARTESIAN_POINT('Ctrl Pts',(0.9866149,2.877925369,7.182554632));
#97948=CARTESIAN_POINT('Ctrl Pts',(1.376928915,2.943232886,7.128940056));
#97949=CARTESIAN_POINT('Ctrl Pts',(1.759134602,3.008559221,7.033345253));
#97950=CARTESIAN_POINT('',(1.58020017063694,3.00855922118764,7.33164152700582));
#97951=CARTESIAN_POINT('',(1.6696673844759,3.00855922150568,7.18249338820299));
#97952=CARTESIAN_POINT('',(1.02398864236711,2.91791835919281,7.42976765700797));
#97953=CARTESIAN_POINT('Origin',(-0.0308560152958731,2.94642874674394,-0.190428015592459));
#97954=CARTESIAN_POINT('Ctrl Pts',(0.991263375971088,2.87870320295771,7.18191457174582));
#97955=CARTESIAN_POINT('Ctrl Pts',(0.996664707981171,2.8855524874312,7.22317185808551));
#97956=CARTESIAN_POINT('Ctrl Pts',(1.00209693091953,2.89224022486283,7.26447634427217));
#97957=CARTESIAN_POINT('Ctrl Pts',(1.01300515576209,2.90530189631038,7.34708089317344));
#97958=CARTESIAN_POINT('Ctrl Pts',(1.01848712055922,2.91168295820948,7.38842607981061));
#97959=CARTESIAN_POINT('Ctrl Pts',(1.02398863947782,2.91791835924874,7.42976764558548));
#97960=CARTESIAN_POINT('Ctrl Pts',(0.431161610006125,3.01309343448858,7.48817560015396));
#97961=CARTESIAN_POINT('Ctrl Pts',(0.445293291560477,3.01082632774429,7.48730837269801));
#97962=CARTESIAN_POINT('Ctrl Pts',(0.459424973114821,3.008559221,7.48644114524202));
#97963=CARTESIAN_POINT('Ctrl Pts',(0.869273043783379,2.942808424,7.46128975060442));
#97964=CARTESIAN_POINT('Ctrl Pts',(1.27392616357086,2.877933005,7.39154817729766));
#97965=CARTESIAN_POINT('Ctrl Pts',(0.178686009798803,3.01309343448857,7.24784936885774));
#97966=CARTESIAN_POINT('Ctrl Pts',(0.192365848399401,3.01082632774429,7.24746042942882));
#97967=CARTESIAN_POINT('Ctrl Pts',(0.206045687,3.008559221,7.24707149000001));
#97968=CARTESIAN_POINT('Ctrl Pts',(0.602789375,2.942808424,7.23579144));
#97969=CARTESIAN_POINT('Ctrl Pts',(0.995930671,2.877933005,7.18126883600001));
#97970=CARTESIAN_POINT('',(0.458902335631921,3.00855922016356,7.48594741351763));
#97971=CARTESIAN_POINT('Origin',(0.0013282379281003,3.08925208342711,-0.189950700615894));
#97972=CARTESIAN_POINT('',(0.332473999383933,3.00855921853322,7.36650945118224));
#97973=CARTESIAN_POINT('Origin',(1.94180609092154E-13,3.10034167700033,
1.34354333214404E-12));
#97974=CARTESIAN_POINT('',(1.02346990113189,3.09925366544343,7.42983912063186));
#97975=CARTESIAN_POINT('Origin',(-0.0278993116907882,3.08928541688475,-0.190850557821854));
#97976=CARTESIAN_POINT('Origin',(-0.00170107075175882,2.94644892730587,
-0.190812579955236));
#97977=CARTESIAN_POINT('Origin',(1.23451663930525E-13,3.10034167700011,
-6.50521303491303E-15));
#97978=CARTESIAN_POINT('',(-0.0328302415903184,3.00855922118746,7.49992815038451));
#97979=CARTESIAN_POINT('Origin',(0.0108017888965188,2.94642871640652,-0.192608996549439));
#97980=CARTESIAN_POINT('',(-0.597654043017233,3.09925366546969,7.47614938614295));
#97981=CARTESIAN_POINT('Origin',(0.0137802093178851,3.08928541963158,-0.192386424768728));
#97982=CARTESIAN_POINT('Origin',(0.0393577271373455,2.94644892036822,-0.186716823481069));
#97983=CARTESIAN_POINT('Ctrl Pts',(-0.848007020840001,2.877925369,7.45446048832));
#97984=CARTESIAN_POINT('Ctrl Pts',(-0.44291711145,2.943232886,7.50054284272));
#97985=CARTESIAN_POINT('Ctrl Pts',(-0.03521899321,3.008559221,7.50245671155));
#97986=CARTESIAN_POINT('Ctrl Pts',(-0.845358323000001,2.877925369,7.452205667));
#97987=CARTESIAN_POINT('Ctrl Pts',(-0.440390945,2.943232886,7.498144086));
#97988=CARTESIAN_POINT('Ctrl Pts',(-0.032830234,3.008559221,7.499928145));
#97989=CARTESIAN_POINT('Ctrl Pts',(-0.580488539,2.877925369,7.226723535));
#97990=CARTESIAN_POINT('Ctrl Pts',(-0.1877743,2.943232886,7.258268414));
#97991=CARTESIAN_POINT('Ctrl Pts',(0.206045687,3.008559221,7.24707149));
#97992=CARTESIAN_POINT('',(0.0866077233954782,3.00855922150568,7.37349981753647));
#97993=CARTESIAN_POINT('Ctrl Pts',(-0.029340091,2.749235821,7.49994261));
#97994=CARTESIAN_POINT('Ctrl Pts',(0.377052547,2.813580595,7.501532435));
#97995=CARTESIAN_POINT('Ctrl Pts',(0.781237513,2.878703203,7.459200222));
#97996=CARTESIAN_POINT('Ctrl Pts',(0.209418136,2.749235821,7.24697482));
#97997=CARTESIAN_POINT('Ctrl Pts',(0.602103436,2.813580595,7.23562726800001));
#97998=CARTESIAN_POINT('Ctrl Pts',(0.991263375,2.878703203,7.181914572));
#97999=CARTESIAN_POINT('',(0.21408150377158,2.75000000010809,7.24683856069753));
#98000=CARTESIAN_POINT('Origin',(-0.0379385088426389,2.94638854356868,-0.192403914175406));
#98001=CARTESIAN_POINT('Ctrl Pts',(0.214081499285152,2.75000000023897,7.24683856080862));
#98002=CARTESIAN_POINT('Ctrl Pts',(0.215310080966762,2.75681548608773,7.28842710418195));
#98003=CARTESIAN_POINT('Ctrl Pts',(0.216481064139149,2.76346377140411,7.33007120365252));
#98004=CARTESIAN_POINT('Ctrl Pts',(0.218715591036004,2.77643548664992,7.41336050560333));
#98005=CARTESIAN_POINT('Ctrl Pts',(0.219780458532496,2.78276663813192,7.45505532086176));
#98006=CARTESIAN_POINT('Ctrl Pts',(0.220796264044522,2.78894740126139,7.49674922945488));
#98007=CARTESIAN_POINT('Ctrl Pts',(1.26042412866189,2.88000589655946,7.39333476721524));
#98008=CARTESIAN_POINT('Ctrl Pts',(1.26448657633095,2.87935454977973,7.39263760060762));
#98009=CARTESIAN_POINT('Ctrl Pts',(1.268549024,2.878703203,7.391940434));
#98010=CARTESIAN_POINT('Ctrl Pts',(1.448039577,2.84992484,7.36113762));
#98011=CARTESIAN_POINT('Ctrl Pts',(1.625823574,2.821428571,7.321659491));
#98012=CARTESIAN_POINT('Ctrl Pts',(1.849718912,2.785541304,7.27194203));
#98013=CARTESIAN_POINT('Ctrl Pts',(2.070158035,2.7492206,7.208636883));
#98014=CARTESIAN_POINT('Ctrl Pts',(0.983369330860882,2.88000589655946,7.18300412502963));
#98015=CARTESIAN_POINT('Ctrl Pts',(0.987316352930441,2.87935454977973,7.18245934851482));
#98016=CARTESIAN_POINT('Ctrl Pts',(0.991263374999999,2.878703203,7.181914572));
#98017=CARTESIAN_POINT('Ctrl Pts',(1.165654095,2.84992484,7.157844788));
#98018=CARTESIAN_POINT('Ctrl Pts',(1.338671059,2.821428571,7.125339276));
#98019=CARTESIAN_POINT('Ctrl Pts',(1.556562952,2.785541304,7.084402899));
#98020=CARTESIAN_POINT('Ctrl Pts',(1.771546394,2.7492206,7.030229255));
#98021=CARTESIAN_POINT('',(1.76693247181021,2.75000000024246,7.03139031398057));
#98022=CARTESIAN_POINT('Ctrl Pts',(1.76693247079244,2.75000000016349,7.03139031557349));
#98023=CARTESIAN_POINT('Ctrl Pts',(1.554222808,2.785926731,7.08484255300001));
#98024=CARTESIAN_POINT('Ctrl Pts',(1.338671059,2.821428571,7.125339276));
#98025=CARTESIAN_POINT('Ctrl Pts',(1.16565409579847,2.84992483975151,7.15784478833025));
#98026=CARTESIAN_POINT('Ctrl Pts',(0.991263377398236,2.8787032050476,7.1819145845472));
#98027=CARTESIAN_POINT('Ctrl Pts',(1.82721365293106,2.78894740126369,7.27401472802548));
#98028=CARTESIAN_POINT('Ctrl Pts',(1.81725845690575,2.78276652545196,7.23351322969728));
#98029=CARTESIAN_POINT('Ctrl Pts',(1.80725542864887,2.77643543151709,7.19302252590466));
#98030=CARTESIAN_POINT('Ctrl Pts',(1.7871684916059,2.7634637717899,7.11216118491727));
#98031=CARTESIAN_POINT('Ctrl Pts',(1.77707263610211,2.75681548728098,7.07174243303508));
#98032=CARTESIAN_POINT('Ctrl Pts',(1.766932470127,2.75000000123112,7.03139031423657));
#98033=CARTESIAN_POINT('Ctrl Pts',(1.583611829,2.749235821,7.330905372));
#98034=CARTESIAN_POINT('Ctrl Pts',(1.980844998,2.813580595,7.24509562400001));
#98035=CARTESIAN_POINT('Ctrl Pts',(2.36648017,2.878703203,7.116865294));
#98036=CARTESIAN_POINT('Ctrl Pts',(1.762407424,2.749235821,7.032525867));
#98037=CARTESIAN_POINT('Ctrl Pts',(2.143472571,2.813580595,6.937027883));
#98038=CARTESIAN_POINT('Ctrl Pts',(2.511987525,2.878703203,6.800913077));
#98039=CARTESIAN_POINT('Origin',(-0.0784132692517919,2.94638885126936,-0.179751477231472));
#98040=CARTESIAN_POINT('Ctrl Pts',(2.82030454263079,2.88000589655946,6.94952877882882));
#98041=CARTESIAN_POINT('Ctrl Pts',(2.8241221423154,2.87935454977973,6.94797460541441));
#98042=CARTESIAN_POINT('Ctrl Pts',(2.827939742,2.878703203,6.946420432));
#98043=CARTESIAN_POINT('Ctrl Pts',(2.996612211,2.84992484,6.877752607));
#98044=CARTESIAN_POINT('Ctrl Pts',(3.161753086,2.821428571,6.800979152));
#98045=CARTESIAN_POINT('Ctrl Pts',(3.369726091,2.785541304,6.704293178));
#98046=CARTESIAN_POINT('Ctrl Pts',(3.571402735,2.7492206,6.595080174));
#98047=CARTESIAN_POINT('Ctrl Pts',(2.50451226091208,2.88000589655946,6.8036741430437));
#98048=CARTESIAN_POINT('Ctrl Pts',(2.50824989295604,2.87935454977973,6.80229361002185));
#98049=CARTESIAN_POINT('Ctrl Pts',(2.511987525,2.878703203,6.800913077));
#98050=CARTESIAN_POINT('Ctrl Pts',(2.677126795,2.84992484,6.739917181));
#98051=CARTESIAN_POINT('Ctrl Pts',(2.839110994,2.821428571,6.670978097));
#98052=CARTESIAN_POINT('Ctrl Pts',(3.043108585,2.785541304,6.584158473));
#98053=CARTESIAN_POINT('Ctrl Pts',(3.241420102,2.7492206,6.485036293));
#98054=CARTESIAN_POINT('',(3.2371636440605,2.75000000044536,6.48716206480851));
#98055=CARTESIAN_POINT('Ctrl Pts',(3.23716364325933,2.75000000162247,6.48716206668083));
#98056=CARTESIAN_POINT('Ctrl Pts',(3.040917665,2.785926731,6.58509091));
#98057=CARTESIAN_POINT('Ctrl Pts',(2.839110994,2.821428571,6.670978097));
#98058=CARTESIAN_POINT('Ctrl Pts',(2.67712679515999,2.84992483971241,6.73991718073424));
#98059=CARTESIAN_POINT('Ctrl Pts',(2.51198753070824,2.87870320492457,6.80091308879405));
#98060=CARTESIAN_POINT('Ctrl Pts',(3.34819256082345,2.7889474012859,6.71115538278797));
#98061=CARTESIAN_POINT('Ctrl Pts',(3.32976346314604,2.78276651747819,6.67374081136571));
#98062=CARTESIAN_POINT('Ctrl Pts',(3.31129000853237,2.77643542761869,6.63634713883759));
#98063=CARTESIAN_POINT('Ctrl Pts',(3.27428990639928,2.76346377185177,6.56169441127519));
#98064=CARTESIAN_POINT('Ctrl Pts',(3.25574124988583,2.75681548744549,6.52439093826907));
#98065=CARTESIAN_POINT('Ctrl Pts',(3.2371636426348,2.7500000013915,6.48716206534674));
#98066=CARTESIAN_POINT('Ctrl Pts',(3.122515819,2.749235821,6.819083146));
#98067=CARTESIAN_POINT('Ctrl Pts',(3.492015338,2.813580595,6.649886193));
#98068=CARTESIAN_POINT('Ctrl Pts',(3.841068843,2.878703203,6.441753654));
#98069=CARTESIAN_POINT('Ctrl Pts',(3.232988499,2.749235821,6.489243821));
#98070=CARTESIAN_POINT('Ctrl Pts',(3.584615312,2.813580595,6.314060784));
#98071=CARTESIAN_POINT('Ctrl Pts',(3.91525393,2.878703203,6.101908444));
#98072=CARTESIAN_POINT('Origin',(-0.115221125141765,2.94638888321458,-0.158692166271711));
#98073=CARTESIAN_POINT('Ctrl Pts',(4.24831064998266,2.88000589655946,6.18077054856216));
#98074=CARTESIAN_POINT('Ctrl Pts',(4.25170489499133,2.87935454977973,6.17843203978108));
#98075=CARTESIAN_POINT('Ctrl Pts',(4.25509914,2.878703203,6.176093531));
#98076=CARTESIAN_POINT('Ctrl Pts',(4.405066589,2.84992484,6.072771527));
#98077=CARTESIAN_POINT('Ctrl Pts',(4.549842538,2.821428571,5.962292586));
#98078=CARTESIAN_POINT('Ctrl Pts',(4.732168624,2.785541304,5.823159028));
#98079=CARTESIAN_POINT('Ctrl Pts',(4.905652612,2.7492206,5.673144847));
#98080=CARTESIAN_POINT('Ctrl Pts',(3.90854698097101,2.88000589655946,6.10621191864682));
#98081=CARTESIAN_POINT('Ctrl Pts',(3.9119004554855,2.87935454977973,6.1040601813234));
#98082=CARTESIAN_POINT('Ctrl Pts',(3.91525393,2.878703203,6.101908444));
#98083=CARTESIAN_POINT('Ctrl Pts',(4.063420022,2.84992484,6.006838537));
#98084=CARTESIAN_POINT('Ctrl Pts',(4.206797255,2.821428571,5.904689396));
#98085=CARTESIAN_POINT('Ctrl Pts',(4.387361843,2.785541304,5.776046115));
#98086=CARTESIAN_POINT('Ctrl Pts',(4.559728608,2.7492206,5.63661024200001));
#98087=CARTESIAN_POINT('',(4.55602864185247,2.75000000024269,5.63960132672671));
#98088=CARTESIAN_POINT('Ctrl Pts',(4.55602864156567,2.75000000016349,5.6396013285999));
#98089=CARTESIAN_POINT('Ctrl Pts',(4.385422592,2.785926731,5.777427735));
#98090=CARTESIAN_POINT('Ctrl Pts',(4.206797255,2.821428571,5.904689396));
#98091=CARTESIAN_POINT('Ctrl Pts',(4.06342002219976,2.84992483978415,6.00683853671871));
#98092=CARTESIAN_POINT('Ctrl Pts',(3.91525393793725,2.87870320492457,6.10190845425346));
#98093=CARTESIAN_POINT('Ctrl Pts',(4.71261370641487,2.78894740132361,5.83448987095168));
#98094=CARTESIAN_POINT('Ctrl Pts',(4.68657244114061,2.78276651684776,5.80191173920188));
#98095=CARTESIAN_POINT('Ctrl Pts',(4.66049235275823,2.77643542728415,5.76936355833918));
#98096=CARTESIAN_POINT('Ctrl Pts',(4.60830916401841,2.763463771782,5.70441009966584));
#98097=CARTESIAN_POINT('Ctrl Pts',(4.58217502077462,2.75681548733964,5.67196617377621));
#98098=CARTESIAN_POINT('Ctrl Pts',(4.55602864065931,2.75000000128407,5.63960132747132));
#98099=CARTESIAN_POINT('Ctrl Pts',(4.51541444,2.749235821,5.988408172));
#98100=CARTESIAN_POINT('Ctrl Pts',(4.839902922,2.813580595,5.743735475));
#98101=CARTESIAN_POINT('Ctrl Pts',(5.136053407,2.878703203,5.465432773));
#98102=CARTESIAN_POINT('Ctrl Pts',(4.552398626,2.749235821,5.642531945));
#98103=CARTESIAN_POINT('Ctrl Pts',(4.858145424,2.813580595,5.39585522));
#98104=CARTESIAN_POINT('Ctrl Pts',(5.135447414,2.878703203,5.117585355));
#98105=CARTESIAN_POINT('Origin',(-0.14664156078291,2.94638884551593,-0.130213051369702));
#98106=CARTESIAN_POINT('Ctrl Pts',(5.47767047366261,2.88000589655946,5.12300635715573));
#98107=CARTESIAN_POINT('Ctrl Pts',(5.48048265283131,2.87935454977973,5.11999285907787));
#98108=CARTESIAN_POINT('Ctrl Pts',(5.483294832,2.878703203,5.116979361));
#98109=CARTESIAN_POINT('Ctrl Pts',(5.607544948,2.84992484,4.98383440000001));
#98110=CARTESIAN_POINT('Ctrl Pts',(5.72518641,2.821428571,4.844815845));
#98111=CARTESIAN_POINT('Ctrl Pts',(5.87334021100001,2.785541304,4.669740434));
#98112=CARTESIAN_POINT('Ctrl Pts',(6.01051962500001,2.7492206,4.485939572));
#98113=CARTESIAN_POINT('Ctrl Pts',(5.12982238961246,2.88000589655946,5.12323001261221));
#98114=CARTESIAN_POINT('Ctrl Pts',(5.13263490180623,2.87935454977973,5.12040768380611));
#98115=CARTESIAN_POINT('Ctrl Pts',(5.135447414,2.878703203,5.117585355));
#98116=CARTESIAN_POINT('Ctrl Pts',(5.259712244,2.84992484,4.992886799));
#98117=CARTESIAN_POINT('Ctrl Pts',(5.377778351,2.821428571,4.862303981));
#98118=CARTESIAN_POINT('Ctrl Pts',(5.526466937,2.785541304,4.69785226000001));
#98119=CARTESIAN_POINT('Ctrl Pts',(5.664829272,2.7492206,4.524622561));
#98120=CARTESIAN_POINT('',(5.66185880360023,2.75000000045047,4.52833909919778));
#98121=CARTESIAN_POINT('Ctrl Pts',(5.66185880364956,2.75000000162248,4.52833910122305));
#98122=CARTESIAN_POINT('Ctrl Pts',(5.524870032,2.785926731,4.69961846000001));
#98123=CARTESIAN_POINT('Ctrl Pts',(5.377778351,2.821428571,4.862303981));
#98124=CARTESIAN_POINT('Ctrl Pts',(5.2597122443229,2.84992483969487,4.99288679854226));
#98125=CARTESIAN_POINT('Ctrl Pts',(5.13544742381051,2.87870320490793,5.11758536321659));
#98126=CARTESIAN_POINT('Ctrl Pts',(5.85667827296398,2.788947401284,4.6850100969931));
#98127=CARTESIAN_POINT('Ctrl Pts',(5.82424314032519,2.78276663833772,4.65879224167537));
#98128=CARTESIAN_POINT('Ctrl Pts',(5.79177555452673,2.77643548702863,4.632611192457));
#98129=CARTESIAN_POINT('Ctrl Pts',(5.72684900691137,2.76346377178021,4.58039391214018));
#98130=CARTESIAN_POINT('Ctrl Pts',(5.69435138024918,2.7568154873266,4.5543265754526));
#98131=CARTESIAN_POINT('Ctrl Pts',(5.66185880267492,2.75000000127586,4.52833910013824));
#98132=CARTESIAN_POINT('Ctrl Pts',(5.697177301,2.749235821,4.877721886));
#98133=CARTESIAN_POINT('Ctrl Pts',(5.961482025,2.813580595,4.56901407));
#98134=CARTESIAN_POINT('Ctrl Pts',(6.190881822,2.878703203,4.23355433));
#98135=CARTESIAN_POINT('Ctrl Pts',(5.658943652,2.749235821,4.531981548));
#98136=CARTESIAN_POINT('Ctrl Pts',(5.90451405500001,2.813580595,4.225345463));
#98137=CARTESIAN_POINT('Ctrl Pts',(6.115513083,2.878703203,3.893969662));
#98138=CARTESIAN_POINT('Origin',(-0.171205151932938,2.94638883973356,-0.0956451587712737));
#98139=CARTESIAN_POINT('Ctrl Pts',(6.45090051407246,2.88000589655946,3.82569608212552));
#98140=CARTESIAN_POINT('Ctrl Pts',(6.45299913303623,2.87935454977973,3.82214850256276));
#98141=CARTESIAN_POINT('Ctrl Pts',(6.455097752,2.878703203,3.818600923));
#98142=CARTESIAN_POINT('Ctrl Pts',(6.54782073800001,2.84992484,3.661858715));
#98143=CARTESIAN_POINT('Ctrl Pts',(6.632826928,2.821428571,3.5008009));
#98144=CARTESIAN_POINT('Ctrl Pts',(6.739880937,2.785541304,3.297969967));
#98145=CARTESIAN_POINT('Ctrl Pts',(6.834341421,2.7492206,3.088976748));
#98146=CARTESIAN_POINT('Ctrl Pts',(6.11123300303657,2.88000589655946,3.90069156461084));
#98147=CARTESIAN_POINT('Ctrl Pts',(6.11337304301828,2.87935454977973,3.89733061330542));
#98148=CARTESIAN_POINT('Ctrl Pts',(6.115513083,2.878703203,3.893969662));
#98149=CARTESIAN_POINT('Ctrl Pts',(6.210066168,2.84992484,3.745473224));
#98150=CARTESIAN_POINT('Ctrl Pts',(6.297300509,2.821428571,3.592562637));
#98151=CARTESIAN_POINT('Ctrl Pts',(6.40716058,2.785541304,3.399992054));
#98152=CARTESIAN_POINT('Ctrl Pts',(6.50504881499999,2.7492206,3.201068558));
#98153=CARTESIAN_POINT('',(6.50294674171202,2.75000000026814,3.2053367675602));
#98154=CARTESIAN_POINT('Ctrl Pts',(6.50294674267293,2.75,3.20533676908474));
#98155=CARTESIAN_POINT('Ctrl Pts',(6.40598069,2.785926731,3.402060249));
#98156=CARTESIAN_POINT('Ctrl Pts',(6.297300509,2.821428571,3.592562637));
#98157=CARTESIAN_POINT('Ctrl Pts',(6.2100661683652,2.8499248397502,3.74547322388404));
#98158=CARTESIAN_POINT('Ctrl Pts',(6.11551309476877,2.87870320492457,3.89396966791537));
#98159=CARTESIAN_POINT('Ctrl Pts',(6.72689107244661,2.78894740126306,3.31646445774121));
#98160=CARTESIAN_POINT('Ctrl Pts',(6.68957747469991,2.78276651961456,3.29783179824251));
#98161=CARTESIAN_POINT('Ctrl Pts',(6.65224119222599,2.77643542866125,3.27924260987598));
#98162=CARTESIAN_POINT('Ctrl Pts',(6.57760775536984,2.76346377180691,3.2422035959284));
#98163=CARTESIAN_POINT('Ctrl Pts',(6.54026619878664,2.75681548744809,3.22373172855374));
#98164=CARTESIAN_POINT('Ctrl Pts',(6.50294674040865,2.75000000137438,3.2053367697946));
#98165=CARTESIAN_POINT('Ctrl Pts',(6.612546483,2.749235821,3.538958747));
#98166=CARTESIAN_POINT('Ctrl Pts',(6.804308854,2.813580595,3.180650644));
#98167=CARTESIAN_POINT('Ctrl Pts',(6.956231483,2.878703203,2.803719592));
#98168=CARTESIAN_POINT('Ctrl Pts',(6.500882762,2.749235821,3.209520729));
#98169=CARTESIAN_POINT('Ctrl Pts',(6.674794172,2.813580595,2.857263248));
#98170=CARTESIAN_POINT('Ctrl Pts',(6.809624158,2.878703203,2.488276275));
#98171=CARTESIAN_POINT('Origin',(-0.187763342433521,2.94638886487291,-0.0566049644485317));
#98172=CARTESIAN_POINT('Ctrl Pts',(7.122493615628,2.88000589655946,2.34950051031494));
#98173=CARTESIAN_POINT('Ctrl Pts',(7.123780545314,2.87935454977973,2.34558473015747));
#98174=CARTESIAN_POINT('Ctrl Pts',(7.125067475,2.878703203,2.34166895));
#98175=CARTESIAN_POINT('Ctrl Pts',(7.181927708,2.84992484,2.168658587));
#98176=CARTESIAN_POINT('Ctrl Pts',(7.230323831,2.821428571,1.993092396));
#98177=CARTESIAN_POINT('Ctrl Pts',(7.291272322,2.785541304,1.77199009));
#98178=CARTESIAN_POINT('Ctrl Pts',(7.338597007,2.7492206,1.547576804));
#98179=CARTESIAN_POINT('Ctrl Pts',(6.80688915428054,2.88000589655946,2.49576111393228));
#98180=CARTESIAN_POINT('Ctrl Pts',(6.80825665614027,2.87935454977973,2.49201869446614));
#98181=CARTESIAN_POINT('Ctrl Pts',(6.809624158,2.878703203,2.488276275));
#98182=CARTESIAN_POINT('Ctrl Pts',(6.87004430000001,2.84992484,2.322925483));
#98183=CARTESIAN_POINT('Ctrl Pts',(6.922367894,2.821428571,2.154837056));
#98184=CARTESIAN_POINT('Ctrl Pts',(6.988262514,2.785541304,1.943151999));
#98185=CARTESIAN_POINT('Ctrl Pts',(7.041099506,2.7492206,1.727836146));
#98186=CARTESIAN_POINT('',(7.03996411640098,2.75000000026578,1.73245645140282));
#98187=CARTESIAN_POINT('Ctrl Pts',(7.03996411761487,2.75,1.73245645286228));
#98188=CARTESIAN_POINT('Ctrl Pts',(6.987554811,2.785926731,1.945425482));
#98189=CARTESIAN_POINT('Ctrl Pts',(6.922367894,2.821428571,2.154837056));
#98190=CARTESIAN_POINT('Ctrl Pts',(6.87004429936856,2.84992483969281,2.32292548252339));
#98191=CARTESIAN_POINT('Ctrl Pts',(6.80962417063931,2.87870320490785,2.48827627862319));
#98192=CARTESIAN_POINT('Ctrl Pts',(7.28256192157162,2.78894740128486,1.79284462688592));
#98193=CARTESIAN_POINT('Ctrl Pts',(7.24211600089717,2.78276663836325,1.78266910448061));
#98194=CARTESIAN_POINT('Ctrl Pts',(7.20165608093829,2.77643548706781,1.77254061309088));
#98195=CARTESIAN_POINT('Ctrl Pts',(7.12080487551314,2.76346377184109,1.75241144266078));
#98196=CARTESIAN_POINT('Ctrl Pts',(7.0803654380908,2.75681548742949,1.74239876794969));
#98197=CARTESIAN_POINT('Ctrl Pts',(7.03996411571497,2.7500000013588,1.73245645344123));
#98198=CARTESIAN_POINT('Ctrl Pts',(7.21872034,2.749235821,2.03471783));
#98199=CARTESIAN_POINT('Ctrl Pts',(7.328973763,2.813580595,1.64356353));
#98200=CARTESIAN_POINT('Ctrl Pts',(7.396315492,2.878703203,1.242786042));
#98201=CARTESIAN_POINT('Ctrl Pts',(7.03884782,2.749235821,1.736986289));
#98202=CARTESIAN_POINT('Ctrl Pts',(7.132968332,2.813580595,1.35557858));
#98203=CARTESIAN_POINT('Ctrl Pts',(7.185324776,2.878703203,0.966233856));
#98204=CARTESIAN_POINT('Origin',(-0.19554187319157,2.94638884092586,-0.0149179997582567));
#98205=CARTESIAN_POINT('Ctrl Pts',(7.46104683197357,2.88000589655946,0.763444906506437));
#98206=CARTESIAN_POINT('Ctrl Pts',(7.46146189698679,2.87935454977973,0.759344023253219));
#98207=CARTESIAN_POINT('Ctrl Pts',(7.461876962,2.878703203,0.75524314));
#98208=CARTESIAN_POINT('Ctrl Pts',(7.480215721,2.84992484,0.574054393));
#98209=CARTESIAN_POINT('Ctrl Pts',(7.489738828,2.821428571,0.392189107));
#98210=CARTESIAN_POINT('Ctrl Pts',(7.501731916,2.785541304,0.163153925));
#98211=CARTESIAN_POINT('Ctrl Pts',(7.499707954,2.7492206,-0.066186111));
#98212=CARTESIAN_POINT('Ctrl Pts',(7.18426273431808,2.88000589655946,0.974131648515827));
#98213=CARTESIAN_POINT('Ctrl Pts',(7.18479375515905,2.87935454977973,0.970182752257913));
#98214=CARTESIAN_POINT('Ctrl Pts',(7.185324776,2.878703203,0.966233856));
#98215=CARTESIAN_POINT('Ctrl Pts',(7.208786795,2.84992484,0.791760329));
#98216=CARTESIAN_POINT('Ctrl Pts',(7.22375305,2.821428571,0.616353689));
#98217=CARTESIAN_POINT('Ctrl Pts',(7.242601061,2.785541304,0.395452316));
#98218=CARTESIAN_POINT('Ctrl Pts',(7.247916209,2.7492206,0.173812037));
#98219=CARTESIAN_POINT('',(7.24780059356986,2.75000000025782,0.178568397596697));
#98220=CARTESIAN_POINT('Ctrl Pts',(7.24780059505537,2.75,0.178568398956853));
#98221=CARTESIAN_POINT('Ctrl Pts',(7.242398635,2.785926731,0.397824782));
#98222=CARTESIAN_POINT('Ctrl Pts',(7.22375305,2.821428571,0.616353689));
#98223=CARTESIAN_POINT('Ctrl Pts',(7.20878679508297,2.84992483970705,0.791760328629913));
#98224=CARTESIAN_POINT('Ctrl Pts',(7.18532478887201,2.87870320490792,0.96623385656718));
#98225=CARTESIAN_POINT('Ctrl Pts',(7.49770826955606,2.78894740128533,0.185393373255829));
#98226=CARTESIAN_POINT('Ctrl Pts',(7.45601972509689,2.78276652118434,0.184150402711579));
#98227=CARTESIAN_POINT('Ctrl Pts',(7.41432882982761,2.776435429465,0.182956410174987));
#98228=CARTESIAN_POINT('Ctrl Pts',(7.33104107382006,2.76346377183417,0.180678478153404));
#98229=CARTESIAN_POINT('Ctrl Pts',(7.28939465918434,2.75681548747345,0.179593178041244));
#98230=CARTESIAN_POINT('Ctrl Pts',(7.24780059333909,2.75000000138697,0.17856839945361));
#98231=CARTESIAN_POINT('Ctrl Pts',(7.48735485800001,2.749235821,0.435335768));
#98232=CARTESIAN_POINT('Ctrl Pts',(7.510944005,2.813580595,0.029625212));
#98233=CARTESIAN_POINT('Ctrl Pts',(7.490556008,2.878703203,-0.376258802));
#98234=CARTESIAN_POINT('Ctrl Pts',(7.247684177,2.749235821,0.183232301));
#98235=CARTESIAN_POINT('Ctrl Pts',(7.25761282,2.813580595,-0.209491436));
#98236=CARTESIAN_POINT('Ctrl Pts',(7.22504759300001,2.878703203,-0.600988584999999));
#98237=CARTESIAN_POINT('Origin',(-0.194177019746913,2.94638878624266,0.0274664884888842));
#98238=CARTESIAN_POINT('Ctrl Pts',(7.4507297913676,2.88000589655946,-0.858308532813974));
#98239=CARTESIAN_POINT('Ctrl Pts',(7.4502535836838,2.87935454977973,-0.862402766406987));
#98240=CARTESIAN_POINT('Ctrl Pts',(7.449777376,2.878703203,-0.866497000000001));
#98241=CARTESIAN_POINT('Ctrl Pts',(7.428737159,2.84992484,-1.047391946));
#98242=CARTESIAN_POINT('Ctrl Pts',(7.398941961,2.821428571,-1.227052509));
#98243=CARTESIAN_POINT('Ctrl Pts',(7.361418864,2.785541304,-1.453311135));
#98244=CARTESIAN_POINT('Ctrl Pts',(7.310140893,2.7492206,-1.676854237));
#98245=CARTESIAN_POINT('Ctrl Pts',(7.22570817320211,2.88000589655946,-0.59304713093671));
#98246=CARTESIAN_POINT('Ctrl Pts',(7.22537788310106,2.87935454977973,-0.597017857968355));
#98247=CARTESIAN_POINT('Ctrl Pts',(7.22504759300001,2.878703203,-0.600988585));
#98248=CARTESIAN_POINT('Ctrl Pts',(7.210454432,2.84992484,-0.776426658));
#98249=CARTESIAN_POINT('Ctrl Pts',(7.187363542,2.821428571,-0.95094969));
#98250=CARTESIAN_POINT('Ctrl Pts',(7.158283632,2.785541304,-1.170738277));
#98251=CARTESIAN_POINT('Ctrl Pts',(7.115828406,2.7492206,-1.38833933));
#98252=CARTESIAN_POINT('',(7.11673797040537,2.75000000043277,-1.38366931702854));
#98253=CARTESIAN_POINT('Ctrl Pts',(7.1167379718967,2.75000000141664,-1.38366931622182));
#98254=CARTESIAN_POINT('Ctrl Pts',(7.14471280398305,2.77401081869193,-1.23978407374445));
#98255=CARTESIAN_POINT('Ctrl Pts',(7.16825029397474,2.79784107588195,-1.09540934537186));
#98256=CARTESIAN_POINT('Ctrl Pts',(7.18736354220351,2.82142857104559,-0.950949689938156));
#98257=CARTESIAN_POINT('Ctrl Pts',(7.20271546736448,2.84037424985117,-0.834918454286328));
#98258=CARTESIAN_POINT('Ctrl Pts',(7.21529795469166,2.85947647450026,-0.718198182562453));
#98259=CARTESIAN_POINT('Ctrl Pts',(7.22504760539514,2.8787032049138,-0.600988586830895));
#98260=CARTESIAN_POINT('Ctrl Pts',(7.36227011198848,2.78894740127213,-1.43072666782516));
#98261=CARTESIAN_POINT('Ctrl Pts',(7.32128900964024,2.7827665194972,-1.42297877156182));
#98262=CARTESIAN_POINT('Ctrl Pts',(7.28031615707141,2.77643542860496,-1.41518254022359));
#98263=CARTESIAN_POINT('Ctrl Pts',(7.19848593954923,2.76346377177154,-1.39950281104338));
#98264=CARTESIAN_POINT('Ctrl Pts',(7.15757988751625,2.75681548741898,-1.39160998951429));
#98265=CARTESIAN_POINT('Ctrl Pts',(7.11673797065868,2.75000000134449,-1.38366931494318));
#98266=CARTESIAN_POINT('Ctrl Pts',(7.40588898400001,2.749235821,-1.18440211));
#98267=CARTESIAN_POINT('Ctrl Pts',(7.341710853,2.813580595,-1.585698348));
#98268=CARTESIAN_POINT('Ctrl Pts',(7.234546451,2.878703203,-1.977710203));
#98269=CARTESIAN_POINT('Ctrl Pts',(7.117626877,2.749235821,-1.379089427));
#98270=CARTESIAN_POINT('Ctrl Pts',(7.042899399,2.813580595,-1.764765866));
#98271=CARTESIAN_POINT('Ctrl Pts',(6.926935215,2.878703203,-2.140109468));
#98272=CARTESIAN_POINT('Origin',(-0.183732929338554,2.94638880069341,0.0685666915785357));
#98273=CARTESIAN_POINT('Ctrl Pts',(7.09202490579439,2.88000589655946,-2.43992841977617));
#98274=CARTESIAN_POINT('Ctrl Pts',(7.0906796923972,2.87935454977973,-2.44382456188808));
#98275=CARTESIAN_POINT('Ctrl Pts',(7.089334479,2.878703203,-2.447720704));
#98276=CARTESIAN_POINT('Ctrl Pts',(7.029899105,2.84992484,-2.619863402));
#98277=CARTESIAN_POINT('Ctrl Pts',(6.962178791,2.821428571,-2.788918514));
#98278=CARTESIAN_POINT('Ctrl Pts',(6.876894047,2.785541304,-3.001820982));
#98279=CARTESIAN_POINT('Ctrl Pts',(6.778759767,2.7492206,-3.209114522));
#98280=CARTESIAN_POINT('Ctrl Pts',(6.92928752908958,2.88000589655946,-2.13249568594101));
#98281=CARTESIAN_POINT('Ctrl Pts',(6.92811137204479,2.87935454977973,-2.13630257697051));
#98282=CARTESIAN_POINT('Ctrl Pts',(6.926935215,2.878703203,-2.140109468));
#98283=CARTESIAN_POINT('Ctrl Pts',(6.874969234,2.84992484,-2.308308798));
#98284=CARTESIAN_POINT('Ctrl Pts',(6.814900903,2.821428571,-2.47378772));
#98285=CARTESIAN_POINT('Ctrl Pts',(6.73925281500001,2.785541304,-2.68218645));
#98286=CARTESIAN_POINT('Ctrl Pts',(6.651012375,2.7492206,-2.885573493));
#98287=CARTESIAN_POINT('',(6.65290458904496,2.75000000047527,-2.88120819072644));
#98288=CARTESIAN_POINT('Ctrl Pts',(6.65290459080522,2.75000000185147,-2.88120818990272));
#98289=CARTESIAN_POINT('Ctrl Pts',(6.740065271,2.785926731,-2.679948262));
#98290=CARTESIAN_POINT('Ctrl Pts',(6.814900903,2.821428571,-2.47378772));
#98291=CARTESIAN_POINT('Ctrl Pts',(6.87496923456513,2.84992483975882,-2.3083087984779));
#98292=CARTESIAN_POINT('Ctrl Pts',(6.92693522677083,2.8787032050476,-2.14010947208691));
#98293=CARTESIAN_POINT('Ctrl Pts',(6.88258038601945,2.78894740126168,-2.97994752053213));
#98294=CARTESIAN_POINT('Ctrl Pts',(6.84422299668878,2.78276652415432,-2.96357105245644));
#98295=CARTESIAN_POINT('Ctrl Pts',(6.80588401050304,2.77643543089794,-2.94714913391392));
#98296=CARTESIAN_POINT('Ctrl Pts',(6.72933760291006,2.76346377181668,-2.91424490424444));
#98297=CARTESIAN_POINT('Ctrl Pts',(6.69108463461263,2.75681548741193,-2.89774302018045));
#98298=CARTESIAN_POINT('Ctrl Pts',(6.65290458957586,2.75000000137046,-2.88120818913158));
#98299=CARTESIAN_POINT('Ctrl Pts',(6.978131972,2.749235821,-2.748758662));
#98300=CARTESIAN_POINT('Ctrl Pts',(6.829187461,2.813580595,-3.126876416));
#98301=CARTESIAN_POINT('Ctrl Pts',(6.640257542,2.878703203,-3.486686073));
#98302=CARTESIAN_POINT('Ctrl Pts',(6.654757254,2.749235821,-2.876926465));
#98303=CARTESIAN_POINT('Ctrl Pts',(6.49886783,2.813580595,-3.237521805));
#98304=CARTESIAN_POINT('Ctrl Pts',(6.304927044,2.878703203,-3.57916121));
#98305=CARTESIAN_POINT('Origin',(-0.164697410767518,2.94638883839802,0.106460730702383));
#98306=CARTESIAN_POINT('Ctrl Pts',(6.40170481785586,2.88000589655946,-3.90745996532277));
#98307=CARTESIAN_POINT('Ctrl Pts',(6.39955349942792,2.87935454977973,-3.91097583666138));
#98308=CARTESIAN_POINT('Ctrl Pts',(6.397402181,2.878703203,-3.914491708));
#98309=CARTESIAN_POINT('Ctrl Pts',(6.302350782,2.84992484,-4.069832956));
#98310=CARTESIAN_POINT('Ctrl Pts',(6.199871879,2.821428571,-4.220377789));
#98311=CARTESIAN_POINT('Ctrl Pts',(6.070813308,2.785541304,-4.409969017));
#98312=CARTESIAN_POINT('Ctrl Pts',(5.93041137,2.7492206,-4.591320179));
#98313=CARTESIAN_POINT('Ctrl Pts',(6.30886110036269,2.88000589655946,-3.5722311118992));
#98314=CARTESIAN_POINT('Ctrl Pts',(6.30689407218134,2.87935454977973,-3.5756961609496));
#98315=CARTESIAN_POINT('Ctrl Pts',(6.304927044,2.878703203,-3.57916121));
#98316=CARTESIAN_POINT('Ctrl Pts',(6.218018115,2.84992484,-3.732256984));
#98317=CARTESIAN_POINT('Ctrl Pts',(6.123781072,2.821428571,-3.880954185));
#98318=CARTESIAN_POINT('Ctrl Pts',(6.005102028,2.785541304,-4.068218566));
#98319=CARTESIAN_POINT('Ctrl Pts',(5.875202398,2.7492206,-4.247881446));
#98320=CARTESIAN_POINT('',(5.87798878412016,2.7500000002675,-4.24402497383028));
#98321=CARTESIAN_POINT('Ctrl Pts',(5.87798878596976,2.74999999999996,-4.24402497389632));
#98322=CARTESIAN_POINT('Ctrl Pts',(6.006376632,2.785926731,-4.06620736));
#98323=CARTESIAN_POINT('Ctrl Pts',(6.123781072,2.821428571,-3.880954185));
#98324=CARTESIAN_POINT('Ctrl Pts',(6.21801811524083,2.84992483970532,-3.73225698449517));
#98325=CARTESIAN_POINT('Ctrl Pts',(6.30492705467579,2.8787032050476,-3.57916121655526));
#98326=CARTESIAN_POINT('Ctrl Pts',(6.08106885136325,2.78894740129956,-4.38982933917005));
#98327=CARTESIAN_POINT('Ctrl Pts',(6.04712868686565,2.78276652304603,-4.36559003441779));
#98328=CARTESIAN_POINT('Ctrl Pts',(6.01321627542074,2.77643543037613,-4.34131030485512));
#98329=CARTESIAN_POINT('Ctrl Pts',(5.94553291982872,2.76346377180304,-4.29272014485417));
#98330=CARTESIAN_POINT('Ctrl Pts',(5.91172170255795,2.75681548751259,-4.26838080876083));
#98331=CARTESIAN_POINT('Ctrl Pts',(5.8779887853427,2.75000000141989,-4.24402497181459));
#98332=CARTESIAN_POINT('Ctrl Pts',(6.224085265,2.749235821,-4.184586314));
#98333=CARTESIAN_POINT('Ctrl Pts',(5.997338854,2.813580595,-4.521845218));
#98334=CARTESIAN_POINT('Ctrl Pts',(5.735477571,2.878703203,-4.832628377));
#98335=CARTESIAN_POINT('Ctrl Pts',(5.88071857899999,2.749235821,-4.24024162));
#98336=CARTESIAN_POINT('Ctrl Pts',(5.650956424,2.813580595,-4.558894822));
#98337=CARTESIAN_POINT('Ctrl Pts',(5.388107493,2.878703203,-4.850855352));
#98338=CARTESIAN_POINT('Origin',(-0.137961245383964,2.94638883689837,0.139377039713766));
#98339=CARTESIAN_POINT('Ctrl Pts',(5.41204812843507,2.88000589655946,-5.19228302529162));
#98340=CARTESIAN_POINT('Ctrl Pts',(5.40919129821753,2.87935454977973,-5.19525422764581));
#98341=CARTESIAN_POINT('Ctrl Pts',(5.406334468,2.878703203,-5.19822543));
#98342=CARTESIAN_POINT('Ctrl Pts',(5.280111541,2.84992484,-5.329501645));
#98343=CARTESIAN_POINT('Ctrl Pts',(5.147665849,2.821428571,-5.454496888));
#98344=CARTESIAN_POINT('Ctrl Pts',(4.980868086,2.785541304,-5.611911801));
#98345=CARTESIAN_POINT('Ctrl Pts',(4.80476352700001,2.7492206,-5.758840808));
#98346=CARTESIAN_POINT('Ctrl Pts',(5.3934393395294,2.88000589655946,-4.84493298157681));
#98347=CARTESIAN_POINT('Ctrl Pts',(5.3907734162647,2.87935454977973,-4.8478941667884));
#98348=CARTESIAN_POINT('Ctrl Pts',(5.388107493,2.878703203,-4.850855352));
#98349=CARTESIAN_POINT('Ctrl Pts',(5.270319381,2.84992484,-4.981688981));
#98350=CARTESIAN_POINT('Ctrl Pts',(5.146320044,2.821428571,-5.106651545));
#98351=CARTESIAN_POINT('Ctrl Pts',(4.990159343,2.785541304,-5.264025303));
#98352=CARTESIAN_POINT('Ctrl Pts',(4.82467448700001,2.7492206,-5.411563184));
#98353=CARTESIAN_POINT('',(4.82822475600757,2.75000000027563,-5.40839586469098));
#98354=CARTESIAN_POINT('Ctrl Pts',(4.82822475768938,2.74999999999996,-5.40839586525515));
#98355=CARTESIAN_POINT('Ctrl Pts',(4.991836498,2.785926731,-5.26233512));
#98356=CARTESIAN_POINT('Ctrl Pts',(5.146320044,2.821428571,-5.106651545));
#98357=CARTESIAN_POINT('Ctrl Pts',(5.27031938038601,2.84992483973463,-4.98168898130263));
#98358=CARTESIAN_POINT('Ctrl Pts',(5.38810750192403,2.87870320504759,-4.8508553615638));
#98359=CARTESIAN_POINT('Ctrl Pts',(4.9952132955519,2.78894740128604,-5.5944476161405));
#98360=CARTESIAN_POINT('Ctrl Pts',(4.96727788840992,2.78276663837147,-5.56347945870876));
#98361=CARTESIAN_POINT('Ctrl Pts',(4.93937747636574,2.77643548707661,-5.53247690297568));
#98362=CARTESIAN_POINT('Ctrl Pts',(4.8837217249102,2.76346377181458,-5.47047256236194));
#98363=CARTESIAN_POINT('Ctrl Pts',(4.85593323279021,2.75681548746043,-5.43943385396049));
#98364=CARTESIAN_POINT('Ctrl Pts',(4.82822475775813,2.75000000134421,-5.40839586289356));
#98365=CARTESIAN_POINT('Ctrl Pts',(5.179007248,2.749235821,-5.42474736));
#98366=CARTESIAN_POINT('Ctrl Pts',(4.88506134700001,2.813580595,-5.705377563));
#98367=CARTESIAN_POINT('Ctrl Pts',(4.562513043,2.878703203,-5.952602349));
#98368=CARTESIAN_POINT('Ctrl Pts',(4.83170403900001,2.749235821,-5.405287789));
#98369=CARTESIAN_POINT('Ctrl Pts',(4.538812577,2.813580595,-5.667098985));
#98370=CARTESIAN_POINT('Ctrl Pts',(4.219346023,2.878703203,-5.895728889));
#98371=CARTESIAN_POINT('Origin',(-0.104773817285174,2.94638886113406,0.165776052385654));
#98372=CARTESIAN_POINT('Ctrl Pts',(4.16933008259264,2.88000589655946,-6.23432070250419));
#98373=CARTESIAN_POINT('Ctrl Pts',(4.16590132279632,2.87935454977973,-6.23660830575209));
#98374=CARTESIAN_POINT('Ctrl Pts',(4.162472563,2.878703203,-6.238895909));
#98375=CARTESIAN_POINT('Ctrl Pts',(4.010980152,2.84992484,-6.339968761));
#98376=CARTESIAN_POINT('Ctrl Pts',(3.854760685,2.821428571,-6.433569776));
#98377=CARTESIAN_POINT('Ctrl Pts',(3.658023008,2.785541304,-6.551447827));
#98378=CARTESIAN_POINT('Ctrl Pts',(3.454450283,2.7492206,-6.65708444));
#98379=CARTESIAN_POINT('Ctrl Pts',(4.2258263484876,2.88000589655946,-5.89109116970949));
#98380=CARTESIAN_POINT('Ctrl Pts',(4.2225861857438,2.87935454977973,-5.89341002935475));
#98381=CARTESIAN_POINT('Ctrl Pts',(4.219346023,2.878703203,-5.895728889));
#98382=CARTESIAN_POINT('Ctrl Pts',(4.076186369,2.84992484,-5.998182738));
#98383=CARTESIAN_POINT('Ctrl Pts',(3.928222811,2.821428571,-6.093567555));
#98384=CARTESIAN_POINT('Ctrl Pts',(3.741882354,2.785541304,-6.213692068));
#98385=CARTESIAN_POINT('Ctrl Pts',(3.548550158,2.7492206,-6.322206243));
#98386=CARTESIAN_POINT('',(3.55269830451331,2.75000000024693,-6.31987617435455));
#98387=CARTESIAN_POINT('Ctrl Pts',(3.55269830625484,2.75000000016345,-6.31987617483064));
#98388=CARTESIAN_POINT('Ctrl Pts',(3.743883638,2.785926731,-6.212401939));
#98389=CARTESIAN_POINT('Ctrl Pts',(3.928222811,2.821428571,-6.093567555));
#98390=CARTESIAN_POINT('Ctrl Pts',(4.0761863682735,2.84992483973599,-5.998182738085));
#98391=CARTESIAN_POINT('Ctrl Pts',(4.21934602997973,2.8787032050476,-5.89572889991465));
#98392=CARTESIAN_POINT('Ctrl Pts',(3.67578711801594,2.78894740127026,-6.53747574106815));
#98393=CARTESIAN_POINT('Ctrl Pts',(3.6551616581691,2.78276651685819,-6.50122560259924));
#98394=CARTESIAN_POINT('Ctrl Pts',(3.63457839151704,2.77643542724564,-6.46495048364397));
#98395=CARTESIAN_POINT('Ctrl Pts',(3.59355312984129,2.76346377175075,-6.39243176256808));
#98396=CARTESIAN_POINT('Ctrl Pts',(3.57308672133439,2.7568154872162,-6.35614501636298));
#98397=CARTESIAN_POINT('Ctrl Pts',(3.55269830576612,2.75000000121139,-6.31987617346905));
#98398=CARTESIAN_POINT('Ctrl Pts',(3.891764609,2.749235821,-6.41125325));
#98399=CARTESIAN_POINT('Ctrl Pts',(3.544363801,2.813580595,-6.622132794));
#98400=CARTESIAN_POINT('Ctrl Pts',(3.176210476,2.878703203,-6.794239252));
#98401=CARTESIAN_POINT('Ctrl Pts',(3.556764388,2.749235821,-6.317588708));
#98402=CARTESIAN_POINT('Ctrl Pts',(3.214438897,2.813580595,-6.510315898));
#98403=CARTESIAN_POINT('Ctrl Pts',(2.853292624,2.878703203,-6.664924696));
#98404=CARTESIAN_POINT('Origin',(-0.0666871484641607,2.94638884487929,0.184423190316368));
#98405=CARTESIAN_POINT('Ctrl Pts',(2.7316587967451,2.88000589655946,-6.98484847227732));
#98406=CARTESIAN_POINT('Ctrl Pts',(2.72781843237254,2.87935454977973,-6.98634551063867));
#98407=CARTESIAN_POINT('Ctrl Pts',(2.723978068,2.878703203,-6.987842549));
#98408=CARTESIAN_POINT('Ctrl Pts',(2.55429979,2.84992484,-7.053985984));
#98409=CARTESIAN_POINT('Ctrl Pts',(2.381611195,2.821428571,-7.111816091));
#98410=CARTESIAN_POINT('Ctrl Pts',(2.164132839,2.785541304,-7.18464543300001));
#98411=CARTESIAN_POINT('Ctrl Pts',(1.942610782,2.7492206,-7.244050203));
#98412=CARTESIAN_POINT('Ctrl Pts',(2.86061841568769,2.88000589655946,-6.66178848243677));
#98413=CARTESIAN_POINT('Ctrl Pts',(2.85695551984384,2.87935454977973,-6.66335658921838));
#98414=CARTESIAN_POINT('Ctrl Pts',(2.853292624,2.878703203,-6.664924696));
#98415=CARTESIAN_POINT('Ctrl Pts',(2.691455413,2.84992484,-6.734208137));
#98416=CARTESIAN_POINT('Ctrl Pts',(2.526446244,2.821428571,-6.795555119));
#98417=CARTESIAN_POINT('Ctrl Pts',(2.318639105,2.785541304,-6.872813497));
#98418=CARTESIAN_POINT('Ctrl Pts',(2.106499568,2.7492206,-6.937229964));
#98419=CARTESIAN_POINT('',(2.11105162895206,2.75000000045156,-6.93584610146047));
#98420=CARTESIAN_POINT('Ctrl Pts',(2.11105163018686,2.75000000149723,-6.93584610247036));
#98421=CARTESIAN_POINT('Ctrl Pts',(2.25127962185001,2.77401081870091,-6.89316514097695));
#98422=CARTESIAN_POINT('Ctrl Pts',(2.38986159184462,2.79784107586595,-6.8463344557346));
#98423=CARTESIAN_POINT('Ctrl Pts',(2.52644624442886,2.82142857108152,-6.79555511891881));
#98424=CARTESIAN_POINT('Ctrl Pts',(2.63615221022049,2.84037424987091,-6.75476871934872));
#98425=CARTESIAN_POINT('Ctrl Pts',(2.74516971923028,2.85947647446867,-6.71121273845926));
#98426=CARTESIAN_POINT('Ctrl Pts',(2.85329262766578,2.87870320485789,-6.66492470846333));
#98427=CARTESIAN_POINT('Ctrl Pts',(2.18448521924249,2.78894740125615,-7.17481876586772));
#98428=CARTESIAN_POINT('Ctrl Pts',(2.17213469480052,2.78276652450666,-7.13498232068391));
#98429=CARTESIAN_POINT('Ctrl Pts',(2.15983072388931,2.77643543109502,-7.09513047430933));
#98430=CARTESIAN_POINT('Ctrl Pts',(2.1353539846267,2.76346377185901,-7.01548795904971));
#98431=CARTESIAN_POINT('Ctrl Pts',(2.123166647678,2.75681548752113,-6.97564990509851));
#98432=CARTESIAN_POINT('Ctrl Pts',(2.11105163107829,2.75000000147961,-6.93584610063728));
#98433=CARTESIAN_POINT('Ctrl Pts',(2.422547381,2.749235821,-7.097976063));
#98434=CARTESIAN_POINT('Ctrl Pts',(2.037935743,2.813580595,-7.22924445600001));
#98435=CARTESIAN_POINT('Ctrl Pts',(1.641391837,2.878703203,-7.318185078));
#98436=CARTESIAN_POINT('Ctrl Pts',(2.115514388,2.749235821,-6.934486201));
#98437=CARTESIAN_POINT('Ctrl Pts',(1.739761628,2.813580595,-7.049117675));
#98438=CARTESIAN_POINT('Ctrl Pts',(1.353822432,2.878703203,-7.12247603199999));
#98439=CARTESIAN_POINT('Origin',(-0.025482542469567,2.9463888725141,0.194447476129106));
#98440=CARTESIAN_POINT('Ctrl Pts',(1.16625818054415,2.88000589655946,-7.40877249081791));
#98441=CARTESIAN_POINT('Ctrl Pts',(1.16218578277208,2.87935454977973,-7.40940896440895));
#98442=CARTESIAN_POINT('Ctrl Pts',(1.158113385,2.878703203,-7.410045438));
#98443=CARTESIAN_POINT('Ctrl Pts',(0.978183208000001,2.84992484,-7.438166661));
#98444=CARTESIAN_POINT('Ctrl Pts',(0.797100213,2.821428571,-7.45752179));
#98445=CARTESIAN_POINT('Ctrl Pts',(0.569050224,2.785541304,-7.481897005));
#98446=CARTESIAN_POINT('Ctrl Pts',(0.33993696,2.7492206,-7.49229223));
#98447=CARTESIAN_POINT('Ctrl Pts',(1.36165114397053,2.88000589655946,-7.12098797003829));
#98448=CARTESIAN_POINT('Ctrl Pts',(1.35773678798527,2.87935454977973,-7.12173200101915));
#98449=CARTESIAN_POINT('Ctrl Pts',(1.353822432,2.878703203,-7.122476032));
#98450=CARTESIAN_POINT('Ctrl Pts',(1.180874993,2.84992484,-7.15534944800001));
#98451=CARTESIAN_POINT('Ctrl Pts',(1.00653586,2.821428571,-7.179790078));
#98452=CARTESIAN_POINT('Ctrl Pts',(0.786978868000001,2.785541304,-7.210569806));
#98453=CARTESIAN_POINT('Ctrl Pts',(0.5659514,2.7492206,-7.227876522));
#98454=CARTESIAN_POINT('',(0.570694525309022,2.75000000042798,-7.22750357172063));
#98455=CARTESIAN_POINT('Ctrl Pts',(0.570694526447554,2.75000000139598,-7.22750357294847));
#98456=CARTESIAN_POINT('Ctrl Pts',(0.716819210598589,2.77401081875601,-7.21596534234186));
#98457=CARTESIAN_POINT('Ctrl Pts',(0.862228424556655,2.79784107595042,-7.20002055938569));
#98458=CARTESIAN_POINT('Ctrl Pts',(1.00653586005971,2.82142857101764,-7.17979007804883));
#98459=CARTESIAN_POINT('Ctrl Pts',(1.12244483064415,2.84037424974774,-7.16354078149041));
#98460=CARTESIAN_POINT('Ctrl Pts',(1.2382768204656,2.85947647457669,-7.14443865681336));
#98461=CARTESIAN_POINT('Ctrl Pts',(1.35382243337963,2.87870320492291,-7.12247604475633));
#98462=CARTESIAN_POINT('Ctrl Pts',(0.591039220362235,2.78894740131128,-7.47667523973043));
#98463=CARTESIAN_POINT('Ctrl Pts',(0.587541101836393,2.78276652346789,-7.43511514349877));
#98464=CARTESIAN_POINT('Ctrl Pts',(0.584091760165538,2.77643543057668,-7.39355002482526));
#98465=CARTESIAN_POINT('Ctrl Pts',(0.577308060245671,2.76346377183966,-7.31050773528907));
#98466=CARTESIAN_POINT('Ctrl Pts',(0.573969660415607,2.75681548743311,-7.26898115542804));
#98467=CARTESIAN_POINT('Ctrl Pts',(0.570694527575213,2.75000000136005,-7.22750357138854));
#98468=CARTESIAN_POINT('Ctrl Pts',(0.840054531,2.749235821,-7.45280540400001));
#98469=CARTESIAN_POINT('Ctrl Pts',(0.436216075,2.813580595,-7.498324682));
#98470=CARTESIAN_POINT('Ctrl Pts',(0.029823541,2.878703203,-7.499940704));
#98471=CARTESIAN_POINT('Ctrl Pts',(0.575345286,2.749235821,-7.227134827));
#98472=CARTESIAN_POINT('Ctrl Pts',(0.183735038,2.813580595,-7.25831054400001));
#98473=CARTESIAN_POINT('Ctrl Pts',(-0.208950992,2.878703203,-7.246988304));
#98474=CARTESIAN_POINT('Origin',(0.0169136900852243,2.94638889602872,0.195379449224228));
#98475=CARTESIAN_POINT('Ctrl Pts',(-0.453675371239687,2.88000589655946,
-7.48627054085738));
#98476=CARTESIAN_POINT('Ctrl Pts',(-0.457789381619843,2.87935454977973,
-7.48601668892869));
#98477=CARTESIAN_POINT('Ctrl Pts',(-0.461903392,2.878703203,-7.485762837));
#98478=CARTESIAN_POINT('Ctrl Pts',(-0.643672133,2.84992484,-7.474546933));
#98479=CARTESIAN_POINT('Ctrl Pts',(-0.824682289,2.821428571,-7.454522059));
#98480=CARTESIAN_POINT('Ctrl Pts',(-1.052640546,2.785541304,-7.429303388));
#98481=CARTESIAN_POINT('Ctrl Pts',(-1.278631936,2.7492206,-7.390202999));
#98482=CARTESIAN_POINT('Ctrl Pts',(-0.200985421661271,2.88000589655946,
-7.24721797370008));
#98483=CARTESIAN_POINT('Ctrl Pts',(-0.204968206830636,2.87935454977973,
-7.24710313885004));
#98484=CARTESIAN_POINT('Ctrl Pts',(-0.208950992,2.878703203,-7.246988304));
#98485=CARTESIAN_POINT('Ctrl Pts',(-0.384921828,2.84992484,-7.241914572));
#98486=CARTESIAN_POINT('Ctrl Pts',(-0.560439023,2.821428571,-7.228306033));
#98487=CARTESIAN_POINT('Ctrl Pts',(-0.781479626,2.785541304,-7.211167885));
#98488=CARTESIAN_POINT('Ctrl Pts',(-1.001060027,2.7492206,-7.180555607));
#98489=CARTESIAN_POINT('',(-0.996347619664787,2.7500000002595,-7.18121100776154));
#98490=CARTESIAN_POINT('Ctrl Pts',(-0.99634761870574,2.74999999999996,-7.18121100943214));
#98491=CARTESIAN_POINT('Ctrl Pts',(-0.779105665,2.785926731,-7.211351947));
#98492=CARTESIAN_POINT('Ctrl Pts',(-0.560439023,2.821428571,-7.228306033));
#98493=CARTESIAN_POINT('Ctrl Pts',(-0.384921828241024,2.84992483977763,
-7.24191457215127));
#98494=CARTESIAN_POINT('Ctrl Pts',(-0.208950993485686,2.87870320492457,
-7.24698831685028));
#98495=CARTESIAN_POINT('Ctrl Pts',(-1.03004311525275,2.788947401301,-7.42893068891883));
#98496=CARTESIAN_POINT('Ctrl Pts',(-1.02452525383604,2.78276651929034,-7.38759022460058));
#98497=CARTESIAN_POINT('Ctrl Pts',(-1.01895868193285,2.77643542852002,-7.34625538356977));
#98498=CARTESIAN_POINT('Ctrl Pts',(-1.00773214704204,2.76346377185447,-7.26369629468472));
#98499=CARTESIAN_POINT('Ctrl Pts',(-1.00206550982274,2.75681548744204,-7.22242292579477));
#98500=CARTESIAN_POINT('Ctrl Pts',(-0.996347617450642,2.75000000138088,
-7.18121100788328));
#98501=CARTESIAN_POINT('Ctrl Pts',(-0.781718335,2.749235821,-7.45914984700001));
#98502=CARTESIAN_POINT('Ctrl Pts',(-1.185900572,2.813580595,-7.41679158));
#98503=CARTESIAN_POINT('Ctrl Pts',(-1.583139272,2.878703203,-7.33100743700001));
#98504=CARTESIAN_POINT('Ctrl Pts',(-0.991726322,2.749235821,-7.18185066));
#98505=CARTESIAN_POINT('Ctrl Pts',(-1.380882798,2.813580595,-7.128112879));
#98506=CARTESIAN_POINT('Ctrl Pts',(-1.7619541,2.878703203,-7.032639458));
#98507=CARTESIAN_POINT('Origin',(0.0585190337265659,2.94638888514094,0.187175510455847));
#98508=CARTESIAN_POINT('Ctrl Pts',(-2.05239556607029,2.88000589655946,-7.21371890228333));
#98509=CARTESIAN_POINT('Ctrl Pts',(-2.05635882253515,2.87935454977973,-7.21258659464167));
#98510=CARTESIAN_POINT('Ctrl Pts',(-2.060322079,2.878703203,-7.211454287));
#98511=CARTESIAN_POINT('Ctrl Pts',(-2.235430081,2.84992484,-7.161425698));
#98512=CARTESIAN_POINT('Ctrl Pts',(-2.407903564,2.821428571,-7.102957161));
#98513=CARTESIAN_POINT('Ctrl Pts',(-2.625111015,2.785541304,-7.029323802));
#98514=CARTESIAN_POINT('Ctrl Pts',(-2.837413424,2.7492206,-6.94255609));
#98515=CARTESIAN_POINT('Ctrl Pts',(-1.7542241324767,2.88000589655946,-7.03457612031035));
#98516=CARTESIAN_POINT('Ctrl Pts',(-1.75808911623835,2.87935454977973,-7.03360778915517));
#98517=CARTESIAN_POINT('Ctrl Pts',(-1.7619541,2.878703203,-7.032639458));
#98518=CARTESIAN_POINT('Ctrl Pts',(-1.932720133,2.84992484,-6.989855819));
#98519=CARTESIAN_POINT('Ctrl Pts',(-2.1012084,2.821428571,-6.938834431));
#98520=CARTESIAN_POINT('Ctrl Pts',(-2.313397001,2.785541304,-6.874579768));
#98521=CARTESIAN_POINT('Ctrl Pts',(-2.521263,2.7492206,-6.797479892));
#98522=CARTESIAN_POINT('',(-2.51680165745917,2.75000000047524,-6.79913299826488));
#98523=CARTESIAN_POINT('Ctrl Pts',(-2.51680165660779,2.75000000185138,-6.7991329999353));
#98524=CARTESIAN_POINT('Ctrl Pts',(-2.31111811,2.785926731,-6.875269858));
#98525=CARTESIAN_POINT('Ctrl Pts',(-2.1012084,2.821428571,-6.938834431));
#98526=CARTESIAN_POINT('Ctrl Pts',(-1.93272013410292,2.84992483971974,-6.98985581810938));
#98527=CARTESIAN_POINT('Ctrl Pts',(-1.76195410407895,2.87870320490793,-7.03263947015886));
#98528=CARTESIAN_POINT('Ctrl Pts',(-2.60296178012173,2.78894740128928,-7.03381759585592));
#98529=CARTESIAN_POINT('Ctrl Pts',(-2.58868622042987,2.78276663834398,-6.99463058061894));
#98530=CARTESIAN_POINT('Ctrl Pts',(-2.57436387749908,2.77643548705439,-6.95545837171158));
#98531=CARTESIAN_POINT('Ctrl Pts',(-2.54565191949826,2.76346377181111,-6.8772424882146));
#98532=CARTESIAN_POINT('Ctrl Pts',(-2.53124521094672,2.75681548741717,-6.83815222720877));
#98533=CARTESIAN_POINT('Ctrl Pts',(-2.51680165578597,2.75000000137606,-6.79913299872689));
#98534=CARTESIAN_POINT('Ctrl Pts',(-2.366938921,2.749235821,-7.116712734));
#98535=CARTESIAN_POINT('Ctrl Pts',(-2.752565827,2.813580595,-6.98845754600001));
#98536=CARTESIAN_POINT('Ctrl Pts',(-3.122076251,2.878703203,-6.819284411));
#98537=CARTESIAN_POINT('Ctrl Pts',(-2.51242591,2.749235821,-6.800751138));
#98538=CARTESIAN_POINT('Ctrl Pts',(-2.880932089,2.813580595,-6.664612578));
#98539=CARTESIAN_POINT('Ctrl Pts',(-3.232570193,2.878703203,-6.489452207));
#98540=CARTESIAN_POINT('Origin',(0.0973881573878738,2.94638888876476,0.17021974700001));
#98541=CARTESIAN_POINT('Ctrl Pts',(-3.55514802690122,2.88000589655946,-6.60386178482548));
#98542=CARTESIAN_POINT('Ctrl Pts',(-3.55877521195061,2.87935454977973,-6.60190396691274));
#98543=CARTESIAN_POINT('Ctrl Pts',(-3.562402397,2.878703203,-6.599946149));
#98544=CARTESIAN_POINT('Ctrl Pts',(-3.722661803,2.84992484,-6.513444156));
#98545=CARTESIAN_POINT('Ctrl Pts',(-3.878533944,2.821428571,-6.419265881));
#98546=CARTESIAN_POINT('Ctrl Pts',(-4.07483421,2.785541304,-6.300660847));
#98547=CARTESIAN_POINT('Ctrl Pts',(-4.263520614,2.7492206,-6.17028297400001));
#98548=CARTESIAN_POINT('Ctrl Pts',(-3.22543727298635,2.88000589655946,-6.49300530576195));
#98549=CARTESIAN_POINT('Ctrl Pts',(-3.22900373299317,2.87935454977973,-6.49122875638097));
#98550=CARTESIAN_POINT('Ctrl Pts',(-3.232570193,2.878703203,-6.48945220700001));
#98551=CARTESIAN_POINT('Ctrl Pts',(-3.390146593,2.84992484,-6.410959176));
#98552=CARTESIAN_POINT('Ctrl Pts',(-3.543727607,2.821428571,-6.324910643));
#98553=CARTESIAN_POINT('Ctrl Pts',(-3.737142503,2.785541304,-6.216543941));
#98554=CARTESIAN_POINT('Ctrl Pts',(-3.923574516,2.7492206,-6.096561573));
#98555=CARTESIAN_POINT('',(-3.91957284629739,2.75000000039545,-6.09913508692617));
#98556=CARTESIAN_POINT('Ctrl Pts',(-3.91957284582379,2.75000000142008,-6.09913508857399));
#98557=CARTESIAN_POINT('Ctrl Pts',(-3.79626135934077,2.77401081874129,-6.17838047435427));
#98558=CARTESIAN_POINT('Ctrl Pts',(-3.67085272138319,2.79784107591957,-6.25368485012352));
#98559=CARTESIAN_POINT('Ctrl Pts',(-3.54372760682947,2.82142857107553,-6.32491064329474));
#98560=CARTESIAN_POINT('Ctrl Pts',(-3.44161962337708,2.84037424986775,-6.38211981217387));
#98561=CARTESIAN_POINT('Ctrl Pts',(-3.33784646698797,2.85947647448721,-6.43701127592068));
#98562=CARTESIAN_POINT('Ctrl Pts',(-3.23257019957148,2.87870320490967,-6.48945221791298));
#98563=CARTESIAN_POINT('Ctrl Pts',(-4.05416884499283,2.78894740127868,-6.30981100949365));
#98564=CARTESIAN_POINT('Ctrl Pts',(-4.03180299006025,2.78276663833503,-6.27460898818553));
#98565=CARTESIAN_POINT('Ctrl Pts',(-4.00939462848932,2.77643548702787,-6.23943148401241));
#98566=CARTESIAN_POINT('Ctrl Pts',(-3.96453983709971,2.76346377177556,-6.16921646676086));
#98567=CARTESIAN_POINT('Ctrl Pts',(-3.94206669854191,2.75681548733472,-6.13413713072467));
#98568=CARTESIAN_POINT('Ctrl Pts',(-3.91957284478361,2.75000000127954,-6.09913508772685));
#98569=CARTESIAN_POINT('Ctrl Pts',(-3.841484074,2.749235821,-6.441506043));
#98570=CARTESIAN_POINT('Ctrl Pts',(-4.190524162,2.813580595,-6.233351005));
#98571=CARTESIAN_POINT('Ctrl Pts',(-4.515028415,2.878703203,-5.988699225));
#98572=CARTESIAN_POINT('Ctrl Pts',(-3.915647254,2.749235821,-6.10165605200001));
#98573=CARTESIAN_POINT('Ctrl Pts',(-4.246272197,2.813580595,-5.8894824));
#98574=CARTESIAN_POINT('Ctrl Pts',(-4.552034896,2.878703203,-5.642825383));
#98575=CARTESIAN_POINT('Origin',(0.131703323042633,2.94638880656141,0.145304330238902));
#98576=CARTESIAN_POINT('Ctrl Pts',(-4.89166571598322,2.88000589655946,-5.68521542954546));
#98577=CARTESIAN_POINT('Ctrl Pts',(-4.8947872264916,2.87935454977973,-5.68252364677273));
#98578=CARTESIAN_POINT('Ctrl Pts',(-4.897908737,2.878703203,-5.679831864));
#98579=CARTESIAN_POINT('Ctrl Pts',(-5.035825996,2.84992484,-5.560901205));
#98580=CARTESIAN_POINT('Ctrl Pts',(-5.167808388,2.821428571,-5.435416862));
#98581=CARTESIAN_POINT('Ctrl Pts',(-5.334022687,2.785541304,-5.277385994));
#98582=CARTESIAN_POINT('Ctrl Pts',(-5.490270318,2.7492206,-5.109494284));
#98583=CARTESIAN_POINT('Ctrl Pts',(-4.5458325508932,2.88000589655946,-5.64782877921422));
#98584=CARTESIAN_POINT('Ctrl Pts',(-4.54893372344661,2.87935454977973,-5.64532708110711));
#98585=CARTESIAN_POINT('Ctrl Pts',(-4.55203489600001,2.878703203,-5.642825383));
#98586=CARTESIAN_POINT('Ctrl Pts',(-4.689053566,2.84992484,-5.532293208));
#98587=CARTESIAN_POINT('Ctrl Pts',(-4.82054605,2.821428571,-5.415241063));
#98588=CARTESIAN_POINT('Ctrl Pts',(-4.986143376,2.785541304,-5.267829429));
#98589=CARTESIAN_POINT('Ctrl Pts',(-5.14242405,2.7492206,-5.11057481));
#98590=CARTESIAN_POINT('',(-5.13906916740632,2.75000000026844,-5.11394839761507));
#98591=CARTESIAN_POINT('Ctrl Pts',(-5.13906916779104,2.74999999999911,-5.11394839941762));
#98592=CARTESIAN_POINT('Ctrl Pts',(-4.984364872,2.785926731,-5.26941262000001));
#98593=CARTESIAN_POINT('Ctrl Pts',(-4.82054605,2.821428571,-5.415241063));
#98594=CARTESIAN_POINT('Ctrl Pts',(-4.68905356671078,2.84992483968629,-5.53229320762546));
#98595=CARTESIAN_POINT('Ctrl Pts',(-4.55203490458502,2.87870320490793,-5.64282539268874));
#98596=CARTESIAN_POINT('Ctrl Pts',(-5.31580748100935,2.78894740125035,-5.29076467304406));
#98597=CARTESIAN_POINT('Ctrl Pts',(-5.28639655245168,2.7827665162488,-5.26119306918344));
#98598=CARTESIAN_POINT('Ctrl Pts',(-5.25695027077263,2.77643542702018,-5.23165544233194));
#98599=CARTESIAN_POINT('Ctrl Pts',(-5.19805027904343,2.76346377184499,-5.17272474019516));
#98600=CARTESIAN_POINT('Ctrl Pts',(-5.1685615301564,2.75681548751552,-5.14329660039426));
#98601=CARTESIAN_POINT('Ctrl Pts',(-5.13906916559948,2.75000000145262,-5.11394839915577));
#98602=CARTESIAN_POINT('Ctrl Pts',(-5.136405701,2.749235821,-5.465101689));
#98603=CARTESIAN_POINT('Ctrl Pts',(-5.432538246,2.813580595,-5.186779898));
#98604=CARTESIAN_POINT('Ctrl Pts',(-5.696862869,2.878703203,-4.878089119));
#98605=CARTESIAN_POINT('Ctrl Pts',(-5.135777285,2.749235821,-5.11725431000001));
#98606=CARTESIAN_POINT('Ctrl Pts',(-5.413061337,2.813580595,-4.838966571));
#98607=CARTESIAN_POINT('Ctrl Pts',(-5.658651506,2.878703203,-4.532346316));
#98608=CARTESIAN_POINT('Origin',(0.159860395255516,2.94638884086943,0.113594925728563));
#98609=CARTESIAN_POINT('Ctrl Pts',(-5.9994545538008,2.88000589655946,-4.50073471974354));
#98610=CARTESIAN_POINT('Ctrl Pts',(-6.0019244314004,2.87935454977973,-4.49743483687177));
#98611=CARTESIAN_POINT('Ctrl Pts',(-6.004394309,2.878703203,-4.494134954));
#98612=CARTESIAN_POINT('Ctrl Pts',(-6.113520563,2.84992484,-4.348336694));
#98613=CARTESIAN_POINT('Ctrl Pts',(-6.215441855,2.821428571,-4.197413792));
#98614=CARTESIAN_POINT('Ctrl Pts',(-6.343798191,2.785541304,-4.007346437));
#98615=CARTESIAN_POINT('Ctrl Pts',(-6.460301084,2.7492206,-3.80979132));
#98616=CARTESIAN_POINT('Ctrl Pts',(-5.65366975057634,2.88000589655946,-4.53856605649532));
#98617=CARTESIAN_POINT('Ctrl Pts',(-5.65616062828817,2.87935454977973,-4.53545618624766));
#98618=CARTESIAN_POINT('Ctrl Pts',(-5.658651506,2.878703203,-4.532346316));
#98619=CARTESIAN_POINT('Ctrl Pts',(-5.768705605,2.84992484,-4.394943357));
#98620=CARTESIAN_POINT('Ctrl Pts',(-5.871961118,2.821428571,-4.25236083));
#98621=CARTESIAN_POINT('Ctrl Pts',(-6.001997726,2.785541304,-4.072797068));
#98622=CARTESIAN_POINT('Ctrl Pts',(-6.12081955,2.7492206,-3.88562325));
#98623=CARTESIAN_POINT('',(-6.11826832419047,2.75000000024419,-3.88963916514864));
#98624=CARTESIAN_POINT('Ctrl Pts',(-6.11826832477835,2.74999999999996,-3.88963916703005));
#98625=CARTESIAN_POINT('Ctrl Pts',(-6.000601142,2.785926731,-4.074725571));
#98626=CARTESIAN_POINT('Ctrl Pts',(-5.871961118,2.821428571,-4.25236083));
#98627=CARTESIAN_POINT('Ctrl Pts',(-5.76870560553419,2.84992483976829,-4.39494335711938));
#98628=CARTESIAN_POINT('Ctrl Pts',(-5.65865151622557,2.8787032050476,-4.53234632367778));
#98629=CARTESIAN_POINT('Ctrl Pts',(-6.32888486674515,2.78894740126507,-4.02432806087191));
#98630=CARTESIAN_POINT('Ctrl Pts',(-6.29380522164559,2.78276663834483,-4.00177075055515));
#98631=CARTESIAN_POINT('Ctrl Pts',(-6.25869729295988,2.77643548704644,-3.97925353934966));
#98632=CARTESIAN_POINT('Ctrl Pts',(-6.18850566656785,2.76346377182085,-3.93436215385666));
#98633=CARTESIAN_POINT('Ctrl Pts',(-6.15338016783904,2.75681548743132,-3.91196123690154));
#98634=CARTESIAN_POINT('Ctrl Pts',(-6.11826832270252,2.75000000136865,-3.88963916714581));
#98635=CARTESIAN_POINT('Ctrl Pts',(-6.19115470600001,2.749235821,-4.233155254));
#98636=CARTESIAN_POINT('Ctrl Pts',(-6.420532878,2.813580595,-3.897680728));
#98637=CARTESIAN_POINT('Ctrl Pts',(-6.612318346,2.878703203,-3.539384988));
#98638=CARTESIAN_POINT('Ctrl Pts',(-6.115764078,2.749235821,-3.893575445));
#98639=CARTESIAN_POINT('Ctrl Pts',(-6.326741745,2.813580595,-3.562186043));
#98640=CARTESIAN_POINT('Ctrl Pts',(-6.500675861,2.878703203,-3.209939773));
#98641=CARTESIAN_POINT('Origin',(0.180542670106106,2.94638889073077,0.0765739682539879));
#98642=CARTESIAN_POINT('Ctrl Pts',(-6.82671556406542,2.88000589655946,-3.10580465625746));
#98643=CARTESIAN_POINT('Ctrl Pts',(-6.82841832003271,2.87935454977973,-3.10205097212873));
#98644=CARTESIAN_POINT('Ctrl Pts',(-6.830121076,2.878703203,-3.098297288));
#98645=CARTESIAN_POINT('Ctrl Pts',(-6.905353703,2.84992484,-2.932448791));
#98646=CARTESIAN_POINT('Ctrl Pts',(-6.972448169,2.821428571,-2.763144319));
#98647=CARTESIAN_POINT('Ctrl Pts',(-7.056944742,2.785541304,-2.549927814));
#98648=CARTESIAN_POINT('Ctrl Pts',(-7.128255352,2.7492206,-2.331946748));
#98649=CARTESIAN_POINT('Ctrl Pts',(-6.49714763659028,2.88000589655946,-3.21708502956251));
#98650=CARTESIAN_POINT('Ctrl Pts',(-6.49891174879514,2.87935454977973,-3.21351240128125));
#98651=CARTESIAN_POINT('Ctrl Pts',(-6.500675861,2.878703203,-3.209939773));
#98652=CARTESIAN_POINT('Ctrl Pts',(-6.578619382,2.84992484,-3.052090841));
#98653=CARTESIAN_POINT('Ctrl Pts',(-6.64880981,2.821428571,-2.890644931));
#98654=CARTESIAN_POINT('Ctrl Pts',(-6.737205333,2.785541304,-2.687325243));
#98655=CARTESIAN_POINT('Ctrl Pts',(-6.813012331,2.7492206,-2.478984264));
#98656=CARTESIAN_POINT('',(-6.81138405458469,2.75000000026527,-2.48345472752655));
#98657=CARTESIAN_POINT('Ctrl Pts',(-6.81138405566465,2.74999999999996,-2.4834547290353));
#98658=CARTESIAN_POINT('Ctrl Pts',(-6.736255972,2.785926731,-2.689508882));
#98659=CARTESIAN_POINT('Ctrl Pts',(-6.64880981,2.821428571,-2.890644931));
#98660=CARTESIAN_POINT('Ctrl Pts',(-6.57861938257659,2.84992483974429,-3.05209084090307));
#98661=CARTESIAN_POINT('Ctrl Pts',(-6.50067587308103,2.87870320492457,-3.2099397776958));
#98662=CARTESIAN_POINT('Ctrl Pts',(-7.04603063056367,2.78894740127283,-2.56971834113614));
#98663=CARTESIAN_POINT('Ctrl Pts',(-7.00692124906874,2.78276652391527,-2.55522922667437));
#98664=CARTESIAN_POINT('Ctrl Pts',(-6.96779397438999,2.77643543079175,-2.54078576580088));
#98665=CARTESIAN_POINT('Ctrl Pts',(-6.88959340745289,2.76346377181563,-2.51203316538067));
#98666=CARTESIAN_POINT('Ctrl Pts',(-6.850473588529,2.75681548744948,-2.49770691330304));
#98667=CARTESIAN_POINT('Ctrl Pts',(-6.81138405359718,2.75000000138084,-2.48345472970154));
#98668=CARTESIAN_POINT('Ctrl Pts',(-6.956412198,2.749235821,-2.803271184));
#98669=CARTESIAN_POINT('Ctrl Pts',(-7.10831053000001,2.813580595,-2.42633034));
#98670=CARTESIAN_POINT('Ctrl Pts',(-7.218589166,2.878703203,-2.035183148));
#98671=CARTESIAN_POINT('Ctrl Pts',(-6.80978454,2.749235821,-2.487837318));
#98672=CARTESIAN_POINT('Ctrl Pts',(-6.944590741,2.813580595,-2.118841655));
#98673=CARTESIAN_POINT('Ctrl Pts',(-7.038735838,2.878703203,-1.737440013));
#98674=CARTESIAN_POINT('Origin',(0.192782843529136,2.94638888841761,0.035972377766566));
#98675=CARTESIAN_POINT('Ctrl Pts',(-7.33476694232736,2.88000589655946,-1.56565061954801));
#98676=CARTESIAN_POINT('Ctrl Pts',(-7.33562295766368,2.87935454977973,-1.561618652274));
#98677=CARTESIAN_POINT('Ctrl Pts',(-7.336478973,2.878703203,-1.557586685));
#98678=CARTESIAN_POINT('Ctrl Pts',(-7.374300178,2.84992484,-1.379442843));
#98679=CARTESIAN_POINT('Ctrl Pts',(-7.403430556,2.821428571,-1.199673288));
#98680=CARTESIAN_POINT('Ctrl Pts',(-7.4401164,2.785541304,-0.973277401));
#98681=CARTESIAN_POINT('Ctrl Pts',(-7.462900322,2.7492206,-0.745062938000001));
#98682=CARTESIAN_POINT('Ctrl Pts',(-7.03682612043755,2.88000589655946,-1.74517668140246));
#98683=CARTESIAN_POINT('Ctrl Pts',(-7.03778097921877,2.87935454977973,-1.74130834720123));
#98684=CARTESIAN_POINT('Ctrl Pts',(-7.038735838,2.878703203,-1.737440013));
#98685=CARTESIAN_POINT('Ctrl Pts',(-7.080924229,2.84992484,-1.566525948));
#98686=CARTESIAN_POINT('Ctrl Pts',(-7.114767544,2.821428571,-1.393765687));
#98687=CARTESIAN_POINT('Ctrl Pts',(-7.157388707,2.785541304,-1.176197076));
#98688=CARTESIAN_POINT('Ctrl Pts',(-7.186636227,2.7492206,-0.95643073));
#98689=CARTESIAN_POINT('',(-7.18600703588704,2.75000000047524,-0.961146708048971));
#98690=CARTESIAN_POINT('Ctrl Pts',(-7.18600703699163,2.75000000185138,-0.961146709604796));
#98691=CARTESIAN_POINT('Ctrl Pts',(-7.156930959,2.785926731,-1.178533747));
#98692=CARTESIAN_POINT('Ctrl Pts',(-7.114767544,2.821428571,-1.393765687));
#98693=CARTESIAN_POINT('Ctrl Pts',(-7.0809242289375,2.84992483971582,-1.56652594736781));
#98694=CARTESIAN_POINT('Ctrl Pts',(-7.03873585046811,2.87870320490792,-1.73744001534874));
#98695=CARTESIAN_POINT('Ctrl Pts',(-7.43371183284565,2.78894740126349,-0.994951447861542));
#98696=CARTESIAN_POINT('Ctrl Pts',(-7.39240207702832,2.78276652412189,-0.989208442067899));
#98697=CARTESIAN_POINT('Ctrl Pts',(-7.35108465833632,2.77643543088597,-0.983513868720913));
#98698=CARTESIAN_POINT('Ctrl Pts',(-7.26853141724985,2.76346377178727,-0.972244298473256));
#98699=CARTESIAN_POINT('Ctrl Pts',(-7.22724647698605,2.75681548737656,-0.966662590939243));
#98700=CARTESIAN_POINT('Ctrl Pts',(-7.18600703548563,2.75000000130361,-0.961146710026586));
#98701=CARTESIAN_POINT('Ctrl Pts',(-7.396395587,2.749235821,-1.242309269));
#98702=CARTESIAN_POINT('Ctrl Pts',(-7.463711481,2.813580595,-0.841527441));
#98703=CARTESIAN_POINT('Ctrl Pts',(-7.48732678,2.878703203,-0.435818406));
#98704=CARTESIAN_POINT('Ctrl Pts',(-7.185387045,2.749235821,-0.965770684));
#98705=CARTESIAN_POINT('Ctrl Pts',(-7.237718391,2.813580595,-0.576422586));
#98706=CARTESIAN_POINT('Ctrl Pts',(-7.24767235000001,2.878703203,-0.18369949));
#98707=CARTESIAN_POINT('Origin',(0.196008725215265,2.94638886097645,-0.00631123273774178));
#98708=CARTESIAN_POINT('Ctrl Pts',(-7.49985277021764,2.88000589655946,0.0477115007758101));
#98709=CARTESIAN_POINT('Ctrl Pts',(-7.49982201860882,2.87935454977973,0.0518332208879051));
#98710=CARTESIAN_POINT('Ctrl Pts',(-7.499791267,2.878703203,0.055954941));
#98711=CARTESIAN_POINT('Ctrl Pts',(-7.498432573,2.84992484,0.23806432));
#98712=CARTESIAN_POINT('Ctrl Pts',(-7.488236759,2.821428571,0.419893133));
#98713=CARTESIAN_POINT('Ctrl Pts',(-7.475396485,2.785541304,0.648882381));
#98714=CARTESIAN_POINT('Ctrl Pts',(-7.448588368,2.7492206,0.876659187));
#98715=CARTESIAN_POINT('Ctrl Pts',(-7.24747043558839,2.88000589655946,-0.191665812214019));
#98716=CARTESIAN_POINT('Ctrl Pts',(-7.2475713927942,2.87935454977973,-0.187682651107009));
#98717=CARTESIAN_POINT('Ctrl Pts',(-7.24767235,2.878703203,-0.18369949));
#98718=CARTESIAN_POINT('Ctrl Pts',(-7.252132928,2.84992484,-0.007712044));
#98719=CARTESIAN_POINT('Ctrl Pts',(-7.248046656,2.821428571,0.168284491));
#98720=CARTESIAN_POINT('Ctrl Pts',(-7.24290054,2.785541304,0.38992876));
#98721=CARTESIAN_POINT('Ctrl Pts',(-7.224221001,2.7492206,0.610844443));
#98722=CARTESIAN_POINT('',(-7.22462031605779,2.75000000025979,0.606103464216765));
#98723=CARTESIAN_POINT('Ctrl Pts',(-7.22462031767412,2.74999999999996,0.606103463201151));
#98724=CARTESIAN_POINT('Ctrl Pts',(-7.242955809,2.785926731,0.387548315));
#98725=CARTESIAN_POINT('Ctrl Pts',(-7.248046656,2.821428571,0.168284491));
#98726=CARTESIAN_POINT('Ctrl Pts',(-7.25213292811546,2.84992483969163,-0.00771204260381877));
#98727=CARTESIAN_POINT('Ctrl Pts',(-7.24767236317298,2.87870320490793,-0.183699489006381));
#98728=CARTESIAN_POINT('Ctrl Pts',(-7.47380093235172,2.78894740127252,0.626338268970036));
#98729=CARTESIAN_POINT('Ctrl Pts',(-7.43222238196124,2.78276652157547,0.623066628776044));
#98730=CARTESIAN_POINT('Ctrl Pts',(-7.39064678568942,2.77643542964108,0.619746043259463));
#98731=CARTESIAN_POINT('Ctrl Pts',(-7.3076009770964,2.76346377183828,0.613005631471951));
#98732=CARTESIAN_POINT('Ctrl Pts',(-7.26608135367996,2.75681548745084,0.609581800093443));
#98733=CARTESIAN_POINT('Ctrl Pts',(-7.22462031606358,2.75000000139655,0.606103461920369));
#98734=CARTESIAN_POINT('Ctrl Pts',(-7.490531739,2.749235821,0.376741646));
#98735=CARTESIAN_POINT('Ctrl Pts',(-7.47011757900001,2.813580595,0.782624346));
#98736=CARTESIAN_POINT('Ctrl Pts',(-7.40596531600001,2.878703203,1.18392472));
#98737=CARTESIAN_POINT('Ctrl Pts',(-7.225008838,2.749235821,0.601454314));
#98738=CARTESIAN_POINT('Ctrl Pts',(-7.192418375,2.813580595,0.992949363));
#98739=CARTESIAN_POINT('Ctrl Pts',(-7.117715759,2.878703203,1.378630618));
#98740=CARTESIAN_POINT('Origin',(0.190069426067424,2.94638891401156,-0.0482997700442647));
#98741=CARTESIAN_POINT('Ctrl Pts',(-7.31425381724154,2.88000589655946,1.65884268319525));
#98742=CARTESIAN_POINT('Ctrl Pts',(-7.31333773662077,2.87935454977973,1.66286142909763));
#98743=CARTESIAN_POINT('Ctrl Pts',(-7.312421656,2.878703203,1.666880175));
#98744=CARTESIAN_POINT('Ctrl Pts',(-7.271946595,2.84992484,1.844439859));
#98745=CARTESIAN_POINT('Ctrl Pts',(-7.222901333,2.821428571,2.019825817));
#98746=CARTESIAN_POINT('Ctrl Pts',(-7.161135338,2.785541304,2.240701145));
#98747=CARTESIAN_POINT('Ctrl Pts',(-7.085988699,2.7492206,2.457389703));
#98748=CARTESIAN_POINT('Ctrl Pts',(-7.11923108909293,2.88000589655946,1.37080713833006));
#98749=CARTESIAN_POINT('Ctrl Pts',(-7.11847342404647,2.87935454977973,1.37471887816503));
#98750=CARTESIAN_POINT('Ctrl Pts',(-7.117715759,2.878703203,1.378630618));
#98751=CARTESIAN_POINT('Ctrl Pts',(-7.084239951,2.84992484,1.551462468));
#98752=CARTESIAN_POINT('Ctrl Pts',(-7.042415162,2.821428571,1.722465874));
#98753=CARTESIAN_POINT('Ctrl Pts',(-6.989742393,2.785541304,1.937821959));
#98754=CARTESIAN_POINT('Ctrl Pts',(-6.92400923,2.7492206,2.149557208));
#98755=CARTESIAN_POINT('',(-6.92541837970349,2.75000000043858,2.1450129119477));
#98756=CARTESIAN_POINT('Ctrl Pts',(-6.92541838123497,2.75000000140029,2.14501291150036));
#98757=CARTESIAN_POINT('Ctrl Pts',(-6.96878595450075,2.7740108187138,2.00499574194987));
#98758=CARTESIAN_POINT('Ctrl Pts',(-7.00779512042091,2.79784107590582,1.86401219475765));
#98759=CARTESIAN_POINT('Ctrl Pts',(-7.04241516218228,2.82142857108703,1.7224658735676));
#98760=CARTESIAN_POINT('Ctrl Pts',(-7.07022227669528,2.84037424985765,1.60877465310127));
#98761=CARTESIAN_POINT('Ctrl Pts',(-7.09535068652136,2.85947647453636,1.49409900678069));
#98762=CARTESIAN_POINT('Ctrl Pts',(-7.11771577132896,2.87870320488967,1.37863062164941));
#98763=CARTESIAN_POINT('Ctrl Pts',(-7.1644234061344,2.78894740128559,2.21834110489946));
#98764=CARTESIAN_POINT('Ctrl Pts',(-7.12452026293291,2.78276652435089,2.20620779999514));
#98765=CARTESIAN_POINT('Ctrl Pts',(-7.08463049941589,2.77643543102928,2.19402732086459));
#98766=CARTESIAN_POINT('Ctrl Pts',(-7.0049752368222,2.76346377186035,2.16959209955829));
#98767=CARTESIAN_POINT('Ctrl Pts',(-6.96516234191877,2.75681548748643,2.15732282375446));
#98768=CARTESIAN_POINT('Ctrl Pts',(-6.92541838025487,2.75000000140094,2.1450129096347));
#98769=CARTESIAN_POINT('Ctrl Pts',(-7.234418952,2.749235821,1.978176541));
#98770=CARTESIAN_POINT('Ctrl Pts',(-7.127229281,2.813580595,2.370181488));
#98771=CARTESIAN_POINT('Ctrl Pts',(-6.978309144,2.878703203,2.748308842));
#98772=CARTESIAN_POINT('Ctrl Pts',(-6.926797248,2.749235821,2.140555977));
#98773=CARTESIAN_POINT('Ctrl Pts',(-6.810808868,2.813580595,2.515892103));
#98774=CARTESIAN_POINT('Ctrl Pts',(-6.65494268900001,2.878703203,2.87649749));
#98775=CARTESIAN_POINT('Origin',(0.175242662804203,2.94638889345237,-0.0880298495019172));
#98776=CARTESIAN_POINT('Ctrl Pts',(-6.78664848652661,2.88000589655946,3.19240822682198));
#98777=CARTESIAN_POINT('Ctrl Pts',(-6.7848899117633,2.87935454977973,3.19613608641099));
#98778=CARTESIAN_POINT('Ctrl Pts',(-6.783131337,2.878703203,3.199863946));
#98779=CARTESIAN_POINT('Ctrl Pts',(-6.705432476,2.84992484,3.364571441));
#98780=CARTESIAN_POINT('Ctrl Pts',(-6.619831069,2.821428571,3.525313691));
#98781=CARTESIAN_POINT('Ctrl Pts',(-6.512027462,2.785541304,3.727747213));
#98782=CARTESIAN_POINT('Ctrl Pts',(-6.392056075,2.7492206,3.923215407));
#98783=CARTESIAN_POINT('Ctrl Pts',(-6.65810440838206,2.88000589655946,2.86918267012378));
#98784=CARTESIAN_POINT('Ctrl Pts',(-6.65652354869103,2.87935454977973,2.87284008006189));
#98785=CARTESIAN_POINT('Ctrl Pts',(-6.654942689,2.878703203,2.87649749));
#98786=CARTESIAN_POINT('Ctrl Pts',(-6.585095788,2.84992484,3.038092318));
#98787=CARTESIAN_POINT('Ctrl Pts',(-6.507488162,2.821428571,3.196106666));
#98788=CARTESIAN_POINT('Ctrl Pts',(-6.40975166,2.785541304,3.395104758));
#98789=CARTESIAN_POINT('Ctrl Pts',(-6.300038482,2.7492206,3.587759067));
#98790=CARTESIAN_POINT('',(-6.30239157604247,2.75000000044397,3.58362393917865));
#98791=CARTESIAN_POINT('Ctrl Pts',(-6.30239157771542,2.75000000149012,3.58362393887883));
#98792=CARTESIAN_POINT('Ctrl Pts',(-6.37484479418816,2.77401081887672,3.45620303955513));
#98793=CARTESIAN_POINT('Ctrl Pts',(-6.44324924287563,2.79784107603871,3.32690142699863));
#98794=CARTESIAN_POINT('Ctrl Pts',(-6.50748816226137,2.82142857106589,3.19610666587472));
#98795=CARTESIAN_POINT('Ctrl Pts',(-6.55908541327254,2.84037424976114,3.09105119099027));
#98796=CARTESIAN_POINT('Ctrl Pts',(-6.60827820948216,2.85947647458613,2.9844584625883));
#98797=CARTESIAN_POINT('Ctrl Pts',(-6.65494270044249,2.87870320494007,2.87649749609288));
#98798=CARTESIAN_POINT('Ctrl Pts',(-6.52004540446191,2.78894740123703,3.70661677599489));
#98799=CARTESIAN_POINT('Ctrl Pts',(-6.4836834607068,2.78276652164253,3.68618913596105));
#98800=CARTESIAN_POINT('Ctrl Pts',(-6.44734474878675,2.7764354296662,3.66571831425722));
#98801=CARTESIAN_POINT('Ctrl Pts',(-6.37480463932654,2.76346377182802,3.62473085209843));
#98802=CARTESIAN_POINT('Ctrl Pts',(-6.33856007921744,2.75681548745698,3.60418982954241));
#98803=CARTESIAN_POINT('Ctrl Pts',(-6.30239157687467,2.75000000139314,3.58362393740054));
#98804=CARTESIAN_POINT('Ctrl Pts',(-6.640032775,2.749235821,3.4871141));
#98805=CARTESIAN_POINT('Ctrl Pts',(-6.451079663,2.813580595,3.846911578));
#98806=CARTESIAN_POINT('Ctrl Pts',(-6.224354992,2.878703203,4.184185097));
#98807=CARTESIAN_POINT('Ctrl Pts',(-6.304696317,2.749235821,3.579567621));
#98808=CARTESIAN_POINT('Ctrl Pts',(-6.110733509,2.813580595,3.921194524));
#98809=CARTESIAN_POINT('Ctrl Pts',(-5.880991895,2.878703203,4.239862537));
#98810=CARTESIAN_POINT('Origin',(0.152221680070309,2.94638885833933,-0.12364368640523));
#98811=CARTESIAN_POINT('Ctrl Pts',(-5.94170701373572,2.88000589655946,4.57670030852734));
#98812=CARTESIAN_POINT('Ctrl Pts',(-5.93918817386786,2.87935454977973,4.57996297126367));
#98813=CARTESIAN_POINT('Ctrl Pts',(-5.936669334,2.878703203,4.583225634));
#98814=CARTESIAN_POINT('Ctrl Pts',(-5.825379787,2.84992484,4.727379402));
#98815=CARTESIAN_POINT('Ctrl Pts',(-5.707224861,2.821428571,4.865961815));
#98816=CARTESIAN_POINT('Ctrl Pts',(-5.558424419,2.785541304,5.040487965));
#98817=CARTESIAN_POINT('Ctrl Pts',(-5.399238013,2.7492206,5.20559592));
#98818=CARTESIAN_POINT('Ctrl Pts',(-5.88565216516249,2.88000589655946,4.23339840973982));
#98819=CARTESIAN_POINT('Ctrl Pts',(-5.88332203008124,2.87935454977973,4.23663047336991));
#98820=CARTESIAN_POINT('Ctrl Pts',(-5.880991895,2.878703203,4.239862537));
#98821=CARTESIAN_POINT('Ctrl Pts',(-5.778039865,2.84992484,4.382664349));
#98822=CARTESIAN_POINT('Ctrl Pts',(-5.668278248,2.821428571,4.520301063));
#98823=CARTESIAN_POINT('Ctrl Pts',(-5.530048064,2.785541304,4.693636231));
#98824=CARTESIAN_POINT('Ctrl Pts',(-5.38148493800001,2.7492206,4.858201299));
#98825=CARTESIAN_POINT('',(-5.38467194767664,2.75000000042058,4.85466869391466));
#98826=CARTESIAN_POINT('Ctrl Pts',(-5.38467194961098,2.75000000141392,4.85466869376423));
#98827=CARTESIAN_POINT('Ctrl Pts',(-5.48282297663001,2.77401081878987,4.74580212481635));
#98828=CARTESIAN_POINT('Ctrl Pts',(-5.57742419173345,2.79784107597051,4.63422844676064));
#98829=CARTESIAN_POINT('Ctrl Pts',(-5.66827824813469,2.8214285710255,4.52030106320043));
#98830=CARTESIAN_POINT('Ctrl Pts',(-5.74125300605112,2.84037424975707,4.42879361097015));
#98831=CARTESIAN_POINT('Ctrl Pts',(-5.81220998726546,2.85947647451415,4.33526795795914));
#98832=CARTESIAN_POINT('Ctrl Pts',(-5.88099190465141,2.87870320491434,4.23986254478712));
#98833=CARTESIAN_POINT('Ctrl Pts',(-5.57079732597209,2.78894740125962,5.0215751666047));
#98834=CARTESIAN_POINT('Ctrl Pts',(-5.53967685848314,2.78276652471571,4.99380838402595));
#98835=CARTESIAN_POINT('Ctrl Pts',(-5.50858833888163,2.77643543117326,4.96600440247965));
#98836=CARTESIAN_POINT('Ctrl Pts',(-5.44655526262357,2.7634637717922,4.91038121850665));
#98837=CARTESIAN_POINT('Ctrl Pts',(-5.41557379272587,2.75681548734966,4.88252892431589));
#98838=CARTESIAN_POINT('Ctrl Pts',(-5.38467194888147,2.75000000126181,4.8546686923725));
#98839=CARTESIAN_POINT('Ctrl Pts',(-5.73516604600001,2.749235821,4.832998079));
#98840=CARTESIAN_POINT('Ctrl Pts',(-5.47328473,2.813580595,5.143764358));
#98841=CARTESIAN_POINT('Ctrl Pts',(-5.179356919,2.878703203,5.424413508));
#98842=CARTESIAN_POINT('Ctrl Pts',(-5.387794793,2.749235821,4.851202662));
#98843=CARTESIAN_POINT('Ctrl Pts',(-5.124927042,2.813580595,5.143146247));
#98844=CARTESIAN_POINT('Ctrl Pts',(-4.832052457,2.878703203,5.404976323));
#98845=CARTESIAN_POINT('Origin',(0.122083007002124,2.9463888135562,-0.153476030171616));
#98846=CARTESIAN_POINT('Ctrl Pts',(-4.81893792566327,2.88000589655946,5.74699097129102));
#98847=CARTESIAN_POINT('Ctrl Pts',(-4.81577659883164,2.87935454977973,5.74963587864552));
#98848=CARTESIAN_POINT('Ctrl Pts',(-4.812615272,2.878703203,5.752280786));
#98849=CARTESIAN_POINT('Ctrl Pts',(-4.672938814,2.84992484,5.86914035499999));
#98850=CARTESIAN_POINT('Ctrl Pts',(-4.527755162,2.821428571,5.979082973));
#98851=CARTESIAN_POINT('Ctrl Pts',(-4.344915628,2.785541304,6.117541102));
#98852=CARTESIAN_POINT('Ctrl Pts',(-4.153957582,2.7492206,6.244568552));
#98853=CARTESIAN_POINT('Ctrl Pts',(-4.83799336891228,2.88000589655946,5.39966514376146));
#98854=CARTESIAN_POINT('Ctrl Pts',(-4.83502291295614,2.87935454977973,5.40232073338072));
#98855=CARTESIAN_POINT('Ctrl Pts',(-4.832052457,2.878703203,5.404976323));
#98856=CARTESIAN_POINT('Ctrl Pts',(-4.70080922,2.84992484,5.522307865));
#98857=CARTESIAN_POINT('Ctrl Pts',(-4.564025943,2.821428571,5.633131207));
#98858=CARTESIAN_POINT('Ctrl Pts',(-4.391765567,2.785541304,5.772698491));
#98859=CARTESIAN_POINT('Ctrl Pts',(-4.211299138,2.7492206,5.901479439));
#98860=CARTESIAN_POINT('',(-4.21517104353124,2.75000000044712,5.89871453642188));
#98861=CARTESIAN_POINT('Ctrl Pts',(-4.21517104541032,2.75000000162255,5.89871453663159));
#98862=CARTESIAN_POINT('Ctrl Pts',(-4.393615631,2.785926731,5.771199548));
#98863=CARTESIAN_POINT('Ctrl Pts',(-4.564025943,2.821428571,5.633131207));
#98864=CARTESIAN_POINT('Ctrl Pts',(-4.70080921954997,2.8499248397042,5.52230786541046));
#98865=CARTESIAN_POINT('Ctrl Pts',(-4.83205246474551,2.87870320492458,5.4049763335841));
#98866=CARTESIAN_POINT('Ctrl Pts',(-4.36106495617808,2.78894740128769,6.10173028302463));
#98867=CARTESIAN_POINT('Ctrl Pts',(-4.33664107985251,2.78276651828651,6.06792265660883));
#98868=CARTESIAN_POINT('Ctrl Pts',(-4.31225644017267,2.77643542799327,6.03408562264512));
#98869=CARTESIAN_POINT('Ctrl Pts',(-4.26363101483272,2.76346377178398,5.96642761673698));
#98870=CARTESIAN_POINT('Ctrl Pts',(-4.23936129430749,2.75681548734638,5.93256639350245));
#98871=CARTESIAN_POINT('Ctrl Pts',(-4.21517104463714,2.75000000130795,5.8987145354583));
#98872=CARTESIAN_POINT('Ctrl Pts',(-4.562129326,2.749235821,5.952896439));
#98873=CARTESIAN_POINT('Ctrl Pts',(-4.239565086,2.813580595,6.200100433));
#98874=CARTESIAN_POINT('Ctrl Pts',(-3.892177873,2.878703203,6.411002371));
#98875=CARTESIAN_POINT('Ctrl Pts',(-4.218965973,2.749235821,5.896000858));
#98876=CARTESIAN_POINT('Ctrl Pts',(-3.899484683,2.813580595,6.124610169));
#98877=CARTESIAN_POINT('Ctrl Pts',(-3.557171616,2.878703203,6.317359424));
#98878=CARTESIAN_POINT('Origin',(0.0862359136157109,2.94638886271948,-0.176132018933817));
#98879=CARTESIAN_POINT('Ctrl Pts',(-3.47084065632979,2.88000589655946,6.6485587228404));
#98880=CARTESIAN_POINT('Ctrl Pts',(-3.4671846626649,2.87935454977973,6.6504622019202));
#98881=CARTESIAN_POINT('Ctrl Pts',(-3.463528669,2.878703203,6.652365681));
#98882=CARTESIAN_POINT('Ctrl Pts',(-3.301996416,2.84992484,6.736466829));
#98883=CARTESIAN_POINT('Ctrl Pts',(-3.136572664,2.821428571,6.812628856));
#98884=CARTESIAN_POINT('Ctrl Pts',(-2.928243412,2.785541304,6.908544816));
#98885=CARTESIAN_POINT('Ctrl Pts',(-2.714442712,2.7492206,6.9915521));
#98886=CARTESIAN_POINT('Ctrl Pts',(-3.56411537921917,2.88000589655946,6.313449537644));
#98887=CARTESIAN_POINT('Ctrl Pts',(-3.56064349760959,2.87935454977973,6.315404480822));
#98888=CARTESIAN_POINT('Ctrl Pts',(-3.557171616,2.878703203,6.317359424));
#98889=CARTESIAN_POINT('Ctrl Pts',(-3.40377396,2.84992484,6.403734403));
#98890=CARTESIAN_POINT('Ctrl Pts',(-3.246364857,2.821428571,6.482562396));
#98891=CARTESIAN_POINT('Ctrl Pts',(-3.048128992,2.785541304,6.581835786));
#98892=CARTESIAN_POINT('Ctrl Pts',(-2.844197672,2.7492206,6.668810959));
#98893=CARTESIAN_POINT('',(-2.84857342605668,2.75000000026644,6.66694304465092));
#98894=CARTESIAN_POINT('Ctrl Pts',(-2.84857342756987,2.75,6.66694304567485));
#98895=CARTESIAN_POINT('Ctrl Pts',(-3.050258032,2.785926731,6.580769596));
#98896=CARTESIAN_POINT('Ctrl Pts',(-3.246364857,2.821428571,6.482562396));
#98897=CARTESIAN_POINT('Ctrl Pts',(-3.40377395943923,2.84992483970815,6.40373440364824));
#98898=CARTESIAN_POINT('Ctrl Pts',(-3.55717162115202,2.87870320490792,6.31735943591912));
#98899=CARTESIAN_POINT('Ctrl Pts',(-2.94741403646362,2.78894740127666,6.89657527325697));
#98900=CARTESIAN_POINT('Ctrl Pts',(-2.9308291392667,2.78276663836071,6.85830838235336));
#98901=CARTESIAN_POINT('Ctrl Pts',(-2.91428838878772,2.77643548708084,6.82002006788011));
#98902=CARTESIAN_POINT('Ctrl Pts',(-2.88134412019285,2.76346377183966,6.74349049123431));
#98903=CARTESIAN_POINT('Ctrl Pts',(-2.86492097451376,2.75681548747854,6.70520365258805));
#98904=CARTESIAN_POINT('Ctrl Pts',(-2.84857342828654,2.75000000140052,6.66694304349615));
#98905=CARTESIAN_POINT('Ctrl Pts',(-3.17577251,2.749235821,6.79444397800001));
#98906=CARTESIAN_POINT('Ctrl Pts',(-2.807608091,2.813580595,6.966526703));
#98907=CARTESIAN_POINT('Ctrl Pts',(-2.423004915,2.878703203,7.097819889));
#98908=CARTESIAN_POINT('Ctrl Pts',(-2.852862993,2.749235821,6.665108607));
#98909=CARTESIAN_POINT('Ctrl Pts',(-2.491706754,2.813580595,6.819694125));
#98910=CARTESIAN_POINT('Ctrl Pts',(-2.115961384,2.878703203,6.93434982));
#98911=CARTESIAN_POINT('Origin',(0.0463567587563665,2.94638889285433,-0.19055282367663));
#98912=CARTESIAN_POINT('Ctrl Pts',(-1.96045073457827,2.88000589655946,7.239247258558));
#98913=CARTESIAN_POINT('Ctrl Pts',(-1.95647102428913,2.87935454977973,7.240320304779));
#98914=CARTESIAN_POINT('Ctrl Pts',(-1.952491314,2.878703203,7.241393351));
#98915=CARTESIAN_POINT('Ctrl Pts',(-1.776656335,2.84992484,7.288803601));
#98916=CARTESIAN_POINT('Ctrl Pts',(-1.598727514,2.821428571,7.327623785));
#98917=CARTESIAN_POINT('Ctrl Pts',(-1.374649788,2.785541304,7.376512652));
#98918=CARTESIAN_POINT('Ctrl Pts',(-1.148003517,2.7492206,7.41161844200001));
#98919=CARTESIAN_POINT('Ctrl Pts',(-2.12358331591636,2.88000589655946,6.93202404846616));
#98920=CARTESIAN_POINT('Ctrl Pts',(-2.11977234995818,2.87935454977973,6.93318693423308));
#98921=CARTESIAN_POINT('Ctrl Pts',(-2.115961384,2.878703203,6.93434982));
#98922=CARTESIAN_POINT('Ctrl Pts',(-1.947582012,2.84992484,6.985729438));
#98923=CARTESIAN_POINT('Ctrl Pts',(-1.776907359,2.821428571,7.028876172));
#98924=CARTESIAN_POINT('Ctrl Pts',(-1.561965294,2.785541304,7.083213754));
#98925=CARTESIAN_POINT('Ctrl Pts',(-1.344104683,2.7492206,7.12431629));
#98926=CARTESIAN_POINT('',(-1.3487796814196,2.7499999998901,7.12343270402948));
#98927=CARTESIAN_POINT('Ctrl Pts',(-1.34877968312061,2.75,7.12343270523327));
#98928=CARTESIAN_POINT('Ctrl Pts',(-1.564273757,2.785926731,7.082630172));
#98929=CARTESIAN_POINT('Ctrl Pts',(-1.776907359,2.821428571,7.028876172));
#98930=CARTESIAN_POINT('Ctrl Pts',(-1.94758201266314,2.84992483974664,6.98572943782307));
#98931=CARTESIAN_POINT('Ctrl Pts',(-2.11596138701272,2.8787032050476,6.93434983239584));
#98932=CARTESIAN_POINT('Ctrl Pts',(-1.39594531129416,2.78894740124099,7.36894406871015));
#98933=CARTESIAN_POINT('Ctrl Pts',(-1.38797426353557,2.7827665245471,7.32800582015064));
#98934=CARTESIAN_POINT('Ctrl Pts',(-1.38005116146418,2.77643543111063,7.28705729346634));
#98935=CARTESIAN_POINT('Ctrl Pts',(-1.36432877629868,2.76346377184232,7.20523524465428));
#98936=CARTESIAN_POINT('Ctrl Pts',(-1.35652013321739,2.75681548748474,7.16431303999871));
#98937=CARTESIAN_POINT('Ctrl Pts',(-1.34877968347368,2.75000000143294,7.12343270338333));
#98938=CARTESIAN_POINT('Ctrl Pts',(-1.6409201,2.749235821,7.318290868));
#98939=CARTESIAN_POINT('Ctrl Pts',(-1.244370462,2.813580595,7.407205928));
#98940=CARTESIAN_POINT('Ctrl Pts',(-0.840534941,2.878703203,7.452751238));
#98941=CARTESIAN_POINT('Ctrl Pts',(-1.353363311,2.749235821,7.122563285));
#98942=CARTESIAN_POINT('Ctrl Pts',(-0.967419387,2.813580595,7.195896764));
#98943=CARTESIAN_POINT('Ctrl Pts',(-0.575811149000001,2.878703203,7.227097725));
#98944=CARTESIAN_POINT('Origin',(0.00430989000333039,2.94638757434166,-0.19606265922411));
#98945=CARTESIAN_POINT('Ctrl Pts',(-0.3583923162207,2.88000589655946,7.49143663814594));
#98946=CARTESIAN_POINT('Ctrl Pts',(-0.35427497611035,2.87935454977973,7.49162907707297));
#98947=CARTESIAN_POINT('Ctrl Pts',(-0.350157636,2.878703203,7.491821516));
#98948=CARTESIAN_POINT('Ctrl Pts',(-0.168241778,2.84992484,7.500324018));
#98949=CARTESIAN_POINT('Ctrl Pts',(0.013872358,2.821428571,7.499987171));
#98950=CARTESIAN_POINT('Ctrl Pts',(0.243220932,2.785541304,7.499562956));
#98951=CARTESIAN_POINT('Ctrl Pts',(0.472115046,2.7492206,7.485125743));
#98952=CARTESIAN_POINT('Ctrl Pts',(-0.583754856471104,2.88000589655946,
7.22646481878787));
#98953=CARTESIAN_POINT('Ctrl Pts',(-0.579783002735552,2.87935454977973,
7.22678127189393));
#98954=CARTESIAN_POINT('Ctrl Pts',(-0.575811149,2.878703203,7.227097725));
#98955=CARTESIAN_POINT('Ctrl Pts',(-0.400323295,2.84992484,7.241079528));
#98956=CARTESIAN_POINT('Ctrl Pts',(-0.224363648,2.821428571,7.24652751));
#98957=CARTESIAN_POINT('Ctrl Pts',(-0.002765835,2.785541304,7.253388519));
#98958=CARTESIAN_POINT('Ctrl Pts',(0.218837146,2.7492206,7.24669651));
#98959=CARTESIAN_POINT('Ctrl Pts',(0.214081503710257,2.74999999962186,7.24683856131898));
#98960=CARTESIAN_POINT('Ctrl Pts',(0.0675659028784404,2.77401081851383,
7.2511668310443));
#98961=CARTESIAN_POINT('Ctrl Pts',(-0.078714851124164,2.79784107628333,
7.25103702122927));
#98962=CARTESIAN_POINT('Ctrl Pts',(-0.224363649180743,2.82142857122736,
7.24652751019394));
#98963=CARTESIAN_POINT('Ctrl Pts',(-0.341350013056901,2.84037424965354,
7.24290543172649));
#98964=CARTESIAN_POINT('Ctrl Pts',(-0.45856829321948,2.85947647439222,7.23643892552997));
#98965=CARTESIAN_POINT('Ctrl Pts',(-0.575811148978606,2.87870320488418,
7.22709773758857));
#98966=CARTESIAN_POINT('Ctrl Pts',(-1.38354074570591,3.00402491777226,7.11681549624605));
#98967=CARTESIAN_POINT('Ctrl Pts',(-1.37010922035295,3.00629206938617,7.11937410662298));
#98968=CARTESIAN_POINT('Ctrl Pts',(-1.356677695,3.008559221,7.121932717));
#98969=CARTESIAN_POINT('Ctrl Pts',(-0.967145401,3.074309666,7.196135858));
#98970=CARTESIAN_POINT('Ctrl Pts',(-0.571843906,3.139297275,7.227412715));
#98971=CARTESIAN_POINT('Ctrl Pts',(-1.18863048763931,3.00402491777233,7.40579634984612));
#98972=CARTESIAN_POINT('Ctrl Pts',(-1.17465535648591,3.00629206938616,7.40798532109787));
#98973=CARTESIAN_POINT('Ctrl Pts',(-1.16068022533253,3.008559221,7.41017429234949));
#98974=CARTESIAN_POINT('Ctrl Pts',(-0.755382632239146,3.074309666,7.47365740173177));
#98975=CARTESIAN_POINT('Ctrl Pts',(-0.345579041149821,3.139297275,7.49255875910434));
#98976=CARTESIAN_POINT('',(-0.576538528010638,3.13852541863614,7.22703973359675));
#98977=CARTESIAN_POINT('Ctrl Pts',(-0.576538527949452,3.13852541811464,
7.22703973501174));
#98978=CARTESIAN_POINT('Ctrl Pts',(-0.580097416125384,3.13166453921389,
7.26849592895408));
#98979=CARTESIAN_POINT('Ctrl Pts',(-0.583636789832934,3.12496635677949,
7.3100051760473));
#98980=CARTESIAN_POINT('Ctrl Pts',(-0.590672705697527,3.11188594211542,
7.39302866755765));
#98981=CARTESIAN_POINT('Ctrl Pts',(-0.594173108964219,3.10549653061751,
7.43458851627657));
#98982=CARTESIAN_POINT('Ctrl Pts',(-0.597654041416069,3.09925366546798,
7.4761493862768));
#98983=CARTESIAN_POINT('Origin',(0.046862716923752,2.94646386697818,-0.190697407010468));
#98984=CARTESIAN_POINT('Ctrl Pts',(-2.121152813,3.13930489,6.932763572));
#98985=CARTESIAN_POINT('Ctrl Pts',(-1.744059979,3.07388663,7.048139138));
#98986=CARTESIAN_POINT('Ctrl Pts',(-1.356677695,3.008559221,7.121932717));
#98987=CARTESIAN_POINT('Ctrl Pts',(-2.428318655,3.13930489,7.0960037));
#98988=CARTESIAN_POINT('Ctrl Pts',(-2.042346724,3.07388663,7.22808689500001));
#98989=CARTESIAN_POINT('Ctrl Pts',(-1.644325536,3.008559221,7.317526463));
#98990=CARTESIAN_POINT('',(-2.11665928922809,3.13852541864585,6.93413681937955));
#98991=CARTESIAN_POINT('Origin',(0.0504307652673577,3.08928610040167,-0.193189497028357));
#98992=CARTESIAN_POINT('Ctrl Pts',(-2.19083234638042,3.0992536654612,7.17288321586642));
#98993=CARTESIAN_POINT('Ctrl Pts',(-2.17849833215872,3.10549658403016,7.13304197249726));
#98994=CARTESIAN_POINT('Ctrl Pts',(-2.16614568311497,3.11188596847193,7.09320643365134));
#98995=CARTESIAN_POINT('Ctrl Pts',(-2.14142655079244,3.12496644434497,7.01363612678527));
#98996=CARTESIAN_POINT('Ctrl Pts',(-2.12904675200634,3.13166458238639,6.97385848625679));
#98997=CARTESIAN_POINT('Ctrl Pts',(-2.11665928998501,3.13852541825092,6.93413682009051));
#98998=CARTESIAN_POINT('Ctrl Pts',(-2.8810992937521,3.00402491751786,6.65300794161889));
#98999=CARTESIAN_POINT('Ctrl Pts',(-2.86853181487605,3.00629206925893,6.65839411430946));
#99000=CARTESIAN_POINT('Ctrl Pts',(-2.855964336,3.008559221,6.663780287));
#99001=CARTESIAN_POINT('Ctrl Pts',(-2.491490572,3.074309666,6.819986528));
#99002=CARTESIAN_POINT('Ctrl Pts',(-2.112154606,3.139297275,6.935510285));
#99003=CARTESIAN_POINT('Ctrl Pts',(-2.75286827026256,3.00402491751786,6.97713252668685));
#99004=CARTESIAN_POINT('Ctrl Pts',(-2.73969043327862,3.00629206925893,6.98227456139302));
#99005=CARTESIAN_POINT('Ctrl Pts',(-2.72651259629476,3.008559221,6.98741659609931));
#99006=CARTESIAN_POINT('Ctrl Pts',(-2.34433762753113,3.074309666,7.13654250770801));
#99007=CARTESIAN_POINT('Ctrl Pts',(-1.94817824988654,3.139297275,7.24309761967647));
#99008=CARTESIAN_POINT('Origin',(0.0867605426050477,2.94646406243098,-0.176162716798953));
#99009=CARTESIAN_POINT('Ctrl Pts',(-3.561900676,3.13930489,6.314694258));
#99010=CARTESIAN_POINT('Ctrl Pts',(-3.218426399,3.07388663,6.508436221));
#99011=CARTESIAN_POINT('Ctrl Pts',(-2.855964336,3.008559221,6.663780287));
#99012=CARTESIAN_POINT('Ctrl Pts',(-3.896976953,3.13930489,6.408086347));
#99013=CARTESIAN_POINT('Ctrl Pts',(-3.548422814,3.07388663,6.620054066));
#99014=CARTESIAN_POINT('Ctrl Pts',(-3.178934004,3.008559221,6.792965376));
#99015=CARTESIAN_POINT('',(-3.55780741585257,3.13852541863812,6.31700137505845));
#99016=CARTESIAN_POINT('Origin',(0.0907828019625706,3.08928565424525,-0.177833967385367));
#99017=CARTESIAN_POINT('Ctrl Pts',(-3.68156976613604,3.09925366549553,6.53422099858765));
#99018=CARTESIAN_POINT('Ctrl Pts',(-3.66095960104766,3.10549653063559,6.49796298013341));
#99019=CARTESIAN_POINT('Ctrl Pts',(-3.64033219339726,3.11188594217017,6.46171406386782));
#99020=CARTESIAN_POINT('Ctrl Pts',(-3.59908558327855,3.12496646037402,6.38931771480979));
#99021=CARTESIAN_POINT('Ctrl Pts',(-3.57844422745511,3.13166459020887,6.35313139156989));
#99022=CARTESIAN_POINT('Ctrl Pts',(-3.55780741727561,3.13852541813074,6.31700137561132));
#99023=CARTESIAN_POINT('Ctrl Pts',(-4.24394083812014,3.00402491760373,5.87811313046301));
#99024=CARTESIAN_POINT('Ctrl Pts',(-4.23282504806003,3.00629206930187,5.8860750137315));
#99025=CARTESIAN_POINT('Ctrl Pts',(-4.221709258,3.008559221,5.894036897));
#99026=CARTESIAN_POINT('Ctrl Pts',(-3.899336413,3.074309666,6.124942208));
#99027=CARTESIAN_POINT('Ctrl Pts',(-3.553703304,3.139297275,6.319311104));
#99028=CARTESIAN_POINT('Ctrl Pts',(-4.18838499015742,3.00402491760373,6.22222574229489));
#99029=CARTESIAN_POINT('Ctrl Pts',(-4.17662062936595,3.00629206930187,6.23008040435059));
#99030=CARTESIAN_POINT('Ctrl Pts',(-4.16485626857438,3.008559221,6.23793506640633));
#99031=CARTESIAN_POINT('Ctrl Pts',(-3.82367400105311,3.074309666,6.46573081819198));
#99032=CARTESIAN_POINT('Ctrl Pts',(-3.45968280922227,3.139297275,6.65495728658097));
#99033=CARTESIAN_POINT('Origin',(0.122601975476209,2.94646403066942,-0.153393243281784));
#99034=CARTESIAN_POINT('Ctrl Pts',(-4.836098022,3.13930489,5.401356859));
#99035=CARTESIAN_POINT('Ctrl Pts',(-4.542302778,3.07388663,5.664406059));
#99036=CARTESIAN_POINT('Ctrl Pts',(-4.221709258,3.008559221,5.894036897));
#99037=CARTESIAN_POINT('Ctrl Pts',(-5.183416941,3.13930489,5.42053399799999));
#99038=CARTESIAN_POINT('Ctrl Pts',(-4.888578597,3.07388663,5.702474866));
#99039=CARTESIAN_POINT('Ctrl Pts',(-4.564899051,3.008559221,5.950772778));
#99040=CARTESIAN_POINT('',(-4.83259642193341,3.13852541864044,5.40448996693194));
#99041=CARTESIAN_POINT('Origin',(0.126887787059965,3.0892861071041,-0.154158578376543));
#99042=CARTESIAN_POINT('Ctrl Pts',(-5.00016107556263,3.09925366546734,5.5900258693423));
#99043=CARTESIAN_POINT('Ctrl Pts',(-4.97223836249971,3.10549653062517,5.55904611943078));
#99044=CARTESIAN_POINT('Ctrl Pts',(-4.94430076676525,3.11188594216358,5.52807896560806));
#99045=CARTESIAN_POINT('Ctrl Pts',(-4.88845539869022,3.12496646175563,5.46624199840628));
#99046=CARTESIAN_POINT('Ctrl Pts',(-4.86051763957211,3.13166459091205,5.43533897604021));
#99047=CARTESIAN_POINT('Ctrl Pts',(-4.83259642384329,3.13852541817872,5.40448996692781));
#99048=CARTESIAN_POINT('Ctrl Pts',(-5.40834042663095,3.00402491769086,4.8283642821389));
#99049=CARTESIAN_POINT('Ctrl Pts',(-5.3991960873154,3.00629206934543,4.83852958706951));
#99050=CARTESIAN_POINT('Ctrl Pts',(-5.390051748,3.008559221,4.848694892));
#99051=CARTESIAN_POINT('Ctrl Pts',(-5.124853618,3.074309666,5.143502397));
#99052=CARTESIAN_POINT('Ctrl Pts',(-4.829084786,3.139297275,5.407627958));
#99053=CARTESIAN_POINT('Ctrl Pts',(-5.4280574831546,3.00402491769085,5.17637459770828));
#99054=CARTESIAN_POINT('Ctrl Pts',(-5.41825668693024,3.00629206934543,5.18657461173586));
#99055=CARTESIAN_POINT('Ctrl Pts',(-5.40845589070588,3.008559221,5.19677462576344));
#99056=CARTESIAN_POINT('Ctrl Pts',(-5.12421962807818,3.074309666,5.49258874122631));
#99057=CARTESIAN_POINT('Ctrl Pts',(-4.8094164452404,3.139297275,5.75563854733654));
#99058=CARTESIAN_POINT('Origin',(0.152710607699467,2.94646400129146,-0.123451173810367));
#99059=CARTESIAN_POINT('Ctrl Pts',(-5.884164799,3.13930489,4.235458017));
#99060=CARTESIAN_POINT('Ctrl Pts',(-5.653786127,3.07388663,4.555514565));
#99061=CARTESIAN_POINT('Ctrl Pts',(-5.390051748,3.008559221,4.848694892));
#99062=CARTESIAN_POINT('Ctrl Pts',(-6.227486113,3.13930489,4.179523504));
#99063=CARTESIAN_POINT('Ctrl Pts',(-6.000149879,3.07388663,4.51825428));
#99064=CARTESIAN_POINT('Ctrl Pts',(-5.737414491,3.008559221,4.830328659));
#99065=CARTESIAN_POINT('',(-5.88141858947571,3.13852541860795,4.23927061567422));
#99066=CARTESIAN_POINT('Origin',(0.157060863461149,3.08928612816204,-0.123277390314245));
#99067=CARTESIAN_POINT('Ctrl Pts',(-6.0849504101184,3.099253665473,4.38444734373401));
#99068=CARTESIAN_POINT('Ctrl Pts',(-6.05102049225407,3.10549658433644,4.36019423237365));
#99069=CARTESIAN_POINT('Ctrl Pts',(-6.01707919397285,3.11188596863484,4.33595694134614));
#99070=CARTESIAN_POINT('Ctrl Pts',(-5.94924644971696,3.12496646698919,4.28757086998459));
#99071=CARTESIAN_POINT('Ctrl Pts',(-5.91531863784531,3.13166459351811,4.26339614570836));
#99072=CARTESIAN_POINT('Ctrl Pts',(-5.88141859215413,3.13852541824126,4.23927061437438));
#99073=CARTESIAN_POINT('Ctrl Pts',(-6.31985202855174,3.00402491761906,3.55284648476577));
#99074=CARTESIAN_POINT('Ctrl Pts',(-6.31310671877591,3.00629206930957,3.56473989338288));
#99075=CARTESIAN_POINT('Ctrl Pts',(-6.306361409,3.008559221,3.576633302));
#99076=CARTESIAN_POINT('Ctrl Pts',(-6.11073836300001,3.074309666,3.921558131));
#99077=CARTESIAN_POINT('Ctrl Pts',(-5.87866363,3.139297275,4.243090139));
#99078=CARTESIAN_POINT('Ctrl Pts',(-6.41392004154672,3.00402491761906,3.88848192939998));
#99079=CARTESIAN_POINT('Ctrl Pts',(-6.40654108388342,3.00629206930957,3.90055035443249));
#99080=CARTESIAN_POINT('Ctrl Pts',(-6.39916212622019,3.008559221,3.912618779465));
#99081=CARTESIAN_POINT('Ctrl Pts',(-6.18516244016494,3.074309666,4.26261931965024));
#99082=CARTESIAN_POINT('Ctrl Pts',(-5.93426711363373,3.139297275,4.587192546093));
#99083=CARTESIAN_POINT('Origin',(0.17567859128684,2.94646403076769,-0.0877366492637827));
#99084=CARTESIAN_POINT('Ctrl Pts',(-6.65709457100001,3.13930489,2.871513865));
#99085=CARTESIAN_POINT('Ctrl Pts',(-6.500904721,3.07388663,3.233612273));
#99086=CARTESIAN_POINT('Ctrl Pts',(-6.306361409,3.008559221,3.576633302));
#99087=CARTESIAN_POINT('Ctrl Pts',(-6.980364955,3.13930489,2.743083136));
#99088=CARTESIAN_POINT('Ctrl Pts',(-6.83116082000001,3.07388663,3.122765145));
#99089=CARTESIAN_POINT('Ctrl Pts',(-6.641654807,3.008559221,3.48402374));
#99090=CARTESIAN_POINT('',(-6.65523216194324,3.13852541861274,2.8758276813969));
#99091=CARTESIAN_POINT('Origin',(0.179889870119069,3.08928612550937,-0.0866317942447253));
#99092=CARTESIAN_POINT('Ctrl Pts',(-6.88521422635454,3.09925366552483,2.97385693256406));
#99093=CARTESIAN_POINT('Ctrl Pts',(-6.84686419892947,3.10549653068322,2.95746491590425));
#99094=CARTESIAN_POINT('Ctrl Pts',(-6.80850595347592,3.11188594219784,2.94109058031538));
#99095=CARTESIAN_POINT('Ctrl Pts',(-6.73185741844377,3.12496645889943,2.90841773763592));
#99096=CARTESIAN_POINT('Ctrl Pts',(-6.69352594351918,3.13166458955811,2.89210167091627));
#99097=CARTESIAN_POINT('Ctrl Pts',(-6.65523216371794,3.13852541826953,2.87582767950766));
#99098=CARTESIAN_POINT('Ctrl Pts',(-6.93585437234022,3.00402491788988,2.1112015374355));
#99099=CARTESIAN_POINT('Ctrl Pts',(-6.93182349567006,3.00629206944494,2.12426692621775));
#99100=CARTESIAN_POINT('Ctrl Pts',(-6.92779261900001,3.008559221,2.137332315));
#99101=CARTESIAN_POINT('Ctrl Pts',(-6.810891773,3.074309666,2.516246166));
#99102=CARTESIAN_POINT('Ctrl Pts',(-6.653362696,3.139297275,2.880150141));
#99103=CARTESIAN_POINT('Ctrl Pts',(-7.09987482717042,3.0040249178898,2.41876816939517));
#99104=CARTESIAN_POINT('Ctrl Pts',(-7.09526274034048,3.00629206944494,2.43214069834475));
#99105=CARTESIAN_POINT('Ctrl Pts',(-7.09065065351051,3.008559221,2.44551322729433));
#99106=CARTESIAN_POINT('Ctrl Pts',(-6.95689393099661,3.074309666,2.8333345563295));
#99107=CARTESIAN_POINT('Ctrl Pts',(-6.78163804750084,3.139297275,3.20425451918572));
#99108=CARTESIAN_POINT('Origin',(0.1904321565972,2.94646407124334,-0.047919731841701));
#99109=CARTESIAN_POINT('Ctrl Pts',(-7.118745999,3.13930489,1.373300916));
#99110=CARTESIAN_POINT('Ctrl Pts',(-7.044048235,3.07388663,1.760509866));
#99111=CARTESIAN_POINT('Ctrl Pts',(-6.92779261899999,3.008559221,2.137332315));
#99112=CARTESIAN_POINT('Ctrl Pts',(-7.406849691,3.13930489,1.178379249));
#99113=CARTESIAN_POINT('Ctrl Pts',(-7.342754274,3.07388663,1.581258982));
#99114=CARTESIAN_POINT('Ctrl Pts',(-7.235338726,3.008559221,1.974809744));
#99115=CARTESIAN_POINT('',(-7.11785447482644,3.13852541860989,1.37791424072262));
#99116=CARTESIAN_POINT('Origin',(0.19430736713235,3.08928609441336,-0.0459353841119275));
#99117=CARTESIAN_POINT('Ctrl Pts',(-7.36353307773095,3.09925366545253,1.42421227703033));
#99118=CARTESIAN_POINT('Ctrl Pts',(-7.3225555122514,3.10549658262431,1.41644755423299));
#99119=CARTESIAN_POINT('Ctrl Pts',(-7.28157424400658,3.11188596777925,1.40870196489128));
#99120=CARTESIAN_POINT('Ctrl Pts',(-7.19969419612704,3.12496645535936,1.39327019884434));
#99121=CARTESIAN_POINT('Ctrl Pts',(-7.15875140609062,3.13166458779982,1.38557572453528));
#99122=CARTESIAN_POINT('Ctrl Pts',(-7.11785447620099,3.13852541823332,1.37791423874308));
#99123=CARTESIAN_POINT('Ctrl Pts',(-7.22754387541306,3.00402491762742,0.570839149256198));
#99124=CARTESIAN_POINT('Ctrl Pts',(-7.22641591070655,3.00629206931375,0.584465596628102));
#99125=CARTESIAN_POINT('Ctrl Pts',(-7.225287946,3.008559221,0.598092044));
#99126=CARTESIAN_POINT('Ctrl Pts',(-7.192575454,3.074309666,0.993277326));
#99127=CARTESIAN_POINT('Ctrl Pts',(-7.116957917,3.139297275,1.382537524));
#99128=CARTESIAN_POINT('Ctrl Pts',(-7.45384735688251,3.00402491762749,0.835955494763049));
#99129=CARTESIAN_POINT('Ctrl Pts',(-7.45221779643275,3.00629206931374,0.850006844585464));
#99130=CARTESIAN_POINT('Ctrl Pts',(-7.45058823598314,3.008559221,0.86405819440788));
#99131=CARTESIAN_POINT('Ctrl Pts',(-7.40332879350009,3.074309666,1.27156621836309));
#99132=CARTESIAN_POINT('Ctrl Pts',(-7.31190712241195,3.139297275,1.67148911287974));
#99133=CARTESIAN_POINT('Origin',(0.196281286854735,2.94646418661912,-0.00586212603608402));
#99134=CARTESIAN_POINT('Ctrl Pts',(-7.247532776,3.13930489,-0.189126057));
#99135=CARTESIAN_POINT('Ctrl Pts',(-7.257819883,3.07388663,0.205087974));
#99136=CARTESIAN_POINT('Ctrl Pts',(-7.225287946,3.008559221,0.598092044));
#99137=CARTESIAN_POINT('Ctrl Pts',(-7.486998367,3.13930489,-0.441424342));
#99138=CARTESIAN_POINT('Ctrl Pts',(-7.511008699,3.07388663,-0.034185093));
#99139=CARTESIAN_POINT('Ctrl Pts',(-7.490706247,3.008559221,0.373255838));
#99140=CARTESIAN_POINT('',(-7.24765382364659,3.13852541862919,-0.184428939472681));
#99141=CARTESIAN_POINT('Origin',(0.199639167738409,3.08928608524063,-0.0030910937600424));
#99142=CARTESIAN_POINT('Ctrl Pts',(-7.49754130656375,3.09925366544167,-0.19202696212638));
#99143=CARTESIAN_POINT('Ctrl Pts',(-7.45585293515826,3.10549653062226,-0.190801194864911));
#99144=CARTESIAN_POINT('Ctrl Pts',(-7.41416452940221,3.11188594215044,-0.189555930012976));
#99145=CARTESIAN_POINT('Ctrl Pts',(-7.33088131199607,3.12496644638324,-0.187025116539695));
#99146=CARTESIAN_POINT('Ctrl Pts',(-7.28924162669241,3.13166458338676,-0.185738207668968));
#99147=CARTESIAN_POINT('Ctrl Pts',(-7.24765382450455,3.13852541823566,-0.184428940115855));
#99148=CARTESIAN_POINT('Ctrl Pts',(-7.18128145949877,3.00402491793428,-0.996215039478427));
#99149=CARTESIAN_POINT('Ctrl Pts',(-7.18310914924944,3.00629206946718,-0.982664692739221));
#99150=CARTESIAN_POINT('Ctrl Pts',(-7.184936839,3.008559221,-0.969114346));
#99151=CARTESIAN_POINT('Ctrl Pts',(-7.237942301,3.074309666,-0.576136058000001));
#99152=CARTESIAN_POINT('Ctrl Pts',(-7.24777209600001,3.139297275,-0.179721011));
#99153=CARTESIAN_POINT('Ctrl Pts',(-7.45928626934456,3.00402491793435,-0.785945525194474));
#99154=CARTESIAN_POINT('Ctrl Pts',(-7.46071543184991,3.00629206946717,-0.77187238178124));
#99155=CARTESIAN_POINT('Ctrl Pts',(-7.4621445943553,3.008559221,-0.757799238368011));
#99156=CARTESIAN_POINT('Ctrl Pts',(-7.50359223001004,3.074309666,-0.349659143376739));
#99157=CARTESIAN_POINT('Ctrl Pts',(-7.50027954852915,3.139297275,0.0605667338100289));
#99158=CARTESIAN_POINT('Origin',(0.192952530454407,2.94646401362825,0.0364696205494065));
#99159=CARTESIAN_POINT('Ctrl Pts',(-7.03743297500001,3.13930489,-1.742709706));
#99160=CARTESIAN_POINT('Ctrl Pts',(-7.132223939,3.07388663,-1.359923604));
#99161=CARTESIAN_POINT('Ctrl Pts',(-7.184936839,3.008559221,-0.969114346));
#99162=CARTESIAN_POINT('Ctrl Pts',(-7.217063321,3.13930489,-2.040587421));
#99163=CARTESIAN_POINT('Ctrl Pts',(-7.328056705,3.07388663,-1.648030711));
#99164=CARTESIAN_POINT('Ctrl Pts',(-7.39581666999999,3.008559221,-1.245751095));
#99165=CARTESIAN_POINT('',(-7.03856093433481,3.13852541864668,-1.7381484266357));
#99166=CARTESIAN_POINT('Origin',(0.195638787581568,3.08928568804237,0.0398981238858506));
#99167=CARTESIAN_POINT('Ctrl Pts',(-7.28097283682832,3.09925366542448,-1.7992872333711));
#99168=CARTESIAN_POINT('Ctrl Pts',(-7.24052262012714,3.10549653059928,-1.78912835643529));
#99169=CARTESIAN_POINT('Ctrl Pts',(-7.20007656102457,3.11188594216363,-1.77895043030792));
#99170=CARTESIAN_POINT('Ctrl Pts',(-7.11928453719344,3.12496644183097,-1.75857536327087));
#99171=CARTESIAN_POINT('Ctrl Pts',(-7.07889499698815,3.13166458114327,-1.74836723648591));
#99172=CARTESIAN_POINT('Ctrl Pts',(-7.03856093505771,3.13852541823511,-1.73814842746672));
#99173=CARTESIAN_POINT('Ctrl Pts',(-6.79923030407032,3.00402491787842,-2.51668732206627));
#99174=CARTESIAN_POINT('Ctrl Pts',(-6.80392818753517,3.00629206943921,-2.5038466740331));
#99175=CARTESIAN_POINT('Ctrl Pts',(-6.80862607100001,3.008559221,-2.491006026));
#99176=CARTESIAN_POINT('Ctrl Pts',(-6.944871011,3.074309666,-2.11860996));
#99177=CARTESIAN_POINT('Ctrl Pts',(-7.039688507,3.139297275,-1.733575992));
#99178=CARTESIAN_POINT('Ctrl Pts',(-7.11593724543511,3.00402491787835,-2.37109660944742));
#99179=CARTESIAN_POINT('Ctrl Pts',(-7.12035830480933,3.00629206943921,-2.35765971580576));
#99180=CARTESIAN_POINT('Ctrl Pts',(-7.12477936418368,3.008559221,-2.34422282216417));
#99181=CARTESIAN_POINT('Ctrl Pts',(-7.25299603317955,3.074309666,-1.95453483145745));
#99182=CARTESIAN_POINT('Ctrl Pts',(-7.33794723813668,3.139297275,-1.55318767880479));
#99183=CARTESIAN_POINT('Origin',(0.180601220226997,2.94646402715384,0.0770959809799848));
#99184=CARTESIAN_POINT('Ctrl Pts',(-6.49827063,3.13930489,-3.214806186));
#99185=CARTESIAN_POINT('Ctrl Pts',(-6.673133131,3.07388663,-2.861346666));
#99186=CARTESIAN_POINT('Ctrl Pts',(-6.808626071,3.008559221,-2.491006026));
#99187=CARTESIAN_POINT('Ctrl Pts',(-6.609666415,3.13930489,-3.5443349));
#99188=CARTESIAN_POINT('Ctrl Pts',(-6.802452925,3.07388663,-3.184816244));
#99189=CARTESIAN_POINT('Ctrl Pts',(-6.955106924,3.008559221,-2.806508092));
#99190=CARTESIAN_POINT('',(-6.50035275870565,3.13852541865559,-3.21059402478549));
#99191=CARTESIAN_POINT('Origin',(0.182487905431642,3.08928570436188,0.0810218689438846));
#99192=CARTESIAN_POINT('Ctrl Pts',(-6.72395416956975,3.09925366545775,-3.32241483335559));
#99193=CARTESIAN_POINT('Ctrl Pts',(-6.68663319932783,3.10549658336818,-3.30379770709166));
#99194=CARTESIAN_POINT('Ctrl Pts',(-6.64932086725242,3.11188596813281,-3.28516311143848));
#99195=CARTESIAN_POINT('Ctrl Pts',(-6.57479782539728,3.12496645509081,-3.2478965415174));
#99196=CARTESIAN_POINT('Ctrl Pts',(-6.53754705603529,3.13166458763075,-3.22924453809411));
#99197=CARTESIAN_POINT('Ctrl Pts',(-6.50035275940382,3.13852541818432,-3.21059402611261));
#99198=CARTESIAN_POINT('Ctrl Pts',(-6.09925469563289,3.00402491764879,-3.91948210370576));
#99199=CARTESIAN_POINT('Ctrl Pts',(-6.10660310531644,3.00629206932443,-3.90795156835288));
#99200=CARTESIAN_POINT('Ctrl Pts',(-6.113951515,3.008559221,-3.896421033));
#99201=CARTESIAN_POINT('Ctrl Pts',(-6.32706527,3.074309666,-3.562020014));
#99202=CARTESIAN_POINT('Ctrl Pts',(-6.50243690800001,3.139297275,-3.206370886));
#99203=CARTESIAN_POINT('Ctrl Pts',(-6.43985490483353,3.00402491764879,-3.84537785166561));
#99204=CARTESIAN_POINT('Ctrl Pts',(-6.447061137608,3.00629206932443,-3.83320550160551));
#99205=CARTESIAN_POINT('Ctrl Pts',(-6.4542673703825,3.008559221,-3.82103315154535));
#99206=CARTESIAN_POINT('Ctrl Pts',(-6.66325780397382,3.074309666,-3.46801864361758));
#99207=CARTESIAN_POINT('Ctrl Pts',(-6.83250066964433,3.139297275,-3.09431676171783));
#99208=CARTESIAN_POINT('Origin',(0.159805770112958,2.94646404539155,0.114117596465717));
#99209=CARTESIAN_POINT('Ctrl Pts',(-5.655256373,3.13930489,-4.536581902));
#99210=CARTESIAN_POINT('Ctrl Pts',(-5.902014034,3.07388663,-4.228976338));
#99211=CARTESIAN_POINT('Ctrl Pts',(-6.113951515,3.008559221,-3.896421033));
#99212=CARTESIAN_POINT('Ctrl Pts',(-5.693208854,3.13930489,-4.882353218));
#99213=CARTESIAN_POINT('Ctrl Pts',(-5.95877400500001,3.07388663,-4.57268331000001));
#99214=CARTESIAN_POINT('Ctrl Pts',(-6.18918411,3.008559221,-4.23603589));
#99215=CARTESIAN_POINT('',(-5.65819531291536,3.13852541863521,-4.53291581460281));
#99216=CARTESIAN_POINT('Origin',(0.160802047155685,3.0892861315675,0.118355714622324));
#99217=CARTESIAN_POINT('Ctrl Pts',(-5.85253087821732,3.09925366548479,-4.69019000880487));
#99218=CARTESIAN_POINT('Ctrl Pts',(-5.82008485761707,3.10549653062906,-4.66398545664411));
#99219=CARTESIAN_POINT('Ctrl Pts',(-5.78765060893418,3.11188594215404,-4.6377653617038));
#99220=CARTESIAN_POINT('Ctrl Pts',(-5.72288094570733,3.12496645732173,-4.58534969921783));
#99221=CARTESIAN_POINT('Ctrl Pts',(-5.69051071395346,3.1316645887218,-4.55912595969914));
#99222=CARTESIAN_POINT('Ctrl Pts',(-5.65819531327755,3.13852541816991,-4.53291581617428));
#99223=CARTESIAN_POINT('Ctrl Pts',(-5.11408471774542,3.00402491766956,-5.13900625685091));
#99224=CARTESIAN_POINT('Ctrl Pts',(-5.1237400498727,3.00629206933482,-5.12932498992548));
#99225=CARTESIAN_POINT('Ctrl Pts',(-5.13339538200001,3.008559221,-5.119643723));
#99226=CARTESIAN_POINT('Ctrl Pts',(-5.41341298900001,3.074309666,-4.838873972));
#99227=CARTESIAN_POINT('Ctrl Pts',(-5.661138586,3.139297275,-4.529239441));
#99228=CARTESIAN_POINT('Ctrl Pts',(-5.46265210565695,3.00402491766956,-5.13985349841155));
#99229=CARTESIAN_POINT('Ctrl Pts',(-5.47230655614691,3.00629206933482,-5.12951485821149));
#99230=CARTESIAN_POINT('Ctrl Pts',(-5.48196100663686,3.008559221,-5.11917621801155));
#99231=CARTESIAN_POINT('Ctrl Pts',(-5.76195304496934,3.074309666,-4.81934175864121));
#99232=CARTESIAN_POINT('Ctrl Pts',(-6.00757396465741,3.139297275,-4.49075903226973));
#99233=CARTESIAN_POINT('Origin',(0.131537820878708,2.94646399269151,0.145803241099463));
#99234=CARTESIAN_POINT('Ctrl Pts',(-4.547808613,3.13930489,-5.64623209));
#99235=CARTESIAN_POINT('Ctrl Pts',(-4.854923321,3.07388663,-5.398863776));
#99236=CARTESIAN_POINT('Ctrl Pts',(-5.133395382,3.008559221,-5.119643723));
#99237=CARTESIAN_POINT('Ctrl Pts',(-4.510543174,3.13930489,-5.992078127));
#99238=CARTESIAN_POINT('Ctrl Pts',(-4.83646943600001,3.07388663,-5.746736787));
#99239=CARTESIAN_POINT('Ctrl Pts',(-5.133861925,3.008559221,-5.46749135700001));
#99240=CARTESIAN_POINT('',(-4.55146694340282,3.1385254185988,-5.64328349840464));
#99241=CARTESIAN_POINT('Origin',(0.131599621199766,3.08928611816713,0.150156326073493));
#99242=CARTESIAN_POINT('Ctrl Pts',(-4.70744974767339,3.09925366547641,-5.8386571123626));
#99243=CARTESIAN_POINT('Ctrl Pts',(-4.68139528364441,3.10549658273153,-5.8060900009365));
#99244=CARTESIAN_POINT('Ctrl Pts',(-4.65535599040796,3.11188596783253,-5.77351065652436));
#99245=CARTESIAN_POINT('Ctrl Pts',(-4.60336851064653,3.12496646117916,-5.70839698870686));
#99246=CARTESIAN_POINT('Ctrl Pts',(-4.57739241382684,3.13166459063262,-5.67582771278378));
#99247=CARTESIAN_POINT('Ctrl Pts',(-4.55146694245507,3.13852541818957,-5.64328350085494));
#99248=CARTESIAN_POINT('Ctrl Pts',(-3.88978582096491,3.00402491769316,-6.11823618949679));
#99249=CARTESIAN_POINT('Ctrl Pts',(-3.90129660298243,3.00629206934662,-6.1108568762484));
#99250=CARTESIAN_POINT('Ctrl Pts',(-3.912807385,3.008559221,-6.103477563));
#99251=CARTESIAN_POINT('Ctrl Pts',(-4.246635534,3.074309666,-5.889467561));
#99252=CARTESIAN_POINT('Ctrl Pts',(-4.55513171500001,3.139297275,-5.640325794));
#99253=CARTESIAN_POINT('Ctrl Pts',(-4.23002176692898,3.00402491769317,-6.19399530754654));
#99254=CARTESIAN_POINT('Ctrl Pts',(-4.24167300366235,3.00629206934662,-6.18597380052345));
#99255=CARTESIAN_POINT('Ctrl Pts',(-4.25332424039563,3.008559221,-6.17795229350047));
#99256=CARTESIAN_POINT('Ctrl Pts',(-4.59122576492328,3.074309666,-5.94531780892835));
#99257=CARTESIAN_POINT('Ctrl Pts',(-4.90173977734594,3.139297275,-5.67721840210349));
#99258=CARTESIAN_POINT('Origin',(0.0971190746813649,2.94646403943336,0.170671054066455));
#99259=CARTESIAN_POINT('Ctrl Pts',(-3.227710377,3.13930489,-6.491870741));
#99260=CARTESIAN_POINT('Ctrl Pts',(-3.580821789,3.07388663,-6.316306345));
#99261=CARTESIAN_POINT('Ctrl Pts',(-3.912807385,3.008559221,-6.103477563));
#99262=CARTESIAN_POINT('Ctrl Pts',(-3.116969508,3.13930489,-6.821620122));
#99263=CARTESIAN_POINT('Ctrl Pts',(-3.488016932,3.07388663,-6.652079238));
#99264=CARTESIAN_POINT('Ctrl Pts',(-3.838486062,3.008559221,-6.443293005));
#99265=CARTESIAN_POINT('',(-3.23191703699021,3.13852541864447,-6.48977751941203));
#99266=CARTESIAN_POINT('Origin',(0.0962436524403354,3.08928611387826,0.174935665362964));
#99267=CARTESIAN_POINT('Ctrl Pts',(-3.34225349900584,3.09925366545698,-6.7141150980915));
#99268=CARTESIAN_POINT('Ctrl Pts',(-3.3238092940059,3.10549653061459,-6.6767087602362));
#99269=CARTESIAN_POINT('Ctrl Pts',(-3.30538229912358,3.11188594216861,-6.63929325890792));
#99270=CARTESIAN_POINT('Ctrl Pts',(-3.26860772366043,3.12496645256281,-6.56452604360213));
#99271=CARTESIAN_POINT('Ctrl Pts',(-3.25024035225307,3.13166458640041,-6.52713410004394));
#99272=CARTESIAN_POINT('Ctrl Pts',(-3.23191703633812,3.13852541819882,-6.48977752054084));
#99273=CARTESIAN_POINT('Ctrl Pts',(-2.48360486417183,3.00402491773169,-6.8113841981799));
#99274=CARTESIAN_POINT('Ctrl Pts',(-2.49643286458595,3.00629206936588,-6.80665188708994));
#99275=CARTESIAN_POINT('Ctrl Pts',(-2.509260865,3.008559221,-6.801919576));
#99276=CARTESIAN_POINT('Ctrl Pts',(-2.881290121,3.074309666,-6.664676193));
#99277=CARTESIAN_POINT('Ctrl Pts',(-3.236131948,3.139297275,-6.487676781));
#99278=CARTESIAN_POINT('Ctrl Pts',(-2.79960031072545,3.00402491773169,-6.95851278007885));
#99279=CARTESIAN_POINT('Ctrl Pts',(-2.8127035348095,3.00629206936588,-6.95318348297372));
#99280=CARTESIAN_POINT('Ctrl Pts',(-2.82580675889353,3.008559221,-6.94785418586859));
#99281=CARTESIAN_POINT('Ctrl Pts',(-3.20581787129103,3.074309666,-6.79329740593167));
#99282=CARTESIAN_POINT('Ctrl Pts',(-3.5667056870988,3.139297275,-6.59821734858096));
#99283=CARTESIAN_POINT('Origin',(0.0581592152221827,2.94646401333924,0.18755850573811));
#99284=CARTESIAN_POINT('Ctrl Pts',(-1.756687991,3.13930489,-7.033956732));
#99285=CARTESIAN_POINT('Ctrl Pts',(-2.13928501,3.07388663,-6.93840544900001));
#99286=CARTESIAN_POINT('Ctrl Pts',(-2.509260865,3.008559221,-6.801919576));
#99287=CARTESIAN_POINT('Ctrl Pts',(-1.577649813,3.13930489,-7.332190741));
#99288=CARTESIAN_POINT('Ctrl Pts',(-1.976468632,3.07388663,-7.24637785700001));
#99289=CARTESIAN_POINT('Ctrl Pts',(-2.363626857,3.008559221,-7.11781343400001));
#99290=CARTESIAN_POINT('',(-1.76124628360345,3.13852541859317,-7.03281675504062));
#99291=CARTESIAN_POINT('Origin',(0.0563876163800928,3.08928612119298,0.191535565089408));
#99292=CARTESIAN_POINT('Ctrl Pts',(-1.82077719099447,3.09925366550455,-7.27562852393233));
#99293=CARTESIAN_POINT('Ctrl Pts',(-1.81080545823739,3.10549653066451,-7.23513176665341));
#99294=CARTESIAN_POINT('Ctrl Pts',(-1.80085250313915,3.11188594219304,-7.19462975998299));
#99295=CARTESIAN_POINT('Ctrl Pts',(-1.78101041491928,3.12496646786567,-7.11370501954715));
#99296=CARTESIAN_POINT('Ctrl Pts',(-1.7711106374316,3.13166459393754,-7.07323888725074));
#99297=CARTESIAN_POINT('Ctrl Pts',(-1.76124628168251,3.13852541820015,-7.03281675696655));
#99298=CARTESIAN_POINT('Ctrl Pts',(-0.961293304380143,3.00402491792402,
-7.18603945161995));
#99299=CARTESIAN_POINT('Ctrl Pts',(-0.974838699690071,3.00629206946205,
-7.18417542030998));
#99300=CARTESIAN_POINT('Ctrl Pts',(-0.988384095,3.008559221,-7.182311389));
#99301=CARTESIAN_POINT('Ctrl Pts',(-1.381218784,3.074309666,-7.128251973));
#99302=CARTESIAN_POINT('Ctrl Pts',(-1.765814248,3.139297275,-7.031671213));
#99303=CARTESIAN_POINT('Ctrl Pts',(-1.23827265637212,3.0040249179241,-7.39765792970278));
#99304=CARTESIAN_POINT('Ctrl Pts',(-1.25221517513604,3.00629206946205,-7.39527003453434));
#99305=CARTESIAN_POINT('Ctrl Pts',(-1.26615769389991,3.008559221,-7.39288213936585));
#99306=CARTESIAN_POINT('Ctrl Pts',(-1.67050949738474,3.074309666,-7.32362996662319));
#99307=CARTESIAN_POINT('Ctrl Pts',(-2.06489640124521,3.139297275,-7.2106909852025));
#99308=CARTESIAN_POINT('Origin',(0.0164799599938099,2.94646400269109,0.195676067964657));
#99309=CARTESIAN_POINT('Ctrl Pts',(-0.203524827,3.13930489,-7.24714272300001));
#99310=CARTESIAN_POINT('Ctrl Pts',(-0.597717642,3.07388663,-7.236072426));
#99311=CARTESIAN_POINT('Ctrl Pts',(-0.988384095,3.008559221,-7.182311389));
#99312=CARTESIAN_POINT('Ctrl Pts',(0.035439035,3.13930489,-7.499916271));
#99313=CARTESIAN_POINT('Ctrl Pts',(-0.372502856,3.07388663,-7.50184390200001));
#99314=CARTESIAN_POINT('Ctrl Pts',(-0.778247087,3.008559221,-7.459512817));
#99315=CARTESIAN_POINT('',(-0.20822160905804,3.13852541863702,-7.24700929639271));
#99316=CARTESIAN_POINT('Origin',(0.0138950876829804,3.08928569839221,0.19918167042057));
#99317=CARTESIAN_POINT('Ctrl Pts',(-0.214163364830849,3.09925366989869,
-7.4969416169044));
#99318=CARTESIAN_POINT('Ctrl Pts',(-0.213130371432416,3.10549653514307,
-7.45524802340234));
#99319=CARTESIAN_POINT('Ctrl Pts',(-0.212116845861233,3.11188594217775,
-7.41355336952049));
#99320=CARTESIAN_POINT('Ctrl Pts',(-0.210135086285302,3.1249664382743,-7.33025533037589));
#99321=CARTESIAN_POINT('Ctrl Pts',(-0.209165779932897,3.13166457940977,
-7.28860701383298));
#99322=CARTESIAN_POINT('Ctrl Pts',(-0.208221608534527,3.13852541825656,
-7.24700929713044));
#99323=CARTESIAN_POINT('Ctrl Pts',(0.589277982209245,3.00680105370404,-7.22601992003964));
#99324=CARTESIAN_POINT('Ctrl Pts',(0.583993199604623,3.00768013735202,-7.22644311151983));
#99325=CARTESIAN_POINT('Ctrl Pts',(0.578708417,3.008559221,-7.226866303));
#99326=CARTESIAN_POINT('Ctrl Pts',(0.183436808,3.074309666,-7.258518613));
#99327=CARTESIAN_POINT('Ctrl Pts',(-0.212929036,3.139297275,-7.246872513));
#99328=CARTESIAN_POINT('Ctrl Pts',(0.363937708262816,3.00680105370404,-7.49137623361797));
#99329=CARTESIAN_POINT('Ctrl Pts',(0.358459120241673,3.00768013735202,-7.4916343573119));
#99330=CARTESIAN_POINT('Ctrl Pts',(0.352980532220529,3.008559221,-7.49189248100584));
#99331=CARTESIAN_POINT('Ctrl Pts',(-0.0567866170036243,3.074309666,-7.51119866168644));
#99332=CARTESIAN_POINT('Ctrl Pts',(-0.466215022260595,3.139297275,-7.48569914997869));
#99333=CARTESIAN_POINT('Origin',(-0.0259698947464153,2.94646402789277,0.194643709377537));
#99334=CARTESIAN_POINT('Ctrl Pts',(1.359154932,3.13930489,-7.121460375));
#99335=CARTESIAN_POINT('Ctrl Pts',(0.971798339000001,3.07388663,-7.195388698));
#99336=CARTESIAN_POINT('Ctrl Pts',(0.578708417,3.008559221,-7.226866303));
#99337=CARTESIAN_POINT('Ctrl Pts',(1.646870792,3.13930489,-7.316954052));
#99338=CARTESIAN_POINT('Ctrl Pts',(1.24888074,3.07388663,-7.40653206300001));
#99339=CARTESIAN_POINT('Ctrl Pts',(0.843522651,3.008559221,-7.45241367199999));
#99340=CARTESIAN_POINT('',(1.3545392753172,3.13852541865081,-7.12233973722032));
#99341=CARTESIAN_POINT('Origin',(-0.0292476493493499,3.08928608977801,0.197509355480461));
#99342=CARTESIAN_POINT('Ctrl Pts',(1.40246450071478,3.0992536654408,-7.36770611019148));
#99343=CARTESIAN_POINT('Ctrl Pts',(1.39451038722841,3.10549658239958,-7.32676488706771));
#99344=CARTESIAN_POINT('Ctrl Pts',(1.3865371282657,3.11188596766313,-7.2858273040236));
#99345=CARTESIAN_POINT('Ctrl Pts',(1.37056594371818,3.12496646028372,-7.20405072874484));
#99346=CARTESIAN_POINT('Ctrl Pts',(1.36255944570165,3.13166459020175,-7.16316782787836));
#99347=CARTESIAN_POINT('Ctrl Pts',(1.35453927636302,3.13852541819903,-7.12233973829615));
#99348=CARTESIAN_POINT('Ctrl Pts',(2.14489347757516,3.00402491757735,-6.92550935161478));
#99349=CARTESIAN_POINT('Ctrl Pts',(2.13181732228758,3.00629206928867,-6.92950516680737));
#99350=CARTESIAN_POINT('Ctrl Pts',(2.118741167,3.008559221,-6.933500982));
#99351=CARTESIAN_POINT('Ctrl Pts',(1.739515099,3.074309666,-7.04938499));
#99352=CARTESIAN_POINT('Ctrl Pts',(1.349912501,3.139297275,-7.12321811));
#99353=CARTESIAN_POINT('Ctrl Pts',(1.9823701178637,3.00402491757735,-7.23386969212132));
#99354=CARTESIAN_POINT('Ctrl Pts',(1.96871357834968,3.00629206928867,-7.23755680916065));
#99355=CARTESIAN_POINT('Ctrl Pts',(1.95505703883561,3.008559221,-7.24124392619998));
#99356=CARTESIAN_POINT('Ctrl Pts',(1.55899904866107,3.074309666,-7.3481752730931));
#99357=CARTESIAN_POINT('Ctrl Pts',(1.15364134055402,3.139297275,-7.41127339163886));
#99358=CARTESIAN_POINT('Origin',(-0.0672054225525906,2.94646403236397,0.184510496212321));
#99359=CARTESIAN_POINT('Ctrl Pts',(2.858282117,3.13930489,-6.662786455));
#99360=CARTESIAN_POINT('Ctrl Pts',(2.49587411,3.07388663,-6.81825659200001));
#99361=CARTESIAN_POINT('Ctrl Pts',(2.118741167,3.008559221,-6.933500982));
#99362=CARTESIAN_POINT('Ctrl Pts',(3.181296702,3.13930489,-6.79185919300001));
#99363=CARTESIAN_POINT('Ctrl Pts',(2.81186806,3.07388663,-6.964899017));
#99364=CARTESIAN_POINT('Ctrl Pts',(2.425850208,3.008559221,-7.096847946));
#99365=CARTESIAN_POINT('',(2.85396340807885,3.13852541866625,-6.66463748776731));
#99366=CARTESIAN_POINT('Origin',(-0.0710225736237424,3.08928608316363,0.186604418638494));
#99367=CARTESIAN_POINT('Ctrl Pts',(2.9535146859888,3.0992536654475,-6.89396482448299));
#99368=CARTESIAN_POINT('Ctrl Pts',(2.93694538232829,3.10549658248996,-6.85569068315969));
#99369=CARTESIAN_POINT('Ctrl Pts',(2.92035816359901,3.11188596772589,-6.81742421322633));
#99370=CARTESIAN_POINT('Ctrl Pts',(2.8871808228278,3.12496646321178,-6.74099284469479));
#99371=CARTESIAN_POINT('Ctrl Pts',(2.87057290089434,3.13166459168363,-6.70278693262248));
#99372=CARTESIAN_POINT('Ctrl Pts',(2.85396340960551,3.13852541826454,-6.66463748835739));
#99373=CARTESIAN_POINT('Ctrl Pts',(3.58352685288815,3.00402491774724,-6.30250609728324));
#99374=CARTESIAN_POINT('Ctrl Pts',(3.5716153934441,3.00629206937366,-6.30921947914162));
#99375=CARTESIAN_POINT('Ctrl Pts',(3.559703934,3.008559221,-6.315932861));
#99376=CARTESIAN_POINT('Ctrl Pts',(3.214255597,3.074309666,-6.51062996));
#99377=CARTESIAN_POINT('Ctrl Pts',(2.84963363,3.139297275,-6.666489944));
#99378=CARTESIAN_POINT('Ctrl Pts',(3.49109155714461,3.00402491774723,-6.63859486252414));
#99379=CARTESIAN_POINT('Ctrl Pts',(3.47854692157417,3.00629206937366,-6.64513152886113));
#99380=CARTESIAN_POINT('Ctrl Pts',(3.46600228600367,3.008559221,-6.65166819519811));
#99381=CARTESIAN_POINT('Ctrl Pts',(3.10219099013011,3.074309666,-6.841240306511));
#99382=CARTESIAN_POINT('Ctrl Pts',(2.71987455123701,3.139297275,-6.9900031514952));
#99383=CARTESIAN_POINT('Origin',(-0.10529845987564,2.94646405132947,0.16574949656218));
#99384=CARTESIAN_POINT('Ctrl Pts',(4.223759206,3.13930489,-5.892568045));
#99385=CARTESIAN_POINT('Ctrl Pts',(3.903245582,3.07388663,-6.122310386));
#99386=CARTESIAN_POINT('Ctrl Pts',(3.559703934,3.008559221,-6.315932861));
#99387=CARTESIAN_POINT('Ctrl Pts',(4.566968713,3.13930489,-5.94918454700001));
#99388=CARTESIAN_POINT('Ctrl Pts',(4.243375555,3.07388663,-6.19759503400001));
#99389=CARTESIAN_POINT('Ctrl Pts',(3.894747705,3.008559221,-6.409441498));
#99390=CARTESIAN_POINT('',(4.21993938413285,3.13852541865766,-5.89530419657678));
#99391=CARTESIAN_POINT('Origin',(-0.109476389222967,3.08928612558317,0.166973696339344));
#99392=CARTESIAN_POINT('Ctrl Pts',(4.36646180685914,3.09925366547009,-6.09786940580673));
#99393=CARTESIAN_POINT('Ctrl Pts',(4.34205207570782,3.10549658240008,-6.06405200370254));
#99394=CARTESIAN_POINT('Ctrl Pts',(4.31762649685015,3.1118859676776,-6.0302459439873));
#99395=CARTESIAN_POINT('Ctrl Pts',(4.26879433194001,3.12496646502922,-5.96273363615785));
#99396=CARTESIAN_POINT('Ctrl Pts',(4.24436155596421,3.13166459254897,-5.92899117441959));
#99397=CARTESIAN_POINT('Ctrl Pts',(4.21993938576901,3.13852541822334,-5.89530419695904));
#99398=CARTESIAN_POINT('Ctrl Pts',(4.85459849685151,3.00402491777864,-5.38480466232962));
#99399=CARTESIAN_POINT('Ctrl Pts',(4.84440869942573,3.00629206938932,-5.3939217006648));
#99400=CARTESIAN_POINT('Ctrl Pts',(4.83421890200001,3.008559221,-5.403038739));
#99401=CARTESIAN_POINT('Ctrl Pts',(4.538701076,3.074309666,-5.66744510900001));
#99402=CARTESIAN_POINT('Ctrl Pts',(4.216109057,3.139297275,-5.898044118));
#99403=CARTESIAN_POINT('Ctrl Pts',(4.8365734368469,3.00402491777864,-5.73290671558476));
#99404=CARTESIAN_POINT('Ctrl Pts',(4.82572727799302,3.00629206938932,-5.74198728403669));
#99405=CARTESIAN_POINT('Ctrl Pts',(4.81488111913914,3.008559221,-5.75106785248864));
#99406=CARTESIAN_POINT('Ctrl Pts',(4.50032792921482,3.074309666,-6.01441654683934));
#99407=CARTESIAN_POINT('Ctrl Pts',(4.15892944979653,3.139297275,-6.24188813282856));
#99408=CARTESIAN_POINT('Origin',(-0.138467891961084,2.94646404519457,0.13923832246165));
#99409=CARTESIAN_POINT('Ctrl Pts',(5.39173801,3.13930489,-4.846819703));
#99410=CARTESIAN_POINT('Ctrl Pts',(5.128105628,3.07388663,-5.14009175));
#99411=CARTESIAN_POINT('Ctrl Pts',(4.834218902,3.008559221,-5.403038739));
#99412=CARTESIAN_POINT('Ctrl Pts',(5.739094344,3.13930489,-4.828332643));
#99413=CARTESIAN_POINT('Ctrl Pts',(5.476467525,3.07388663,-5.140498395));
#99414=CARTESIAN_POINT('Ctrl Pts',(5.181531129,3.008559221,-5.42233668900001));
#99415=CARTESIAN_POINT('',(5.38859568422891,3.13852541862581,-4.85031303434529));
#99416=CARTESIAN_POINT('Origin',(-0.142811494543745,3.08928612771913,0.139535953325501));
#99417=CARTESIAN_POINT('Ctrl Pts',(5.57523802689835,3.09925366543971,-5.0166443907419));
#99418=CARTESIAN_POINT('Ctrl Pts',(5.54412949788754,3.10549653059208,-4.9888652217637));
#99419=CARTESIAN_POINT('Ctrl Pts',(5.51300753522168,3.11188594214901,-4.96110018408167));
#99420=CARTESIAN_POINT('Ctrl Pts',(5.45080379357747,3.12496645952399,-4.90566366378266));
#99421=CARTESIAN_POINT('Ctrl Pts',(5.41968859661435,3.13166458985593,-4.87796239430588));
#99422=CARTESIAN_POINT('Ctrl Pts',(5.38859568661649,3.1385254182622,-4.85031303352164));
#99423=CARTESIAN_POINT('Ctrl Pts',(5.89867451036487,3.00402491759344,-4.21531574453703));
#99424=CARTESIAN_POINT('Ctrl Pts',(5.89068283818242,3.00629206929675,-4.22641013726852));
#99425=CARTESIAN_POINT('Ctrl Pts',(5.882691166,3.008559221,-4.23750453));
#99426=CARTESIAN_POINT('Ctrl Pts',(5.650921937,3.074309666,-4.559256823));
#99427=CARTESIAN_POINT('Ctrl Pts',(5.385443911,3.139297275,-4.853812304));
#99428=CARTESIAN_POINT('Ctrl Pts',(5.95590251824537,3.00402491759345,-4.55915422034929));
#99429=CARTESIAN_POINT('Ctrl Pts',(5.94726199003128,3.00629206929675,-4.57035409416915));
#99430=CARTESIAN_POINT('Ctrl Pts',(5.93862146181731,3.008559221,-4.58155396798899));
#99431=CARTESIAN_POINT('Ctrl Pts',(5.68803453625319,3.074309666,-4.90636535425118));
#99432=CARTESIAN_POINT('Ctrl Pts',(5.40351742967199,3.139297275,-5.20190936246538));
#99433=CARTESIAN_POINT('Origin',(-0.165164502112501,2.94646446502014,0.106218016553463));
#99434=CARTESIAN_POINT('Ctrl Pts',(6.307605137,3.13930489,-3.574439458));
#99435=CARTESIAN_POINT('Ctrl Pts',(6.113181154,3.07388663,-3.917528137));
#99436=CARTESIAN_POINT('Ctrl Pts',(5.882691166,3.008559221,-4.23750453));
#99437=CARTESIAN_POINT('Ctrl Pts',(6.64286630100001,3.13930489,-3.481713272));
#99438=CARTESIAN_POINT('Ctrl Pts',(6.453485961,3.07388663,-3.843037764));
#99439=CARTESIAN_POINT('Ctrl Pts',(6.226031915,3.008559221,-4.181689442));
#99440=CARTESIAN_POINT('',(6.30528723953085,3.13852541858252,-3.57852662505442));
#99441=CARTESIAN_POINT('Origin',(-0.169468734258327,3.08928610863066,0.105573437156782));
#99442=CARTESIAN_POINT('Ctrl Pts',(6.52332231319454,3.09925366544933,-3.70084665970846));
#99443=CARTESIAN_POINT('Ctrl Pts',(6.48696938400141,3.10549653060211,-3.68040436650827));
#99444=CARTESIAN_POINT('Ctrl Pts',(6.45060637303851,3.11188594215306,-3.65997876206266));
#99445=CARTESIAN_POINT('Ctrl Pts',(6.37793973874896,3.12496645377077,-3.61921030050866));
#99446=CARTESIAN_POINT('Ctrl Pts',(6.34159702665588,3.13166458699902,-3.59884550943043));
#99447=CARTESIAN_POINT('Ctrl Pts',(6.30528724135634,3.13852541819247,-3.5785266235761));
#99448=CARTESIAN_POINT('Ctrl Pts',(6.66693505965315,3.00402491762771,-2.84872334858325));
#99449=CARTESIAN_POINT('Ctrl Pts',(6.66151519482659,3.00629206931389,-2.8612763337916));
#99450=CARTESIAN_POINT('Ctrl Pts',(6.65609533,3.008559221,-2.873829319));
#99451=CARTESIAN_POINT('Ctrl Pts',(6.498911968,3.074309666,-3.237882756));
#99452=CARTESIAN_POINT('Ctrl Pts',(6.302961392,3.139297275,-3.582621622));
#99453=CARTESIAN_POINT('Ctrl Pts',(6.7967402167303,3.00402491762771,-3.17222074183296));
#99454=CARTESIAN_POINT('Ctrl Pts',(6.7907093411173,3.00629206931389,-3.18501622689353));
#99455=CARTESIAN_POINT('Ctrl Pts',(6.78467846550414,3.008559221,-3.19781171195412));
#99456=CARTESIAN_POINT('Ctrl Pts',(6.60977496975106,3.074309666,-3.56889797048598));
#99457=CARTESIAN_POINT('Ctrl Pts',(6.39544294078199,3.139297275,-3.91869509171463));
#99458=CARTESIAN_POINT('Origin',(-0.184134812493184,2.94646404232351,0.0682281691969916));
#99459=CARTESIAN_POINT('Ctrl Pts',(6.928535658,3.13930489,-2.134922397));
#99460=CARTESIAN_POINT('Ctrl Pts',(6.812411124,3.07388663,-2.511785262));
#99461=CARTESIAN_POINT('Ctrl Pts',(6.65609533,3.008559221,-2.873829319));
#99462=CARTESIAN_POINT('Ctrl Pts',(7.236025213,3.13930489,-1.972292858));
#99463=CARTESIAN_POINT('Ctrl Pts',(7.128746565,3.07388663,-2.365880959));
#99464=CARTESIAN_POINT('Ctrl Pts',(6.979410369,3.008559221,-2.745511045));
#99465=CARTESIAN_POINT('',(6.92715057170216,3.13852541858868,-2.13941228764284));
#99466=CARTESIAN_POINT('Origin',(-0.188201868409005,3.08928612478781,0.0666744331105723));
#99467=CARTESIAN_POINT('Ctrl Pts',(7.16638329785451,3.0992536654575,-2.21200145241879));
#99468=CARTESIAN_POINT('Ctrl Pts',(7.12648545168685,3.10549658374615,-2.1998517903871));
#99469=CARTESIAN_POINT('Ctrl Pts',(7.08658186675109,3.11188596832624,-2.18772075263819));
#99470=CARTESIAN_POINT('Ctrl Pts',(7.00685022097463,3.12496646406064,-2.16352664264606));
#99471=CARTESIAN_POINT('Ctrl Pts',(6.96697938663559,3.1316645920718,-2.1514505879326));
#99472=CARTESIAN_POINT('Ctrl Pts',(6.92715057360104,3.13852541822036,-2.13941228563729));
#99473=CARTESIAN_POINT('Ctrl Pts',(7.12345713528118,3.00402491764723,-1.34892781591291));
#99474=CARTESIAN_POINT('Ctrl Pts',(7.12086250464065,3.00629206932365,-1.36235242995646));
#99475=CARTESIAN_POINT('Ctrl Pts',(7.118267874,3.008559221,-1.375777044));
#99476=CARTESIAN_POINT('Ctrl Pts',(7.04302009900001,3.074309666,-1.76510889));
#99477=CARTESIAN_POINT('Ctrl Pts',(6.925759405,3.139297275,-2.143911534));
#99478=CARTESIAN_POINT('Ctrl Pts',(7.31976989663,3.00402491764723,-1.6369577478844));
#99479=CARTESIAN_POINT('Ctrl Pts',(7.3166306705952,3.00629206932366,-1.65075054153846));
#99480=CARTESIAN_POINT('Ctrl Pts',(7.3134914445603,3.008559221,-1.66454333519246));
#99481=CARTESIAN_POINT('Ctrl Pts',(7.22244967135065,3.074309666,-2.06455288462094));
#99482=CARTESIAN_POINT('Ctrl Pts',(7.08832464742211,3.139297275,-2.45224699367283));
#99483=CARTESIAN_POINT('Origin',(-0.194497013819791,2.94646404265204,0.0270495149303721));
#99484=CARTESIAN_POINT('Ctrl Pts',(7.225495552,3.13930489,-0.595578738));
#99485=CARTESIAN_POINT('Ctrl Pts',(7.193100321,3.07388663,-0.988594101));
#99486=CARTESIAN_POINT('Ctrl Pts',(7.118267874,3.008559221,-1.375777044));
#99487=CARTESIAN_POINT('Ctrl Pts',(7.490835629,3.13930489,-0.370650221));
#99488=CARTESIAN_POINT('Ctrl Pts',(7.47067490300001,3.07388663,-0.77809819));
#99489=CARTESIAN_POINT('Ctrl Pts',(7.406439351,3.008559221,-1.180955603));
#99490=CARTESIAN_POINT('',(7.22510804225623,3.13852541859739,-0.60026140928089));
#99491=CARTESIAN_POINT('Origin',(-0.198134895537586,3.08928611241096,0.0246577965307507));
#99492=CARTESIAN_POINT('Ctrl Pts',(7.47435216496847,3.0992536654315,-0.619725515399642));
#99493=CARTESIAN_POINT('Ctrl Pts',(7.43277529403877,3.10549658313059,-0.616436763639562));
#99494=CARTESIAN_POINT('Ctrl Pts',(7.39119681605539,3.11188596802581,-0.613167433926877));
#99495=CARTESIAN_POINT('Ctrl Pts',(7.30812831330693,3.12496645117645,-0.606678922198451));
#99496=CARTESIAN_POINT('Ctrl Pts',(7.26659359855861,3.13166458574274,-0.603456246411873));
#99497=CARTESIAN_POINT('Ctrl Pts',(7.22510804347203,3.13852541824124,-0.600261407597791));
#99498=CARTESIAN_POINT('Ctrl Pts',(7.2468942729035,3.00402491774289,0.213942082252785));
#99499=CARTESIAN_POINT('Ctrl Pts',(7.24724619845171,3.00629206937144,0.200273559626389));
#99500=CARTESIAN_POINT('Ctrl Pts',(7.247598124,3.008559221,0.186605037));
#99501=CARTESIAN_POINT('Ctrl Pts',(7.25780443800001,3.074309666,-0.209800494));
#99502=CARTESIAN_POINT('Ctrl Pts',(7.22471660500001,3.139297275,-0.604954526));
#99503=CARTESIAN_POINT('Ctrl Pts',(7.50053527194251,3.00402491774289,-0.0251524289314449));
#99504=CARTESIAN_POINT('Ctrl Pts',(7.50043448218546,3.00629206937144,-0.0392975952519484));
#99505=CARTESIAN_POINT('Ctrl Pts',(7.50033369242839,3.008559221,-0.0534427615724517));
#99506=CARTESIAN_POINT('Ctrl Pts',(7.49741065398017,3.074309666,-0.46367160046222));
#99507=CARTESIAN_POINT('Ctrl Pts',(7.4497641724016,3.139297275,-0.871134551944614));
#99508=CARTESIAN_POINT('Origin',(-0.195764717091161,2.94646402749331,-0.0153939945164652));
#99509=CARTESIAN_POINT('Ctrl Pts',(7.184599304,3.13930489,0.971613522));
#99510=CARTESIAN_POINT('Ctrl Pts',(7.237448142,3.07388663,0.580822623));
#99511=CARTESIAN_POINT('Ctrl Pts',(7.247598124,3.008559221,0.186605037));
#99512=CARTESIAN_POINT('Ctrl Pts',(7.395382895,3.13930489,1.248323608));
#99513=CARTESIAN_POINT('Ctrl Pts',(7.463282786,3.07388663,0.846067586));
#99514=CARTESIAN_POINT('Ctrl Pts',(7.487151461,3.008559221,0.43882001));
#99515=CARTESIAN_POINT('',(7.1852274901126,3.13852541864547,0.966957026736903));
#99516=CARTESIAN_POINT('Origin',(-0.198803195774695,3.08928614354635,-0.0185118389669156));
#99517=CARTESIAN_POINT('Ctrl Pts',(7.43282863154986,3.09925366549633,1.00152809855961));
#99518=CARTESIAN_POINT('Ctrl Pts',(7.39151716795886,3.10549653063858,0.995802211064652));
#99519=CARTESIAN_POINT('Ctrl Pts',(7.3502077780297,3.11188594216789,0.990056936559549));
#99520=CARTESIAN_POINT('Ctrl Pts',(7.2676863353547,3.12496645651863,0.978536450388539));
#99521=CARTESIAN_POINT('Ctrl Pts',(7.22642991707295,3.13166458834483,0.972755048399541));
#99522=CARTESIAN_POINT('Ctrl Pts',(7.18522749108296,3.13852541819917,0.966957027865251));
#99523=CARTESIAN_POINT('Ctrl Pts',(7.0314746878512,3.00402491773125,1.76680828720298));
#99524=CARTESIAN_POINT('Ctrl Pts',(7.03475671392561,3.00629206936566,1.75353498060149));
#99525=CARTESIAN_POINT('Ctrl Pts',(7.03803874,3.008559221,1.740261674));
#99526=CARTESIAN_POINT('Ctrl Pts',(7.133221908,3.074309666,1.35531794));
#99527=CARTESIAN_POINT('Ctrl Pts',(7.185854086,3.139297275,0.962289484));
#99528=CARTESIAN_POINT('Ctrl Pts',(7.3305839542102,3.00402491773132,1.5878289905596));
#99529=CARTESIAN_POINT('Ctrl Pts',(7.33352631350798,3.00629206936565,1.57399286353143));
#99530=CARTESIAN_POINT('Ctrl Pts',(7.33646867280563,3.008559221,1.5601567365032));
#99531=CARTESIAN_POINT('Ctrl Pts',(7.42180104768545,3.074309666,1.15889045356046));
#99532=CARTESIAN_POINT('Ctrl Pts',(7.46286100368629,3.139297275,0.750711174192357));
#99533=CARTESIAN_POINT('Origin',(-0.187878458688848,2.94646404251924,-0.0571176862107536));
#99534=CARTESIAN_POINT('Ctrl Pts',(6.807759179,3.13930489,2.493374213));
#99535=CARTESIAN_POINT('Ctrl Pts',(6.943380931,3.07388663,2.123080726));
#99536=CARTESIAN_POINT('Ctrl Pts',(7.03803874,3.008559221,1.740261674));
#99537=CARTESIAN_POINT('Ctrl Pts',(6.954130278,3.13930489,2.808927212));
#99538=CARTESIAN_POINT('Ctrl Pts',(7.10691586000001,3.07388663,2.430672182));
#99539=CARTESIAN_POINT('Ctrl Pts',(7.21777269,3.008559221,2.038076888));
#99540=CARTESIAN_POINT('',(6.80937368675612,3.13852541865695,2.48896162520118));
#99541=CARTESIAN_POINT('Origin',(-0.190175948613255,3.08928616020992,-0.0608158988611399));
#99542=CARTESIAN_POINT('Ctrl Pts',(7.0437542927345,3.09925366545663,2.57595137079219));
#99543=CARTESIAN_POINT('Ctrl Pts',(7.0046395647728,3.10549653061555,2.56147860792988));
#99544=CARTESIAN_POINT('Ctrl Pts',(6.96553102956378,3.11188594217194,2.54698735705091));
#99545=CARTESIAN_POINT('Ctrl Pts',(6.88741540061047,3.1249664658905,2.51799652197818));
#99546=CARTESIAN_POINT('Ctrl Pts',(6.84836639463171,3.13166459299201,2.50348138654226));
#99547=CARTESIAN_POINT('Ctrl Pts',(6.80937368765278,3.13852541825584,2.48896162659276));
#99548=CARTESIAN_POINT('Ctrl Pts',(6.4872711614844,3.00402491769784,3.23706050114662));
#99549=CARTESIAN_POINT('Ctrl Pts',(6.49332982424221,3.00629206934896,3.22480305557334));
#99550=CARTESIAN_POINT('Ctrl Pts',(6.499388487,3.008559221,3.21254561));
#99551=CARTESIAN_POINT('Ctrl Pts',(6.67509785,3.074309666,2.857063214));
#99552=CARTESIAN_POINT('Ctrl Pts',(6.810989017,3.139297275,2.484537907));
#99553=CARTESIAN_POINT('Ctrl Pts',(6.81786267768776,3.00402491769792,3.12656529035612));
#99554=CARTESIAN_POINT('Ctrl Pts',(6.82371060462596,3.00629206934896,3.11368516447345));
#99555=CARTESIAN_POINT('Ctrl Pts',(6.82955853156421,3.008559221,3.10080503859081));
#99556=CARTESIAN_POINT('Ctrl Pts',(6.99915627256187,3.074309666,2.72726407671965));
#99557=CARTESIAN_POINT('Ctrl Pts',(7.12700274973683,3.139297275,2.33745447873579));
#99558=CARTESIAN_POINT('Origin',(-0.171207237288136,2.94646404933259,-0.0961705711161648));
#99559=CARTESIAN_POINT('Ctrl Pts',(6.1125958,3.13930489,3.898547497));
#99560=CARTESIAN_POINT('Ctrl Pts',(6.324648946,3.07388663,3.566065933));
#99561=CARTESIAN_POINT('Ctrl Pts',(6.499388487,3.008559221,3.21254561));
#99562=CARTESIAN_POINT('Ctrl Pts',(6.18771025700001,3.13930489,4.238188502));
#99563=CARTESIAN_POINT('Ctrl Pts',(6.418237448,3.07388663,3.901621248));
#99564=CARTESIAN_POINT('Ctrl Pts',(6.61089889,3.008559221,3.542035555));
#99565=CARTESIAN_POINT('',(6.11512113789756,3.13852541863676,3.89458514483244));
#99566=CARTESIAN_POINT('Origin',(-0.172655948838892,3.08928607379705,-0.100276158918187));
#99567=CARTESIAN_POINT('Ctrl Pts',(6.32532183146937,3.09925366549066,4.02992602048575));
#99568=CARTESIAN_POINT('Ctrl Pts',(6.2902328002514,3.10549653065328,4.00738311236375));
#99569=CARTESIAN_POINT('Ctrl Pts',(6.25515379151119,3.1118859421876,3.98482347979379));
#99570=CARTESIAN_POINT('Ctrl Pts',(6.18509676441884,3.1249664417325,3.93971796624069));
#99571=CARTESIAN_POINT('Ctrl Pts',(6.15008095873197,3.13166458108201,3.91714776028921));
#99572=CARTESIAN_POINT('Ctrl Pts',(6.11512113813432,3.13852541820545,3.89458514567334));
#99573=CARTESIAN_POINT('Ctrl Pts',(5.63973004598923,3.00402491772892,4.55595136266774));
#99574=CARTESIAN_POINT('Ctrl Pts',(5.64828204899462,3.00629206936446,4.54528292283387));
#99575=CARTESIAN_POINT('Ctrl Pts',(5.656834052,3.008559221,4.534614483));
#99576=CARTESIAN_POINT('Ctrl Pts',(5.90485363500001,3.074309666,4.225215387));
#99577=CARTESIAN_POINT('Ctrl Pts',(6.117649671,3.139297275,3.890612098));
#99578=CARTESIAN_POINT('Ctrl Pts',(5.98634572077683,3.00402491772885,4.51910687246945));
#99579=CARTESIAN_POINT('Ctrl Pts',(5.99482577269543,3.00629206936446,4.5077850082868));
#99580=CARTESIAN_POINT('Ctrl Pts',(6.00330582461399,3.008559221,4.49646314410407));
#99581=CARTESIAN_POINT('Ctrl Pts',(6.24923872937746,3.074309666,4.16811386363588));
#99582=CARTESIAN_POINT('Ctrl Pts',(6.45789376755824,3.139297275,3.81490101079385));
#99583=CARTESIAN_POINT('Origin',(-0.146530587758711,2.94646404338753,-0.13072658550779));
#99584=CARTESIAN_POINT('Ctrl Pts',(5.131614236,3.13930489,5.121429033));
#99585=CARTESIAN_POINT('Ctrl Pts',(5.410183404,3.07388663,4.842305862));
#99586=CARTESIAN_POINT('Ctrl Pts',(5.65683405200001,3.008559221,4.534614483));
#99587=CARTESIAN_POINT('Ctrl Pts',(5.131959782,3.13930489,5.469276808));
#99588=CARTESIAN_POINT('Ctrl Pts',(5.429449386,3.07388663,5.190134841));
#99589=CARTESIAN_POINT('Ctrl Pts',(5.694906805,3.008559221,4.880372576));
#99590=CARTESIAN_POINT('',(5.13493232112406,3.13852541864172,5.11810219084313));
#99591=CARTESIAN_POINT('Origin',(-0.147063037517937,3.08928614843898,-0.135047780559689));
#99592=CARTESIAN_POINT('Ctrl Pts',(5.31112435157406,3.09925366548821,5.29546580809369));
#99593=CARTESIAN_POINT('Ctrl Pts',(5.28170174133006,3.105496530638,5.26590683617213));
#99594=CARTESIAN_POINT('Ctrl Pts',(5.25229251438716,3.11188594219092,5.23633368521849));
#99595=CARTESIAN_POINT('Ctrl Pts',(5.19356970549456,3.12496644806188,5.17722249498176));
#99596=CARTESIAN_POINT('Ctrl Pts',(5.16422449209147,3.13166458422919,5.14765261981693));
#99597=CARTESIAN_POINT('Ctrl Pts',(5.13493232125686,3.13852541826792,5.11810219192745));
#99598=CARTESIAN_POINT('Ctrl Pts',(4.52848142132521,3.00402491763025,5.66181100194064));
#99599=CARTESIAN_POINT('Ctrl Pts',(4.53912688266261,3.00629206931516,5.65323041197036));
#99600=CARTESIAN_POINT('Ctrl Pts',(4.549772344,3.008559221,5.644649822));
#99601=CARTESIAN_POINT('Ctrl Pts',(4.85850502600001,3.074309666,5.395801184));
#99602=CARTESIAN_POINT('Ctrl Pts',(5.138255826,3.139297275,5.114765592));
#99603=CARTESIAN_POINT('Ctrl Pts',(4.87491389009784,3.00402491763025,5.70034004019262));
#99604=CARTESIAN_POINT('Ctrl Pts',(4.88562954947645,3.00629206931516,5.69110583519945));
#99605=CARTESIAN_POINT('Ctrl Pts',(4.89634520885503,3.008559221,5.68187163020624));
#99606=CARTESIAN_POINT('Ctrl Pts',(5.20711372836752,3.074309666,5.41406727834801));
#99607=CARTESIAN_POINT('Ctrl Pts',(5.48682085039762,3.139297275,5.11396701104593));
#99608=CARTESIAN_POINT('Origin',(-0.11500256774619,2.94646401003658,-0.159170189428783));
#99609=CARTESIAN_POINT('Ctrl Pts',(3.910684093,3.13930489,6.104838239));
#99610=CARTESIAN_POINT('Ctrl Pts',(4.2427437,3.07388663,5.89212495));
#99611=CARTESIAN_POINT('Ctrl Pts',(4.549772344,3.008559221,5.644649822));
#99612=CARTESIAN_POINT('Ctrl Pts',(3.836244571,3.13930489,6.444627809));
#99613=CARTESIAN_POINT('Ctrl Pts',(4.186786305,3.07388663,6.235963497));
#99614=CARTESIAN_POINT('Ctrl Pts',(4.512627207,3.008559221,5.9905088));
#99615=CARTESIAN_POINT('',(3.91463977674163,3.1385254186077,6.10230246674704));
#99616=CARTESIAN_POINT('Origin',(-0.11459335387161,3.08928615979693,-0.163504429968793));
#99617=CARTESIAN_POINT('Ctrl Pts',(4.04858459986334,3.09925366545567,6.31339549972613));
#99618=CARTESIAN_POINT('Ctrl Pts',(4.02620398819062,3.10549658386035,6.27820230864598));
#99619=CARTESIAN_POINT('Ctrl Pts',(4.00383978723332,3.11188596840282,6.24299860631463));
#99620=CARTESIAN_POINT('Ctrl Pts',(3.95919710098266,3.12496645742458,6.17264582573996));
#99621=CARTESIAN_POINT('Ctrl Pts',(3.93689462839475,3.13166458883223,6.13745895129201));
#99622=CARTESIAN_POINT('Ctrl Pts',(3.91463977556472,3.1385254182671,6.10230246879974));
#99623=CARTESIAN_POINT('Ctrl Pts',(3.20548603911016,3.00402491768037,6.50293065189639));
#99624=CARTESIAN_POINT('Ctrl Pts',(3.21772718855505,3.00629206934018,6.49683913094818));
#99625=CARTESIAN_POINT('Ctrl Pts',(3.229968338,3.008559221,6.49074761));
#99626=CARTESIAN_POINT('Ctrl Pts',(3.584978123,3.074309666,6.31408531600001));
#99627=CARTESIAN_POINT('Ctrl Pts',(3.918602849,3.139297275,6.099758332));
#99628=CARTESIAN_POINT('Ctrl Pts',(3.53553650510488,3.00402491768037,6.61503164296334));
#99629=CARTESIAN_POINT('Ctrl Pts',(3.54798671931566,3.00629206934018,6.60831687860393));
#99630=CARTESIAN_POINT('Ctrl Pts',(3.56043693352648,3.008559221,6.60160211424467));
#99631=CARTESIAN_POINT('Ctrl Pts',(3.92150987770271,3.074309666,6.40686492373528));
#99632=CARTESIAN_POINT('Ctrl Pts',(4.25919028778872,3.139297275,6.17390959721214));
#99633=CARTESIAN_POINT('Origin',(-0.0780968644948271,2.94646402648455,-0.180170798700373));
#99634=CARTESIAN_POINT('Ctrl Pts',(2.506894708,3.13930489,6.802791995));
#99635=CARTESIAN_POINT('Ctrl Pts',(2.876918016,3.07388663,6.666434823));
#99636=CARTESIAN_POINT('Ctrl Pts',(3.229968338,3.008559221,6.49074761));
#99637=CARTESIAN_POINT('Ctrl Pts',(2.361150828,3.13930489,7.118635176));
#99638=CARTESIAN_POINT('Ctrl Pts',(2.748353749,3.07388663,6.990205431));
#99639=CARTESIAN_POINT('Ctrl Pts',(3.119342177,3.008559221,6.820535491));
#99640=CARTESIAN_POINT('',(2.51130302525059,3.13852541863486,6.8011658629826));
#99641=CARTESIAN_POINT('Origin',(-0.0767657578311959,3.0892861107107,-0.184316315789026));
#99642=CARTESIAN_POINT('Ctrl Pts',(2.59673753170469,3.09925366545958,7.03611783518109));
#99643=CARTESIAN_POINT('Ctrl Pts',(2.58244578398988,3.10549653063277,6.99693660543637));
#99644=CARTESIAN_POINT('Ctrl Pts',(2.56817213627037,3.11188594218907,6.95774812676784));
#99645=CARTESIAN_POINT('Ctrl Pts',(2.53969691770555,3.12496644121774,6.87944323712604));
#99646=CARTESIAN_POINT('Ctrl Pts',(2.52547998361091,3.13166458086886,6.84028458819026));
#99647=CARTESIAN_POINT('Ctrl Pts',(2.51130302490646,3.13852541827308,6.80116586366728));
#99648=CARTESIAN_POINT('Ctrl Pts',(1.73260569247021,3.00402491780393,7.0399804913979));
#99649=CARTESIAN_POINT('Ctrl Pts',(1.74587014723511,3.00629206940196,7.03666287219902));
#99650=CARTESIAN_POINT('Ctrl Pts',(1.759134602,3.008559221,7.033345253));
#99651=CARTESIAN_POINT('Ctrl Pts',(2.143821627,3.074309666,6.93712983500001));
#99652=CARTESIAN_POINT('Ctrl Pts',(2.515720358,3.139297275,6.79953315100001));
#99653=CARTESIAN_POINT('Ctrl Pts',(2.03084136254015,3.00402491780392,7.22041171771373));
#99654=CARTESIAN_POINT('Ctrl Pts',(2.04444397313732,3.00629206940197,7.21653036895605));
#99655=CARTESIAN_POINT('Ctrl Pts',(2.05804658373455,3.008559221,7.21264902019841));
#99656=CARTESIAN_POINT('Ctrl Pts',(2.4525405825932,3.074309666,7.1000846869461));
#99657=CARTESIAN_POINT('Ctrl Pts',(2.83240472211033,3.139297275,6.94516703341138));
#99658=CARTESIAN_POINT('Origin',(-0.0375396041755813,2.94646404903966,-0.192746987544548));
#99659=CARTESIAN_POINT('Ctrl Pts',(0.985885713,3.13930489,7.182654757));
#99660=CARTESIAN_POINT('Ctrl Pts',(1.376570843,3.07388663,7.129029614));
#99661=CARTESIAN_POINT('Ctrl Pts',(1.759134602,3.008559221,7.033345253));
#99662=CARTESIAN_POINT('Ctrl Pts',(0.775652296,3.13930489,7.459783074));
#99663=CARTESIAN_POINT('Ctrl Pts',(1.181411227,3.07388663,7.417593128));
#99664=CARTESIAN_POINT('Ctrl Pts',(1.580200173,3.008559221,7.331641522));
#99665=CARTESIAN_POINT('',(0.990540537957797,3.13852541858696,7.18201430105442));
#99666=CARTESIAN_POINT('Origin',(-0.0353484116042134,3.08928611100659,-0.196509256625923));
#99667=CARTESIAN_POINT('Ctrl Pts',(1.02346990277173,3.09925366544172,7.42983912041204));
#99668=CARTESIAN_POINT('Ctrl Pts',(1.01793509438376,3.10549653059944,7.38850162286539));
#99669=CARTESIAN_POINT('Ctrl Pts',(1.01241952112971,3.11188594212621,7.34716093692004));
#99670=CARTESIAN_POINT('Ctrl Pts',(1.00144325721373,3.12496646100666,7.26456531650114));
#99671=CARTESIAN_POINT('Ctrl Pts',(0.995976668043184,3.13166459052523,7.22326602139092));
#99672=CARTESIAN_POINT('Ctrl Pts',(0.99054053586425,3.13852541814021,7.18201430276513));
#99673=CARTESIAN_POINT('Ctrl Pts',(0.178710629076645,3.00402491789854,7.24784866891218));
#99674=CARTESIAN_POINT('Ctrl Pts',(0.192378158038323,3.0062920694493,7.24746007945602));
#99675=CARTESIAN_POINT('Ctrl Pts',(0.206045687,3.008559221,7.24707149000001));
#99676=CARTESIAN_POINT('Ctrl Pts',(0.602422414,3.074309666,7.235801873));
#99677=CARTESIAN_POINT('Ctrl Pts',(0.99520558,3.139297275,7.181369358));
#99678=CARTESIAN_POINT('Ctrl Pts',(0.431186334731839,3.00402491789854,7.48817336586714));
#99679=CARTESIAN_POINT('Ctrl Pts',(0.445305298819396,3.0062920694493,7.48730692008476));
#99680=CARTESIAN_POINT('Ctrl Pts',(0.45942426290696,3.008559221,7.48644047430236));
#99681=CARTESIAN_POINT('Ctrl Pts',(0.868893215879408,3.074309666,7.461312380972));
#99682=CARTESIAN_POINT('Ctrl Pts',(1.27317905962692,3.139297275,7.3916761777119));
#99683=CARTESIAN_POINT('Origin',(0.00477268321224331,2.94646447851623,-0.196313054001395));
#99684=CARTESIAN_POINT('Ctrl Pts',(-0.581222202,3.13930489,7.226664566));
#99685=CARTESIAN_POINT('Ctrl Pts',(-0.188143253,3.07388663,7.258278904));
#99686=CARTESIAN_POINT('Ctrl Pts',(0.206045687,3.008559221,7.24707149000001));
#99687=CARTESIAN_POINT('Ctrl Pts',(-0.846114875,3.13930489,7.452119807));
#99688=CARTESIAN_POINT('Ctrl Pts',(-0.440772771,3.07388663,7.498142414));
#99689=CARTESIAN_POINT('Ctrl Pts',(-0.032830234,3.008559221,7.499928145));
#99690=CARTESIAN_POINT('Origin',(0.0077217778851673,3.08928625812933,-0.199516394736223));
#99691=CARTESIAN_POINT('Ctrl Pts',(0.214081497,2.75,7.24683856));
#99692=CARTESIAN_POINT('Ctrl Pts',(0.606773411,2.81435393,7.235237905));
#99693=CARTESIAN_POINT('Ctrl Pts',(0.995912368,2.879481221,7.181271375));
#99694=CARTESIAN_POINT('Ctrl Pts',(0.467202875,2.75,7.485433954));
#99695=CARTESIAN_POINT('Ctrl Pts',(0.872823804,2.81435393,7.46011715000001));
#99696=CARTESIAN_POINT('Ctrl Pts',(1.27333392,2.879481221,7.391117691));
#99697=CARTESIAN_POINT('',(0.467202886311634,2.75,7.48543395315807));
#99698=CARTESIAN_POINT('',(1.02739270828442,2.83963938427222,7.42929769337341));
#99699=CARTESIAN_POINT('Origin',(-0.0426544601547765,2.94636923496794,-0.183656325683895));
#99700=CARTESIAN_POINT('Ctrl Pts',(0.991263375807224,2.87870320272917,7.181914572441));
#99701=CARTESIAN_POINT('Ctrl Pts',(0.997239354637858,2.87185457193071,7.22308853581347));
#99702=CARTESIAN_POINT('Ctrl Pts',(1.00324258046769,2.86518067056541,7.26431437598536));
#99703=CARTESIAN_POINT('Ctrl Pts',(1.01528456492317,2.8521708113185,7.34676107373081));
#99704=CARTESIAN_POINT('Ctrl Pts',(1.02133053850809,2.84582706798436,7.38803131637516));
#99705=CARTESIAN_POINT('Ctrl Pts',(1.02739270989943,2.8396393842762,7.42929769313675));
#99706=CARTESIAN_POINT('',(0.340642197483777,2.74999999814853,7.36613625646894));
#99707=CARTESIAN_POINT('Origin',(1.68756068147369E-13,2.84071505699956,
1.43158054854986E-12));
#99708=CARTESIAN_POINT('',(1.02739270828441,2.66036061572777,7.42929769337331));
#99709=CARTESIAN_POINT('Origin',(-0.0426544601514964,2.55363076502388,-0.183656325612771));
#99710=CARTESIAN_POINT('',(1.58832892548214,2.75,7.32988480226283));
#99711=CARTESIAN_POINT('Ctrl Pts',(1.58832892514213,2.75000000173941,7.32988480199432));
#99712=CARTESIAN_POINT('Ctrl Pts',(1.44013430592371,2.72598918212329,7.36199742168401));
#99713=CARTESIAN_POINT('Ctrl Pts',(1.29133537739194,2.70215892392441,7.3895315483916));
#99714=CARTESIAN_POINT('Ctrl Pts',(1.14235084253717,2.6785714288812,7.41249179069507));
#99715=CARTESIAN_POINT('Ctrl Pts',(1.1041082303364,2.67251679083289,7.41838542008151));
#99716=CARTESIAN_POINT('Ctrl Pts',(1.06578665338603,2.66644617724574,7.42398821998536));
#99717=CARTESIAN_POINT('Ctrl Pts',(1.02739270835229,2.66036061551156,7.42929769361639));
#99718=CARTESIAN_POINT('Ctrl Pts',(1.0273927083523,2.83963938448845,7.42929769361639));
#99719=CARTESIAN_POINT('Ctrl Pts',(1.06578665338584,2.83355382275425,7.42398821998572));
#99720=CARTESIAN_POINT('Ctrl Pts',(1.10410823026581,2.82748320916963,7.41838542016399));
#99721=CARTESIAN_POINT('Ctrl Pts',(1.14235084253684,2.8214285711188,7.41249179069551));
#99722=CARTESIAN_POINT('Ctrl Pts',(1.2913353776657,2.79784107606577,7.38953154807236));
#99723=CARTESIAN_POINT('Ctrl Pts',(1.44013430592352,2.77401081787668,7.36199742168431));
#99724=CARTESIAN_POINT('Ctrl Pts',(1.58832892514213,2.74999999826059,7.32988480199431));
#99725=CARTESIAN_POINT('Ctrl Pts',(0.986554849,2.879480225,7.18256288));
#99726=CARTESIAN_POINT('Ctrl Pts',(1.163317088,2.85030975,7.158283853));
#99727=CARTESIAN_POINT('Ctrl Pts',(1.338671059,2.821428571,7.125339276));
#99728=CARTESIAN_POINT('Ctrl Pts',(1.554222808,2.785926731,7.08484255300001));
#99729=CARTESIAN_POINT('Ctrl Pts',(1.766932466,2.75,7.031390308));
#99730=CARTESIAN_POINT('Ctrl Pts',(1.77080069057172,2.74934665560115,7.03041825393595));
#99731=CARTESIAN_POINT('Ctrl Pts',(1.77466891514343,2.7486933112023,7.02944619987189));
#99732=CARTESIAN_POINT('Ctrl Pts',(0.77634725,2.879480225,7.459710782));
#99733=CARTESIAN_POINT('Ctrl Pts',(0.959930074,2.85030975,7.440604944));
#99734=CARTESIAN_POINT('Ctrl Pts',(1.142350843,2.821428571,7.412491791));
#99735=CARTESIAN_POINT('Ctrl Pts',(1.366589369,2.785926731,7.377934037));
#99736=CARTESIAN_POINT('Ctrl Pts',(1.588328914,2.75,7.329884805));
#99737=CARTESIAN_POINT('Ctrl Pts',(1.59236135128825,2.74934665560115,7.32901100725324));
#99738=CARTESIAN_POINT('Ctrl Pts',(1.5963937885765,2.7486933112023,7.32813720950648));
#99739=CARTESIAN_POINT('',(1.67763070119454,2.75000000185147,7.18063755388459));
#99740=CARTESIAN_POINT('Ctrl Pts',(1.766932466,2.75,7.031390308));
#99741=CARTESIAN_POINT('Ctrl Pts',(2.147949663,2.81435393,6.935643716));
#99742=CARTESIAN_POINT('Ctrl Pts',(2.516389559,2.879481221,6.79928552));
#99743=CARTESIAN_POINT('Ctrl Pts',(2.065426964,2.75,7.20999386));
#99744=CARTESIAN_POINT('Ctrl Pts',(2.456122336,2.81435393,7.098072439));
#99745=CARTESIAN_POINT('Ctrl Pts',(2.832435904,2.879481221,6.944588314));
#99746=CARTESIAN_POINT('',(2.06542697487382,2.75,7.20999385677276));
#99747=CARTESIAN_POINT('',(2.60045223338147,2.83963938432456,7.03474577907832));
#99748=CARTESIAN_POINT('Origin',(-0.0811379622534811,2.94636923733788,-0.170193277971202));
#99749=CARTESIAN_POINT('Ctrl Pts',(2.51198752654408,2.87870320280854,6.80091307558165));
#99750=CARTESIAN_POINT('Ctrl Pts',(2.52667497498449,2.87185457194135,6.8398397562541));
#99751=CARTESIAN_POINT('Ctrl Pts',(2.54140018575414,2.86518067050631,6.8788112436685));
#99752=CARTESIAN_POINT('Ctrl Pts',(2.57088423815875,2.85217081128638,6.95674171291582));
#99753=CARTESIAN_POINT('Ctrl Pts',(2.58566074252707,2.84582706798929,6.99574737455167));
#99754=CARTESIAN_POINT('Ctrl Pts',(2.60045223490396,2.83963938432854,7.03474577850149));
#99755=CARTESIAN_POINT('',(1.91617972610113,2.74999999814853,7.12069208101268));
#99756=CARTESIAN_POINT('Origin',(3.25043811311154E-13,2.84071505699967,
9.72312508285E-13));
#99757=CARTESIAN_POINT('',(2.60045223338141,2.66036061567541,7.03474577907809));
#99758=CARTESIAN_POINT('Origin',(-0.081137962209949,2.55363076264363,-0.170193277808389));
#99759=CARTESIAN_POINT('',(3.12690324058091,2.75,6.81707240076085));
#99760=CARTESIAN_POINT('Ctrl Pts',(3.12690324023566,2.7500000017394,6.81707240066876));
#99761=CARTESIAN_POINT('Ctrl Pts',(2.98907659225498,2.72598918212324,6.88029170751296));
#99762=CARTESIAN_POINT('Ctrl Pts',(2.84967552346095,2.70215892392428,6.93916947253795));
#99763=CARTESIAN_POINT('Ctrl Pts',(2.7091099382986,2.67857142886255,6.99362018802513));
#99764=CARTESIAN_POINT('Ctrl Pts',(2.67302837304287,2.67251679079023,7.00759705909646));
#99765=CARTESIAN_POINT('Ctrl Pts',(2.63680716970682,2.66644617720861,7.02130687482412));
#99766=CARTESIAN_POINT('Ctrl Pts',(2.60045223349521,2.66036061545778,7.03474577928741));
#99767=CARTESIAN_POINT('Ctrl Pts',(2.6004522334952,2.83963938454222,7.03474577928741));
#99768=CARTESIAN_POINT('Ctrl Pts',(2.63680716970653,2.83355382279137,7.02130687482507));
#99769=CARTESIAN_POINT('Ctrl Pts',(2.67302837322312,2.82748320918882,7.00759705891095));
#99770=CARTESIAN_POINT('Ctrl Pts',(2.70910993830944,2.82142857113746,6.99362018799814));
#99771=CARTESIAN_POINT('Ctrl Pts',(2.84967552281257,2.79784107615723,6.93916947312821));
#99772=CARTESIAN_POINT('Ctrl Pts',(2.9890765922547,2.77401081787686,6.88029170751378));
#99773=CARTESIAN_POINT('Ctrl Pts',(3.12690324023566,2.7499999982606,6.81707240066876));
#99774=CARTESIAN_POINT('Ctrl Pts',(2.507528449,2.879480225,6.802558422));
#99775=CARTESIAN_POINT('Ctrl Pts',(2.674938811,2.85030975,6.740848368));
#99776=CARTESIAN_POINT('Ctrl Pts',(2.839110994,2.821428571,6.670978097));
#99777=CARTESIAN_POINT('Ctrl Pts',(3.040917665,2.785926731,6.58509091));
#99778=CARTESIAN_POINT('Ctrl Pts',(3.237163637,2.75,6.48716206));
#99779=CARTESIAN_POINT('Ctrl Pts',(3.24073246174509,2.74934665560115,6.48538117808137));
#99780=CARTESIAN_POINT('Ctrl Pts',(3.24430128649018,2.7486933112023,6.48360029616274));
#99781=CARTESIAN_POINT('Ctrl Pts',(2.361813993,2.879480225,7.118415179));
#99782=CARTESIAN_POINT('Ctrl Pts',(2.536997563,2.85030975,7.060291145));
#99783=CARTESIAN_POINT('Ctrl Pts',(2.709109939,2.821428571,6.993620188));
#99784=CARTESIAN_POINT('Ctrl Pts',(2.920676996,2.785926731,6.911665721));
#99785=CARTESIAN_POINT('Ctrl Pts',(3.12690323,2.75,6.817072406));
#99786=CARTESIAN_POINT('Ctrl Pts',(3.1306535504753,2.74934665560115,6.8153521823447));
#99787=CARTESIAN_POINT('Ctrl Pts',(3.13440387095059,2.7486933112023,6.8136319586894));
#99788=CARTESIAN_POINT('',(3.18203344387054,2.75000000185146,6.65211722803926));
#99789=CARTESIAN_POINT('Ctrl Pts',(3.237163637,2.75,6.48716206));
#99790=CARTESIAN_POINT('Ctrl Pts',(3.588690177,2.81435393,6.311746536));
#99791=CARTESIAN_POINT('Ctrl Pts',(3.919203171,2.879481221,6.099372632));
#99792=CARTESIAN_POINT('Ctrl Pts',(3.567073983,2.75,6.597422466));
#99793=CARTESIAN_POINT('Ctrl Pts',(3.924575317,2.81435393,6.40412975));
#99794=CARTESIAN_POINT('Ctrl Pts',(4.259096333,2.879481221,6.173337705));
#99795=CARTESIAN_POINT('',(3.56707399302919,2.75,6.59742246070181));
#99796=CARTESIAN_POINT('',(4.05191750198777,2.83963938428845,6.31125697077989));
#99797=CARTESIAN_POINT('Origin',(-0.115827529813538,2.94636920761577,-0.148772020898219));
#99798=CARTESIAN_POINT('Ctrl Pts',(3.9152539318276,2.87870320278185,6.10190844318095));
#99799=CARTESIAN_POINT('Ctrl Pts',(3.93796608157822,2.87185457197069,6.1367676721412));
#99800=CARTESIAN_POINT('Ctrl Pts',(3.96072474276779,2.86518067058185,6.17166254250291));
#99801=CARTESIAN_POINT('Ctrl Pts',(4.00627222155147,2.85217081136344,6.24143284080794));
#99802=CARTESIAN_POINT('Ctrl Pts',(4.02908832386645,2.84582706798215,6.27635006047718));
#99803=CARTESIAN_POINT('Ctrl Pts',(4.05191750339012,2.83963938429247,6.31125696986346));
#99804=CARTESIAN_POINT('',(3.40211882019941,2.74999999814853,6.54229225769611));
#99805=CARTESIAN_POINT('Origin',(1.66750294128271E-13,2.84071505700011,
1.39645239816133E-13));
#99806=CARTESIAN_POINT('',(4.05191750198764,2.66036061571151,6.31125697077964));
#99807=CARTESIAN_POINT('Origin',(-0.115827529770104,2.55363079237376,-0.14877202081415));
#99808=CARTESIAN_POINT('',(4.51926703516983,2.75,5.98550127055907));
#99809=CARTESIAN_POINT('Ctrl Pts',(4.51926703485033,2.75000000173941,5.98550127059301));
#99810=CARTESIAN_POINT('Ctrl Pts',(4.39825297998733,2.72598918212333,6.07687120025204));
#99811=CARTESIAN_POINT('Ctrl Pts',(4.27476800964676,2.70215892392453,6.16433954508843));
#99812=CARTESIAN_POINT('Ctrl Pts',(4.14919406351116,2.67857142889851,6.24773467905231));
#99813=CARTESIAN_POINT('Ctrl Pts',(4.11696067960482,2.67251679086577,6.26914124840894));
#99814=CARTESIAN_POINT('Ctrl Pts',(4.08453351292944,2.66644617725385,6.29031702417241));
#99815=CARTESIAN_POINT('Ctrl Pts',(4.05191750219905,2.66036061550164,6.31125697104795));
#99816=CARTESIAN_POINT('Ctrl Pts',(4.05191750219919,2.83963938449833,6.3112569710482));
#99817=CARTESIAN_POINT('Ctrl Pts',(4.08453351292954,2.83355382274611,6.29031702417293));
#99818=CARTESIAN_POINT('Ctrl Pts',(4.11696067950133,2.82748320915847,6.26914124834338));
#99819=CARTESIAN_POINT('Ctrl Pts',(4.14919406351669,2.82142857110149,6.24773467901926));
#99820=CARTESIAN_POINT('Ctrl Pts',(4.27476801007775,2.79784107598091,6.16433954518152));
#99821=CARTESIAN_POINT('Ctrl Pts',(4.39825297998724,2.77401081787664,6.07687120025258));
#99822=CARTESIAN_POINT('Ctrl Pts',(4.51926703485033,2.74999999826059,5.98550127059301));
#99823=CARTESIAN_POINT('Ctrl Pts',(3.911252806,2.879480225,6.104473891));
#99824=CARTESIAN_POINT('Ctrl Pts',(4.06148337,2.85030975,6.00821830500001));
#99825=CARTESIAN_POINT('Ctrl Pts',(4.206797255,2.821428571,5.904689396));
#99826=CARTESIAN_POINT('Ctrl Pts',(4.385422592,2.785926731,5.777427735));
#99827=CARTESIAN_POINT('Ctrl Pts',(4.556028634,2.75,5.63960132400001));
#99828=CARTESIAN_POINT('Ctrl Pts',(4.55913118463147,2.74934665560115,5.63709488628262));
#99829=CARTESIAN_POINT('Ctrl Pts',(4.56223373526293,2.7486933112023,5.63458844856525));
#99830=CARTESIAN_POINT('Ctrl Pts',(3.836844939,2.879480225,6.444270394));
#99831=CARTESIAN_POINT('Ctrl Pts',(3.995437865,2.85030975,6.349845979));
#99832=CARTESIAN_POINT('Ctrl Pts',(4.149194064,2.821428571,6.247734679));
#99833=CARTESIAN_POINT('Ctrl Pts',(4.338197014,2.785926731,6.122215598));
#99834=CARTESIAN_POINT('Ctrl Pts',(4.519267026,2.75,5.98550127800001));
#99835=CARTESIAN_POINT('Ctrl Pts',(4.52255986881779,2.74934665560115,5.98301506417736));
#99836=CARTESIAN_POINT('Ctrl Pts',(4.52585271163557,2.7486933112023,5.98052885035472));
#99837=CARTESIAN_POINT('',(4.53764783906171,2.75000000185146,5.81255129392586));
#99838=CARTESIAN_POINT('Ctrl Pts',(4.556028634,2.75,5.63960132400001));
#99839=CARTESIAN_POINT('Ctrl Pts',(4.861627526,2.81435393,5.392719102));
#99840=CARTESIAN_POINT('Ctrl Pts',(5.138759199,2.879481221,5.114259858));
#99841=CARTESIAN_POINT('Ctrl Pts',(4.901928588,2.75,5.676362931));
#99842=CARTESIAN_POINT('Ctrl Pts',(5.209519519,2.81435393,5.41073707200001));
#99843=CARTESIAN_POINT('Ctrl Pts',(5.486606152,2.879481221,5.113428687));
#99844=CARTESIAN_POINT('',(4.90192859649301,2.75,5.67636292348124));
#99845=CARTESIAN_POINT('',(5.31391961162131,2.83963938432021,5.29266080113455));
#99846=CARTESIAN_POINT('Origin',(-0.1451010862056,2.94636923250028,-0.120394251048356));
#99847=CARTESIAN_POINT('Ctrl Pts',(5.13544741478264,2.87870320266467,5.11758535350932));
#99848=CARTESIAN_POINT('Ctrl Pts',(5.16512227092593,2.87185457185746,5.14674715239094));
#99849=CARTESIAN_POINT('Ctrl Pts',(5.1948502129185,2.86518067047536,5.17593376078539));
#99850=CARTESIAN_POINT('Ctrl Pts',(5.25433136878464,2.85217081127113,5.23428150693977));
#99851=CARTESIAN_POINT('Ctrl Pts',(5.28412021299232,2.84582706799665,5.26347759348871));
#99852=CARTESIAN_POINT('Ctrl Pts',(5.31391961274871,2.83963938432419,5.29266079998418));
#99853=CARTESIAN_POINT('',(4.72897861982077,2.74999999814853,5.65798212012754));
#99854=CARTESIAN_POINT('Origin',(-4.38017677684144E-14,2.84071505699989,
6.50521303491303E-14));
#99855=CARTESIAN_POINT('',(5.31391961162116,2.66036061567976,5.29266080113437));
#99856=CARTESIAN_POINT('Origin',(-0.145101086098398,2.55363076748073,-0.120394250919469));
#99857=CARTESIAN_POINT('',(5.70031492639775,2.75,4.87405475279786));
#99858=CARTESIAN_POINT('Ctrl Pts',(5.70031492605116,2.75000000173941,4.8740547528639));
#99859=CARTESIAN_POINT('Ctrl Pts',(5.60177194666881,2.72598918212334,4.98930294874716));
#99860=CARTESIAN_POINT('Ctrl Pts',(5.49997709495883,2.70215892392439,5.10127195060386));
#99861=CARTESIAN_POINT('Ctrl Pts',(5.39526648644324,2.67857142887792,5.20971203926714));
#99862=CARTESIAN_POINT('Ctrl Pts',(5.36838848047096,2.67251679080437,5.23754735998662));
#99863=CARTESIAN_POINT('Ctrl Pts',(5.34127160873142,2.66644617720303,5.2651989404272));
#99864=CARTESIAN_POINT('Ctrl Pts',(5.31391961177441,2.66036061545698,5.29266080123764));
#99865=CARTESIAN_POINT('Ctrl Pts',(5.3139196117744,2.83963938454303,5.29266080123765));
#99866=CARTESIAN_POINT('Ctrl Pts',(5.34127160873155,2.83355382279695,5.26519894042819));
#99867=CARTESIAN_POINT('Ctrl Pts',(5.36838848046974,2.827483209194,5.23754735980595));
#99868=CARTESIAN_POINT('Ctrl Pts',(5.3952664864407,2.82142857112209,5.20971203921784));
#99869=CARTESIAN_POINT('Ctrl Pts',(5.49997709495177,2.79784107608189,5.10127195106572));
#99870=CARTESIAN_POINT('Ctrl Pts',(5.60177194666888,2.77401081787662,4.98930294874803));
#99871=CARTESIAN_POINT('Ctrl Pts',(5.70031492605117,2.74999999826059,4.87405475286389));
#99872=CARTESIAN_POINT('Ctrl Pts',(5.132091328,2.879480225,5.120950947));
#99873=CARTESIAN_POINT('Ctrl Pts',(5.258117479,2.85030975,4.994650632));
#99874=CARTESIAN_POINT('Ctrl Pts',(5.377778351,2.821428571,4.862303981));
#99875=CARTESIAN_POINT('Ctrl Pts',(5.524870032,2.785926731,4.69961846));
#99876=CARTESIAN_POINT('Ctrl Pts',(5.661858795,2.75,4.528339098));
#99877=CARTESIAN_POINT('Ctrl Pts',(5.6643499996969,2.74934665560115,4.52522430272956));
#99878=CARTESIAN_POINT('Ctrl Pts',(5.6668412043938,2.7486933112023,4.52210950745911));
#99879=CARTESIAN_POINT('Ctrl Pts',(5.13246928,2.879480225,5.468798688));
#99880=CARTESIAN_POINT('Ctrl Pts',(5.267055933,2.85030975,5.342489072));
#99881=CARTESIAN_POINT('Ctrl Pts',(5.395266487,2.821428571,5.209712039));
#99882=CARTESIAN_POINT('Ctrl Pts',(5.552867761,2.785926731,5.046497477));
#99883=CARTESIAN_POINT('Ctrl Pts',(5.700314919,2.75,4.874054762));
#99884=CARTESIAN_POINT('Ctrl Pts',(5.70299631449924,2.74934665560115,4.87091881061139));
#99885=CARTESIAN_POINT('Ctrl Pts',(5.70567770999847,2.7486933112023,4.86778285922278));
#99886=CARTESIAN_POINT('',(5.68108686432912,2.75000000185146,4.70119692114325));
#99887=CARTESIAN_POINT('Ctrl Pts',(5.661858795,2.75,4.528339098));
#99888=CARTESIAN_POINT('Ctrl Pts',(5.907240575,2.81435393,4.221534117));
#99889=CARTESIAN_POINT('Ctrl Pts',(6.118032557,2.879481221,3.890009978));
#99890=CARTESIAN_POINT('Ctrl Pts',(6.007574459,2.75,4.489882974));
#99891=CARTESIAN_POINT('Ctrl Pts',(6.250872378,2.81435393,4.164344342));
#99892=CARTESIAN_POINT('Ctrl Pts',(6.457568365,2.879481221,3.814421426));
#99893=CARTESIAN_POINT('',(6.0075744657785,2.75,4.48988296490629));
#99894=CARTESIAN_POINT('',(6.32744874633466,2.83963938435354,4.0265856945531));
#99895=CARTESIAN_POINT('Origin',(-0.167589759079224,2.9463692414211,-0.0863869564722602));
#99896=CARTESIAN_POINT('Ctrl Pts',(6.11551308399302,2.87870320275711,3.89396966050874));
#99897=CARTESIAN_POINT('Ctrl Pts',(6.15076308335111,2.87185457194778,3.91607045570484));
#99898=CARTESIAN_POINT('Ctrl Pts',(6.1860702606457,2.86518067056699,3.93818406853816));
#99899=CARTESIAN_POINT('Ctrl Pts',(6.256703820957,2.85217081132701,3.98238098655727));
#99900=CARTESIAN_POINT('Ctrl Pts',(6.29207251402559,2.84582706805614,4.00449076384202));
#99901=CARTESIAN_POINT('Ctrl Pts',(6.32744874717936,2.83963938435753,4.02658569320178));
#99902=CARTESIAN_POINT('',(5.83471663402968,2.74999999814853,4.5091110269037));
#99903=CARTESIAN_POINT('Origin',(1.65752828129584E-12,2.84071505699922,
1.06338549077378E-12));
#99904=CARTESIAN_POINT('',(6.32744874633445,2.66036061564643,4.02658569455294));
#99905=CARTESIAN_POINT('Origin',(-0.167589758930268,2.55363075855824,-0.0863869563564529));
#99906=CARTESIAN_POINT('',(6.61482242727647,2.75,3.53470285143859));
#99907=CARTESIAN_POINT('Ctrl Pts',(6.61482242692228,2.75000000173941,3.53470285156161));
#99908=CARTESIAN_POINT('Ctrl Pts',(6.54335828239023,2.72598918212333,3.6684404372531));
#99909=CARTESIAN_POINT('Ctrl Pts',(6.46801336322534,2.70215892392438,3.79967455044767));
#99910=CARTESIAN_POINT('Ctrl Pts',(6.38906224448245,2.67857142887702,3.9280890552822));
#99911=CARTESIAN_POINT('Ctrl Pts',(6.36879640248986,2.67251679078551,3.96105157831173));
#99912=CARTESIAN_POINT('Ctrl Pts',(6.34825778061731,2.66644617717233,3.99388600610648));
#99913=CARTESIAN_POINT('Ctrl Pts',(6.32744874646083,2.66036061541843,4.02658569459093));
#99914=CARTESIAN_POINT('Ctrl Pts',(6.32744874646082,2.83963938458158,4.02658569459094));
#99915=CARTESIAN_POINT('Ctrl Pts',(6.34825778061771,2.83355382282764,3.99388600610754));
#99916=CARTESIAN_POINT('Ctrl Pts',(6.36879640248882,2.82748320921173,3.96105157825919));
#99917=CARTESIAN_POINT('Ctrl Pts',(6.38906224448281,2.82142857112299,3.92808905528369));
#99918=CARTESIAN_POINT('Ctrl Pts',(6.46801336323162,2.79784107608627,3.79967455065886));
#99919=CARTESIAN_POINT('Ctrl Pts',(6.54335828239052,2.77401081787664,3.66844043725405));
#99920=CARTESIAN_POINT('Ctrl Pts',(6.61482242692228,2.74999999826059,3.53470285156161));
#99921=CARTESIAN_POINT('Ctrl Pts',(6.112958964,2.879480225,3.897978027));
#99922=CARTESIAN_POINT('Ctrl Pts',(6.20888786,2.85030975,3.747538647));
#99923=CARTESIAN_POINT('Ctrl Pts',(6.297300509,2.821428571,3.592562637));
#99924=CARTESIAN_POINT('Ctrl Pts',(6.40598069,2.785926731,3.402060249));
#99925=CARTESIAN_POINT('Ctrl Pts',(6.502946732,2.75,3.205336768));
#99926=CARTESIAN_POINT('Ctrl Pts',(6.50471010480504,2.74934665560115,3.20175925953051));
#99927=CARTESIAN_POINT('Ctrl Pts',(6.50647347761008,2.7486933112023,3.19818175106102));
#99928=CARTESIAN_POINT('Ctrl Pts',(6.188105062,2.879480225,4.237612033));
#99929=CARTESIAN_POINT('Ctrl Pts',(6.29239232,2.85030975,4.085323313));
#99930=CARTESIAN_POINT('Ctrl Pts',(6.389062245,2.821428571,3.928089055));
#99931=CARTESIAN_POINT('Ctrl Pts',(6.50789258200001,2.785926731,3.734810744));
#99932=CARTESIAN_POINT('Ctrl Pts',(6.614822422,2.75,3.534702862));
#99933=CARTESIAN_POINT('Ctrl Pts',(6.61676699112971,2.74934665560115,3.53106380661613));
#99934=CARTESIAN_POINT('Ctrl Pts',(6.61871156025942,2.7486933112023,3.52742475123226));
#99935=CARTESIAN_POINT('',(6.55888458225382,2.75000000185146,3.37001980477476));
#99936=CARTESIAN_POINT('Ctrl Pts',(6.502946732,2.75,3.205336768));
#99937=CARTESIAN_POINT('Ctrl Pts',(6.676637621,2.81435393,2.852954888));
#99938=CARTESIAN_POINT('Ctrl Pts',(6.81123351300001,2.879481221,2.483867554));
#99939=CARTESIAN_POINT('Ctrl Pts',(6.832312826,2.75,3.093461079));
#99940=CARTESIAN_POINT('Ctrl Pts',(6.999941392,2.81435393,2.723231498));
#99941=CARTESIAN_POINT('Ctrl Pts',(7.126581858,2.879481221,2.337056058));
#99942=CARTESIAN_POINT('',(6.83231283068604,2.75,3.09346106867118));
#99943=CARTESIAN_POINT('',(7.04511341073837,2.8396393842543,2.57223191590152));
#99944=CARTESIAN_POINT('Origin',(-0.182242366147894,2.94636923907614,-0.0483404868385445));
#99945=CARTESIAN_POINT('Ctrl Pts',(6.80962415850719,2.87870320272689,2.48827627372443));
#99946=CARTESIAN_POINT('Ctrl Pts',(6.84880105018254,2.87185457190863,2.50228265672233));
#99947=CARTESIAN_POINT('Ctrl Pts',(6.88803653853397,2.86518067051122,2.51628926610237));
#99948=CARTESIAN_POINT('Ctrl Pts',(6.96651975635637,2.85217081129629,2.54426875701519));
#99949=CARTESIAN_POINT('Ctrl Pts',(7.0058144982252,2.84582706793473,2.55825839662235));
#99950=CARTESIAN_POINT('Ctrl Pts',(7.04511341129873,2.8396393842583,2.57223191432735));
#99951=CARTESIAN_POINT('',(6.6676297839099,2.74999999814853,3.14939891310519));
#99952=CARTESIAN_POINT('Origin',(-2.03613167992778E-12,2.84071505700056,
-7.66314095512755E-13));
#99953=CARTESIAN_POINT('',(7.04511341073833,2.66036061574569,2.57223191590147));
#99954=CARTESIAN_POINT('Origin',(-0.182242366131465,2.55363076092139,-0.0483404868305065));
#99955=CARTESIAN_POINT('',(7.22002818281552,2.75,2.03007217453226));
#99956=CARTESIAN_POINT('Ctrl Pts',(7.22002818256322,2.75000000173941,2.03007217474743));
#99957=CARTESIAN_POINT('Ctrl Pts',(7.17898445787291,2.72598918212316,2.17604572814847));
#99958=CARTESIAN_POINT('Ctrl Pts',(7.13361251627696,2.70215892392443,2.32040859113163));
#99959=CARTESIAN_POINT('Ctrl Pts',(7.08411255356873,2.67857142888421,2.46279299334046));
#99960=CARTESIAN_POINT('Ctrl Pts',(7.07140648396715,2.67251679085757,2.49934142753215));
#99961=CARTESIAN_POINT('Ctrl Pts',(7.05840647505362,2.66644617727519,2.53582340086089));
#99962=CARTESIAN_POINT('Ctrl Pts',(7.04511341106862,2.66036061553643,2.57223191598709));
#99963=CARTESIAN_POINT('Ctrl Pts',(7.04511341106867,2.83963938446356,2.57223191598713));
#99964=CARTESIAN_POINT('Ctrl Pts',(7.05840647505371,2.8335538227248,2.53582340086099));
#99965=CARTESIAN_POINT('Ctrl Pts',(7.07140648393755,2.82748320914873,2.499341427539));
#99966=CARTESIAN_POINT('Ctrl Pts',(7.0841125535688,2.82142857111579,2.46279299334067));
#99967=CARTESIAN_POINT('Ctrl Pts',(7.13361251639273,2.79784107605103,2.32040859110585));
#99968=CARTESIAN_POINT('Ctrl Pts',(7.17898445787293,2.77401081787663,2.1760457281486));
#99969=CARTESIAN_POINT('Ctrl Pts',(7.22002818256322,2.74999999826059,2.03007217474743));
#99970=CARTESIAN_POINT('Ctrl Pts',(6.807991433,2.879480225,2.492739988));
#99971=CARTESIAN_POINT('Ctrl Pts',(6.869337544,2.85030975,2.325195919));
#99972=CARTESIAN_POINT('Ctrl Pts',(6.922367894,2.821428571,2.154837056));
#99973=CARTESIAN_POINT('Ctrl Pts',(6.987554811,2.785926731,1.945425482));
#99974=CARTESIAN_POINT('Ctrl Pts',(7.039964107,2.75,1.732456454));
#99975=CARTESIAN_POINT('Ctrl Pts',(7.04091719454892,2.74934665560115,1.72858351266358));
#99976=CARTESIAN_POINT('Ctrl Pts',(7.04187028209783,2.7486933112023,1.72471057132716));
#99977=CARTESIAN_POINT('Ctrl Pts',(6.954391929,2.879480225,2.808279349));
#99978=CARTESIAN_POINT('Ctrl Pts',(7.023503436,2.85030975,2.637132378));
#99979=CARTESIAN_POINT('Ctrl Pts',(7.084112554,2.821428571,2.462792993));
#99980=CARTESIAN_POINT('Ctrl Pts',(7.15861558,2.785926731,2.248488411));
#99981=CARTESIAN_POINT('Ctrl Pts',(7.22002818,2.75,2.030072186));
#99982=CARTESIAN_POINT('Ctrl Pts',(7.22114499684117,2.74934665560115,2.02610018483959));
#99983=CARTESIAN_POINT('Ctrl Pts',(7.22226181368234,2.7486933112023,2.02212818367918));
#99984=CARTESIAN_POINT('',(7.12999614643287,2.75000000185147,1.88126430888441));
#99985=CARTESIAN_POINT('Ctrl Pts',(7.039964107,2.75,1.732456454));
#99986=CARTESIAN_POINT('Ctrl Pts',(7.133842512,2.81435393,1.35097466));
#99987=CARTESIAN_POINT('Ctrl Pts',(7.18594876,2.879481221,0.961582244));
#99988=CARTESIAN_POINT('Ctrl Pts',(7.337579839,2.75,1.552392382));
#99989=CARTESIAN_POINT('Ctrl Pts',(7.421700926,2.81435393,1.154783377));
#99990=CARTESIAN_POINT('Ctrl Pts',(7.46236430400001,2.879481221,0.750412547000001));
#99991=CARTESIAN_POINT('',(7.33757984131742,2.75,1.55239237089712));
#99992=CARTESIAN_POINT('',(7.43335640120693,2.83963938428037,0.997603432181168));
#99993=CARTESIAN_POINT('Origin',(-0.188373354874297,2.94636921314844,-0.00803358028075435));
#99994=CARTESIAN_POINT('Ctrl Pts',(7.18532477572594,2.8787032027058,0.966233854084377));
#99995=CARTESIAN_POINT('Ctrl Pts',(7.22659669178231,2.87185457188186,0.971490902133333));
#99996=CARTESIAN_POINT('Ctrl Pts',(7.26792588317493,2.86518067048678,0.976735574680769));
#99997=CARTESIAN_POINT('Ctrl Pts',(7.35058897048162,2.85217081126976,0.9871893489177));
#99998=CARTESIAN_POINT('Ctrl Pts',(7.39197238182782,2.8458270679546,0.992404710569672));
#99999=CARTESIAN_POINT('Ctrl Pts',(7.43335640141232,2.83963938428435,0.997603430550835));
#100000=CARTESIAN_POINT('',(7.18877197556053,2.74999999814853,1.64242440679273));
#100001=CARTESIAN_POINT('Origin',(-4.66640615037761E-13,2.840715057,-5.7516925250356E-14));
#100002=CARTESIAN_POINT('',(7.43335640120675,2.66036061571961,0.997603432181095));
#100003=CARTESIAN_POINT('Origin',(-0.188373354749872,2.55363078683776,-0.00803358025205148));
#100004=CARTESIAN_POINT('',(7.48763344524873,2.75,0.430517578193262));
#100005=CARTESIAN_POINT('Ctrl Pts',(7.48763344508452,2.75000000173941,0.430517578459702));
#100006=CARTESIAN_POINT('Ctrl Pts',(7.4789292985699,2.72598918212316,0.581901539071339));
#100007=CARTESIAN_POINT('Ctrl Pts',(7.46565187590449,2.70215892392418,0.732642904818717));
#100008=CARTESIAN_POINT('Ctrl Pts',(7.44791763247454,2.67857142884723,0.882339467482308));
#100009=CARTESIAN_POINT('Ctrl Pts',(7.44336545647058,2.67251679079159,0.920764849139752));
#100010=CARTESIAN_POINT('Ctrl Pts',(7.43851192655382,2.66644617724562,0.959188511968675));
#100011=CARTESIAN_POINT('Ctrl Pts',(7.43335640149295,2.66036061550664,0.997603432185768));
#100012=CARTESIAN_POINT('Ctrl Pts',(7.43335640149294,2.83963938449337,0.997603432185807));
#100013=CARTESIAN_POINT('Ctrl Pts',(7.43851192655439,2.83355382275437,0.959188511969271));
#100014=CARTESIAN_POINT('Ctrl Pts',(7.4433654566666,2.82748320916823,0.92076484908148));
#100015=CARTESIAN_POINT('Ctrl Pts',(7.4479176324752,2.82142857115279,0.882339467483236));
#100016=CARTESIAN_POINT('Ctrl Pts',(7.46565187514419,2.79784107623236,0.732642905049655));
#100017=CARTESIAN_POINT('Ctrl Pts',(7.47892929857034,2.77401081787663,0.5819015390719));
#100018=CARTESIAN_POINT('Ctrl Pts',(7.48763344508452,2.74999999826059,0.430517578459712));
#100019=CARTESIAN_POINT('Ctrl Pts',(7.184689789,2.879480225,0.970944197));
#100020=CARTESIAN_POINT('Ctrl Pts',(7.20858464,2.85030975,0.794129615));
#100021=CARTESIAN_POINT('Ctrl Pts',(7.22375305,2.821428571,0.616353689));
#100022=CARTESIAN_POINT('Ctrl Pts',(7.24239863499999,2.785926731,0.397824782));
#100023=CARTESIAN_POINT('Ctrl Pts',(7.247800585,2.75,0.178568402));
#100024=CARTESIAN_POINT('Ctrl Pts',(7.24789882198614,2.74934665560115,0.174581122228147));
#100025=CARTESIAN_POINT('Ctrl Pts',(7.24799705897229,2.7486933112023,0.170593842456293));
#100026=CARTESIAN_POINT('Ctrl Pts',(7.395499158,2.879480225,1.247634645));
#100027=CARTESIAN_POINT('Ctrl Pts',(7.426203336,2.85030975,1.065632063));
#100028=CARTESIAN_POINT('Ctrl Pts',(7.447917633,2.821428571,0.882339467));
#100029=CARTESIAN_POINT('Ctrl Pts',(7.474609669,2.785926731,0.657029259));
#100030=CARTESIAN_POINT('Ctrl Pts',(7.487633445,2.75,0.43051759));
#100031=CARTESIAN_POINT('Ctrl Pts',(7.48787028845513,2.74934665560115,0.426398369405861));
#100032=CARTESIAN_POINT('Ctrl Pts',(7.48810713191026,2.7486933112023,0.422279148811721));
#100033=CARTESIAN_POINT('',(7.36771701547478,2.75000000185146,0.304542984513805));
#100034=CARTESIAN_POINT('Ctrl Pts',(7.247800585,2.75,0.178568402));
#100035=CARTESIAN_POINT('Ctrl Pts',(7.257476856,2.81435393,-0.214175642));
#100036=CARTESIAN_POINT('Ctrl Pts',(7.22465703,2.879481221,-0.605665581999999));
#100037=CARTESIAN_POINT('Ctrl Pts',(7.499749774,2.75,-0.061264458));
#100038=CARTESIAN_POINT('Ctrl Pts',(7.49642997300001,2.81435393,-0.467661132000001));
#100039=CARTESIAN_POINT('Ctrl Pts',(7.449214889,2.879481221,-0.871319421));
#100040=CARTESIAN_POINT('',(7.49974977376454,2.75,-0.061264469340567));
#100041=CARTESIAN_POINT('',(7.47402390826455,2.83963938428077,-0.623671879939793));
#100042=CARTESIAN_POINT('Origin',(-0.185696566482395,2.94636920236734,0.0326489605617519));
#100043=CARTESIAN_POINT('Ctrl Pts',(7.22504759274717,2.87870320280466,-0.60098858640385));
#100044=CARTESIAN_POINT('Ctrl Pts',(7.26648470406984,2.87185457197965,-0.604726687300666));
#100045=CARTESIAN_POINT('Ctrl Pts',(7.30797509130833,2.8651806705829,-0.608489186847638));
#100046=CARTESIAN_POINT('Ctrl Pts',(7.39095281381384,2.85217081134085,-0.616049936504215));
#100047=CARTESIAN_POINT('Ctrl Pts',(7.43248985279003,2.84582706797145,-0.619852717380044));
#100048=CARTESIAN_POINT('Ctrl Pts',(7.47402390811265,2.83963938428477,-0.623671881598194));
#100049=CARTESIAN_POINT('',(7.37377517959144,2.74999999814853,0.0586519605043138));
#100050=CARTESIAN_POINT('Origin',(5.5944832100252E-14,2.84071505699989,
9.62873173120798E-14));
#100051=CARTESIAN_POINT('',(7.47402390826407,2.66036061571915,-0.623671879939818));
#100052=CARTESIAN_POINT('Origin',(-0.185696566312097,2.5536307976139,0.0326489605633622));
#100053=CARTESIAN_POINT('',(7.40512528964675,2.75,-1.18916754157494));
#100054=CARTESIAN_POINT('Ctrl Pts',(7.4051252896016,2.75000000173941,-1.18916754128873));
#100055=CARTESIAN_POINT('Ctrl Pts',(7.42916771795374,2.72598918212316,-1.03945171928497));
#100056=CARTESIAN_POINT('Ctrl Pts',(7.44860565166737,2.7021589239243,-0.889380349572321));
#100057=CARTESIAN_POINT('Ctrl Pts',(7.46346636079052,2.67857142886505,-0.739371271367419));
#100058=CARTESIAN_POINT('Ctrl Pts',(7.46728093354585,2.67251679082236,-0.700865670528982));
#100059=CARTESIAN_POINT('Ctrl Pts',(7.47080082797672,2.66644617725542,-0.662296966240046));
#100060=CARTESIAN_POINT('Ctrl Pts',(7.47402390859826,2.66036061551054,-0.623671880000571));
#100061=CARTESIAN_POINT('Ctrl Pts',(7.47402390859875,2.8396393844894,-0.623671880000552));
#100062=CARTESIAN_POINT('Ctrl Pts',(7.47080082797757,2.83355382274451,-0.662296966239768));
#100063=CARTESIAN_POINT('Ctrl Pts',(7.46728093347334,2.82748320915981,-0.700865670689327));
#100064=CARTESIAN_POINT('Ctrl Pts',(7.4634663607916,2.82142857113497,-0.73937127136646));
#100065=CARTESIAN_POINT('Ctrl Pts',(7.44860565195505,2.79784107614504,-0.889380348944392));
#100066=CARTESIAN_POINT('Ctrl Pts',(7.42916771795445,2.77401081787664,-1.03945171928441));
#100067=CARTESIAN_POINT('Ctrl Pts',(7.4051252896016,2.74999999826059,-1.18916754128874));
#100068=CARTESIAN_POINT('Ctrl Pts',(7.22574379878017,2.880540329927,-0.589982327261686));
#100069=CARTESIAN_POINT('Ctrl Pts',(7.21096041357039,2.85083482787434,-0.771040212929628));
#100070=CARTESIAN_POINT('Ctrl Pts',(7.18712761817257,2.821428571,-0.951130479136298));
#100071=CARTESIAN_POINT('Ctrl Pts',(7.15835455504156,2.785926731,-1.16855141510238));
#100072=CARTESIAN_POINT('Ctrl Pts',(7.11649154232713,2.75,-1.38383550852302));
#100073=CARTESIAN_POINT('Ctrl Pts',(7.11541813743386,2.74907880665164,-1.3893555842256));
#100074=CARTESIAN_POINT('Ctrl Pts',(7.11434473254058,2.74815761330328,-1.39487565992819));
#100075=CARTESIAN_POINT('Ctrl Pts',(7.49113016545384,2.880540329927,-0.36464893196537));
#100076=CARTESIAN_POINT('Ctrl Pts',(7.48199303513689,2.85083482787434,-0.552356692243661));
#100077=CARTESIAN_POINT('Ctrl Pts',(7.463466361,2.821428571,-0.739371272));
#100078=CARTESIAN_POINT('Ctrl Pts',(7.441099318,2.785926731,-0.965151851));
#100079=CARTESIAN_POINT('Ctrl Pts',(7.405125292,2.75,-1.18916753));
#100080=CARTESIAN_POINT('Ctrl Pts',(7.40420288596577,2.74907880665164,-1.1949114913257));
#100081=CARTESIAN_POINT('Ctrl Pts',(7.40328047993151,2.74815761330329,-1.2006554526514));
#100082=CARTESIAN_POINT('',(7.26093162549449,2.75000000185147,-1.28641843181972));
#100083=CARTESIAN_POINT('Ctrl Pts',(7.11673796300001,2.75,-1.383669311));
#100084=CARTESIAN_POINT('Ctrl Pts',(7.041759648,2.81435393,-1.769311329));
#100085=CARTESIAN_POINT('Ctrl Pts',(6.925548367,2.879481221,-2.14459316));
#100086=CARTESIAN_POINT('Ctrl Pts',(7.311239744,2.75,-1.672056639));
#100087=CARTESIAN_POINT('Ctrl Pts',(7.220634287,2.81435393,-2.068238326));
#100088=CARTESIAN_POINT('Ctrl Pts',(7.087748465,2.879481221,-2.452309461));
#100089=CARTESIAN_POINT('',(7.31123974150887,2.75,-1.67205665006523));
#100090=CARTESIAN_POINT('',(7.1652143640651,2.83963938426122,-2.21578498726053));
#100091=CARTESIAN_POINT('Origin',(-0.174336251871083,2.94636921029586,0.0718048408766353));
#100092=CARTESIAN_POINT('Ctrl Pts',(6.92693521455026,2.87870320272253,-2.14010946892607));
#100093=CARTESIAN_POINT('Ctrl Pts',(6.96659996794133,2.87185457192133,-2.15266792919406));
#100094=CARTESIAN_POINT('Ctrl Pts',(7.00631150668629,2.8651806705447,-2.16526167034536));
#100095=CARTESIAN_POINT('Ctrl Pts',(7.08572391840278,2.85217081130674,-2.1904834112367));
#100096=CARTESIAN_POINT('Ctrl Pts',(7.12547235876744,2.84582706796812,-2.20312652055182));
#100097=CARTESIAN_POINT('Ctrl Pts',(7.16521436356818,2.8396393842652,-2.2157849888226));
#100098=CARTESIAN_POINT('',(7.21398885111807,2.74999999814853,-1.52786298624658));
#100099=CARTESIAN_POINT('Origin',(-1.04083408558608E-14,2.84071505699967,
-1.3238108526048E-13));
#100100=CARTESIAN_POINT('',(7.16521436406483,2.66036061573874,-2.21578498726049));
#100101=CARTESIAN_POINT('Origin',(-0.174336251676337,2.55363078968169,0.0718048408357719));
#100102=CARTESIAN_POINT('',(6.97636170529881,2.75,-2.75324850883221));
#100103=CARTESIAN_POINT('Ctrl Pts',(6.97636170523082,2.75000000173941,-2.75324850850928));
#100104=CARTESIAN_POINT('Ctrl Pts',(7.03202651153764,2.72598918212314,-2.61220137043643));
#100105=CARTESIAN_POINT('Ctrl Pts',(7.08327090563027,2.70215892392449,-2.46981716683914));
#100106=CARTESIAN_POINT('Ctrl Pts',(7.13003169698747,2.67857142889278,-2.32650983045378));
#100107=CARTESIAN_POINT('Ctrl Pts',(7.14203465313809,2.6725167908538,-2.28972448961772));
#100108=CARTESIAN_POINT('Ctrl Pts',(7.15376338573902,2.6664461772565,-2.25281417336172));
#100109=CARTESIAN_POINT('Ctrl Pts',(7.16521436431504,2.66036061552466,-2.21578498737305));
#100110=CARTESIAN_POINT('Ctrl Pts',(7.16521436431505,2.83963938447534,-2.21578498737302));
#100111=CARTESIAN_POINT('Ctrl Pts',(7.15376338574019,2.83355382274348,-2.25281417336128));
#100112=CARTESIAN_POINT('Ctrl Pts',(7.14203465296253,2.82748320916324,-2.28972448961258));
#100113=CARTESIAN_POINT('Ctrl Pts',(7.13003169690104,2.82142857110724,-2.32650983049405));
#100114=CARTESIAN_POINT('Ctrl Pts',(7.08327090589077,2.79784107600908,-2.46981716705734));
#100115=CARTESIAN_POINT('Ctrl Pts',(7.03202651153861,2.77401081787666,-2.61220137043596));
#100116=CARTESIAN_POINT('Ctrl Pts',(6.97636170523082,2.74999999826059,-2.75324850850928));
#100117=CARTESIAN_POINT('Ctrl Pts',(6.928336737,2.879480225,-2.135567854));
#100118=CARTESIAN_POINT('Ctrl Pts',(6.87578060099999,2.85030975,-2.30607361));
#100119=CARTESIAN_POINT('Ctrl Pts',(6.814900903,2.821428571,-2.47378772));
#100120=CARTESIAN_POINT('Ctrl Pts',(6.740065271,2.785926731,-2.679948262));
#100121=CARTESIAN_POINT('Ctrl Pts',(6.652904584,2.75,-2.881208184));
#100122=CARTESIAN_POINT('Ctrl Pts',(6.6513195261596,2.74934665560115,-2.88486818976984));
#100123=CARTESIAN_POINT('Ctrl Pts',(6.64973446831921,2.7486933112023,-2.88852819553969));
#100124=CARTESIAN_POINT('Ctrl Pts',(7.23584144200001,2.879480225,-1.972966961));
#100125=CARTESIAN_POINT('Ctrl Pts',(7.187286899,2.85030975,-2.15104038));
#100126=CARTESIAN_POINT('Ctrl Pts',(7.130031697,2.821428571,-2.326509831));
#100127=CARTESIAN_POINT('Ctrl Pts',(7.059651433,2.785926731,-2.542203533));
#100128=CARTESIAN_POINT('Ctrl Pts',(6.97636171000001,2.75,-2.753248498));
#100129=CARTESIAN_POINT('Ctrl Pts',(6.9748470474496,2.74934665560115,-2.75708644935127));
#100130=CARTESIAN_POINT('Ctrl Pts',(6.97333238489921,2.7486933112023,-2.76092440070255));
#100131=CARTESIAN_POINT('',(6.81463314260797,2.75000000185147,-2.81722835162395));
#100132=CARTESIAN_POINT('Ctrl Pts',(6.652904584,2.75,-2.881208184));
#100133=CARTESIAN_POINT('Ctrl Pts',(6.49677758500001,2.81435393,-3.241715985));
#100134=CARTESIAN_POINT('Ctrl Pts',(6.302608759,2.879481221,-3.583241945));
#100135=CARTESIAN_POINT('Ctrl Pts',(6.78086427000001,2.75,-3.20466531));
#100136=CARTESIAN_POINT('Ctrl Pts',(6.607209766,2.81435393,-3.572106995));
#100137=CARTESIAN_POINT('Ctrl Pts',(6.394866801,2.879481221,-3.918632236));
#100138=CARTESIAN_POINT('',(6.78086426520829,2.75,-3.20466532028041));
#100139=CARTESIAN_POINT('',(6.5213673600565,2.83963938426449,-3.70429045185705));
#100140=CARTESIAN_POINT('Origin',(-0.154824635565474,2.94636926992071,0.107603327694034));
#100141=CARTESIAN_POINT('Ctrl Pts',(6.30492704407009,2.8787032026541,-3.57916121100237));
#100142=CARTESIAN_POINT('Ctrl Pts',(6.34096475976856,2.87185457189683,-3.59995281093015));
#100143=CARTESIAN_POINT('Ctrl Pts',(6.37704058264914,2.86518067055398,-3.62078892438102));
#100144=CARTESIAN_POINT('Ctrl Pts',(6.44917444755483,2.8521708113417,-3.66249231621842));
#100145=CARTESIAN_POINT('Ctrl Pts',(6.48527569685389,2.84582706798045,-3.68338457656364));
#100146=CARTESIAN_POINT('Ctrl Pts',(6.52136735922969,2.83963938426847,-3.70429045328561));
#100147=CARTESIAN_POINT('',(6.71688442225607,2.74999999814853,-3.04293675747159));
#100148=CARTESIAN_POINT('Origin',(-6.65266453037106E-13,2.84071505699989,
3.67761376907083E-13));
#100149=CARTESIAN_POINT('',(6.52136736005646,2.6603606157355,-3.70429045185702));
#100150=CARTESIAN_POINT('Origin',(-0.15482463553375,2.55363073007556,0.107603327679747));
#100151=CARTESIAN_POINT('',(6.2213912019492,2.75,-4.18859063547911));
#100152=CARTESIAN_POINT('Ctrl Pts',(6.22139120208406,2.75000000173934,-4.18859063523788));
#100153=CARTESIAN_POINT('Ctrl Pts',(6.30607556111986,2.72598918212307,-4.06280738917551));
#100154=CARTESIAN_POINT('Ctrl Pts',(6.38673028461759,2.70215892392445,-3.93476807920542));
#100155=CARTESIAN_POINT('Ctrl Pts',(6.46320467600042,2.67857142888631,-3.8048633764564));
#100156=CARTESIAN_POINT('Ctrl Pts',(6.48283477051439,2.67251679084892,-3.77151833718257));
#100157=CARTESIAN_POINT('Ctrl Pts',(6.50222391884417,2.66644617725987,-3.73799229439273));
#100158=CARTESIAN_POINT('Ctrl Pts',(6.52136736030762,2.66036061552477,-3.70429045203774));
#100159=CARTESIAN_POINT('Ctrl Pts',(6.52136736030762,2.83963938447523,-3.70429045203774));
#100160=CARTESIAN_POINT('Ctrl Pts',(6.50222391884436,2.83355382274013,-3.7379922943927));
#100161=CARTESIAN_POINT('Ctrl Pts',(6.482834770476,2.82748320916001,-3.77151833714848));
#100162=CARTESIAN_POINT('Ctrl Pts',(6.46320467600067,2.82142857111369,-3.80486337645633));
#100163=CARTESIAN_POINT('Ctrl Pts',(6.38673028476825,2.79784107604075,-3.93476807933803));
#100164=CARTESIAN_POINT('Ctrl Pts',(6.30607556112001,2.77401081787675,-4.06280738917544));
#100165=CARTESIAN_POINT('Ctrl Pts',(6.22139120208405,2.74999999826065,-4.18859063523787));
#100166=CARTESIAN_POINT('Ctrl Pts',(6.307272113,2.879480225,-3.575027062));
#100167=CARTESIAN_POINT('Ctrl Pts',(6.219291012,2.85030975,-3.730248473));
#100168=CARTESIAN_POINT('Ctrl Pts',(6.123781072,2.821428571,-3.880954185));
#100169=CARTESIAN_POINT('Ctrl Pts',(6.006376632,2.785926731,-4.06620736));
#100170=CARTESIAN_POINT('Ctrl Pts',(5.87798878,2.75,-4.244024965));
#100171=CARTESIAN_POINT('Ctrl Pts',(5.87565398689053,2.74934665560115,-4.247258661276));
#100172=CARTESIAN_POINT('Ctrl Pts',(5.87331919378106,2.7486933112023,-4.25049235755201));
#100173=CARTESIAN_POINT('Ctrl Pts',(6.64254191400001,2.879480225,-3.48233211));
#100174=CARTESIAN_POINT('Ctrl Pts',(6.556842028,2.85030975,-3.64580448));
#100175=CARTESIAN_POINT('Ctrl Pts',(6.463204676,2.821428571,-3.804863377));
#100176=CARTESIAN_POINT('Ctrl Pts',(6.348102093,2.785926731,-4.000384604));
#100177=CARTESIAN_POINT('Ctrl Pts',(6.221391209,2.75,-4.188590626));
#100178=CARTESIAN_POINT('Ctrl Pts',(6.21908691233759,2.74934665560115,-4.19201324049569));
#100179=CARTESIAN_POINT('Ctrl Pts',(6.21678261567518,2.7486933112023,-4.19543585499139));
#100180=CARTESIAN_POINT('',(6.04968998792708,2.75000000185138,-4.21630780493103));
#100181=CARTESIAN_POINT('Ctrl Pts',(5.87798878,2.75,-4.244024965));
#100182=CARTESIAN_POINT('Ctrl Pts',(5.648013423,2.81435393,-4.562541604));
#100183=CARTESIAN_POINT('Ctrl Pts',(5.38496617,2.879481221,-4.854342319));
#100184=CARTESIAN_POINT('Ctrl Pts',(5.933423119,2.75,-4.587427393));
#100185=CARTESIAN_POINT('Ctrl Pts',(5.684839461,2.81435393,-4.90894791));
#100186=CARTESIAN_POINT('Ctrl Pts',(5.402968272,2.879481221,-5.201724123));
#100187=CARTESIAN_POINT('',(5.93342311214813,2.75,-4.58742740203919));
#100188=CARTESIAN_POINT('',(5.5725884661497,2.83963938431518,-5.01958741169361));
#100189=CARTESIAN_POINT('Origin',(-0.128073249550485,2.9463692159568,0.138370213108596));
#100190=CARTESIAN_POINT('Ctrl Pts',(5.38810749189843,2.87870320268935,-4.85085535321375));
#100191=CARTESIAN_POINT('Ctrl Pts',(5.41883308675611,2.871854571875,-4.87890790060259));
#100192=CARTESIAN_POINT('Ctrl Pts',(5.4495863287704,2.86518067048863,-4.90701211292848));
#100193=CARTESIAN_POINT('Ctrl Pts',(5.5110687475944,2.852170811308,-4.96324715123295));
#100194=CARTESIAN_POINT('Ctrl Pts',(5.5418347513048,2.84582706798285,-4.99141166354931));
#100195=CARTESIAN_POINT('Ctrl Pts',(5.57258846503531,2.83963938431916,-5.01958741291084));
#100196=CARTESIAN_POINT('',(5.9057059426159,2.74999999814853,-4.41572618820698));
#100197=CARTESIAN_POINT('Origin',(-5.20850723662036E-13,2.84071505700067,
4.48426018540005E-13));
#100198=CARTESIAN_POINT('',(5.57258846614968,2.66036061568482,-5.01958741169357));
#100199=CARTESIAN_POINT('Origin',(-0.128073249529073,2.55363078404042,0.138370213093019));
#100200=CARTESIAN_POINT('',(5.17551536021189,2.75,-5.42807891888395));
#100201=CARTESIAN_POINT('Ctrl Pts',(5.1755153602599,2.75000000173934,-5.42807891853518));
#100202=CARTESIAN_POINT('Ctrl Pts',(5.28525952558719,2.7259891821231,-5.32344104899518));
#100203=CARTESIAN_POINT('Ctrl Pts',(5.39155325324616,2.7021589239245,-5.21573360859195));
#100204=CARTESIAN_POINT('Ctrl Pts',(5.49416538711631,2.67857142889486,-5.1053057395091));
#100205=CARTESIAN_POINT('Ctrl Pts',(5.52050473880592,2.67251679084257,-5.07696017883811));
#100206=CARTESIAN_POINT('Ctrl Pts',(5.54664768791324,2.66644617722575,-5.04838604997926));
#100207=CARTESIAN_POINT('Ctrl Pts',(5.57258846635438,2.66036061547379,-5.01958741192256));
#100208=CARTESIAN_POINT('Ctrl Pts',(5.57258846635438,2.83963938452621,-5.01958741192256));
#100209=CARTESIAN_POINT('Ctrl Pts',(5.54664768791338,2.83355382277425,-5.04838604997928));
#100210=CARTESIAN_POINT('Ctrl Pts',(5.52050473877698,2.82748320917711,-5.07696017874644));
#100211=CARTESIAN_POINT('Ctrl Pts',(5.49416538711348,2.82142857110514,-5.1053057395091));
#100212=CARTESIAN_POINT('Ctrl Pts',(5.39155325334494,2.79784107599881,-5.21573360894922));
#100213=CARTESIAN_POINT('Ctrl Pts',(5.28525952558731,2.77401081787672,-5.32344104899515));
#100214=CARTESIAN_POINT('Ctrl Pts',(5.1755153602599,2.74999999826065,-5.42807891853518));
#100215=CARTESIAN_POINT('Ctrl Pts',(5.391286454,2.879480225,-4.84732197900001));
#100216=CARTESIAN_POINT('Ctrl Pts',(5.271994288,2.85030975,-4.980001063));
#100217=CARTESIAN_POINT('Ctrl Pts',(5.146320044,2.821428571,-5.106651545));
#100218=CARTESIAN_POINT('Ctrl Pts',(4.991836498,2.785926731,-5.26233512));
#100219=CARTESIAN_POINT('Ctrl Pts',(4.828224754,2.75,-5.408395855));
#100220=CARTESIAN_POINT('Ctrl Pts',(4.82524939794747,2.74934665560115,-5.41105203774884));
#100221=CARTESIAN_POINT('Ctrl Pts',(4.82227404189494,2.7486933112023,-5.41370822049767));
#100222=CARTESIAN_POINT('Ctrl Pts',(5.73864450900001,2.879480225,-4.828867279));
#100223=CARTESIAN_POINT('Ctrl Pts',(5.619806511,2.85030975,-4.970094815));
#100224=CARTESIAN_POINT('Ctrl Pts',(5.494165387,2.821428571,-5.10530574));
#100225=CARTESIAN_POINT('Ctrl Pts',(5.33972255400001,2.785926731,-5.271512136));
#100226=CARTESIAN_POINT('Ctrl Pts',(5.175515369,2.75,-5.428078911));
#100227=CARTESIAN_POINT('Ctrl Pts',(5.17252918457452,2.74934665560115,-5.43092615099776));
#100228=CARTESIAN_POINT('Ctrl Pts',(5.16954300014905,2.7486933112023,-5.43377339099553));
#100229=CARTESIAN_POINT('',(5.00187005305336,2.75000000185138,-5.41823739079755));
#100230=CARTESIAN_POINT('Ctrl Pts',(4.828224754,2.75,-5.408395855));
#100231=CARTESIAN_POINT('Ctrl Pts',(4.535154431,2.81435393,-5.670027848));
#100232=CARTESIAN_POINT('Ctrl Pts',(4.215528549,2.879481221,-5.898459041));
#100233=CARTESIAN_POINT('Ctrl Pts',(4.808541698,2.75,-5.75568647));
#100234=CARTESIAN_POINT('Ctrl Pts',(4.49665238,2.81435393,-6.016251877));
#100235=CARTESIAN_POINT('Ctrl Pts',(4.158432951,2.879481221,-6.241589172));
#100236=CARTESIAN_POINT('',(4.80854168926236,2.75,-5.75568647723186));
#100237=CARTESIAN_POINT('',(4.36324152879854,2.83963938426255,-6.10017404315626));
#100238=CARTESIAN_POINT('Origin',(-0.0953336098313168,2.94636920711836,
0.162667358570282));
#100239=CARTESIAN_POINT('Ctrl Pts',(4.21934602295708,2.87870320271879,-5.89572888998683));
#100240=CARTESIAN_POINT('Ctrl Pts',(4.24332280172585,2.87185457190337,-5.92973067904311));
#100241=CARTESIAN_POINT('Ctrl Pts',(4.2673154748862,2.86518067052144,-5.9637888683585));
#100242=CARTESIAN_POINT('Ctrl Pts',(4.31527159774156,2.85217081130269,-6.03192606541324));
#100243=CARTESIAN_POINT('Ctrl Pts',(4.33926377175047,2.84582706794485,-6.06604588857911));
#100244=CARTESIAN_POINT('Ctrl Pts',(4.36324152744183,2.83963938426654,-6.10017404411018));
#100245=CARTESIAN_POINT('',(4.81838321729762,2.74999999814853,-5.58204117001184));
#100246=CARTESIAN_POINT('Origin',(-1.45283091113058E-13,2.84071505700011,
1.50920942409982E-13));
#100247=CARTESIAN_POINT('',(4.36324152879854,2.66036061573744,-6.10017404315625));
#100248=CARTESIAN_POINT('Origin',(-0.0953336098246177,2.55363079288176,
0.162667358561808));
#100249=CARTESIAN_POINT('',(3.88763817265509,2.75,-6.41375626569998));
#100250=CARTESIAN_POINT('Ctrl Pts',(3.88763817284382,2.75000000173934,-6.41375626547999));
#100251=CARTESIAN_POINT('Ctrl Pts',(4.01731062957616,2.72598918212306,-6.33515652268646));
#100252=CARTESIAN_POINT('Ctrl Pts',(4.14427318472604,2.70215892392422,-6.25281723181124));
#100253=CARTESIAN_POINT('Ctrl Pts',(4.26822503138358,2.67857142885272,-6.16702968037998));
#100254=CARTESIAN_POINT('Ctrl Pts',(4.30004204137926,2.67251679081034,-6.14500900501089));
#100255=CARTESIAN_POINT('Ctrl Pts',(4.33171637566225,2.66644617726505,-6.122722884807));
#100256=CARTESIAN_POINT('Ctrl Pts',(4.36324152896542,2.66036061552908,-6.10017404344581));
#100257=CARTESIAN_POINT('Ctrl Pts',(4.36324152896542,2.83963938447092,-6.10017404344581));
#100258=CARTESIAN_POINT('Ctrl Pts',(4.33171637566227,2.83355382273495,-6.12272288480701));
#100259=CARTESIAN_POINT('Ctrl Pts',(4.30004204116324,2.82748320915638,-6.14500900512305));
#100260=CARTESIAN_POINT('Ctrl Pts',(4.26822503138362,2.82142857114729,-6.16702968037998));
#100261=CARTESIAN_POINT('Ctrl Pts',(4.14427318556775,2.79784107620545,-6.25281723137432));
#100262=CARTESIAN_POINT('Ctrl Pts',(4.01731062957619,2.77401081787675,-6.33515652268643));
#100263=CARTESIAN_POINT('Ctrl Pts',(3.88763817284382,2.74999999826065,-6.41375626547999));
#100264=CARTESIAN_POINT('Ctrl Pts',(4.223210233,2.879480225,-5.892961507));
#100265=CARTESIAN_POINT('Ctrl Pts',(4.07818497,2.85030975,-5.996894338));
#100266=CARTESIAN_POINT('Ctrl Pts',(3.928222811,2.821428571,-6.093567555));
#100267=CARTESIAN_POINT('Ctrl Pts',(3.743883638,2.785926731,-6.212401939));
#100268=CARTESIAN_POINT('Ctrl Pts',(3.552698305,2.75,-6.319876166));
#100269=CARTESIAN_POINT('Ctrl Pts',(3.54922151034096,2.74934665560115,-6.3218306350618));
#100270=CARTESIAN_POINT('Ctrl Pts',(3.54574471568191,2.7486933112023,-6.3237851041236));
#100271=CARTESIAN_POINT('Ctrl Pts',(4.566414464,2.879480225,-5.949609982));
#100272=CARTESIAN_POINT('Ctrl Pts',(4.419995088,2.85030975,-6.061989039));
#100273=CARTESIAN_POINT('Ctrl Pts',(4.268225031,2.821428571,-6.167029681));
#100274=CARTESIAN_POINT('Ctrl Pts',(4.081663524,2.785926731,-6.29614962));
#100275=CARTESIAN_POINT('Ctrl Pts',(3.887638183,2.75,-6.41375626));
#100276=CARTESIAN_POINT('Ctrl Pts',(3.88410974146778,2.74934665560115,-6.41589499172907));
#100277=CARTESIAN_POINT('Ctrl Pts',(3.88058129993557,2.7486933112023,-6.41803372345814));
#100278=CARTESIAN_POINT('',(3.7201682340746,2.75000000185138,-6.36681621879948));
#100279=CARTESIAN_POINT('Ctrl Pts',(3.552698305,2.75,-6.319876166));
#100280=CARTESIAN_POINT('Ctrl Pts',(3.210236658,2.81435393,-6.512389893));
#100281=CARTESIAN_POINT('Ctrl Pts',(2.848977497,2.879481221,-6.666770374));
#100282=CARTESIAN_POINT('Ctrl Pts',(3.458818211,2.75,-6.654816044));
#100283=CARTESIAN_POINT('Ctrl Pts',(3.098206832,2.81435393,-6.84224259300001));
#100284=CARTESIAN_POINT('Ctrl Pts',(2.719453928,2.879481221,-6.989604448));
#100285=CARTESIAN_POINT('',(3.45881820097473,2.75,-6.65481604930514));
#100286=CARTESIAN_POINT('',(2.94987426729199,2.83963938428779,-6.89552331626262));
#100287=CARTESIAN_POINT('Origin',(-0.0581360810472636,2.94636920663246,
0.179358157749951));
#100288=CARTESIAN_POINT('Ctrl Pts',(2.85329262215939,2.87870320274543,-6.66492469653363));
#100289=CARTESIAN_POINT('Ctrl Pts',(2.86939945776764,2.87185457193515,-6.70328584159086));
#100290=CARTESIAN_POINT('Ctrl Pts',(2.88550969177699,2.86518067054803,-6.74170548506837));
#100291=CARTESIAN_POINT('Ctrl Pts',(2.91769714417173,2.85217081132374,-6.81855882132505));
#100292=CARTESIAN_POINT('Ctrl Pts',(2.93379364116285,2.84582706797916,-6.85703855007138));
#100293=CARTESIAN_POINT('Ctrl Pts',(2.9498742657648,2.83963938429177,-6.89552331690139));
#100294=CARTESIAN_POINT('',(3.50575824788625,2.74999999814853,-6.48734611046546));
#100295=CARTESIAN_POINT('Origin',(2.43511807940244E-13,2.84071505700011,
-7.83227649403528E-13));
#100296=CARTESIAN_POINT('',(2.949874267292,2.66036061571221,-6.89552331626262));
#100297=CARTESIAN_POINT('Origin',(-0.0581360810464882,2.55363079336866,
0.179358157747066));
#100298=CARTESIAN_POINT('',(2.41797934471617,2.75,-7.09953349747217));
#100299=CARTESIAN_POINT('Ctrl Pts',(2.41797934490384,2.75000000173934,-7.09953349716892));
#100300=CARTESIAN_POINT('Ctrl Pts',(2.56151675261816,2.72598918212304,-7.05064711788722));
#100301=CARTESIAN_POINT('Ctrl Pts',(2.70321150762957,2.70215892392445,-6.99752607038529));
#100302=CARTESIAN_POINT('Ctrl Pts',(2.84270721710102,2.67857142888649,-6.94039016746389));
#100303=CARTESIAN_POINT('Ctrl Pts',(2.87851415700855,2.67251679084317,-6.92572403990961));
#100304=CARTESIAN_POINT('Ctrl Pts',(2.91423882038528,2.6664461772466,-6.91076800243955));
#100305=CARTESIAN_POINT('Ctrl Pts',(2.94987426738843,2.66036061550281,-6.89552331657164));
#100306=CARTESIAN_POINT('Ctrl Pts',(2.94987426738843,2.83963938449719,-6.89552331657164));
#100307=CARTESIAN_POINT('Ctrl Pts',(2.91423882038527,2.8335538227534,-6.91076800243956));
#100308=CARTESIAN_POINT('Ctrl Pts',(2.87851415728558,2.82748320916599,-6.92572403998946));
#100309=CARTESIAN_POINT('Ctrl Pts',(2.84270721710102,2.82142857111351,-6.94039016746388));
#100310=CARTESIAN_POINT('Ctrl Pts',(2.70321150655026,2.79784107603985,-6.99752607007421));
#100311=CARTESIAN_POINT('Ctrl Pts',(2.56151675261817,2.77401081787678,-7.05064711788719));
#100312=CARTESIAN_POINT('Ctrl Pts',(2.41797934490384,2.74999999826065,-7.09953349716892));
#100313=CARTESIAN_POINT('Ctrl Pts',(2.86334288997134,2.88054032922091,-6.66038437985894));
#100314=CARTESIAN_POINT('Ctrl Pts',(2.69645140622961,2.85083482752464,-6.7321321221731));
#100315=CARTESIAN_POINT('Ctrl Pts',(2.52617600579015,2.821428571,-6.79543136056091));
#100316=CARTESIAN_POINT('Ctrl Pts',(2.32060444466131,2.785926731,-6.87185181346664));
#100317=CARTESIAN_POINT('Ctrl Pts',(2.11078936785013,2.75,-6.93570622463011));
#100318=CARTESIAN_POINT('Ctrl Pts',(2.10540952396099,2.74907880688478,-6.93734350813192));
#100319=CARTESIAN_POINT('Ctrl Pts',(2.10002968007185,2.74815761376957,-6.93898079163371));
#100320=CARTESIAN_POINT('Ctrl Pts',(3.18673687309472,2.88054032922091,-6.78930836744132));
#100321=CARTESIAN_POINT('Ctrl Pts',(3.01661489805259,2.85083482752464,-6.86915950063725));
#100322=CARTESIAN_POINT('Ctrl Pts',(2.842707217,2.821428571,-6.940390168));
#100323=CARTESIAN_POINT('Ctrl Pts',(2.632750443,2.785926731,-7.026386145));
#100324=CARTESIAN_POINT('Ctrl Pts',(2.417979356,2.75,-7.099533494));
#100325=CARTESIAN_POINT('Ctrl Pts',(2.41247243563221,2.74907880688478,-7.10140905663594));
#100326=CARTESIAN_POINT('Ctrl Pts',(2.40696551526442,2.74815761376956,-7.10328461927189));
#100327=CARTESIAN_POINT('',(2.26451548255993,2.75000000185138,-7.01768979653022));
#100328=CARTESIAN_POINT('Ctrl Pts',(2.111051631,2.75,-6.93584609200001));
#100329=CARTESIAN_POINT('Ctrl Pts',(1.735211787,2.81435393,-7.050239824));
#100330=CARTESIAN_POINT('Ctrl Pts',(1.349211424,2.879481221,-7.12335093400001));
#100331=CARTESIAN_POINT('Ctrl Pts',(1.947364229,2.75,-7.242773817));
#100332=CARTESIAN_POINT('Ctrl Pts',(1.554892575,2.81435393,-7.34829765));
#100333=CARTESIAN_POINT('Ctrl Pts',(1.153316261,2.879481221,-7.410793588));
#100334=CARTESIAN_POINT('',(1.94736421802029,2.75,-7.24277381984604));
#100335=CARTESIAN_POINT('',(1.39857416315072,2.83963938425915,-7.36844558274882));
#100336=CARTESIAN_POINT('Origin',(-0.0182202012778113,2.94636924245329,
0.187662522287977));
#100337=CARTESIAN_POINT('Ctrl Pts',(1.35382242975619,2.87870320279233,-7.12247603185831));
#100338=CARTESIAN_POINT('Ctrl Pts',(1.36130618454109,2.8718545719451,-7.1634028081296));
#100339=CARTESIAN_POINT('Ctrl Pts',(1.36878068266059,2.8651806705191,-7.20438744592115));
#100340=CARTESIAN_POINT('Ctrl Pts',(1.38369441476349,2.85217081129476,-7.28636334460521));
#100341=CARTESIAN_POINT('Ctrl Pts',(1.39114258031019,2.84582706794182,-7.32740370979372));
#100342=CARTESIAN_POINT('Ctrl Pts',(1.39857416152078,2.83963938426313,-7.36844558304456));
#100343=CARTESIAN_POINT('',(2.02920791894779,2.74999999814853,-7.08930995766353));
#100344=CARTESIAN_POINT('Origin',(-2.39825520553794E-13,2.84071505700044,
1.3240276930393E-12));
#100345=CARTESIAN_POINT('',(1.39857416315073,2.66036061574086,-7.36844558274881));
#100346=CARTESIAN_POINT('Origin',(-0.0182202012776395,2.5536307575481,0.187662522285998));
#100347=CARTESIAN_POINT('',(0.835258490224588,2.75,-7.45334443388523));
#100348=CARTESIAN_POINT('Ctrl Pts',(0.835258490482039,2.75000000173934,
-7.45334443370948));
#100349=CARTESIAN_POINT('Ctrl Pts',(0.985949199742631,2.72598918212304,
-7.43645729020576));
#100350=CARTESIAN_POINT('Ctrl Pts',(1.13575066492352,2.70215892392457,-7.41503836687994));
#100351=CARTESIAN_POINT('Ctrl Pts',(1.28426757234363,2.67857142890408,-7.38922572369872));
#100352=CARTESIAN_POINT('Ctrl Pts',(1.32239014986553,2.67251679087538,-7.38259991596011));
#100353=CARTESIAN_POINT('Ctrl Pts',(1.36049469628082,2.66644617726638,-7.37567328884459));
#100354=CARTESIAN_POINT('Ctrl Pts',(1.39857416317938,2.66036061553191,-7.36844558307566));
#100355=CARTESIAN_POINT('Ctrl Pts',(1.39857416317937,2.83963938446809,-7.36844558307567));
#100356=CARTESIAN_POINT('Ctrl Pts',(1.36049469628082,2.83355382273362,-7.37567328884459));
#100357=CARTESIAN_POINT('Ctrl Pts',(1.32239014995584,2.82748320915589,-7.38259991584564));
#100358=CARTESIAN_POINT('Ctrl Pts',(1.28426757232936,2.82142857109592,-7.38922572368795));
#100359=CARTESIAN_POINT('Ctrl Pts',(1.1357506645018,2.79784107595362,-7.4150383672732));
#100360=CARTESIAN_POINT('Ctrl Pts',(0.985949199742657,2.77401081787678,
-7.43645729020573));
#100361=CARTESIAN_POINT('Ctrl Pts',(0.835258490482038,2.74999999826065,
-7.45334443370947));
#100362=CARTESIAN_POINT('Ctrl Pts',(1.36461376391627,2.88054032957737,-7.12020237567227));
#100363=CARTESIAN_POINT('Ctrl Pts',(1.18620046619936,2.85083482770118,-7.15439595949493));
#100364=CARTESIAN_POINT('Ctrl Pts',(1.00629854418785,2.821428571,-7.17961111971661));
#100365=CARTESIAN_POINT('Ctrl Pts',(0.789104992932871,2.785926731,-7.21005309657259));
#100366=CARTESIAN_POINT('Ctrl Pts',(0.570468464739401,2.75,-7.22731058680332));
#100367=CARTESIAN_POINT('Ctrl Pts',(0.564862430624157,2.74907880681559,
-7.22775308412879));
#100368=CARTESIAN_POINT('Ctrl Pts',(0.559256396508915,2.74815761363118,
-7.22819558145427));
#100369=CARTESIAN_POINT('Ctrl Pts',(1.65273212970456,2.88054032957737,-7.31563233797624));
#100370=CARTESIAN_POINT('Ctrl Pts',(1.46942187764671,2.85083482770118,-7.35704540162157));
#100371=CARTESIAN_POINT('Ctrl Pts',(1.284267572,2.821428571,-7.389225724));
#100372=CARTESIAN_POINT('Ctrl Pts',(1.060732878,2.785926731,-7.428076663));
#100373=CARTESIAN_POINT('Ctrl Pts',(0.835258502,2.75,-7.453344433));
#100374=CARTESIAN_POINT('Ctrl Pts',(0.829477139414281,2.74907880681559,
-7.45399232098928));
#100375=CARTESIAN_POINT('Ctrl Pts',(0.823695776828564,2.74815761363118,
-7.45464020897858));
#100376=CARTESIAN_POINT('',(0.702976504056814,2.75000000185138,-7.34042399909589));
#100377=CARTESIAN_POINT('Ctrl Pts',(0.570694529,2.75,-7.227503563));
#100378=CARTESIAN_POINT('Ctrl Pts',(0.179050341,2.81435393,-7.258428376));
#100379=CARTESIAN_POINT('Ctrl Pts',(-0.213642275,2.879481221,-7.246851522));
#100380=CARTESIAN_POINT('Ctrl Pts',(0.344853659,2.75,-7.492067535));
#100381=CARTESIAN_POINT('Ctrl Pts',(-0.06112673,2.81435393,-7.510754476));
#100382=CARTESIAN_POINT('Ctrl Pts',(-0.466749192,2.879481221,-7.485462256));
#100383=CARTESIAN_POINT('Ctrl Pts',(-0.208950993846245,2.8787032027828,
-7.24698830451023));
#100384=CARTESIAN_POINT('Ctrl Pts',(-0.210440252485708,2.87185457196389,
-7.28856702129115));
#100385=CARTESIAN_POINT('Ctrl Pts',(-0.211950989736505,2.86518067057272,
-7.33020025685042));
#100386=CARTESIAN_POINT('Ctrl Pts',(-0.215008327563085,2.85217081134745,
-7.41346561591905));
#100387=CARTESIAN_POINT('Ctrl Pts',(-0.216556761366686,2.84582706794544,
-7.45514761582421));
#100388=CARTESIAN_POINT('Ctrl Pts',(-0.21812171594292,2.83963938424759,
-7.49682752321784));
#100389=CARTESIAN_POINT('',(0.457774082526124,2.74999999814853,-7.35978554971367));
#100390=CARTESIAN_POINT('Ctrl Pts',(-0.204199974,2.879480225,-7.247123731));
#100391=CARTESIAN_POINT('Ctrl Pts',(-0.382551049,2.85030975,-7.242098388));
#100392=CARTESIAN_POINT('Ctrl Pts',(-0.560439023,2.821428571,-7.228306033));
#100393=CARTESIAN_POINT('Ctrl Pts',(-0.779105665,2.785926731,-7.211351947));
#100394=CARTESIAN_POINT('Ctrl Pts',(-0.996347613999999,2.75,-7.181211));
#100395=CARTESIAN_POINT('Ctrl Pts',(-1.00029826040238,2.74934665560115,
-7.18066287278802));
#100396=CARTESIAN_POINT('Ctrl Pts',(-1.00424890680475,2.7486933112023,-7.18011474557605));
#100397=CARTESIAN_POINT('Ctrl Pts',(0.034740338,2.879480225,-7.49991954));
#100398=CARTESIAN_POINT('Ctrl Pts',(-0.14983202,2.85030975,-7.500774497));
#100399=CARTESIAN_POINT('Ctrl Pts',(-0.334222997,2.821428571,-7.492549298));
#100400=CARTESIAN_POINT('Ctrl Pts',(-0.560883377,2.785926731,-7.482438573));
#100401=CARTESIAN_POINT('Ctrl Pts',(-0.786518112,2.75,-7.45864527));
#100402=CARTESIAN_POINT('Ctrl Pts',(-0.790621385139384,2.74934665560115,
-7.45821257766166));
#100403=CARTESIAN_POINT('Ctrl Pts',(-0.794724658278769,2.7486933112023,
-7.45777988532332));
#100404=CARTESIAN_POINT('',(-0.891432874411234,2.75000000185138,-7.31992813361032));
#100405=CARTESIAN_POINT('Ctrl Pts',(-0.996347614,2.75,-7.181211));
#100406=CARTESIAN_POINT('Ctrl Pts',(-1.3854833,2.81435393,-7.127220885));
#100407=CARTESIAN_POINT('Ctrl Pts',(-1.766506299,2.879481221,-7.031497386));
#100408=CARTESIAN_POINT('Ctrl Pts',(-1.273781884,2.75,-7.391040503));
#100409=CARTESIAN_POINT('Ctrl Pts',(-1.674287817,2.81435393,-7.32201677));
#100410=CARTESIAN_POINT('Ctrl Pts',(-2.064989971,2.879481221,-7.210119029));
#100411=CARTESIAN_POINT('',(-1.27378189515849,2.75,-7.39104050096434));
#100412=CARTESIAN_POINT('',(-1.82461846250296,2.83963938428032,-7.27466614086713));
#100413=CARTESIAN_POINT('Origin',(0.0622612227616864,2.94636923860537,0.177968265673633));
#100414=CARTESIAN_POINT('Ctrl Pts',(-1.76195410140001,2.87870320274956,
-7.03263945744517));
#100415=CARTESIAN_POINT('Ctrl Pts',(-1.77234673711184,2.87185457193404,
-7.07292594060115));
#100416=CARTESIAN_POINT('Ctrl Pts',(-1.78277206917022,2.86518067054195,
-7.11326105058591));
#100417=CARTESIAN_POINT('Ctrl Pts',(-1.80365751908978,2.85217081132598,
-7.19392247482129));
#100418=CARTESIAN_POINT('Ctrl Pts',(-1.8141301492228,2.84582706796081,-7.23429710511575));
#100419=CARTESIAN_POINT('Ctrl Pts',(-1.82461846412333,2.83963938428433,
-7.27466614044675));
#100420=CARTESIAN_POINT('',(-1.13506476035904,2.74999999814853,-7.28612574973044));
#100421=CARTESIAN_POINT('Origin',(1.92337465398928E-13,2.84071505700033,
8.8557633448616E-13));
#100422=CARTESIAN_POINT('',(-1.82461846250295,2.66036061571968,-7.27466614086712));
#100423=CARTESIAN_POINT('Origin',(0.0622612227626687,2.55363076139464,0.177968265676951));
#100424=CARTESIAN_POINT('',(-2.3715180240997,2.75,-7.11518813898183));
#100425=CARTESIAN_POINT('Ctrl Pts',(-2.37151802375132,2.75000000173934,
-7.11518813880764));
#100426=CARTESIAN_POINT('Ctrl Pts',(-2.22766411164902,2.7259891821231,-7.16313516951371));
#100427=CARTESIAN_POINT('Ctrl Pts',(-2.08271441129929,2.70215892392426,
-7.20659588422854));
#100428=CARTESIAN_POINT('Ctrl Pts',(-1.93708566943587,2.67857142885868,
-7.24552959465705));
#100429=CARTESIAN_POINT('Ctrl Pts',(-1.89970445058239,2.67251679081792,
-7.25552342898784));
#100430=CARTESIAN_POINT('Ctrl Pts',(-1.86221328573061,2.66644617725889,
-7.26523667630949));
#100431=CARTESIAN_POINT('Ctrl Pts',(-1.82461846261757,2.66036061550997,
-7.27466614118873));
#100432=CARTESIAN_POINT('Ctrl Pts',(-1.82461846261757,2.83963938449003,
-7.27466614118873));
#100433=CARTESIAN_POINT('Ctrl Pts',(-1.86221328573062,2.83355382274111,
-7.2652366763095));
#100434=CARTESIAN_POINT('Ctrl Pts',(-1.89970445061032,2.8274832091563,-7.25552342919053));
#100435=CARTESIAN_POINT('Ctrl Pts',(-1.93708566943587,2.82142857114132,
-7.24552959465706));
#100436=CARTESIAN_POINT('Ctrl Pts',(-2.0827144111905,2.79784107617617,-7.20659588343893));
#100437=CARTESIAN_POINT('Ctrl Pts',(-2.22766411164898,2.77401081787672,
-7.16313516951369));
#100438=CARTESIAN_POINT('Ctrl Pts',(-2.37151802375131,2.74999999826065,
-7.11518813880763));
#100439=CARTESIAN_POINT('Ctrl Pts',(-1.75734327,2.879480225,-7.033793047));
#100440=CARTESIAN_POINT('Ctrl Pts',(-1.930444297,2.85030975,-6.990544984));
#100441=CARTESIAN_POINT('Ctrl Pts',(-2.1012084,2.821428571,-6.938834431));
#100442=CARTESIAN_POINT('Ctrl Pts',(-2.31111811,2.785926731,-6.875269858));
#100443=CARTESIAN_POINT('Ctrl Pts',(-2.516801651,2.75,-6.799132993));
#100444=CARTESIAN_POINT('Ctrl Pts',(-2.52054210234939,2.74934665560115,
-6.79774840851628));
#100445=CARTESIAN_POINT('Ctrl Pts',(-2.52428255369877,2.7486933112023,-6.79636382403254));
#100446=CARTESIAN_POINT('Ctrl Pts',(-1.578332876,2.879480225,-7.332043735));
#100447=CARTESIAN_POINT('Ctrl Pts',(-1.758773826,2.85030975,-7.29320110200001));
#100448=CARTESIAN_POINT('Ctrl Pts',(-1.93708567,2.821428571,-7.245529595));
#100449=CARTESIAN_POINT('Ctrl Pts',(-2.156273349,2.785926731,-7.18692997));
#100450=CARTESIAN_POINT('Ctrl Pts',(-2.371518013,2.75,-7.115188143));
#100451=CARTESIAN_POINT('Ctrl Pts',(-2.37543233784093,2.74934665560115,
-7.11388348433696));
#100452=CARTESIAN_POINT('Ctrl Pts',(-2.37934666268186,2.7486933112023,-7.11257882567393));
#100453=CARTESIAN_POINT('',(-2.44415984284571,2.75000000185138,-6.95716056418973));
#100454=CARTESIAN_POINT('Ctrl Pts',(-2.516801651,2.75,-6.799132993));
#100455=CARTESIAN_POINT('Ctrl Pts',(-2.885233281,2.81435393,-6.662752466));
#100456=CARTESIAN_POINT('Ctrl Pts',(-3.236770452,2.879481221,-6.487358248));
#100457=CARTESIAN_POINT('Ctrl Pts',(-2.832856802,2.75,-6.944416631));
#100458=CARTESIAN_POINT('Ctrl Pts',(-3.209161066,2.81435393,-6.79090969800001));
#100459=CARTESIAN_POINT('Ctrl Pts',(-3.566674115,2.879481221,-6.59763865));
#100460=CARTESIAN_POINT('',(-2.83285681245535,2.75,-6.94441662660179));
#100461=CARTESIAN_POINT('',(-3.34579807948844,2.83963938429423,-6.71234945516635));
#100462=CARTESIAN_POINT('Origin',(0.0990635273127888,2.94636920486568,0.16042320697258));
#100463=CARTESIAN_POINT('Ctrl Pts',(-3.23257019394498,2.8787032027684,-6.4894522063135));
#100464=CARTESIAN_POINT('Ctrl Pts',(-3.25138025846878,2.87185457193376,
-6.52656270441233));
#100465=CARTESIAN_POINT('Ctrl Pts',(-3.27023270836533,2.86518067053059,
-6.56371366377399));
#100466=CARTESIAN_POINT('Ctrl Pts',(-3.30796968985539,2.85217081132906,
-6.63799951434366));
#100467=CARTESIAN_POINT('Ctrl Pts',(-3.32687682777823,2.84582706796692,
-6.67517890235472));
#100468=CARTESIAN_POINT('Ctrl Pts',(-3.34579808097769,2.83963938429823,
-6.71234945440893));
#100469=CARTESIAN_POINT('',(-2.67482923721307,2.74999999814853,-6.87177480782995));
#100470=CARTESIAN_POINT('Origin',(-8.69530142333375E-14,2.84071505699933,
-1.02348685082632E-13));
#100471=CARTESIAN_POINT('',(-3.34579807948842,2.66036061570577,-6.71234945516632));
#100472=CARTESIAN_POINT('Origin',(0.0990635273070517,2.55363079513323,0.160423206958388));
#100473=CARTESIAN_POINT('',(-3.84562837697436,2.75,-6.43903272068618));
#100474=CARTESIAN_POINT('Ctrl Pts',(-3.84562837659874,2.75000000173934,
-6.43903272059439));
#100475=CARTESIAN_POINT('Ctrl Pts',(-3.71544488347682,2.72598918212305,
-6.51678311509396));
#100476=CARTESIAN_POINT('Ctrl Pts',(-3.58322679552254,2.70215892392445,
-6.5903876432404));
#100477=CARTESIAN_POINT('Ctrl Pts',(-3.44937236946746,2.67857142888618,
-6.6597169799323));
#100478=CARTESIAN_POINT('Ctrl Pts',(-3.41501348176197,2.67251679084659,
-6.67751302125371));
#100479=CARTESIAN_POINT('Ctrl Pts',(-3.38048690047503,2.66644617724843,
-6.69505867042727));
#100480=CARTESIAN_POINT('Ctrl Pts',(-3.34579807966921,2.66036061549648,
-6.71234945545536));
#100481=CARTESIAN_POINT('Ctrl Pts',(-3.34579807966923,2.83963938450351,
-6.7123494554554));
#100482=CARTESIAN_POINT('Ctrl Pts',(-3.38048690047503,2.83355382275157,
-6.69505867042736));
#100483=CARTESIAN_POINT('Ctrl Pts',(-3.41501348171708,2.82748320916218,
-6.67751302126219));
#100484=CARTESIAN_POINT('Ctrl Pts',(-3.44937236946741,2.82142857111382,
-6.65971697993242));
#100485=CARTESIAN_POINT('Ctrl Pts',(-3.58322679569734,2.79784107604138,
-6.59038764320792));
#100486=CARTESIAN_POINT('Ctrl Pts',(-3.71544488347676,2.77401081787677,
-6.51678311509403));
#100487=CARTESIAN_POINT('Ctrl Pts',(-3.84562837659873,2.74999999826065,
-6.43903272059438));
#100488=CARTESIAN_POINT('Ctrl Pts',(-3.22260332935241,2.88054032962933,
-6.49417280112119));
#100489=CARTESIAN_POINT('Ctrl Pts',(-3.38532999374888,2.85083482772692,
-6.41342294922764));
#100490=CARTESIAN_POINT('Ctrl Pts',(-3.54380823152172,2.821428571,-6.32462455818216));
#100491=CARTESIAN_POINT('Ctrl Pts',(-3.73513721104557,2.785926731,-6.21741926817495));
#100492=CARTESIAN_POINT('Ctrl Pts',(-3.91963602296178,2.75,-6.09884464776978));
#100493=CARTESIAN_POINT('Ctrl Pts',(-3.92436673545407,2.74907880688562,
-6.09580428977402));
#100494=CARTESIAN_POINT('Ctrl Pts',(-3.92909744794634,2.74815761377124,
-6.09276393177824));
#100495=CARTESIAN_POINT('Ctrl Pts',(-3.11150347067144,2.88054032962933,
-6.82411504555695));
#100496=CARTESIAN_POINT('Ctrl Pts',(-3.28249760950799,2.85083482772692,
-6.74614906006595));
#100497=CARTESIAN_POINT('Ctrl Pts',(-3.44937237,2.821428571,-6.65971698));
#100498=CARTESIAN_POINT('Ctrl Pts',(-3.650838376,2.785926731,-6.55536851));
#100499=CARTESIAN_POINT('Ctrl Pts',(-3.845628367,2.75,-6.439032727));
#100500=CARTESIAN_POINT('Ctrl Pts',(-3.85062295441346,2.74907880688562,
-6.43604977477271));
#100501=CARTESIAN_POINT('Ctrl Pts',(-3.85561754182692,2.74815761377124,
-6.43306682254543));
#100502=CARTESIAN_POINT('',(-3.88260061277304,2.75000000185138,-6.26908389894731));
#100503=CARTESIAN_POINT('Ctrl Pts',(-3.919572839,2.75,-6.099135083));
#100504=CARTESIAN_POINT('Ctrl Pts',(-4.250072961,2.81435393,-5.886741148));
#100505=CARTESIAN_POINT('Ctrl Pts',(-4.555686816,2.879481221,-5.63987744800001));
#100506=CARTESIAN_POINT('Ctrl Pts',(-4.259470484,2.75,-6.173079555));
#100507=CARTESIAN_POINT('Ctrl Pts',(-4.593977511,2.81435393,-5.942267236));
#100508=CARTESIAN_POINT('Ctrl Pts',(-4.901584541,2.879481221,-5.67666002));
#100509=CARTESIAN_POINT('',(-4.25947049338054,2.75,-6.17307954862385));
#100510=CARTESIAN_POINT('',(-4.71053189666572,2.83963938430234,-5.83617076883909));
#100511=CARTESIAN_POINT('Origin',(0.131233580395995,2.94636921249293,0.135376684318178));
#100512=CARTESIAN_POINT('Ctrl Pts',(-4.55203489665337,2.87870320274035,
-5.64282538217238));
#100513=CARTESIAN_POINT('Ctrl Pts',(-4.57838285257828,2.87185457192953,
-5.67502464964238));
#100514=CARTESIAN_POINT('Ctrl Pts',(-4.60478090062114,2.86518067054936,
-5.70725432072026));
#100515=CARTESIAN_POINT('Ctrl Pts',(-4.65760487443965,2.85217081131047,
-5.77169107409159));
#100516=CARTESIAN_POINT('Ctrl Pts',(-4.68406244312412,2.84582706798356,
-5.80393675270542));
#100517=CARTESIAN_POINT('Ctrl Pts',(-4.71053189794207,2.83963938430632,
-5.83617076779177));
#100518=CARTESIAN_POINT('',(-4.08952167106617,2.74999999814853,-6.13610731262445));
#100519=CARTESIAN_POINT('Origin',(-3.57786716920216E-13,2.84071505699989,
-4.45823933326039E-13));
#100520=CARTESIAN_POINT('',(-4.71053189666556,2.66036061569762,-5.83617076883885));
#100521=CARTESIAN_POINT('Origin',(0.131233580279342,2.55363078748444,0.135376684142551));
#100522=CARTESIAN_POINT('',(-5.1399214203484,2.75,-5.4617952896511));
#100523=CARTESIAN_POINT('Ctrl Pts',(-5.1399214199973,2.75000000173934,-5.46179528967991));
#100524=CARTESIAN_POINT('Ctrl Pts',(-5.02949558164935,2.72598918212305,
-5.56571352588234));
#100525=CARTESIAN_POINT('Ctrl Pts',(-4.91619147725867,2.70215892392415,
-5.66602020133334));
#100526=CARTESIAN_POINT('Ctrl Pts',(-4.80037025126701,2.67857142884375,
-5.76250340104977));
#100527=CARTESIAN_POINT('Ctrl Pts',(-4.77064027777155,2.67251679078282,
-5.78726952594611));
#100528=CARTESIAN_POINT('Ctrl Pts',(-4.74069270475776,2.66644617723471,
-5.81182716194082));
#100529=CARTESIAN_POINT('Ctrl Pts',(-4.71053189688486,2.66036061548689,
-5.83617076905788));
#100530=CARTESIAN_POINT('Ctrl Pts',(-4.71053189688485,2.83963938451312,
-5.83617076905789));
#100531=CARTESIAN_POINT('Ctrl Pts',(-4.7406927047578,2.83355382276527,-5.8118271619421));
#100532=CARTESIAN_POINT('Ctrl Pts',(-4.77064027797896,2.82748320917259,
-5.78726952596174));
#100533=CARTESIAN_POINT('Ctrl Pts',(-4.80037025126685,2.82142857115626,
-5.7625034010515));
#100534=CARTESIAN_POINT('Ctrl Pts',(-4.91619147645074,2.79784107624942,
-5.66602020128021));
#100535=CARTESIAN_POINT('Ctrl Pts',(-5.02949558164928,2.77401081787677,
-5.56571352588347));
#100536=CARTESIAN_POINT('Ctrl Pts',(-5.13992141999731,2.74999999826065,
-5.46179528967991));
#100537=CARTESIAN_POINT('Ctrl Pts',(-4.548334599,2.879480225,-5.64580839));
#100538=CARTESIAN_POINT('Ctrl Pts',(-4.687277446,2.85030975,-5.533874277));
#100539=CARTESIAN_POINT('Ctrl Pts',(-4.82054605,2.821428571,-5.415241063));
#100540=CARTESIAN_POINT('Ctrl Pts',(-4.984364872,2.785926731,-5.26941262000001));
#100541=CARTESIAN_POINT('Ctrl Pts',(-5.139069158,2.75,-5.113948395));
#100542=CARTESIAN_POINT('Ctrl Pts',(-5.14188252776459,2.74934665560115,
-5.11112120538942));
#100543=CARTESIAN_POINT('Ctrl Pts',(-5.14469589752919,2.7486933112023,-5.10829401577884));
#100544=CARTESIAN_POINT('Ctrl Pts',(-4.511101379,2.879480225,-5.991657896));
#100545=CARTESIAN_POINT('Ctrl Pts',(-4.658555551,2.85030975,-5.880640089));
#100546=CARTESIAN_POINT('Ctrl Pts',(-4.800370252,2.821428571,-5.762503401));
#100547=CARTESIAN_POINT('Ctrl Pts',(-4.974694258,2.785926731,-5.617285305));
#100548=CARTESIAN_POINT('Ctrl Pts',(-5.139921412,2.75,-5.461795298));
#100549=CARTESIAN_POINT('Ctrl Pts',(-5.14292614503858,2.74934665560115,
-5.4589676395317));
#100550=CARTESIAN_POINT('Ctrl Pts',(-5.14593087807715,2.7486933112023,-5.4561399810634));
#100551=CARTESIAN_POINT('',(-5.13949529324341,2.75000000185138,-5.2878718384879));
#100552=CARTESIAN_POINT('Ctrl Pts',(-5.139069158,2.75,-5.113948395));
#100553=CARTESIAN_POINT('Ctrl Pts',(-5.416183953,2.81435393,-4.83547235600001));
#100554=CARTESIAN_POINT('Ctrl Pts',(-5.661584328,2.879481221,-4.528682248));
#100555=CARTESIAN_POINT('Ctrl Pts',(-5.48691606,2.75,-5.113096141));
#100556=CARTESIAN_POINT('Ctrl Pts',(-5.763984674,2.81435393,-4.815770962));
#100557=CARTESIAN_POINT('Ctrl Pts',(-6.007302322,2.879481221,-4.490247077));
#100558=CARTESIAN_POINT('',(-5.48691606779505,2.75000000000002,-5.11309613274603));
#100559=CARTESIAN_POINT('',(-5.85500647817754,2.83963938428039,-4.68709922414167));
#100560=CARTESIAN_POINT('Origin',(0.157267369836855,2.94636927201175,0.104000280378761));
#100561=CARTESIAN_POINT('Ctrl Pts',(-5.6586515072673,2.87870320275799,-4.53234631572629));
#100562=CARTESIAN_POINT('Ctrl Pts',(-5.69130535301401,2.87185457194846,
-4.55812875035173));
#100563=CARTESIAN_POINT('Ctrl Pts',(-5.72401465585923,2.86518067057082,
-4.58393010943499));
#100564=CARTESIAN_POINT('Ctrl Pts',(-5.7894556316736,2.85217081134139,-4.63550477407209));
#100565=CARTESIAN_POINT('Ctrl Pts',(-5.82222650503423,2.84582706798315,
-4.66130897145861));
#100566=CARTESIAN_POINT('Ctrl Pts',(-5.85500647919594,2.83963938428437,
-4.68709922284821));
#100567=CARTESIAN_POINT('',(-5.31299261697924,2.74999999814684,-5.11352225970951));
#100568=CARTESIAN_POINT('Origin',(-2.55871712706579E-14,2.84071505700033,
2.47198095326695E-14));
#100569=CARTESIAN_POINT('',(-5.85500647817749,2.66036061571961,-4.68709922414165));
#100570=CARTESIAN_POINT('Origin',(0.157267369807963,2.55363072798491,0.104000280351224));
#100571=CARTESIAN_POINT('',(-6.19387745226799,2.75,-4.22917037999045));
#100572=CARTESIAN_POINT('Ctrl Pts',(-6.19387745202191,2.75000000173934,
-4.22917038015593));
#100573=CARTESIAN_POINT('Ctrl Pts',(-6.10837265719485,2.72598918212311,
-4.35439735677576));
#100574=CARTESIAN_POINT('Ctrl Pts',(-6.01928050973812,2.70215892392435,
-4.47671595142935));
#100575=CARTESIAN_POINT('Ctrl Pts',(-5.92690815539044,2.67857142887217,
-4.59584156796461));
#100576=CARTESIAN_POINT('Ctrl Pts',(-5.90319723703065,2.67251679082422,
-4.62641973990005));
#100577=CARTESIAN_POINT('Ctrl Pts',(-5.8792289873938,2.66644617724722,-4.65684107515696));
#100578=CARTESIAN_POINT('Ctrl Pts',(-5.85500647842804,2.66036061550761,
-4.68709922429958));
#100579=CARTESIAN_POINT('Ctrl Pts',(-5.85500647842804,2.83963938449239,
-4.68709922429957));
#100580=CARTESIAN_POINT('Ctrl Pts',(-5.87922898739386,2.83355382275278,
-4.65684107515717));
#100581=CARTESIAN_POINT('Ctrl Pts',(-5.90319723711639,2.82748320916694,
-4.6264197401748));
#100582=CARTESIAN_POINT('Ctrl Pts',(-5.92690815539048,2.82142857112784,
-4.59584156796493));
#100583=CARTESIAN_POINT('Ctrl Pts',(-6.01928050940444,2.79784107611009,
-4.47671595036035));
#100584=CARTESIAN_POINT('Ctrl Pts',(-6.10837265719485,2.77401081787671,
-4.35439735677597));
#100585=CARTESIAN_POINT('Ctrl Pts',(-6.1938774520219,2.74999999826065,-4.22917038015593));
#100586=CARTESIAN_POINT('Ctrl Pts',(-5.655678979,2.879480225,-4.536055036));
#100587=CARTESIAN_POINT('Ctrl Pts',(-5.767310893,2.85030975,-4.396869275));
#100588=CARTESIAN_POINT('Ctrl Pts',(-5.871961118,2.821428571,-4.25236083));
#100589=CARTESIAN_POINT('Ctrl Pts',(-6.000601142,2.785926731,-4.074725571));
#100590=CARTESIAN_POINT('Ctrl Pts',(-6.118268315,2.75,-3.889639164));
#100591=CARTESIAN_POINT('Ctrl Pts',(-6.12040814754998,2.74934665560115,
-3.88627328116149));
#100592=CARTESIAN_POINT('Ctrl Pts',(-6.12254798009995,2.7486933112023,-3.88290739832298));
#100593=CARTESIAN_POINT('Ctrl Pts',(-5.693663671,2.879480225,-4.881822815));
#100594=CARTESIAN_POINT('Ctrl Pts',(-5.8138049,2.85030975,-4.741702254));
#100595=CARTESIAN_POINT('Ctrl Pts',(-5.926908156,2.821428571,-4.595841568));
#100596=CARTESIAN_POINT('Ctrl Pts',(-6.06593896600001,2.785926731,-4.416544081));
#100597=CARTESIAN_POINT('Ctrl Pts',(-6.193877446,2.75,-4.22917039));
#100598=CARTESIAN_POINT('Ctrl Pts',(-6.19620406706957,2.74934665560115,
-4.22576291183265));
#100599=CARTESIAN_POINT('Ctrl Pts',(-6.19853068813914,2.7486933112023,-4.22235543366531));
#100600=CARTESIAN_POINT('',(-6.15607288682832,2.75000000185138,-4.05940476740313));
#100601=CARTESIAN_POINT('Ctrl Pts',(-6.118268315,2.75,-3.889639164));
#100602=CARTESIAN_POINT('Ctrl Pts',(-6.32904020300001,2.81435393,-3.55810225));
#100603=CARTESIAN_POINT('Ctrl Pts',(-6.502752449,2.879481221,-3.205730898));
#100604=CARTESIAN_POINT('Ctrl Pts',(-6.45779954,2.75,-3.814030034));
#100605=CARTESIAN_POINT('Ctrl Pts',(-6.664474319,2.81435393,-3.464094591));
#100606=CARTESIAN_POINT('Ctrl Pts',(-6.832125323,2.879481221,-3.093875171));
#100607=CARTESIAN_POINT('',(-6.45779954578553,2.75,-3.81403002424441));
#100608=CARTESIAN_POINT('',(-6.72570746383011,2.83963938432043,-3.31886412904555));
#100609=CARTESIAN_POINT('Origin',(0.175947461605686,2.94636924508285,0.067760940793829));
#100610=CARTESIAN_POINT('Ctrl Pts',(-6.50067586214128,2.8787032027215,-3.20993977181558));
#100611=CARTESIAN_POINT('Ctrl Pts',(-6.53810874055978,2.87185457190171,
-3.22809981590397));
#100612=CARTESIAN_POINT('Ctrl Pts',(-6.57559984766339,2.86518067052256,
-3.24626642040999));
#100613=CARTESIAN_POINT('Ctrl Pts',(-6.65059787826818,2.85217081130526,
-3.28256742285789));
#100614=CARTESIAN_POINT('Ctrl Pts',(-6.68814972626432,2.84582706800102,
-3.30072356335558));
#100615=CARTESIAN_POINT('Ctrl Pts',(-6.72570746453642,2.83963938432441,
-3.31886412758459));
#100616=CARTESIAN_POINT('',(-6.288033933505,2.74999999814853,-3.85183458919698));
#100617=CARTESIAN_POINT('Origin',(-1.03302782994419E-12,2.84071505699978,
-5.41450564939261E-13));
#100618=CARTESIAN_POINT('',(-6.7257074638301,2.66036061567957,-3.31886412904556));
#100619=CARTESIAN_POINT('Origin',(0.175947461606183,2.55363075491703,0.0677609407940782));
#100620=CARTESIAN_POINT('',(-6.95821465711167,2.75,-2.79879416493425));
#100621=CARTESIAN_POINT('Ctrl Pts',(-6.958214656765,2.75000000173934,-2.79879416509168));
#100622=CARTESIAN_POINT('Ctrl Pts',(-6.9016290152138,2.72598918212306,-2.93947440757433));
#100623=CARTESIAN_POINT('Ctrl Pts',(-6.84091467506888,2.70215892392413,
-3.07808543914549));
#100624=CARTESIAN_POINT('Ctrl Pts',(-6.77631042134925,2.67857142884028,
-3.21428329038083));
#100625=CARTESIAN_POINT('Ctrl Pts',(-6.7597272540588,2.67251679076156,-3.24924370862982));
#100626=CARTESIAN_POINT('Ctrl Pts',(-6.74285905662865,2.66644617720877,
-3.28410627512915));
#100627=CARTESIAN_POINT('Ctrl Pts',(-6.72570746404163,2.66036061546033,
-3.31886412911155));
#100628=CARTESIAN_POINT('Ctrl Pts',(-6.72570746404163,2.83963938453967,
-3.31886412911154));
#100629=CARTESIAN_POINT('Ctrl Pts',(-6.74285905662865,2.83355382279123,
-3.28410627512915));
#100630=CARTESIAN_POINT('Ctrl Pts',(-6.75972725426173,2.82748320918954,
-3.24924370852248));
#100631=CARTESIAN_POINT('Ctrl Pts',(-6.77631042134924,2.82142857115972,
-3.21428329038083));
#100632=CARTESIAN_POINT('Ctrl Pts',(-6.84091467427833,2.79784107626641,
-3.07808543956365));
#100633=CARTESIAN_POINT('Ctrl Pts',(-6.90162901521376,2.77401081787676,
-2.93947440757435));
#100634=CARTESIAN_POINT('Ctrl Pts',(-6.958214656765,2.74999999826065,-2.79879416509168));
#100635=CARTESIAN_POINT('Ctrl Pts',(-6.498570095,2.879480225,-3.21420079));
#100636=CARTESIAN_POINT('Ctrl Pts',(-6.577671293,2.85030975,-3.054271554));
#100637=CARTESIAN_POINT('Ctrl Pts',(-6.64880981,2.821428571,-2.890644931));
#100638=CARTESIAN_POINT('Ctrl Pts',(-6.736255972,2.785926731,-2.689508882));
#100639=CARTESIAN_POINT('Ctrl Pts',(-6.811384045,2.75,-2.483454729));
#100640=CARTESIAN_POINT('Ctrl Pts',(-6.81275028412961,2.74934665560115,
-2.47970753789814));
#100641=CARTESIAN_POINT('Ctrl Pts',(-6.81411652325921,2.7486933112023,-2.47596034679627));
#100642=CARTESIAN_POINT('Ctrl Pts',(-6.609996578,2.879480225,-3.543719125));
#100643=CARTESIAN_POINT('Ctrl Pts',(-6.69720719300001,2.85030975,-3.381047692));
#100644=CARTESIAN_POINT('Ctrl Pts',(-6.776310422,2.821428571,-3.21428329));
#100645=CARTESIAN_POINT('Ctrl Pts',(-6.87354710900001,2.785926731,-3.009290165));
#100646=CARTESIAN_POINT('Ctrl Pts',(-6.958214653,2.75,-2.798794176));
#100647=CARTESIAN_POINT('Ctrl Pts',(-6.9597543718694,2.74934665560115,-2.79496620803394));
#100648=CARTESIAN_POINT('Ctrl Pts',(-6.96129409073881,2.7486933112023,-2.79113824006787));
#100649=CARTESIAN_POINT('',(-6.88479935311732,2.75000000185138,-2.6411244417671));
#100650=CARTESIAN_POINT('Ctrl Pts',(-6.811384045,2.75,-2.483454729));
#100651=CARTESIAN_POINT('Ctrl Pts',(-6.945957567,2.81435393,-2.114359238));
#100652=CARTESIAN_POINT('Ctrl Pts',(-7.039859092,2.879481221,-1.732883135));
#100653=CARTESIAN_POINT('Ctrl Pts',(-7.12672349100001,2.75,-2.336624121));
#100654=CARTESIAN_POINT('Ctrl Pts',(-7.253340552,2.81435393,-1.950441006));
#100655=CARTESIAN_POINT('Ctrl Pts',(-7.33748573700001,2.879481221,-1.5528371));
#100656=CARTESIAN_POINT('',(-7.12672349453342,2.75,-2.33662411022232));
#100657=CARTESIAN_POINT('',(-7.28192184370656,2.83963938427376,-1.79544263556377));
#100658=CARTESIAN_POINT('Origin',(0.186400573970105,2.94636923522301,0.0283532430203706));
#100659=CARTESIAN_POINT('Ctrl Pts',(-7.03873583813264,2.87870320277747,
-1.73744001214091));
#100660=CARTESIAN_POINT('Ctrl Pts',(-7.07919742953855,2.87185457196145,
-1.74712852185622));
#100661=CARTESIAN_POINT('Ctrl Pts',(-7.11971729855279,2.86518067056953,
-1.75681092128746));
#100662=CARTESIAN_POINT('Ctrl Pts',(-7.20076555952284,2.85217081132604,
-1.7761408666784));
#100663=CARTESIAN_POINT('Ctrl Pts',(-7.24134249982081,2.84582706798385,
-1.78579998946225));
#100664=CARTESIAN_POINT('Ctrl Pts',(-7.28192184408587,2.83963938427774,
-1.79544263397008));
#100665=CARTESIAN_POINT('',(-6.96905377175724,2.74999999814853,-2.41003941413528));
#100666=CARTESIAN_POINT('Origin',(2.18575157973078E-13,2.84071505699989,
8.64109131470947E-14));
#100667=CARTESIAN_POINT('',(-7.28192184370656,2.66036061572624,-1.79544263556378));
#100668=CARTESIAN_POINT('Origin',(0.18640057397059,2.55363076477878,0.0283532430206035));
#100669=CARTESIAN_POINT('',(-7.3971934794137,2.75,-1.23754944427177));
#100670=CARTESIAN_POINT('Ctrl Pts',(-7.39719347933202,2.75000000173934,
-1.23754944453735));
#100671=CARTESIAN_POINT('Ctrl Pts',(-7.37217287192558,2.72598918212305,
-1.38710490209901));
#100672=CARTESIAN_POINT('Ctrl Pts',(-7.34267527326005,2.70215892392471,
-1.53552707352338));
#100673=CARTESIAN_POINT('Ctrl Pts',(-7.30885994283025,2.67857142892459,
-1.682428699378));
#100674=CARTESIAN_POINT('Ctrl Pts',(-7.30017993773283,2.67251679088925,
-1.7201366528899));
#100675=CARTESIAN_POINT('Ctrl Pts',(-7.29120053043776,2.66644617724762,
-1.75781031566047));
#100676=CARTESIAN_POINT('Ctrl Pts',(-7.28192184397542,2.66036061551178,
-1.79544263559539));
#100677=CARTESIAN_POINT('Ctrl Pts',(-7.28192184397542,2.83963938448822,
-1.79544263559538));
#100678=CARTESIAN_POINT('Ctrl Pts',(-7.29120053043776,2.83355382275238,
-1.75781031566047));
#100679=CARTESIAN_POINT('Ctrl Pts',(-7.30017993742646,2.82748320916779,
-1.72013665290894));
#100680=CARTESIAN_POINT('Ctrl Pts',(-7.30885994269999,2.82142857107541,
-1.68242869918427));
#100681=CARTESIAN_POINT('Ctrl Pts',(-7.34267527381588,2.79784107585308,
-1.53552707250072));
#100682=CARTESIAN_POINT('Ctrl Pts',(-7.37217287192555,2.77401081787677,
-1.38710490209903));
#100683=CARTESIAN_POINT('Ctrl Pts',(-7.39719347933202,2.74999999826065,
-1.23754944453735));
#100684=CARTESIAN_POINT('Ctrl Pts',(-7.037595296,2.879480225,-1.742054088));
#100685=CARTESIAN_POINT('Ctrl Pts',(-7.080467094,2.85030975,-1.568859488));
#100686=CARTESIAN_POINT('Ctrl Pts',(-7.114767544,2.821428571,-1.393765687));
#100687=CARTESIAN_POINT('Ctrl Pts',(-7.156930959,2.785926731,-1.178533747));
#100688=CARTESIAN_POINT('Ctrl Pts',(-7.186007028,2.75,-0.961146711));
#100689=CARTESIAN_POINT('Ctrl Pts',(-7.18653578990772,2.74934665560115,
-0.9571934261227));
#100690=CARTESIAN_POINT('Ctrl Pts',(-7.18706455181544,2.7486933112023,-0.953240141245399));
#100691=CARTESIAN_POINT('Ctrl Pts',(-7.217253392,2.879480225,-2.039915067));
#100692=CARTESIAN_POINT('Ctrl Pts',(-7.26745552200001,2.85030975,-1.862299097));
#100693=CARTESIAN_POINT('Ctrl Pts',(-7.308859943,2.821428571,-1.682428699));
#100694=CARTESIAN_POINT('Ctrl Pts',(-7.359755829,2.785926731,-1.461325186));
#100695=CARTESIAN_POINT('Ctrl Pts',(-7.39719347800001,2.75,-1.237549456));
#100696=CARTESIAN_POINT('Ctrl Pts',(-7.39787429914903,2.74934665560115,
-1.23347998973562));
#100697=CARTESIAN_POINT('Ctrl Pts',(-7.39855512029806,2.7486933112023,-1.22941052347124));
#100698=CARTESIAN_POINT('',(-7.2916002547138,2.75000000185138,-1.09934807213293));
#100699=CARTESIAN_POINT('Ctrl Pts',(-7.186007028,2.75,-0.961146711));
#100700=CARTESIAN_POINT('Ctrl Pts',(-7.238089675,2.81435393,-0.571751139));
#100701=CARTESIAN_POINT('Ctrl Pts',(-7.247789749,2.879481221,-0.179007682));
#100702=CARTESIAN_POINT('Ctrl Pts',(-7.462409772,2.75,-0.749960261));
#100703=CARTESIAN_POINT('Ctrl Pts',(-7.503048642,2.81435393,-0.345586968));
#100704=CARTESIAN_POINT('Ctrl Pts',(-7.499753473,2.879481221,0.060809907));
#100705=CARTESIAN_POINT('',(-7.46240977317129,2.75,-0.749960249718469));
#100706=CARTESIAN_POINT('',(-7.49764165152831,2.83963938428599,-0.188068240164113));
#100707=CARTESIAN_POINT('Origin',(0.18813789085566,2.94636921308583,-0.0123802379614946));
#100708=CARTESIAN_POINT('Ctrl Pts',(-7.24767235005792,2.87870320272657,
-0.183699488584397));
#100709=CARTESIAN_POINT('Ctrl Pts',(-7.28927071525243,2.87185457192322,
-0.184463440225009));
#100710=CARTESIAN_POINT('Ctrl Pts',(-7.33092468187684,2.86518067054497,
-0.185208896527471));
#100711=CARTESIAN_POINT('Ctrl Pts',(-7.41423344644177,2.85217081131025,
-0.186663938230128));
#100712=CARTESIAN_POINT('Ctrl Pts',(-7.45593814635207,2.84582706796522,
-0.187374393336462));
#100713=CARTESIAN_POINT('Ctrl Pts',(-7.49764165155662,2.83963938428999,
-0.188068238498512));
#100714=CARTESIAN_POINT('',(-7.32420840133381,2.74999999814853,-0.855553474581588));
#100715=CARTESIAN_POINT('Origin',(6.61363325216158E-13,2.84071505700056,
8.93111539584934E-14));
#100716=CARTESIAN_POINT('',(-7.49764165152831,2.66036061571401,-0.188068240164119));
#100717=CARTESIAN_POINT('Origin',(0.188137890860158,2.55363078691417,-0.0123802379614915));
#100718=CARTESIAN_POINT('',(-7.49028775502938,2.75,0.381561712766595));
#100719=CARTESIAN_POINT('Ctrl Pts',(-7.49028775483674,2.75000000173934,
0.381561712481001));
#100720=CARTESIAN_POINT('Ctrl Pts',(-7.49800211813204,2.72598918212311,
0.230124087868946));
#100721=CARTESIAN_POINT('Ctrl Pts',(-7.50110053690817,2.70215892392423,
0.0788308326963932));
#100722=CARTESIAN_POINT('Ctrl Pts',(-7.49965529763164,2.67857142885476,
-0.0719056115850236));
#100723=CARTESIAN_POINT('Ctrl Pts',(-7.49928432131415,2.67251679080789,
-0.110597918899535));
#100724=CARTESIAN_POINT('Ctrl Pts',(-7.4986135715597,2.66644617725217,-0.149321099433654));
#100725=CARTESIAN_POINT('Ctrl Pts',(-7.49764165186744,2.66036061550535,
-0.188068240139857));
#100726=CARTESIAN_POINT('Ctrl Pts',(-7.49764165186744,2.83963938449465,
-0.188068240139847));
#100727=CARTESIAN_POINT('Ctrl Pts',(-7.49861357155971,2.83355382274783,
-0.149321099433649));
#100728=CARTESIAN_POINT('Ctrl Pts',(-7.4992843213749,2.8274832091614,-0.110597918759457));
#100729=CARTESIAN_POINT('Ctrl Pts',(-7.49965529763164,2.82142857114524,
-0.0719056115850307));
#100730=CARTESIAN_POINT('Ctrl Pts',(-7.50110053667153,2.79784107619542,
0.0788308321506787));
#100731=CARTESIAN_POINT('Ctrl Pts',(-7.49800211813201,2.77401081787671,
0.230124087868916));
#100732=CARTESIAN_POINT('Ctrl Pts',(-7.49028775483674,2.74999999826065,
0.381561712481007));
#100733=CARTESIAN_POINT('Ctrl Pts',(-7.247550363,2.879480225,-0.188450873));
#100734=CARTESIAN_POINT('Ctrl Pts',(-7.252188123,2.85030975,-0.010089297));
#100735=CARTESIAN_POINT('Ctrl Pts',(-7.248046656,2.821428571,0.168284491));
#100736=CARTESIAN_POINT('Ctrl Pts',(-7.242955809,2.785926731,0.387548315));
#100737=CARTESIAN_POINT('Ctrl Pts',(-7.224620308,2.75,0.606103459));
#100738=CARTESIAN_POINT('Ctrl Pts',(-7.22428686834254,2.74934665560115,
0.610077986467366));
#100739=CARTESIAN_POINT('Ctrl Pts',(-7.22395342868507,2.7486933112023,0.614052513934733));
#100740=CARTESIAN_POINT('Ctrl Pts',(-7.487039458,2.879480225,-0.440726847));
#100741=CARTESIAN_POINT('Ctrl Pts',(-7.497885707,2.85030975,-0.256471467));
#100742=CARTESIAN_POINT('Ctrl Pts',(-7.499655298,2.821428571,-0.071905611));
#100743=CARTESIAN_POINT('Ctrl Pts',(-7.501830546,2.785926731,0.154969736));
#100744=CARTESIAN_POINT('Ctrl Pts',(-7.490287756,2.75,0.381561701));
#100745=CARTESIAN_POINT('Ctrl Pts',(-7.49007784496764,2.74934665560115,
0.385682381814436));
#100746=CARTESIAN_POINT('Ctrl Pts',(-7.48986793393528,2.7486933112023,0.389803062628871));
#100747=CARTESIAN_POINT('',(-7.35745403123015,2.75000000185138,0.493832591469735));
#100748=CARTESIAN_POINT('Ctrl Pts',(-7.224620308,2.75,0.606103459));
#100749=CARTESIAN_POINT('Ctrl Pts',(-7.19177675500001,2.81435393,0.997591409));
#100750=CARTESIAN_POINT('Ctrl Pts',(-7.116821813,2.879481221,1.383237971));
#100751=CARTESIAN_POINT('Ctrl Pts',(-7.44916206600001,2.75,0.871770907));
#100752=CARTESIAN_POINT('Ctrl Pts',(-7.401922517,2.81435393,1.275426333));
#100753=CARTESIAN_POINT('Ctrl Pts',(-7.311341072,2.879481221,1.671613511));
#100754=CARTESIAN_POINT('',(-7.4491620646855,2.75,0.871770918265686));
#100755=CARTESIAN_POINT('',(-7.36278006843227,2.83963938429796,1.4281000172255));
#100756=CARTESIAN_POINT('Origin',(0.181077865154473,2.94636922108518,-0.052534871448249));
#100757=CARTESIAN_POINT('Ctrl Pts',(-7.11771575851598,2.87870320271664,
1.37863061888998));
#100758=CARTESIAN_POINT('Ctrl Pts',(-7.15850580391357,2.87185457189991,
1.38682694679702));
#100759=CARTESIAN_POINT('Ctrl Pts',(-7.1993461750297,2.86518067050694,1.39505329048376));
#100760=CARTESIAN_POINT('Ctrl Pts',(-7.28102001766141,2.85217081130069,
1.41154118876166));
#100761=CARTESIAN_POINT('Ctrl Pts',(-7.32190241154598,2.84582706797934,
1.41981262145295));
#100762=CARTESIAN_POINT('Ctrl Pts',(-7.36278006810718,2.83963938430194,
1.428100018832));
#100763=CARTESIAN_POINT('',(-7.33689118584801,2.74999999814853,0.738937194438185));
#100764=CARTESIAN_POINT('Origin',(1.19479079407903E-12,2.84071505700056,
-3.3957212042246E-13));
#100765=CARTESIAN_POINT('',(-7.36278006843227,2.66036061570204,1.4281000172255));
#100766=CARTESIAN_POINT('Origin',(0.181077865154028,2.5536307789163,-0.0525348714478818));
#100767=CARTESIAN_POINT('',(-7.23314450045272,2.75,1.98283146826368));
#100768=CARTESIAN_POINT('Ctrl Pts',(-7.23314450039587,2.75000000173934,
1.98283146796251));
#100769=CARTESIAN_POINT('Ctrl Pts',(-7.27323311869183,2.72598918212307,
1.83659273035069));
#100770=CARTESIAN_POINT('Ctrl Pts',(-7.30878267557167,2.70215892392438,
1.68950269573436));
#100771=CARTESIAN_POINT('Ctrl Pts',(-7.33977510491094,2.67857142887669,
1.54197970238118));
#100772=CARTESIAN_POINT('Ctrl Pts',(-7.34773050433874,2.67251679082118,
1.50411225081318));
#100773=CARTESIAN_POINT('Ctrl Pts',(-7.35539977549778,2.66644617723181,
1.46615020532329));
#100774=CARTESIAN_POINT('Ctrl Pts',(-7.36278006869151,2.66036061548774,
1.42810001731005));
#100775=CARTESIAN_POINT('Ctrl Pts',(-7.36278006869151,2.83963938451226,
1.42810001731005));
#100776=CARTESIAN_POINT('Ctrl Pts',(-7.35539977549778,2.83355382276819,
1.4661502053233));
#100777=CARTESIAN_POINT('Ctrl Pts',(-7.34773050418597,2.82748320917567,
1.50411225092341));
#100778=CARTESIAN_POINT('Ctrl Pts',(-7.33977510486803,2.82142857112331,
1.54197970240722));
#100779=CARTESIAN_POINT('Ctrl Pts',(-7.30878267595674,2.7978410760879,1.68950269543247));
#100780=CARTESIAN_POINT('Ctrl Pts',(-7.27323311869181,2.77401081787675,
1.83659273035066));
#100781=CARTESIAN_POINT('Ctrl Pts',(-7.23314450039587,2.74999999826065,
1.98283146796251));
#100782=CARTESIAN_POINT('Ctrl Pts',(-7.11959786607701,2.88054032779396,
1.36776416485828));
#100783=CARTESIAN_POINT('Ctrl Pts',(-7.08532534214618,2.8508348268179,1.54616231001887));
#100784=CARTESIAN_POINT('Ctrl Pts',(-7.04216107449507,2.821428571,1.72262009544759));
#100785=CARTESIAN_POINT('Ctrl Pts',(-6.99004934207468,2.785926731,1.93565558493594));
#100786=CARTESIAN_POINT('Ctrl Pts',(-6.92515542781633,2.75,2.145151485466));
#100787=CARTESIAN_POINT('Ctrl Pts',(-6.92349149172195,2.74907880754079,
2.15052314156808));
#100788=CARTESIAN_POINT('Ctrl Pts',(-6.92182755562759,2.74815761508157,
2.15589479767016));
#100789=CARTESIAN_POINT('Ctrl Pts',(-7.40779135236163,2.88054032779396,
1.17244499782585));
#100790=CARTESIAN_POINT('Ctrl Pts',(-7.37841300668275,2.8508348268179,1.35806450323592));
#100791=CARTESIAN_POINT('Ctrl Pts',(-7.339775105,2.821428571,1.541979703));
#100792=CARTESIAN_POINT('Ctrl Pts',(-7.293128004,2.785926731,1.764018444));
#100793=CARTESIAN_POINT('Ctrl Pts',(-7.233144504,2.75,1.982831457));
#100794=CARTESIAN_POINT('Ctrl Pts',(-7.23160647517469,2.74907880754079,
1.98844201192505));
#100795=CARTESIAN_POINT('Ctrl Pts',(-7.23006844634938,2.74815761508157,
1.9940525668501));
#100796=CARTESIAN_POINT('',(-7.0792814352825,2.75000000185138,2.06392219203608));
#100797=CARTESIAN_POINT('Ctrl Pts',(-6.925418373,2.75,2.145012905));
#100798=CARTESIAN_POINT('Ctrl Pts',(-6.809184347,2.81435393,2.520287691));
#100799=CARTESIAN_POINT('Ctrl Pts',(-6.653079198,2.879481221,2.880804954));
#100800=CARTESIAN_POINT('Ctrl Pts',(-7.087599821,2.75,2.452739036));
#100801=CARTESIAN_POINT('Ctrl Pts',(-6.954690722,2.81435393,2.836802116));
#100802=CARTESIAN_POINT('Ctrl Pts',(-6.781058488,2.879481221,3.204254325));
#100803=CARTESIAN_POINT('',(-7.08759981726226,2.75,2.45273904670858));
#100804=CARTESIAN_POINT('',(-6.88364307283612,2.83963938426474,2.97749190505679));
#100805=CARTESIAN_POINT('Origin',(0.165550829136227,2.94636919898514,-0.0902329832633514));
#100806=CARTESIAN_POINT('Ctrl Pts',(-6.65494268792754,2.8787032027829,2.87649749144771));
#100807=CARTESIAN_POINT('Ctrl Pts',(-6.69301711670703,2.87185457193056,
2.89327084769831));
#100808=CARTESIAN_POINT('Ctrl Pts',(-6.73113424203585,2.86518067051512,
2.91008433647982));
#100809=CARTESIAN_POINT('Ctrl Pts',(-6.8073541850895,2.85217081127456,2.94374421864197));
#100810=CARTESIAN_POINT('Ctrl Pts',(-6.84550265796655,2.84582706793118,
2.96061077606773));
#100811=CARTESIAN_POINT('Ctrl Pts',(-6.8836430721632,2.83963938426872,2.97749190657861));
#100812=CARTESIAN_POINT('',(-7.00650909341606,2.74999999814853,2.29887598142312));
#100813=CARTESIAN_POINT('Origin',(-1.346145417358E-12,2.84071505700011,
5.42317926677249E-13));
#100814=CARTESIAN_POINT('',(-6.88364307283612,2.66036061573526,2.97749190505678));
#100815=CARTESIAN_POINT('Origin',(0.165550829137875,2.55363080101485,-0.090232983264088));
#100816=CARTESIAN_POINT('',(-6.63778744815122,2.75,3.49138622725718));
#100817=CARTESIAN_POINT('Ctrl Pts',(-6.63778744812353,2.75000000173934,
3.49138622693142));
#100818=CARTESIAN_POINT('Ctrl Pts',(-6.708375822714,2.72598918212332,3.35718433829753));
#100819=CARTESIAN_POINT('Ctrl Pts',(-6.77471426039344,2.70215892392423,
3.22117529108411));
#100820=CARTESIAN_POINT('Ctrl Pts',(-6.83669518688489,2.67857142885406,
3.08376375931997));
#100821=CARTESIAN_POINT('Ctrl Pts',(-6.85260497599632,2.67251679081341,
3.04849180343724));
#100822=CARTESIAN_POINT('Ctrl Pts',(-6.86825566148464,2.66644617726573,
3.0130659561535));
#100823=CARTESIAN_POINT('Ctrl Pts',(-6.8836430731335,2.66036061552687,2.97749190522106));
#100824=CARTESIAN_POINT('Ctrl Pts',(-6.8836430731335,2.83963938447313,2.97749190522107));
#100825=CARTESIAN_POINT('Ctrl Pts',(-6.86825566148464,2.83355382273427,
3.01306595615351));
#100826=CARTESIAN_POINT('Ctrl Pts',(-6.85260497602587,2.82748320915501,
3.04849180358285));
#100827=CARTESIAN_POINT('Ctrl Pts',(-6.83669518688489,2.82142857114594,
3.08376375931997));
#100828=CARTESIAN_POINT('Ctrl Pts',(-6.77471426027832,2.79784107619884,
3.22117529051684));
#100829=CARTESIAN_POINT('Ctrl Pts',(-6.708375822714,2.77401081787672,3.35718433829754));
#100830=CARTESIAN_POINT('Ctrl Pts',(-6.63778744812352,2.74999999826066,
3.49138622693142));
#100831=CARTESIAN_POINT('Ctrl Pts',(-6.65911676148846,2.88054032844669,
2.86628968296735));
#100832=CARTESIAN_POINT('Ctrl Pts',(-6.58729518161321,2.85083482714118,
3.03314940069317));
#100833=CARTESIAN_POINT('Ctrl Pts',(-6.50720686179461,2.821428571,3.19620266055702));
#100834=CARTESIAN_POINT('Ctrl Pts',(-6.41051713982161,2.785926731,3.39305501682207));
#100835=CARTESIAN_POINT('Ctrl Pts',(-6.30210498255076,2.75,3.58370274611001));
#100836=CARTESIAN_POINT('Ctrl Pts',(-6.2993252004271,2.7490788073302,3.58859111991541));
#100837=CARTESIAN_POINT('Ctrl Pts',(-6.29654541830346,2.7481576146604,3.59347949372081));
#100838=CARTESIAN_POINT('Ctrl Pts',(-6.98256029174724,2.88054032844669,
2.73749004926488));
#100839=CARTESIAN_POINT('Ctrl Pts',(-6.91396608765727,2.85083482714118,
2.91245439970453));
#100840=CARTESIAN_POINT('Ctrl Pts',(-6.836695187,2.821428571,3.08376376));
#100841=CARTESIAN_POINT('Ctrl Pts',(-6.74340690300001,2.785926731,3.290583611));
#100842=CARTESIAN_POINT('Ctrl Pts',(-6.637787454,2.75,3.491386217));
#100843=CARTESIAN_POINT('Ctrl Pts',(-6.63507927934845,2.7490788073302,3.49653497068772));
#100844=CARTESIAN_POINT('Ctrl Pts',(-6.63237110469693,2.7481576146604,3.50168372437542));
#100845=CARTESIAN_POINT('',(-6.47008950698529,2.75000000185139,3.53750508408639));
#100846=CARTESIAN_POINT('Ctrl Pts',(-6.302391571,2.75,3.583623931));
#100847=CARTESIAN_POINT('Ctrl Pts',(-6.108202046,2.81435393,3.925138122));
#100848=CARTESIAN_POINT('Ctrl Pts',(-5.878245994,2.879481221,4.243668699));
#100849=CARTESIAN_POINT('Ctrl Pts',(-6.39462928600001,2.75,3.919019814));
#100850=CARTESIAN_POINT('Ctrl Pts',(-6.182265318,2.81435393,4.265532185));
#100851=CARTESIAN_POINT('Ctrl Pts',(-5.933701147,2.879481221,4.587067767));
#100852=CARTESIAN_POINT('',(-6.39462927992378,2.75,3.91901982357883));
#100853=CARTESIAN_POINT('',(-6.0826345771943,2.8396393843766,4.38765957983895));
#100854=CARTESIAN_POINT('Origin',(0.142282719380422,2.94636928188172,-0.123711824272659));
#100855=CARTESIAN_POINT('Ctrl Pts',(-5.88099189386276,2.87870320273351,
4.23986253753841));
#100856=CARTESIAN_POINT('Ctrl Pts',(-5.91457038781333,2.87185457194718,
4.2644286186552));
#100857=CARTESIAN_POINT('Ctrl Pts',(-5.94818195278064,2.86518067058278,
4.2890430724903));
#100858=CARTESIAN_POINT('Ctrl Pts',(-6.01538403650056,2.85217081134544,
4.33830103996495));
#100859=CARTESIAN_POINT('Ctrl Pts',(-6.04901480760903,2.84582706809447,
4.36297406019775));
#100860=CARTESIAN_POINT('Ctrl Pts',(-6.08263457640376,2.83963938437968,
4.38765958091638));
#100861=CARTESIAN_POINT('',(-6.34851042265171,2.74999999814853,3.75132188239731));
#100862=CARTESIAN_POINT('Ctrl Pts',(-5.8872627585203,2.8805403289085,4.23079068185782));
#100863=CARTESIAN_POINT('Ctrl Pts',(-5.78125041957623,2.85083482736991,
4.37830979712559));
#100864=CARTESIAN_POINT('Ctrl Pts',(-5.66798288841052,2.821428571,4.52033434203316));
#100865=CARTESIAN_POINT('Ctrl Pts',(-5.53123628067281,2.785926731,4.69179896798155));
#100866=CARTESIAN_POINT('Ctrl Pts',(-5.38437511387682,2.75,4.85468405041332));
#100867=CARTESIAN_POINT('Ctrl Pts',(-5.38060946525645,2.74907880723015,
4.85886056622971));
#100868=CARTESIAN_POINT('Ctrl Pts',(-5.37684381663609,2.7481576144603,4.8630370820461));
#100869=CARTESIAN_POINT('Ctrl Pts',(-6.23083247311669,2.8805403289085,4.17453311033498));
#100870=CARTESIAN_POINT('Ctrl Pts',(-6.12622979866047,2.85083482736991,
4.33066116654239));
#100871=CARTESIAN_POINT('Ctrl Pts',(-6.013939,2.821428571,4.48135445));
#100872=CARTESIAN_POINT('Ctrl Pts',(-5.87837158900001,2.785926731,4.663284745));
#100873=CARTESIAN_POINT('Ctrl Pts',(-5.73205484,2.75,4.836687639));
#100874=CARTESIAN_POINT('Ctrl Pts',(-5.72830315072755,2.74907880723015,
4.84113384069378));
#100875=CARTESIAN_POINT('Ctrl Pts',(-5.72455146145511,2.7481576144603,4.84558004238754));
#100876=CARTESIAN_POINT('',(-5.73205483199695,2.75,4.83668764768363));
#100877=CARTESIAN_POINT('Ctrl Pts',(-6.08263457751693,2.83963938452334,
4.38765958010009));
#100878=CARTESIAN_POINT('Ctrl Pts',(-6.05995954582765,2.83355382275396,
4.41909409084215));
#100879=CARTESIAN_POINT('Ctrl Pts',(-6.03705925485745,2.82748320915825,
4.45032726682969));
#100880=CARTESIAN_POINT('Ctrl Pts',(-6.01393899979816,2.82142857110512,
4.4813544495293));
#100881=CARTESIAN_POINT('Ctrl Pts',(-5.92386773399068,2.79784107599885,
4.60222930969558));
#100882=CARTESIAN_POINT('Ctrl Pts',(-5.82984232843352,2.77401081787658,
4.72079773781478));
#100883=CARTESIAN_POINT('Ctrl Pts',(-5.73205483213063,2.74999999826059,
4.83668764743604));
#100884=CARTESIAN_POINT('',(-5.55836338494564,2.75000000185147,4.84567817116543));
#100885=CARTESIAN_POINT('Origin',(6.31439345255558E-13,2.84071505699967,
-5.21718085400025E-13));
#100886=CARTESIAN_POINT('',(-6.08263457777298,2.66036061569962,4.38765957990834));
#100887=CARTESIAN_POINT('Origin',(0.142282947892951,2.55363074788761,-0.123711959058361));
#100888=CARTESIAN_POINT('Ctrl Pts',(-5.73205483213063,2.75000000173941,
4.83668764743604));
#100889=CARTESIAN_POINT('Ctrl Pts',(-5.82984232843352,2.72598918212338,
4.72079773781479));
#100890=CARTESIAN_POINT('Ctrl Pts',(-5.9238677351341,2.7021589239245,4.60222930920695));
#100891=CARTESIAN_POINT('Ctrl Pts',(-6.01393899979815,2.67857142889489,
4.48135444952932));
#100892=CARTESIAN_POINT('Ctrl Pts',(-6.0370592546571,2.67251679083703,4.45032726683011));
#100893=CARTESIAN_POINT('Ctrl Pts',(-6.0599595461582,2.66644617722229,4.4190940906906));
#100894=CARTESIAN_POINT('Ctrl Pts',(-6.08263457793126,2.66036061548051,
4.38765958006493));
#100895=CARTESIAN_POINT('Ctrl Pts',(-5.384671945,2.75,4.854668686));
#100896=CARTESIAN_POINT('Ctrl Pts',(-5.121607007,2.81435393,5.14645345700001));
#100897=CARTESIAN_POINT('Ctrl Pts',(-4.828552541,2.879481221,5.408103212));
#100898=CARTESIAN_POINT('Ctrl Pts',(-5.40265299200001,2.75,5.202051581));
#100899=CARTESIAN_POINT('Ctrl Pts',(-5.120764059,2.81435393,5.49481071));
#100900=CARTESIAN_POINT('Ctrl Pts',(-4.808890534,2.879481221,5.75539502));
#100901=CARTESIAN_POINT('',(-5.40265298407939,2.75,5.20205158911868));
#100902=CARTESIAN_POINT('',(-5.39366246066081,2.74999999814853,5.0283601419087));
#100903=CARTESIAN_POINT('',(-4.99720885004651,2.83963938428276,5.59266517060532));
#100904=CARTESIAN_POINT('Origin',(0.112362020446343,2.94636922241594,-0.151406233933549));
#100905=CARTESIAN_POINT('Ctrl Pts',(-4.83205245537769,2.87870320275158,
5.40497632385788));
#100906=CARTESIAN_POINT('Ctrl Pts',(-4.8595649216461,2.87185457192515,5.43618644745341));
#100907=CARTESIAN_POINT('Ctrl Pts',(-4.88709928706816,2.86518067051737,
5.46745092225138));
#100908=CARTESIAN_POINT('Ctrl Pts',(-4.94214121631759,2.85217081129803,
5.53000372745823));
#100909=CARTESIAN_POINT('Ctrl Pts',(-4.96968174897597,2.84582706796719,
5.5613295283599));
#100910=CARTESIAN_POINT('Ctrl Pts',(-4.99720884880956,2.83963938428673,
5.59266517169271));
#100911=CARTESIAN_POINT('Origin',(-2.57172755313562E-13,2.84071505700022,
2.98806118737005E-13));
#100912=CARTESIAN_POINT('',(-4.55829770235788,2.75,5.95583092881941));
#100913=CARTESIAN_POINT('Ctrl Pts',(-4.99720885021896,2.8396393844946,5.59266517084824));
#100914=CARTESIAN_POINT('Ctrl Pts',(-4.96830645736748,2.83355382275415,
5.61849029850888));
#100915=CARTESIAN_POINT('Ctrl Pts',(-4.93922735261419,2.82748320916757,
5.64407037449145));
#100916=CARTESIAN_POINT('Ctrl Pts',(-4.90997770917938,2.82142857112666,
5.66940198742473));
#100917=CARTESIAN_POINT('Ctrl Pts',(-4.79602773926675,2.79784107610431,
5.76808820007588));
#100918=CARTESIAN_POINT('Ctrl Pts',(-4.67871188691834,2.77401081787663,
5.86367188157641));
#100919=CARTESIAN_POINT('Ctrl Pts',(-4.55829770249563,2.74999999826059,
5.95583092854622));
#100920=CARTESIAN_POINT('',(-4.99720885004652,2.66036061571725,5.59266517060532));
#100921=CARTESIAN_POINT('Origin',(0.112362020508088,2.55363077759231,-0.151406233995569));
#100922=CARTESIAN_POINT('Ctrl Pts',(-4.55829770249563,2.75000000173941,
5.95583092854622));
#100923=CARTESIAN_POINT('Ctrl Pts',(-4.67871188691833,2.72598918212333,
5.86367188157641));
#100924=CARTESIAN_POINT('Ctrl Pts',(-4.7960277391387,2.70215892392436,5.76808820019688));
#100925=CARTESIAN_POINT('Ctrl Pts',(-4.90997770917935,2.67857142887334,
5.66940198742472));
#100926=CARTESIAN_POINT('Ctrl Pts',(-4.93922735264703,2.67251679082507,
5.64407037446037));
#100927=CARTESIAN_POINT('Ctrl Pts',(-4.96830645736746,2.66644617724585,
5.61849029850887));
#100928=CARTESIAN_POINT('Ctrl Pts',(-4.99720885021896,2.66036061550539,
5.59266517084823));
#100929=CARTESIAN_POINT('Ctrl Pts',(-4.83559480800001,2.879480225,5.401807369));
#100930=CARTESIAN_POINT('Ctrl Pts',(-4.702656805,2.85030975,5.520810931));
#100931=CARTESIAN_POINT('Ctrl Pts',(-4.564025943,2.821428571,5.633131207));
#100932=CARTESIAN_POINT('Ctrl Pts',(-4.393615631,2.785926731,5.771199548));
#100933=CARTESIAN_POINT('Ctrl Pts',(-4.215171043,2.75,5.89871452800001));
#100934=CARTESIAN_POINT('Ctrl Pts',(-4.21192594474503,2.74934665560115,
5.90103344752409));
#100935=CARTESIAN_POINT('Ctrl Pts',(-4.20868084649006,2.7486933112023,5.90335236704817));
#100936=CARTESIAN_POINT('Ctrl Pts',(-5.182911938,2.879480225,5.421016864));
#100937=CARTESIAN_POINT('Ctrl Pts',(-5.049501192,2.85030975,5.54856787));
#100938=CARTESIAN_POINT('Ctrl Pts',(-4.909977709,2.821428571,5.669401988));
#100939=CARTESIAN_POINT('Ctrl Pts',(-4.738470154,2.785926731,5.817935867));
#100940=CARTESIAN_POINT('Ctrl Pts',(-4.558297712,2.75,5.955830922));
#100941=CARTESIAN_POINT('Ctrl Pts',(-4.55502119191227,2.74934665560115,
5.95833860804061));
#100942=CARTESIAN_POINT('Ctrl Pts',(-4.55174467182455,2.7486933112023,5.96084629408121));
#100943=CARTESIAN_POINT('',(-4.38673436825944,2.75000000185146,5.92727273183888));
#100944=CARTESIAN_POINT('Ctrl Pts',(-4.215171043,2.75,5.89871452800001));
#100945=CARTESIAN_POINT('Ctrl Pts',(-3.895531316,2.81435393,6.127126348));
#100946=CARTESIAN_POINT('Ctrl Pts',(-3.553081338,2.879481221,6.31966083));
#100947=CARTESIAN_POINT('Ctrl Pts',(-4.158054649,2.75,6.241841198));
#100948=CARTESIAN_POINT('Ctrl Pts',(-3.819821564,2.81435393,6.467157993));
#100949=CARTESIAN_POINT('Ctrl Pts',(-3.459221545,2.879481221,6.654606397));
#100950=CARTESIAN_POINT('',(-4.15805463949679,2.75,6.24184120419392));
#100951=CARTESIAN_POINT('',(-3.67811919046932,2.83963938434862,6.53616395242618));
#100952=CARTESIAN_POINT('Origin',(0.077187090066142,2.9463692329547,-0.172020802380906));
#100953=CARTESIAN_POINT('Ctrl Pts',(-3.55717161501909,2.87870320271742,
6.31735942479319));
#100954=CARTESIAN_POINT('Ctrl Pts',(-3.57733160092653,2.87185457192173,
6.35375423980345));
#100955=CARTESIAN_POINT('Ctrl Pts',(-3.5975012901241,2.86518067055048,6.39020684292654));
#100956=CARTESIAN_POINT('Ctrl Pts',(-3.63780936552281,2.85217081133915,
6.46312958584068));
#100957=CARTESIAN_POINT('Ctrl Pts',(-3.65797189449222,2.84582706805202,
6.49964340700815));
#100958=CARTESIAN_POINT('Ctrl Pts',(-3.67811918906675,2.83963938435261,
6.53616395320061));
#100959=CARTESIAN_POINT('',(-4.18661283653578,2.7499999981484,6.07027786952739));
#100960=CARTESIAN_POINT('Origin',(8.23993651088983E-15,2.840715057,-8.23993651088983E-14));
#100961=CARTESIAN_POINT('',(-3.67811919046927,2.66036061565136,6.5361639524261));
#100962=CARTESIAN_POINT('Origin',(0.0771870900262217,2.55363076703895,-0.172020802323091));
#100963=CARTESIAN_POINT('',(-3.17139963915191,2.75,6.79648617466084));
#100964=CARTESIAN_POINT('Ctrl Pts',(-3.17139963931085,2.75000000173941,
6.79648617435012));
#100965=CARTESIAN_POINT('Ctrl Pts',(-3.30881007717435,2.72598918212335,
6.73236724563488));
#100966=CARTESIAN_POINT('Ctrl Pts',(-3.44393081564739,2.70215892392454,
6.66423769797584));
#100967=CARTESIAN_POINT('Ctrl Pts',(-3.57643131729758,2.67857142890089,
6.59235458861174));
#100968=CARTESIAN_POINT('Ctrl Pts',(-3.6104426685576,2.6725167908205,6.57390302330991));
#100969=CARTESIAN_POINT('Ctrl Pts',(-3.64434088045567,2.66644617717984,
6.55517214304717));
#100970=CARTESIAN_POINT('Ctrl Pts',(-3.67811919051385,2.66036061542591,
6.53616395257749));
#100971=CARTESIAN_POINT('Ctrl Pts',(-3.67811919051385,2.8396393845741,6.53616395257749));
#100972=CARTESIAN_POINT('Ctrl Pts',(-3.64434088045605,2.83355382282015,
6.55517214304733));
#100973=CARTESIAN_POINT('Ctrl Pts',(-3.61044266852075,2.82748320920675,
6.57390302316407));
#100974=CARTESIAN_POINT('Ctrl Pts',(-3.57643131723044,2.82142857109912,
6.59235458858938));
#100975=CARTESIAN_POINT('Ctrl Pts',(-3.44393081546194,2.79784107596927,
6.6642376984347));
#100976=CARTESIAN_POINT('Ctrl Pts',(-3.30881007717469,2.77401081787661,
6.732367245635));
#100977=CARTESIAN_POINT('Ctrl Pts',(-3.17139963931086,2.74999999826059,
6.79648617435011));
#100978=CARTESIAN_POINT('Ctrl Pts',(-3.56131238,2.879480225,6.315026059));
#100979=CARTESIAN_POINT('Ctrl Pts',(-3.405900146,2.85030975,6.402669643));
#100980=CARTESIAN_POINT('Ctrl Pts',(-3.246364857,2.821428571,6.482562396));
#100981=CARTESIAN_POINT('Ctrl Pts',(-3.050258032,2.785926731,6.580769596));
#100982=CARTESIAN_POINT('Ctrl Pts',(-2.848573427,2.75,6.666943035));
#100983=CARTESIAN_POINT('Ctrl Pts',(-2.84490569817126,2.74934665560115,
6.66851013927399));
#100984=CARTESIAN_POINT('Ctrl Pts',(-2.84123796934252,2.7486933112023,6.67007724354796));
#100985=CARTESIAN_POINT('Ctrl Pts',(-3.896379956,2.879480225,6.408449363));
#100986=CARTESIAN_POINT('Ctrl Pts',(-3.738668582,2.85030975,6.50433893));
#100987=CARTESIAN_POINT('Ctrl Pts',(-3.576431317,2.821428571,6.592354589));
#100988=CARTESIAN_POINT('Ctrl Pts',(-3.37700312,2.785926731,6.700546775));
#100989=CARTESIAN_POINT('Ctrl Pts',(-3.17139965,2.75,6.79648617));
#100990=CARTESIAN_POINT('Ctrl Pts',(-3.16766065477918,2.74934665560115,
6.7982308727494));
#100991=CARTESIAN_POINT('Ctrl Pts',(-3.16392165955837,2.7486933112023,6.79997557549878));
#100992=CARTESIAN_POINT('',(-3.00998652800533,2.75000000185147,6.73171460719254));
#100993=CARTESIAN_POINT('Ctrl Pts',(-2.848573427,2.75,6.666943035));
#100994=CARTESIAN_POINT('Ctrl Pts',(-2.48730491,2.81435393,6.82130162));
#100995=CARTESIAN_POINT('Ctrl Pts',(-2.111472,2.879481221,6.93571813100001));
#100996=CARTESIAN_POINT('Ctrl Pts',(-2.719030292,2.75,6.989769257));
#100997=CARTESIAN_POINT('Ctrl Pts',(-2.340268458,2.81435393,7.137108156));
#100998=CARTESIAN_POINT('Ctrl Pts',(-1.947803201,2.879481221,7.242655776));
#100999=CARTESIAN_POINT('',(-2.71903028147046,2.75,6.98976926121724));
#101000=CARTESIAN_POINT('',(-2.18704476574115,2.83963938432791,7.17403897303378));
#101001=CARTESIAN_POINT('Origin',(0.0384031144212466,2.94636922736759,-0.18459196964046));
#101002=CARTESIAN_POINT('Ctrl Pts',(-2.11596138231835,2.87870320278422,
6.9343498201285));
#101003=CARTESIAN_POINT('Ctrl Pts',(-2.12782622978281,2.87185457194067,
6.97422754562859));
#101004=CARTESIAN_POINT('Ctrl Pts',(-2.13968813088101,2.86518067053237,
7.01416379420402));
#101005=CARTESIAN_POINT('Ctrl Pts',(-2.1633775919085,2.85217081131246,7.09404668855678));
#101006=CARTESIAN_POINT('Ctrl Pts',(-2.17521934002718,2.84582706801463,
7.13404118468278));
#101007=CARTESIAN_POINT('Ctrl Pts',(-2.18704476419215,2.83963938433189,
7.17403897349237));
#101008=CARTESIAN_POINT('',(-2.78380184885462,2.74999999814853,6.82835615033994));
#101009=CARTESIAN_POINT('Origin',(4.54822811357669E-13,2.840715057,-1.85745516190217E-12));
#101010=CARTESIAN_POINT('',(-2.18704476574113,2.66036061567209,7.17403897303371));
#101011=CARTESIAN_POINT('Origin',(0.0384031144027247,2.55363077262798,-0.184591969595875));
#101012=CARTESIAN_POINT('',(-1.63621045241957,2.75,7.31934528129139));
#101013=CARTESIAN_POINT('Ctrl Pts',(-1.63621045262561,2.75000000173941,
7.31934528095056));
#101014=CARTESIAN_POINT('Ctrl Pts',(-1.78419198574281,2.72598918212331,
7.28626459934368));
#101015=CARTESIAN_POINT('Ctrl Pts',(-1.93079951578136,2.70215892392453,
7.24877484738345));
#101016=CARTESIAN_POINT('Ctrl Pts',(-2.0756549731527,2.67857142889793,7.2070560165367));
#101017=CARTESIAN_POINT('Ctrl Pts',(-2.11283769872407,2.67251679082882,
7.19634727361592));
#101018=CARTESIAN_POINT('Ctrl Pts',(-2.14996997488054,2.6664461772002,7.18534142458151));
#101019=CARTESIAN_POINT('Ctrl Pts',(-2.18704476576501,2.66036061545065,
7.17403897323128));
#101020=CARTESIAN_POINT('Ctrl Pts',(-2.18704476576502,2.83963938454935,
7.17403897323128));
#101021=CARTESIAN_POINT('Ctrl Pts',(-2.1499699748808,2.83355382279979,7.1853414245817));
#101022=CARTESIAN_POINT('Ctrl Pts',(-2.1128376989978,2.82748320919473,7.19634727365132));
#101023=CARTESIAN_POINT('Ctrl Pts',(-2.07565497315309,2.82142857110207,
7.20705601653691));
#101024=CARTESIAN_POINT('Ctrl Pts',(-1.93079951471658,2.79784107598374,
7.24877484724666));
#101025=CARTESIAN_POINT('Ctrl Pts',(-1.78419198574305,2.77401081787665,
7.28626459934383));
#101026=CARTESIAN_POINT('Ctrl Pts',(-1.63621045262561,2.74999999826059,
7.31934528095056));
#101027=CARTESIAN_POINT('Ctrl Pts',(-2.120506944,2.879480225,6.93296115));
#101028=CARTESIAN_POINT('Ctrl Pts',(-1.949887382,2.85030975,6.98514663800001));
#101029=CARTESIAN_POINT('Ctrl Pts',(-1.776907359,2.821428571,7.028876172));
#101030=CARTESIAN_POINT('Ctrl Pts',(-1.564273757,2.785926731,7.082630172));
#101031=CARTESIAN_POINT('Ctrl Pts',(-1.348779684,2.75,7.123432695));
#101032=CARTESIAN_POINT('Ctrl Pts',(-1.34486082353981,2.74934665560115,
7.12417470795578));
#101033=CARTESIAN_POINT('Ctrl Pts',(-1.34094196307961,2.7486933112023,7.12491672091157));
#101034=CARTESIAN_POINT('Ctrl Pts',(-2.427657577,2.879480225,7.096229893));
#101035=CARTESIAN_POINT('Ctrl Pts',(-2.253019985,2.85030975,7.155974331));
#101036=CARTESIAN_POINT('Ctrl Pts',(-2.075654973,2.821428571,7.207056017));
#101037=CARTESIAN_POINT('Ctrl Pts',(-1.857631174,2.785926731,7.269847562));
#101038=CARTESIAN_POINT('Ctrl Pts',(-1.636210464,2.75,7.319345279));
#101039=CARTESIAN_POINT('Ctrl Pts',(-1.63218382487528,2.74934665560115,
7.32024541812365));
#101040=CARTESIAN_POINT('Ctrl Pts',(-1.62815718575056,2.7486933112023,7.3211455572473));
#101041=CARTESIAN_POINT('',(-1.49249506274193,2.75000000185147,7.22138898932679));
#101042=CARTESIAN_POINT('Ctrl Pts',(-1.348779684,2.75,7.123432695));
#101043=CARTESIAN_POINT('Ctrl Pts',(-0.962774892000001,2.81435393,7.196520411));
#101044=CARTESIAN_POINT('Ctrl Pts',(-0.571132578,2.879481221,7.227468961));
#101045=CARTESIAN_POINT('Ctrl Pts',(-1.1528671,2.75,7.41086347500001));
#101046=CARTESIAN_POINT('Ctrl Pts',(-0.751286999,2.81435393,7.473335074));
#101047=CARTESIAN_POINT('Ctrl Pts',(-0.345307744,2.879481221,7.49204662));
#101048=CARTESIAN_POINT('',(-1.15286708880857,2.75,7.41086347684554));
#101049=CARTESIAN_POINT('',(-0.593706557887295,2.83963938429001,7.47646390471328));
#101050=CARTESIAN_POINT('Origin',(-0.00217653894457756,2.94636924407997,
-0.188531935449823));
#101051=CARTESIAN_POINT('Ctrl Pts',(-0.575811147992967,2.87870320269475,
7.22709772493196));
#101052=CARTESIAN_POINT('Ctrl Pts',(-0.578826069595871,2.87185457189305,
7.26859372276947));
#101053=CARTESIAN_POINT('Ctrl Pts',(-0.581825533002033,2.86518067051596,
7.31014624196717));
#101054=CARTESIAN_POINT('Ctrl Pts',(-0.587788686380652,2.85217081130779,
7.39325405240357));
#101055=CARTESIAN_POINT('Ctrl Pts',(-0.590755946430203,2.84582706796969,
7.43485912546498));
#101056=CARTESIAN_POINT('Ctrl Pts',(-0.593706556239983,2.83963938429398,
7.47646390483069));
#101057=CARTESIAN_POINT('',(-1.25082338067054,2.74999999814853,7.26714808695003));
#101058=CARTESIAN_POINT('Origin',(7.34360624610533E-14,2.84071505699978,
-7.24680732089311E-13));
#101059=CARTESIAN_POINT('',(-0.593706557887282,2.66036061570999,7.47646390471321));
#101060=CARTESIAN_POINT('Origin',(-0.00217653895281604,2.55363075591576,
-0.188531935399019));
#101061=CARTESIAN_POINT('',(-0.0245138841973356,2.75,7.49995993759332));
#101062=CARTESIAN_POINT('Ctrl Pts',(-0.0245138844723349,2.7500000017394,
7.49995993745986));
#101063=CARTESIAN_POINT('Ctrl Pts',(-0.176147060361898,2.72598918212328,
7.49946431871023));
#101064=CARTESIAN_POINT('Ctrl Pts',(-0.327386176079984,2.70215892392418,
7.49436734156413));
#101065=CARTESIAN_POINT('Ctrl Pts',(-0.477823308499627,2.67857142884758,
7.48476351549384));
#101066=CARTESIAN_POINT('Ctrl Pts',(-0.516438785871464,2.67251679079197,
7.48229832387388));
#101067=CARTESIAN_POINT('Ctrl Pts',(-0.555068861913598,2.66644617724321,
7.4795321272271));
#101068=CARTESIAN_POINT('Ctrl Pts',(-0.593706557878843,2.66036061549942,
7.47646390502461));
#101069=CARTESIAN_POINT('Ctrl Pts',(-0.593706557878851,2.83963938450059,
7.47646390502461));
#101070=CARTESIAN_POINT('Ctrl Pts',(-0.555068861913804,2.83355382275679,
7.47953212722733));
#101071=CARTESIAN_POINT('Ctrl Pts',(-0.516438785815961,2.82748320916829,
7.4822983240761));
#101072=CARTESIAN_POINT('Ctrl Pts',(-0.477823308499939,2.82142857115242,
7.48476351549411));
#101073=CARTESIAN_POINT('Ctrl Pts',(-0.327386176297452,2.7978410762306,
7.49436734077764));
#101074=CARTESIAN_POINT('Ctrl Pts',(-0.176147060362065,2.77401081787682,
7.49946431871042));
#101075=CARTESIAN_POINT('Ctrl Pts',(-0.0245138844723352,2.7499999982606,
7.49995993745986));
#101076=CARTESIAN_POINT('Ctrl Pts',(-0.586785048244814,2.88054032958409,
7.22600414473736));
#101077=CARTESIAN_POINT('Ctrl Pts',(-0.405720639388154,2.85083482770451,
7.24070741365988));
#101078=CARTESIAN_POINT('Ctrl Pts',(-0.224147072116056,2.821428571,7.24632394240433));
#101079=CARTESIAN_POINT('Ctrl Pts',(-0.00493536232790208,2.785926731,7.25310471367341));
#101080=CARTESIAN_POINT('Ctrl Pts',(0.214285371684215,2.75,7.24662227317082));
#101081=CARTESIAN_POINT('Ctrl Pts',(0.219906386668887,2.74907880660006,
7.24645605761933));
#101082=CARTESIAN_POINT('Ctrl Pts',(0.225527401653559,2.74815761320013,
7.24628984206785));
#101083=CARTESIAN_POINT('Ctrl Pts',(-0.852084755314493,2.88054032958409,
7.45143956339864));
#101084=CARTESIAN_POINT('Ctrl Pts',(-0.665371536520333,2.85083482770451,
7.47279053664977));
#101085=CARTESIAN_POINT('Ctrl Pts',(-0.477823308,2.821428571,7.484763516));
#101086=CARTESIAN_POINT('Ctrl Pts',(-0.251398459,2.785926731,7.499218357));
#101087=CARTESIAN_POINT('Ctrl Pts',(-0.024513896,2.75,7.499959938));
#101088=CARTESIAN_POINT('Ctrl Pts',(-0.0186963736102467,2.74907880660006,
7.49997895279773));
#101089=CARTESIAN_POINT('Ctrl Pts',(-0.0128788512204935,2.74815761320013,
7.49999796759543));
#101090=CARTESIAN_POINT('',(0.0947838119950076,2.75000000185146,7.37339924885223));
#101091=CARTESIAN_POINT('Ctrl Pts',(-1.649106096,3.007773793,7.31645058));
#101092=CARTESIAN_POINT('Ctrl Pts',(-1.248920843,3.07352872,7.40665114));
#101093=CARTESIAN_POINT('Ctrl Pts',(-0.841285031000001,3.138525418,7.452666603));
#101094=CARTESIAN_POINT('Ctrl Pts',(-0.837226499918957,3.13917254249503,
7.45312474524682));
#101095=CARTESIAN_POINT('Ctrl Pts',(-0.833167968837915,3.13981966699007,
7.45358288749364));
#101096=CARTESIAN_POINT('Ctrl Pts',(-1.361330525,3.007773793,7.121044811));
#101097=CARTESIAN_POINT('Ctrl Pts',(-0.971833309999999,3.07352872,7.195505015));
#101098=CARTESIAN_POINT('Ctrl Pts',(-0.576538529,3.138525418,7.22703973500001));
#101099=CARTESIAN_POINT('Ctrl Pts',(-0.572602868521616,3.13917254249503,
7.22735370309967));
#101100=CARTESIAN_POINT('Ctrl Pts',(-0.568667208043231,3.13981966699007,
7.22766767119934));
#101101=CARTESIAN_POINT('',(-0.841285032614871,3.13852541850725,7.45266660087849));
#101102=CARTESIAN_POINT('',(-0.708911788726928,3.13852541943002,7.33985316815712));
#101103=CARTESIAN_POINT('',(-1.40333520077077,3.04797057326662,7.36754032226984));
#101104=CARTESIAN_POINT('Origin',(0.0511750932729073,2.9464821042826,-0.1817606101355));
#101105=CARTESIAN_POINT('Ctrl Pts',(-1.35667769724235,3.00855922358375,
7.12193272858185));
#101106=CARTESIAN_POINT('Ctrl Pts',(-1.36448211669332,3.01545478679876,
7.16280006053993));
#101107=CARTESIAN_POINT('Ctrl Pts',(-1.37227545237948,3.02218156071882,
7.20372368936741));
#101108=CARTESIAN_POINT('Ctrl Pts',(-1.387824204079,3.03530792012134,7.28557967537735));
#101109=CARTESIAN_POINT('Ctrl Pts',(-1.39558848094672,3.04171498175703,
7.32655869520993));
#101110=CARTESIAN_POINT('Ctrl Pts',(-1.4033352045952,3.04797057332674,7.36754031585559));
#101111=CARTESIAN_POINT('Ctrl Pts',(-1.96108872313986,3.13983235804358,
7.23907434966038));
#101112=CARTESIAN_POINT('Ctrl Pts',(-1.95715442456993,3.13917888802179,
7.2401355763302));
#101113=CARTESIAN_POINT('Ctrl Pts',(-1.953220126,3.138525418,7.241196803));
#101114=CARTESIAN_POINT('Ctrl Pts',(-1.559352402,3.073105688,7.347437579));
#101115=CARTESIAN_POINT('Ctrl Pts',(-1.156285027,3.007781414,7.41033096));
#101116=CARTESIAN_POINT('Ctrl Pts',(-2.12419422451127,3.13983235804358,
6.93183676660003));
#101117=CARTESIAN_POINT('Ctrl Pts',(-2.12042675825564,3.13917888802179,
6.93298679330002));
#101118=CARTESIAN_POINT('Ctrl Pts',(-2.116659292,3.138525418,6.93413682));
#101119=CARTESIAN_POINT('Ctrl Pts',(-1.739493367,3.073105688,7.04926748200001));
#101120=CARTESIAN_POINT('Ctrl Pts',(-1.352065021,3.007781414,7.122809851));
#101121=CARTESIAN_POINT('',(-1.95322012318267,3.13852541980573,7.24119677028181));
#101122=CARTESIAN_POINT('Origin',(0.0426114486941837,3.08928602504253,-0.188292761037378));
#101123=CARTESIAN_POINT('',(-2.03493969893267,3.13852541968788,7.08766681439043));
#101124=CARTESIAN_POINT('Origin',(1.51788304147971E-15,3.22948687199989,
-4.08527378592538E-13));
#101125=CARTESIAN_POINT('',(-1.39671107502148,3.22840427021682,7.36879896407947));
#101126=CARTESIAN_POINT('Origin',(0.0135835823359337,3.08929955170748,-0.190873985323708));
#101127=CARTESIAN_POINT('Ctrl Pts',(-1.95322012332207,3.13852541968788,
7.24119679148189));
#101128=CARTESIAN_POINT('Ctrl Pts',(-1.72094870099522,3.176642188,7.30384904600832));
#101129=CARTESIAN_POINT('Ctrl Pts',(-1.48513956599495,3.214285714,7.35148695600817));
#101130=CARTESIAN_POINT('Ctrl Pts',(-1.44097732348694,3.22133557899821,
7.36040856533142));
#101131=CARTESIAN_POINT('Ctrl Pts',(-1.39671108389569,3.22840426981341,
7.36879896225412));
#101132=CARTESIAN_POINT('Ctrl Pts',(-3.183371514,3.007773793,6.790886967));
#101133=CARTESIAN_POINT('Ctrl Pts',(-2.811932824,3.07352872,6.965006689));
#101134=CARTESIAN_POINT('Ctrl Pts',(-2.423719275,3.138525418,7.097575986));
#101135=CARTESIAN_POINT('Ctrl Pts',(-2.4198541171598,3.13917254249503,7.09889588134881));
#101136=CARTESIAN_POINT('Ctrl Pts',(-2.4159889593196,3.13981966699007,7.10021577669762));
#101137=CARTESIAN_POINT('Ctrl Pts',(-2.860317511,3.007773793,6.661912919));
#101138=CARTESIAN_POINT('Ctrl Pts',(-2.495933268,3.07352872,6.818362672));
#101139=CARTESIAN_POINT('Ctrl Pts',(-2.116659292,3.138525418,6.93413682000001));
#101140=CARTESIAN_POINT('Ctrl Pts',(-2.1128831389376,3.13917254249503,6.93528949835702));
#101141=CARTESIAN_POINT('Ctrl Pts',(-2.10910698587521,3.13981966699007,
6.93644217671404));
#101142=CARTESIAN_POINT('',(-2.42371927611826,3.13852541850768,7.09757598357859));
#101143=CARTESIAN_POINT('',(-2.27018929184914,3.1385254194313,7.01585640029839));
#101144=CARTESIAN_POINT('',(-2.95432939001173,3.0479705733085,6.89361573776188));
#101145=CARTESIAN_POINT('Origin',(0.0890517505241159,2.94648211656367,-0.166509866620262));
#101146=CARTESIAN_POINT('Ctrl Pts',(-2.85596434015128,3.00855922361461,
6.66378029826412));
#101147=CARTESIAN_POINT('Ctrl Pts',(-2.87237156518513,3.0154547868692,6.702014455108));
#101148=CARTESIAN_POINT('Ctrl Pts',(-2.8887800676319,3.02218156079834,6.74030597523103));
#101149=CARTESIAN_POINT('Ctrl Pts',(-2.92156191564258,3.0353079202082,6.81690569145188));
#101150=CARTESIAN_POINT('Ctrl Pts',(-2.9379539459452,3.04171498182537,6.85525755432722));
#101151=CARTESIAN_POINT('Ctrl Pts',(-2.95432939247112,3.04797057336922,
6.89361573063811));
#101152=CARTESIAN_POINT('Ctrl Pts',(-3.47142655900055,3.13983235804358,
6.64825270764319));
#101153=CARTESIAN_POINT('Ctrl Pts',(-3.46781237450027,3.13917888802179,
6.6501348813216));
#101154=CARTESIAN_POINT('Ctrl Pts',(-3.46419819,3.138525418,6.652017055));
#101155=CARTESIAN_POINT('Ctrl Pts',(-3.1023775,3.073105688,6.840443899));
#101156=CARTESIAN_POINT('Ctrl Pts',(-2.722253834,3.007781414,6.988514439));
#101157=CARTESIAN_POINT('Ctrl Pts',(-3.56467174548097,3.13983235804358,
6.31313530783206));
#101158=CARTESIAN_POINT('Ctrl Pts',(-3.56123958224049,3.13917888802179,
6.31506834141603));
#101159=CARTESIAN_POINT('Ctrl Pts',(-3.557807419,3.138525418,6.317001375));
#101160=CARTESIAN_POINT('Ctrl Pts',(-3.214209113,3.073105688,6.51051987000001));
#101161=CARTESIAN_POINT('Ctrl Pts',(-2.851648061,3.007781414,6.665628503));
#101162=CARTESIAN_POINT('',(-3.46419818021678,3.13852541980584,6.65201702365357));
#101163=CARTESIAN_POINT('Origin',(0.0820926261211432,3.08928600358673,-0.174730455447152));
#101164=CARTESIAN_POINT('',(-3.51100279528937,3.13852541968789,6.48450921998705));
#101165=CARTESIAN_POINT('Origin',(-3.64725610824124E-13,3.22948687200033,
8.43509290193722E-13));
#101166=CARTESIAN_POINT('',(-2.94813070307675,3.22840427021118,6.89626894456007));
#101167=CARTESIAN_POINT('Origin',(0.0542983013444376,3.08929950335629,-0.183491481227457));
#101168=CARTESIAN_POINT('Ctrl Pts',(-3.46419818490878,3.13852541968789,
6.65201704432619));
#101169=CARTESIAN_POINT('Ctrl Pts',(-3.25082552099696,3.176642188,6.76313601400966));
#101170=CARTESIAN_POINT('Ctrl Pts',(-3.03077021499666,3.214285714,6.86035217000956));
#101171=CARTESIAN_POINT('Ctrl Pts',(-2.98955834350168,3.22133557899461,
6.87855877362988));
#101172=CARTESIAN_POINT('Ctrl Pts',(-2.94813071139113,3.22840426981375,
6.89626894081897));
#101173=CARTESIAN_POINT('Ctrl Pts',(-4.568786018,3.007773793,5.947789028));
#101174=CARTESIAN_POINT('Ctrl Pts',(-4.243461951,3.07352872,6.197686266));
#101175=CARTESIAN_POINT('Ctrl Pts',(-3.892823099,3.138525418,6.41061060400001));
#101176=CARTESIAN_POINT('Ctrl Pts',(-3.88933204488461,3.13917254249503,
6.41273053561112));
#101177=CARTESIAN_POINT('Ctrl Pts',(-3.88584099076922,3.13981966699007,
6.41485046722225));
#101178=CARTESIAN_POINT('Ctrl Pts',(-4.22555923,3.007773793,5.891277382));
#101179=CARTESIAN_POINT('Ctrl Pts',(-3.90332616,3.07352872,6.122401268));
#101180=CARTESIAN_POINT('Ctrl Pts',(-3.557807419,3.138525418,6.317001375));
#101181=CARTESIAN_POINT('Ctrl Pts',(-3.55436734207803,3.13917254249503,
6.31893886567032));
#101182=CARTESIAN_POINT('Ctrl Pts',(-3.55092726515605,3.13981966699007,
6.32087635634062));
#101183=CARTESIAN_POINT('',(-3.89282309958503,3.13852541850725,6.41061060139456));
#101184=CARTESIAN_POINT('',(-3.72531526656647,3.13852541943003,6.36380598507066));
#101185=CARTESIAN_POINT('',(-4.36718242045613,3.0479705733016,6.09735334318613));
#101186=CARTESIAN_POINT('Origin',(0.122764508923577,2.94648211407493,-0.143473532378355));
#101187=CARTESIAN_POINT('Ctrl Pts',(-4.22170926527457,3.00855922354818,
5.89403690575471));
#101188=CARTESIAN_POINT('Ctrl Pts',(-4.24595211177457,3.01545478679473,
5.92785010094362));
#101189=CARTESIAN_POINT('Ctrl Pts',(-4.27020853745607,3.02218156074601,
5.96171904382587));
#101190=CARTESIAN_POINT('Ctrl Pts',(-4.3186906387285,3.03530792016112,6.02948077315774));
#101191=CARTESIAN_POINT('Ctrl Pts',(-4.34294394943307,3.04171498180012,
6.06341218901963));
#101192=CARTESIAN_POINT('Ctrl Pts',(-4.36718242130857,3.04797057336225,
6.09735333570621));
#101193=CARTESIAN_POINT('Ctrl Pts',(-4.81944434632715,3.13983235804358,
5.74656615832854));
#101194=CARTESIAN_POINT('Ctrl Pts',(-4.81631927116357,3.13917888802179,
5.74918127066428));
#101195=CARTESIAN_POINT('Ctrl Pts',(-4.813194196,3.138525418,5.751796383));
#101196=CARTESIAN_POINT('Ctrl Pts',(-4.500338875,3.073105688,6.01359866500001));
#101197=CARTESIAN_POINT('Ctrl Pts',(-4.160933077,3.007781414,6.23992275));
#101198=CARTESIAN_POINT('Ctrl Pts',(-4.83846917719169,3.13983235804358,
5.39923865803316));
#101199=CARTESIAN_POINT('Ctrl Pts',(-4.83553280109584,3.13917888802179,
5.40186431201658));
#101200=CARTESIAN_POINT('Ctrl Pts',(-4.83259642500001,3.138525418,5.404489966));
#101201=CARTESIAN_POINT('Ctrl Pts',(-4.538632012,3.073105688,5.667347586));
#101202=CARTESIAN_POINT('Ctrl Pts',(-4.217891208,3.007781414,5.896769773));
#101203=CARTESIAN_POINT('',(-4.81319417970427,3.13852541980591,5.7517963544844));
#101204=CARTESIAN_POINT('Origin',(0.117735124629917,3.08928604967561,-0.152997718666201));
#101205=CARTESIAN_POINT('',(-4.82289530257677,3.13852541968789,5.57814318135047));
#101206=CARTESIAN_POINT('Origin',(5.61833565781988E-13,3.22948687200044,
-9.40653804848424E-13));
#101207=CARTESIAN_POINT('',(-4.36169901671411,3.22840427023201,6.10127705377287));
#101208=CARTESIAN_POINT('Origin',(0.0924741257385808,3.08929953180407,-0.167529084643822));
#101209=CARTESIAN_POINT('Ctrl Pts',(-4.81319418873319,3.13852541968789,
5.7517963736712));
#101210=CARTESIAN_POINT('Ctrl Pts',(-4.62869735299911,3.176642188,5.9061862590101));
#101211=CARTESIAN_POINT('Ctrl Pts',(-4.43468541799878,3.214285714,6.04843494201006));
#101212=CARTESIAN_POINT('Ctrl Pts',(-4.39835093887207,3.22133557899724,
6.0750752195256));
#101213=CARTESIAN_POINT('Ctrl Pts',(-4.36169902396167,3.22840426981355,
6.10127704866005));
#101214=CARTESIAN_POINT('Ctrl Pts',(-5.740569165,3.007773793,4.826579084));
#101215=CARTESIAN_POINT('Ctrl Pts',(-5.476571513,3.07352872,5.140568922));
#101216=CARTESIAN_POINT('Ctrl Pts',(-5.179902842,3.138525418,5.423892195));
#101217=CARTESIAN_POINT('Ctrl Pts',(-5.17694912942966,3.13917254249503,
5.42671303722142));
#101218=CARTESIAN_POINT('Ctrl Pts',(-5.17399541685932,3.13981966699007,
5.42953387944285));
#101219=CARTESIAN_POINT('Ctrl Pts',(-5.393218496,3.007773793,4.845172263));
#101220=CARTESIAN_POINT('Ctrl Pts',(-5.12820386,3.07352872,5.140163186));
#101221=CARTESIAN_POINT('Ctrl Pts',(-4.832596425,3.138525418,5.404489966));
#101222=CARTESIAN_POINT('Ctrl Pts',(-4.82965327837888,3.13917254249503,
5.40712167406049));
#101223=CARTESIAN_POINT('Ctrl Pts',(-4.82671013175777,3.13981966699007,
5.40975338212096));
#101224=CARTESIAN_POINT('',(-5.17990284201368,3.13852541850726,5.42389219232864));
#101225=CARTESIAN_POINT('',(-5.00624963993739,3.13852541943003,5.41419107454764));
#101226=CARTESIAN_POINT('',(-5.57583085480616,3.04797057328096,5.01598548285496));
#101227=CARTESIAN_POINT('Origin',(0.150736866359442,2.94648216097497,-0.113728428632556));
#101228=CARTESIAN_POINT('Ctrl Pts',(-5.39005175674981,3.00855922359023,
4.84869489944727));
#101229=CARTESIAN_POINT('Ctrl Pts',(-5.42099665668092,3.01545478682458,
4.87650606540874));
#101230=CARTESIAN_POINT('Ctrl Pts',(-5.45196680211484,3.02218156072737,
4.90436875647179));
#101231=CARTESIAN_POINT('Ctrl Pts',(-5.51388218774758,3.03530792014147,
4.96012403551547));
#101232=CARTESIAN_POINT('Ctrl Pts',(-5.54486272091281,3.04171498177744,
4.98804840882984));
#101233=CARTESIAN_POINT('Ctrl Pts',(-5.57583085399527,3.04797057334128,
5.01598547540733));
#101234=CARTESIAN_POINT('Ctrl Pts',(-5.9421102725929,3.13983235804358,4.57617656251187));
#101235=CARTESIAN_POINT('Ctrl Pts',(-5.93962043179645,3.13917888802179,
4.57940233375594));
#101236=CARTESIAN_POINT('Ctrl Pts',(-5.93713059100001,3.138525418,4.582628105));
#101237=CARTESIAN_POINT('Ctrl Pts',(-5.687869405,3.073105688,4.905564241));
#101238=CARTESIAN_POINT('Ctrl Pts',(-5.405051715,3.007781414,5.199559208));
#101239=CARTESIAN_POINT('Ctrl Pts',(-5.88602516750172,3.13983235804358,
4.23287960957504));
#101240=CARTESIAN_POINT('Ctrl Pts',(-5.88372188025086,3.13917888802179,
4.23607511128751));
#101241=CARTESIAN_POINT('Ctrl Pts',(-5.881418593,3.138525418,4.239270613));
#101242=CARTESIAN_POINT('Ctrl Pts',(-5.650833524,3.073105688,4.559176427));
#101243=CARTESIAN_POINT('Ctrl Pts',(-5.386910449,3.007781414,4.852184643));
#101244=CARTESIAN_POINT('',(-5.93713056884798,3.13852541976328,4.5826280811928));
#101245=CARTESIAN_POINT('Origin',(0.147872621769565,3.08928602335869,-0.124111231483713));
#101246=CARTESIAN_POINT('',(-5.90927458573466,3.13852541968789,4.41094936739357));
#101247=CARTESIAN_POINT('Origin',(-6.52689707836274E-13,3.22948687199956,
5.54677831443584E-13));
#101248=CARTESIAN_POINT('',(-5.57131913161687,3.22840427018799,5.02099622948482));
#101249=CARTESIAN_POINT('Origin',(0.126325665212076,3.08929953797125,-0.143732892740396));
#101250=CARTESIAN_POINT('Ctrl Pts',(-5.93713058189749,3.13852541968789,
4.58262809745036));
#101251=CARTESIAN_POINT('Ctrl Pts',(-5.79013644100131,3.176642188,4.77306979901004));
#101252=CARTESIAN_POINT('Ctrl Pts',(-5.63123965900098,3.214285714,4.95369961801008));
#101253=CARTESIAN_POINT('Ctrl Pts',(-5.60148153190861,3.2213355789788,4.98752789928355));
#101254=CARTESIAN_POINT('Ctrl Pts',(-5.57131913758477,3.22840426981253,
5.02099622261143));
#101255=CARTESIAN_POINT('Ctrl Pts',(-6.643929679,3.007773793,3.479683667));
#101256=CARTESIAN_POINT('Ctrl Pts',(-6.453602679,3.07352872,3.843084288));
#101257=CARTESIAN_POINT('Ctrl Pts',(-6.224776085,3.138525418,4.183558616));
#101258=CARTESIAN_POINT('Ctrl Pts',(-6.22249782627842,3.13917254249503,
4.18694846939808));
#101259=CARTESIAN_POINT('Ctrl Pts',(-6.22021956755684,3.13981966699007,
4.19033832279615));
#101260=CARTESIAN_POINT('Ctrl Pts',(-6.308696859,3.007773793,3.572512274));
#101261=CARTESIAN_POINT('Ctrl Pts',(-6.113292446,3.07352872,3.917576786));
#101262=CARTESIAN_POINT('Ctrl Pts',(-5.881418593,3.138525418,4.239270613));
#101263=CARTESIAN_POINT('Ctrl Pts',(-5.87910999495346,3.13917254249503,
4.24247348271121));
#101264=CARTESIAN_POINT('Ctrl Pts',(-5.87680139690693,3.13981966699007,
4.24567635242242));
#101265=CARTESIAN_POINT('',(-6.22477608441923,3.13852541850725,4.18355861340267));
#101266=CARTESIAN_POINT('',(-6.05309734400731,3.13852541943003,4.21141460730296));
#101267=CARTESIAN_POINT('',(-6.52375963486162,3.04797057325993,3.70007571645805));
#101268=CARTESIAN_POINT('Origin',(0.17166106789941,2.9464821192333,-0.0786655901702615));
#101269=CARTESIAN_POINT('Ctrl Pts',(-6.30636141922387,3.00855922362562,
3.57663330860406));
#101270=CARTESIAN_POINT('Ctrl Pts',(-6.34256142316941,3.01545478687365,
3.59714202626727));
#101271=CARTESIAN_POINT('Ctrl Pts',(-6.37879715852299,3.02218156074315,
3.61769563720488));
#101272=CARTESIAN_POINT('Ctrl Pts',(-6.45125073357316,3.03530792015397,
3.65883741109778));
#101273=CARTESIAN_POINT('Ctrl Pts',(-6.48750987375242,3.04171498177261,
3.67944902917069));
#101274=CARTESIAN_POINT('Ctrl Pts',(-6.52375963243751,3.04797057331986,
3.70007570940484));
#101275=CARTESIAN_POINT('Ctrl Pts',(-6.78692972648235,3.13983235804358,
3.19181003665553));
#101276=CARTESIAN_POINT('Ctrl Pts',(-6.78519154224117,3.13917888802179,
3.19549563332777));
#101277=CARTESIAN_POINT('Ctrl Pts',(-6.783453358,3.138525418,3.19918123));
#101278=CARTESIAN_POINT('Ctrl Pts',(-6.609441483,3.073105688,3.568151085));
#101279=CARTESIAN_POINT('Ctrl Pts',(-6.396436141,3.007781414,3.916070057));
#101280=CARTESIAN_POINT('Ctrl Pts',(-6.65835716353885,3.13983235804358,
2.86859581532773));
#101281=CARTESIAN_POINT('Ctrl Pts',(-6.65679466426943,3.13917888802179,
2.87221174666387));
#101282=CARTESIAN_POINT('Ctrl Pts',(-6.655232165,3.138525418,2.875827678));
#101283=CARTESIAN_POINT('Ctrl Pts',(-6.49880834,3.073105688,3.237823246));
#101284=CARTESIAN_POINT('Ctrl Pts',(-6.304043745,3.007781414,3.580716752));
#101285=CARTESIAN_POINT('',(-6.78345333124599,3.13852541976318,3.19918121151157));
#101286=CARTESIAN_POINT('Origin',(0.171095824460236,3.08928604518906,-0.0894214078364035));
#101287=CARTESIAN_POINT('',(-6.71934275718553,3.13852541968788,3.03750446354416));
#101288=CARTESIAN_POINT('Origin',(-4.65773253299773E-13,3.22948687199922,
2.87530416143156E-13));
#101289=CARTESIAN_POINT('',(-6.52043055618455,3.22840427020818,3.70593920108148));
#101290=CARTESIAN_POINT('Origin',(0.154270784387071,3.08929955107671,-0.113216334442104));
#101291=CARTESIAN_POINT('Ctrl Pts',(-6.78345334748772,3.13852541968788,
3.19918122458446));
#101292=CARTESIAN_POINT('Ctrl Pts',(-6.68083518500339,3.176642188,3.41676990000944));
#101293=CARTESIAN_POINT('Ctrl Pts',(-6.56448339300309,3.214285714,3.62733480500954));
#101294=CARTESIAN_POINT('Ctrl Pts',(-6.54269307504985,3.22133557898338,
3.66676931770777));
#101295=CARTESIAN_POINT('Ctrl Pts',(-6.52043056059152,3.22840426981355,
3.70593919332983));
#101296=CARTESIAN_POINT('Ctrl Pts',(-7.236627425,3.007773793,1.970082109));
#101297=CARTESIAN_POINT('Ctrl Pts',(-7.128870556,3.07352872,2.365901304));
#101298=CARTESIAN_POINT('Ctrl Pts',(-6.978585717,3.138525418,2.747606485));
#101299=CARTESIAN_POINT('Ctrl Pts',(-6.97708944098073,3.13917254249503,
2.75140684378909));
#101300=CARTESIAN_POINT('Ctrl Pts',(-6.97559316496146,3.13981966699007,
2.75520720257818));
#101301=CARTESIAN_POINT('Ctrl Pts',(-6.929187568,3.007773793,2.132805581));
#101302=CARTESIAN_POINT('Ctrl Pts',(-6.812530272,3.07352872,2.511808849));
#101303=CARTESIAN_POINT('Ctrl Pts',(-6.655232165,3.138525418,2.875827678));
#101304=CARTESIAN_POINT('Ctrl Pts',(-6.65366606301029,3.13917254249503,
2.87945194674207));
#101305=CARTESIAN_POINT('Ctrl Pts',(-6.65209996102059,3.13981966699007,
2.88307621548415));
#101306=CARTESIAN_POINT('',(-6.97858571586415,3.13852541850724,2.74760648259996));
#101307=CARTESIAN_POINT('',(-6.81690894434307,3.13852541943002,2.81171707339485));
#101308=CARTESIAN_POINT('',(-7.16664466580176,3.04797057323609,2.21115452164468));
#101309=CARTESIAN_POINT('Origin',(0.18455854297556,2.9464821110578,-0.0399243888134687));
#101310=CARTESIAN_POINT('Ctrl Pts',(-6.92779263031792,3.00855922359982,
2.13733231839922));
#101311=CARTESIAN_POINT('Ctrl Pts',(-6.96755506624603,3.01545478682721,
2.1495796229758));
#101312=CARTESIAN_POINT('Ctrl Pts',(-7.00736204937631,3.02218156074204,
2.16186309011969));
#101313=CARTESIAN_POINT('Ctrl Pts',(-7.08696596538827,3.03530792012699,
2.18646761537362));
#101314=CARTESIAN_POINT('Ctrl Pts',(-7.12680827576463,3.04171498174729,
2.19880270198573));
#101315=CARTESIAN_POINT('Ctrl Pts',(-7.16664466189622,3.04797057329574,
2.21115451533576));
#101316=CARTESIAN_POINT('Ctrl Pts',(-7.31439988922279,3.13983235804358,
1.65819802060071));
#101317=CARTESIAN_POINT('Ctrl Pts',(-7.31349463711139,3.13917888802179,
1.66217110830035));
#101318=CARTESIAN_POINT('Ctrl Pts',(-7.312589385,3.138525418,1.666144196));
#101319=CARTESIAN_POINT('Ctrl Pts',(-7.221963424,3.073105688,2.06389515));
#101320=CARTESIAN_POINT('Ctrl Pts',(-7.088730323,3.007781414,2.449469822));
#101321=CARTESIAN_POINT('Ctrl Pts',(-7.11935177812158,3.13983235804358,
1.37017966895271));
#101322=CARTESIAN_POINT('Ctrl Pts',(-7.11860312756079,3.13917888802179,
1.37404695297636));
#101323=CARTESIAN_POINT('Ctrl Pts',(-7.117854477,3.138525418,1.377914237));
#101324=CARTESIAN_POINT('Ctrl Pts',(-7.0429061,3.073105688,1.765073048));
#101325=CARTESIAN_POINT('Ctrl Pts',(-6.926406962,3.007781414,2.141818525));
#101326=CARTESIAN_POINT('',(-7.31258935489774,3.13852541976228,1.6661441837052));
#101327=CARTESIAN_POINT('Origin',(0.186318504438061,3.08928605858041,-0.0505501868150156));
#101328=CARTESIAN_POINT('',(-7.21522192883811,3.13852541968788,1.5220292267485));
#101329=CARTESIAN_POINT('Origin',(4.38017677684144E-14,3.22948687199956,
-7.3075226425523E-14));
#101330=CARTESIAN_POINT('',(-7.16465389455188,3.2284042702292,2.21759657501191));
#101331=CARTESIAN_POINT('Origin',(0.175002196689876,3.08929950069257,-0.0774057478759155));
#101332=CARTESIAN_POINT('Ctrl Pts',(-7.31258937356945,3.13852541968788,
1.6661441929711));
#101333=CARTESIAN_POINT('Ctrl Pts',(-7.25914550000535,3.176642188,1.90070563800849));
#101334=CARTESIAN_POINT('Ctrl Pts',(-7.19077917900507,3.214285714,2.13135984800866));
#101335=CARTESIAN_POINT('Ctrl Pts',(-7.17797556110879,3.22133557899793,
2.17455667813255));
#101336=CARTESIAN_POINT('Ctrl Pts',(-7.16465389719845,3.22840426981355,
2.21759656650944));
#101337=CARTESIAN_POINT('Ctrl Pts',(-7.490948515,3.007773793,0.368361701));
#101338=CARTESIAN_POINT('Ctrl Pts',(-7.470800368,3.07352872,0.778091405));
#101339=CARTESIAN_POINT('Ctrl Pts',(-7.406084436,3.138525418,1.183179329));
#101340=CARTESIAN_POINT('Ctrl Pts',(-7.4054401068863,3.13917254249503,1.18721249262722));
#101341=CARTESIAN_POINT('Ctrl Pts',(-7.40479577777259,3.13981966699007,
1.19124565625443));
#101342=CARTESIAN_POINT('Ctrl Pts',(-7.225677168,3.007773793,0.59337127));
#101343=CARTESIAN_POINT('Ctrl Pts',(-7.193221754,3.07352872,0.988591523));
#101344=CARTESIAN_POINT('Ctrl Pts',(-7.117854477,3.138525418,1.377914237));
#101345=CARTESIAN_POINT('Ctrl Pts',(-7.117104100249,3.13917254249503,1.38179043798336));
#101346=CARTESIAN_POINT('Ctrl Pts',(-7.11635372349801,3.13981966699007,
1.38566663896671));
#101347=CARTESIAN_POINT('',(-7.4060844343901,3.13852541850726,1.18317932687253));
#101348=CARTESIAN_POINT('',(-7.26196945802254,3.13852541943002,1.28054677436567));
#101349=CARTESIAN_POINT('',(-7.47442535668232,3.0479705732519,0.618842199152955));
#101350=CARTESIAN_POINT('Origin',(0.188826312889078,2.94648211665553,0.000683638074364806));
#101351=CARTESIAN_POINT('Ctrl Pts',(-7.22528795810141,3.00855922362978,
0.598092045178342));
#101352=CARTESIAN_POINT('Ctrl Pts',(-7.26675357867071,3.01545478683311,
0.601505266195231));
#101353=CARTESIAN_POINT('Ctrl Pts',(-7.30827047911143,3.02218156077703,
0.604944228025243));
#101354=CARTESIAN_POINT('Ctrl Pts',(-7.39130254515032,3.03530792014544,
0.611861024277268));
#101355=CARTESIAN_POINT('Ctrl Pts',(-7.43286504331963,3.04171498176303,
0.615342804424618));
#101356=CARTESIAN_POINT('Ctrl Pts',(-7.47442535151781,3.0479705733117,0.618842193790382));
#101357=CARTESIAN_POINT('Ctrl Pts',(-7.49985684282223,3.13983235804358,
0.0470505078652194));
#101358=CARTESIAN_POINT('Ctrl Pts',(-7.49982685141112,3.13917888802179,
0.0511253094326098));
#101359=CARTESIAN_POINT('Ctrl Pts',(-7.49979686,3.138525418,0.055200111));
#101360=CARTESIAN_POINT('Ctrl Pts',(-7.496794381,3.073105688,0.463133772));
#101361=CARTESIAN_POINT('Ctrl Pts',(-7.449563353,3.007781414,0.868335101));
#101362=CARTESIAN_POINT('Ctrl Pts',(-7.24745341654421,3.13983235804358,
-0.192304556630875));
#101363=CARTESIAN_POINT('Ctrl Pts',(-7.2475536207721,3.13917888802179,-0.188366749815437));
#101364=CARTESIAN_POINT('Ctrl Pts',(-7.247653825,3.138525418,-0.184428943));
#101365=CARTESIAN_POINT('Ctrl Pts',(-7.25768540000001,3.073105688,0.209789996));
#101366=CARTESIAN_POINT('Ctrl Pts',(-7.224899088,3.007781414,0.602771245));
#101367=CARTESIAN_POINT('',(-7.49979682771917,3.13852541980542,0.0552001049644113));
#101368=CARTESIAN_POINT('Origin',(0.192829366040071,3.08928604866555,-0.00931538846567845));
#101369=CARTESIAN_POINT('',(-7.37372534259178,3.13852541968788,-0.0646144055263606));
#101370=CARTESIAN_POINT('Origin',(-4.03323208164608E-14,3.22948687200056,
9.69378386155711E-14));
#101371=CARTESIAN_POINT('',(-7.47386597982596,3.22840427019247,0.625561598002911));
#101372=CARTESIAN_POINT('Origin',(0.187550563655007,3.08929957882852,-0.0379757253992395));
#101373=CARTESIAN_POINT('Ctrl Pts',(-7.49979684818555,3.13852541968788,
0.0552001104991303));
#101374=CARTESIAN_POINT('Ctrl Pts',(-7.49802624000704,3.176642188,0.295766492007143));
#101375=CARTESIAN_POINT('Ctrl Pts',(-7.48084212200681,3.214285714,0.535724874007362));
#101376=CARTESIAN_POINT('Ctrl Pts',(-7.47762388722127,3.22133557897867,
0.580664185511631));
#101377=CARTESIAN_POINT('Ctrl Pts',(-7.47386598048774,3.22840426981254,
0.625561589035954));
#101378=CARTESIAN_POINT('Ctrl Pts',(-7.395001179,3.007773793,-1.250582891));
#101379=CARTESIAN_POINT('Ctrl Pts',(-7.463403859,3.07352872,-0.846101184));
#101380=CARTESIAN_POINT('Ctrl Pts',(-7.487282879,3.138525418,-0.436571978));
#101381=CARTESIAN_POINT('Ctrl Pts',(-7.48752062490456,3.13917254249503,
-0.432494595782302));
#101382=CARTESIAN_POINT('Ctrl Pts',(-7.48775837080912,3.13981966699007,
-0.428417213564603));
#101383=CARTESIAN_POINT('Ctrl Pts',(-7.184302134,3.007773793,-0.973808422));
#101384=CARTESIAN_POINT('Ctrl Pts',(-7.237566182,3.07352872,-0.580851245));
#101385=CARTESIAN_POINT('Ctrl Pts',(-7.247653825,3.138525418,-0.184428943));
#101386=CARTESIAN_POINT('Ctrl Pts',(-7.24775426026954,3.13917254249503,
-0.180482056621221));
#101387=CARTESIAN_POINT('Ctrl Pts',(-7.24785469553907,3.13981966699007,
-0.176535170242441));
#101388=CARTESIAN_POINT('',(-7.48728287696554,3.13852541850724,-0.436571979715327));
#101389=CARTESIAN_POINT('',(-7.36746835163082,3.13852541943002,-0.310500469259762));
#101390=CARTESIAN_POINT('',(-7.43271022601071,3.0479705733026,-1.0024064970043));
#101391=CARTESIAN_POINT('Origin',(0.184264765153066,2.94648210271064,0.0412597353598802));
#101392=CARTESIAN_POINT('Ctrl Pts',(-7.18493685111983,3.00855922368414,
-0.969114347424904));
#101393=CARTESIAN_POINT('Ctrl Pts',(-7.22616677032159,3.01545478688936,
-0.974694808421183));
#101394=CARTESIAN_POINT('Ctrl Pts',(-7.26745230375002,3.02218156080068,
-0.980261154022604));
#101395=CARTESIAN_POINT('Ctrl Pts',(-7.35003003322002,3.03530792018507,
-0.991355508549004));
#101396=CARTESIAN_POINT('Ctrl Pts',(-7.39136930315834,3.04171498180619,
-0.996889839063651));
#101397=CARTESIAN_POINT('Ctrl Pts',(-7.43271021980434,3.04797057336331,
-1.00240650126442));
#101398=CARTESIAN_POINT('Ctrl Pts',(-7.33462882668321,3.13983235804358,
-1.56629703347738));
#101399=CARTESIAN_POINT('Ctrl Pts',(-7.33547549834161,3.13917888802179,
-1.56231105123869));
#101400=CARTESIAN_POINT('Ctrl Pts',(-7.33632217,3.138525418,-1.558325069));
#101401=CARTESIAN_POINT('Ctrl Pts',(-7.421083566,3.073105688,-1.159283226));
#101402=CARTESIAN_POINT('Ctrl Pts',(-7.462063081,3.007781414,-0.753402005));
#101403=CARTESIAN_POINT('Ctrl Pts',(-7.03667218785752,3.13983235804358,
-1.74579683426311));
#101404=CARTESIAN_POINT('Ctrl Pts',(-7.03761656142876,3.13917888802179,
-1.74197263213155));
#101405=CARTESIAN_POINT('Ctrl Pts',(-7.038560935,3.138525418,-1.73814843));
#101406=CARTESIAN_POINT('Ctrl Pts',(-7.133103396,3.073105688,-1.355302603));
#101407=CARTESIAN_POINT('Ctrl Pts',(-7.185562962,3.007781414,-0.964460949));
#101408=CARTESIAN_POINT('',(-7.33632213717586,3.13852541980608,-1.55832506796128));
#101409=CARTESIAN_POINT('Origin',(0.190323629021206,3.08928601948903,0.0323550041314696));
#101410=CARTESIAN_POINT('',(-7.18744155484115,3.13852541968788,-1.64823673929096));
#101411=CARTESIAN_POINT('Origin',(-6.5746019739521E-13,3.22948687199956,
-2.0491421059976E-14));
#101412=CARTESIAN_POINT('',(-7.43360839863754,3.2284042701966,-0.995723944406123));
#101413=CARTESIAN_POINT('Origin',(0.191329551313522,3.08929953639508,0.00322996651958354));
#101414=CARTESIAN_POINT('Ctrl Pts',(-7.33632215835401,3.13852541968788,
-1.55832506694945));
#101415=CARTESIAN_POINT('Ctrl Pts',(-7.38630760700842,3.176642188,-1.32300236499454));
#101416=CARTESIAN_POINT('Ctrl Pts',(-7.42110920300824,3.214285714,-1.08495999999427));
#101417=CARTESIAN_POINT('Ctrl Pts',(-7.42762683215621,3.22133557897501,
-1.04037951929082));
#101418=CARTESIAN_POINT('Ctrl Pts',(-7.43360839747068,3.22840426981253,
-0.995723953228806));
#101419=CARTESIAN_POINT('Ctrl Pts',(-6.953271806,3.007773793,-2.811051617));
#101420=CARTESIAN_POINT('Ctrl Pts',(-7.10702688,3.07352872,-2.430731022));
#101421=CARTESIAN_POINT('Ctrl Pts',(-7.218384296,3.138525418,-2.035909664));
#101422=CARTESIAN_POINT('Ctrl Pts',(-7.2194930001929,3.13917254249503,-2.03197871704752));
#101423=CARTESIAN_POINT('Ctrl Pts',(-7.2206017043858,3.13981966699007,-2.02804777009504));
#101424=CARTESIAN_POINT('Ctrl Pts',(-6.806997118,3.007773793,-2.495453915));
#101425=CARTESIAN_POINT('Ctrl Pts',(-6.943490059,3.07352872,-2.123134053));
#101426=CARTESIAN_POINT('Ctrl Pts',(-7.038560935,3.138525418,-1.73814843));
#101427=CARTESIAN_POINT('Ctrl Pts',(-7.03950748604824,3.13917254249503,
-1.73431541025369));
#101428=CARTESIAN_POINT('Ctrl Pts',(-7.04045403709647,3.13981966699007,
-1.73048239050737));
#101429=CARTESIAN_POINT('',(-7.21838429364368,3.13852541850724,-2.03590966522802));
#101430=CARTESIAN_POINT('',(-7.12847261325636,3.13852541943002,-1.8870290554756));
#101431=CARTESIAN_POINT('',(-7.04344982493227,3.04797057330757,-2.57678377911017));
#101432=CARTESIAN_POINT('Origin',(0.17108717423595,2.94648207320262,0.0799066117954211));
#101433=CARTESIAN_POINT('Ctrl Pts',(-6.8086260823428,3.00855922361795,-2.49100602981249));
#101434=CARTESIAN_POINT('Ctrl Pts',(-6.84769243471522,3.01545478683609,
-2.5053192366488));
#101435=CARTESIAN_POINT('Ctrl Pts',(-6.886816135416,3.02218156075082,-2.51963061349986));
#101436=CARTESIAN_POINT('Ctrl Pts',(-6.96507828505715,3.03530792016389,
-2.54821735912404));
#101437=CARTESIAN_POINT('Ctrl Pts',(-7.00426134831103,3.04171498179865,
-2.56250902116351));
#101438=CARTESIAN_POINT('Ctrl Pts',(-7.04344981795141,3.04797057336821,
-2.57678378194846));
#101439=CARTESIAN_POINT('Ctrl Pts',(-6.82644171740222,3.13983235804358,
-3.10640626662274));
#101440=CARTESIAN_POINT('Ctrl Pts',(-6.82812546270111,3.13917888802179,
-3.10269548381137));
#101441=CARTESIAN_POINT('Ctrl Pts',(-6.829809208,3.138525418,-3.098984701));
#101442=CARTESIAN_POINT('Ctrl Pts',(-6.99837113000001,3.073105688,-2.727493429));
#101443=CARTESIAN_POINT('Ctrl Pts',(-7.125645032,3.007781414,-2.33991087));
#101444=CARTESIAN_POINT('Ctrl Pts',(-6.49686398890001,3.13983235804358,
-3.21765759201994));
#101445=CARTESIAN_POINT('Ctrl Pts',(-6.49860837395001,3.13917888802179,
-3.21412581000997));
#101446=CARTESIAN_POINT('Ctrl Pts',(-6.50035275900001,3.138525418,-3.210594028));
#101447=CARTESIAN_POINT('Ctrl Pts',(-6.674985405,3.073105688,-2.857022758));
#101448=CARTESIAN_POINT('Ctrl Pts',(-6.81023789800001,3.007781414,-2.486596021));
#101449=CARTESIAN_POINT('',(-6.82980917617189,3.13852541980549,-3.09898469292473));
#101450=CARTESIAN_POINT('Origin',(0.178918748265815,3.08928601856382,0.0725125769354081));
#101451=CARTESIAN_POINT('',(-6.66508098798106,3.13852541968788,-3.15478935503292));
#101452=CARTESIAN_POINT('Origin',(-6.49653941753314E-13,3.22948687199978,
-2.65846372693446E-13));
#101453=CARTESIAN_POINT('',(-7.04576355038251,3.22840427021457,-2.5704505416214));
#101454=CARTESIAN_POINT('Origin',(0.186162053929123,3.08929956872846,0.0442846701300559));
#101455=CARTESIAN_POINT('Ctrl Pts',(-6.82980919706723,3.13852541968788,
-3.09898469649379));
#101456=CARTESIAN_POINT('Ctrl Pts',(-6.92921343900949,3.176642188,-2.87990910299644));
#101457=CARTESIAN_POINT('Ctrl Pts',(-7.01437346500937,3.214285714,-2.65491334999614));
#101458=CARTESIAN_POINT('Ctrl Pts',(-7.03032220117711,3.2213355789857,-2.61277623396586));
#101459=CARTESIAN_POINT('Ctrl Pts',(-7.04576354739409,3.22840426981256,
-2.57045054996743));
#101460=CARTESIAN_POINT('Ctrl Pts',(-6.18641517199999,3.007773793,-4.240078693));
#101461=CARTESIAN_POINT('Ctrl Pts',(-6.418333224,3.07352872,-3.901702578));
#101462=CARTESIAN_POINT('Ctrl Pts',(-6.611962085,3.138525418,-3.540050477));
#101463=CARTESIAN_POINT('Ctrl Pts',(-6.61388990568557,3.13917254249503,
-3.53644977203438));
#101464=CARTESIAN_POINT('Ctrl Pts',(-6.61581772637116,3.13981966699007,
-3.53284906706876));
#101465=CARTESIAN_POINT('Ctrl Pts',(-6.111404481,3.007773793,-3.900414756));
#101466=CARTESIAN_POINT('Ctrl Pts',(-6.324744057,3.07352872,-3.566141474));
#101467=CARTESIAN_POINT('Ctrl Pts',(-6.50035275900001,3.138525418,-3.210594028));
#101468=CARTESIAN_POINT('Ctrl Pts',(-6.50210116616686,3.13917254249503,
-3.20705410261097));
#101469=CARTESIAN_POINT('Ctrl Pts',(-6.50384957333372,3.13981966699007,
-3.20351417722194));
#101470=CARTESIAN_POINT('',(-6.61196208242836,3.13852541850727,-3.54005047773679));
#101471=CARTESIAN_POINT('',(-6.55615741798682,3.13852541943002,-3.37532226029513));
#101472=CARTESIAN_POINT('',(-6.32484553890956,3.04797057324976,-4.030673515416));
#101473=CARTESIAN_POINT('Origin',(0.149909447659728,2.94648211908025,0.114816963127455));
#101474=CARTESIAN_POINT('Ctrl Pts',(-6.11395152485902,3.00855922359023,
-3.89642103948571));
#101475=CARTESIAN_POINT('Ctrl Pts',(-6.14902761123259,3.01545478679443,
-3.91879772231694));
#101476=CARTESIAN_POINT('Ctrl Pts',(-6.18416009886821,3.02218156074056,
-3.94118494628396));
#101477=CARTESIAN_POINT('Ctrl Pts',(-6.2544472177817,3.0353079201198,-3.98592739811759));
#101478=CARTESIAN_POINT('Ctrl Pts',(-6.28964191806543,3.04171498174985,
-4.00830812928556));
#101479=CARTESIAN_POINT('Ctrl Pts',(-6.32484553155734,3.0479705733095,-4.03067351655581));
#101480=CARTESIAN_POINT('Ctrl Pts',(-5.9990577812363,3.13983235804358,-4.50126339560797));
#101481=CARTESIAN_POINT('Ctrl Pts',(-6.00149987011815,3.13917888802179,
-4.49800132430398));
#101482=CARTESIAN_POINT('Ctrl Pts',(-6.003941959,3.138525418,-4.494739253));
#101483=CARTESIAN_POINT('Ctrl Pts',(-6.248422639,3.073105688,-4.168169071));
#101484=CARTESIAN_POINT('Ctrl Pts',(-6.456039741,3.007781414,-3.817008103));
#101485=CARTESIAN_POINT('Ctrl Pts',(-5.65326964992618,3.13983235804358,
-4.53906425736617));
#101486=CARTESIAN_POINT('Ctrl Pts',(-5.6557324809631,3.13917888802179,-4.53599003768308));
#101487=CARTESIAN_POINT('Ctrl Pts',(-5.658195312,3.138525418,-4.532915818));
#101488=CARTESIAN_POINT('Ctrl Pts',(-5.904752516,3.073105688,-4.225151705));
#101489=CARTESIAN_POINT('Ctrl Pts',(-6.11647367900001,3.007781414,-3.892460627));
#101490=CARTESIAN_POINT('',(-6.00394192964676,3.13852541980585,-4.49473923827281));
#101491=CARTESIAN_POINT('Origin',(0.159147628181055,3.08928603080669,0.10927948382582));
#101492=CARTESIAN_POINT('',(-5.83106864191144,3.13852541968788,-4.51382752721755));
#101493=CARTESIAN_POINT('Origin',(-2.86663054405167E-13,3.22948687200044,
-1.5330618718945E-13));
#101494=CARTESIAN_POINT('',(-6.32846662957753,3.22840427021542,-4.02498572848737));
#101495=CARTESIAN_POINT('Origin',(0.172289535163268,3.08929953212073,0.0832684844022252));
#101496=CARTESIAN_POINT('Ctrl Pts',(-6.00394194929151,3.13852541968788,
-4.49473924624893));
#101497=CARTESIAN_POINT('Ctrl Pts',(-6.14811695100994,3.176642188,-4.30215449199858));
#101498=CARTESIAN_POINT('Ctrl Pts',(-6.27965341900987,3.214285714,-4.10072590299827));
#101499=CARTESIAN_POINT('Ctrl Pts',(-6.30428751723109,3.22133557899334,
-4.0630024360247));
#101500=CARTESIAN_POINT('Ctrl Pts',(-6.32846662470299,3.22840426981355,
-4.02498573602417));
#101501=CARTESIAN_POINT('Ctrl Pts',(-5.13028864,3.007773793,-5.47084440199999));
#101502=CARTESIAN_POINT('Ctrl Pts',(-5.429525439,3.07352872,-5.190234859));
#101503=CARTESIAN_POINT('Ctrl Pts',(-5.696371877,3.138525418,-4.878662465));
#101504=CARTESIAN_POINT('Ctrl Pts',(-5.69902867144889,3.13917254249503,
-4.8755603669806));
#101505=CARTESIAN_POINT('Ctrl Pts',(-5.70168546589777,3.13981966699007,
-4.87245826896118));
#101506=CARTESIAN_POINT('Ctrl Pts',(-5.130049363,3.007773793,-5.122996538));
#101507=CARTESIAN_POINT('Ctrl Pts',(-5.410260054,3.07352872,-4.842400082));
#101508=CARTESIAN_POINT('Ctrl Pts',(-5.658195312,3.138525418,-4.532915818));
#101509=CARTESIAN_POINT('Ctrl Pts',(-5.66066382168697,3.13917254249503,
-4.5298345099609));
#101510=CARTESIAN_POINT('Ctrl Pts',(-5.66313233137395,3.13981966699007,
-4.52675320192181));
#101511=CARTESIAN_POINT('',(-5.69637187435097,3.13852541850723,-4.8786624651115));
#101512=CARTESIAN_POINT('',(-5.67728358890492,3.13852541943002,-4.70578914825017));
#101513=CARTESIAN_POINT('',(-5.31049850488852,3.04797057322864,-5.29609343840933));
#101514=CARTESIAN_POINT('Origin',(0.121722443726788,2.9464820914821,0.144358776216413));
#101515=CARTESIAN_POINT('Ctrl Pts',(-5.13339538944628,3.00855922360106,
-5.11964373170498));
#101516=CARTESIAN_POINT('Ctrl Pts',(-5.16284109107939,3.01545478677039,
-5.14903758173383));
#101517=CARTESIAN_POINT('Ctrl Pts',(-5.1923396093951,3.02218156072343,-5.17845385122894));
#101518=CARTESIAN_POINT('Ctrl Pts',(-5.25136514995679,3.03530792008805,
-5.23725990226701));
#101519=CARTESIAN_POINT('Ctrl Pts',(-5.28092582206647,3.04171498172015,
-5.26668320461477));
#101520=CARTESIAN_POINT('Ctrl Pts',(-5.31049849750202,3.04797057328804,
-5.29609343790255));
#101521=CARTESIAN_POINT('Ctrl Pts',(-4.89116456977673,3.13983235804358,
-5.68564645093098));
#101522=CARTESIAN_POINT('Ctrl Pts',(-4.89425081288837,3.13917888802179,
-5.68298562196549));
#101523=CARTESIAN_POINT('Ctrl Pts',(-4.897337056,3.138525418,-5.68032479300001));
#101524=CARTESIAN_POINT('Ctrl Pts',(-5.20630485,3.073105688,-5.41394576));
#101525=CARTESIAN_POINT('Ctrl Pts',(-5.484557207,3.007781414,-5.11562628));
#101526=CARTESIAN_POINT('Ctrl Pts',(-4.54533470543984,3.13983235804358,
-5.64822932251851));
#101527=CARTESIAN_POINT('Ctrl Pts',(-4.54840082321992,3.13917888802179,
-5.64575641225926));
#101528=CARTESIAN_POINT('Ctrl Pts',(-4.551466941,3.138525418,-5.643283502));
#101529=CARTESIAN_POINT('Ctrl Pts',(-4.85841996200001,3.073105688,-5.395717254));
#101530=CARTESIAN_POINT('Ctrl Pts',(-5.136709949,3.007781414,-5.1163181));
#101531=CARTESIAN_POINT('',(-4.8973370310442,3.13852541976208,-5.68032477216621));
#101532=CARTESIAN_POINT('Origin',(0.131934875247602,3.08928601505222,0.140936509631236));
#101533=CARTESIAN_POINT('',(-4.72440200654202,3.13852541968788,-5.66180414078946));
#101534=CARTESIAN_POINT('Origin',(8.46978737145676E-13,3.22948687200067,
8.92515228390067E-13));
#101535=CARTESIAN_POINT('',(-5.31525764263672,3.22840427020599,-5.29131705602687));
#101536=CARTESIAN_POINT('Origin',(0.150361561841226,3.08929951791396,0.118359186089775));
#101537=CARTESIAN_POINT('Ctrl Pts',(-4.89733704796982,3.13852541968788,
-5.68032478431973));
#101538=CARTESIAN_POINT('Ctrl Pts',(-5.07954134901011,3.176642188,-5.52323591800075));
#101539=CARTESIAN_POINT('Ctrl Pts',(-5.25130375901012,3.214285714,-5.35479307000043));
#101540=CARTESIAN_POINT('Ctrl Pts',(-5.28347135607228,3.22133557898738,
-5.32324715960407));
#101541=CARTESIAN_POINT('Ctrl Pts',(-5.3152576362352,3.22840426981355,-5.291317062339));
#101542=CARTESIAN_POINT('Ctrl Pts',(-3.834275513,3.007773793,-6.445799508));
#101543=CARTESIAN_POINT('Ctrl Pts',(-4.186839079,3.07352872,-6.236077526));
#101544=CARTESIAN_POINT('Ctrl Pts',(-4.51442565,3.138525418,-5.989153617));
#101545=CARTESIAN_POINT('Ctrl Pts',(-4.51768718944525,3.13917254249503,
-5.98669517657394));
#101546=CARTESIAN_POINT('Ctrl Pts',(-4.52094872889051,3.13981966699007,
-5.98423673614789));
#101547=CARTESIAN_POINT('Ctrl Pts',(-3.908818839,3.007773793,-6.106032696));
#101548=CARTESIAN_POINT('Ctrl Pts',(-4.242798303,3.07352872,-5.892233444));
#101549=CARTESIAN_POINT('Ctrl Pts',(-4.551466941,3.138525418,-5.643283502));
#101550=CARTESIAN_POINT('Ctrl Pts',(-4.55454012844867,3.13917254249503,
-5.64080488984796));
#101551=CARTESIAN_POINT('Ctrl Pts',(-4.55761331589734,3.13981966699007,
-5.63832627769592));
#101552=CARTESIAN_POINT('',(-4.51442564736557,3.13852541850725,-5.98915361657509));
#101553=CARTESIAN_POINT('',(-4.53294628858464,3.13852541943002,-5.81621856488957));
#101554=CARTESIAN_POINT('',(-4.04783846321783,3.04797057326586,-6.3138739184838));
#101555=CARTESIAN_POINT('Origin',(0.0878437618876299,2.94648209802678,0.167150436905271));
#101556=CARTESIAN_POINT('Ctrl Pts',(-3.91280739158268,3.008559223625,-6.10347757308111));
#101557=CARTESIAN_POINT('Ctrl Pts',(-3.93524586011906,3.01545478681085,
-6.138514166815));
#101558=CARTESIAN_POINT('Ctrl Pts',(-3.95773109096271,3.0221815607577,-6.17358400974169));
#101559=CARTESIAN_POINT('Ctrl Pts',(-4.00273508442949,3.03530792013278,
-6.24370395450373));
#101560=CARTESIAN_POINT('Ctrl Pts',(-4.02527950415133,3.04171498176201,
-6.27879402706656));
#101561=CARTESIAN_POINT('Ctrl Pts',(-4.04783845603459,3.04797057332588,
-6.31387391645986));
#101562=CARTESIAN_POINT('Ctrl Pts',(-3.55456593991965,3.13983235804358,
-6.60417499745422));
#101563=CARTESIAN_POINT('Ctrl Pts',(-3.55815202795982,3.13917888802179,
-6.60223982822711));
#101564=CARTESIAN_POINT('Ctrl Pts',(-3.561738116,3.138525418,-6.600304659));
#101565=CARTESIAN_POINT('Ctrl Pts',(-3.920746033,3.073105688,-6.406572362));
#101566=CARTESIAN_POINT('Ctrl Pts',(-4.256622874,3.007781414,-6.175043458));
#101567=CARTESIAN_POINT('Ctrl Pts',(-3.22486496249061,3.13983235804358,
-6.49328946261242));
#101568=CARTESIAN_POINT('Ctrl Pts',(-3.2283909987453,3.13917888802179,-6.49153349230621));
#101569=CARTESIAN_POINT('Ctrl Pts',(-3.231917035,3.138525418,-6.48977752200001));
#101570=CARTESIAN_POINT('Ctrl Pts',(-3.58491309,3.073105688,-6.313985061));
#101571=CARTESIAN_POINT('Ctrl Pts',(-3.916759371,3.007781414,-6.100942225));
#101572=CARTESIAN_POINT('',(-3.56173809610214,3.13852541976265,-6.60030463329241));
#101573=CARTESIAN_POINT('Origin',(0.0985531836936841,3.08928598123718,0.166003673652068));
#101574=CARTESIAN_POINT('',(-3.39682758479658,3.13852541968788,-6.54504108567515));
#101575=CARTESIAN_POINT('Origin',(5.42101086242752E-13,3.22948687200056,
8.91647866652079E-13));
#101576=CARTESIAN_POINT('',(-4.05351311580907,3.22840427022695,-6.31023227897596));
#101577=CARTESIAN_POINT('Origin',(0.121402364643847,3.08929956194483,0.147915157976117));
#101578=CARTESIAN_POINT('Ctrl Pts',(-3.56173811002333,3.13852541968788,
-6.60030464879634));
#101579=CARTESIAN_POINT('Ctrl Pts',(-3.7734520380093,3.176642188,-6.4860569710028));
#101580=CARTESIAN_POINT('Ctrl Pts',(-3.97740897200938,3.214285714,-6.35847606500249));
#101581=CARTESIAN_POINT('Ctrl Pts',(-4.01560594677838,3.22133557899676,
-6.33458276279003));
#101582=CARTESIAN_POINT('Ctrl Pts',(-4.05351310833931,3.22840426981258,
-6.31023228380055));
#101583=CARTESIAN_POINT('Ctrl Pts',(-2.358975924,3.007773793,-7.11935619199999));
#101584=CARTESIAN_POINT('Ctrl Pts',(-2.748380777,3.07352872,-6.990328138));
#101585=CARTESIAN_POINT('Ctrl Pts',(-3.121389897,3.138525418,-6.819598603));
#101586=CARTESIAN_POINT('Ctrl Pts',(-3.12510367548184,3.13917254249503,
-6.8178987741237));
#101587=CARTESIAN_POINT('Ctrl Pts',(-3.12881745396368,3.13981966699007,
-6.81619894524741));
#101588=CARTESIAN_POINT('Ctrl Pts',(-2.50481629,3.007773793,-6.803557551));
#101589=CARTESIAN_POINT('Ctrl Pts',(-2.876948019,3.07352872,-6.66655252));
#101590=CARTESIAN_POINT('Ctrl Pts',(-3.231917035,3.138525418,-6.489777522));
#101591=CARTESIAN_POINT('Ctrl Pts',(-3.23545120138537,3.13917254249503,
-6.48801750287848));
#101592=CARTESIAN_POINT('Ctrl Pts',(-3.23898536777074,3.13981966699007,
-6.48625748375697));
#101593=CARTESIAN_POINT('',(-3.12138989451244,3.13852541850726,-6.81959860202427));
#101594=CARTESIAN_POINT('',(-3.17665345808772,3.13852541943002,-6.65468806627697));
#101595=CARTESIAN_POINT('',(-2.59590599360655,3.0479705733211,-7.03642467113093));
#101596=CARTESIAN_POINT('Origin',(0.0498576734522127,2.94648212933595,0.182126481435873));
#101597=CARTESIAN_POINT('Ctrl Pts',(-2.50926086840672,3.00855922369567,
-6.80191958692094));
#101598=CARTESIAN_POINT('Ctrl Pts',(-2.52364290616179,3.01545478692602,
-6.84096065214121));
#101599=CARTESIAN_POINT('Ctrl Pts',(-2.53806346503707,3.02218156078119,
-6.88004424097906));
#101600=CARTESIAN_POINT('Ctrl Pts',(-2.56694157478864,3.03530792019364,
-6.95819934879997));
#101601=CARTESIAN_POINT('Ctrl Pts',(-2.58141559011017,3.04171498182181,
-6.99731541877659));
#101602=CARTESIAN_POINT('Ctrl Pts',(-2.59590598689054,3.04797057338195,
-7.03642466765963));
#101603=CARTESIAN_POINT('Ctrl Pts',(-2.05175975706096,3.13983235804358,
-7.2138996612507));
#101604=CARTESIAN_POINT('Ctrl Pts',(-2.05567800853048,3.13917888802179,
-7.21278063812536));
#101605=CARTESIAN_POINT('Ctrl Pts',(-2.05959626,3.138525418,-7.211661615));
#101606=CARTESIAN_POINT('Ctrl Pts',(-2.451857488,3.073105688,-7.099634761));
#101607=CARTESIAN_POINT('Ctrl Pts',(-2.829653587,3.007781414,-6.945722466));
#101608=CARTESIAN_POINT('Ctrl Pts',(-1.75360411761002,3.13983235804358,
-7.03473060324848));
#101609=CARTESIAN_POINT('Ctrl Pts',(-1.75742519880501,3.13917888802179,
-7.03377368012423));
#101610=CARTESIAN_POINT('Ctrl Pts',(-1.76124628,3.138525418,-7.032816757));
#101611=CARTESIAN_POINT('Ctrl Pts',(-2.143779666,3.073105688,-6.937017944));
#101612=CARTESIAN_POINT('Ctrl Pts',(-2.513665477,3.007781414,-6.800293072));
#101613=CARTESIAN_POINT('',(-2.05959624554176,3.13852541980597,-7.21166158551047));
#101614=CARTESIAN_POINT('Origin',(0.0605632130569449,3.08928603561543,0.183308723200907));
#101615=CARTESIAN_POINT('',(-1.91042128011643,3.13852541968788,-7.12223918328643));
#101616=CARTESIAN_POINT('Origin',(-1.12106504635001E-13,3.22948687199956,
-3.78603398631938E-13));
#101617=CARTESIAN_POINT('',(-2.60223082099891,3.22840427021944,-7.03408805428349));
#101618=CARTESIAN_POINT('Origin',(0.0867666093238001,3.0892995251928,0.170554746126368));
#101619=CARTESIAN_POINT('Ctrl Pts',(-2.05959625635551,3.13852541968788,
-7.21166160374947));
#101620=CARTESIAN_POINT('Ctrl Pts',(-2.29092030400738,3.176642188,-7.14559720900411));
#101621=CARTESIAN_POINT('Ctrl Pts',(-2.5175349620075,3.214285714,-7.06484378600387));
#101622=CARTESIAN_POINT('Ctrl Pts',(-2.55997526625953,3.2213355789953,-7.04972031639188));
#101623=CARTESIAN_POINT('Ctrl Pts',(-2.60223081258653,3.22840426981265,
-7.03408805734967));
#101624=CARTESIAN_POINT('Ctrl Pts',(-0.773373243,3.007773793,-7.460019693));
#101625=CARTESIAN_POINT('Ctrl Pts',(-1.181411245,3.07352872,-7.417718777));
#101626=CARTESIAN_POINT('Ctrl Pts',(-1.582401422,3.138525418,-7.331166738));
#101627=CARTESIAN_POINT('Ctrl Pts',(-1.586393787363,3.13917254249503,-7.33030500276951));
#101628=CARTESIAN_POINT('Ctrl Pts',(-1.590386152726,3.13981966699007,-7.32944326753902));
#101629=CARTESIAN_POINT('Ctrl Pts',(-0.983691316,3.007773793,-7.18295561700001));
#101630=CARTESIAN_POINT('Ctrl Pts',(-1.376574843,3.07352872,-7.12915100900001));
#101631=CARTESIAN_POINT('Ctrl Pts',(-1.76124628,3.138525418,-7.032816757));
#101632=CARTESIAN_POINT('Ctrl Pts',(-1.76507617162653,3.13917254249503,
-7.03185762744268));
#101633=CARTESIAN_POINT('Ctrl Pts',(-1.76890606325307,3.13981966699007,
-7.03089849788536));
#101634=CARTESIAN_POINT('',(-1.58240141979824,3.13852541850725,-7.33116673650153));
#101635=CARTESIAN_POINT('',(-1.67182384246077,3.13852541943002,-7.18199174948777));
#101636=CARTESIAN_POINT('',(-1.02259184491922,3.04797057332665,-7.42996002711352));
#101637=CARTESIAN_POINT('Origin',(0.00954017391375017,2.94648215635932,
0.188586111446705));
#101638=CARTESIAN_POINT('Ctrl Pts',(-0.98838409649014,3.00855922368921,
-7.18231140053146));
#101639=CARTESIAN_POINT('Ctrl Pts',(-0.994037214996654,3.0154547869579,
-7.22353142049163));
#101640=CARTESIAN_POINT('Ctrl Pts',(-0.999718812719134,3.02218156078833,
-7.26480125048925));
#101641=CARTESIAN_POINT('Ctrl Pts',(-1.01112073015354,3.0353079202144,-7.34733707545125));
#101642=CARTESIAN_POINT('Ctrl Pts',(-1.01684755219726,3.04171498183755,
-7.38865011893273));
#101643=CARTESIAN_POINT('Ctrl Pts',(-1.02259183909231,3.04797057338766,
-7.42996002228574));
#101644=CARTESIAN_POINT('Ctrl Pts',(-0.453015568348983,3.13983235804358,
-7.48631039345565));
#101645=CARTESIAN_POINT('Ctrl Pts',(-0.457082770174492,3.13917888802179,
-7.48605984072783));
#101646=CARTESIAN_POINT('Ctrl Pts',(-0.461149972,3.138525418,-7.485809288));
#101647=CARTESIAN_POINT('Ctrl Pts',(-0.868322813,3.073105688,-7.46072613));
#101648=CARTESIAN_POINT('Ctrl Pts',(-1.270372842,3.007781414,-7.391627212));
#101649=CARTESIAN_POINT('Ctrl Pts',(-0.200346692749638,3.13983235804358,
-7.24723556060148));
#101650=CARTESIAN_POINT('Ctrl Pts',(-0.204284149374819,3.13917888802179,
-7.24712242930074));
#101651=CARTESIAN_POINT('Ctrl Pts',(-0.208221606,3.138525418,-7.24700929800001));
#101652=CARTESIAN_POINT('Ctrl Pts',(-0.602405487000001,3.073105688,-7.235683577));
#101653=CARTESIAN_POINT('Ctrl Pts',(-0.99303538,3.007781414,-7.181669773));
#101654=CARTESIAN_POINT('',(-0.461149964227287,3.13852541980534,-7.48580925609884));
#101655=CARTESIAN_POINT('Origin',(0.0197412726344003,3.08928600276568,0.192041965304161));
#101656=CARTESIAN_POINT('',(-0.334685799463248,3.13852541968788,-7.36640929252461));
#101657=CARTESIAN_POINT('Origin',(-3.29326409892472E-14,3.22948687200011,
3.54750950837257E-13));
#101658=CARTESIAN_POINT('',(-1.02927110501602,3.2284042702107,-7.42903768943116));
#101659=CARTESIAN_POINT('Origin',(0.0480737921300024,3.08929955132135,0.185219410294131));
#101660=CARTESIAN_POINT('Ctrl Pts',(-0.461149970859381,3.13852541968788,
-7.48580927622917));
#101661=CARTESIAN_POINT('Ctrl Pts',(-0.701267683007476,3.176642188,-7.47101726400662));
#101662=CARTESIAN_POINT('Ctrl Pts',(-0.93994381500768,3.214285714,-7.44086726300637));
#101663=CARTESIAN_POINT('Ctrl Pts',(-0.984642987471772,3.2213355789848,
-7.43522078275191));
#101664=CARTESIAN_POINT('Ctrl Pts',(-1.02927109619218,3.22840426981355,
-7.42903769066228));
#101665=CARTESIAN_POINT('Ctrl Pts',(0.848391511,3.007773793,-7.451860965));
#101666=CARTESIAN_POINT('Ctrl Pts',(0.440799764,3.07352872,-7.498265129));
#101667=CARTESIAN_POINT('Ctrl Pts',(0.030578384,3.138525418,-7.499937664));
#101668=CARTESIAN_POINT('Ctrl Pts',(0.0264941103129808,3.13917254249503,
-7.49995431620543));
#101669=CARTESIAN_POINT('Ctrl Pts',(0.0224098366259617,3.13981966699007,
-7.49997096841086));
#101670=CARTESIAN_POINT('Ctrl Pts',(0.583429972,3.007773793,-7.226486661));
#101671=CARTESIAN_POINT('Ctrl Pts',(0.188165442,3.07352872,-7.25839832));
#101672=CARTESIAN_POINT('Ctrl Pts',(-0.208221606,3.138525418,-7.247009298));
#101673=CARTESIAN_POINT('Ctrl Pts',(-0.212168141380535,3.13917254249503,
-7.24689590585336));
#101674=CARTESIAN_POINT('Ctrl Pts',(-0.216114676761069,3.13981966699007,
-7.24678251370672));
#101675=CARTESIAN_POINT('',(0.0305783858254823,3.13852541850725,-7.49993766206233));
#101676=CARTESIAN_POINT('',(-0.0888216022330979,3.13852541943002,-7.37347348110561));
#101677=CARTESIAN_POINT('',(0.598537562247386,3.04797057329688,-7.47607870979874));
#101678=CARTESIAN_POINT('Origin',(-0.0312233212322582,2.94648213638327,
0.186228177115241));
#101679=CARTESIAN_POINT('Ctrl Pts',(0.57870841876267,3.00855922356026,-7.22686631446595));
#101680=CARTESIAN_POINT('Ctrl Pts',(0.58204855259275,3.01545478674394,-7.26833788632441));
#101681=CARTESIAN_POINT('Ctrl Pts',(0.585371580930391,3.02218156076013,
-7.30986422746823));
#101682=CARTESIAN_POINT('Ctrl Pts',(0.591978996394136,3.03530792013989,
-7.39292148582055));
#101683=CARTESIAN_POINT('Ctrl Pts',(0.595267147374943,3.04171498178307,
-7.43449975095489));
#101684=CARTESIAN_POINT('Ctrl Pts',(0.59853756682197,3.04797057335751,-7.47607870383028));
#101685=CARTESIAN_POINT('Ctrl Pts',(1.16691112465914,3.13983235804358,-7.40866957357816));
#101686=CARTESIAN_POINT('Ctrl Pts',(1.16288515032957,3.13917888802179,-7.40929920678909));
#101687=CARTESIAN_POINT('Ctrl Pts',(1.158859176,3.138525418,-7.40992884));
#101688=CARTESIAN_POINT('Ctrl Pts',(0.755813673,3.073105688,-7.472962236));
#101689=CARTESIAN_POINT('Ctrl Pts',(0.348309125,3.007781414,-7.491907685));
#101690=CARTESIAN_POINT('Ctrl Pts',(1.36227871992292,3.13983235804358,-7.12086783712926));
#101691=CARTESIAN_POINT('Ctrl Pts',(1.35840899896146,3.13917888802179,-7.12160378756463));
#101692=CARTESIAN_POINT('Ctrl Pts',(1.354539278,3.138525418,-7.122339738));
#101693=CARTESIAN_POINT('Ctrl Pts',(0.967136502,3.073105688,-7.19601668900001));
#101694=CARTESIAN_POINT('Ctrl Pts',(0.574027948,3.007781414,-7.227239578));
#101695=CARTESIAN_POINT('',(1.15885917628989,3.13852541976333,-7.40992880748018));
#101696=CARTESIAN_POINT('Origin',(-0.0220036510827664,3.08928604246497,
0.191796247293505));
#101697=CARTESIAN_POINT('',(1.25669921667914,3.13852541968789,-7.26613429078503));
#101698=CARTESIAN_POINT('Origin',(1.20100801591187E-13,3.22948687200011,
-1.8028113724089E-12));
#101699=CARTESIAN_POINT('',(0.591816183700481,3.22840427021323,-7.47661377888631));
#101700=CARTESIAN_POINT('Origin',(0.00713314255942156,3.08929953360765,
0.191223796675345));
#101701=CARTESIAN_POINT('Ctrl Pts',(1.15885917458283,3.13852541968788,-7.4099288282602));
#101702=CARTESIAN_POINT('Ctrl Pts',(0.921175435994036,3.176642188,-7.44710085400819));
#101703=CARTESIAN_POINT('Ctrl Pts',(0.681598059993781,3.214285714,-7.46896405700799));
#101704=CARTESIAN_POINT('Ctrl Pts',(0.636730102971802,3.22133557898984,
-7.47305858888712));
#101705=CARTESIAN_POINT('Ctrl Pts',(0.591816192611198,3.22840426981315,
-7.47661377814827));
#101706=CARTESIAN_POINT('Ctrl Pts',(2.430486421,3.007773793,-7.0952615));
#101707=CARTESIAN_POINT('Ctrl Pts',(2.042399466,3.07352872,-7.228200938));
#101708=CARTESIAN_POINT('Ctrl Pts',(1.64212838,3.138525418,-7.31801984));
#101709=CARTESIAN_POINT('Ctrl Pts',(1.63814317409917,3.13917254249503,-7.31891410099156));
#101710=CARTESIAN_POINT('Ctrl Pts',(1.63415796819833,3.13981966699007,-7.31980836198311));
#101711=CARTESIAN_POINT('Ctrl Pts',(2.123270722,3.007773793,-6.932115221));
#101712=CARTESIAN_POINT('Ctrl Pts',(1.744107321,3.07352872,-7.048250993));
#101713=CARTESIAN_POINT('Ctrl Pts',(1.354539278,3.138525418,-7.12233973800001));
#101714=CARTESIAN_POINT('Ctrl Pts',(1.35066063445556,3.13917254249503,-7.12307738534472));
#101715=CARTESIAN_POINT('Ctrl Pts',(1.34678199091112,3.13981966699007,-7.12381503268945));
#101716=CARTESIAN_POINT('',(1.64212838139077,3.13852541850725,-7.31801983771826));
#101717=CARTESIAN_POINT('',(1.49833383758464,3.13852541943002,-7.22017978721851));
#101718=CARTESIAN_POINT('',(2.19168001780487,3.04797057328338,-7.1726242606184));
#101719=CARTESIAN_POINT('Origin',(-0.0705268460826172,2.9464821631811,0.175162031611241));
#101720=CARTESIAN_POINT('Ctrl Pts',(2.11874117040445,3.00855922370958,-6.93350099351421));
#101721=CARTESIAN_POINT('Ctrl Pts',(2.13091837590938,3.01545478694813,-6.97328495323188));
#101722=CARTESIAN_POINT('Ctrl Pts',(2.1430906492882,3.02218156082002,-7.01312607782696));
#101723=CARTESIAN_POINT('Ctrl Pts',(2.16739844252111,3.03530792020108,-7.09282110458575));
#101724=CARTESIAN_POINT('Ctrl Pts',(2.1795478163059,3.04171498180817,-7.13272043750306));
#101725=CARTESIAN_POINT('Ctrl Pts',(2.19168002095519,3.04797057334374,-7.17262425381494));
#101726=CARTESIAN_POINT('Ctrl Pts',(2.7322743505124,3.13983235804358,-6.98460759756821));
#101727=CARTESIAN_POINT('Ctrl Pts',(2.7284778537562,3.13917888802179,-6.98608797578411));
#101728=CARTESIAN_POINT('Ctrl Pts',(2.724681357,3.138525418,-6.987568354));
#101729=CARTESIAN_POINT('Ctrl Pts',(2.344609151,3.073105688,-7.135770934));
#101730=CARTESIAN_POINT('Ctrl Pts',(1.950704544,3.007781414,-7.24187488));
#101731=CARTESIAN_POINT('Ctrl Pts',(2.86120549389769,3.13983235804358,-6.661536248119));
#101732=CARTESIAN_POINT('Ctrl Pts',(2.85758445244885,3.13917888802179,-6.6630868680595));
#101733=CARTESIAN_POINT('Ctrl Pts',(2.853963411,3.138525418,-6.664637488));
#101734=CARTESIAN_POINT('Ctrl Pts',(2.491456263,3.073105688,-6.819872058));
#101735=CARTESIAN_POINT('Ctrl Pts',(2.114250367,3.007781414,-6.934871692));
#101736=CARTESIAN_POINT('',(2.72468135066201,3.13852541980582,-6.98756832177496));
#101737=CARTESIAN_POINT('Origin',(-0.0627196471463952,3.08928604481397,
0.182581748066019));
#101738=CARTESIAN_POINT('',(2.78932237430421,3.13852541968788,-6.82610292496196));
#101739=CARTESIAN_POINT('Origin',(-2.31043482956661E-13,3.22948687200044,
7.12971348626468E-13));
#101740=CARTESIAN_POINT('',(2.18523080594797,3.22840427023862,-7.17459171825009));
#101741=CARTESIAN_POINT('Origin',(-0.0341410904281592,3.08929951162922,
0.188286562003838));
#101742=CARTESIAN_POINT('Ctrl Pts',(2.72468135309239,3.13852541968788,-6.98756834283909));
#101743=CARTESIAN_POINT('Ctrl Pts',(2.50054541499605,3.176642188,-7.07496628600903));
#101744=CARTESIAN_POINT('Ctrl Pts',(2.27126916799576,3.214285714,-7.14782039300889));
#101745=CARTESIAN_POINT('Ctrl Pts',(2.22833040210814,3.22133557900871,-7.16146448151981));
#101746=CARTESIAN_POINT('Ctrl Pts',(2.18523081450453,3.22840426981356,-7.17459171559583));
#101747=CARTESIAN_POINT('Ctrl Pts',(3.898934487,3.007773793,-6.406895494));
#101748=CARTESIAN_POINT('Ctrl Pts',(3.548498839,3.07352872,-6.620154104));
#101749=CARTESIAN_POINT('Ctrl Pts',(3.176894277,3.138525418,-6.79391954300001));
#101750=CARTESIAN_POINT('Ctrl Pts',(3.17319448267296,3.13917254249503,-6.79564959814783));
#101751=CARTESIAN_POINT('Ctrl Pts',(3.16949468834593,3.13981966699007,-6.79737965329567));
#101752=CARTESIAN_POINT('Ctrl Pts',(3.563829693,3.007773793,-6.313605778));
#101753=CARTESIAN_POINT('Ctrl Pts',(3.21849668,3.07352872,-6.508535283));
#101754=CARTESIAN_POINT('Ctrl Pts',(2.853963411,3.138525418,-6.664637488));
#101755=CARTESIAN_POINT('Ctrl Pts',(2.85033402035581,3.13917254249503,-6.66619168326981));
#101756=CARTESIAN_POINT('Ctrl Pts',(2.84670462971162,3.13981966699007,-6.6677458785396));
#101757=CARTESIAN_POINT('',(3.17689427783338,3.13852541850723,-6.7939195404758));
#101758=CARTESIAN_POINT('',(3.01542885200097,3.13852541943002,-6.72927851191472));
#101759=CARTESIAN_POINT('',(3.68234195126533,3.04797057322359,-6.53378587281428));
#101760=CARTESIAN_POINT('Origin',(-0.106532830040017,2.9464820989943,0.155905996139329));
#101761=CARTESIAN_POINT('Ctrl Pts',(3.55970394000874,3.00855922362529,-6.31593287126577));
#101762=CARTESIAN_POINT('Ctrl Pts',(3.58014882442165,3.01545478682465,-6.35216896468786));
#101763=CARTESIAN_POINT('Ctrl Pts',(3.60060118097571,3.0221815607465,-6.38846194717738));
#101764=CARTESIAN_POINT('Ctrl Pts',(3.64147274623553,3.03530792011833,-6.4610682912835));
#101765=CARTESIAN_POINT('Ctrl Pts',(3.66191525145192,3.04171498173437,-6.49742304369186));
#101766=CARTESIAN_POINT('Ctrl Pts',(3.68234195274149,3.0479705732829,-6.53378586556781));
#101767=CARTESIAN_POINT('Ctrl Pts',(4.16987946444665,3.13983235804358,-6.23395313325984));
#101768=CARTESIAN_POINT('Ctrl Pts',(4.16648996522332,3.13917888802179,-6.23621503562992));
#101769=CARTESIAN_POINT('Ctrl Pts',(4.163100466,3.138525418,-6.238476938));
#101770=CARTESIAN_POINT('Ctrl Pts',(3.82377331,3.073105688,-6.46491891300001));
#101771=CARTESIAN_POINT('Ctrl Pts',(3.461887187,3.007781414,-6.653220055));
#101772=CARTESIAN_POINT('Ctrl Pts',(4.22634547911204,3.13983235804358,-5.89071862761956));
#101773=CARTESIAN_POINT('Ctrl Pts',(4.22314243305602,3.13917888802179,-5.89301141180978));
#101774=CARTESIAN_POINT('Ctrl Pts',(4.219939387,3.138525418,-5.895304196));
#101775=CARTESIAN_POINT('Ctrl Pts',(3.899278299,3.073105688,-6.12483779));
#101776=CARTESIAN_POINT('Ctrl Pts',(3.555612789,3.007781414,-6.318236914));
#101777=CARTESIAN_POINT('',(4.16310045288277,3.13852541980557,-6.23847690789766));
#101778=CARTESIAN_POINT('Origin',(-0.10050314211654,3.08928601196563,0.164830506409255));
#101779=CARTESIAN_POINT('',(4.19151991788259,3.13852541968788,-6.06689057295364));
#101780=CARTESIAN_POINT('Origin',(-8.87744738831131E-13,3.22948687200044,
1.49229587020905E-12));
#101781=CARTESIAN_POINT('',(3.67646646406889,3.22840427021341,-6.53709372269269));
#101782=CARTESIAN_POINT('Origin',(-0.073818884042236,3.08929956416316,0.176545072854689));
#101783=CARTESIAN_POINT('Ctrl Pts',(4.16310045978442,3.13852541968788,-6.23847692794034));
#101784=CARTESIAN_POINT('Ctrl Pts',(3.96299266999802,3.176642188,-6.37201415700994));
#101785=CARTESIAN_POINT('Ctrl Pts',(3.75473825299771,3.214285714,-6.49245259100987));
#101786=CARTESIAN_POINT('Ctrl Pts',(3.71573644753807,3.22133557899732,-6.51500825378087));
#101787=CARTESIAN_POINT('Ctrl Pts',(3.67646647191127,3.22840426981354,-6.53709371808503));
#101788=CARTESIAN_POINT('Ctrl Pts',(5.18507271,3.007773793,-5.418950174));
#101789=CARTESIAN_POINT('Ctrl Pts',(4.888674351,3.07352872,-5.702556223));
#101790=CARTESIAN_POINT('Ctrl Pts',(4.563112129,3.138525418,-5.952143118));
#101791=CARTESIAN_POINT('Ctrl Pts',(4.55987074451438,3.13917254249503,-5.95462807182634));
#101792=CARTESIAN_POINT('Ctrl Pts',(4.55662936002876,3.13981966699007,-5.95711302565267));
#101793=CARTESIAN_POINT('Ctrl Pts',(4.837747949,3.007773793,-5.399879145));
#101794=CARTESIAN_POINT('Ctrl Pts',(4.542392711,3.07352872,-5.664487697));
#101795=CARTESIAN_POINT('Ctrl Pts',(4.219939387,3.138525418,-5.895304196));
#101796=CARTESIAN_POINT('Ctrl Pts',(4.21672895553369,3.13917254249503,-5.89760226674754));
#101797=CARTESIAN_POINT('Ctrl Pts',(4.21351852406738,3.13981966699007,-5.89990033749508));
#101798=CARTESIAN_POINT('',(4.5631121292891,3.13852541850725,-5.95214311534969));
#101799=CARTESIAN_POINT('',(4.39152576504318,3.13852541943002,-5.92372365177857));
#101800=CARTESIAN_POINT('',(5.00082166817462,3.04797057327088,-5.58943491989446));
#101801=CARTESIAN_POINT('Origin',(-0.137557002453182,2.94648211136749,0.12935920701272));
#101802=CARTESIAN_POINT('Ctrl Pts',(4.8342189097993,3.00855922380044,-5.40303874779572));
#101803=CARTESIAN_POINT('Ctrl Pts',(4.86197549338503,3.01545478703697,-5.43403261591302));
#101804=CARTESIAN_POINT('Ctrl Pts',(4.88975160317973,3.02218156082008,-5.46508043598458));
#101805=CARTESIAN_POINT('Ctrl Pts',(4.94527583198523,3.03530792020206,-5.52720310594268));
#101806=CARTESIAN_POINT('Ctrl Pts',(4.97305559995048,3.04171498179997,-5.5583133700908));
#101807=CARTESIAN_POINT('Ctrl Pts',(5.00082166815137,3.04797057333098,-5.58943491241765));
#101808=CARTESIAN_POINT('Ctrl Pts',(5.41250564892147,3.13983235804358,-5.19180595003168));
#101809=CARTESIAN_POINT('Ctrl Pts',(5.40968163646074,3.13917888802179,-5.19474361251584));
#101810=CARTESIAN_POINT('Ctrl Pts',(5.40685762400001,3.138525418,-5.197681275));
#101811=CARTESIAN_POINT('Ctrl Pts',(5.12414208000001,3.073105688,-5.49177447));
#101812=CARTESIAN_POINT('Ctrl Pts',(4.81119583200001,3.007781414,-5.753468055));
#101813=CARTESIAN_POINT('Ctrl Pts',(5.39386624760078,3.13983235804358,-4.84445755122613));
#101814=CARTESIAN_POINT('Ctrl Pts',(5.39123096780039,3.13917888802179,-4.84738529161306));
#101815=CARTESIAN_POINT('Ctrl Pts',(5.388595688,3.138525418,-4.850313032));
#101816=CARTESIAN_POINT('Ctrl Pts',(5.124774415,3.073105688,-5.143412913));
#101817=CARTESIAN_POINT('Ctrl Pts',(4.830718708,3.007781414,-5.406168399));
#101818=CARTESIAN_POINT('',(5.40685760454955,3.1385254197632,-5.19768124893519));
#101819=CARTESIAN_POINT('Origin',(-0.133587032587033,3.08928604981775,0.139371560321166));
#101820=CARTESIAN_POINT('',(5.39772664886391,3.13852541968788,-5.02399716116693));
#101821=CARTESIAN_POINT('Origin',(1.1067535776732E-12,3.22948687199922,
-1.24639881748934E-12));
#101822=CARTESIAN_POINT('',(4.9957946363652,3.22840427022511,-5.5939284900372));
#101823=CARTESIAN_POINT('Origin',(-0.110044981485926,3.08929957773932,0.15654863207421));
#101824=CARTESIAN_POINT('Ctrl Pts',(5.40685761576715,3.13852541968788,-5.19768126651046));
#101825=CARTESIAN_POINT('Ctrl Pts',(5.24013479200018,3.176642188,-5.37111372800878));
#101826=CARTESIAN_POINT('Ctrl Pts',(5.0626399509999,3.214285714,-5.53350492300877));
#101827=CARTESIAN_POINT('Ctrl Pts',(5.02939878672657,3.22133557899626,-5.56391748211061));
#101828=CARTESIAN_POINT('Ctrl Pts',(4.99579464301703,3.22840426981362,-5.59392848408735));
#101829=CARTESIAN_POINT('Ctrl Pts',(6.228762696,3.007773793,-4.177620768));
#101830=CARTESIAN_POINT('Ctrl Pts',(6.000260882,3.07352872,-4.51831315));
#101831=CARTESIAN_POINT('Ctrl Pts',(5.73596393,3.138525418,-4.832051096));
#101832=CARTESIAN_POINT('Ctrl Pts',(5.73333251891506,3.13917254249503,-4.83517475483384));
#101833=CARTESIAN_POINT('Ctrl Pts',(5.73070110783012,3.13981966699007,-4.83829841366768));
#101834=CARTESIAN_POINT('Ctrl Pts',(5.885458487,3.007773793,-4.233660165));
#101835=CARTESIAN_POINT('Ctrl Pts',(5.653891507,3.07352872,-4.555574961));
#101836=CARTESIAN_POINT('Ctrl Pts',(5.388595688,3.138525418,-4.850313032));
#101837=CARTESIAN_POINT('Ctrl Pts',(5.38595433192827,3.13917254249503,-4.8532475230008));
#101838=CARTESIAN_POINT('Ctrl Pts',(5.38331297585654,3.13981966699007,-4.85618201400161));
#101839=CARTESIAN_POINT('',(5.73596392970722,3.13852541850725,-4.83205109335266));
#101840=CARTESIAN_POINT('',(5.56227981475606,3.13852541943002,-4.84118205738657));
#101841=CARTESIAN_POINT('',(6.08546852191175,3.04797057323436,-4.3837282020756));
#101842=CARTESIAN_POINT('Origin',(-0.162149709194065,2.94648212629685,0.0967644123793421));
#101843=CARTESIAN_POINT('Ctrl Pts',(5.88269117573789,3.00855922365084,-4.23750453653349));
#101844=CARTESIAN_POINT('Ctrl Pts',(5.91646159104702,3.01545478684441,-4.26180694017313));
#101845=CARTESIAN_POINT('Ctrl Pts',(5.95026267506045,3.02218156076831,-4.28615783749173));
#101846=CARTESIAN_POINT('Ctrl Pts',(6.01784331581345,3.03530792012776,-4.33489204606716));
#101847=CARTESIAN_POINT('Ctrl Pts',(6.05166139551355,3.04171498174435,-4.35930314069436));
#101848=CARTESIAN_POINT('Ctrl Pts',(6.08546852022469,3.0479705732939,-4.38372819485558));
#101849=CARTESIAN_POINT('Ctrl Pts',(6.40204908504071,3.13983235804358,-3.90689568945038));
#101850=CARTESIAN_POINT('Ctrl Pts',(6.39992260702036,3.13917888802179,-3.91037175022519));
#101851=CARTESIAN_POINT('Ctrl Pts',(6.397796129,3.138525418,-3.913847811));
#101852=CARTESIAN_POINT('Ctrl Pts',(6.18491166100001,3.073105688,-4.261840756));
#101853=CARTESIAN_POINT('Ctrl Pts',(5.93553830800001,3.007781414,-4.584690283));
#101854=CARTESIAN_POINT('Ctrl Pts',(6.30917582457058,3.13983235804358,-3.57167502459223));
#101855=CARTESIAN_POINT('Ctrl Pts',(6.30723153378529,3.13917888802179,-3.57510082329612));
#101856=CARTESIAN_POINT('Ctrl Pts',(6.305287243,3.138525418,-3.578526622));
#101857=CARTESIAN_POINT('Ctrl Pts',(6.110641775,3.073105688,-3.921487766));
#101858=CARTESIAN_POINT('Ctrl Pts',(5.87994559000001,3.007781414,-4.241313459));
#101859=CARTESIAN_POINT('',(6.397796104402,3.13852541976232,-3.91384778973847));
#101860=CARTESIAN_POINT('Origin',(-0.160424606371967,3.08928602904207,0.10739586321264));
#101861=CARTESIAN_POINT('',(6.35154168067892,3.13852541968788,-3.74618722552173));
#101862=CARTESIAN_POINT('Origin',(4.10695782937509E-13,3.22948687199889,
-4.39752401160121E-13));
#101863=CARTESIAN_POINT('',(6.08152500365499,3.22840427021624,-4.38919737818779));
#101864=CARTESIAN_POINT('Origin',(-0.141125708614549,3.08929954404176,0.129232339770062));
#101865=CARTESIAN_POINT('Ctrl Pts',(6.39779611913472,3.13852541968788,-3.91384780447908));
#101866=CARTESIAN_POINT('Ctrl Pts',(6.27225403500211,3.176642188,-4.11906599100872));
#101867=CARTESIAN_POINT('Ctrl Pts',(6.13381823100183,3.214285714,-4.31581671400877));
#101868=CARTESIAN_POINT('Ctrl Pts',(6.10789202802801,3.22133557898932,-4.35266411204301));
#101869=CARTESIAN_POINT('Ctrl Pts',(6.08152500887293,3.2284042698136,-4.38919737096436));
#101870=CARTESIAN_POINT('Ctrl Pts',(6.981202661,3.007773793,-2.740950457));
#101871=CARTESIAN_POINT('Ctrl Pts',(6.831281884,3.07352872,-3.122798776));
#101872=CARTESIAN_POINT('Ctrl Pts',(6.640608432,3.138525418,-3.486017736));
#101873=CARTESIAN_POINT('Ctrl Pts',(6.63871003615623,3.13917254249503,-3.48963404103255));
#101874=CARTESIAN_POINT('Ctrl Pts',(6.63681164031246,3.13981966699007,-3.4932503460651));
#101875=CARTESIAN_POINT('Ctrl Pts',(6.657971528,3.007773793,-2.869479942));
#101876=CARTESIAN_POINT('Ctrl Pts',(6.50102062000001,3.07352872,-3.233648604));
#101877=CARTESIAN_POINT('Ctrl Pts',(6.30528724300001,3.138525418,-3.578526622));
#101878=CARTESIAN_POINT('Ctrl Pts',(6.30333846919071,3.13917254249503,-3.58196031971256));
#101879=CARTESIAN_POINT('Ctrl Pts',(6.30138969538143,3.13981966699007,-3.58539401742512));
#101880=CARTESIAN_POINT('',(6.64060843113851,3.13852541850724,-3.48601773348335));
#101881=CARTESIAN_POINT('',(6.4729478416998,3.13852541943002,-3.5322721713038));
#101882=CARTESIAN_POINT('',(6.88556563105117,3.04797057325362,-2.97304322568093));
#101883=CARTESIAN_POINT('Origin',(-0.179160225268817,2.94648210547569,0.0596447132767219));
#101884=CARTESIAN_POINT('Ctrl Pts',(6.65609534086921,3.00855922359392,-2.87382932423474));
#101885=CARTESIAN_POINT('Ctrl Pts',(6.6943005212506,3.01545478683807,-2.89030390998496));
#101886=CARTESIAN_POINT('Ctrl Pts',(6.73254607753589,3.02218156072765,-2.90681926266647));
#101887=CARTESIAN_POINT('Ctrl Pts',(6.8090231348598,3.03530792013855,-2.93988625227469));
#101888=CARTESIAN_POINT('Ctrl Pts',(6.84729823036446,3.04171498176221,-2.95645674151876));
#101889=CARTESIAN_POINT('Ctrl Pts',(6.88556562787249,3.04797057331347,-2.97304321894631));
#101890=CARTESIAN_POINT('Ctrl Pts',(7.09223982166471,3.13983235804358,-2.43930332935916));
#101891=CARTESIAN_POINT('Ctrl Pts',(7.09091030983235,3.13917888802179,-2.44315525167958));
#101892=CARTESIAN_POINT('Ctrl Pts',(7.089580798,3.138525418,-2.447007174));
#101893=CARTESIAN_POINT('Ctrl Pts',(6.956481647,3.073105688,-2.832628105));
#101894=CARTESIAN_POINT('Ctrl Pts',(6.782341609,3.007781414,-3.201537489));
#101895=CARTESIAN_POINT('Ctrl Pts',(6.92947535176304,3.13983235804358,-2.1318849430597));
#101896=CARTESIAN_POINT('Ctrl Pts',(6.92831296288152,3.13917888802179,-2.13564861352985));
#101897=CARTESIAN_POINT('Ctrl Pts',(6.927150574,3.138525418,-2.139412284));
#101898=CARTESIAN_POINT('Ctrl Pts',(6.81078231800001,3.073105688,-2.516198208));
#101899=CARTESIAN_POINT('Ctrl Pts',(6.654232751,3.007781414,-2.878139415));
#101900=CARTESIAN_POINT('',(7.0895807693367,3.13852541980578,-2.44700715796875));
#101901=CARTESIAN_POINT('Origin',(-0.179760882835231,3.08928603680601,0.0703984541554009));
#101902=CARTESIAN_POINT('',(7.00836568274272,3.13852541968788,-2.29320973895468));
#101903=CARTESIAN_POINT('Origin',(3.20923843055709E-13,3.22948687200022,
5.42101086242752E-15));
#101904=CARTESIAN_POINT('',(6.88289002147178,3.2284042702058,-2.97923227547513));
#101905=CARTESIAN_POINT('Origin',(-0.165607402433887,3.08929956023117,0.0958731051008638));
#101906=CARTESIAN_POINT('Ctrl Pts',(7.08958078696342,3.13852541968788,-2.44700716975202));
#101907=CARTESIAN_POINT('Ctrl Pts',(7.01108965100386,3.176642188,-2.67441530600791));
#101908=CARTESIAN_POINT('Ctrl Pts',(6.9181859880036,3.214285714,-2.89632571200803));
#101909=CARTESIAN_POINT('Ctrl Pts',(6.90078702682232,3.22133557898884,-2.93788500570877));
#101910=CARTESIAN_POINT('Ctrl Pts',(6.88289002496,3.22840426981237,-2.97923226718436));
#101911=CARTESIAN_POINT('Ctrl Pts',(7.407209349,3.007773793,-1.176116349));
#101912=CARTESIAN_POINT('Ctrl Pts',(7.342879738,3.07352872,-1.581265802));
#101913=CARTESIAN_POINT('Ctrl Pts',(7.234745464,3.138525418,-1.97698206));
#101914=CARTESIAN_POINT('Ctrl Pts',(7.23366885027021,3.13917254249503,-1.98092191681603));
#101915=CARTESIAN_POINT('Ctrl Pts',(7.23259223654041,3.13981966699007,-1.98486177363207));
#101916=CARTESIAN_POINT('Ctrl Pts',(7.11916522,3.007773793,-1.371126025));
#101917=CARTESIAN_POINT('Ctrl Pts',(7.044169235,3.07352872,-1.760520432));
#101918=CARTESIAN_POINT('Ctrl Pts',(6.927150574,3.138525418,-2.139412284));
#101919=CARTESIAN_POINT('Ctrl Pts',(6.92598550493897,3.13917254249503,-2.14318463253374));
#101920=CARTESIAN_POINT('Ctrl Pts',(6.92482043587793,3.13981966699007,-2.14695698106747));
#101921=CARTESIAN_POINT('',(7.23474546263686,3.13852541850726,-1.97698205770052));
#101922=CARTESIAN_POINT('',(7.08094802144716,3.13852541943002,-2.05819716358091));
#101923=CARTESIAN_POINT('',(7.36370134438744,3.04797057330458,-1.42334205253659));
#101924=CARTESIAN_POINT('Origin',(-0.187793154152902,2.94648211929427,0.019736057114943));
#101925=CARTESIAN_POINT('Ctrl Pts',(7.11826788532725,3.00855922357092,-1.37577704600417));
#101926=CARTESIAN_POINT('Ctrl Pts',(7.15912139880288,3.01545478681724,-1.38365348071187));
#101927=CARTESIAN_POINT('Ctrl Pts',(7.20002310803504,3.02218156072704,-1.39156104960523));
#101928=CARTESIAN_POINT('Ctrl Pts',(7.28182059976212,3.03530792015462,-1.40741464472073));
#101929=CARTESIAN_POINT('Ctrl Pts',(7.32276301033261,3.04171498179586,-1.41536971100774));
#101930=CARTESIAN_POINT('Ctrl Pts',(7.36370133986324,3.04797057336533,-1.42334204651203));
#101931=CARTESIAN_POINT('Ctrl Pts',(7.45080530628486,3.13983235804358,-0.8576518564782));
#101932=CARTESIAN_POINT('Ctrl Pts',(7.45033492714243,3.13917888802179,-0.8616995287391));
#101933=CARTESIAN_POINT('Ctrl Pts',(7.449864548,3.138525418,-0.865747201));
#101934=CARTESIAN_POINT('Ctrl Pts',(7.402774283,3.073105688,-1.270964912));
#101935=CARTESIAN_POINT('Ctrl Pts',(7.312010155,3.007781414,-1.668684361));
#101936=CARTESIAN_POINT('Ctrl Pts',(7.2257603139574,3.13983235804358,-0.592410290582772));
#101937=CARTESIAN_POINT('Ctrl Pts',(7.2254341789787,3.13917888802179,-0.596335847791386));
#101938=CARTESIAN_POINT('Ctrl Pts',(7.225108044,3.138525418,-0.600261405));
#101939=CARTESIAN_POINT('Ctrl Pts',(7.192458249,3.073105688,-0.99325402));
#101940=CARTESIAN_POINT('Ctrl Pts',(7.11737538400001,3.007781414,-1.380386771));
#101941=CARTESIAN_POINT('',(7.44986451655801,3.13852541980588,-0.865747191503968));
#101942=CARTESIAN_POINT('Origin',(-0.190691700192834,3.0892860583674,0.0301092810209785));
#101943=CARTESIAN_POINT('',(7.33748629495884,3.13852541968788,-0.733004313422165));
#101944=CARTESIAN_POINT('Origin',(-5.10008701937181E-13,3.22948687200011,
7.92551788086904E-14));
#101945=CARTESIAN_POINT('',(7.36241875121879,3.22840427023676,-1.42996158253138));
#101946=CARTESIAN_POINT('Origin',(-0.182345328124276,3.08929952089793,0.0580309238824359));
#101947=CARTESIAN_POINT('Ctrl Pts',(7.4498645363088,3.13852541968788,-0.865747199224515));
#101948=CARTESIAN_POINT('Ctrl Pts',(7.42209450600614,3.176642188,-1.10471193400775));
#101949=CARTESIAN_POINT('Ctrl Pts',(7.37906705800589,3.214285714,-1.34140573900794));
#101950=CARTESIAN_POINT('Ctrl Pts',(7.3710088942515,3.22133557900333,-1.38573366195178));
#101951=CARTESIAN_POINT('Ctrl Pts',(7.36241875294202,3.22840426981265,-1.42996157381253));
#101952=CARTESIAN_POINT('Ctrl Pts',(7.48686316,3.007773793,0.443711652));
#101953=CARTESIAN_POINT('Ctrl Pts',(7.511132695,3.07352872,0.034205403));
#101954=CARTESIAN_POINT('Ctrl Pts',(7.49059384,3.138525418,-0.375504901));
#101955=CARTESIAN_POINT('Ctrl Pts',(7.49038934967081,3.13917254249503,-0.379584086277783));
#101956=CARTESIAN_POINT('Ctrl Pts',(7.49018485934161,3.13981966699007,-0.383663271555565));
#101957=CARTESIAN_POINT('Ctrl Pts',(7.247474658,3.007773793,0.191340221));
#101958=CARTESIAN_POINT('Ctrl Pts',(7.257940325,3.07352872,-0.205072282));
#101959=CARTESIAN_POINT('Ctrl Pts',(7.225108044,3.138525418,-0.600261405));
#101960=CARTESIAN_POINT('Ctrl Pts',(7.22478115703625,3.13917254249503,-0.6041960135191));
#101961=CARTESIAN_POINT('Ctrl Pts',(7.2244542700725,3.13981966699007,-0.6081306220382));
#101962=CARTESIAN_POINT('',(7.35785094258044,3.1385254194309,-0.487883144246335));
#101963=CARTESIAN_POINT('Ctrl Pts',(7.24759813528023,3.00855922363686,0.186605038200589));
#101964=CARTESIAN_POINT('Ctrl Pts',(7.28918971675842,3.01545478684859,0.187695047633154));
#101965=CARTESIAN_POINT('Ctrl Pts',(7.33083506030774,3.02218156075999,0.188765011538209));
#101966=CARTESIAN_POINT('Ctrl Pts',(7.41412822615322,3.03530792015269,0.19086610716728));
#101967=CARTESIAN_POINT('Ctrl Pts',(7.45582352988066,3.04171498178109,0.191898433839794));
#101968=CARTESIAN_POINT('Ctrl Pts',(7.49751856038283,3.0479705733412,0.192913017772022));
#101969=CARTESIAN_POINT('Ctrl Pts',(7.46097941612226,3.13983235804358,0.764102464106214));
#101970=CARTESIAN_POINT('Ctrl Pts',(7.46139016406113,3.13917888802179,0.760048306553106));
#101971=CARTESIAN_POINT('Ctrl Pts',(7.461800912,3.138525418,0.755994149));
#101972=CARTESIAN_POINT('Ctrl Pts',(7.50292141999999,3.073105688,0.350127187));
#101973=CARTESIAN_POINT('Ctrl Pts',(7.499777232,3.007781414,-0.057805406));
#101974=CARTESIAN_POINT('Ctrl Pts',(7.18417675373603,3.13983235804358,0.974764808487867));
#101975=CARTESIAN_POINT('Ctrl Pts',(7.18470212236801,3.13917888802179,0.970860919243934));
#101976=CARTESIAN_POINT('Ctrl Pts',(7.185227491,3.138525418,0.96695703));
#101977=CARTESIAN_POINT('Ctrl Pts',(7.237822825,3.073105688,0.576133623));
#101978=CARTESIAN_POINT('Ctrl Pts',(7.247717455,3.007781414,0.181911224));
#101979=CARTESIAN_POINT('',(7.32351420272364,3.13852541968788,0.86147557909768));
#101980=CARTESIAN_POINT('Ctrl Pts',(7.21643957,3.007773793,2.042792189));
#101981=CARTESIAN_POINT('Ctrl Pts',(7.328173436,3.07352872,1.648077202));
#101982=CARTESIAN_POINT('Ctrl Pts',(7.396190372,3.138525418,1.24353045));
#101983=CARTESIAN_POINT('Ctrl Pts',(7.39686756679169,3.13917254249503,1.23950267442584));
#101984=CARTESIAN_POINT('Ctrl Pts',(7.39754476158338,3.13981966699007,1.23547489885168));
#101985=CARTESIAN_POINT('Ctrl Pts',(7.036900237,3.007773793,1.74485961));
#101986=CARTESIAN_POINT('Ctrl Pts',(7.132338192,3.07352872,1.359964821));
#101987=CARTESIAN_POINT('Ctrl Pts',(7.18522749100001,3.138525418,0.96695703));
#101988=CARTESIAN_POINT('Ctrl Pts',(7.185754070995,3.13917254249503,0.963044139405232));
#101989=CARTESIAN_POINT('Ctrl Pts',(7.18628065099001,3.13981966699007,0.959131248810464));
#101990=CARTESIAN_POINT('',(7.39619036979386,3.13852541850725,1.243530451497));
#101991=CARTESIAN_POINT('',(7.29070893018589,3.13852541943002,1.1052437486685));
#101992=CARTESIAN_POINT('',(7.28076015326005,3.04797057328962,1.80014768114074));
#101993=CARTESIAN_POINT('Origin',(-0.178723583592237,2.94648210035276,-0.0609403866795913));
#101994=CARTESIAN_POINT('Ctrl Pts',(7.03803875139297,3.00855922357189,1.74026167702851));
#101995=CARTESIAN_POINT('Ctrl Pts',(7.07842362489373,3.01545478679328,1.75026716357868));
#101996=CARTESIAN_POINT('Ctrl Pts',(7.11886531302015,3.02218156075358,1.76026463048229));
#101997=CARTESIAN_POINT('Ctrl Pts',(7.19975945737551,3.03530792015482,1.78022217259254));
#101998=CARTESIAN_POINT('Ctrl Pts',(7.24025802834496,3.04171498178902,1.79019362198331));
#101999=CARTESIAN_POINT('Ctrl Pts',(7.28076014663648,3.04797057335003,1.80014768467118));
#102000=CARTESIAN_POINT('Ctrl Pts',(7.12228642016887,3.13983235804358,2.35012820286911));
#102001=CARTESIAN_POINT('Ctrl Pts',(7.12355908908444,3.13917888802179,2.34625712793456));
#102002=CARTESIAN_POINT('Ctrl Pts',(7.124831758,3.138525418,2.342386053));
#102003=CARTESIAN_POINT('Ctrl Pts',(7.252240291,3.073105688,1.954847729));
#102004=CARTESIAN_POINT('Ctrl Pts',(7.336863062,3.007781414,1.555776466));
#102005=CARTESIAN_POINT('Ctrl Pts',(6.80666907381407,3.13983235804358,2.496360987497));
#102006=CARTESIAN_POINT('Ctrl Pts',(6.80802138040703,3.13917888802179,2.4926613077485));
#102007=CARTESIAN_POINT('Ctrl Pts',(6.809373687,3.138525418,2.488961628));
#102008=CARTESIAN_POINT('Ctrl Pts',(6.944754851,3.073105688,2.118581898));
#102009=CARTESIAN_POINT('Ctrl Pts',(7.039164313,3.007781414,1.735703252));
#102010=CARTESIAN_POINT('',(7.12483172548045,3.13852541980596,2.34238604841789));
#102011=CARTESIAN_POINT('Origin',(-0.185709916198784,3.08928601941837,-0.0527429847199418));
#102012=CARTESIAN_POINT('',(6.96710272593122,3.13852541968788,2.41567383060393));
#102013=CARTESIAN_POINT('Origin',(1.19609183668601E-12,3.22948687199989,
2.5652223401007E-13));
#102014=CARTESIAN_POINT('',(7.28237557194861,3.22840427022627,1.79360141154214));
#102015=CARTESIAN_POINT('Origin',(-0.189858677544151,3.08929957468348,-0.0238973877759271));
#102016=CARTESIAN_POINT('Ctrl Pts',(7.12483174664295,3.13852541968788,2.3423860497028));
#102017=CARTESIAN_POINT('Ctrl Pts',(7.19996703800783,3.176642188,2.11384719699605));
#102018=CARTESIAN_POINT('Ctrl Pts',(7.2603015320077,3.214285714,1.8809629609958));
#102019=CARTESIAN_POINT('Ctrl Pts',(7.27160095263314,3.22133557899429,1.83734849258618));
#102020=CARTESIAN_POINT('Ctrl Pts',(7.28237556986395,3.22840426981362,1.79360142017328));
#102021=CARTESIAN_POINT('Ctrl Pts',(6.60858328699999,3.007773793,3.546354034));
#102022=CARTESIAN_POINT('Ctrl Pts',(6.802556932,3.07352872,3.184886742));
#102023=CARTESIAN_POINT('Ctrl Pts',(6.955949263,3.138525418,2.804419699));
#102024=CARTESIAN_POINT('Ctrl Pts',(6.95747647804007,3.13917254249503,2.80063166744372));
#102025=CARTESIAN_POINT('Ctrl Pts',(6.95900369308013,3.13981966699007,2.79684363588743));
#102026=CARTESIAN_POINT('Ctrl Pts',(6.497288181,3.007773793,3.216791304));
#102027=CARTESIAN_POINT('Ctrl Pts',(6.67323585300001,3.07352872,2.86141148));
#102028=CARTESIAN_POINT('Ctrl Pts',(6.809373687,3.138525418,2.488961628));
#102029=CARTESIAN_POINT('Ctrl Pts',(6.81072911165684,3.13917254249503,2.48525341773983));
#102030=CARTESIAN_POINT('Ctrl Pts',(6.81208453631367,3.13981966699007,2.48154520747966));
#102031=CARTESIAN_POINT('',(6.9559492605235,3.13852541850726,2.80441969999317));
#102032=CARTESIAN_POINT('',(6.88266147185314,3.13852541943002,2.64669067168334));
#102033=CARTESIAN_POINT('',(6.7235614876778,3.04797057331005,3.3232094438561));
#102034=CARTESIAN_POINT('Origin',(-0.161444725667562,2.94648211734716,-0.0979359062490287));
#102035=CARTESIAN_POINT('Ctrl Pts',(6.49938849766569,3.00855922363798,3.21254561543738));
#102036=CARTESIAN_POINT('Ctrl Pts',(6.53667831154149,3.01545478684796,3.23099873311303));
#102037=CARTESIAN_POINT('Ctrl Pts',(6.57402533564303,3.02218156079055,3.24945623212677));
#102038=CARTESIAN_POINT('Ctrl Pts',(6.64873793835688,3.0353079201812,3.28633702758897));
#102039=CARTESIAN_POINT('Ctrl Pts',(6.68614610838593,3.04171498180963,3.3047813455693));
#102040=CARTESIAN_POINT('Ctrl Pts',(6.72356148043066,3.04797057337082,3.32320944593047));
#102041=CARTESIAN_POINT('Ctrl Pts',(6.45056322737556,3.13983235804358,3.82626455831516));
#102042=CARTESIAN_POINT('Ctrl Pts',(6.45263830868778,3.13917888802179,3.82275757315758));
#102043=CARTESIAN_POINT('Ctrl Pts',(6.45471339,3.138525418,3.819250588));
#102044=CARTESIAN_POINT('Ctrl Pts',(6.662452467,3.073105688,3.468161763));
#102045=CARTESIAN_POINT('Ctrl Pts',(6.830885329,3.007781414,3.096611959));
#102046=CARTESIAN_POINT('Ctrl Pts',(6.11088911360346,3.13983235804358,3.90123010271037));
#102047=CARTESIAN_POINT('Ctrl Pts',(6.11300512580173,3.13917888802179,3.89790762535519));
#102048=CARTESIAN_POINT('Ctrl Pts',(6.115121138,3.138525418,3.894585148));
#102049=CARTESIAN_POINT('Ctrl Pts',(6.326957859,3.073105688,3.561967638));
#102050=CARTESIAN_POINT('Ctrl Pts',(6.50146767100001,3.007781414,3.208335726));
#102051=CARTESIAN_POINT('',(6.45471335922989,3.13852541980593,3.81925057653514));
#102052=CARTESIAN_POINT('Origin',(-0.170029793294556,3.0892859931606,-0.0914319448838835));
#102053=CARTESIAN_POINT('',(6.28491726947836,3.13852541968788,3.85691785907291));
#102054=CARTESIAN_POINT('Origin',(-3.28730098697605E-13,3.22948687200044,
-1.06902334207071E-13));
#102055=CARTESIAN_POINT('',(6.72654639328731,3.2284042702405,3.31716348977603));
#102056=CARTESIAN_POINT('Origin',(-0.180282775615583,3.08929951594535,-0.0641527183463853));
#102057=CARTESIAN_POINT('Ctrl Pts',(6.45471337961771,3.13852541968788,3.81925058233835));
#102058=CARTESIAN_POINT('Ctrl Pts',(6.57722114700879,3.176642188,3.61220670799775));
#102059=CARTESIAN_POINT('Ctrl Pts',(6.68620828100871,3.214285714,3.39773730899748));
#102060=CARTESIAN_POINT('Ctrl Pts',(6.70661934883691,3.22133557901279,3.35757156380995));
#102061=CARTESIAN_POINT('Ctrl Pts',(6.72654638920165,3.2284042698136,3.31716349782817));
#102062=CARTESIAN_POINT('Ctrl Pts',(5.69171699500001,3.007773793,4.884092306));
#102063=CARTESIAN_POINT('Ctrl Pts',(5.958860426,3.07352872,4.572774518));
#102064=CARTESIAN_POINT('Ctrl Pts',(6.190455698,3.138525418,4.2341774));
#102065=CARTESIAN_POINT('Ctrl Pts',(6.19276152241965,3.13917254249503,4.23080623660635));
#102066=CARTESIAN_POINT('Ctrl Pts',(6.1950673468393,3.13981966699007,4.2274350732127));
#102067=CARTESIAN_POINT('Ctrl Pts',(5.653870151,3.007773793,4.538309411));
#102068=CARTESIAN_POINT('Ctrl Pts',(5.902100421,3.07352872,4.229061719));
#102069=CARTESIAN_POINT('Ctrl Pts',(6.115121138,3.138525418,3.894585148));
#102070=CARTESIAN_POINT('Ctrl Pts',(6.11724202918621,3.13917254249503,3.89125500987346));
#102071=CARTESIAN_POINT('Ctrl Pts',(6.1193629203724,3.13981966699007,3.88792487174692));
#102072=CARTESIAN_POINT('',(6.19045569537371,3.13852541850724,4.23417740041519));
#102073=CARTESIAN_POINT('',(6.15278841316754,3.13852541943002,4.06438128131554));
#102074=CARTESIAN_POINT('',(5.8519765592091,3.04797057325383,4.69088162618691));
#102075=CARTESIAN_POINT('Origin',(-0.136617110471591,2.94648208787109,-0.130352228523811));
#102076=CARTESIAN_POINT('Ctrl Pts',(5.65683406098952,3.0085592236328,4.53461449072007));
#102077=CARTESIAN_POINT('Ctrl Pts',(5.68928518494542,3.01545478683192,4.56065239240518));
#102078=CARTESIAN_POINT('Ctrl Pts',(5.72179123963888,3.02218156074882,4.58670687140468));
#102079=CARTESIAN_POINT('Ctrl Pts',(5.78682882246822,3.03530792013085,4.63878641527706));
#102080=CARTESIAN_POINT('Ctrl Pts',(5.8193974271448,3.04171498175484,4.66484116602169));
#102081=CARTESIAN_POINT('Ctrl Pts',(5.85197655176899,3.04797057331367,4.69088162653268));
#102082=CARTESIAN_POINT('Ctrl Pts',(5.47721886760685,3.13983235804358,5.12348903528974));
#102083=CARTESIAN_POINT('Ctrl Pts',(5.47999933280343,3.13917888802179,5.12051012264487));
#102084=CARTESIAN_POINT('Ctrl Pts',(5.482779798,3.138525418,5.11753121));
#102085=CARTESIAN_POINT('Ctrl Pts',(5.761135769,3.073105688,4.819308408));
#102086=CARTESIAN_POINT('Ctrl Pts',(6.00550299000001,3.007781414,4.492653318));
#102087=CARTESIAN_POINT('Ctrl Pts',(5.12937076913739,3.13983235804358,5.12368203318865));
#102088=CARTESIAN_POINT('Ctrl Pts',(5.1321515445687,3.13917888802179,5.12089211359433));
#102089=CARTESIAN_POINT('Ctrl Pts',(5.13493232,3.138525418,5.118102194));
#102090=CARTESIAN_POINT('Ctrl Pts',(5.413319349,3.073105688,4.838799731));
#102091=CARTESIAN_POINT('Ctrl Pts',(5.659769626,3.007781414,4.530949987));
#102092=CARTESIAN_POINT('',(5.48277977040895,3.1385254198058,5.11753119218416));
#102093=CARTESIAN_POINT('Origin',(-0.146399510967205,3.08928604665587,-0.125845777516614));
#102094=CARTESIAN_POINT('',(5.30885606626935,3.13852541968788,5.1178166944593));
#102095=CARTESIAN_POINT('Origin',(-8.60856524953491E-13,3.22948687200056,
-7.23813370351323E-13));
#102096=CARTESIAN_POINT('',(5.8561913810091,3.2284042702163,4.68561868987122));
#102097=CARTESIAN_POINT('Origin',(-0.162276638324688,3.08929955310546,-0.101408132844909));
#102098=CARTESIAN_POINT('Ctrl Pts',(5.4827797890775,3.13852541968788,5.11753120223883));
#102099=CARTESIAN_POINT('Ctrl Pts',(5.64693170600921,3.176642188,4.94166344799969));
#102100=CARTESIAN_POINT('Ctrl Pts',(5.7994753620092,3.214285714,4.75563723599939));
#102101=CARTESIAN_POINT('Ctrl Pts',(5.82804367834116,3.22133557899689,4.72079831996769));
#102102=CARTESIAN_POINT('Ctrl Pts',(5.85619137527324,3.2284042698127,4.68561869685597));
#102103=CARTESIAN_POINT('Ctrl Pts',(4.508712341,3.007773793,5.99345585));
#102104=CARTESIAN_POINT('Ctrl Pts',(4.83653423,3.07352872,5.74684444));
#102105=CARTESIAN_POINT('Ctrl Pts',(5.135503304,3.138525418,5.465949672));
#102106=CARTESIAN_POINT('Ctrl Pts',(5.13847991999737,3.13917254249504,5.46315300862336));
#102107=CARTESIAN_POINT('Ctrl Pts',(5.14145653599473,3.13981966699007,5.4603563452467));
#102108=CARTESIAN_POINT('Ctrl Pts',(4.546083437,3.007773793,5.647621215));
#102109=CARTESIAN_POINT('Ctrl Pts',(4.854989334,3.07352872,5.398965732));
#102110=CARTESIAN_POINT('Ctrl Pts',(5.13493232,3.138525418,5.118102194));
#102111=CARTESIAN_POINT('Ctrl Pts',(5.1377195071807,3.13917254249504,5.11530584155758));
#102112=CARTESIAN_POINT('Ctrl Pts',(5.14050669436141,3.13981966699007,5.11250948911516));
#102113=CARTESIAN_POINT('',(5.13550330134345,3.13852541850725,5.4659496718453));
#102114=CARTESIAN_POINT('',(5.13521780570783,3.13852541943004,5.29202593910573));
#102115=CARTESIAN_POINT('',(4.70675971130458,3.04797057329693,5.83921339746965));
#102116=CARTESIAN_POINT('Origin',(-0.105401058942916,2.94648212894648,-0.156673128795994));
#102117=CARTESIAN_POINT('Ctrl Pts',(4.54977235062775,3.00855922349068,5.6446498313131));
#102118=CARTESIAN_POINT('Ctrl Pts',(4.57586740607629,3.01545478669787,5.67705501364761));
#102119=CARTESIAN_POINT('Ctrl Pts',(4.60201254479472,3.02218156072021,5.70948819475089));
#102120=CARTESIAN_POINT('Ctrl Pts',(4.65433402260645,3.03530792012531,5.774331305732));
#102121=CARTESIAN_POINT('Ctrl Pts',(4.68054019026196,3.0417149817775,5.80677819834263));
#102122=CARTESIAN_POINT('Ctrl Pts',(4.70675970388043,3.04797057335741,5.83921339628418));
#102123=CARTESIAN_POINT('Ctrl Pts',(4.24776584072616,3.13983235804358,6.18114485999083));
#102124=CARTESIAN_POINT('Ctrl Pts',(4.25112167836308,3.13917888802179,6.17883331049541));
#102125=CARTESIAN_POINT('Ctrl Pts',(4.254477516,3.138525418,6.176521761));
#102126=CARTESIAN_POINT('Ctrl Pts',(4.590434767,3.073105688,5.945109548));
#102127=CARTESIAN_POINT('Ctrl Pts',(4.899310006,3.007781414,5.678623201));
#102128=CARTESIAN_POINT('Ctrl Pts',(3.90800874862701,3.13983235804358,6.10655628662292));
#102129=CARTESIAN_POINT('Ctrl Pts',(3.9113242613135,3.13917888802179,6.10442937831146));
#102130=CARTESIAN_POINT('Ctrl Pts',(3.914639774,3.138525418,6.10230247));
#102131=CARTESIAN_POINT('Ctrl Pts',(4.246560042,3.073105688,5.889374925));
#102132=CARTESIAN_POINT('Ctrl Pts',(4.55342704399999,3.007781414,5.641702062));
#102133=CARTESIAN_POINT('',(4.25447749288633,3.13852541980575,6.17652173767152));
#102134=CARTESIAN_POINT('Origin',(-0.115923519980704,3.08928602198266,-0.154374961645372));
#102135=CARTESIAN_POINT('',(4.08455865372042,3.13852541968788,6.13941210969829));
#102136=CARTESIAN_POINT('Origin',(-8.94683632735038E-13,3.22948687200078,
-9.59302082215174E-13));
#102137=CARTESIAN_POINT('',(4.71200736843668,3.22840427022025,5.8349795680853));
#102138=CARTESIAN_POINT('Origin',(-0.136683026005425,3.08929956840681,-0.133922036616551));
#102139=CARTESIAN_POINT('Ctrl Pts',(4.25447750895388,3.13852541968788,6.17652175150207));
#102140=CARTESIAN_POINT('Ctrl Pts',(4.45259801400849,3.176642188,6.04005349700157));
#102141=CARTESIAN_POINT('Ctrl Pts',(4.64156542100854,3.214285714,5.8911688520013));
#102142=CARTESIAN_POINT('Ctrl Pts',(4.6769551631131,3.2213355789938,5.86328579409405));
#102143=CARTESIAN_POINT('Ctrl Pts',(4.7120073614679,3.22840426981363,5.83497957368301));
#102144=CARTESIAN_POINT('Ctrl Pts',(3.11488531,3.007773793,6.82257206));
#102145=CARTESIAN_POINT('Ctrl Pts',(3.488057068,3.07352872,6.652198303));
#102146=CARTESIAN_POINT('Ctrl Pts',(3.840420483,3.138525418,6.442140212));
#102147=CARTESIAN_POINT('Ctrl Pts',(3.84392870732549,3.13917254249503,6.44004881750999));
#102148=CARTESIAN_POINT('Ctrl Pts',(3.84743693165098,3.13981966699007,6.43795742301998));
#102149=CARTESIAN_POINT('Ctrl Pts',(3.225726914,3.007773793,6.492856527));
#102150=CARTESIAN_POINT('Ctrl Pts',(3.580864341,3.07352872,6.316420107));
#102151=CARTESIAN_POINT('Ctrl Pts',(3.914639774,3.138525418,6.10230247));
#102152=CARTESIAN_POINT('Ctrl Pts',(3.91796293140924,3.13917254249503,6.10017065758514));
#102153=CARTESIAN_POINT('Ctrl Pts',(3.92128608881848,3.13981966699007,6.09803884517028));
#102154=CARTESIAN_POINT('',(3.84042048042683,3.13852541850725,6.44214021129259));
#102155=CARTESIAN_POINT('',(3.87753012104247,3.13852541943002,6.2722213456103));
#102156=CARTESIAN_POINT('',(3.34146001010757,3.04797057324922,6.7145100401353));
#102157=CARTESIAN_POINT('Origin',(-0.0692568059026771,2.94648211319721,
-0.175668415170304));
#102158=CARTESIAN_POINT('Ctrl Pts',(3.22996834292612,3.00855922362653,6.49074762063523));
#102159=CARTESIAN_POINT('Ctrl Pts',(3.24848715409963,3.01545478681904,6.52800485343035));
#102160=CARTESIAN_POINT('Ctrl Pts',(3.26704885853801,3.02218156076036,6.56530019640403));
#102161=CARTESIAN_POINT('Ctrl Pts',(3.30420773701181,3.03530792012851,6.63987488250295));
#102162=CARTESIAN_POINT('Ctrl Pts',(3.3228260961376,3.04171498175259,6.677196736047));
#102163=CARTESIAN_POINT('Ctrl Pts',(3.34146000322131,3.04797057330893,6.71451003732055));
#102164=CARTESIAN_POINT('Ctrl Pts',(2.81969200434841,3.13983235804358,6.94977722071898));
#102165=CARTESIAN_POINT('Ctrl Pts',(2.82346629917421,3.13917888802179,6.94824111985949));
#102166=CARTESIAN_POINT('Ctrl Pts',(2.827240594,3.138525418,6.946705019));
#102167=CARTESIAN_POINT('Ctrl Pts',(3.205090136,3.073105688,6.79292397300001));
#102168=CARTESIAN_POINT('Ctrl Pts',(3.564030731,3.007781414,6.599066975));
#102169=CARTESIAN_POINT('Ctrl Pts',(2.50391258247664,3.13983235804358,6.80389475530675));
#102170=CARTESIAN_POINT('Ctrl Pts',(2.50760780273832,3.13917888802179,6.80253031015338));
#102171=CARTESIAN_POINT('Ctrl Pts',(2.511303023,3.138525418,6.801165865));
#102172=CARTESIAN_POINT('Ctrl Pts',(2.881236308,3.073105688,6.664569494));
#102173=CARTESIAN_POINT('Ctrl Pts',(3.234171275,3.007781414,6.48865441900001));
#102174=CARTESIAN_POINT('',(2.82724057644168,3.13852541980569,6.94670499124702));
#102175=CARTESIAN_POINT('Origin',(-0.0800272701647023,3.08928603326539,
-0.17568595985035));
#102176=CARTESIAN_POINT('',(2.66927181826374,3.13852541968788,6.87393543820857));
#102177=CARTESIAN_POINT('Origin',(-3.16587034365767E-14,3.22948687199933,
1.64798730217797E-13));
#102178=CARTESIAN_POINT('',(3.34749512821828,3.22840427023067,6.71150328635333));
#102179=CARTESIAN_POINT('Origin',(-0.104698240449298,3.0892995303119,-0.16017393657233));
#102180=CARTESIAN_POINT('Ctrl Pts',(2.82724058916065,3.13852541968788,6.94670500820955));
#102181=CARTESIAN_POINT('Ctrl Pts',(3.05006578700813,3.176642188,6.85601735800344));
#102182=CARTESIAN_POINT('Ctrl Pts',(3.26662104000823,3.214285714,6.75123596000317));
#102183=CARTESIAN_POINT('Ctrl Pts',(3.30717742265074,3.221335578992,6.73161254089966));
#102184=CARTESIAN_POINT('Ctrl Pts',(3.34749512040879,3.2284042698127,6.71150329039929));
#102185=CARTESIAN_POINT('Ctrl Pts',(1.575409703,3.007773793,7.332672382));
#102186=CARTESIAN_POINT('Ctrl Pts',(1.976482234,3.07352872,7.246502767));
#102187=CARTESIAN_POINT('Ctrl Pts',(2.365763869,3.138525418,7.117103436));
#102188=CARTESIAN_POINT('Ctrl Pts',(2.36963966098986,3.13917254249503,7.11581510167983));
#102189=CARTESIAN_POINT('Ctrl Pts',(2.37351545297971,3.13981966699007,7.11452676735966));
#102190=CARTESIAN_POINT('Ctrl Pts',(1.754538986,3.007773793,7.034493084));
#102191=CARTESIAN_POINT('Ctrl Pts',(2.139302112,3.07352872,6.938525699));
#102192=CARTESIAN_POINT('Ctrl Pts',(2.511303023,3.138525418,6.801165865));
#102193=CARTESIAN_POINT('Ctrl Pts',(2.5150067634836,3.13917254249503,6.7997982737846));
#102194=CARTESIAN_POINT('Ctrl Pts',(2.5187105039672,3.13981966699007,6.79843068256919));
#102195=CARTESIAN_POINT('',(2.36576386665506,3.13852541850724,7.11710343474332));
#102196=CARTESIAN_POINT('',(2.43853343772574,3.13852541943002,6.95913465339936));
#102197=CARTESIAN_POINT('',(1.81991735276004,3.04797057334258,7.27584365642433));
#102198=CARTESIAN_POINT('Origin',(-0.0298740646503137,2.94648209465332,
-0.186449427984996));
#102199=CARTESIAN_POINT('Ctrl Pts',(1.75913460499466,3.00855922359267,7.03334526460901));
#102200=CARTESIAN_POINT('Ctrl Pts',(1.76921125282428,3.01545478682352,7.07371244114721));
#102201=CARTESIAN_POINT('Ctrl Pts',(1.77932159850542,3.02218156078112,7.11412605755525));
#102202=CARTESIAN_POINT('Ctrl Pts',(1.79958036974931,3.03530792019689,7.19494528964447));
#102203=CARTESIAN_POINT('Ctrl Pts',(1.80974034659752,3.04171498183564,7.23539697594034));
#102204=CARTESIAN_POINT('Ctrl Pts',(1.81991734640429,3.04797057340381,7.27584365226265));
#102205=CARTESIAN_POINT('Ctrl Pts',(1.25977250362045,3.13983235804358,7.39344572270518));
#102206=CARTESIAN_POINT('Ctrl Pts',(1.26378877381022,3.13917888802179,7.39275689685259));
#102207=CARTESIAN_POINT('Ctrl Pts',(1.267805044,3.138525418,7.392068071));
#102208=CARTESIAN_POINT('Ctrl Pts',(1.669879053,3.073105688,7.323108823));
#102209=CARTESIAN_POINT('Ctrl Pts',(2.062101341,3.007781414,7.210945712));
#102210=CARTESIAN_POINT('Ctrl Pts',(0.982736247106169,3.13983235804358,
7.18309066712261));
#102211=CARTESIAN_POINT('Ctrl Pts',(0.986638390553085,3.13917888802179,
7.18255248506131));
#102212=CARTESIAN_POINT('Ctrl Pts',(0.990540534,3.138525418,7.182014303));
#102213=CARTESIAN_POINT('Ctrl Pts',(1.381189167,3.073105688,7.1281362));
#102214=CARTESIAN_POINT('Ctrl Pts',(1.763689251,3.007781414,7.032204507));
#102215=CARTESIAN_POINT('',(1.26780503335226,3.13852541976232,7.39206804027773));
#102216=CARTESIAN_POINT('Origin',(-0.0403889916659433,3.08928603899375,
-0.188782065731093));
#102217=CARTESIAN_POINT('',(1.12917279935051,3.13852541968788,7.28704118539612));
#102218=CARTESIAN_POINT('Origin',(-9.63855731339613E-14,3.229486871999,
-4.21537804662364E-13));
#102219=CARTESIAN_POINT('',(1.82645773643408,3.22840427022337,7.27420457056872));
#102220=CARTESIAN_POINT('Origin',(-0.067817762799324,3.08929952515512,-0.178936091177111));
#102221=CARTESIAN_POINT('Ctrl Pts',(1.26780504159327,3.13852541968788,7.39206805942139));
#102222=CARTESIAN_POINT('Ctrl Pts',(1.50491587500718,3.176642188,7.35140146700508));
#102223=CARTESIAN_POINT('Ctrl Pts',(1.73893308900733,3.214285714,7.29562277800485));
#102224=CARTESIAN_POINT('Ctrl Pts',(1.78275974095652,3.2213355789919,7.28517656685318));
#102225=CARTESIAN_POINT('Ctrl Pts',(1.8264577278493,3.22840426981285,7.27420457278075));
#102226=CARTESIAN_POINT('Ctrl Pts',(-0.03773031,3.007773793,7.499905094));
#102227=CARTESIAN_POINT('Ctrl Pts',(0.372489288,3.07352872,7.501968815));
#102228=CARTESIAN_POINT('Ctrl Pts',(0.780486765999999,3.138525418,7.459278813));
#102229=CARTESIAN_POINT('Ctrl Pts',(0.784548897924391,3.13917254249503,
7.4588537799316));
#102230=CARTESIAN_POINT('Ctrl Pts',(0.788611029848782,3.13981966699007,
7.45842874686319));
#102231=CARTESIAN_POINT('Ctrl Pts',(0.201310764,3.007773793,7.247204563));
#102232=CARTESIAN_POINT('Ctrl Pts',(0.597708493,3.07352872,7.236193541));
#102233=CARTESIAN_POINT('Ctrl Pts',(0.990540534000001,3.138525418,7.182014303));
#102234=CARTESIAN_POINT('Ctrl Pts',(0.994451674780801,3.13917254249503,
7.18147488002758));
#102235=CARTESIAN_POINT('Ctrl Pts',(0.998362815561602,3.13981966699007,
7.18093545705518));
#102236=CARTESIAN_POINT('',(0.78048676397796,3.13852541850725,7.45927881126957));
#102237=CARTESIAN_POINT('',(0.885513641295908,3.13852541943002,7.32064655905286));
#102238=CARTESIAN_POINT('',(0.213277382521218,3.04797057327008,7.49696690910154));
#102239=CARTESIAN_POINT('Origin',(0.0109054915341743,2.94648208325206,-0.188512453073895));
#102240=CARTESIAN_POINT('Ctrl Pts',(0.206045687659719,3.00855922379005,
7.24707150198745));
#102241=CARTESIAN_POINT('Ctrl Pts',(0.207208999418826,3.0154547870171,7.28866109792215));
#102242=CARTESIAN_POINT('Ctrl Pts',(0.208395237953114,3.02218156082844,
7.33030329111373));
#102243=CARTESIAN_POINT('Ctrl Pts',(0.210806624555049,3.03530792020359,
7.41358805137751));
#102244=CARTESIAN_POINT('Ctrl Pts',(0.212033149998714,3.04171498179988,
7.45527809421898));
#102245=CARTESIAN_POINT('Ctrl Pts',(0.213277377398708,3.04797057333011,
7.49696690365892));
#102246=CARTESIAN_POINT('Ctrl Pts',(-0.359052559442651,3.13983235804358,
7.49140492024465));
#102247=CARTESIAN_POINT('Ctrl Pts',(-0.354982110221325,3.13917888802179,
7.49159557812232));
#102248=CARTESIAN_POINT('Ctrl Pts',(-0.350911661,3.138525418,7.491786236));
#102249=CARTESIAN_POINT('Ctrl Pts',(0.056586281,3.073105688,7.510873243));
#102250=CARTESIAN_POINT('Ctrl Pts',(0.463750383,3.007781414,7.485648641));
#102251=CARTESIAN_POINT('Ctrl Pts',(-0.584391742461101,3.13983235804358,
7.22641324335268));
#102252=CARTESIAN_POINT('Ctrl Pts',(-0.58046513573055,3.13917888802179,
7.22672648917634));
#102253=CARTESIAN_POINT('Ctrl Pts',(-0.576538529,3.138525418,7.227039735));
#102254=CARTESIAN_POINT('Ctrl Pts',(-0.183440845,3.073105688,7.25839918));
#102255=CARTESIAN_POINT('Ctrl Pts',(0.210739078,3.007781414,7.246936528));
#102256=CARTESIAN_POINT('',(-0.350911665282579,3.13852541980569,7.49178620343906));
#102257=CARTESIAN_POINT('Origin',(0.00113783564030897,3.08928603443716,
-0.193050966742221));
#102258=CARTESIAN_POINT('',(-0.46372508454669,3.13852541968788,7.35941298615868));
#102259=CARTESIAN_POINT('Origin',(-2.81079413216867E-14,3.22948687199989,
-7.26415455565288E-13));
#102260=CARTESIAN_POINT('',(0.220017210746863,3.22840427020573,7.49677213367687));
#102261=CARTESIAN_POINT('Origin',(-0.0277662652739613,3.08929952349658,
-0.189331667288006));
#102262=CARTESIAN_POINT('Ctrl Pts',(-0.350911660861536,3.13852541968788,
7.49178622417456));
#102263=CARTESIAN_POINT('Ctrl Pts',(-0.110602231994232,3.176642188,7.50304221400634));
#102264=CARTESIAN_POINT('Ctrl Pts',(0.129934559005965,3.214285714,7.49887438300615));
#102265=CARTESIAN_POINT('Ctrl Pts',(0.17498219508154,3.22133557898442,7.4980938331641));
#102266=CARTESIAN_POINT('Ctrl Pts',(0.220017201815362,3.22840426981251,
7.49677213391338));
#102267=CARTESIAN_POINT('Ctrl Pts',(0.467202875,2.75,7.485433954));
#102268=CARTESIAN_POINT('Ctrl Pts',(0.872823804,2.68564607,7.46011715000001));
#102269=CARTESIAN_POINT('Ctrl Pts',(1.27333392,2.620518779,7.391117691));
#102270=CARTESIAN_POINT('Ctrl Pts',(0.214081497,2.75,7.24683856));
#102271=CARTESIAN_POINT('Ctrl Pts',(0.606773411,2.68564607,7.235237905));
#102272=CARTESIAN_POINT('Ctrl Pts',(0.995912368,2.620518779,7.181271375));
#102273=CARTESIAN_POINT('',(0.991263371367775,2.62129679675086,7.18191455012789));
#102274=CARTESIAN_POINT('Origin',(-0.0379383924044535,2.55361184896654,
-0.192401840764767));
#102275=CARTESIAN_POINT('Ctrl Pts',(1.02739270989941,2.66036061572379,7.42929769313666));
#102276=CARTESIAN_POINT('Ctrl Pts',(1.02133053819476,2.65417293169584,7.38803131424235));
#102277=CARTESIAN_POINT('Ctrl Pts',(1.01528456429805,2.64782918802562,7.34676106946382));
#102278=CARTESIAN_POINT('Ctrl Pts',(1.00324257965832,2.63481932854071,7.2643143704311));
#102279=CARTESIAN_POINT('Ctrl Pts',(0.997239354252857,2.62814542762809,
7.22308853316094));
#102280=CARTESIAN_POINT('Ctrl Pts',(0.991263375807131,2.62129679727074,
7.18191457244044));
#102281=CARTESIAN_POINT('Ctrl Pts',(0.77634725,2.620519775,7.459710782));
#102282=CARTESIAN_POINT('Ctrl Pts',(0.959930074,2.64969025,7.440604944));
#102283=CARTESIAN_POINT('Ctrl Pts',(1.142350843,2.678571429,7.412491791));
#102284=CARTESIAN_POINT('Ctrl Pts',(1.366589369,2.714073269,7.377934037));
#102285=CARTESIAN_POINT('Ctrl Pts',(1.588328914,2.75,7.329884805));
#102286=CARTESIAN_POINT('Ctrl Pts',(1.59236135128825,2.75065334439885,7.32901100725324));
#102287=CARTESIAN_POINT('Ctrl Pts',(1.5963937885765,2.7513066887977,7.32813720950648));
#102288=CARTESIAN_POINT('Ctrl Pts',(0.986554849,2.620519775,7.18256288));
#102289=CARTESIAN_POINT('Ctrl Pts',(1.163317088,2.64969025,7.158283853));
#102290=CARTESIAN_POINT('Ctrl Pts',(1.338671059,2.678571429,7.125339276));
#102291=CARTESIAN_POINT('Ctrl Pts',(1.554222808,2.714073269,7.08484255300001));
#102292=CARTESIAN_POINT('Ctrl Pts',(1.766932466,2.75,7.031390308));
#102293=CARTESIAN_POINT('Ctrl Pts',(1.77080069057172,2.75065334439885,7.03041825393595));
#102294=CARTESIAN_POINT('Ctrl Pts',(1.77466891514343,2.7513066887977,7.02944619987189));
#102295=CARTESIAN_POINT('Ctrl Pts',(1.76693247047358,2.75000000176745,7.03139031538271));
#102296=CARTESIAN_POINT('Ctrl Pts',(1.62477277725516,2.72598918233424,7.06711390973909));
#102297=CARTESIAN_POINT('Ctrl Pts',(1.48188408168206,2.70215892406901,7.09843317048902));
#102298=CARTESIAN_POINT('Ctrl Pts',(1.33867105724405,2.67857142871079,7.1253392763299));
#102299=CARTESIAN_POINT('Ctrl Pts',(1.22364114774488,2.65962575335661,7.1469504875505));
#102300=CARTESIAN_POINT('Ctrl Pts',(1.10777325899891,2.6405235296523,7.16583362630432));
#102301=CARTESIAN_POINT('Ctrl Pts',(0.991263374345238,2.62129679692748,
7.18191457191139));
#102302=CARTESIAN_POINT('Ctrl Pts',(2.065426964,2.75,7.20999386));
#102303=CARTESIAN_POINT('Ctrl Pts',(2.456122336,2.68564607,7.098072439));
#102304=CARTESIAN_POINT('Ctrl Pts',(2.832435904,2.620518779,6.944588314));
#102305=CARTESIAN_POINT('Ctrl Pts',(1.766932466,2.75,7.031390308));
#102306=CARTESIAN_POINT('Ctrl Pts',(2.147949663,2.68564607,6.935643716));
#102307=CARTESIAN_POINT('Ctrl Pts',(2.516389559,2.620518779,6.79928552));
#102308=CARTESIAN_POINT('',(2.51198751719057,2.62129679673515,6.80091305603547));
#102309=CARTESIAN_POINT('Origin',(-0.078412607116547,2.55361160406602,-0.179749174256227));
#102310=CARTESIAN_POINT('Ctrl Pts',(2.60045223490387,2.66036061567143,7.03474577850128));
#102311=CARTESIAN_POINT('Ctrl Pts',(2.58566074166918,2.65417293165183,6.99574737228981));
#102312=CARTESIAN_POINT('Ctrl Pts',(2.57088423644442,2.64782918797765,6.95674170839051));
#102313=CARTESIAN_POINT('Ctrl Pts',(2.54140015100389,2.63481931413965,6.87881115181285));
#102314=CARTESIAN_POINT('Ctrl Pts',(2.52667495880192,2.62814542051295,6.83983971336488));
#102315=CARTESIAN_POINT('Ctrl Pts',(2.51198752653413,2.62129679718683,6.80091307555531));
#102316=CARTESIAN_POINT('Ctrl Pts',(2.361813993,2.620519775,7.118415179));
#102317=CARTESIAN_POINT('Ctrl Pts',(2.536997563,2.64969025,7.060291145));
#102318=CARTESIAN_POINT('Ctrl Pts',(2.709109939,2.678571429,6.993620188));
#102319=CARTESIAN_POINT('Ctrl Pts',(2.920676996,2.714073269,6.911665721));
#102320=CARTESIAN_POINT('Ctrl Pts',(3.12690323,2.75,6.817072406));
#102321=CARTESIAN_POINT('Ctrl Pts',(3.1306535504753,2.75065334439885,6.8153521823447));
#102322=CARTESIAN_POINT('Ctrl Pts',(3.13440387095059,2.7513066887977,6.8136319586894));
#102323=CARTESIAN_POINT('Ctrl Pts',(2.507528449,2.620519775,6.802558422));
#102324=CARTESIAN_POINT('Ctrl Pts',(2.674938811,2.64969025,6.740848368));
#102325=CARTESIAN_POINT('Ctrl Pts',(2.839110994,2.678571429,6.670978097));
#102326=CARTESIAN_POINT('Ctrl Pts',(3.040917665,2.714073269,6.58509091));
#102327=CARTESIAN_POINT('Ctrl Pts',(3.237163637,2.75,6.48716206));
#102328=CARTESIAN_POINT('Ctrl Pts',(3.24073246174509,2.75065334439885,6.48538117808137));
#102329=CARTESIAN_POINT('Ctrl Pts',(3.24430128649018,2.7513066887977,6.48360029616274));
#102330=CARTESIAN_POINT('Ctrl Pts',(3.23716364320858,2.75000000185344,6.48716206666387));
#102331=CARTESIAN_POINT('Ctrl Pts',(3.10600708091653,2.72598918232688,6.55261059477203));
#102332=CARTESIAN_POINT('Ctrl Pts',(2.97319175854747,2.70215892403026,6.61391447450941));
#102333=CARTESIAN_POINT('Ctrl Pts',(2.83911099237912,2.67857142871485,6.67097809768983));
#102334=CARTESIAN_POINT('Ctrl Pts',(2.73141618969899,2.65962575340867,6.71681208068242));
#102335=CARTESIAN_POINT('Ctrl Pts',(2.62231654513112,2.64052352980419,6.76016191311457));
#102336=CARTESIAN_POINT('Ctrl Pts',(2.51198752491407,2.62129679699288,6.80091307706755));
#102337=CARTESIAN_POINT('Ctrl Pts',(3.567073983,2.75,6.597422466));
#102338=CARTESIAN_POINT('Ctrl Pts',(3.924575317,2.68564607,6.40412975));
#102339=CARTESIAN_POINT('Ctrl Pts',(4.259096333,2.620518779,6.17333770500001));
#102340=CARTESIAN_POINT('Ctrl Pts',(3.237163637,2.75,6.48716206));
#102341=CARTESIAN_POINT('Ctrl Pts',(3.588690177,2.68564607,6.311746536));
#102342=CARTESIAN_POINT('Ctrl Pts',(3.919203171,2.620518779,6.099372632));
#102343=CARTESIAN_POINT('',(3.91525391814552,2.62129679671748,6.10190842548336));
#102344=CARTESIAN_POINT('Origin',(-0.115220002471641,2.55361156385018,-0.158690101272749));
#102345=CARTESIAN_POINT('Ctrl Pts',(4.05191750338997,2.6603606157075,6.31125696986323));
#102346=CARTESIAN_POINT('Ctrl Pts',(4.02908832265019,2.6541729316882,6.27635005861745));
#102347=CARTESIAN_POINT('Ctrl Pts',(4.0062722191201,2.64782918796055,6.24143283708704));
#102348=CARTESIAN_POINT('Ctrl Pts',(3.96072473936658,2.63481932842818,6.17166253728937));
#102349=CARTESIAN_POINT('Ctrl Pts',(3.93796607992139,2.62814542752971,6.13676766959823));
#102350=CARTESIAN_POINT('Ctrl Pts',(3.9152539318273,2.62129679721806,6.10190844318046));
#102351=CARTESIAN_POINT('Ctrl Pts',(3.836844939,2.620519775,6.444270394));
#102352=CARTESIAN_POINT('Ctrl Pts',(3.995437865,2.64969025,6.349845979));
#102353=CARTESIAN_POINT('Ctrl Pts',(4.149194064,2.678571429,6.247734679));
#102354=CARTESIAN_POINT('Ctrl Pts',(4.338197014,2.714073269,6.122215598));
#102355=CARTESIAN_POINT('Ctrl Pts',(4.519267026,2.75,5.98550127800001));
#102356=CARTESIAN_POINT('Ctrl Pts',(4.52255986881779,2.75065334439885,5.98301506417736));
#102357=CARTESIAN_POINT('Ctrl Pts',(4.52585271163557,2.7513066887977,5.98052885035472));
#102358=CARTESIAN_POINT('Ctrl Pts',(3.911252806,2.620519775,6.104473891));
#102359=CARTESIAN_POINT('Ctrl Pts',(4.06148337,2.64969025,6.008218305));
#102360=CARTESIAN_POINT('Ctrl Pts',(4.206797255,2.678571429,5.904689396));
#102361=CARTESIAN_POINT('Ctrl Pts',(4.385422592,2.714073269,5.777427735));
#102362=CARTESIAN_POINT('Ctrl Pts',(4.556028634,2.75,5.63960132400001));
#102363=CARTESIAN_POINT('Ctrl Pts',(4.55913118463147,2.75065334439885,5.63709488628262));
#102364=CARTESIAN_POINT('Ctrl Pts',(4.56223373526293,2.7513066887977,5.63458844856525));
#102365=CARTESIAN_POINT('Ctrl Pts',(4.55602864119576,2.75000000176928,5.63960132856059));
#102366=CARTESIAN_POINT('Ctrl Pts',(4.44200794567386,2.72598918228978,5.73171449093605));
#102367=CARTESIAN_POINT('Ctrl Pts',(4.32547629386789,2.70215892402793,5.82013648845238));
#102368=CARTESIAN_POINT('Ctrl Pts',(4.20679725367195,2.67857142873605,5.90468939694617));
#102369=CARTESIAN_POINT('Ctrl Pts',(4.11147324763285,2.65962575344072,5.97260300576642));
#102370=CARTESIAN_POINT('Ctrl Pts',(4.01424322389773,2.64052352968139,6.03839254209647));
#102371=CARTESIAN_POINT('Ctrl Pts',(3.91525393011497,2.62129679688094,6.10190844418719));
#102372=CARTESIAN_POINT('Ctrl Pts',(4.901928588,2.75,5.676362931));
#102373=CARTESIAN_POINT('Ctrl Pts',(5.209519519,2.68564607,5.41073707200001));
#102374=CARTESIAN_POINT('Ctrl Pts',(5.486606152,2.620518779,5.113428687));
#102375=CARTESIAN_POINT('Ctrl Pts',(4.556028634,2.75,5.63960132400001));
#102376=CARTESIAN_POINT('Ctrl Pts',(4.861627526,2.68564607,5.392719102));
#102377=CARTESIAN_POINT('Ctrl Pts',(5.138759199,2.620518779,5.114259858));
#102378=CARTESIAN_POINT('',(5.13544739786056,2.62129679675748,5.11758533942526));
#102379=CARTESIAN_POINT('Origin',(-0.146640035537037,2.55361159747453,-0.130211287635851));
#102380=CARTESIAN_POINT('Ctrl Pts',(5.31391961274854,2.66036061567578,5.29266079998403));
#102381=CARTESIAN_POINT('Ctrl Pts',(5.28412021133306,2.65417293165882,5.26347759186377));
#102382=CARTESIAN_POINT('Ctrl Pts',(5.25433136546702,2.64782918802237,5.23428150368819));
#102383=CARTESIAN_POINT('Ctrl Pts',(5.19485020828765,2.63481932849264,5.17593375624));
#102384=CARTESIAN_POINT('Ctrl Pts',(5.16512226866306,2.62814542762031,5.14674715016722));
#102385=CARTESIAN_POINT('Ctrl Pts',(5.13544741478222,2.62129679733524,5.11758535350893));
#102386=CARTESIAN_POINT('Ctrl Pts',(5.13246928,2.620519775,5.468798688));
#102387=CARTESIAN_POINT('Ctrl Pts',(5.267055933,2.64969025,5.342489072));
#102388=CARTESIAN_POINT('Ctrl Pts',(5.395266487,2.678571429,5.209712039));
#102389=CARTESIAN_POINT('Ctrl Pts',(5.552867761,2.714073269,5.046497477));
#102390=CARTESIAN_POINT('Ctrl Pts',(5.700314919,2.75,4.874054762));
#102391=CARTESIAN_POINT('Ctrl Pts',(5.70299631449924,2.75065334439885,4.87091881061139));
#102392=CARTESIAN_POINT('Ctrl Pts',(5.70567770999848,2.7513066887977,4.86778285922278));
#102393=CARTESIAN_POINT('Ctrl Pts',(5.132091328,2.620519775,5.120950947));
#102394=CARTESIAN_POINT('Ctrl Pts',(5.258117479,2.64969025,4.994650632));
#102395=CARTESIAN_POINT('Ctrl Pts',(5.377778351,2.678571429,4.862303981));
#102396=CARTESIAN_POINT('Ctrl Pts',(5.524870032,2.714073269,4.69961846));
#102397=CARTESIAN_POINT('Ctrl Pts',(5.661858795,2.75,4.528339098));
#102398=CARTESIAN_POINT('Ctrl Pts',(5.6643499996969,2.75065334439885,4.52522430272956));
#102399=CARTESIAN_POINT('Ctrl Pts',(5.6668412043938,2.7513066887977,4.52210950745911));
#102400=CARTESIAN_POINT('Ctrl Pts',(5.66185880358697,2.75000000189433,4.52833910123001));
#102401=CARTESIAN_POINT('Ctrl Pts',(5.57030545547846,2.72598918234126,4.64280978801909));
#102402=CARTESIAN_POINT('Ctrl Pts',(5.47550636442511,2.70215892403391,4.75421538847654));
#102403=CARTESIAN_POINT('Ctrl Pts',(5.37777835008841,2.67857142877804,4.86230398217638));
#102404=CARTESIAN_POINT('Ctrl Pts',(5.29928238471252,2.65962575348233,4.94912165257316));
#102405=CARTESIAN_POINT('Ctrl Pts',(5.21846835055042,2.64052352972735,5.03427464719514));
#102406=CARTESIAN_POINT('Ctrl Pts',(5.13544741336457,2.62129679700693,5.11758535493291));
#102407=CARTESIAN_POINT('Ctrl Pts',(6.007574459,2.75,4.489882974));
#102408=CARTESIAN_POINT('Ctrl Pts',(6.250872378,2.68564607,4.164344342));
#102409=CARTESIAN_POINT('Ctrl Pts',(6.457568365,2.620518779,3.814421426));
#102410=CARTESIAN_POINT('Ctrl Pts',(5.661858795,2.75,4.528339098));
#102411=CARTESIAN_POINT('Ctrl Pts',(5.907240575,2.68564607,4.221534117));
#102412=CARTESIAN_POINT('Ctrl Pts',(6.118032557,2.620518779,3.890009978));
#102413=CARTESIAN_POINT('',(6.11551306419439,2.62129679673686,3.89396965038792));
#102414=CARTESIAN_POINT('Origin',(-0.171203284020705,2.55361160305888,-0.0956437659882275));
#102415=CARTESIAN_POINT('Ctrl Pts',(6.32744874717913,2.66036061564244,4.02658569320165));
#102416=CARTESIAN_POINT('Ctrl Pts',(6.29207251207898,2.65417293160338,4.00449076262624));
#102417=CARTESIAN_POINT('Ctrl Pts',(6.25670381706409,2.64782918797476,3.98238098412373));
#102418=CARTESIAN_POINT('Ctrl Pts',(6.18607025531124,2.63481932843167,3.93818406519795));
#102419=CARTESIAN_POINT('Ctrl Pts',(6.15076308075667,2.62814542754816,3.91607045407821));
#102420=CARTESIAN_POINT('Ctrl Pts',(6.11551308399253,2.6212967972428,3.89396966050844));
#102421=CARTESIAN_POINT('Ctrl Pts',(6.188105062,2.620519775,4.237612033));
#102422=CARTESIAN_POINT('Ctrl Pts',(6.29239232,2.64969025,4.085323313));
#102423=CARTESIAN_POINT('Ctrl Pts',(6.389062245,2.678571429,3.928089055));
#102424=CARTESIAN_POINT('Ctrl Pts',(6.50789258200001,2.714073269,3.734810744));
#102425=CARTESIAN_POINT('Ctrl Pts',(6.614822422,2.75,3.534702862));
#102426=CARTESIAN_POINT('Ctrl Pts',(6.61676699112971,2.75065334439885,3.53106380661613));
#102427=CARTESIAN_POINT('Ctrl Pts',(6.61871156025942,2.7513066887977,3.52742475123226));
#102428=CARTESIAN_POINT('Ctrl Pts',(6.112958964,2.620519775,3.897978027));
#102429=CARTESIAN_POINT('Ctrl Pts',(6.20888786,2.64969025,3.747538647));
#102430=CARTESIAN_POINT('Ctrl Pts',(6.297300509,2.678571429,3.592562637));
#102431=CARTESIAN_POINT('Ctrl Pts',(6.40598069,2.714073269,3.402060249));
#102432=CARTESIAN_POINT('Ctrl Pts',(6.502946732,2.75,3.205336768));
#102433=CARTESIAN_POINT('Ctrl Pts',(6.50471010480504,2.75065334439885,3.20175925953051));
#102434=CARTESIAN_POINT('Ctrl Pts',(6.50647347761008,2.7513066887977,3.19818175106102));
#102435=CARTESIAN_POINT('Ctrl Pts',(6.50294674220238,2.75000000214517,3.20533676924456));
#102436=CARTESIAN_POINT('Ctrl Pts',(6.43814167428525,2.72598918262104,3.33681245823215));
#102437=CARTESIAN_POINT('Ctrl Pts',(6.3695078439607,2.70215892421632,3.46599246044649));
#102438=CARTESIAN_POINT('Ctrl Pts',(6.29730050853279,2.67857142883765,3.59256263798011));
#102439=CARTESIAN_POINT('Ctrl Pts',(6.23930296822854,2.65962575352119,3.69422487150057));
#102440=CARTESIAN_POINT('Ctrl Pts',(6.17868369763219,2.64052352964207,3.7947596654705));
#102441=CARTESIAN_POINT('Ctrl Pts',(6.11551308270665,2.62129679686781,3.89396966220073));
#102442=CARTESIAN_POINT('Ctrl Pts',(6.832312826,2.75,3.093461079));
#102443=CARTESIAN_POINT('Ctrl Pts',(6.99994139199999,2.68564607,2.723231498));
#102444=CARTESIAN_POINT('Ctrl Pts',(7.126581858,2.620518779,2.337056058));
#102445=CARTESIAN_POINT('Ctrl Pts',(6.502946732,2.75,3.205336768));
#102446=CARTESIAN_POINT('Ctrl Pts',(6.676637621,2.68564607,2.852954888));
#102447=CARTESIAN_POINT('Ctrl Pts',(6.811233513,2.620518779,2.483867554));
#102448=CARTESIAN_POINT('',(6.80962413708076,2.62129679675697,2.48827626789476));
#102449=CARTESIAN_POINT('Origin',(-0.187761390900419,2.55361154127052,-0.0566040674048424));
#102450=CARTESIAN_POINT('Ctrl Pts',(7.04511341129868,2.66036061574169,2.57223191432732));
#102451=CARTESIAN_POINT('Ctrl Pts',(7.00581449606116,2.65417293172453,2.55825839585287));
#102452=CARTESIAN_POINT('Ctrl Pts',(6.96651975202736,2.64782918800484,2.54426875547398));
#102453=CARTESIAN_POINT('Ctrl Pts',(6.88803653220672,2.63481932842121,2.51628926384458));
#102454=CARTESIAN_POINT('Ctrl Pts',(6.84880104706384,2.62814542754618,2.50228265560733));
#102455=CARTESIAN_POINT('Ctrl Pts',(6.80962415850665,2.62129679727301,2.48827627372423));
#102456=CARTESIAN_POINT('Ctrl Pts',(6.954391929,2.620519775,2.808279349));
#102457=CARTESIAN_POINT('Ctrl Pts',(7.023503436,2.64969025,2.637132378));
#102458=CARTESIAN_POINT('Ctrl Pts',(7.084112554,2.678571429,2.462792993));
#102459=CARTESIAN_POINT('Ctrl Pts',(7.15861558,2.714073269,2.248488411));
#102460=CARTESIAN_POINT('Ctrl Pts',(7.22002818,2.75,2.030072186));
#102461=CARTESIAN_POINT('Ctrl Pts',(7.22114499684117,2.75065334439885,2.02610018483959));
#102462=CARTESIAN_POINT('Ctrl Pts',(7.22226181368234,2.7513066887977,2.02212818367917));
#102463=CARTESIAN_POINT('Ctrl Pts',(6.80799143300001,2.620519775,2.492739988));
#102464=CARTESIAN_POINT('Ctrl Pts',(6.86933754400001,2.64969025,2.325195919));
#102465=CARTESIAN_POINT('Ctrl Pts',(6.922367894,2.678571429,2.154837056));
#102466=CARTESIAN_POINT('Ctrl Pts',(6.987554811,2.714073269,1.945425482));
#102467=CARTESIAN_POINT('Ctrl Pts',(7.039964107,2.75,1.732456454));
#102468=CARTESIAN_POINT('Ctrl Pts',(7.04091719454892,2.75065334439885,1.72858351266357));
#102469=CARTESIAN_POINT('Ctrl Pts',(7.04187028209783,2.7513066887977,1.72471057132715));
#102470=CARTESIAN_POINT('Ctrl Pts',(7.03996411719344,2.75000000212625,1.73245645311726));
#102471=CARTESIAN_POINT('Ctrl Pts',(7.00493754211565,2.72598918242031,1.87478948781914));
#102472=CARTESIAN_POINT('Ctrl Pts',(6.96567821485752,2.702158924025,2.01570357841255));
#102473=CARTESIAN_POINT('Ctrl Pts',(6.92236789383464,2.67857142882524,2.154837057327));
#102474=CARTESIAN_POINT('Ctrl Pts',(6.88758067885014,2.65962575364295,2.26659024058532));
#102475=CARTESIAN_POINT('Ctrl Pts',(6.84999066209724,2.64052352987875,2.37780593736967));
#102476=CARTESIAN_POINT('Ctrl Pts',(6.80962415816835,2.62129679701491,2.48827627564519));
#102477=CARTESIAN_POINT('Ctrl Pts',(7.337579839,2.75,1.552392382));
#102478=CARTESIAN_POINT('Ctrl Pts',(7.421700926,2.68564607,1.154783377));
#102479=CARTESIAN_POINT('Ctrl Pts',(7.462364304,2.620518779,0.750412547000001));
#102480=CARTESIAN_POINT('Ctrl Pts',(7.039964107,2.75,1.732456454));
#102481=CARTESIAN_POINT('Ctrl Pts',(7.133842512,2.68564607,1.35097466));
#102482=CARTESIAN_POINT('Ctrl Pts',(7.18594876,2.620518779,0.961582243999999));
#102483=CARTESIAN_POINT('',(7.1853247538099,2.62129679675021,0.966233853240022));
#102484=CARTESIAN_POINT('Origin',(-0.195539767315837,2.5536115669031,-0.0149175448622552));
#102485=CARTESIAN_POINT('Ctrl Pts',(7.43335640141215,2.66036061571562,0.997603430550806));
#102486=CARTESIAN_POINT('Ctrl Pts',(7.39197237950679,2.65417293169836,0.992404710278094));
#102487=CARTESIAN_POINT('Ctrl Pts',(7.35058896583797,2.64782918801841,0.987189348332478));
#102488=CARTESIAN_POINT('Ctrl Pts',(7.26792587647577,2.63481932843988,0.976735573831541));
#102489=CARTESIAN_POINT('Ctrl Pts',(7.22659668848171,2.62814542757044,0.971490901712906));
#102490=CARTESIAN_POINT('Ctrl Pts',(7.18532477572538,2.62129679729411,0.966233854084293));
#102491=CARTESIAN_POINT('Ctrl Pts',(7.395499158,2.620519775,1.247634645));
#102492=CARTESIAN_POINT('Ctrl Pts',(7.426203336,2.64969025,1.065632063));
#102493=CARTESIAN_POINT('Ctrl Pts',(7.447917633,2.678571429,0.882339467));
#102494=CARTESIAN_POINT('Ctrl Pts',(7.474609669,2.714073269,0.657029259));
#102495=CARTESIAN_POINT('Ctrl Pts',(7.487633445,2.75,0.43051759));
#102496=CARTESIAN_POINT('Ctrl Pts',(7.48787028845513,2.75065334439885,0.426398369405856));
#102497=CARTESIAN_POINT('Ctrl Pts',(7.48810713191026,2.7513066887977,0.422279148811712));
#102498=CARTESIAN_POINT('Ctrl Pts',(7.184689789,2.620519775,0.970944197));
#102499=CARTESIAN_POINT('Ctrl Pts',(7.20858464,2.64969025,0.794129615));
#102500=CARTESIAN_POINT('Ctrl Pts',(7.22375305,2.678571429,0.616353689));
#102501=CARTESIAN_POINT('Ctrl Pts',(7.24239863499999,2.714073269,0.397824782));
#102502=CARTESIAN_POINT('Ctrl Pts',(7.247800585,2.75,0.178568402));
#102503=CARTESIAN_POINT('Ctrl Pts',(7.24789882198614,2.75065334439885,0.174581122228142));
#102504=CARTESIAN_POINT('Ctrl Pts',(7.24799705897229,2.7513066887977,0.170593842456285));
#102505=CARTESIAN_POINT('Ctrl Pts',(7.24780059470928,2.75000000206258,0.178568399286295));
#102506=CARTESIAN_POINT('Ctrl Pts',(7.24419031691365,2.72598918247015,0.325103444596959));
#102507=CARTESIAN_POINT('Ctrl Pts',(7.2361412148389,2.70215892409394,0.471162636311407));
#102508=CARTESIAN_POINT('Ctrl Pts',(7.22375304994782,2.67857142872828,0.616353690779953));
#102509=CARTESIAN_POINT('Ctrl Pts',(7.2138027715959,2.65962575337623,0.732972371121796));
#102510=CARTESIAN_POINT('Ctrl Pts',(7.20099967605123,2.64052352972992,0.84966864890671));
#102511=CARTESIAN_POINT('Ctrl Pts',(7.18532477574293,2.62129679699644,0.966233856230039));
#102512=CARTESIAN_POINT('Ctrl Pts',(7.499749774,2.75,-0.061264458));
#102513=CARTESIAN_POINT('Ctrl Pts',(7.496429973,2.68564607,-0.467661132));
#102514=CARTESIAN_POINT('Ctrl Pts',(7.449214889,2.620518779,-0.871319421));
#102515=CARTESIAN_POINT('Ctrl Pts',(7.247800585,2.75,0.178568402));
#102516=CARTESIAN_POINT('Ctrl Pts',(7.257476856,2.68564607,-0.214175642));
#102517=CARTESIAN_POINT('Ctrl Pts',(7.22465703000001,2.620518779,-0.605665582));
#102518=CARTESIAN_POINT('',(7.22504757083151,2.62129679672876,-0.600988582846018));
#102519=CARTESIAN_POINT('Origin',(-0.194175117513026,2.55361157223225,0.0274664925956096));
#102520=CARTESIAN_POINT('Ctrl Pts',(7.47402390811217,2.66036061571516,-0.623671881598151));
#102521=CARTESIAN_POINT('Ctrl Pts',(7.43248985057937,2.65417293169921,-0.619852717176769));
#102522=CARTESIAN_POINT('Ctrl Pts',(7.39095280939218,2.64782918798386,-0.616049936099405));
#102523=CARTESIAN_POINT('Ctrl Pts',(7.30797508488674,2.63481932839231,-0.608489186264437));
#102524=CARTESIAN_POINT('Ctrl Pts',(7.26648470091488,2.62814542749891,-0.604726687016057));
#102525=CARTESIAN_POINT('Ctrl Pts',(7.2250475927466,2.62129679719525,-0.600988586403805));
#102526=CARTESIAN_POINT('Ctrl Pts',(7.490801066,2.620519775,-0.37134807));
#102527=CARTESIAN_POINT('Ctrl Pts',(7.481662223,2.64969025,-0.555696023));
#102528=CARTESIAN_POINT('Ctrl Pts',(7.463466361,2.678571429,-0.739371272));
#102529=CARTESIAN_POINT('Ctrl Pts',(7.441099318,2.714073269,-0.965151851));
#102530=CARTESIAN_POINT('Ctrl Pts',(7.405125292,2.75,-1.18916753));
#102531=CARTESIAN_POINT('Ctrl Pts',(7.40447108751947,2.75065334439885,-1.19324135984913));
#102532=CARTESIAN_POINT('Ctrl Pts',(7.40381688303893,2.7513066887977,-1.19731518969825));
#102533=CARTESIAN_POINT('Ctrl Pts',(7.225440036,2.620519775,-0.596251866));
#102534=CARTESIAN_POINT('Ctrl Pts',(7.21076633,2.64969025,-0.774069308000001));
#102535=CARTESIAN_POINT('Ctrl Pts',(7.187363542,2.678571429,-0.95094969));
#102536=CARTESIAN_POINT('Ctrl Pts',(7.158595948,2.714073269,-1.168377763));
#102537=CARTESIAN_POINT('Ctrl Pts',(7.11673796300001,2.75,-1.383669311));
#102538=CARTESIAN_POINT('Ctrl Pts',(7.11597675597432,2.75065334439885,-1.38758448844839));
#102539=CARTESIAN_POINT('Ctrl Pts',(7.11521554894864,2.7513066887977,-1.39149966589679));
#102540=CARTESIAN_POINT('Ctrl Pts',(7.11673797190381,2.75000000204555,-1.38366931564545));
#102541=CARTESIAN_POINT('Ctrl Pts',(7.14471280393736,2.72598918246571,-1.23978407453484));
#102542=CARTESIAN_POINT('Ctrl Pts',(7.16825029390894,2.70215892410217,-1.09540934625179));
#102543=CARTESIAN_POINT('Ctrl Pts',(7.18736354224324,2.67857142879351,-0.95094968867717));
#102544=CARTESIAN_POINT('Ctrl Pts',(7.20271546464417,2.65962575353111,-0.83491847416344));
#102545=CARTESIAN_POINT('Ctrl Pts',(7.21529794894784,2.6405235296564,-0.718198202331916));
#102546=CARTESIAN_POINT('Ctrl Pts',(7.22504759310139,2.62129679694117,-0.600988584663608));
#102547=CARTESIAN_POINT('Ctrl Pts',(7.311239744,2.75,-1.672056639));
#102548=CARTESIAN_POINT('Ctrl Pts',(7.220634287,2.68564607,-2.068238326));
#102549=CARTESIAN_POINT('Ctrl Pts',(7.087748465,2.620518779,-2.452309461));
#102550=CARTESIAN_POINT('Ctrl Pts',(7.11673796300001,2.75,-1.383669311));
#102551=CARTESIAN_POINT('Ctrl Pts',(7.04175964800001,2.68564607,-1.769311329));
#102552=CARTESIAN_POINT('Ctrl Pts',(6.925548367,2.620518779,-2.14459316));
#102553=CARTESIAN_POINT('',(6.92693519374711,2.62129679672952,-2.14010946067906));
#102554=CARTESIAN_POINT('Origin',(-0.183731048098391,2.55361156244326,0.0685662800179587));
#102555=CARTESIAN_POINT('Ctrl Pts',(7.16521436356792,2.66036061573476,-2.21578498882252));
#102556=CARTESIAN_POINT('Ctrl Pts',(7.12547235665399,2.65417293170283,-2.20312651987865));
#102557=CARTESIAN_POINT('Ctrl Pts',(7.08572391417432,2.64782918801842,-2.19048340989173));
#102558=CARTESIAN_POINT('Ctrl Pts',(7.0063114127143,2.63481931404231,-2.16526164050143));
#102559=CARTESIAN_POINT('Ctrl Pts',(6.96659992419542,2.62814542052546,-2.15266791534343));
#102560=CARTESIAN_POINT('Ctrl Pts',(6.92693521452292,2.62129679727275,-2.14010946891741));
#102561=CARTESIAN_POINT('Ctrl Pts',(7.235841442,2.620519775,-1.972966961));
#102562=CARTESIAN_POINT('Ctrl Pts',(7.18728689900001,2.64969025,-2.15104038));
#102563=CARTESIAN_POINT('Ctrl Pts',(7.130031697,2.678571429,-2.326509831));
#102564=CARTESIAN_POINT('Ctrl Pts',(7.059651433,2.714073269,-2.542203533));
#102565=CARTESIAN_POINT('Ctrl Pts',(6.97636171000001,2.75,-2.753248498));
#102566=CARTESIAN_POINT('Ctrl Pts',(6.9748470474496,2.75065334439885,-2.75708644935128));
#102567=CARTESIAN_POINT('Ctrl Pts',(6.97333238489921,2.7513066887977,-2.76092440070255));
#102568=CARTESIAN_POINT('Ctrl Pts',(6.928336737,2.620519775,-2.135567854));
#102569=CARTESIAN_POINT('Ctrl Pts',(6.875780601,2.64969025,-2.30607361));
#102570=CARTESIAN_POINT('Ctrl Pts',(6.814900903,2.678571429,-2.47378772));
#102571=CARTESIAN_POINT('Ctrl Pts',(6.740065271,2.714073269,-2.679948262));
#102572=CARTESIAN_POINT('Ctrl Pts',(6.652904584,2.75,-2.881208184));
#102573=CARTESIAN_POINT('Ctrl Pts',(6.6513195261596,2.75065334439885,-2.88486818976985));
#102574=CARTESIAN_POINT('Ctrl Pts',(6.6497344683192,2.7513066887977,-2.8885281955397));
#102575=CARTESIAN_POINT('Ctrl Pts',(6.65290459080522,2.75000000185146,-2.88120818990272));
#102576=CARTESIAN_POINT('Ctrl Pts',(6.71115646016654,2.72598918232521,-2.74670066785988));
#102577=CARTESIAN_POINT('Ctrl Pts',(6.76517995624436,2.70215892402454,-2.6107612053006));
#102578=CARTESIAN_POINT('Ctrl Pts',(6.81490090360504,2.67857142871297,-2.47378771833322));
#102579=CARTESIAN_POINT('Ctrl Pts',(6.85483718843397,2.65962575339801,-2.36376945786321));
#102580=CARTESIAN_POINT('Ctrl Pts',(6.89221690912954,2.64052352967758,-2.25248290397871));
#102581=CARTESIAN_POINT('Ctrl Pts',(6.92693521473911,2.6212967969307,-2.14010946713021));
#102582=CARTESIAN_POINT('Ctrl Pts',(6.78086427000001,2.75,-3.20466531));
#102583=CARTESIAN_POINT('Ctrl Pts',(6.607209766,2.68564607,-3.572106995));
#102584=CARTESIAN_POINT('Ctrl Pts',(6.394866801,2.620518779,-3.918632236));
#102585=CARTESIAN_POINT('Ctrl Pts',(6.652904584,2.75,-2.881208184));
#102586=CARTESIAN_POINT('Ctrl Pts',(6.49677758500001,2.68564607,-3.241715985));
#102587=CARTESIAN_POINT('Ctrl Pts',(6.302608759,2.620518779,-3.583241945));
#102588=CARTESIAN_POINT('',(6.30492702512,2.62129679675646,-3.57916119849814));
#102589=CARTESIAN_POINT('Origin',(-0.164695427352005,2.5536115784274,0.106459792061169));
#102590=CARTESIAN_POINT('Ctrl Pts',(6.52136735922966,2.66036061573153,-3.70429045328558));
#102591=CARTESIAN_POINT('Ctrl Pts',(6.48527569502537,2.65417293170606,-3.68338457550447));
#102592=CARTESIAN_POINT('Ctrl Pts',(6.44917444389617,2.6478291880154,-3.6624923141011));
#102593=CARTESIAN_POINT('Ctrl Pts',(6.37704057755396,2.6348193285101,-3.6207889214374));
#102594=CARTESIAN_POINT('Ctrl Pts',(6.3409647573002,2.62814542763408,-3.59995280950605));
#102595=CARTESIAN_POINT('Ctrl Pts',(6.30492704406959,2.6212967973458,-3.57916121100208));
#102596=CARTESIAN_POINT('Ctrl Pts',(6.64254191400001,2.620519775,-3.48233211));
#102597=CARTESIAN_POINT('Ctrl Pts',(6.556842028,2.64969025,-3.64580448));
#102598=CARTESIAN_POINT('Ctrl Pts',(6.463204676,2.678571429,-3.804863377));
#102599=CARTESIAN_POINT('Ctrl Pts',(6.348102093,2.714073269,-4.000384604));
#102600=CARTESIAN_POINT('Ctrl Pts',(6.221391209,2.75,-4.188590626));
#102601=CARTESIAN_POINT('Ctrl Pts',(6.21908691233759,2.75065334439885,-4.19201324049569));
#102602=CARTESIAN_POINT('Ctrl Pts',(6.21678261567518,2.7513066887977,-4.19543585499139));
#102603=CARTESIAN_POINT('Ctrl Pts',(6.307272113,2.620519775,-3.575027062));
#102604=CARTESIAN_POINT('Ctrl Pts',(6.219291012,2.64969025,-3.730248473));
#102605=CARTESIAN_POINT('Ctrl Pts',(6.123781072,2.678571429,-3.880954185));
#102606=CARTESIAN_POINT('Ctrl Pts',(6.006376632,2.714073269,-4.06620736));
#102607=CARTESIAN_POINT('Ctrl Pts',(5.87798878,2.75,-4.244024965));
#102608=CARTESIAN_POINT('Ctrl Pts',(5.87565398689053,2.75065334439885,-4.247258661276));
#102609=CARTESIAN_POINT('Ctrl Pts',(5.87331919378106,2.7513066887977,-4.25049235755201));
#102610=CARTESIAN_POINT('Ctrl Pts',(5.87798878589075,2.75000000214011,-4.24402497340688));
#102611=CARTESIAN_POINT('Ctrl Pts',(5.96379390012507,2.72598918248584,-4.12518459223727));
#102612=CARTESIAN_POINT('Ctrl Pts',(6.04577732236949,2.70215892409288,-4.00403677323589));
#102613=CARTESIAN_POINT('Ctrl Pts',(6.12378107301353,2.6785714287419,-3.88095418361733));
#102614=CARTESIAN_POINT('Ctrl Pts',(6.18643434290713,2.65962575347408,-3.78209320983747));
#102615=CARTESIAN_POINT('Ctrl Pts',(6.2468634659768,2.64052352978639,-3.68144400870869));
#102616=CARTESIAN_POINT('Ctrl Pts',(6.304927044608,2.62129679704562,-3.57916120950667));
#102617=CARTESIAN_POINT('Ctrl Pts',(5.933423119,2.75,-4.587427393));
#102618=CARTESIAN_POINT('Ctrl Pts',(5.684839461,2.68564607,-4.90894791));
#102619=CARTESIAN_POINT('Ctrl Pts',(5.402968272,2.620518779,-5.201724123));
#102620=CARTESIAN_POINT('Ctrl Pts',(5.87798878,2.75,-4.244024965));
#102621=CARTESIAN_POINT('Ctrl Pts',(5.648013423,2.68564607,-4.562541604));
#102622=CARTESIAN_POINT('Ctrl Pts',(5.38496617,2.620518779,-4.854342319));
#102623=CARTESIAN_POINT('',(5.38810747655047,2.62129679676453,-4.85085533687023));
#102624=CARTESIAN_POINT('Origin',(-0.137959584860747,2.55361155743023,0.139375774651469));
#102625=CARTESIAN_POINT('Ctrl Pts',(5.57258846503529,2.66036061568084,-5.0195874129108));
#102626=CARTESIAN_POINT('Ctrl Pts',(5.54183474961983,2.65417293167813,-4.99141166200556));
#102627=CARTESIAN_POINT('Ctrl Pts',(5.51106874422187,2.64782918799662,-4.96324714814558));
#102628=CARTESIAN_POINT('Ctrl Pts',(5.44958625629412,2.63481931415693,-4.90701204664053));
#102629=CARTESIAN_POINT('Ctrl Pts',(5.41883305299396,2.62814542059962,-4.87890786977764));
#102630=CARTESIAN_POINT('Ctrl Pts',(5.38810749187737,2.62129679730596,-4.85085535319451));
#102631=CARTESIAN_POINT('Ctrl Pts',(5.73864450900001,2.620519775,-4.828867279));
#102632=CARTESIAN_POINT('Ctrl Pts',(5.619806511,2.64969025,-4.970094815));
#102633=CARTESIAN_POINT('Ctrl Pts',(5.494165387,2.678571429,-5.10530574));
#102634=CARTESIAN_POINT('Ctrl Pts',(5.33972255400001,2.714073269,-5.271512136));
#102635=CARTESIAN_POINT('Ctrl Pts',(5.175515369,2.75,-5.428078911));
#102636=CARTESIAN_POINT('Ctrl Pts',(5.17252918457452,2.75065334439885,-5.43092615099776));
#102637=CARTESIAN_POINT('Ctrl Pts',(5.16954300014905,2.7513066887977,-5.43377339099553));
#102638=CARTESIAN_POINT('Ctrl Pts',(5.391286454,2.620519775,-4.84732197900001));
#102639=CARTESIAN_POINT('Ctrl Pts',(5.271994288,2.64969025,-4.980001063));
#102640=CARTESIAN_POINT('Ctrl Pts',(5.146320044,2.678571429,-5.106651545));
#102641=CARTESIAN_POINT('Ctrl Pts',(4.991836498,2.714073269,-5.26233512));
#102642=CARTESIAN_POINT('Ctrl Pts',(4.828224754,2.75,-5.408395855));
#102643=CARTESIAN_POINT('Ctrl Pts',(4.82524939794747,2.75065334439885,-5.41105203774884));
#102644=CARTESIAN_POINT('Ctrl Pts',(4.82227404189494,2.7513066887977,-5.41370822049767));
#102645=CARTESIAN_POINT('Ctrl Pts',(4.82822475771829,2.75000000220518,-5.40839586474511));
#102646=CARTESIAN_POINT('Ctrl Pts',(4.9375709645692,2.72598918255007,-5.3107794688955));
#102647=CARTESIAN_POINT('Ctrl Pts',(5.04368086000124,2.70215892412742,-5.21008803075968));
#102648=CARTESIAN_POINT('Ctrl Pts',(5.14632004501918,2.67857142879894,-5.10665154411776));
#102649=CARTESIAN_POINT('Ctrl Pts',(5.22876070350902,2.65962575356672,-5.0235704863683));
#102650=CARTESIAN_POINT('Ctrl Pts',(5.30941363040642,2.64052352974731,-4.93826488256848));
#102651=CARTESIAN_POINT('Ctrl Pts',(5.38810749292814,2.62129679694484,-4.85085535157521));
#102652=CARTESIAN_POINT('Ctrl Pts',(4.808541698,2.75,-5.75568647));
#102653=CARTESIAN_POINT('Ctrl Pts',(4.49665238,2.68564607,-6.016251877));
#102654=CARTESIAN_POINT('Ctrl Pts',(4.158432951,2.620518779,-6.241589172));
#102655=CARTESIAN_POINT('Ctrl Pts',(4.828224754,2.75,-5.408395855));
#102656=CARTESIAN_POINT('Ctrl Pts',(4.535154431,2.68564607,-5.670027848));
#102657=CARTESIAN_POINT('Ctrl Pts',(4.215528549,2.620518779,-5.898459041));
#102658=CARTESIAN_POINT('',(4.21934601090526,2.62129679674693,-5.89572887059208));
#102659=CARTESIAN_POINT('Origin',(-0.104772268716402,2.55361159886235,0.165774192984351));
#102660=CARTESIAN_POINT('Ctrl Pts',(4.36324152744183,2.66036061573346,-6.10017404411017));
#102661=CARTESIAN_POINT('Ctrl Pts',(4.33926377051569,2.65417293173651,-6.06604588682158));
#102662=CARTESIAN_POINT('Ctrl Pts',(4.31527159526947,2.64782918804367,-6.0319260618976));
#102663=CARTESIAN_POINT('Ctrl Pts',(4.26731541777163,2.63481931396713,-5.96378878721195));
#102664=CARTESIAN_POINT('Ctrl Pts',(4.24332277513809,2.62814542050229,-5.92973064133862));
#102665=CARTESIAN_POINT('Ctrl Pts',(4.21934602294037,2.62129679727644,-5.89572888996312));
#102666=CARTESIAN_POINT('Ctrl Pts',(4.566414464,2.620519775,-5.949609982));
#102667=CARTESIAN_POINT('Ctrl Pts',(4.419995088,2.64969025,-6.061989039));
#102668=CARTESIAN_POINT('Ctrl Pts',(4.268225031,2.678571429,-6.167029681));
#102669=CARTESIAN_POINT('Ctrl Pts',(4.081663524,2.714073269,-6.29614962));
#102670=CARTESIAN_POINT('Ctrl Pts',(3.887638183,2.75,-6.41375626));
#102671=CARTESIAN_POINT('Ctrl Pts',(3.88410974146778,2.75065334439885,-6.41589499172907));
#102672=CARTESIAN_POINT('Ctrl Pts',(3.88058129993557,2.7513066887977,-6.41803372345814));
#102673=CARTESIAN_POINT('Ctrl Pts',(4.223210233,2.620519775,-5.892961507));
#102674=CARTESIAN_POINT('Ctrl Pts',(4.07818497,2.64969025,-5.996894338));
#102675=CARTESIAN_POINT('Ctrl Pts',(3.928222811,2.678571429,-6.093567555));
#102676=CARTESIAN_POINT('Ctrl Pts',(3.743883638,2.714073269,-6.212401939));
#102677=CARTESIAN_POINT('Ctrl Pts',(3.552698305,2.75,-6.319876166));
#102678=CARTESIAN_POINT('Ctrl Pts',(3.54922151034096,2.75065334439885,-6.3218306350618));
#102679=CARTESIAN_POINT('Ctrl Pts',(3.54574471568191,2.7513066887977,-6.3237851041236));
#102680=CARTESIAN_POINT('Ctrl Pts',(3.55269830635737,2.75000000180332,-6.31987617446485));
#102681=CARTESIAN_POINT('Ctrl Pts',(3.68047269970421,2.7259891823433,-6.24804819932019));
#102682=CARTESIAN_POINT('Ctrl Pts',(3.80574748764423,2.70215892406801,-6.17252136266766));
#102683=CARTESIAN_POINT('Ctrl Pts',(3.92822281185286,2.67857142883575,-6.0935675544502));
#102684=CARTESIAN_POINT('Ctrl Pts',(4.02659602465126,2.65962575356054,-6.03015118985405));
#102685=CARTESIAN_POINT('Ctrl Pts',(4.12370151429173,2.6405235297314,-5.96417797883247));
#102686=CARTESIAN_POINT('Ctrl Pts',(4.21934602375908,2.62129679691319,-5.89572888850613));
#102687=CARTESIAN_POINT('Ctrl Pts',(3.458818211,2.75,-6.654816044));
#102688=CARTESIAN_POINT('Ctrl Pts',(3.098206832,2.68564607,-6.84224259300001));
#102689=CARTESIAN_POINT('Ctrl Pts',(2.719453928,2.620518779,-6.989604448));
#102690=CARTESIAN_POINT('Ctrl Pts',(3.552698305,2.75,-6.319876166));
#102691=CARTESIAN_POINT('Ctrl Pts',(3.210236658,2.68564607,-6.512389893));
#102692=CARTESIAN_POINT('Ctrl Pts',(2.848977497,2.620518779,-6.666770374));
#102693=CARTESIAN_POINT('',(2.85329261535825,2.6212967967578,-6.66492467544232));
#102694=CARTESIAN_POINT('Origin',(-0.066686121994719,2.55361157478581,0.184421228183209));
#102695=CARTESIAN_POINT('Ctrl Pts',(2.94987426576481,2.66036061570823,-6.89552331690139));
#102696=CARTESIAN_POINT('Ctrl Pts',(2.93379364027752,2.65417293168017,-6.85703854795253));
#102697=CARTESIAN_POINT('Ctrl Pts',(2.91769714239881,2.64782918797754,-6.81855881708673));
#102698=CARTESIAN_POINT('Ctrl Pts',(2.88550968917187,2.63481932838112,-6.74170547885327));
#102699=CARTESIAN_POINT('Ctrl Pts',(2.86939945647989,2.6281454275173,-6.70328583852385));
#102700=CARTESIAN_POINT('Ctrl Pts',(2.85329262215917,2.62129679725448,-6.6649246965331));
#102701=CARTESIAN_POINT('Ctrl Pts',(3.180663955,2.620519775,-6.792155535));
#102702=CARTESIAN_POINT('Ctrl Pts',(3.013509606,2.64969025,-6.870431394));
#102703=CARTESIAN_POINT('Ctrl Pts',(2.842707217,2.678571429,-6.940390168));
#102704=CARTESIAN_POINT('Ctrl Pts',(2.632750443,2.714073269,-7.026386145));
#102705=CARTESIAN_POINT('Ctrl Pts',(2.417979356,2.75,-7.099533494));
#102706=CARTESIAN_POINT('Ctrl Pts',(2.41407364337821,2.75065334439885,-7.10086371273768));
#102707=CARTESIAN_POINT('Ctrl Pts',(2.41016793075642,2.7513066887977,-7.10219393147536));
#102708=CARTESIAN_POINT('Ctrl Pts',(2.857661396,2.620519775,-6.66305270500001));
#102709=CARTESIAN_POINT('Ctrl Pts',(2.693684256,2.64969025,-6.7333795));
#102710=CARTESIAN_POINT('Ctrl Pts',(2.526446244,2.678571429,-6.795555119));
#102711=CARTESIAN_POINT('Ctrl Pts',(2.320870939,2.714073269,-6.871983747));
#102712=CARTESIAN_POINT('Ctrl Pts',(2.111051631,2.75,-6.935846092));
#102713=CARTESIAN_POINT('Ctrl Pts',(2.10723596879426,2.75065334439885,-6.93700745859924));
#102714=CARTESIAN_POINT('Ctrl Pts',(2.10342030658853,2.7513066887977,-6.93816882519847));
#102715=CARTESIAN_POINT('Ctrl Pts',(2.11105163072352,2.75000000211533,-6.93584610220118));
#102716=CARTESIAN_POINT('Ctrl Pts',(2.25127962127389,2.72598918249932,-6.89316514142643));
#102717=CARTESIAN_POINT('Ctrl Pts',(2.38986159126746,2.70215892411409,-6.84633445600132));
#102718=CARTESIAN_POINT('Ctrl Pts',(2.52644624583777,2.6785714287138,-6.79555511846654));
#102719=CARTESIAN_POINT('Ctrl Pts',(2.63615219227389,2.65962575336085,-6.75476872620667));
#102720=CARTESIAN_POINT('Ctrl Pts',(2.74516969954801,2.64052352965217,-6.71121274234204));
#102721=CARTESIAN_POINT('Ctrl Pts',(2.85329262422745,2.62129679697703,-6.66492469606858));
#102722=CARTESIAN_POINT('Ctrl Pts',(1.947364229,2.75,-7.242773817));
#102723=CARTESIAN_POINT('Ctrl Pts',(1.554892575,2.68564607,-7.34829765));
#102724=CARTESIAN_POINT('Ctrl Pts',(1.153316261,2.620518779,-7.410793588));
#102725=CARTESIAN_POINT('Ctrl Pts',(2.111051631,2.75,-6.93584609200001));
#102726=CARTESIAN_POINT('Ctrl Pts',(1.735211787,2.68564607,-7.050239824));
#102727=CARTESIAN_POINT('Ctrl Pts',(1.349211424,2.620518779,-7.12335093400001));
#102728=CARTESIAN_POINT('',(1.35382242820159,2.62129679672353,-7.12247600992274));
#102729=CARTESIAN_POINT('Origin',(-0.0254819632860184,2.55361154608468,
0.194445344653661));
#102730=CARTESIAN_POINT('Ctrl Pts',(1.39857416152078,2.66036061573687,-7.36844558304455));
#102731=CARTESIAN_POINT('Ctrl Pts',(1.39114257989476,2.65417293171228,-7.32740370749941));
#102732=CARTESIAN_POINT('Ctrl Pts',(1.38369441393053,2.64782918799579,-7.28636334001544));
#102733=CARTESIAN_POINT('Ctrl Pts',(1.36878066512432,2.6348193141661,-7.20438734954117));
#102734=CARTESIAN_POINT('Ctrl Pts',(1.36130617631967,2.62814542053127,-7.16340276316861));
#102735=CARTESIAN_POINT('Ctrl Pts',(1.35382242975113,2.62129679720304,-7.1224760318306));
#102736=CARTESIAN_POINT('Ctrl Pts',(1.646189134,2.620519775,-7.317107443));
#102737=CARTESIAN_POINT('Ctrl Pts',(1.466115765,2.64969025,-7.35762001300001));
#102738=CARTESIAN_POINT('Ctrl Pts',(1.284267572,2.678571429,-7.389225724));
#102739=CARTESIAN_POINT('Ctrl Pts',(1.060732878,2.714073269,-7.428076663));
#102740=CARTESIAN_POINT('Ctrl Pts',(0.835258502,2.75,-7.453344433));
#102741=CARTESIAN_POINT('Ctrl Pts',(0.831158145063998,2.75065334439885,
-7.45380393921004));
#102742=CARTESIAN_POINT('Ctrl Pts',(0.827057788127997,2.7513066887977,-7.45426344542008));
#102743=CARTESIAN_POINT('Ctrl Pts',(1.358491487,2.620519775,-7.121586964));
#102744=CARTESIAN_POINT('Ctrl Pts',(1.18322986,2.64969025,-7.155019319));
#102745=CARTESIAN_POINT('Ctrl Pts',(1.00653586,2.678571429,-7.179790078));
#102746=CARTESIAN_POINT('Ctrl Pts',(0.789336895,2.714073269,-7.210239234));
#102747=CARTESIAN_POINT('Ctrl Pts',(0.570694529000001,2.75,-7.227503563));
#102748=CARTESIAN_POINT('Ctrl Pts',(0.566718415359787,2.75065334439885,
-7.22781752289387));
#102749=CARTESIAN_POINT('Ctrl Pts',(0.562742301719575,2.7513066887977,-7.22813148278776));
#102750=CARTESIAN_POINT('Ctrl Pts',(0.57069452699854,2.75000000202792,-7.22750357280113));
#102751=CARTESIAN_POINT('Ctrl Pts',(0.716819209619973,2.72598918245556,
-7.21596534231266));
#102752=CARTESIAN_POINT('Ctrl Pts',(0.862228423498231,2.7021589240943,-7.2000205595361));
#102753=CARTESIAN_POINT('Ctrl Pts',(1.00653586114367,2.67857142881306,-7.17979007783967));
#102754=CARTESIAN_POINT('Ctrl Pts',(1.12244481134483,2.65962575358551,-7.16354078428866));
#102755=CARTESIAN_POINT('Ctrl Pts',(1.23827679923776,2.64052352976744,-7.14443865663331));
#102756=CARTESIAN_POINT('Ctrl Pts',(1.35382243243794,2.62129679689708,-7.12247603205826));
#102757=CARTESIAN_POINT('Ctrl Pts',(0.344853659,2.75,-7.492067535));
#102758=CARTESIAN_POINT('Ctrl Pts',(-0.06112673,2.68564607,-7.510754476));
#102759=CARTESIAN_POINT('Ctrl Pts',(-0.466749192,2.620518779,-7.485462256));
#102760=CARTESIAN_POINT('Ctrl Pts',(0.570694529,2.75,-7.227503563));
#102761=CARTESIAN_POINT('Ctrl Pts',(0.179050341,2.68564607,-7.258428376));
#102762=CARTESIAN_POINT('Ctrl Pts',(-0.213642275,2.620518779,-7.246851522));
#102763=CARTESIAN_POINT('',(-0.208950991335437,2.62129679670998,-7.24698828190642));
#102764=CARTESIAN_POINT('Origin',(0.0169137971775209,2.55361155556727,0.195377074967155));
#102765=CARTESIAN_POINT('Ctrl Pts',(-0.218121715942913,2.66036061575241,
-7.49682752321785));
#102766=CARTESIAN_POINT('Ctrl Pts',(-0.216556761285011,2.65417293173166,
-7.45514761364917));
#102767=CARTESIAN_POINT('Ctrl Pts',(-0.215008327401407,2.64782918799023,
-7.41346561156725));
#102768=CARTESIAN_POINT('Ctrl Pts',(-0.211950989513393,2.6348193284523,
-7.33020025072329));
#102769=CARTESIAN_POINT('Ctrl Pts',(-0.21044025237885,2.62814542754474,
-7.28856701830798));
#102770=CARTESIAN_POINT('Ctrl Pts',(-0.208950993846219,2.6212967972171,
-7.24698830450965));
#102771=CARTESIAN_POINT('Ctrl Pts',(0.034740338,2.620519775,-7.49991954));
#102772=CARTESIAN_POINT('Ctrl Pts',(-0.14983202,2.64969025,-7.500774497));
#102773=CARTESIAN_POINT('Ctrl Pts',(-0.334222997,2.678571429,-7.492549298));
#102774=CARTESIAN_POINT('Ctrl Pts',(-0.560883377,2.714073269,-7.482438573));
#102775=CARTESIAN_POINT('Ctrl Pts',(-0.786518112,2.75,-7.45864527));
#102776=CARTESIAN_POINT('Ctrl Pts',(-0.790621385139384,2.75065334439885,
-7.45821257766166));
#102777=CARTESIAN_POINT('Ctrl Pts',(-0.794724658278768,2.7513066887977,
-7.45777988532332));
#102778=CARTESIAN_POINT('Ctrl Pts',(-0.204199974,2.620519775,-7.247123731));
#102779=CARTESIAN_POINT('Ctrl Pts',(-0.382551049,2.64969025,-7.242098388));
#102780=CARTESIAN_POINT('Ctrl Pts',(-0.560439023,2.678571429,-7.228306033));
#102781=CARTESIAN_POINT('Ctrl Pts',(-0.779105665,2.714073269,-7.211351947));
#102782=CARTESIAN_POINT('Ctrl Pts',(-0.996347613999999,2.75,-7.181211));
#102783=CARTESIAN_POINT('Ctrl Pts',(-1.00029826040238,2.75065334439885,
-7.18066287278802));
#102784=CARTESIAN_POINT('Ctrl Pts',(-1.00424890680475,2.7513066887977,-7.18011474557605));
#102785=CARTESIAN_POINT('Ctrl Pts',(-0.996347618322142,2.7500000020761,
-7.18121100914202));
#102786=CARTESIAN_POINT('Ctrl Pts',(-0.851158871176989,2.72598918253573,
-7.20135502381853));
#102787=CARTESIAN_POINT('Ctrl Pts',(-0.705721587186126,2.70215892416151,
-7.21704170399089));
#102788=CARTESIAN_POINT('Ctrl Pts',(-0.560439021319831,2.67857142875185,
-7.22830603329573));
#102789=CARTESIAN_POINT('Ctrl Pts',(-0.443746839286387,2.65962575341567,
-7.23735363741317));
#102790=CARTESIAN_POINT('Ctrl Pts',(-0.32651654668961,2.6405235296885,-7.24359856009063));
#102791=CARTESIAN_POINT('Ctrl Pts',(-0.208950991956025,2.62129679689047,
-7.24698830445382));
#102792=CARTESIAN_POINT('Ctrl Pts',(-1.273781884,2.75,-7.391040503));
#102793=CARTESIAN_POINT('Ctrl Pts',(-1.674287817,2.68564607,-7.32201677));
#102794=CARTESIAN_POINT('Ctrl Pts',(-2.064989971,2.620518779,-7.210119029));
#102795=CARTESIAN_POINT('Ctrl Pts',(-0.996347614,2.75,-7.181211));
#102796=CARTESIAN_POINT('Ctrl Pts',(-1.3854833,2.68564607,-7.127220885));
#102797=CARTESIAN_POINT('Ctrl Pts',(-1.766506299,2.620518779,-7.031497386));
#102798=CARTESIAN_POINT('',(-1.76195409432501,2.62129679672433,-7.03263943647596));
#102799=CARTESIAN_POINT('Origin',(0.0585186503573701,2.55361154586131,0.187173271427979));
#102800=CARTESIAN_POINT('Ctrl Pts',(-1.82461846412332,2.66036061571567,
-7.27466614044675));
#102801=CARTESIAN_POINT('Ctrl Pts',(-1.8141301486489,2.65417293170062,-7.2342971029069));
#102802=CARTESIAN_POINT('Ctrl Pts',(-1.80365751794335,2.64782918797959,
-7.19392247040153));
#102803=CARTESIAN_POINT('Ctrl Pts',(-1.78277206752517,2.63481932841364,
-7.11326104422478));
#102804=CARTESIAN_POINT('Ctrl Pts',(-1.77234673630568,2.62814542753473,
-7.07292593747618));
#102805=CARTESIAN_POINT('Ctrl Pts',(-1.76195410139986,2.62129679725034,
-7.03263945744462));
#102806=CARTESIAN_POINT('Ctrl Pts',(-1.578332876,2.620519775,-7.332043735));
#102807=CARTESIAN_POINT('Ctrl Pts',(-1.758773826,2.64969025,-7.29320110200001));
#102808=CARTESIAN_POINT('Ctrl Pts',(-1.93708567,2.678571429,-7.245529595));
#102809=CARTESIAN_POINT('Ctrl Pts',(-2.156273349,2.714073269,-7.18692997));
#102810=CARTESIAN_POINT('Ctrl Pts',(-2.371518013,2.75,-7.115188143));
#102811=CARTESIAN_POINT('Ctrl Pts',(-2.37543233784093,2.75065334439885,
-7.11388348433696));
#102812=CARTESIAN_POINT('Ctrl Pts',(-2.37934666268186,2.7513066887977,-7.11257882567393));
#102813=CARTESIAN_POINT('Ctrl Pts',(-1.75734327,2.620519775,-7.033793047));
#102814=CARTESIAN_POINT('Ctrl Pts',(-1.930444297,2.64969025,-6.990544984));
#102815=CARTESIAN_POINT('Ctrl Pts',(-2.1012084,2.678571429,-6.938834431));
#102816=CARTESIAN_POINT('Ctrl Pts',(-2.31111811,2.714073269,-6.875269858));
#102817=CARTESIAN_POINT('Ctrl Pts',(-2.516801651,2.75,-6.799132993));
#102818=CARTESIAN_POINT('Ctrl Pts',(-2.52054210234939,2.75065334439885,
-6.79774840851628));
#102819=CARTESIAN_POINT('Ctrl Pts',(-2.52428255369877,2.7513066887977,-6.79636382403254));
#102820=CARTESIAN_POINT('Ctrl Pts',(-2.5168016566078,2.75000000185138,-6.7991329999353));
#102821=CARTESIAN_POINT('Ctrl Pts',(-2.37933770907025,2.72598918241709,
-6.85001734795752));
#102822=CARTESIAN_POINT('Ctrl Pts',(-2.24067284049077,2.70215892412675,
-6.89660199923303));
#102823=CARTESIAN_POINT('Ctrl Pts',(-2.10120839845448,2.67857142876085,
-6.93883443167389));
#102824=CARTESIAN_POINT('Ctrl Pts',(-1.98918938248059,2.65962575341989,
-6.97275587723097));
#102825=CARTESIAN_POINT('Ctrl Pts',(-1.87604234262511,2.64052352971441,
-7.00405584468662));
#102826=CARTESIAN_POINT('Ctrl Pts',(-1.76195409969139,2.62129679698603,
-7.03263945807132));
#102827=CARTESIAN_POINT('Ctrl Pts',(-2.832856802,2.75,-6.944416631));
#102828=CARTESIAN_POINT('Ctrl Pts',(-3.209161066,2.68564607,-6.79090969800001));
#102829=CARTESIAN_POINT('Ctrl Pts',(-3.566674115,2.620518779,-6.59763865));
#102830=CARTESIAN_POINT('Ctrl Pts',(-2.516801651,2.75,-6.799132993));
#102831=CARTESIAN_POINT('Ctrl Pts',(-2.885233281,2.68564607,-6.662752466));
#102832=CARTESIAN_POINT('Ctrl Pts',(-3.236770452,2.620518779,-6.487358248));
#102833=CARTESIAN_POINT('',(-3.23257018276947,2.62129679674423,-6.48945218719692));
#102834=CARTESIAN_POINT('Origin',(0.0973871803849591,2.55361159636233,0.170217400774161));
#102835=CARTESIAN_POINT('Ctrl Pts',(-3.34579808097766,2.66036061570176,
-6.7123494544089));
#102836=CARTESIAN_POINT('Ctrl Pts',(-3.3268768267527,2.65417293169771,-6.67517890034009));
#102837=CARTESIAN_POINT('Ctrl Pts',(-3.30796968780511,2.64782918798304,
-6.63799951031197));
#102838=CARTESIAN_POINT('Ctrl Pts',(-3.27023266366539,2.63481931404014,
-6.56371357577716));
#102839=CARTESIAN_POINT('Ctrl Pts',(-3.25138023767489,2.6281454204954,-6.52656266338797));
#102840=CARTESIAN_POINT('Ctrl Pts',(-3.23257019393207,2.6212967972269,-6.48945220628804));
#102841=CARTESIAN_POINT('Ctrl Pts',(-3.117605,2.620519775,-6.82132971400001));
#102842=CARTESIAN_POINT('Ctrl Pts',(-3.285477323,2.64969025,-6.74460573));
#102843=CARTESIAN_POINT('Ctrl Pts',(-3.44937237,2.678571429,-6.65971698));
#102844=CARTESIAN_POINT('Ctrl Pts',(-3.650838376,2.714073269,-6.55536851));
#102845=CARTESIAN_POINT('Ctrl Pts',(-3.845628367,2.75,-6.439032727));
#102846=CARTESIAN_POINT('Ctrl Pts',(-3.84917071404994,2.75065334439885,
-6.4369171063996));
#102847=CARTESIAN_POINT('Ctrl Pts',(-3.85271306109988,2.7513066887977,-6.43480148579919));
#102848=CARTESIAN_POINT('Ctrl Pts',(-3.228315149,2.620519775,-6.491570018));
#102849=CARTESIAN_POINT('Ctrl Pts',(-3.388072114,2.64969025,-6.41212146700001));
#102850=CARTESIAN_POINT('Ctrl Pts',(-3.543727607,2.678571429,-6.324910643));
#102851=CARTESIAN_POINT('Ctrl Pts',(-3.735065241,2.714073269,-6.217707792));
#102852=CARTESIAN_POINT('Ctrl Pts',(-3.919572839,2.75,-6.099135083));
#102853=CARTESIAN_POINT('Ctrl Pts',(-3.92292819592626,2.75065334439885,
-6.09697878285453));
#102854=CARTESIAN_POINT('Ctrl Pts',(-3.92628355285251,2.7513066887977,-6.09482248270906));
#102855=CARTESIAN_POINT('Ctrl Pts',(-3.91957284540621,2.75000000173482,
-6.09913508878106));
#102856=CARTESIAN_POINT('Ctrl Pts',(-3.79626135957307,2.72598918222916,
-6.17838047388788));
#102857=CARTESIAN_POINT('Ctrl Pts',(-3.67085272169801,2.70215892397846,
-6.25368484994515));
#102858=CARTESIAN_POINT('Ctrl Pts',(-3.54372760583484,2.67857142879977,
-6.32491064390992));
#102859=CARTESIAN_POINT('Ctrl Pts',(-3.4416196408124,2.65962575360389,-6.38211980256457));
#102860=CARTESIAN_POINT('Ctrl Pts',(-3.33784648368696,2.64052352982283,
-6.43701126295269));
#102861=CARTESIAN_POINT('Ctrl Pts',(-3.23257019267236,2.62129679701602,
-6.48945220717682));
#102862=CARTESIAN_POINT('Ctrl Pts',(-4.259470484,2.75,-6.173079555));
#102863=CARTESIAN_POINT('Ctrl Pts',(-4.593977511,2.68564607,-5.942267236));
#102864=CARTESIAN_POINT('Ctrl Pts',(-4.901584541,2.620518779,-5.67666002));
#102865=CARTESIAN_POINT('Ctrl Pts',(-3.919572839,2.75,-6.099135083));
#102866=CARTESIAN_POINT('Ctrl Pts',(-4.250072961,2.68564607,-5.886741148));
#102867=CARTESIAN_POINT('Ctrl Pts',(-4.555686816,2.620518779,-5.63987744800001));
#102868=CARTESIAN_POINT('',(-4.55203488165151,2.62129679675248,-5.64282536603537));
#102869=CARTESIAN_POINT('Origin',(0.131702096318875,2.55361160479069,0.145302536969056));
#102870=CARTESIAN_POINT('Ctrl Pts',(-4.71053189794187,2.66036061569364,
-5.83617076779155));
#102871=CARTESIAN_POINT('Ctrl Pts',(-4.68406244165634,2.65417293167332,
-5.803936750918));
#102872=CARTESIAN_POINT('Ctrl Pts',(-4.65760487150524,2.64782918798595,
-5.77169107051523));
#102873=CARTESIAN_POINT('Ctrl Pts',(-4.60478083769685,2.63481931393408,
-5.70725424395961));
#102874=CARTESIAN_POINT('Ctrl Pts',(-4.57838282326677,2.62814542045161,
-5.67502461382145));
#102875=CARTESIAN_POINT('Ctrl Pts',(-4.55203489663523,2.62129679725494,
-5.64282538215023));
#102876=CARTESIAN_POINT('Ctrl Pts',(-4.511101379,2.620519775,-5.991657896));
#102877=CARTESIAN_POINT('Ctrl Pts',(-4.658555551,2.64969025,-5.880640089));
#102878=CARTESIAN_POINT('Ctrl Pts',(-4.800370252,2.678571429,-5.762503401));
#102879=CARTESIAN_POINT('Ctrl Pts',(-4.974694258,2.714073269,-5.617285305));
#102880=CARTESIAN_POINT('Ctrl Pts',(-5.139921412,2.75,-5.461795298));
#102881=CARTESIAN_POINT('Ctrl Pts',(-5.14292614503858,2.75065334439885,
-5.4589676395317));
#102882=CARTESIAN_POINT('Ctrl Pts',(-5.14593087807715,2.7513066887977,-5.4561399810634));
#102883=CARTESIAN_POINT('Ctrl Pts',(-4.548334599,2.620519775,-5.64580839));
#102884=CARTESIAN_POINT('Ctrl Pts',(-4.687277446,2.64969025,-5.533874277));
#102885=CARTESIAN_POINT('Ctrl Pts',(-4.82054605,2.678571429,-5.415241063));
#102886=CARTESIAN_POINT('Ctrl Pts',(-4.984364872,2.714073269,-5.26941262000001));
#102887=CARTESIAN_POINT('Ctrl Pts',(-5.139069158,2.75,-5.113948395));
#102888=CARTESIAN_POINT('Ctrl Pts',(-5.14188252776459,2.75065334439885,
-5.11112120538942));
#102889=CARTESIAN_POINT('Ctrl Pts',(-5.14469589752919,2.7513066887977,-5.10829401577884));
#102890=CARTESIAN_POINT('Ctrl Pts',(-5.13906916729271,2.75000000215022,
-5.11394839941884));
#102891=CARTESIAN_POINT('Ctrl Pts',(-5.03567604992564,2.72598918253933,
-5.21784939570737));
#102892=CARTESIAN_POINT('Ctrl Pts',(-4.92938761055078,2.70215892413535,
-5.31835234710694));
#102893=CARTESIAN_POINT('Ctrl Pts',(-4.82054604927562,2.67857142885136,
-5.41524106427285));
#102894=CARTESIAN_POINT('Ctrl Pts',(-4.73312359013776,2.65962575362265,
-5.49306289968832));
#102895=CARTESIAN_POINT('Ctrl Pts',(-4.64357663284416,2.64052352977815,
-5.56897918933333));
#102896=CARTESIAN_POINT('Ctrl Pts',(-4.5520348957225,2.62129679707988,-5.64282538356341));
#102897=CARTESIAN_POINT('Ctrl Pts',(-5.48691606000001,2.75,-5.113096141));
#102898=CARTESIAN_POINT('Ctrl Pts',(-5.763984674,2.68564607,-4.815770962));
#102899=CARTESIAN_POINT('Ctrl Pts',(-6.007302322,2.620518779,-4.490247077));
#102900=CARTESIAN_POINT('Ctrl Pts',(-5.13906915800001,2.75,-5.113948395));
#102901=CARTESIAN_POINT('Ctrl Pts',(-5.416183953,2.68564607,-4.835472356));
#102902=CARTESIAN_POINT('Ctrl Pts',(-5.661584328,2.620518779,-4.528682248));
#102903=CARTESIAN_POINT('',(-5.65865148836948,2.62129679673279,-4.53234630297675));
#102904=CARTESIAN_POINT('Origin',(0.159858817764672,2.55361156890335,0.113593444025223));
#102905=CARTESIAN_POINT('Ctrl Pts',(-5.85500647919589,2.66036061571563,
-4.68709922284819));
#102906=CARTESIAN_POINT('Ctrl Pts',(-5.82222650337217,2.65417293170312,
-4.66130897015096));
#102907=CARTESIAN_POINT('Ctrl Pts',(-5.7894556283497,2.64782918801518,-4.63550477145482));
#102908=CARTESIAN_POINT('Ctrl Pts',(-5.72401457821685,2.63481931397628,
-4.58393004824197));
#102909=CARTESIAN_POINT('Ctrl Pts',(-5.69130531690168,2.62814542047764,
-4.55812872183861));
#102910=CARTESIAN_POINT('Ctrl Pts',(-5.6586515072447,2.62129679723727,-4.53234631570846));
#102911=CARTESIAN_POINT('Ctrl Pts',(-5.693663671,2.620519775,-4.881822815));
#102912=CARTESIAN_POINT('Ctrl Pts',(-5.8138049,2.64969025,-4.741702254));
#102913=CARTESIAN_POINT('Ctrl Pts',(-5.926908156,2.678571429,-4.595841568));
#102914=CARTESIAN_POINT('Ctrl Pts',(-6.06593896600001,2.714073269,-4.416544081));
#102915=CARTESIAN_POINT('Ctrl Pts',(-6.193877446,2.75,-4.22917039));
#102916=CARTESIAN_POINT('Ctrl Pts',(-6.19620406706957,2.75065334439885,
-4.22576291183265));
#102917=CARTESIAN_POINT('Ctrl Pts',(-6.19853068813914,2.7513066887977,-4.22235543366531));
#102918=CARTESIAN_POINT('Ctrl Pts',(-5.655678979,2.620519775,-4.536055036));
#102919=CARTESIAN_POINT('Ctrl Pts',(-5.767310893,2.64969025,-4.396869275));
#102920=CARTESIAN_POINT('Ctrl Pts',(-5.871961118,2.678571429,-4.25236083));
#102921=CARTESIAN_POINT('Ctrl Pts',(-6.000601142,2.714073269,-4.074725571));
#102922=CARTESIAN_POINT('Ctrl Pts',(-6.118268315,2.75,-3.889639164));
#102923=CARTESIAN_POINT('Ctrl Pts',(-6.12040814754998,2.75065334439885,
-3.88627328116149));
#102924=CARTESIAN_POINT('Ctrl Pts',(-6.12254798009995,2.7513066887977,-3.88290739832298));
#102925=CARTESIAN_POINT('Ctrl Pts',(-6.11826832433658,2.75000000195366,
-3.88963916712843));
#102926=CARTESIAN_POINT('Ctrl Pts',(-6.03962812370742,2.72598918244455,
-4.01333747952319));
#102927=CARTESIAN_POINT('Ctrl Pts',(-5.95742981306564,2.7021589241026,-4.13433960064318));
#102928=CARTESIAN_POINT('Ctrl Pts',(-5.87196111701464,2.67857142872806,
-4.25236083136066));
#102929=CARTESIAN_POINT('Ctrl Pts',(-5.80331193947458,2.65962575341578,
-4.34715647935858));
#102930=CARTESIAN_POINT('Ctrl Pts',(-5.73217829903779,2.64052352969838,
-4.44054783755659));
#102931=CARTESIAN_POINT('Ctrl Pts',(-5.65865150590329,2.62129679689485,
-4.53234631705455));
#102932=CARTESIAN_POINT('Ctrl Pts',(-6.45779954,2.75,-3.814030034));
#102933=CARTESIAN_POINT('Ctrl Pts',(-6.664474319,2.68564607,-3.464094591));
#102934=CARTESIAN_POINT('Ctrl Pts',(-6.832125323,2.620518779,-3.093875171));
#102935=CARTESIAN_POINT('Ctrl Pts',(-6.118268315,2.75,-3.889639164));
#102936=CARTESIAN_POINT('Ctrl Pts',(-6.32904020300001,2.68564607,-3.55810225));
#102937=CARTESIAN_POINT('Ctrl Pts',(-6.502752449,2.620518779,-3.205730898));
#102938=CARTESIAN_POINT('',(-6.50067584106015,2.62129679674404,-3.20993976355605));
#102939=CARTESIAN_POINT('Origin',(0.180540677085579,2.55361154875563,0.0765727896387824));
#102940=CARTESIAN_POINT('Ctrl Pts',(-6.72570746453641,2.66036061567559,
-3.3188641275846));
#102941=CARTESIAN_POINT('Ctrl Pts',(-6.68814972429273,2.65417293167416,
-3.30072356240331));
#102942=CARTESIAN_POINT('Ctrl Pts',(-6.65059787432564,2.64782918802872,
-3.28256742095169));
#102943=CARTESIAN_POINT('Ctrl Pts',(-6.57559984230319,2.63481932852972,
-3.24626641781343));
#102944=CARTESIAN_POINT('Ctrl Pts',(-6.53810873796849,2.6281454276242,-3.22809981464685));
#102945=CARTESIAN_POINT('Ctrl Pts',(-6.50067586214077,2.62129679727841,
-3.20993977181534));
#102946=CARTESIAN_POINT('Ctrl Pts',(-6.609996578,2.620519775,-3.543719125));
#102947=CARTESIAN_POINT('Ctrl Pts',(-6.69720719300001,2.64969025,-3.381047692));
#102948=CARTESIAN_POINT('Ctrl Pts',(-6.776310422,2.678571429,-3.21428329));
#102949=CARTESIAN_POINT('Ctrl Pts',(-6.87354710900001,2.714073269,-3.009290165));
#102950=CARTESIAN_POINT('Ctrl Pts',(-6.958214653,2.75,-2.798794176));
#102951=CARTESIAN_POINT('Ctrl Pts',(-6.9597543718694,2.75065334439885,-2.79496620803394));
#102952=CARTESIAN_POINT('Ctrl Pts',(-6.96129409073881,2.7513066887977,-2.79113824006787));
#102953=CARTESIAN_POINT('Ctrl Pts',(-6.498570095,2.620519775,-3.21420079));
#102954=CARTESIAN_POINT('Ctrl Pts',(-6.577671293,2.64969025,-3.054271554));
#102955=CARTESIAN_POINT('Ctrl Pts',(-6.64880981,2.678571429,-2.890644931));
#102956=CARTESIAN_POINT('Ctrl Pts',(-6.736255972,2.714073269,-2.689508882));
#102957=CARTESIAN_POINT('Ctrl Pts',(-6.811384045,2.75,-2.483454729));
#102958=CARTESIAN_POINT('Ctrl Pts',(-6.81275028412961,2.75065334439885,
-2.47970753789814));
#102959=CARTESIAN_POINT('Ctrl Pts',(-6.81411652325921,2.7513066887977,-2.47596034679627));
#102960=CARTESIAN_POINT('Ctrl Pts',(-6.81138405521894,2.75000000212232,
-2.48345472924284));
#102961=CARTESIAN_POINT('Ctrl Pts',(-6.76117389920765,2.725989182386,-2.62116636306209));
#102962=CARTESIAN_POINT('Ctrl Pts',(-6.70690921864762,2.70215892399437,
-2.75700972931182));
#102963=CARTESIAN_POINT('Ctrl Pts',(-6.64880980919581,2.67857142867351,
-2.89064493284972));
#102964=CARTESIAN_POINT('Ctrl Pts',(-6.60214387345002,2.65962575339749,
-2.99798185511659));
#102965=CARTESIAN_POINT('Ctrl Pts',(-6.55274967912501,2.64052352965437,
-3.10448140515898));
#102966=CARTESIAN_POINT('Ctrl Pts',(-6.50067586096218,2.62129679690187,
-3.20993977341216));
#102967=CARTESIAN_POINT('Ctrl Pts',(-7.12672349100001,2.75,-2.336624121));
#102968=CARTESIAN_POINT('Ctrl Pts',(-7.253340552,2.68564607,-1.950441006));
#102969=CARTESIAN_POINT('Ctrl Pts',(-7.33748573700001,2.620518779,-1.5528371));
#102970=CARTESIAN_POINT('Ctrl Pts',(-6.811384045,2.75,-2.483454729));
#102971=CARTESIAN_POINT('Ctrl Pts',(-6.945957567,2.68564607,-2.114359238));
#102972=CARTESIAN_POINT('Ctrl Pts',(-7.039859092,2.620518779,-1.732883135));
#102973=CARTESIAN_POINT('',(-7.03873581629141,2.62129679674192,-1.73744000847421));
#102974=CARTESIAN_POINT('Origin',(0.192780490359736,2.55361158252651,0.0359716161125356));
#102975=CARTESIAN_POINT('Ctrl Pts',(-7.28192184408587,2.66036061572226,
-1.79544263397009));
#102976=CARTESIAN_POINT('Ctrl Pts',(-7.24134249763625,2.65417293168304,
-1.78579998894316));
#102977=CARTESIAN_POINT('Ctrl Pts',(-7.20076555515356,2.64782918799088,
-1.77614086563833));
#102978=CARTESIAN_POINT('Ctrl Pts',(-7.11971729231985,2.63481932841169,
-1.75681091979893));
#102979=CARTESIAN_POINT('Ctrl Pts',(-7.07919742648692,2.62814542752202,
-1.74712852112551));
#102980=CARTESIAN_POINT('Ctrl Pts',(-7.03873583813208,2.62129679722243,
-1.73744001214078));
#102981=CARTESIAN_POINT('Ctrl Pts',(-7.217253392,2.620519775,-2.039915067));
#102982=CARTESIAN_POINT('Ctrl Pts',(-7.26745552200001,2.64969025,-1.862299097));
#102983=CARTESIAN_POINT('Ctrl Pts',(-7.308859943,2.678571429,-1.682428699));
#102984=CARTESIAN_POINT('Ctrl Pts',(-7.359755829,2.714073269,-1.461325186));
#102985=CARTESIAN_POINT('Ctrl Pts',(-7.39719347800001,2.75,-1.237549456));
#102986=CARTESIAN_POINT('Ctrl Pts',(-7.39787429914903,2.75065334439885,
-1.23347998973562));
#102987=CARTESIAN_POINT('Ctrl Pts',(-7.39855512029806,2.7513066887977,-1.22941052347124));
#102988=CARTESIAN_POINT('Ctrl Pts',(-7.037595296,2.620519775,-1.742054088));
#102989=CARTESIAN_POINT('Ctrl Pts',(-7.080467094,2.64969025,-1.568859488));
#102990=CARTESIAN_POINT('Ctrl Pts',(-7.114767544,2.678571429,-1.393765687));
#102991=CARTESIAN_POINT('Ctrl Pts',(-7.156930959,2.714073269,-1.178533747));
#102992=CARTESIAN_POINT('Ctrl Pts',(-7.186007028,2.75,-0.961146711));
#102993=CARTESIAN_POINT('Ctrl Pts',(-7.18653578990772,2.75065334439885,
-0.9571934261227));
#102994=CARTESIAN_POINT('Ctrl Pts',(-7.18706455181544,2.7513066887977,-0.953240141245399));
#102995=CARTESIAN_POINT('Ctrl Pts',(-7.18600703699163,2.75000000185139,
-0.961146709604796));
#102996=CARTESIAN_POINT('Ctrl Pts',(-7.16657469761462,2.7259891822928,-1.10643242097761));
#102997=CARTESIAN_POINT('Ctrl Pts',(-7.14278100306208,2.70215892400084,
-1.25076514649307));
#102998=CARTESIAN_POINT('Ctrl Pts',(-7.11476754411235,2.67857142885841,
-1.39376568827563));
#102999=CARTESIAN_POINT('Ctrl Pts',(-7.09226689836446,2.65962575370281,
-1.50862492879154));
#103000=CARTESIAN_POINT('Ctrl Pts',(-7.06692176743887,2.64052352974924,
-1.62325287091066));
#103001=CARTESIAN_POINT('Ctrl Pts',(-7.03873583780033,2.62129679695612,
-1.73744001381952));
#103002=CARTESIAN_POINT('Ctrl Pts',(-7.462409772,2.75,-0.749960261));
#103003=CARTESIAN_POINT('Ctrl Pts',(-7.503048642,2.68564607,-0.345586968));
#103004=CARTESIAN_POINT('Ctrl Pts',(-7.499753473,2.620518779,0.060809907));
#103005=CARTESIAN_POINT('Ctrl Pts',(-7.186007028,2.75,-0.961146711));
#103006=CARTESIAN_POINT('Ctrl Pts',(-7.238089675,2.68564607,-0.571751139));
#103007=CARTESIAN_POINT('Ctrl Pts',(-7.247789749,2.620518779,-0.179007682));
#103008=CARTESIAN_POINT('',(-7.24767232795708,2.62129679675596,-0.183699489826389));
#103009=CARTESIAN_POINT('Origin',(0.196006361824517,2.55361159069313,-0.00631146489151906));
#103010=CARTESIAN_POINT('Ctrl Pts',(-7.49764165155661,2.66036061571001,
-0.188068238498516));
#103011=CARTESIAN_POINT('Ctrl Pts',(-7.45593814404777,2.65417293169288,
-0.18737439329813));
#103012=CARTESIAN_POINT('Ctrl Pts',(-7.41423344183167,2.64782918798851,
-0.186663938151601));
#103013=CARTESIAN_POINT('Ctrl Pts',(-7.33092467541011,2.63481932842647,
-0.185208896412547));
#103014=CARTESIAN_POINT('Ctrl Pts',(-7.28927071209075,2.62814542755626,
-0.184463440166955));
#103015=CARTESIAN_POINT('Ctrl Pts',(-7.24767235005735,2.62129679727333,
-0.183699488584394));
#103016=CARTESIAN_POINT('Ctrl Pts',(-7.487039458,2.620519775,-0.440726847));
#103017=CARTESIAN_POINT('Ctrl Pts',(-7.497885707,2.64969025,-0.256471467));
#103018=CARTESIAN_POINT('Ctrl Pts',(-7.499655298,2.678571429,-0.071905611));
#103019=CARTESIAN_POINT('Ctrl Pts',(-7.501830546,2.714073269,0.154969736));
#103020=CARTESIAN_POINT('Ctrl Pts',(-7.490287756,2.75,0.381561701));
#103021=CARTESIAN_POINT('Ctrl Pts',(-7.49007784496764,2.75065334439885,
0.385682381814436));
#103022=CARTESIAN_POINT('Ctrl Pts',(-7.48986793393528,2.7513066887977,0.389803062628871));
#103023=CARTESIAN_POINT('Ctrl Pts',(-7.247550363,2.620519775,-0.188450873));
#103024=CARTESIAN_POINT('Ctrl Pts',(-7.252188123,2.64969025,-0.010089297));
#103025=CARTESIAN_POINT('Ctrl Pts',(-7.248046656,2.678571429,0.168284491));
#103026=CARTESIAN_POINT('Ctrl Pts',(-7.242955809,2.714073269,0.387548315));
#103027=CARTESIAN_POINT('Ctrl Pts',(-7.224620308,2.75,0.606103459));
#103028=CARTESIAN_POINT('Ctrl Pts',(-7.22428686834254,2.75065334439885,
0.610077986467366));
#103029=CARTESIAN_POINT('Ctrl Pts',(-7.22395342868507,2.7513066887977,0.614052513934733));
#103030=CARTESIAN_POINT('Ctrl Pts',(-7.22462031736331,2.75000000207842,
0.606103462833411));
#103031=CARTESIAN_POINT('Ctrl Pts',(-7.23687442859809,2.72598918256373,
0.460037072307496));
#103032=CARTESIAN_POINT('Ctrl Pts',(-7.24466428685568,2.70215892418055,
0.313963824585473));
#103033=CARTESIAN_POINT('Ctrl Pts',(-7.24804665632304,2.67857142884258,
0.168284489740948));
#103034=CARTESIAN_POINT('Ctrl Pts',(-7.25076340467764,2.65962575351862,
0.0512736197741986));
#103035=CARTESIAN_POINT('Ctrl Pts',(-7.25065244802159,2.64052352961112,
-0.0661228385726127));
#103036=CARTESIAN_POINT('Ctrl Pts',(-7.24767235001763,2.62129679697412,
-0.183699490421209));
#103037=CARTESIAN_POINT('Ctrl Pts',(-7.44916206600001,2.75,0.871770907));
#103038=CARTESIAN_POINT('Ctrl Pts',(-7.401922517,2.68564607,1.275426333));
#103039=CARTESIAN_POINT('Ctrl Pts',(-7.311341072,2.620518779,1.671613511));
#103040=CARTESIAN_POINT('Ctrl Pts',(-7.224620308,2.75,0.606103459));
#103041=CARTESIAN_POINT('Ctrl Pts',(-7.19177675500001,2.68564607,0.997591409));
#103042=CARTESIAN_POINT('Ctrl Pts',(-7.116821813,2.620518779,1.383237971));
#103043=CARTESIAN_POINT('',(-7.11771573692104,2.62129679676499,1.37863061339408));
#103044=CARTESIAN_POINT('Origin',(0.190067036668271,2.55361154355146,-0.0482994856586152));
#103045=CARTESIAN_POINT('Ctrl Pts',(-7.36278006810718,2.66036061569806,
1.42810001883199));
#103046=CARTESIAN_POINT('Ctrl Pts',(-7.32190240929651,2.65417293168015,
1.41981262099689));
#103047=CARTESIAN_POINT('Ctrl Pts',(-7.28102001316054,2.64782918800092,
1.41154118785102));
#103048=CARTESIAN_POINT('Ctrl Pts',(-7.19934616913844,2.6348193285361,1.39505328929647));
#103049=CARTESIAN_POINT('Ctrl Pts',(-7.15850580107923,2.6281454276242,1.38682694622748));
#103050=CARTESIAN_POINT('Ctrl Pts',(-7.11771575851542,2.62129679728327,
1.37863061888986));
#103051=CARTESIAN_POINT('Ctrl Pts',(-7.40673988,2.620519775,1.17906927));
#103052=CARTESIAN_POINT('Ctrl Pts',(-7.37772309,2.64969025,1.361348485));
#103053=CARTESIAN_POINT('Ctrl Pts',(-7.339775105,2.678571429,1.541979703));
#103054=CARTESIAN_POINT('Ctrl Pts',(-7.293128004,2.714073269,1.764018444));
#103055=CARTESIAN_POINT('Ctrl Pts',(-7.233144504,2.75,1.982831457));
#103056=CARTESIAN_POINT('Ctrl Pts',(-7.23205367601043,2.75065334439885,
1.98681067393568));
#103057=CARTESIAN_POINT('Ctrl Pts',(-7.23096284802087,2.7513066887977,1.99078989087137));
#103058=CARTESIAN_POINT('Ctrl Pts',(-7.11861803000001,2.620519775,1.373964096));
#103059=CARTESIAN_POINT('Ctrl Pts',(-7.084804895,2.64969025,1.549152658));
#103060=CARTESIAN_POINT('Ctrl Pts',(-7.042415162,2.678571429,1.722465874));
#103061=CARTESIAN_POINT('Ctrl Pts',(-6.990308095,2.714073269,1.93550905));
#103062=CARTESIAN_POINT('Ctrl Pts',(-6.925418373,2.75,2.145012905));
#103063=CARTESIAN_POINT('Ctrl Pts',(-6.92423832306972,2.75065334439885,
2.14882283054546));
#103064=CARTESIAN_POINT('Ctrl Pts',(-6.92305827313945,2.7513066887977,2.15263275609092));
#103065=CARTESIAN_POINT('Ctrl Pts',(-6.92541838129421,2.75000000210847,
2.145012910917));
#103066=CARTESIAN_POINT('Ctrl Pts',(-6.96878595413734,2.72598918243438,
2.0049957425919));
#103067=CARTESIAN_POINT('Ctrl Pts',(-7.00779512022632,2.70215892404854,
1.86401219552958));
#103068=CARTESIAN_POINT('Ctrl Pts',(-7.04241516236796,2.6785714287493,1.72246587249559));
#103069=CARTESIAN_POINT('Ctrl Pts',(-7.07022227218096,2.65962575346698,
1.60877467199151));
#103070=CARTESIAN_POINT('Ctrl Pts',(-7.09535067827354,2.6405235297452,1.49409902583102));
#103071=CARTESIAN_POINT('Ctrl Pts',(-7.11771575821681,2.62129679697527,
1.37863061748385));
#103072=CARTESIAN_POINT('Ctrl Pts',(-7.087599821,2.75,2.452739036));
#103073=CARTESIAN_POINT('Ctrl Pts',(-6.954690722,2.68564607,2.836802116));
#103074=CARTESIAN_POINT('Ctrl Pts',(-6.781058488,2.620518779,3.204254325));
#103075=CARTESIAN_POINT('Ctrl Pts',(-6.925418373,2.75,2.145012905));
#103076=CARTESIAN_POINT('Ctrl Pts',(-6.809184347,2.68564607,2.520287691));
#103077=CARTESIAN_POINT('Ctrl Pts',(-6.653079198,2.620518779,2.880804954));
#103078=CARTESIAN_POINT('',(-6.654942668555,2.621296796722,2.87649748087442));
#103079=CARTESIAN_POINT('Origin',(0.17524062960169,2.55361151296453,-0.0880291569088504));
#103080=CARTESIAN_POINT('Ctrl Pts',(-6.8836430721632,2.66036061573128,2.9774919065786));
#103081=CARTESIAN_POINT('Ctrl Pts',(-6.84550265583457,2.65417293172294,
2.9606107751241));
#103082=CARTESIAN_POINT('Ctrl Pts',(-6.80735418082379,2.64782918801609,
2.94374421675597));
#103083=CARTESIAN_POINT('Ctrl Pts',(-6.73113415227105,2.63481931414431,
2.91008429684051));
#103084=CARTESIAN_POINT('Ctrl Pts',(-6.69301707486491,2.62814542054318,
2.89327082926511));
#103085=CARTESIAN_POINT('Ctrl Pts',(-6.65494268790158,2.62129679721243,
2.87649749143627));
#103086=CARTESIAN_POINT('Ctrl Pts',(-6.980109378,2.620519775,2.743733418));
#103087=CARTESIAN_POINT('Ctrl Pts',(-6.912586341,2.64969025,2.915513294));
#103088=CARTESIAN_POINT('Ctrl Pts',(-6.836695187,2.678571429,3.08376376));
#103089=CARTESIAN_POINT('Ctrl Pts',(-6.74340690300001,2.714073269,3.290583611));
#103090=CARTESIAN_POINT('Ctrl Pts',(-6.637787454,2.75,3.491386217));
#103091=CARTESIAN_POINT('Ctrl Pts',(-6.63586671494324,2.75065334439885,
3.49503790626459));
#103092=CARTESIAN_POINT('Ctrl Pts',(-6.63394597588646,2.7513066887977,3.49868959552918));
#103093=CARTESIAN_POINT('Ctrl Pts',(-6.65682703,2.620519775,2.872134031));
#103094=CARTESIAN_POINT('Ctrl Pts',(-6.586144065,2.64969025,3.035957957));
#103095=CARTESIAN_POINT('Ctrl Pts',(-6.507488162,2.678571429,3.196106666));
#103096=CARTESIAN_POINT('Ctrl Pts',(-6.41080134400001,2.714073269,3.392967532));
#103097=CARTESIAN_POINT('Ctrl Pts',(-6.302391571,2.75,3.583623931));
#103098=CARTESIAN_POINT('Ctrl Pts',(-6.30042008859683,2.75065334439885,
3.58709110674698));
#103099=CARTESIAN_POINT('Ctrl Pts',(-6.29844860619365,2.7513066887977,3.59055828249396));
#103100=CARTESIAN_POINT('Ctrl Pts',(-6.30239157792162,2.75000000206173,
3.58362393832676));
#103101=CARTESIAN_POINT('Ctrl Pts',(-6.37484479333945,2.72598918245582,
3.45620304037037));
#103102=CARTESIAN_POINT('Ctrl Pts',(-6.44324924246583,2.70215892407921,
3.32690142786726));
#103103=CARTESIAN_POINT('Ctrl Pts',(-6.50748816256116,2.67857142879395,
3.19610666485744));
#103104=CARTESIAN_POINT('Ctrl Pts',(-6.55908540503802,2.65962575352184,
3.09105120863447));
#103105=CARTESIAN_POINT('Ctrl Pts',(-6.6082781975179,2.64052352964498,2.9844584793457));
#103106=CARTESIAN_POINT('Ctrl Pts',(-6.654942688836,2.62129679689933,2.876497489609));
#103107=CARTESIAN_POINT('Ctrl Pts',(-6.39462928600001,2.75,3.919019814));
#103108=CARTESIAN_POINT('Ctrl Pts',(-6.182265318,2.68564607,4.265532185));
#103109=CARTESIAN_POINT('Ctrl Pts',(-5.933701147,2.620518779,4.587067767));
#103110=CARTESIAN_POINT('Ctrl Pts',(-6.302391571,2.75,3.583623931));
#103111=CARTESIAN_POINT('Ctrl Pts',(-6.108202046,2.68564607,3.925138122));
#103112=CARTESIAN_POINT('Ctrl Pts',(-5.878245994,2.620518779,4.243668699));
#103113=CARTESIAN_POINT('',(-5.88099187697605,2.62129679673668,4.23986252331473));
#103114=CARTESIAN_POINT('Origin',(0.152219762000134,2.55361156885222,-0.123642510782943));
#103115=CARTESIAN_POINT('Ctrl Pts',(-6.08263457681295,2.66036061569563,
4.38765958121683));
#103116=CARTESIAN_POINT('Ctrl Pts',(-6.04901480627198,2.6541729316607,4.36297405921584));
#103117=CARTESIAN_POINT('Ctrl Pts',(-6.01538403300628,2.64782918799544,
4.33830103740138));
#103118=CARTESIAN_POINT('Ctrl Pts',(-5.94818187354502,2.6348193140604,4.28904301441427));
#103119=CARTESIAN_POINT('Ctrl Pts',(-5.91457035089412,2.62814542052291,
4.26442859164504));
#103120=CARTESIAN_POINT('Ctrl Pts',(-5.88099189383972,2.6212967972618,4.23986253752156));
#103121=CARTESIAN_POINT('Ctrl Pts',(-6.227096719,2.620519775,4.180103641));
#103122=CARTESIAN_POINT('Ctrl Pts',(-6.124224737,2.64969025,4.333351942));
#103123=CARTESIAN_POINT('Ctrl Pts',(-6.013939,2.678571429,4.48135445));
#103124=CARTESIAN_POINT('Ctrl Pts',(-5.87837158900001,2.714073269,4.663284745));
#103125=CARTESIAN_POINT('Ctrl Pts',(-5.73205484,2.75,4.836687639));
#103126=CARTESIAN_POINT('Ctrl Pts',(-5.72939400151689,2.75065334439885,
4.83984105169261));
#103127=CARTESIAN_POINT('Ctrl Pts',(-5.72673316303378,2.7513066887977,4.84299446438521));
#103128=CARTESIAN_POINT('Ctrl Pts',(-5.88377019600001,2.620519775,4.23600617));
#103129=CARTESIAN_POINT('Ctrl Pts',(-5.779522458,2.64969025,4.380805236));
#103130=CARTESIAN_POINT('Ctrl Pts',(-5.668278248,2.678571429,4.520301063));
#103131=CARTESIAN_POINT('Ctrl Pts',(-5.531532647,2.714073269,4.69177462400001));
#103132=CARTESIAN_POINT('Ctrl Pts',(-5.384671945,2.75,4.854668686));
#103133=CARTESIAN_POINT('Ctrl Pts',(-5.38200121447729,2.75065334439885,
4.85763099066985));
#103134=CARTESIAN_POINT('Ctrl Pts',(-5.37933048395458,2.7513066887977,4.8605932953397));
#103135=CARTESIAN_POINT('Ctrl Pts',(-5.38467194950976,2.75000000185146,
4.85466869376947));
#103136=CARTESIAN_POINT('Ctrl Pts',(-5.48282297559008,2.72598918230731,
4.74580212529041));
#103137=CARTESIAN_POINT('Ctrl Pts',(-5.57742419140515,2.70215892400846,
4.63422844718347));
#103138=CARTESIAN_POINT('Ctrl Pts',(-5.66827824886269,2.67857142885437,
4.5203010622626));
#103139=CARTESIAN_POINT('Ctrl Pts',(-5.74125299381477,2.65962575370558,
4.42879362677771));
#103140=CARTESIAN_POINT('Ctrl Pts',(-5.81220997162734,2.64052352979421,
4.33526797231565));
#103141=CARTESIAN_POINT('Ctrl Pts',(-5.88099189479517,2.62129679697574,
4.23986253611313));
#103142=CARTESIAN_POINT('Ctrl Pts',(-5.40265299200001,2.75,5.202051581));
#103143=CARTESIAN_POINT('Ctrl Pts',(-5.120764059,2.68564607,5.49481071));
#103144=CARTESIAN_POINT('Ctrl Pts',(-4.808890534,2.620518779,5.75539502));
#103145=CARTESIAN_POINT('Ctrl Pts',(-5.384671945,2.75,4.854668686));
#103146=CARTESIAN_POINT('Ctrl Pts',(-5.121607007,2.68564607,5.14645345700001));
#103147=CARTESIAN_POINT('Ctrl Pts',(-4.828552541,2.620518779,5.408103212));
#103148=CARTESIAN_POINT('',(-4.83205244227338,2.62129679674723,5.40497630621078));
#103149=CARTESIAN_POINT('Origin',(0.122081501320788,2.55361158027122,-0.153474593694516));
#103150=CARTESIAN_POINT('Ctrl Pts',(-4.99720884880956,2.66036061571327,
5.59266517169272));
#103151=CARTESIAN_POINT('Ctrl Pts',(-4.96968174741625,2.65417293168221,
5.5613295265844));
#103152=CARTESIAN_POINT('Ctrl Pts',(-4.94214121319586,2.64782918798291,
5.53000372390746));
#103153=CARTESIAN_POINT('Ctrl Pts',(-4.88709922210057,2.63481931410792,
5.46745084842157));
#103154=CARTESIAN_POINT('Ctrl Pts',(-4.85956489132207,2.62814542052642,
5.43618641305384));
#103155=CARTESIAN_POINT('Ctrl Pts',(-4.83205245535895,2.62129679724376,
5.40497632383663));
#103156=CARTESIAN_POINT('Ctrl Pts',(-5.182911938,2.620519775,5.421016864));
#103157=CARTESIAN_POINT('Ctrl Pts',(-5.049501192,2.64969025,5.54856787));
#103158=CARTESIAN_POINT('Ctrl Pts',(-4.909977709,2.678571429,5.669401988));
#103159=CARTESIAN_POINT('Ctrl Pts',(-4.738470154,2.714073269,5.817935867));
#103160=CARTESIAN_POINT('Ctrl Pts',(-4.558297712,2.75,5.955830922));
#103161=CARTESIAN_POINT('Ctrl Pts',(-4.55502119191227,2.75065334439885,
5.95833860804061));
#103162=CARTESIAN_POINT('Ctrl Pts',(-4.55174467182455,2.7513066887977,5.96084629408121));
#103163=CARTESIAN_POINT('Ctrl Pts',(-4.83559480800001,2.620519775,5.401807369));
#103164=CARTESIAN_POINT('Ctrl Pts',(-4.702656805,2.64969025,5.520810931));
#103165=CARTESIAN_POINT('Ctrl Pts',(-4.564025943,2.678571429,5.633131207));
#103166=CARTESIAN_POINT('Ctrl Pts',(-4.393615631,2.714073269,5.771199548));
#103167=CARTESIAN_POINT('Ctrl Pts',(-4.215171043,2.75,5.89871452800001));
#103168=CARTESIAN_POINT('Ctrl Pts',(-4.21192594474503,2.75065334439885,
5.90103344752409));
#103169=CARTESIAN_POINT('Ctrl Pts',(-4.20868084649006,2.7513066887977,5.90335236704817));
#103170=CARTESIAN_POINT('Ctrl Pts',(-4.21517104541964,2.75000000186761,
5.89871453657559));
#103171=CARTESIAN_POINT('Ctrl Pts',(-4.33443044977284,2.72598918235011,
5.81349277726625));
#103172=CARTESIAN_POINT('Ctrl Pts',(-4.45080498379104,2.70215892405622,
5.72486409502537));
#103173=CARTESIAN_POINT('Ctrl Pts',(-4.56402594458306,2.67857142870357,
5.63313120586397));
#103174=CARTESIAN_POINT('Ctrl Pts',(-4.65496597508599,2.65962575335656,
5.55945057512922));
#103175=CARTESIAN_POINT('Ctrl Pts',(-4.74436926877494,2.64052352971437,
5.48336515216562));
#103176=CARTESIAN_POINT('Ctrl Pts',(-4.832052457168,2.62129679698418,5.4049763228133));
#103177=CARTESIAN_POINT('Ctrl Pts',(-4.158054649,2.75,6.241841198));
#103178=CARTESIAN_POINT('Ctrl Pts',(-3.819821564,2.68564607,6.467157993));
#103179=CARTESIAN_POINT('Ctrl Pts',(-3.459221545,2.620518779,6.654606397));
#103180=CARTESIAN_POINT('Ctrl Pts',(-4.215171043,2.75,5.898714528));
#103181=CARTESIAN_POINT('Ctrl Pts',(-3.895531316,2.68564607,6.127126348));
#103182=CARTESIAN_POINT('Ctrl Pts',(-3.553081338,2.620518779,6.31966083));
#103183=CARTESIAN_POINT('',(-3.55717160563945,2.62129679674548,6.31735940436044));
#103184=CARTESIAN_POINT('Origin',(0.0862346281103571,2.55361157933354,-0.176130081684605));
#103185=CARTESIAN_POINT('Ctrl Pts',(-3.67811918906671,2.66036061564738,
6.53616395320052));
#103186=CARTESIAN_POINT('Ctrl Pts',(-3.65797189341086,2.65417293161587,
6.49964340504796));
#103187=CARTESIAN_POINT('Ctrl Pts',(-3.63780936335807,2.64782918797976,
6.46312958192037));
#103188=CARTESIAN_POINT('Ctrl Pts',(-3.59750124233113,2.63481931400623,
6.39020675646657));
#103189=CARTESIAN_POINT('Ctrl Pts',(-3.5773315786538,2.628145420512,6.35375419959446));
#103190=CARTESIAN_POINT('Ctrl Pts',(-3.55717161500516,2.62129679727785,
6.31735942476804));
#103191=CARTESIAN_POINT('Ctrl Pts',(-3.896379956,2.620519775,6.408449363));
#103192=CARTESIAN_POINT('Ctrl Pts',(-3.738668582,2.64969025,6.50433893));
#103193=CARTESIAN_POINT('Ctrl Pts',(-3.576431317,2.678571429,6.592354589));
#103194=CARTESIAN_POINT('Ctrl Pts',(-3.37700312,2.714073269,6.700546775));
#103195=CARTESIAN_POINT('Ctrl Pts',(-3.17139965,2.75,6.79648617));
#103196=CARTESIAN_POINT('Ctrl Pts',(-3.16766065477918,2.75065334439885,
6.7982308727494));
#103197=CARTESIAN_POINT('Ctrl Pts',(-3.16392165955837,2.7513066887977,6.79997557549878));
#103198=CARTESIAN_POINT('Ctrl Pts',(-3.56131238,2.620519775,6.315026059));
#103199=CARTESIAN_POINT('Ctrl Pts',(-3.405900146,2.64969025,6.402669643));
#103200=CARTESIAN_POINT('Ctrl Pts',(-3.246364857,2.678571429,6.482562396));
#103201=CARTESIAN_POINT('Ctrl Pts',(-3.050258032,2.714073269,6.580769596));
#103202=CARTESIAN_POINT('Ctrl Pts',(-2.848573427,2.75,6.666943035));
#103203=CARTESIAN_POINT('Ctrl Pts',(-2.84490569817126,2.75065334439885,
6.66851013927399));
#103204=CARTESIAN_POINT('Ctrl Pts',(-2.84123796934252,2.7513066887977,6.67007724354796));
#103205=CARTESIAN_POINT('Ctrl Pts',(-2.84857342775376,2.75000000213149,
6.66694304521659));
#103206=CARTESIAN_POINT('Ctrl Pts',(-2.98336477202329,2.72598918264424,
6.6093509695434));
#103207=CARTESIAN_POINT('Ctrl Pts',(-3.11607108096161,2.70215892424239,
6.54781146106226));
#103208=CARTESIAN_POINT('Ctrl Pts',(-3.24636485877381,2.67857142870499,
6.48256239523189));
#103209=CARTESIAN_POINT('Ctrl Pts',(-3.35101792035801,2.65962575324877,
6.43015379474618));
#103210=CARTESIAN_POINT('Ctrl Pts',(-3.45468713136439,2.64052352963869,
6.37506627208961));
#103211=CARTESIAN_POINT('Ctrl Pts',(-3.5571716164275,2.62129679689988,6.31735942346803));
#103212=CARTESIAN_POINT('Ctrl Pts',(-2.719030292,2.75,6.989769257));
#103213=CARTESIAN_POINT('Ctrl Pts',(-2.340268458,2.68564607,7.137108156));
#103214=CARTESIAN_POINT('Ctrl Pts',(-1.947803201,2.620518779,7.242655776));
#103215=CARTESIAN_POINT('Ctrl Pts',(-2.848573427,2.75,6.666943035));
#103216=CARTESIAN_POINT('Ctrl Pts',(-2.48730491,2.68564607,6.82130162));
#103217=CARTESIAN_POINT('Ctrl Pts',(-2.111472,2.620518779,6.93571813100001));
#103218=CARTESIAN_POINT('',(-2.11596137812195,2.62129679672014,6.93434979846242));
#103219=CARTESIAN_POINT('Origin',(0.0463559295408789,2.55361154041299,-0.190550696625532));
#103220=CARTESIAN_POINT('Ctrl Pts',(-2.18704476419214,2.6603606156681,7.17403897349229));
#103221=CARTESIAN_POINT('Ctrl Pts',(-2.17521933937601,2.65417293164464,
7.13404118248025));
#103222=CARTESIAN_POINT('Ctrl Pts',(-2.16337759060393,2.64782918798867,
7.09404668415066));
#103223=CARTESIAN_POINT('Ctrl Pts',(-2.13968810290276,2.63481931408485,
7.01416369986587));
#103224=CARTESIAN_POINT('Ctrl Pts',(-2.12782621669689,2.62814542050594,
6.97422750164678));
#103225=CARTESIAN_POINT('Ctrl Pts',(-2.11596138231027,2.62129679721111,
6.93434982010131));
#103226=CARTESIAN_POINT('Ctrl Pts',(-2.427657577,2.620519775,7.096229893));
#103227=CARTESIAN_POINT('Ctrl Pts',(-2.253019985,2.64969025,7.155974331));
#103228=CARTESIAN_POINT('Ctrl Pts',(-2.075654973,2.678571429,7.207056017));
#103229=CARTESIAN_POINT('Ctrl Pts',(-1.857631174,2.714073269,7.269847562));
#103230=CARTESIAN_POINT('Ctrl Pts',(-1.636210464,2.75,7.319345279));
#103231=CARTESIAN_POINT('Ctrl Pts',(-1.63218382487528,2.75065334439885,
7.32024541812365));
#103232=CARTESIAN_POINT('Ctrl Pts',(-1.62815718575056,2.7513066887977,7.3211455572473));
#103233=CARTESIAN_POINT('Ctrl Pts',(-2.120506944,2.620519775,6.93296115));
#103234=CARTESIAN_POINT('Ctrl Pts',(-1.949887382,2.64969025,6.98514663800001));
#103235=CARTESIAN_POINT('Ctrl Pts',(-1.776907359,2.678571429,7.028876172));
#103236=CARTESIAN_POINT('Ctrl Pts',(-1.564273757,2.714073269,7.082630172));
#103237=CARTESIAN_POINT('Ctrl Pts',(-1.348779684,2.75,7.123432695));
#103238=CARTESIAN_POINT('Ctrl Pts',(-1.34486082353981,2.75065334439885,
7.12417470795578));
#103239=CARTESIAN_POINT('Ctrl Pts',(-1.34094196307961,2.7513066887977,7.12491672091157));
#103240=CARTESIAN_POINT('Ctrl Pts',(-1.34877968337738,2.750000001968,7.12343270485655));
#103241=CARTESIAN_POINT('Ctrl Pts',(-1.49280027486478,2.7259891824288,7.09616325474652));
#103242=CARTESIAN_POINT('Ctrl Pts',(-1.63563315914257,2.7021589240906,7.06459043961242));
#103243=CARTESIAN_POINT('Ctrl Pts',(-1.77690736049493,2.67857142875836,
7.02887617166257));
#103244=CARTESIAN_POINT('Ctrl Pts',(-1.89037999086808,2.65962575344708,
7.0001901698149));
#103245=CARTESIAN_POINT('Ctrl Pts',(-2.0034676622742,2.64052352984786,6.96867637909595));
#103246=CARTESIAN_POINT('Ctrl Pts',(-2.11596138470524,2.62129679691545,
6.93434981992751));
#103247=CARTESIAN_POINT('Ctrl Pts',(-1.1528671,2.75,7.41086347500001));
#103248=CARTESIAN_POINT('Ctrl Pts',(-0.751286999,2.68564607,7.473335074));
#103249=CARTESIAN_POINT('Ctrl Pts',(-0.345307744,2.620518779,7.49204662));
#103250=CARTESIAN_POINT('Ctrl Pts',(-1.348779684,2.75,7.123432695));
#103251=CARTESIAN_POINT('Ctrl Pts',(-0.962774892000001,2.68564607,7.196520411));
#103252=CARTESIAN_POINT('Ctrl Pts',(-0.571132578,2.620518779,7.227468961));
#103253=CARTESIAN_POINT('',(-0.575811147881845,2.62129679676424,7.22709770249865));
#103254=CARTESIAN_POINT('Origin',(0.00430938273576355,2.55361156966043,
-0.196060777350408));
#103255=CARTESIAN_POINT('Ctrl Pts',(-0.593706556239983,2.66036061570601,
7.47646390483063));
#103256=CARTESIAN_POINT('Ctrl Pts',(-0.59075594627258,2.65417293169975,
7.43485912324236));
#103257=CARTESIAN_POINT('Ctrl Pts',(-0.587788686063486,2.64782918801413,
7.39325404795638));
#103258=CARTESIAN_POINT('Ctrl Pts',(-0.581825532548915,2.63481932848156,
7.31014623567884));
#103259=CARTESIAN_POINT('Ctrl Pts',(-0.578826069372865,2.62814542760037,
7.26859371970006));
#103260=CARTESIAN_POINT('Ctrl Pts',(-0.575811147992927,2.62129679730516,
7.22709772493138));
#103261=CARTESIAN_POINT('Ctrl Pts',(-0.845420628,2.620519775,7.452198599));
#103262=CARTESIAN_POINT('Ctrl Pts',(-0.662022678,2.64969025,7.473004326));
#103263=CARTESIAN_POINT('Ctrl Pts',(-0.477823308,2.678571429,7.484763516));
#103264=CARTESIAN_POINT('Ctrl Pts',(-0.251398459,2.714073269,7.499218357));
#103265=CARTESIAN_POINT('Ctrl Pts',(-0.024513896,2.75,7.499959938));
#103266=CARTESIAN_POINT('Ctrl Pts',(-0.0203878941541442,2.75065334439885,
7.49997342399717));
#103267=CARTESIAN_POINT('Ctrl Pts',(-0.0162618923082885,2.7513066887977,
7.49998690999434));
#103268=CARTESIAN_POINT('Ctrl Pts',(-0.58054896,2.620519775,7.226718682));
#103269=CARTESIAN_POINT('Ctrl Pts',(-0.40270005,2.64969025,7.24100594));
#103270=CARTESIAN_POINT('Ctrl Pts',(-0.224363648,2.678571429,7.24652751));
#103271=CARTESIAN_POINT('Ctrl Pts',(-0.00514578,2.714073269,7.253314833));
#103272=CARTESIAN_POINT('Ctrl Pts',(0.214081497,2.75,7.24683856));
#103273=CARTESIAN_POINT('Ctrl Pts',(0.218068247520193,2.75065334439885,
7.24672078594786));
#103274=CARTESIAN_POINT('Ctrl Pts',(0.222054998040385,2.7513066887977,7.24660301189572));
#103275=CARTESIAN_POINT('Ctrl Pts',(0.214081503589313,2.75000000123159,
7.2468385607603));
#103276=CARTESIAN_POINT('Ctrl Pts',(0.0675659067429764,2.72598918224881,
7.25116683047458));
#103277=CARTESIAN_POINT('Ctrl Pts',(-0.0787148477332593,2.70215892417189,
7.25103702132724));
#103278=CARTESIAN_POINT('Ctrl Pts',(-0.224363649566028,2.67857142874639,
7.24652750995151));
#103279=CARTESIAN_POINT('Ctrl Pts',(-0.341349993970045,2.6596257535192,
7.24290543231094));
#103280=CARTESIAN_POINT('Ctrl Pts',(-0.458568273036239,2.64052352972813,
7.23643892294451));
#103281=CARTESIAN_POINT('Ctrl Pts',(-0.575811149698002,2.6212967970204,
7.2270977247663));
#103282=CARTESIAN_POINT('Ctrl Pts',(-1.353502885,3.268101717,7.122536763));
#103283=CARTESIAN_POINT('Ctrl Pts',(-0.967849888,3.203647866,7.19582279300001));
#103284=CARTESIAN_POINT('Ctrl Pts',(-0.576538529,3.138525418,7.227039735));
#103285=CARTESIAN_POINT('Ctrl Pts',(-1.64106351,3.268101717,7.318258711));
#103286=CARTESIAN_POINT('Ctrl Pts',(-1.244813059,3.203647866,7.407114842));
#103287=CARTESIAN_POINT('Ctrl Pts',(-0.841285031,3.138525418,7.452666603));
#103288=CARTESIAN_POINT('',(-1.34892078812789,3.26733592570993,7.12340597604384));
#103289=CARTESIAN_POINT('Origin',(0.00747049262276644,3.08931098836207,
-0.196900007873446));
#103290=CARTESIAN_POINT('Ctrl Pts',(-1.39671106560661,3.22840426963636,
7.3687989657909));
#103291=CARTESIAN_POINT('Ctrl Pts',(-1.38863728046114,3.23458082925561,
7.32788102997847));
#103292=CARTESIAN_POINT('Ctrl Pts',(-1.38061063134402,3.24090849484843,
7.28695168322483));
#103293=CARTESIAN_POINT('Ctrl Pts',(-1.36468010339121,3.25387487492678,
7.20516874180313));
#103294=CARTESIAN_POINT('Ctrl Pts',(-1.35676670818485,3.26052132406272,
7.16426632904137));
#103295=CARTESIAN_POINT('Ctrl Pts',(-1.34892078979801,3.26733592512212,
7.12340597672159));
#103296=CARTESIAN_POINT('Ctrl Pts',(-2.116659292,3.138525418,6.93413682));
#103297=CARTESIAN_POINT('Ctrl Pts',(-1.894237241,3.176642188,7.002031601));
#103298=CARTESIAN_POINT('Ctrl Pts',(-1.667921256,3.214285714,7.055532488));
#103299=CARTESIAN_POINT('Ctrl Pts',(-1.506869744,3.241073689,7.093604914));
#103300=CARTESIAN_POINT('Ctrl Pts',(-1.344248775,3.268112745,7.124289104));
#103301=CARTESIAN_POINT('Ctrl Pts',(-1.953220126,3.138525418,7.241196803));
#103302=CARTESIAN_POINT('Ctrl Pts',(-1.720948701,3.176642188,7.30384904599999));
#103303=CARTESIAN_POINT('Ctrl Pts',(-1.485139566,3.214285714,7.351486956));
#103304=CARTESIAN_POINT('Ctrl Pts',(-1.317332516,3.241073689,7.385387158));
#103305=CARTESIAN_POINT('Ctrl Pts',(-1.148153419,3.268112745,7.411595221));
#103306=CARTESIAN_POINT('Ctrl Pts',(-2.11665928286731,3.13852541956508,
6.93413682278777));
#103307=CARTESIAN_POINT('Ctrl Pts',(-1.96799497161502,3.16400222517069,
6.97951690431297));
#103308=CARTESIAN_POINT('Ctrl Pts',(-1.81825525112624,3.18928040270946,
7.01999367228996));
#103309=CARTESIAN_POINT('Ctrl Pts',(-1.66792125646245,3.21428571392205,
7.05553248789925));
#103310=CARTESIAN_POINT('Ctrl Pts',(-1.56236435696929,3.23184317457392,
7.08048603968294));
#103311=CARTESIAN_POINT('Ctrl Pts',(-1.45597993658122,3.24953506289061,
7.10313276635206));
#103312=CARTESIAN_POINT('Ctrl Pts',(-1.34892078643843,3.26733592560455,
7.12340597794321));
#103313=CARTESIAN_POINT('Ctrl Pts',(-2.852993603,3.268101717,6.665052701));
#103314=CARTESIAN_POINT('Ctrl Pts',(-2.492111289,3.203647866,6.819529339));
#103315=CARTESIAN_POINT('Ctrl Pts',(-2.116659292,3.138525418,6.93413682));
#103316=CARTESIAN_POINT('Ctrl Pts',(-3.175905654,3.268101717,6.794381744));
#103317=CARTESIAN_POINT('Ctrl Pts',(-2.808020759,3.203647866,6.966342602));
#103318=CARTESIAN_POINT('Ctrl Pts',(-2.423719275,3.138525418,7.097575986));
#103319=CARTESIAN_POINT('',(-2.84870549026513,3.26733592567,6.66688660531189));
#103320=CARTESIAN_POINT('Origin',(0.0496234282582414,3.08931098430521,-0.190690422862081));
#103321=CARTESIAN_POINT('Ctrl Pts',(-2.94813069419871,3.22840426962259,
6.89626894829274));
#103322=CARTESIAN_POINT('Ctrl Pts',(-2.93144952302421,3.23458082924873,
6.85804327623306));
#103323=CARTESIAN_POINT('Ctrl Pts',(-2.91481193279318,3.24090849487191,
6.81979632704499));
#103324=CARTESIAN_POINT('Ctrl Pts',(-2.88167293465831,3.25387487579441,
6.74335001312293));
#103325=CARTESIAN_POINT('Ctrl Pts',(-2.86515174144485,3.26052132458631,
6.70510502432325));
#103326=CARTESIAN_POINT('Ctrl Pts',(-2.84870548936965,3.26733592513142,
6.66688660775784));
#103327=CARTESIAN_POINT('Ctrl Pts',(-3.557807419,3.138525418,6.31700137500001));
#103328=CARTESIAN_POINT('Ctrl Pts',(-3.355180843,3.176642188,6.43112298));
#103329=CARTESIAN_POINT('Ctrl Pts',(-3.145657109,3.214285714,6.532024292));
#103330=CARTESIAN_POINT('Ctrl Pts',(-2.996555338,3.241073689,6.603827921));
#103331=CARTESIAN_POINT('Ctrl Pts',(-2.84433255,3.268112745,6.668753433));
#103332=CARTESIAN_POINT('Ctrl Pts',(-3.46419819,3.138525418,6.652017055));
#103333=CARTESIAN_POINT('Ctrl Pts',(-3.250825521,3.176642188,6.763136014));
#103334=CARTESIAN_POINT('Ctrl Pts',(-3.030770215,3.214285714,6.86035217));
#103335=CARTESIAN_POINT('Ctrl Pts',(-2.874173942,3.241073689,6.929533359));
#103336=CARTESIAN_POINT('Ctrl Pts',(-2.714584117,3.268112745,6.991497198));
#103337=CARTESIAN_POINT('Ctrl Pts',(-3.55780740986131,3.13852541971911,
6.31700138014702));
#103338=CARTESIAN_POINT('Ctrl Pts',(-3.42237416380755,3.16400222531233,
6.39327893298748));
#103339=CARTESIAN_POINT('Ctrl Pts',(-3.28483658365421,3.18928040279562,
6.4649989898295));
#103340=CARTESIAN_POINT('Ctrl Pts',(-3.14565710871316,3.21428571404078,
6.53202429228031));
#103341=CARTESIAN_POINT('Ctrl Pts',(-3.04793235033307,3.23184317406293,
6.57908605590825));
#103342=CARTESIAN_POINT('Ctrl Pts',(-2.94890351649419,3.24953506217978,
6.62407281963628));
#103343=CARTESIAN_POINT('Ctrl Pts',(-2.84870549087026,3.26733592486962,
6.66688660706085));
#103344=CARTESIAN_POINT('Ctrl Pts',(-4.219081511,3.268101717,5.895918181));
#103345=CARTESIAN_POINT('Ctrl Pts',(-3.899844336,3.203647866,6.12436227200001));
#103346=CARTESIAN_POINT('Ctrl Pts',(-3.557807419,3.138525418,6.317001375));
#103347=CARTESIAN_POINT('Ctrl Pts',(-4.562245979,3.268101717,5.952807038));
#103348=CARTESIAN_POINT('Ctrl Pts',(-4.23992853,3.203647866,6.199831924));
#103349=CARTESIAN_POINT('Ctrl Pts',(-3.892823099,3.138525418,6.410610604));
#103350=CARTESIAN_POINT('',(-4.21528788507473,3.26733592572405,5.89863103008845));
#103351=CARTESIAN_POINT('Origin',(0.0894560049937093,3.08931096832741,-0.175564515937652));
#103352=CARTESIAN_POINT('Ctrl Pts',(-4.3616990090963,3.22840426965525,6.10127705919986));
#103353=CARTESIAN_POINT('Ctrl Pts',(-4.3371904445687,3.23458082933408,6.06753104051369));
#103354=CARTESIAN_POINT('Ctrl Pts',(-4.31271986853268,3.24090849489276,
6.03375487412336));
#103355=CARTESIAN_POINT('Ctrl Pts',(-4.26392214546335,3.2538748222234,5.96622001644638));
#103356=CARTESIAN_POINT('Ctrl Pts',(-4.23956555893764,3.26052129816919,
5.93242059420358));
#103357=CARTESIAN_POINT('Ctrl Pts',(-4.21528788745792,3.26733592508906,
5.89863103001385));
#103358=CARTESIAN_POINT('Ctrl Pts',(-4.832596425,3.138525418,5.404489966));
#103359=CARTESIAN_POINT('Ctrl Pts',(-4.659239917,3.176642188,5.559502196));
#103360=CARTESIAN_POINT('Ctrl Pts',(-4.476305531,3.214285714,5.703085901));
#103361=CARTESIAN_POINT('Ctrl Pts',(-4.346125334,3.241073689,5.805263274));
#103362=CARTESIAN_POINT('Ctrl Pts',(-4.211418497,3.268112745,5.901394263));
#103363=CARTESIAN_POINT('Ctrl Pts',(-4.813194196,3.138525418,5.751796383));
#103364=CARTESIAN_POINT('Ctrl Pts',(-4.628697353,3.176642188,5.906186259));
#103365=CARTESIAN_POINT('Ctrl Pts',(-4.434685418,3.214285714,6.048434942));
#103366=CARTESIAN_POINT('Ctrl Pts',(-4.29662219,3.241073689,6.149662283));
#103367=CARTESIAN_POINT('Ctrl Pts',(-4.15408388,3.268112745,6.244484536));
#103368=CARTESIAN_POINT('Ctrl Pts',(-4.83259641748162,3.13852541965311,
5.4044899727228));
#103369=CARTESIAN_POINT('Ctrl Pts',(-4.71672694397057,3.1640022253197,5.50809834390426));
#103370=CARTESIAN_POINT('Ctrl Pts',(-4.59782260794536,3.1892804028295,5.60770814008636));
#103371=CARTESIAN_POINT('Ctrl Pts',(-4.47630553135839,3.21428571392579,
5.70308590073554));
#103372=CARTESIAN_POINT('Ctrl Pts',(-4.39098240876368,3.23184317448963,
5.77005532255571));
#103373=CARTESIAN_POINT('Ctrl Pts',(-4.30393963736397,3.24953506284712,
5.83527859361555));
#103374=CARTESIAN_POINT('Ctrl Pts',(-4.21528788457339,3.26733592566267,
5.89863103222262));
#103375=CARTESIAN_POINT('Ctrl Pts',(-5.387889857,3.268101717,4.851097081));
#103376=CARTESIAN_POINT('Ctrl Pts',(-5.125224996,3.203647866,5.142826832));
#103377=CARTESIAN_POINT('Ctrl Pts',(-4.83259642500001,3.138525418,5.404489966));
#103378=CARTESIAN_POINT('Ctrl Pts',(-5.735260753,3.268101717,4.832885691));
#103379=CARTESIAN_POINT('Ctrl Pts',(-5.47358195600001,3.203647866,5.143423997));
#103380=CARTESIAN_POINT('Ctrl Pts',(-5.179902842,3.138525418,5.423892195));
#103381=CARTESIAN_POINT('',(-5.38476810601465,3.26733592571324,4.85456202254636));
#103382=CARTESIAN_POINT('Origin',(0.125105784914014,3.08931094753363,-0.152229559399517));
#103383=CARTESIAN_POINT('Ctrl Pts',(-5.57131912513468,3.22840426958941,
5.02099623658913));
#103384=CARTESIAN_POINT('Ctrl Pts',(-5.54012916105509,3.2345808292255,4.99330779814539));
#103385=CARTESIAN_POINT('Ctrl Pts',(-5.50896981606804,3.24090849483476,
4.96558175001598));
#103386=CARTESIAN_POINT('Ctrl Pts',(-5.44679470544814,3.25387487499183,
4.9101156618356));
#103387=CARTESIAN_POINT('Ctrl Pts',(-5.41574182084466,3.26052132410651,
4.88234251745498));
#103388=CARTESIAN_POINT('Ctrl Pts',(-5.38476810759784,3.26733592515923,
4.85456202178235));
#103389=CARTESIAN_POINT('Ctrl Pts',(-5.881418593,3.138525418,4.239270613));
#103390=CARTESIAN_POINT('Ctrl Pts',(-5.745438112,3.176642188,4.427925268));
#103391=CARTESIAN_POINT('Ctrl Pts',(-5.597646882,3.214285714,4.607477551));
#103392=CARTESIAN_POINT('Ctrl Pts',(-5.492475341,3.241073689,4.73525096800001));
#103393=CARTESIAN_POINT('Ctrl Pts',(-5.381583195,3.268112745,4.858092456));
#103394=CARTESIAN_POINT('Ctrl Pts',(-5.937130591,3.138525418,4.582628105));
#103395=CARTESIAN_POINT('Ctrl Pts',(-5.790136441,3.176642188,4.773069799));
#103396=CARTESIAN_POINT('Ctrl Pts',(-5.631239659,3.214285714,4.953699618));
#103397=CARTESIAN_POINT('Ctrl Pts',(-5.518165158,3.241073689,5.082239832));
#103398=CARTESIAN_POINT('Ctrl Pts',(-5.399343297,3.268112745,5.20548671700001));
#103399=CARTESIAN_POINT('Ctrl Pts',(-5.88141858688418,3.13852541971433,
4.23927062148488));
#103400=CARTESIAN_POINT('Ctrl Pts',(-5.79053081512884,3.16400222534549,
4.36536519804455));
#103401=CARTESIAN_POINT('Ctrl Pts',(-5.69581955833051,3.18928040283087,
4.48820708978384));
#103402=CARTESIAN_POINT('Ctrl Pts',(-5.59764688247275,3.21428571388678,
4.60747755075093));
#103403=CARTESIAN_POINT('Ctrl Pts',(-5.52871501357167,3.23184317443036,
4.69122321399006));
#103404=CARTESIAN_POINT('Ctrl Pts',(-5.45772832847149,3.24953506289523,
4.77363322429347));
#103405=CARTESIAN_POINT('Ctrl Pts',(-5.38476810582414,3.26733592560558,
4.85456202488883));
#103406=CARTESIAN_POINT('Ctrl Pts',(-6.304766461,3.268101717,3.579444073));
#103407=CARTESIAN_POINT('Ctrl Pts',(-6.110955831,3.203647866,3.920818525));
#103408=CARTESIAN_POINT('Ctrl Pts',(-5.881418593,3.138525418,4.239270613));
#103409=CARTESIAN_POINT('Ctrl Pts',(-6.640101108,3.268101717,3.48698398));
#103410=CARTESIAN_POINT('Ctrl Pts',(-6.45129677200001,3.203647866,3.846515279));
#103411=CARTESIAN_POINT('Ctrl Pts',(-6.224776085,3.138525418,4.183558616));
#103412=CARTESIAN_POINT('',(-6.30246255512824,3.26733592574253,3.58349909006738));
#103413=CARTESIAN_POINT('Origin',(0.154905874552772,3.08931093362247,-0.121776565780059));
#103414=CARTESIAN_POINT('Ctrl Pts',(-6.52043055152078,3.22840426961869,
3.70593920925317));
#103415=CARTESIAN_POINT('Ctrl Pts',(-6.4840175953753,3.23458082929635,3.68560303135103));
#103416=CARTESIAN_POINT('Ctrl Pts',(-6.44762645791188,3.24090849487083,
3.66522354115463));
#103417=CARTESIAN_POINT('Ctrl Pts',(-6.37498139769519,3.25387487497803,
3.62442003059789));
#103418=CARTESIAN_POINT('Ctrl Pts',(-6.3386841072753,3.2605213240895,3.60397165931456));
#103419=CARTESIAN_POINT('Ctrl Pts',(-6.30246255720574,3.26733592512396,
3.58349908911351));
#103420=CARTESIAN_POINT('Ctrl Pts',(-6.655232165,3.138525418,2.875827678));
#103421=CARTESIAN_POINT('Ctrl Pts',(-6.562986005,3.176642188,3.089303476));
#103422=CARTESIAN_POINT('Ctrl Pts',(-6.457248486,3.214285714,3.296428672));
#103423=CARTESIAN_POINT('Ctrl Pts',(-6.382003305,3.241073689,3.44382359));
#103424=CARTESIAN_POINT('Ctrl Pts',(-6.30011104500001,3.268112745,3.587631646));
#103425=CARTESIAN_POINT('Ctrl Pts',(-6.783453358,3.138525418,3.19918123));
#103426=CARTESIAN_POINT('Ctrl Pts',(-6.680835185,3.176642188,3.4167699));
#103427=CARTESIAN_POINT('Ctrl Pts',(-6.564483393,3.214285714,3.627334805));
#103428=CARTESIAN_POINT('Ctrl Pts',(-6.481684858,3.241073689,3.777177496));
#103429=CARTESIAN_POINT('Ctrl Pts',(-6.392135422,3.268112745,3.923086125));
#103430=CARTESIAN_POINT('Ctrl Pts',(-6.65523216073996,3.13852541976028,
2.87582768785858));
#103431=CARTESIAN_POINT('Ctrl Pts',(-6.59357590057777,3.16400222528848,
3.01851242710704));
#103432=CARTESIAN_POINT('Ctrl Pts',(-6.52748631577757,3.18928040276481,
3.15884246419534));
#103433=CARTESIAN_POINT('Ctrl Pts',(-6.45724848623745,3.21428571391547,
3.29642867153488));
#103434=CARTESIAN_POINT('Ctrl Pts',(-6.40793104801386,3.23184317453693,
3.39303472214997));
#103435=CARTESIAN_POINT('Ctrl Pts',(-6.35631970871314,3.24953506296906,
3.48877807130775));
#103436=CARTESIAN_POINT('Ctrl Pts',(-6.30246255541806,3.26733592572747,
3.583499092464));
#103437=CARTESIAN_POINT('Ctrl Pts',(-6.926839193,3.268101717,2.140420238));
#103438=CARTESIAN_POINT('Ctrl Pts',(-6.810945164,3.203647866,2.515477101));
#103439=CARTESIAN_POINT('Ctrl Pts',(-6.655232165,3.138525418,2.875827678));
#103440=CARTESIAN_POINT('Ctrl Pts',(-7.234457715,3.268101717,1.978034774));
#103441=CARTESIAN_POINT('Ctrl Pts',(-7.127356121,3.203647866,2.369747783));
#103442=CARTESIAN_POINT('Ctrl Pts',(-6.978585717,3.138525418,2.747606485));
#103443=CARTESIAN_POINT('',(-6.92546085991525,3.26733592573375,2.14487572253998));
#103444=CARTESIAN_POINT('Origin',(0.177462766279987,3.08931095639599,-0.0856293580043394));
#103445=CARTESIAN_POINT('Ctrl Pts',(-7.16465389175981,3.22840426965055,
2.21759658398079));
#103446=CARTESIAN_POINT('Ctrl Pts',(-7.12472057319778,3.23458082930576,
2.20556356384048));
#103447=CARTESIAN_POINT('Ctrl Pts',(-7.08479925237754,3.24090849485858,
2.19348355363704));
#103448=CARTESIAN_POINT('Ctrl Pts',(-7.0050810446984,3.25387487495275,2.16925054701254));
#103449=CARTESIAN_POINT('Ctrl Pts',(-6.96523656935363,3.26052132407379,
2.15708309174497));
#103450=CARTESIAN_POINT('Ctrl Pts',(-6.92546086156653,3.26733592512786,
2.14487572139872));
#103451=CARTESIAN_POINT('Ctrl Pts',(-7.117854477,3.138525418,1.377914237));
#103452=CARTESIAN_POINT('Ctrl Pts',(-7.073655968,3.176642188,1.606229286));
#103453=CARTESIAN_POINT('Ctrl Pts',(-7.014916327,3.214285714,1.831242452));
#103454=CARTESIAN_POINT('Ctrl Pts',(-6.973115887,3.241073689,1.991366848));
#103455=CARTESIAN_POINT('Ctrl Pts',(-6.92405270400001,3.268112745,2.149417167));
#103456=CARTESIAN_POINT('Ctrl Pts',(-7.312589385,3.138525418,1.666144196));
#103457=CARTESIAN_POINT('Ctrl Pts',(-7.2591455,3.176642188,1.900705638));
#103458=CARTESIAN_POINT('Ctrl Pts',(-7.190779179,3.214285714,2.131359848));
#103459=CARTESIAN_POINT('Ctrl Pts',(-7.142128177,3.241073689,2.295498538));
#103460=CARTESIAN_POINT('Ctrl Pts',(-7.086038399,3.268112745,2.457246386));
#103461=CARTESIAN_POINT('Ctrl Pts',(-7.11785447504281,3.13852541968788,
1.3779142471102));
#103462=CARTESIAN_POINT('Ctrl Pts',(-7.08831270552661,3.16400222537653,
1.53051737006383));
#103463=CARTESIAN_POINT('Ctrl Pts',(-7.05393506819967,3.18928040286292,
1.68177387602203));
#103464=CARTESIAN_POINT('Ctrl Pts',(-7.01491632751934,3.21428571383937,
1.83124245149837));
#103465=CARTESIAN_POINT('Ctrl Pts',(-6.98751934921584,3.23184317436136,
1.93619169720647));
#103466=CARTESIAN_POINT('Ctrl Pts',(-6.95769664389279,3.24953506294541,
2.04079153279387));
#103467=CARTESIAN_POINT('Ctrl Pts',(-6.92546086076598,3.26733592567063,
2.14487572491838));
#103468=CARTESIAN_POINT('Ctrl Pts',(-7.225020623,3.268101717,0.601312732));
#103469=CARTESIAN_POINT('Ctrl Pts',(-7.192462271,3.203647866,0.992514764));
#103470=CARTESIAN_POINT('Ctrl Pts',(-7.117854477,3.138525418,1.377914237));
#103471=CARTESIAN_POINT('Ctrl Pts',(-7.49053912000001,3.268101717,0.376594861));
#103472=CARTESIAN_POINT('Ctrl Pts',(-7.47014822,3.203647866,0.782173513));
#103473=CARTESIAN_POINT('Ctrl Pts',(-7.406084436,3.138525418,1.183179329));
#103474=CARTESIAN_POINT('',(-7.22463231197984,3.26733592574723,0.605960350813484));
#103475=CARTESIAN_POINT('Origin',(0.191721488831114,3.08931097958864,-0.0454781312283063));
#103476=CARTESIAN_POINT('Ctrl Pts',(-7.47386597901678,3.22840426959478,
0.625561607462148));
#103477=CARTESIAN_POINT('Ctrl Pts',(-7.43227953574014,3.23458082926715,
0.622394395629625));
#103478=CARTESIAN_POINT('Ctrl Pts',(-7.39069470803807,3.24090849486445,
0.619178713171061));
#103479=CARTESIAN_POINT('Ctrl Pts',(-7.30763088765172,3.25387487500532,
0.612649318894864));
#103480=CARTESIAN_POINT('Ctrl Pts',(-7.26610231080442,3.26052132413581,
0.609331716384318));
#103481=CARTESIAN_POINT('Ctrl Pts',(-7.22463231304457,3.2673359252016,0.605960349082846));
#103482=CARTESIAN_POINT('Ctrl Pts',(-7.247653825,3.138525418,-0.184428943));
#103483=CARTESIAN_POINT('Ctrl Pts',(-7.25356963899999,3.176642188,0.048049601));
#103484=CARTESIAN_POINT('Ctrl Pts',(-7.244574478,3.214285714,0.28042937));
#103485=CARTESIAN_POINT('Ctrl Pts',(-7.238173321,3.241073689,0.445796006));
#103486=CARTESIAN_POINT('Ctrl Pts',(-7.224233354,3.268112745,0.61069833));
#103487=CARTESIAN_POINT('Ctrl Pts',(-7.49979686,3.138525418,0.055200111));
#103488=CARTESIAN_POINT('Ctrl Pts',(-7.49802624,3.176642188,0.295766492));
#103489=CARTESIAN_POINT('Ctrl Pts',(-7.480842122,3.214285714,0.535724874));
#103490=CARTESIAN_POINT('Ctrl Pts',(-7.46861352000001,3.241073689,0.706484620000001));
#103491=CARTESIAN_POINT('Ctrl Pts',(-7.448606097,3.268112745,0.876508537));
#103492=CARTESIAN_POINT('Ctrl Pts',(-7.24765382527071,3.13852541974422,
-0.184428932361817));
#103493=CARTESIAN_POINT('Ctrl Pts',(-7.25160788627811,3.16400222524267,
-0.0290429788910136));
#103494=CARTESIAN_POINT('Ctrl Pts',(-7.25054965684747,3.18928040272498,
0.126067409913584));
#103495=CARTESIAN_POINT('Ctrl Pts',(-7.24457447826883,3.21428571386402,
0.28042936941594));
#103496=CARTESIAN_POINT('Ctrl Pts',(-7.24037901156516,3.23184317446808,
0.38881450124409));
#103497=CARTESIAN_POINT('Ctrl Pts',(-7.23373941729894,3.24953506294951,
0.497379850505409));
#103498=CARTESIAN_POINT('Ctrl Pts',(-7.2246323132945,3.26733592571272,0.605960352805634));
#103499=CARTESIAN_POINT('Ctrl Pts',(-7.18536811800001,3.268101717,-0.96591149));
#103500=CARTESIAN_POINT('Ctrl Pts',(-7.237667836,3.203647866,-0.57685646));
#103501=CARTESIAN_POINT('Ctrl Pts',(-7.247653825,3.138525418,-0.184428943));
#103502=CARTESIAN_POINT('Ctrl Pts',(-7.396371241,3.268101717,-1.24245421));
#103503=CARTESIAN_POINT('Ctrl Pts',(-7.46364449,3.203647866,-0.84197432));
#103504=CARTESIAN_POINT('Ctrl Pts',(-7.487282879,3.138525418,-0.436571978));
#103505=CARTESIAN_POINT('',(-7.18598798619975,3.26733592573614,-0.961289054106258));
#103506=CARTESIAN_POINT('Origin',(0.197015451307481,3.08931093639002,-0.00320043798352432));
#103507=CARTESIAN_POINT('Ctrl Pts',(-7.43360839986677,3.22840426960252,
-0.995723935096498));
#103508=CARTESIAN_POINT('Ctrl Pts',(-7.39231336740992,3.23458082928339,
-0.989877243158041));
#103509=CARTESIAN_POINT('Ctrl Pts',(-7.35100949329422,3.24090849484591,
-0.984078236009551));
#103510=CARTESIAN_POINT('Ctrl Pts',(-7.26848403180813,3.25387487499032,
-0.972598710641352));
#103511=CARTESIAN_POINT('Ctrl Pts',(-7.22721318341613,3.26052132411662,
-0.966911333061405));
#103512=CARTESIAN_POINT('Ctrl Pts',(-7.18598798673272,3.26733592517209,
-0.961289056132491));
#103513=CARTESIAN_POINT('Ctrl Pts',(-7.038560935,3.138525418,-1.73814843));
#103514=CARTESIAN_POINT('Ctrl Pts',(-7.094314455,3.176642188,-1.51237683));
#103515=CARTESIAN_POINT('Ctrl Pts',(-7.135484378,3.214285714,-1.283496277));
#103516=CARTESIAN_POINT('Ctrl Pts',(-7.164781814,3.241073689,-1.120619762));
#103517=CARTESIAN_POINT('Ctrl Pts',(-7.18661688100001,3.268112745,-0.956576082));
#103518=CARTESIAN_POINT('Ctrl Pts',(-7.33632217,3.138525418,-1.558325069));
#103519=CARTESIAN_POINT('Ctrl Pts',(-7.386307607,3.176642188,-1.323002365));
#103520=CARTESIAN_POINT('Ctrl Pts',(-7.421109203,3.214285714,-1.08496));
#103521=CARTESIAN_POINT('Ctrl Pts',(-7.445874796,3.241073689,-0.915563734));
#103522=CARTESIAN_POINT('Ctrl Pts',(-7.462885252,3.268112745,-0.745213877));
#103523=CARTESIAN_POINT('Ctrl Pts',(-7.03856093736968,3.13852541962007,
-1.73814842040409));
#103524=CARTESIAN_POINT('Ctrl Pts',(-7.07582594128906,3.16400222522755,
-1.58724530956614));
#103525=CARTESIAN_POINT('Ctrl Pts',(-7.10813660163031,3.18928040274743,
-1.43553382686493));
#103526=CARTESIAN_POINT('Ctrl Pts',(-7.13548437796271,3.21428571388022,
-1.28349627766317));
#103527=CARTESIAN_POINT('Ctrl Pts',(-7.15468659746866,3.23184317448197,
-1.17674322920128));
#103528=CARTESIAN_POINT('Ctrl Pts',(-7.17154057430262,3.24953506288593,
-1.06928876128343));
#103529=CARTESIAN_POINT('Ctrl Pts',(-7.18598798786616,3.26733592567761,
-0.961289052512922));
#103530=CARTESIAN_POINT('Ctrl Pts',(-6.80973578600001,3.268101717,-2.487970763));
#103531=CARTESIAN_POINT('Ctrl Pts',(-6.944448097,3.203647866,-2.119254517));
#103532=CARTESIAN_POINT('Ctrl Pts',(-7.038560935,3.138525418,-1.73814843));
#103533=CARTESIAN_POINT('Ctrl Pts',(-6.956357263,3.268101717,-2.803407502));
#103534=CARTESIAN_POINT('Ctrl Pts',(-7.108149039,3.203647866,-2.42675237));
#103535=CARTESIAN_POINT('Ctrl Pts',(-7.218384296,3.138525418,-2.035909664));
#103536=CARTESIAN_POINT('',(-6.81133484954207,3.26733592570866,-2.48358965115484));
#103537=CARTESIAN_POINT('Origin',(0.193097258795751,3.08931093160372,0.0392268551923727));
#103538=CARTESIAN_POINT('Ctrl Pts',(-7.04576355357133,3.22840426963018,
-2.5704505328325));
#103539=CARTESIAN_POINT('Ctrl Pts',(-7.00669084204283,3.23458082930848,
-2.55586332204927));
#103540=CARTESIAN_POINT('Ctrl Pts',(-6.96759924474046,3.24090849486114,
-2.54132078042704));
#103541=CARTESIAN_POINT('Ctrl Pts',(-6.88947094156835,3.25387487495917,
-2.51236910518395));
#103542=CARTESIAN_POINT('Ctrl Pts',(-6.85038760072907,3.26052132408289,
-2.49794268283183));
#103543=CARTESIAN_POINT('Ctrl Pts',(-6.81133484970225,3.26733592511703,
-2.48358965305668));
#103544=CARTESIAN_POINT('Ctrl Pts',(-6.50035275900001,3.138525418,-3.210594028));
#103545=CARTESIAN_POINT('Ctrl Pts',(-6.60333701300001,3.176642188,-3.002086202));
#103546=CARTESIAN_POINT('Ctrl Pts',(-6.692746959,3.214285714,-2.787407065));
#103547=CARTESIAN_POINT('Ctrl Pts',(-6.756373074,3.241073689,-2.634636595));
#103548=CARTESIAN_POINT('Ctrl Pts',(-6.812962191,3.268112745,-2.479122059));
#103549=CARTESIAN_POINT('Ctrl Pts',(-6.829809208,3.138525418,-3.098984701));
#103550=CARTESIAN_POINT('Ctrl Pts',(-6.929213439,3.176642188,-2.879909103));
#103551=CARTESIAN_POINT('Ctrl Pts',(-7.014373465,3.214285714,-2.65491335));
#103552=CARTESIAN_POINT('Ctrl Pts',(-7.074975242,3.241073689,-2.494801346));
#103553=CARTESIAN_POINT('Ctrl Pts',(-7.128208186,3.268112745,-2.332090918));
#103554=CARTESIAN_POINT('Ctrl Pts',(-6.50035276356033,3.13852541968788,
-3.2105940187669));
#103555=CARTESIAN_POINT('Ctrl Pts',(-6.56918624068039,3.16400222532293,
-3.07122981342278));
#103556=CARTESIAN_POINT('Ctrl Pts',(-6.63335497953997,3.18928040281912,
-2.93001109800961));
#103557=CARTESIAN_POINT('Ctrl Pts',(-6.69274695865615,3.21428571385523,
-2.78740706582561));
#103558=CARTESIAN_POINT('Ctrl Pts',(-6.73444899117437,3.23184317440716,
-2.68727775405561));
#103559=CARTESIAN_POINT('Ctrl Pts',(-6.77400846551075,3.24953506287852,
-2.58595861844934));
#103560=CARTESIAN_POINT('Ctrl Pts',(-6.81133485153371,3.26733592560304,
-2.48358964988351));
#103561=CARTESIAN_POINT('Ctrl Pts',(-6.115687778,3.268101717,-3.893695289));
#103562=CARTESIAN_POINT('Ctrl Pts',(-6.326513683,3.203647866,-3.562558589));
#103563=CARTESIAN_POINT('Ctrl Pts',(-6.50035275900001,3.138525418,-3.210594028));
#103564=CARTESIAN_POINT('Ctrl Pts',(-6.191071751,3.268101717,-4.233276576));
#103565=CARTESIAN_POINT('Ctrl Pts',(-6.42028444,3.203647866,-3.898058176));
#103566=CARTESIAN_POINT('Ctrl Pts',(-6.61196208500001,3.138525418,-3.540050477));
#103567=CARTESIAN_POINT('',(-6.11819126500725,3.26733592574228,-3.88976035605099));
#103568=CARTESIAN_POINT('Origin',(0.180150236425488,3.08931097286523,0.0798200253232612));
#103569=CARTESIAN_POINT('Ctrl Pts',(-6.32846663464854,3.22840426962889,
-4.02498572048465));
#103570=CARTESIAN_POINT('Ctrl Pts',(-6.29344324060942,3.23458082928833,
-4.00234007261691));
#103571=CARTESIAN_POINT('Ctrl Pts',(-6.25839179944015,3.24090849488502,
-3.97973398944361));
#103572=CARTESIAN_POINT('Ctrl Pts',(-6.18831384716743,3.25387487495712,
-3.93466391254327));
#103573=CARTESIAN_POINT('Ctrl Pts',(-6.15324550754099,3.2605213240867,-3.91217300887544));
#103574=CARTESIAN_POINT('Ctrl Pts',(-6.11819126540562,3.26733592513327,
-3.88976035782639));
#103575=CARTESIAN_POINT('Ctrl Pts',(-5.658195312,3.138525418,-4.532915818));
#103576=CARTESIAN_POINT('Ctrl Pts',(-5.803594871,3.176642188,-4.351421359));
#103577=CARTESIAN_POINT('Ctrl Pts',(-5.93706413,3.214285714,-4.160981797));
#103578=CARTESIAN_POINT('Ctrl Pts',(-6.032043837,3.241073689,-4.025460749));
#103579=CARTESIAN_POINT('Ctrl Pts',(-6.120740961,3.268112745,-3.885747044));
#103580=CARTESIAN_POINT('Ctrl Pts',(-6.003941959,3.138525418,-4.494739253));
#103581=CARTESIAN_POINT('Ctrl Pts',(-6.14811695100001,3.176642188,-4.302154492));
#103582=CARTESIAN_POINT('Ctrl Pts',(-6.279653419,3.214285714,-4.100725903));
#103583=CARTESIAN_POINT('Ctrl Pts',(-6.373257709,3.241073689,-3.957384819));
#103584=CARTESIAN_POINT('Ctrl Pts',(-6.460224029,3.268112745,-3.80992198));
#103585=CARTESIAN_POINT('Ctrl Pts',(-5.65819531856153,3.13852541972012,
-4.53291580980959));
#103586=CARTESIAN_POINT('Ctrl Pts',(-5.7553786917797,3.16400222526261,-4.41160702510859));
#103587=CARTESIAN_POINT('Ctrl Pts',(-5.84840505051902,3.18928040275261,
-4.28748430692079));
#103588=CARTESIAN_POINT('Ctrl Pts',(-5.93706412966269,3.21428571390487,
-4.16098179748129));
#103589=CARTESIAN_POINT('Ctrl Pts',(-5.99931603428507,3.23184317451593,
-4.07215815694336));
#103590=CARTESIAN_POINT('Ctrl Pts',(-6.05973124909473,3.24953506284523,
-3.98171192458526));
#103591=CARTESIAN_POINT('Ctrl Pts',(-6.11819126715086,3.26733592561034,
-3.8897603553223));
#103592=CARTESIAN_POINT('Ctrl Pts',(-5.135677006,3.268101717,-5.117354951));
#103593=CARTESIAN_POINT('Ctrl Pts',(-5.41275852000001,3.203647866,-4.83928138000001));
#103594=CARTESIAN_POINT('Ctrl Pts',(-5.658195312,3.138525418,-4.532915818));
#103595=CARTESIAN_POINT('Ctrl Pts',(-5.136298605,3.268101717,-5.465202342));
#103596=CARTESIAN_POINT('Ctrl Pts',(-5.432214475,3.203647866,-5.187095114));
#103597=CARTESIAN_POINT('Ctrl Pts',(-5.696371877,3.138525418,-4.878662465));
#103598=CARTESIAN_POINT('',(-5.13896785769969,3.26733592570463,-5.11405019018087));
#103599=CARTESIAN_POINT('Origin',(0.15877957359841,3.08931098806011,0.116680933289348));
#103600=CARTESIAN_POINT('Ctrl Pts',(-5.31525764932106,3.2284042696144,-5.29131704928888));
#103601=CARTESIAN_POINT('Ctrl Pts',(-5.28592122767291,3.23458082926818,
-5.2616718497513));
#103602=CARTESIAN_POINT('Ctrl Pts',(-5.25654890943951,3.24090849485085,
-5.23205926065519));
#103603=CARTESIAN_POINT('Ctrl Pts',(-5.19779807493308,3.25387487494942,
-5.17297820876393));
#103604=CARTESIAN_POINT('Ctrl Pts',(-5.16838449306854,3.26052132408546,
-5.14347447343562));
#103605=CARTESIAN_POINT('Ctrl Pts',(-5.13896785708805,3.26733592514502,
-5.11405019156049));
#103606=CARTESIAN_POINT('Ctrl Pts',(-4.551466941,3.138525418,-5.643283502));
#103607=CARTESIAN_POINT('Ctrl Pts',(-4.732483083,3.176642188,-5.49728889));
#103608=CARTESIAN_POINT('Ctrl Pts',(-4.903770781,3.214285714,-5.339993645));
#103609=CARTESIAN_POINT('Ctrl Pts',(-5.025662935,3.241073689,-5.228058833));
#103610=CARTESIAN_POINT('Ctrl Pts',(-5.142320686,3.268112745,-5.110678816));
#103611=CARTESIAN_POINT('Ctrl Pts',(-4.897337056,3.138525418,-5.680324793));
#103612=CARTESIAN_POINT('Ctrl Pts',(-5.079541349,3.176642188,-5.523235918));
#103613=CARTESIAN_POINT('Ctrl Pts',(-5.251303759,3.214285714,-5.35479307));
#103614=CARTESIAN_POINT('Ctrl Pts',(-5.373533729,3.241073689,-5.234925376));
#103615=CARTESIAN_POINT('Ctrl Pts',(-5.490166976,3.268112745,-5.109605325));
#103616=CARTESIAN_POINT('Ctrl Pts',(-4.55146694901572,3.13852541968788,
-5.64328349553509));
#103617=CARTESIAN_POINT('Ctrl Pts',(-4.67245603173969,3.16400222519247,
-5.54570239561382));
#103618=CARTESIAN_POINT('Ctrl Pts',(-4.78999020139523,3.18928040269112,
-5.44447951512049));
#103619=CARTESIAN_POINT('Ctrl Pts',(-4.90377078064891,3.21428571390971,
-5.33999364537984));
#103620=CARTESIAN_POINT('Ctrl Pts',(-4.98366172793508,3.23184317458137,
-5.26662897113917));
#103621=CARTESIAN_POINT('Ctrl Pts',(-5.06210773487276,3.24953506279931,
-5.19128480698234));
#103622=CARTESIAN_POINT('Ctrl Pts',(-5.13896786002726,3.26733592552427,
-5.11405018991181));
#103623=CARTESIAN_POINT('Ctrl Pts',(-3.915527685,3.268101717,-6.101732783));
#103624=CARTESIAN_POINT('Ctrl Pts',(-4.245908786,3.203647866,-5.889724753));
#103625=CARTESIAN_POINT('Ctrl Pts',(-4.551466941,3.138525418,-5.643283502));
#103626=CARTESIAN_POINT('Ctrl Pts',(-3.841357845,3.268101717,-6.44158132));
#103627=CARTESIAN_POINT('Ctrl Pts',(-4.190140199,3.203647866,-6.23358925));
#103628=CARTESIAN_POINT('Ctrl Pts',(-4.51442565,3.138525418,-5.989153617));
#103629=CARTESIAN_POINT('',(-3.91945202400498,3.26733592572801,-6.09921272121348));
#103630=CARTESIAN_POINT('Origin',(0.129984324620748,3.08931095259013,0.148085736451091));
#103631=CARTESIAN_POINT('Ctrl Pts',(-4.05351312369227,3.22840426964832,
-6.31023227389369));
#103632=CARTESIAN_POINT('Ctrl Pts',(-4.0312354129448,3.23458082931858,-6.27497369893178));
#103633=CARTESIAN_POINT('Ctrl Pts',(-4.00891563470743,3.24090849486757,
-6.23973925566169));
#103634=CARTESIAN_POINT('Ctrl Pts',(-3.96423904174856,3.25387487499089,
-6.16940979302766));
#103635=CARTESIAN_POINT('Ctrl Pts',(-3.9418555640506,3.26052132411323,-6.13427278810945));
#103636=CARTESIAN_POINT('Ctrl Pts',(-3.91945202338612,3.26733592516335,
-6.09921272249568));
#103637=CARTESIAN_POINT('Ctrl Pts',(-3.231917035,3.138525418,-6.489777522));
#103638=CARTESIAN_POINT('Ctrl Pts',(-3.440085645,3.176642188,-6.386109302));
#103639=CARTESIAN_POINT('Ctrl Pts',(-3.641182561,3.214285714,-6.269313324));
#103640=CARTESIAN_POINT('Ctrl Pts',(-3.78428762,3.241073689,-6.18619869600001));
#103641=CARTESIAN_POINT('Ctrl Pts',(-3.923451211,3.268112745,-6.096640927));
#103642=CARTESIAN_POINT('Ctrl Pts',(-3.561738116,3.138525418,-6.600304659));
#103643=CARTESIAN_POINT('Ctrl Pts',(-3.773452038,3.176642188,-6.48605697100001));
#103644=CARTESIAN_POINT('Ctrl Pts',(-3.977408972,3.214285714,-6.358476065));
#103645=CARTESIAN_POINT('Ctrl Pts',(-4.122549284,3.241073689,-6.267686641));
#103646=CARTESIAN_POINT('Ctrl Pts',(-4.263395817,3.268112745,-6.170369204));
#103647=CARTESIAN_POINT('Ctrl Pts',(-3.23191704421808,3.13852541968788,
-6.48977751740939));
#103648=CARTESIAN_POINT('Ctrl Pts',(-3.37105452078987,3.16400222522259,
-6.42048688524908));
#103649=CARTESIAN_POINT('Ctrl Pts',(-3.50760073455668,3.18928040271179,
-6.34689691151957));
#103650=CARTESIAN_POINT('Ctrl Pts',(-3.64118256069049,3.21428571388654,
-6.26931332443069));
#103651=CARTESIAN_POINT('Ctrl Pts',(-3.73497693796392,3.2318431745299,-6.2148380678272));
#103652=CARTESIAN_POINT('Ctrl Pts',(-3.8277856892367,3.24953506285817,-6.15811898082334));
#103653=CARTESIAN_POINT('Ctrl Pts',(-3.91945202642927,3.26733592557389,
-6.09921272133924));
#103654=CARTESIAN_POINT('Ctrl Pts',(-2.512292641,3.268101717,-6.80080037100001));
#103655=CARTESIAN_POINT('Ctrl Pts',(-2.880525075,3.203647866,-6.664771142));
#103656=CARTESIAN_POINT('Ctrl Pts',(-3.231917035,3.138525418,-6.489777522));
#103657=CARTESIAN_POINT('Ctrl Pts',(-2.366799461,3.268101717,-7.116759116));
#103658=CARTESIAN_POINT('Ctrl Pts',(-2.752139625,3.203647866,-6.988607681));
#103659=CARTESIAN_POINT('Ctrl Pts',(-3.121389897,3.138525418,-6.819598603));
#103660=CARTESIAN_POINT('',(-2.51666697029969,3.26733592572713,-6.79918284407265));
#103661=CARTESIAN_POINT('Origin',(0.0951113227613803,3.08931096500382,0.172566420176966));
#103662=CARTESIAN_POINT('Ctrl Pts',(-2.60223082985599,3.22840426963563,
-7.03408805099015));
#103663=CARTESIAN_POINT('Ctrl Pts',(-2.58805351091312,3.23458082930022,
-6.99486475264879));
#103664=CARTESIAN_POINT('Ctrl Pts',(-2.57382992032545,3.24090849487529,
-6.95565597828295));
#103665=CARTESIAN_POINT('Ctrl Pts',(-2.54531659672928,3.25387487496946,
-6.87736663252218));
#103666=CARTESIAN_POINT('Ctrl Pts',(-2.53100984964101,3.26052132409144,
-6.83823932508442));
#103667=CARTESIAN_POINT('Ctrl Pts',(-2.5166669689879,3.26733592513527,-6.79918284529232));
#103668=CARTESIAN_POINT('Ctrl Pts',(-1.76124628,3.138525418,-7.032816757));
#103669=CARTESIAN_POINT('Ctrl Pts',(-1.986833627,3.176642188,-6.976322341));
#103670=CARTESIAN_POINT('Ctrl Pts',(-2.208336691,3.214285714,-6.905486881));
#103671=CARTESIAN_POINT('Ctrl Pts',(-2.365963221,3.241073689,-6.855078784));
#103672=CARTESIAN_POINT('Ctrl Pts',(-2.521125518,3.268112745,-6.79753088400001));
#103673=CARTESIAN_POINT('Ctrl Pts',(-2.05959626,3.138525418,-7.211661615));
#103674=CARTESIAN_POINT('Ctrl Pts',(-2.290920304,3.176642188,-7.14559720900001));
#103675=CARTESIAN_POINT('Ctrl Pts',(-2.517534962,3.214285714,-7.064843786));
#103676=CARTESIAN_POINT('Ctrl Pts',(-2.678799016,3.241073689,-7.007377845));
#103677=CARTESIAN_POINT('Ctrl Pts',(-2.837273008,3.268112745,-6.942613476));
#103678=CARTESIAN_POINT('Ctrl Pts',(-1.76124628998941,3.13852541968788,
-7.03281675449832));
#103679=CARTESIAN_POINT('Ctrl Pts',(-1.91202624773565,3.1640022252232,-6.99505654399892));
#103680=CARTESIAN_POINT('Ctrl Pts',(-2.06119975543362,3.18928040271826,
-6.95254046279405));
#103681=CARTESIAN_POINT('Ctrl Pts',(-2.20833669058812,3.21428571391941,
-6.90548688118375));
#103682=CARTESIAN_POINT('Ctrl Pts',(-2.31164877748298,3.23184317459871,
-6.8724482441944));
#103683=CARTESIAN_POINT('Ctrl Pts',(-2.41448063853639,3.24953506284485,
-6.83700635608134));
#103684=CARTESIAN_POINT('Ctrl Pts',(-2.51666697237623,3.26733592557854,
-6.7991828447383));
#103685=CARTESIAN_POINT('Ctrl Pts',(-0.991585586000001,3.268101717,-7.181870093));
#103686=CARTESIAN_POINT('Ctrl Pts',(-1.380451213,3.203647866,-7.128180239));
#103687=CARTESIAN_POINT('Ctrl Pts',(-1.76124628,3.138525418,-7.032816757));
#103688=CARTESIAN_POINT('Ctrl Pts',(-0.781572165,3.268101717,-7.459165164));
#103689=CARTESIAN_POINT('Ctrl Pts',(-1.18545206,3.203647866,-7.416846584));
#103690=CARTESIAN_POINT('Ctrl Pts',(-1.582401422,3.138525418,-7.331166738));
#103691=CARTESIAN_POINT('',(-0.996205365808877,3.26733592575295,-7.18123073379648));
#103692=CARTESIAN_POINT('Origin',(0.0557910408913048,3.08931098047701,0.188978248038894));
#103693=CARTESIAN_POINT('Ctrl Pts',(-1.02927111432491,3.22840426962271,
-7.42903768812463));
#103694=CARTESIAN_POINT('Ctrl Pts',(-1.02385710291355,3.23458082929551,
-7.38768370417306));
#103695=CARTESIAN_POINT('Ctrl Pts',(-1.01839477946308,3.24090849484858,
-7.34633395786893));
#103696=CARTESIAN_POINT('Ctrl Pts',(-1.00737797670184,3.25387487498619,
-7.26374545175727));
#103697=CARTESIAN_POINT('Ctrl Pts',(-1.00181692801302,3.26052132410948,
-7.22245739145548));
#103698=CARTESIAN_POINT('Ctrl Pts',(-0.996205364803589,3.2673359251782,
-7.18123073508118));
#103699=CARTESIAN_POINT('Ctrl Pts',(-0.208221606,3.138525418,-7.247009298));
#103700=CARTESIAN_POINT('Ctrl Pts',(-0.440679476,3.176642188,-7.240330301));
#103701=CARTESIAN_POINT('Ctrl Pts',(-0.672231452,3.214285714,-7.218767545));
#103702=CARTESIAN_POINT('Ctrl Pts',(-0.837009012,3.241073689,-7.203423007));
#103703=CARTESIAN_POINT('Ctrl Pts',(-1.000914798,3.268112745,-7.180575852));
#103704=CARTESIAN_POINT('Ctrl Pts',(-0.461149972000001,3.138525418,-7.485809288));
#103705=CARTESIAN_POINT('Ctrl Pts',(-0.701267683,3.176642188,-7.471017264));
#103706=CARTESIAN_POINT('Ctrl Pts',(-0.939943815,3.214285714,-7.440867263));
#103707=CARTESIAN_POINT('Ctrl Pts',(-1.109791084,3.241073689,-7.419411849));
#103708=CARTESIAN_POINT('Ctrl Pts',(-1.278482467,3.268112745,-7.390228859));
#103709=CARTESIAN_POINT('Ctrl Pts',(-0.208221615909558,3.1385254196249,
-7.24700929771528));
#103710=CARTESIAN_POINT('Ctrl Pts',(-0.363593751790943,3.16400222523584,
-7.24254513361163));
#103711=CARTESIAN_POINT('Ctrl Pts',(-0.518419366784687,3.18928040275688,
-7.23309094882667));
#103712=CARTESIAN_POINT('Ctrl Pts',(-0.672231451173942,3.21428571381686,
-7.21876754535419));
#103713=CARTESIAN_POINT('Ctrl Pts',(-0.78023048864515,3.23184317437099,
-7.20871037919489));
#103714=CARTESIAN_POINT('Ctrl Pts',(-0.888277156888164,3.24953506287325,
-7.19620291266289));
#103715=CARTESIAN_POINT('Ctrl Pts',(-0.996205367738843,3.2673359256217,
-7.18123073489443));
#103716=CARTESIAN_POINT('Ctrl Pts',(0.57548691,3.268101717,-7.22712355100001));
#103717=CARTESIAN_POINT('Ctrl Pts',(0.184171013,3.203647866,-7.258283552));
#103718=CARTESIAN_POINT('Ctrl Pts',(-0.208221606,3.138525418,-7.247009298));
#103719=CARTESIAN_POINT('Ctrl Pts',(0.840200577,3.268101717,-7.45278894));
#103720=CARTESIAN_POINT('Ctrl Pts',(0.436665925,3.203647866,-7.498281983));
#103721=CARTESIAN_POINT('Ctrl Pts',(0.030578384,3.138525418,-7.49993766400001));
#103722=CARTESIAN_POINT('',(0.57083769428385,3.26733592572195,-7.22749225621831));
#103723=CARTESIAN_POINT('Origin',(0.013861946971019,3.08931094139413,0.196553253651505));
#103724=CARTESIAN_POINT('Ctrl Pts',(0.591816174293092,3.2284042696266,-7.47661377961472));
#103725=CARTESIAN_POINT('Ctrl Pts',(0.588213725055049,3.23458082929749,
-7.43506277647234));
#103726=CARTESIAN_POINT('Ctrl Pts',(0.58465936936327,3.24090849486392,-7.39350552617535));
#103727=CARTESIAN_POINT('Ctrl Pts',(0.577664518215184,3.25387487498635,
-7.31047960671268));
#103728=CARTESIAN_POINT('Ctrl Pts',(0.574219840398537,3.26052132408112,
-7.26896137744006));
#103729=CARTESIAN_POINT('Ctrl Pts',(0.5708376961645,3.26733592511452,-7.22749225731375));
#103730=CARTESIAN_POINT('Ctrl Pts',(1.354539278,3.138525418,-7.12233973800001));
#103731=CARTESIAN_POINT('Ctrl Pts',(1.126080358,3.176642188,-7.16578846299999));
#103732=CARTESIAN_POINT('Ctrl Pts',(0.895306583,3.214285714,-7.194506663));
#103733=CARTESIAN_POINT('Ctrl Pts',(0.731082809,3.241073689,-7.214943176));
#103734=CARTESIAN_POINT('Ctrl Pts',(0.566097586,3.268112745,-7.227865074));
#103735=CARTESIAN_POINT('Ctrl Pts',(1.158859176,3.138525418,-7.40992884));
#103736=CARTESIAN_POINT('Ctrl Pts',(0.921175436,3.176642188,-7.447100854));
#103737=CARTESIAN_POINT('Ctrl Pts',(0.68159806,3.214285714,-7.468964057));
#103738=CARTESIAN_POINT('Ctrl Pts',(0.511109446,3.241073689,-7.48452240000001));
#103739=CARTESIAN_POINT('Ctrl Pts',(0.340088494,3.268112745,-7.492285353));
#103740=CARTESIAN_POINT('Ctrl Pts',(1.35453926809449,3.13852541965266,-7.12233973988385));
#103741=CARTESIAN_POINT('Ctrl Pts',(1.20183998324743,3.16400222535949,-7.15138036208737));
#103742=CARTESIAN_POINT('Ctrl Pts',(1.0486017351784,3.18928040286008,-7.17543014167008));
#103743=CARTESIAN_POINT('Ctrl Pts',(0.895306583377108,3.21428571393849,
-7.19450666295307));
#103744=CARTESIAN_POINT('Ctrl Pts',(0.787670510382668,3.23184317448289,
-7.20790122789566));
#103745=CARTESIAN_POINT('Ctrl Pts',(0.679461177112904,3.24953506300473,
-7.21891301928234));
#103746=CARTESIAN_POINT('Ctrl Pts',(0.570837692521339,3.2673359256781,-7.22749225782456));
#103747=CARTESIAN_POINT('Ctrl Pts',(2.115650277,3.268101717,-6.934444744));
#103748=CARTESIAN_POINT('Ctrl Pts',(1.740181607,3.203647866,-7.04899759200001));
#103749=CARTESIAN_POINT('Ctrl Pts',(1.354539278,3.138525418,-7.122339738));
#103750=CARTESIAN_POINT('Ctrl Pts',(2.422686474,3.268101717,-7.097928589));
#103751=CARTESIAN_POINT('Ctrl Pts',(2.038365897,3.203647866,-7.229106051));
#103752=CARTESIAN_POINT('Ctrl Pts',(1.64212838,3.138525418,-7.31801984));
#103753=CARTESIAN_POINT('',(2.11118901820754,3.26733592571401,-6.93580427368901));
#103754=CARTESIAN_POINT('Origin',(-0.0287152861479012,3.08931093193192,
0.194937927107114));
#103755=CARTESIAN_POINT('Ctrl Pts',(2.18523079690076,3.22840426966378,-7.17459172099073));
#103756=CARTESIAN_POINT('Ctrl Pts',(2.17278033341084,3.2345808293003,-7.13478657745776));
#103757=CARTESIAN_POINT('Ctrl Pts',(2.16037549600587,3.24090849486495,-7.09496499386631));
#103758=CARTESIAN_POINT('Ctrl Pts',(2.13569606206944,3.25387487492689,-7.01538386064082));
#103759=CARTESIAN_POINT('Ctrl Pts',(2.12340672683014,3.26052132405336,-6.97557680812192));
#103760=CARTESIAN_POINT('Ctrl Pts',(2.11118902049569,3.26733592510254,-6.93580427394857));
#103761=CARTESIAN_POINT('Ctrl Pts',(2.853963411,3.138525418,-6.664637488));
#103762=CARTESIAN_POINT('Ctrl Pts',(2.640185925,3.176642188,-6.75618232100001));
#103763=CARTESIAN_POINT('Ctrl Pts',(2.420981077,3.214285714,-6.833838645));
#103764=CARTESIAN_POINT('Ctrl Pts',(2.264990009,3.241073689,-6.88910062));
#103765=CARTESIAN_POINT('Ctrl Pts',(2.106639876,3.268112745,-6.937187358));
#103766=CARTESIAN_POINT('Ctrl Pts',(2.724681357,3.138525418,-6.98756835400001));
#103767=CARTESIAN_POINT('Ctrl Pts',(2.500545415,3.176642188,-7.074966286));
#103768=CARTESIAN_POINT('Ctrl Pts',(2.271269168,3.214285714,-7.147820393));
#103769=CARTESIAN_POINT('Ctrl Pts',(2.108111067,3.241073689,-7.199665003));
#103770=CARTESIAN_POINT('Ctrl Pts',(1.942757295,3.268112745,-7.244010912));
#103771=CARTESIAN_POINT('Ctrl Pts',(2.85396340153355,3.13852541968788,-6.66463749205377));
#103772=CARTESIAN_POINT('Ctrl Pts',(2.71107701654535,3.16400222536125,-6.72582499334367));
#103773=CARTESIAN_POINT('Ctrl Pts',(2.56659138536508,3.18928040285373,-6.78225419606807));
#103774=CARTESIAN_POINT('Ctrl Pts',(2.42098107764421,3.21428571387529,-6.83383864491471));
#103775=CARTESIAN_POINT('Ctrl Pts',(2.31874091118993,3.23184317441783,-6.87005862604735));
#103776=CARTESIAN_POINT('Ctrl Pts',(2.21542866235714,3.24953506278157,-6.90407477618169));
#103777=CARTESIAN_POINT('Ctrl Pts',(2.11118901681379,3.26733592566732,-6.9358042756577));
#103778=CARTESIAN_POINT('Ctrl Pts',(3.556888188,3.268101717,-6.317519008));
#103779=CARTESIAN_POINT('Ctrl Pts',(3.214823244,3.203647866,-6.510108339));
#103780=CARTESIAN_POINT('Ctrl Pts',(2.853963411,3.138525418,-6.664637488));
#103781=CARTESIAN_POINT('Ctrl Pts',(3.891890244,3.268101717,-6.411176985));
#103782=CARTESIAN_POINT('Ctrl Pts',(3.544754146,3.203647866,-6.621905155));
#103783=CARTESIAN_POINT('Ctrl Pts',(3.176894277,3.138525418,-6.793919543));
#103784=CARTESIAN_POINT('',(3.55282348998685,3.26733592572958,-6.31980579081641));
#103785=CARTESIAN_POINT('Origin',(-0.0699498340693178,3.08931098608908,
0.184207423807791));
#103786=CARTESIAN_POINT('Ctrl Pts',(3.67646645566667,3.22840426962795,-6.53709372735245));
#103787=CARTESIAN_POINT('Ctrl Pts',(3.65575014810974,3.23458082925275,-6.50089568761823));
#103788=CARTESIAN_POINT('Ctrl Pts',(3.6350748655154,3.24090849486529,-6.4646717835873));
#103789=CARTESIAN_POINT('Ctrl Pts',(3.59386483163922,3.25387487496164,-6.39225656160744));
#103790=CARTESIAN_POINT('Ctrl Pts',(3.57330547452155,3.26052132407031,-6.35602201976155));
#103791=CARTESIAN_POINT('Ctrl Pts',(3.55282349185555,3.26733592510644,-6.31980579111858));
#103792=CARTESIAN_POINT('Ctrl Pts',(4.219939387,3.138525418,-5.895304196));
#103793=CARTESIAN_POINT('Ctrl Pts',(4.030839333,3.176642188,-6.030664602));
#103794=CARTESIAN_POINT('Ctrl Pts',(3.833453187,3.214285714,-6.153627927));
#103795=CARTESIAN_POINT('Ctrl Pts',(3.692988795,3.241073689,-6.241131377));
#103796=CARTESIAN_POINT('Ctrl Pts',(3.548678026,3.268112745,-6.322134471));
#103797=CARTESIAN_POINT('Ctrl Pts',(4.163100466,3.138525418,-6.238476938));
#103798=CARTESIAN_POINT('Ctrl Pts',(3.96299267,3.176642188,-6.372014157));
#103799=CARTESIAN_POINT('Ctrl Pts',(3.754738253,3.214285714,-6.492452591));
#103800=CARTESIAN_POINT('Ctrl Pts',(3.606539757,3.241073689,-6.578159272));
#103801=CARTESIAN_POINT('Ctrl Pts',(3.454584923,3.268112745,-6.657014572));
#103802=CARTESIAN_POINT('Ctrl Pts',(4.21993937862631,3.13852541968788,-5.89530420199401));
#103803=CARTESIAN_POINT('Ctrl Pts',(4.09354710207681,3.16400222536351,-5.98577752262913));
#103804=CARTESIAN_POINT('Ctrl Pts',(3.96457007535463,3.18928040285766,-6.07194758173095));
#103805=CARTESIAN_POINT('Ctrl Pts',(3.83345318714864,3.21428571397165,-6.15362792690741));
#103806=CARTESIAN_POINT('Ctrl Pts',(3.74138956432755,3.2318431745597,-6.2109797190739));
#103807=CARTESIAN_POINT('Ctrl Pts',(3.64780516492101,3.24953506295641,-6.26640966964533));
#103808=CARTESIAN_POINT('Ctrl Pts',(3.55282348911443,3.26733592560357,-6.31980579292579));
#103809=CARTESIAN_POINT('Ctrl Pts',(4.831809961,3.268101717,-5.405193105));
#103810=CARTESIAN_POINT('Ctrl Pts',(4.539143318,3.203647866,-5.666813656));
#103811=CARTESIAN_POINT('Ctrl Pts',(4.219939387,3.138525418,-5.895304196));
#103812=CARTESIAN_POINT('Ctrl Pts',(5.179113551,3.268101717,-5.424645871));
#103813=CARTESIAN_POINT('Ctrl Pts',(4.88539363,3.203647866,-5.70507133300001));
#103814=CARTESIAN_POINT('Ctrl Pts',(4.563112129,3.138525418,-5.952143118));
#103815=CARTESIAN_POINT('',(4.82833188398055,3.26733592573913,-5.40830021374329));
#103816=CARTESIAN_POINT('Origin',(-0.107913616441742,3.08931095515453,0.164863647656065));
#103817=CARTESIAN_POINT('Ctrl Pts',(4.99579462933179,3.22840426964393,-5.59392849629774));
#103818=CARTESIAN_POINT('Ctrl Pts',(4.96778114867766,3.23458082931661,-5.56303014017645));
#103819=CARTESIAN_POINT('Ctrl Pts',(4.93980217423524,3.24090849488393,-5.53209770576372));
#103820=CARTESIAN_POINT('Ctrl Pts',(4.88398847580303,3.25387487498294,-5.4702344506208));
#103821=CARTESIAN_POINT('Ctrl Pts',(4.85612042961005,3.26052132408991,-5.43926670631695));
#103822=CARTESIAN_POINT('Ctrl Pts',(4.82833188572363,3.2673359251254,-5.40830021382373));
#103823=CARTESIAN_POINT('Ctrl Pts',(5.388595688,3.138525418,-4.850313032));
#103824=CARTESIAN_POINT('Ctrl Pts',(5.233015174,3.176642188,-5.023159709));
#103825=CARTESIAN_POINT('Ctrl Pts',(5.066677286,3.214285714,-5.185680407));
#103826=CARTESIAN_POINT('Ctrl Pts',(4.948307528,3.241073689,-5.301333767));
#103827=CARTESIAN_POINT('Ctrl Pts',(4.824783936,3.268112745,-5.411465603));
#103828=CARTESIAN_POINT('Ctrl Pts',(5.406857624,3.138525418,-5.197681275));
#103829=CARTESIAN_POINT('Ctrl Pts',(5.240134792,3.176642188,-5.371113728));
#103830=CARTESIAN_POINT('Ctrl Pts',(5.062639951,3.214285714,-5.533504923));
#103831=CARTESIAN_POINT('Ctrl Pts',(4.936330656,3.241073689,-5.649066125));
#103832=CARTESIAN_POINT('Ctrl Pts',(4.804880001,3.268112745,-5.75874362900001));
#103833=CARTESIAN_POINT('Ctrl Pts',(5.38859568103647,3.13852541970604,-4.85031303973633));
#103834=CARTESIAN_POINT('Ctrl Pts',(5.28460747541426,3.16400222529863,-4.96584174750943));
#103835=CARTESIAN_POINT('Ctrl Pts',(5.17716987523629,3.18928040278646,-5.07772344700988));
#103836=CARTESIAN_POINT('Ctrl Pts',(5.06667728632456,3.21428571392649,-5.18568040670526));
#103837=CARTESIAN_POINT('Ctrl Pts',(4.98909499935702,3.23184317453923,-5.26148230335792));
#103838=CARTESIAN_POINT('Ctrl Pts',(4.90961435227911,3.24953506289354,-5.33573421173237));
#103839=CARTESIAN_POINT('Ctrl Pts',(4.82833188365589,3.2673359255739,-5.40830021600123));
#103840=CARTESIAN_POINT('Ctrl Pts',(5.88080167,3.268101717,-4.240126379));
#103841=CARTESIAN_POINT('Ctrl Pts',(5.651218096,3.203647866,-4.558545065));
#103842=CARTESIAN_POINT('Ctrl Pts',(5.38859568799999,3.138525418,-4.850313032));
#103843=CARTESIAN_POINT('Ctrl Pts',(6.224167265,3.268101717,-4.184464345));
#103844=CARTESIAN_POINT('Ctrl Pts',(5.997597537,3.203647866,-4.521474716));
#103845=CARTESIAN_POINT('Ctrl Pts',(5.73596393,3.138525418,-4.832051096));
#103846=CARTESIAN_POINT('',(5.87807284531811,3.26733592573095,-4.24390852964466));
#103847=CARTESIAN_POINT('Origin',(-0.140831311052029,3.08931092092322,0.137810866124939));
#103848=CARTESIAN_POINT('Ctrl Pts',(6.08152499813999,3.22840426963123,-4.38919738580149));
#103849=CARTESIAN_POINT('Ctrl Pts',(6.04752422391984,3.23458082931669,-4.36504348632207));
#103850=CARTESIAN_POINT('Ctrl Pts',(6.01354982343028,3.24090849488865,-4.34084888746317));
#103851=CARTESIAN_POINT('Ctrl Pts',(5.9457422472682,3.25387487500342,-4.29243025597143));
#103852=CARTESIAN_POINT('Ctrl Pts',(5.91186859103641,3.26052132410905,-4.2681773263534));
#103853=CARTESIAN_POINT('Ctrl Pts',(5.87807284750703,3.26733592513226,-4.24390852857892));
#103854=CARTESIAN_POINT('Ctrl Pts',(6.30528724300001,3.138525418,-3.578526622));
#103855=CARTESIAN_POINT('Ctrl Pts',(6.190501041,3.176642188,-3.780777451));
#103856=CARTESIAN_POINT('Ctrl Pts',(6.062989186,3.214285714,-3.975256234));
#103857=CARTESIAN_POINT('Ctrl Pts',(5.972248902,3.241073689,-4.113651681));
#103858=CARTESIAN_POINT('Ctrl Pts',(5.875288312,3.268112745,-4.247762617));
#103859=CARTESIAN_POINT('Ctrl Pts',(6.397796129,3.138525418,-3.913847811));
#103860=CARTESIAN_POINT('Ctrl Pts',(6.272254035,3.176642188,-4.119065991));
#103861=CARTESIAN_POINT('Ctrl Pts',(6.133818231,3.214285714,-4.315816714));
#103862=CARTESIAN_POINT('Ctrl Pts',(6.03530422,3.241073689,-4.455828924));
#103863=CARTESIAN_POINT('Ctrl Pts',(5.93050422900001,3.268112745,-4.59120023400001));
#103864=CARTESIAN_POINT('Ctrl Pts',(6.3052872377432,3.13852541974561,-3.57852663126237));
#103865=CARTESIAN_POINT('Ctrl Pts',(6.22856547558023,3.16400222534719,-3.71370873221474));
#103866=CARTESIAN_POINT('Ctrl Pts',(6.14769096485557,3.18928040281778,-3.84607060772969));
#103867=CARTESIAN_POINT('Ctrl Pts',(6.06298918650265,3.21428571386929,-3.97525623361275));
#103868=CARTESIAN_POINT('Ctrl Pts',(6.00351589840414,3.23184317440521,-4.06596382168667));
#103869=CARTESIAN_POINT('Ctrl Pts',(5.94185542949822,3.24953506300735,-4.15556575210618));
#103870=CARTESIAN_POINT('Ctrl Pts',(5.87807284550827,3.26733592570877,-4.24390853185449));
#103871=CARTESIAN_POINT('Ctrl Pts',(6.65481363,3.268101717,-2.876796057));
#103872=CARTESIAN_POINT('Ctrl Pts',(6.499048197,3.203647866,-3.237123972));
#103873=CARTESIAN_POINT('Ctrl Pts',(6.305287243,3.138525418,-3.578526622));
#103874=CARTESIAN_POINT('Ctrl Pts',(6.978185836,3.268101717,-2.748621917));
#103875=CARTESIAN_POINT('Ctrl Pts',(6.82936045,3.203647866,-3.126458967));
#103876=CARTESIAN_POINT('Ctrl Pts',(6.640608432,3.138525418,-3.486017736));
#103877=CARTESIAN_POINT('',(6.65296165370764,3.26733592574237,-2.88107639920788));
#103878=CARTESIAN_POINT('Origin',(-0.167164222473216,3.0893109714355,0.104314448279226));
#103879=CARTESIAN_POINT('Ctrl Pts',(6.8828900176845,3.22840426961484,-2.97923228418363));
#103880=CARTESIAN_POINT('Ctrl Pts',(6.84449178843485,3.23458082927717,-2.96295225087537));
#103881=CARTESIAN_POINT('Ctrl Pts',(6.80611056664103,3.24090849489122,-2.946626800043));
#103882=CARTESIAN_POINT('Ctrl Pts',(6.72947971953556,3.25387487496616,-2.91391679399286));
#103883=CARTESIAN_POINT('Ctrl Pts',(6.69118434737886,3.26052132410795,-2.89751271921047));
#103884=CARTESIAN_POINT('Ctrl Pts',(6.6529616554568,3.26733592515834,-2.88107639836296));
#103885=CARTESIAN_POINT('Ctrl Pts',(6.927150574,3.138525418,-2.139412284));
#103886=CARTESIAN_POINT('Ctrl Pts',(6.85852596,3.176642188,-2.361610241));
#103887=CARTESIAN_POINT('Ctrl Pts',(6.775802451,3.214285714,-2.578953498));
#103888=CARTESIAN_POINT('Ctrl Pts',(6.716934554,3.241073689,-2.733619816));
#103889=CARTESIAN_POINT('Ctrl Pts',(6.651070736,3.268112745,-2.885438973));
#103890=CARTESIAN_POINT('Ctrl Pts',(7.089580798,3.138525418,-2.447007174));
#103891=CARTESIAN_POINT('Ctrl Pts',(7.011089651,3.176642188,-2.674415306));
#103892=CARTESIAN_POINT('Ctrl Pts',(6.918185988,3.214285714,-2.896325712));
#103893=CARTESIAN_POINT('Ctrl Pts',(6.852073667,3.241073689,-3.054242115));
#103894=CARTESIAN_POINT('Ctrl Pts',(6.778824671,3.268112745,-3.208977419));
#103895=CARTESIAN_POINT('Ctrl Pts',(6.92715057096117,3.13852541968788,-2.13941229383933));
#103896=CARTESIAN_POINT('Ctrl Pts',(6.8812826770035,3.16400222537056,-2.28792682359604));
#103897=CARTESIAN_POINT('Ctrl Pts',(6.83075285815803,3.1892804028607,-2.43457978110859));
#103898=CARTESIAN_POINT('Ctrl Pts',(6.77580245144929,3.21428571385279,-2.57895349743044));
#103899=CARTESIAN_POINT('Ctrl Pts',(6.7372190656392,3.23184317436579,-2.68032539196548));
#103900=CARTESIAN_POINT('Ctrl Pts',(6.69626195096635,3.24953506283404,-2.78108765672484));
#103901=CARTESIAN_POINT('Ctrl Pts',(6.65296165431191,3.26733592567481,-2.88107640154563));
#103902=CARTESIAN_POINT('Ctrl Pts',(7.1176539,3.268101717,-1.378949948));
#103903=CARTESIAN_POINT('Ctrl Pts',(7.042990027,3.203647866,-1.764338561));
#103904=CARTESIAN_POINT('Ctrl Pts',(6.92715057400001,3.138525418,-2.139412284));
#103905=CARTESIAN_POINT('Ctrl Pts',(7.405912192,3.268101717,-1.184256983));
#103906=CARTESIAN_POINT('Ctrl Pts',(7.341790058,3.203647866,-1.585253472));
#103907=CARTESIAN_POINT('Ctrl Pts',(7.234745464,3.138525418,-1.97698206));
#103908=CARTESIAN_POINT('',(7.11676537017746,3.26733592564584,-1.38352833888187));
#103909=CARTESIAN_POINT('Origin',(-0.185680395541384,3.08931094970989,0.065940249265263));
#103910=CARTESIAN_POINT('Ctrl Pts',(7.36241874941721,3.22840426966299,-1.42996159172976));
#103911=CARTESIAN_POINT('Ctrl Pts',(7.32141852347748,3.23458082931197,-1.42231666088157));
#103912=CARTESIAN_POINT('Ctrl Pts',(7.28042514453175,3.24090849482907,-1.41462371828302));
#103913=CARTESIAN_POINT('Ctrl Pts',(7.19855419931416,3.25387487491436,-1.39915182095323));
#103914=CARTESIAN_POINT('Ctrl Pts',(7.1576277604363,3.26052132403564,-1.3913636373889));
#103915=CARTESIAN_POINT('Ctrl Pts',(7.11676537032653,3.26733592507926,-1.38352833765408));
#103916=CARTESIAN_POINT('Ctrl Pts',(7.22510804400001,3.138525418,-0.600261405));
#103917=CARTESIAN_POINT('Ctrl Pts',(7.205853827,3.176642188,-0.832016762));
#103918=CARTESIAN_POINT('Ctrl Pts',(7.171786724,3.214285714,-1.062061763));
#103919=CARTESIAN_POINT('Ctrl Pts',(7.147543812,3.241073689,-1.225766926));
#103920=CARTESIAN_POINT('Ctrl Pts',(7.115856484,3.268112745,-1.38819541));
#103921=CARTESIAN_POINT('Ctrl Pts',(7.449864548,3.138525418,-0.865747201));
#103922=CARTESIAN_POINT('Ctrl Pts',(7.422094506,3.176642188,-1.104711934));
#103923=CARTESIAN_POINT('Ctrl Pts',(7.379067058,3.214285714,-1.341405739));
#103924=CARTESIAN_POINT('Ctrl Pts',(7.348447764,3.241073689,-1.509842339));
#103925=CARTESIAN_POINT('Ctrl Pts',(7.310174806,3.268112745,-1.676706386));
#103926=CARTESIAN_POINT('Ctrl Pts',(7.22510804312559,3.13852541973103,-0.600261415524939));
#103927=CARTESIAN_POINT('Ctrl Pts',(7.21223874827869,3.16400222530692,-0.755163999666638));
#103928=CARTESIAN_POINT('Ctrl Pts',(7.19441633930332,3.18928040278829,-0.909250710107161));
#103929=CARTESIAN_POINT('Ctrl Pts',(7.17178672409929,3.21428571389028,-1.06206176232951));
#103930=CARTESIAN_POINT('Ctrl Pts',(7.1558973568498,3.2318431745165,-1.16935792614114));
#103931=CARTESIAN_POINT('Ctrl Pts',(7.1375587053205,3.24953506279988,-1.27656899333765));
#103932=CARTESIAN_POINT('Ctrl Pts',(7.11676537124032,3.26733592538515,-1.38352834137664));
#103933=CARTESIAN_POINT('Ctrl Pts',(7.247680585,3.268101717,0.183374327));
#103934=CARTESIAN_POINT('Ctrl Pts',(7.257609471,3.203647866,-0.209054639));
#103935=CARTESIAN_POINT('Ctrl Pts',(7.225108044,3.138525418,-0.600261405));
#103936=CARTESIAN_POINT('Ctrl Pts',(7.487346326,3.268101717,0.435482491));
#103937=CARTESIAN_POINT('Ctrl Pts',(7.510925723,3.203647866,0.030076714));
#103938=CARTESIAN_POINT('Ctrl Pts',(7.49059384,3.138525418,-0.375504901));
#103939=CARTESIAN_POINT('',(7.24779704613829,3.26733592573548,0.178711968919609));
#103940=CARTESIAN_POINT('Origin',(-0.195514704512931,3.08931097303294,0.0244827985403307));
#103941=CARTESIAN_POINT('Ctrl Pts',(7.49768896349623,3.22840426965684,0.18617251498347));
#103942=CARTESIAN_POINT('Ctrl Pts',(7.45600386584464,3.23458082930064,0.184824874873088));
#103943=CARTESIAN_POINT('Ctrl Pts',(7.41431513378787,3.24090849486615,0.183525596007401));
#103944=CARTESIAN_POINT('Ctrl Pts',(7.33103228512314,3.25387487500965,0.181035935899268));
#103945=CARTESIAN_POINT('Ctrl Pts',(7.28938845447293,3.2605213241582,0.179844061555137));
#103946=CARTESIAN_POINT('Ctrl Pts',(7.24779704649391,3.26733592525333,0.178711970411889));
#103947=CARTESIAN_POINT('Ctrl Pts',(7.18522749100001,3.138525418,0.96695703));
#103948=CARTESIAN_POINT('Ctrl Pts',(7.216243979,3.176642188,0.736480897));
#103949=CARTESIAN_POINT('Ctrl Pts',(7.23242622,3.214285714,0.5044908));
#103950=CARTESIAN_POINT('Ctrl Pts',(7.243941865,3.241073689,0.339401464));
#103951=CARTESIAN_POINT('Ctrl Pts',(7.247912692,3.268112745,0.173958629));
#103952=CARTESIAN_POINT('Ctrl Pts',(7.461800912,3.138525418,0.755994149));
#103953=CARTESIAN_POINT('Ctrl Pts',(7.486050472,3.176642188,0.516646541000001));
#103954=CARTESIAN_POINT('Ctrl Pts',(7.494911153,3.214285714,0.276236876));
#103955=CARTESIAN_POINT('Ctrl Pts',(7.501216611,3.241073689,0.105155986));
#103956=CARTESIAN_POINT('Ctrl Pts',(7.499709291,3.268112745,-0.066034427));
#103957=CARTESIAN_POINT('Ctrl Pts',(7.18522749238694,3.13852541970443,0.966957019694023));
#103958=CARTESIAN_POINT('Ctrl Pts',(7.20595855182675,3.16400222522679,0.812909454265956));
#103959=CARTESIAN_POINT('Ctrl Pts',(7.22167690884421,3.18928040272318,0.658593914269724));
#103960=CARTESIAN_POINT('Ctrl Pts',(7.23242622034782,3.21428571381248,0.504490800783123));
#103961=CARTESIAN_POINT('Ctrl Pts',(7.23997384168336,3.23184317440338,0.396287417808053));
#103962=CARTESIAN_POINT('Ctrl Pts',(7.24511114796464,3.2495350629339,0.287640616691123));
#103963=CARTESIAN_POINT('Ctrl Pts',(7.24779704763703,3.26733592561058,0.178711967189));
#103964=CARTESIAN_POINT('Ctrl Pts',(7.03881378,3.268101717,1.737124223));
#103965=CARTESIAN_POINT('Ctrl Pts',(7.132871163,3.203647866,1.356004445));
#103966=CARTESIAN_POINT('Ctrl Pts',(7.185227491,3.138525418,0.96695703));
#103967=CARTESIAN_POINT('Ctrl Pts',(7.218680466,3.268101717,2.034859288));
#103968=CARTESIAN_POINT('Ctrl Pts',(7.328858849,3.203647866,1.644000547));
#103969=CARTESIAN_POINT('Ctrl Pts',(7.39619037200001,3.138525418,1.24353045));
#103970=CARTESIAN_POINT('',(7.03992978765218,3.26733592573162,1.73259590431476));
#103971=CARTESIAN_POINT('Origin',(-0.19620638574868,3.0893109602979,-0.0181194053157016));
#103972=CARTESIAN_POINT('Ctrl Pts',(7.28237557417294,3.22840426964679,1.79360140244549));
#103973=CARTESIAN_POINT('Ctrl Pts',(7.24195475358925,3.23458082933613,1.78332420568998));
#103974=CARTESIAN_POINT('Ctrl Pts',(7.20151998757062,3.24090849489714,1.77309345819916));
#103975=CARTESIAN_POINT('Ctrl Pts',(7.12071944905017,3.25387487502398,1.75275865431607));
#103976=CARTESIAN_POINT('Ctrl Pts',(7.08030544586912,3.26052132414294,1.74264245270595));
#103977=CARTESIAN_POINT('Ctrl Pts',(7.03992978822808,3.2673359251799,1.73259590600152));
#103978=CARTESIAN_POINT('Ctrl Pts',(6.809373687,3.138525418,2.488961628));
#103979=CARTESIAN_POINT('Ctrl Pts',(6.889210582,3.176642188,2.270541528));
#103980=CARTESIAN_POINT('Ctrl Pts',(6.954885505,3.214285714,2.047453934));
#103981=CARTESIAN_POINT('Ctrl Pts',(7.001621248,3.241073689,1.888699818));
#103982=CARTESIAN_POINT('Ctrl Pts',(7.04106455800001,3.268112745,1.727978555));
#103983=CARTESIAN_POINT('Ctrl Pts',(7.124831758,3.138525418,2.342386053));
#103984=CARTESIAN_POINT('Ctrl Pts',(7.199967038,3.176642188,2.113847197));
#103985=CARTESIAN_POINT('Ctrl Pts',(7.260301532,3.214285714,1.880962961));
#103986=CARTESIAN_POINT('Ctrl Pts',(7.303236907,3.241073689,1.715237335));
#103987=CARTESIAN_POINT('Ctrl Pts',(7.338565706,3.268112745,1.547725229));
#103988=CARTESIAN_POINT('Ctrl Pts',(6.80937369053532,3.13852541968788,2.48896161832797));
#103989=CARTESIAN_POINT('Ctrl Pts',(6.86273574210131,3.16400222528892,2.34297216457238));
#103990=CARTESIAN_POINT('Ctrl Pts',(6.91125989225883,3.18928040278009,2.19564341859102));
#103991=CARTESIAN_POINT('Ctrl Pts',(6.95488550497705,3.21428571389738,2.04745393452308));
#103992=CARTESIAN_POINT('Ctrl Pts',(6.98551719578398,3.23184317447546,1.94340280208701));
#103993=CARTESIAN_POINT('Ctrl Pts',(7.01389024523924,3.249535062973,1.83840047195019));
#103994=CARTESIAN_POINT('Ctrl Pts',(7.03992978951053,3.26733592562892,1.73259590295414));
#103995=CARTESIAN_POINT('Ctrl Pts',(6.500819867,3.268101717,3.209648121));
#103996=CARTESIAN_POINT('Ctrl Pts',(6.67460772600001,3.203647866,2.857658268));
#103997=CARTESIAN_POINT('Ctrl Pts',(6.809373687,3.138525418,2.488961628));
#103998=CARTESIAN_POINT('Ctrl Pts',(6.612477132,3.268101717,3.539088327));
#103999=CARTESIAN_POINT('Ctrl Pts',(6.804102681,3.203647866,3.18105274));
#104000=CARTESIAN_POINT('Ctrl Pts',(6.955949263,3.138525418,2.804419699));
#104001=CARTESIAN_POINT('',(6.50288323752183,3.26733592574725,3.20546558011673));
#104002=CARTESIAN_POINT('Origin',(-0.187724223664845,3.08931099242651,-0.0598744337741502));
#104003=CARTESIAN_POINT('Ctrl Pts',(6.72654639743712,3.22840426967264,3.31716348119342));
#104004=CARTESIAN_POINT('Ctrl Pts',(6.6892798868357,3.23458082931749,3.2984372779879));
#104005=CARTESIAN_POINT('Ctrl Pts',(6.6519897713015,3.2409084948931,3.27975344013471));
#104006=CARTESIAN_POINT('Ctrl Pts',(6.57744968623373,3.25387487500758,3.24252432532321));
#104007=CARTESIAN_POINT('Ctrl Pts',(6.54015522430933,3.26052132413064,3.22395681883508));
#104008=CARTESIAN_POINT('Ctrl Pts',(6.50288323759506,3.26733592520138,3.20546558181229));
#104009=CARTESIAN_POINT('Ctrl Pts',(6.115121138,3.138525418,3.894585148));
#104010=CARTESIAN_POINT('Ctrl Pts',(6.240045355,3.176642188,3.69843416));
#104011=CARTESIAN_POINT('Ctrl Pts',(6.352142073,3.214285714,3.494680397));
#104012=CARTESIAN_POINT('Ctrl Pts',(6.431912603,3.241073689,3.349684667));
#104013=CARTESIAN_POINT('Ctrl Pts',(6.50498407100001,3.268112745,3.201200124));
#104014=CARTESIAN_POINT('Ctrl Pts',(6.45471339,3.138525418,3.819250588));
#104015=CARTESIAN_POINT('Ctrl Pts',(6.577221147,3.176642188,3.612206708));
#104016=CARTESIAN_POINT('Ctrl Pts',(6.686208281,3.214285714,3.397737309));
#104017=CARTESIAN_POINT('Ctrl Pts',(6.763765961,3.241073689,3.245116092));
#104018=CARTESIAN_POINT('Ctrl Pts',(6.834278944,3.268112745,3.089114974));
#104019=CARTESIAN_POINT('Ctrl Pts',(6.1151211433741,3.13852541963974,3.8945851395618));
#104020=CARTESIAN_POINT('Ctrl Pts',(6.1986190363352,3.16400222521114,3.76348010129596));
#104021=CARTESIAN_POINT('Ctrl Pts',(6.27768004407713,3.18928040272125,3.63002707695493));
#104022=CARTESIAN_POINT('Ctrl Pts',(6.35214207269071,3.21428571380303,3.49468039798569));
#104023=CARTESIAN_POINT('Ctrl Pts',(6.40442552953867,3.23184317433645,3.39964683133381));
#104024=CARTESIAN_POINT('Ctrl Pts',(6.45470762996514,3.24953506283669,3.30319876439432));
#104025=CARTESIAN_POINT('Ctrl Pts',(6.50288323951224,3.2673359256285,3.20546557920868));
#104026=CARTESIAN_POINT('Ctrl Pts',(5.658854841,3.268101717,4.53209244));
#104027=CARTESIAN_POINT('Ctrl Pts',(5.904247051,3.203647866,4.225691167));
#104028=CARTESIAN_POINT('Ctrl Pts',(6.11512113800001,3.138525418,3.894585148));
#104029=CARTESIAN_POINT('Ctrl Pts',(5.697081715,3.268101717,4.877833528));
#104030=CARTESIAN_POINT('Ctrl Pts',(5.961194234,3.203647866,4.569362444));
#104031=CARTESIAN_POINT('Ctrl Pts',(6.190455698,3.138525418,4.2341774));
#104032=CARTESIAN_POINT('',(5.6617690946082,3.26733592567607,4.52845124890004));
#104033=CARTESIAN_POINT('Origin',(-0.170464175807428,3.08931094541484,-0.0988298078200384));
#104034=CARTESIAN_POINT('Ctrl Pts',(5.85619138690672,3.22840426963792,4.68561868236563));
#104035=CARTESIAN_POINT('Ctrl Pts',(5.82382172680805,3.23458082926551,4.65931908942937));
#104036=CARTESIAN_POINT('Ctrl Pts',(5.79141990628079,3.2409084948322,4.63305579687645));
#104037=CARTESIAN_POINT('Ctrl Pts',(5.72662568622392,3.25387487490412,4.58067316335606));
#104038=CARTESIAN_POINT('Ctrl Pts',(5.69419461305615,3.26052132402377,4.55452254790572));
#104039=CARTESIAN_POINT('Ctrl Pts',(5.66176909404866,3.26733592507081,4.52845125034263));
#104040=CARTESIAN_POINT('Ctrl Pts',(5.13493232,3.138525418,5.118102194));
#104041=CARTESIAN_POINT('Ctrl Pts',(5.299102543,3.176642188,4.953392122));
#104042=CARTESIAN_POINT('Ctrl Pts',(5.452379538,3.214285714,4.77849949));
#104043=CARTESIAN_POINT('Ctrl Pts',(5.561454873,3.241073689,4.654041985));
#104044=CARTESIAN_POINT('Ctrl Pts',(5.664737759,3.268112745,4.524737133));
#104045=CARTESIAN_POINT('Ctrl Pts',(5.482779798,3.138525418,5.11753121));
#104046=CARTESIAN_POINT('Ctrl Pts',(5.646931706,3.176642188,4.941663448));
#104047=CARTESIAN_POINT('Ctrl Pts',(5.799475362,3.214285714,4.755637236));
#104048=CARTESIAN_POINT('Ctrl Pts',(5.908028837,3.241073689,4.623256827));
#104049=CARTESIAN_POINT('Ctrl Pts',(6.010428894,3.268112745,4.486061135));
#104050=CARTESIAN_POINT('Ctrl Pts',(5.13493232726974,3.13852541968788,5.11810218670635));
#104051=CARTESIAN_POINT('Ctrl Pts',(5.24466179475057,3.16400222542499,5.00801189012052));
#104052=CARTESIAN_POINT('Ctrl Pts',(5.35056285532906,3.18928040292007,4.89467470347088));
#104053=CARTESIAN_POINT('Ctrl Pts',(5.45237953812021,3.21428571400291,4.77849948997936));
#104054=CARTESIAN_POINT('Ctrl Pts',(5.52387004438808,3.23184317456548,4.69692715254307));
#104055=CARTESIAN_POINT('Ctrl Pts',(5.59371006074637,3.24953506288096,4.61354315344578));
#104056=CARTESIAN_POINT('Ctrl Pts',(5.6617690969508,3.26733592546731,4.5284512482931));
#104057=CARTESIAN_POINT('Ctrl Pts',(4.552288053,3.268101717,5.642621154));
#104058=CARTESIAN_POINT('Ctrl Pts',(4.857810345,3.203647866,5.396135444));
#104059=CARTESIAN_POINT('Ctrl Pts',(5.13493232,3.138525418,5.118102194));
#104060=CARTESIAN_POINT('Ctrl Pts',(4.51529709,3.268101717,5.988496655));
#104061=CARTESIAN_POINT('Ctrl Pts',(4.839546969,3.203647866,5.744013838));
#104062=CARTESIAN_POINT('Ctrl Pts',(5.135503304,3.138525418,5.465949672));
#104063=CARTESIAN_POINT('',(4.55591692092414,3.26733592572585,5.63969156909739));
#104064=CARTESIAN_POINT('Origin',(-0.145233333313992,3.08931099796829,-0.133163996178347));
#104065=CARTESIAN_POINT('Ctrl Pts',(4.71200737576507,3.22840426963644,5.83497956214701));
#104066=CARTESIAN_POINT('Ctrl Pts',(4.68604813527371,3.23458082930412,5.80233631877584));
#104067=CARTESIAN_POINT('Ctrl Pts',(4.66004968290258,3.24090849487674,5.7697216137166));
#104068=CARTESIAN_POINT('Ctrl Pts',(4.60803103346474,3.25387487499756,5.70463481473088));
#104069=CARTESIAN_POINT('Ctrl Pts',(4.58197979008192,3.26052132414438,5.67212386389294));
#104070=CARTESIAN_POINT('Ctrl Pts',(4.55591692004631,3.26733592521512,5.63969157057812));
#104071=CARTESIAN_POINT('Ctrl Pts',(3.914639774,3.138525418,6.10230247));
#104072=CARTESIAN_POINT('Ctrl Pts',(4.110379585,3.176642188,5.976734973));
#104073=CARTESIAN_POINT('Ctrl Pts',(4.297669796,3.214285714,5.838881257));
#104074=CARTESIAN_POINT('Ctrl Pts',(4.430949694,3.241073689,5.740781472));
#104075=CARTESIAN_POINT('Ctrl Pts',(4.559614604,3.268112745,5.636702463));
#104076=CARTESIAN_POINT('Ctrl Pts',(4.254477516,3.138525418,6.176521761));
#104077=CARTESIAN_POINT('Ctrl Pts',(4.452598014,3.176642188,6.040053497));
#104078=CARTESIAN_POINT('Ctrl Pts',(4.641565421,3.214285714,5.891168852));
#104079=CARTESIAN_POINT('Ctrl Pts',(4.776038851,3.241073689,5.785219212));
#104080=CARTESIAN_POINT('Ctrl Pts',(4.90553787,3.268112745,5.673244064));
#104081=CARTESIAN_POINT('Ctrl Pts',(3.91463978266771,3.13852541968788,6.10230246443964));
#104082=CARTESIAN_POINT('Ctrl Pts',(4.04546999514332,3.16400222533056,6.01837461000903));
#104083=CARTESIAN_POINT('Ctrl Pts',(4.17325929301746,3.18928040281961,5.93045278158138));
#104084=CARTESIAN_POINT('Ctrl Pts',(4.29766979596682,3.21428571398577,5.83888125705783));
#104085=CARTESIAN_POINT('Ctrl Pts',(4.38502453499581,3.23184317464813,5.77458438070685));
#104086=CARTESIAN_POINT('Ctrl Pts',(4.47115682528837,3.24953506301695,5.70816339197302));
#104087=CARTESIAN_POINT('Ctrl Pts',(4.5559169233774,3.26733592566823,5.63969156895996));
#104088=CARTESIAN_POINT('Ctrl Pts',(3.232861335,3.268101717,6.489307173));
#104089=CARTESIAN_POINT('Ctrl Pts',(3.584227827,3.203647866,6.314262424));
#104090=CARTESIAN_POINT('Ctrl Pts',(3.914639774,3.138525418,6.10230247));
#104091=CARTESIAN_POINT('Ctrl Pts',(3.122382191,3.268101717,6.819144334));
#104092=CARTESIAN_POINT('Ctrl Pts',(3.491607867,3.203647866,6.650081528));
#104093=CARTESIAN_POINT('Ctrl Pts',(3.840420483,3.138525418,6.442140212));
#104094=CARTESIAN_POINT('',(3.23703513325096,3.26733592572603,6.48722618092339));
#104095=CARTESIAN_POINT('Origin',(-0.113211494847973,3.08931099930371,-0.161271503760252));
#104096=CARTESIAN_POINT('Ctrl Pts',(3.3474951365056,3.22840426965528,6.71150328220225));
#104097=CARTESIAN_POINT('Ctrl Pts',(3.32916014099174,3.23458082935693,6.6740427501092));
#104098=CARTESIAN_POINT('Ctrl Pts',(3.31078071561423,3.24090849490936,6.63660166006154));
#104099=CARTESIAN_POINT('Ctrl Pts',(3.27396951324241,3.25387503634,6.56185315250801));
#104100=CARTESIAN_POINT('Ctrl Pts',(3.25551646985801,3.26052140343644,6.52450253885886));
#104101=CARTESIAN_POINT('Ctrl Pts',(3.23703513444458,3.26733592526798,6.48722618166755));
#104102=CARTESIAN_POINT('Ctrl Pts',(2.511303023,3.138525418,6.801165865));
#104103=CARTESIAN_POINT('Ctrl Pts',(2.729459846,3.176642188,6.720612339));
#104104=CARTESIAN_POINT('Ctrl Pts',(2.94200579,3.214285714,6.626243425));
#104105=CARTESIAN_POINT('Ctrl Pts',(3.093258233,3.241073689,6.559088397));
#104106=CARTESIAN_POINT('Ctrl Pts',(3.241288939,3.268112745,6.485101851));
#104107=CARTESIAN_POINT('Ctrl Pts',(2.827240594,3.138525418,6.946705019));
#104108=CARTESIAN_POINT('Ctrl Pts',(3.050065787,3.176642188,6.85601735800001));
#104109=CARTESIAN_POINT('Ctrl Pts',(3.26662104,3.214285714,6.75123596));
#104110=CARTESIAN_POINT('Ctrl Pts',(3.420726596,3.241073689,6.676671176));
#104111=CARTESIAN_POINT('Ctrl Pts',(3.571269346,3.268112745,6.595152406));
#104112=CARTESIAN_POINT('Ctrl Pts',(2.51130303206539,3.13852541958392,6.80116586165265));
#104113=CARTESIAN_POINT('Ctrl Pts',(2.65711651481935,3.1640022252604,6.74732482170336));
#104114=CARTESIAN_POINT('Ctrl Pts',(2.80081876440615,3.18928040278802,6.68892947800552));
#104115=CARTESIAN_POINT('Ctrl Pts',(2.94200578981347,3.21428571395176,6.62624342515397));
#104116=CARTESIAN_POINT('Ctrl Pts',(3.04114014826,3.23184317395206,6.58222846251681));
#104117=CARTESIAN_POINT('Ctrl Pts',(3.13953726152714,3.2495350620974,6.53587625704981));
#104118=CARTESIAN_POINT('Ctrl Pts',(3.2370351341919,3.26733592505327,6.48722618256294));
#104119=CARTESIAN_POINT('Ctrl Pts',(1.762269613,3.268101717,7.032560402));
#104120=CARTESIAN_POINT('Ctrl Pts',(2.1430508,3.203647866,6.937141511));
#104121=CARTESIAN_POINT('Ctrl Pts',(2.511303023,3.138525418,6.801165865));
#104122=CARTESIAN_POINT('Ctrl Pts',(1.583468171,3.268101717,7.330936403));
#104123=CARTESIAN_POINT('Ctrl Pts',(1.980405062,3.203647866,7.245198798));
#104124=CARTESIAN_POINT('Ctrl Pts',(2.365763869,3.138525418,7.117103436));
#104125=CARTESIAN_POINT('',(1.76679318523583,3.26733592572127,7.03142530529778));
#104126=CARTESIAN_POINT('Origin',(-0.075896083697797,3.08931092501544,-0.181838197832388));
#104127=CARTESIAN_POINT('Ctrl Pts',(1.82645774549794,3.22840426964308,7.27420456827652));
#104128=CARTESIAN_POINT('Ctrl Pts',(1.81660431903139,3.23458082932623,7.23367836066828));
#104129=CARTESIAN_POINT('Ctrl Pts',(1.80670332193979,3.24090849486778,7.19316158940839));
#104130=CARTESIAN_POINT('Ctrl Pts',(1.7868217117759,3.25387487498457,7.11224834650389));
#104131=CARTESIAN_POINT('Ctrl Pts',(1.77682923752812,3.26052132408962,7.07180357369656));
#104132=CARTESIAN_POINT('Ctrl Pts',(1.76679318372669,3.26733592512765,7.03142530650721));
#104133=CARTESIAN_POINT('Ctrl Pts',(0.990540534000001,3.138525418,7.182014303));
#104134=CARTESIAN_POINT('Ctrl Pts',(1.220913599,3.176642188,7.150241342));
#104135=CARTESIAN_POINT('Ctrl Pts',(1.448776863,3.214285714,7.103769816));
#104136=CARTESIAN_POINT('Ctrl Pts',(1.610929454,3.241073689,7.07069964));
#104137=CARTESIAN_POINT('Ctrl Pts',(1.771404205,3.268112745,7.03026508300001));
#104138=CARTESIAN_POINT('Ctrl Pts',(1.267805044,3.138525418,7.392068071));
#104139=CARTESIAN_POINT('Ctrl Pts',(1.504915875,3.176642188,7.351401467));
#104140=CARTESIAN_POINT('Ctrl Pts',(1.738933089,3.214285714,7.295622778));
#104141=CARTESIAN_POINT('Ctrl Pts',(1.905464967,3.241073689,7.255929416));
#104142=CARTESIAN_POINT('Ctrl Pts',(2.070012238,3.268112745,7.208678751));
#104143=CARTESIAN_POINT('Ctrl Pts',(0.990540544201338,3.13852541968788,
7.18201430159303));
#104144=CARTESIAN_POINT('Ctrl Pts',(1.14451922017561,3.16400222521989,7.16077762395493));
#104145=CARTESIAN_POINT('Ctrl Pts',(1.29741506331278,3.18928040271736,7.13463926685995));
#104146=CARTESIAN_POINT('Ctrl Pts',(1.44877686277554,3.21428571395516,7.1037698160864));
#104147=CARTESIAN_POINT('Ctrl Pts',(1.55505543508907,3.23184317462731,7.08209485501571));
#104148=CARTESIAN_POINT('Ctrl Pts',(1.66111643389606,3.24953506298842,7.057978808402));
#104149=CARTESIAN_POINT('Ctrl Pts',(1.76679318731429,3.26733592562012,7.03142530616991));
#104150=CARTESIAN_POINT('Ctrl Pts',(0.209276124,3.268101717,7.246978923));
#104151=CARTESIAN_POINT('Ctrl Pts',(0.601667098,3.203647866,7.235647572));
#104152=CARTESIAN_POINT('Ctrl Pts',(0.990540534,3.138525418,7.18201430300001));
#104153=CARTESIAN_POINT('Ctrl Pts',(-0.029487061,3.268101717,7.499942034));
#104154=CARTESIAN_POINT('Ctrl Pts',(0.376600717,3.203647866,7.501538624));
#104155=CARTESIAN_POINT('Ctrl Pts',(0.780486766,3.138525418,7.459278813));
#104156=CARTESIAN_POINT('',(0.213937949517071,3.26733592599679,7.24684279804168));
#104157=CARTESIAN_POINT('Origin',(-0.0350318247030968,3.08931099397693,
-0.193902277461947));
#104158=CARTESIAN_POINT('Ctrl Pts',(0.220017220171418,3.22840426961572,
7.49677213338353));
#104159=CARTESIAN_POINT('Ctrl Pts',(0.219106098112348,3.23458082928566,
7.45507521069873));
#104160=CARTESIAN_POINT('Ctrl Pts',(0.218146489016196,3.24090849485656,
7.41337727728728));
#104161=CARTESIAN_POINT('Ctrl Pts',(0.216123655392674,3.25387487502344,
7.33008178262261));
#104162=CARTESIAN_POINT('Ctrl Pts',(0.215059230316357,3.2605213241711,7.28843449952145));
#104163=CARTESIAN_POINT('Ctrl Pts',(0.213937947891238,3.26733592525954,
7.24684279881095));
#104164=CARTESIAN_POINT('Ctrl Pts',(-0.576538529,3.138525418,7.22703973500001));
#104165=CARTESIAN_POINT('Ctrl Pts',(-0.344721211,3.176642188,7.245533007));
#104166=CARTESIAN_POINT('Ctrl Pts',(-0.112195259,3.214285714,7.249131826));
#104167=CARTESIAN_POINT('Ctrl Pts',(0.053275404,3.241073689,7.251692825));
#104168=CARTESIAN_POINT('Ctrl Pts',(0.218690579,3.268112745,7.246700934));
#104169=CARTESIAN_POINT('Ctrl Pts',(-0.350911661,3.138525418,7.491786236));
#104170=CARTESIAN_POINT('Ctrl Pts',(-0.110602232,3.176642188,7.503042214));
#104171=CARTESIAN_POINT('Ctrl Pts',(0.129934559,3.214285714,7.498874383));
#104172=CARTESIAN_POINT('Ctrl Pts',(0.301105915,3.241073689,7.495908461));
#104173=CARTESIAN_POINT('Ctrl Pts',(0.471963657,3.268112745,7.48513529));
#104174=CARTESIAN_POINT('Ctrl Pts',(-0.576538527796137,3.13852541819795,
7.22703973509604));
#104175=CARTESIAN_POINT('Ctrl Pts',(-0.421594524022473,3.16400222467753,
7.23940042350238));
#104176=CARTESIAN_POINT('Ctrl Pts',(-0.266654323353934,3.18928040268826,
7.24674125354813));
#104177=CARTESIAN_POINT('Ctrl Pts',(-0.112195259170487,3.21428571394946,
7.24913182614134));
#104178=CARTESIAN_POINT('Ctrl Pts',(-0.00374194548841267,3.23184317462932,
7.25081036419421));
#104179=CARTESIAN_POINT('Ctrl Pts',(0.105023642990151,3.24953506292902,
7.25005811714051));
#104180=CARTESIAN_POINT('Ctrl Pts',(0.213937950775892,3.26733592562386,
7.24684279936316));
#104181=CARTESIAN_POINT('Ctrl Pts',(0.209418136,2.750764179,7.24697482));
#104182=CARTESIAN_POINT('Ctrl Pts',(0.602103436,2.686419405,7.23562726800001));
#104183=CARTESIAN_POINT('Ctrl Pts',(0.991263375,2.621296797,7.181914572));
#104184=CARTESIAN_POINT('Ctrl Pts',(-0.029340091,2.750764179,7.49994261));
#104185=CARTESIAN_POINT('Ctrl Pts',(0.377052547,2.686419405,7.501532435));
#104186=CARTESIAN_POINT('Ctrl Pts',(0.781237513,2.621296797,7.459200222));
#104187=CARTESIAN_POINT('',(0.220796265851338,2.71105259873596,7.49674922941056));
#104188=CARTESIAN_POINT('',(0.78123750409061,2.62129679635371,7.45920022219058));
#104189=CARTESIAN_POINT('Origin',(-0.0306335706061751,2.55359536576098,
-0.188118757216246));
#104190=CARTESIAN_POINT('',(0.886250432112382,2.62129679507543,7.32055739843915));
#104191=CARTESIAN_POINT('Ctrl Pts',(0.220796264044513,2.7110525987386,7.49674922945498));
#104192=CARTESIAN_POINT('Ctrl Pts',(0.21978045853249,2.71723336186804,7.45505532086205));
#104193=CARTESIAN_POINT('Ctrl Pts',(0.218715591035989,2.72356451335006,
7.41336050560342));
#104194=CARTESIAN_POINT('Ctrl Pts',(0.216481064139124,2.73653622859594,
7.3300712036522));
#104195=CARTESIAN_POINT('Ctrl Pts',(0.215310080965755,2.74318451391785,
7.28842710414731));
#104196=CARTESIAN_POINT('Ctrl Pts',(0.214081499284118,2.74999999976668,
7.24683856077415));
#104197=CARTESIAN_POINT('Ctrl Pts',(0.973607978338463,2.61844385667099,
7.1840212125146));
#104198=CARTESIAN_POINT('Ctrl Pts',(0.982251746853771,2.61987032683551,
7.18282857737324));
#104199=CARTESIAN_POINT('Ctrl Pts',(0.990895515369072,2.621296797,7.18163594223189));
#104200=CARTESIAN_POINT('Ctrl Pts',(1.16527946970092,2.65007516,7.15757509057275));
#104201=CARTESIAN_POINT('Ctrl Pts',(1.33829010954023,2.678571429,7.12507882876051));
#104202=CARTESIAN_POINT('Ctrl Pts',(1.56242740907838,2.71548867740086,7.0829795422579));
#104203=CARTESIAN_POINT('Ctrl Pts',(1.78347548629995,2.75286253809926,7.02687582964737));
#104204=CARTESIAN_POINT('Ctrl Pts',(1.25075524478722,2.61844385667099,7.3949940680899));
#104205=CARTESIAN_POINT('Ctrl Pts',(1.25965213439361,2.61987032683551,7.39346725104492));
#104206=CARTESIAN_POINT('Ctrl Pts',(1.268549024,2.621296797,7.391940434));
#104207=CARTESIAN_POINT('Ctrl Pts',(1.448039577,2.65007516,7.36113762));
#104208=CARTESIAN_POINT('Ctrl Pts',(1.625823574,2.678571429,7.321659491));
#104209=CARTESIAN_POINT('Ctrl Pts',(1.85614481325012,2.71548867740086,7.27051511554235));
#104210=CARTESIAN_POINT('Ctrl Pts',(2.08279609425964,2.75286253809926,7.20499551915523));
#104211=CARTESIAN_POINT('',(1.2685490159974,2.62129679728566,7.39194043464768));
#104212=CARTESIAN_POINT('',(1.82721365441677,2.71105259873355,7.274014727662));
#104213=CARTESIAN_POINT('Ctrl Pts',(1.26854901542751,2.62129679564634,7.3919404353506));
#104214=CARTESIAN_POINT('Ctrl Pts',(1.38846606602389,2.64052352569893,7.3713611762831));
#104215=CARTESIAN_POINT('Ctrl Pts',(1.50762429264484,2.65962575012036,7.34790643424406));
#104216=CARTESIAN_POINT('Ctrl Pts',(1.62582357463579,2.67857142910191,7.32165949085882));
#104217=CARTESIAN_POINT('Ctrl Pts',(1.69306819243097,2.68934979355907,7.30672737260246));
#104218=CARTESIAN_POINT('Ctrl Pts',(1.76021149589615,2.700178795349,7.29084549616751));
#104219=CARTESIAN_POINT('Ctrl Pts',(1.8272136579073,2.71105259956491,7.27401472665962));
#104220=CARTESIAN_POINT('Ctrl Pts',(1.76693247010815,2.74999999878156,7.03139031416154));
#104221=CARTESIAN_POINT('Ctrl Pts',(1.77707263608141,2.74318451273276,7.0717424329524));
#104222=CARTESIAN_POINT('Ctrl Pts',(1.78716849160209,2.7365362282126,7.11216118490206));
#104223=CARTESIAN_POINT('Ctrl Pts',(1.80725542865157,2.72356456848111,7.19302252591549));
#104224=CARTESIAN_POINT('Ctrl Pts',(1.81725845691741,2.7172334745408,7.23351322974473));
#104225=CARTESIAN_POINT('Ctrl Pts',(1.82721365293153,2.71105259873601,7.27401472802745));
#104226=CARTESIAN_POINT('',(1.12851976597305,2.62129679787127,7.28587737450813));
#104227=CARTESIAN_POINT('Origin',(-6.51605505663788E-14,2.71213386199978,
-4.91794105439425E-13));
#104228=CARTESIAN_POINT('',(1.82013710546422,2.53084202099703,7.27578867997899));
#104229=CARTESIAN_POINT('Origin',(-0.043300880352663,2.55357150927427,-0.188109139924416));
#104230=CARTESIAN_POINT('',(2.36648016134961,2.62129679635371,7.11686529608004));
#104231=CARTESIAN_POINT('Origin',(-0.0266746806644327,2.41079133695599,
-0.185773302817498));
#104232=CARTESIAN_POINT('Origin',(-0.0703573078924483,2.55359539449515,
-0.177135215677642));
#104233=CARTESIAN_POINT('Ctrl Pts',(1.762407424,2.750764179,7.032525867));
#104234=CARTESIAN_POINT('Ctrl Pts',(2.143472571,2.686419405,6.937027883));
#104235=CARTESIAN_POINT('Ctrl Pts',(2.511987525,2.621296797,6.800913077));
#104236=CARTESIAN_POINT('Ctrl Pts',(1.583611829,2.750764179,7.330905372));
#104237=CARTESIAN_POINT('Ctrl Pts',(1.980844998,2.686419405,7.245095624));
#104238=CARTESIAN_POINT('Ctrl Pts',(2.36648017,2.621296797,7.11686529400001));
#104239=CARTESIAN_POINT('',(2.43923383619956,2.62129679507541,6.95888918946105));
#104240=CARTESIAN_POINT('Ctrl Pts',(2.4951977760081,2.61844385818249,6.80676585075237));
#104241=CARTESIAN_POINT('Ctrl Pts',(2.50338307239038,2.61987032759123,6.80374294562012));
#104242=CARTESIAN_POINT('Ctrl Pts',(2.51156836877267,2.621296797,6.80072004048786));
#104243=CARTESIAN_POINT('Ctrl Pts',(2.67670295147414,2.65007516,6.73973432240921));
#104244=CARTESIAN_POINT('Ctrl Pts',(2.83868296268772,2.678571429,6.67080563183334));
#104245=CARTESIAN_POINT('Ctrl Pts',(3.04852995024692,2.71548867657569,6.58150771068758));
#104246=CARTESIAN_POINT('Ctrl Pts',(3.25234940257738,2.75286253643016,6.47919687125863));
#104247=CARTESIAN_POINT('Ctrl Pts',(2.81121842139337,2.61844385818249,6.95322780681343));
#104248=CARTESIAN_POINT('Ctrl Pts',(2.81957908169667,2.61987032759123,6.9498241194067));
#104249=CARTESIAN_POINT('Ctrl Pts',(2.827939742,2.621296797,6.94642043200001));
#104250=CARTESIAN_POINT('Ctrl Pts',(2.996612211,2.65007516,6.877752607));
#104251=CARTESIAN_POINT('Ctrl Pts',(3.161753086,2.678571429,6.800979152));
#104252=CARTESIAN_POINT('Ctrl Pts',(3.37569500904041,2.71548867657569,6.70151824740522));
#104253=CARTESIAN_POINT('Ctrl Pts',(3.58296252864191,2.75286253643016,6.5888071390405));
#104254=CARTESIAN_POINT('',(2.82793973434138,2.62129679728565,6.94642043436071));
#104255=CARTESIAN_POINT('',(3.34819256234123,2.71105259871154,6.71115538203994));
#104256=CARTESIAN_POINT('Ctrl Pts',(2.82793973391823,2.62129679564642,6.94642043516145));
#104257=CARTESIAN_POINT('Ctrl Pts',(2.94062925804215,2.64052352569915,6.90054368625749));
#104258=CARTESIAN_POINT('Ctrl Pts',(3.051959555225,2.65962575012078,6.85202180692739));
#104259=CARTESIAN_POINT('Ctrl Pts',(3.16175308677398,2.67857142917795,6.80097915141693));
#104260=CARTESIAN_POINT('Ctrl Pts',(3.22421559883867,2.6893497936752,6.77194053245832));
#104261=CARTESIAN_POINT('Ctrl Pts',(3.2863749950427,2.70017879535709,6.74199614030809));
#104262=CARTESIAN_POINT('Ctrl Pts',(3.34819256604841,2.71105259960124,6.71115538033925));
#104263=CARTESIAN_POINT('Ctrl Pts',(3.23716364257135,2.74999999863177,6.4871620652196));
#104264=CARTESIAN_POINT('Ctrl Pts',(3.25574124978409,2.74318451259148,6.52439093806489));
#104265=CARTESIAN_POINT('Ctrl Pts',(3.2742899063226,2.73653622817571,6.56169441112101));
#104266=CARTESIAN_POINT('Ctrl Pts',(3.31129000836468,2.72356457243949,6.6363471384988));
#104267=CARTESIAN_POINT('Ctrl Pts',(3.32976346291393,2.71723348259965,6.67374081089451));
#104268=CARTESIAN_POINT('Ctrl Pts',(3.34819256082344,2.7110525987141,6.71115538278798));
#104269=CARTESIAN_POINT('',(2.66838386743254,2.62129679787125,6.87293921965941));
#104270=CARTESIAN_POINT('Origin',(-2.45897052719712E-13,2.71213386199967,
-5.34294830600857E-13));
#104271=CARTESIAN_POINT('',(3.34166280795518,2.53084202104404,6.71440910846402));
#104272=CARTESIAN_POINT('Origin',(-0.0827265554844064,2.55357150385517,
-0.174403115639424));
#104273=CARTESIAN_POINT('',(3.84106883469457,2.6212967963465,6.44175365808321));
#104274=CARTESIAN_POINT('Origin',(-0.0659866317829577,2.41079129086726,
-0.17569542402967));
#104275=CARTESIAN_POINT('Origin',(-0.106791213493976,2.55359538133709,-0.157869104366971));
#104276=CARTESIAN_POINT('Ctrl Pts',(3.232988499,2.750764179,6.489243821));
#104277=CARTESIAN_POINT('Ctrl Pts',(3.584615312,2.686419405,6.314060784));
#104278=CARTESIAN_POINT('Ctrl Pts',(3.91525393,2.621296797,6.101908444));
#104279=CARTESIAN_POINT('Ctrl Pts',(3.122515819,2.750764179,6.819083146));
#104280=CARTESIAN_POINT('Ctrl Pts',(3.492015338,2.686419405,6.649886193));
#104281=CARTESIAN_POINT('Ctrl Pts',(3.841068843,2.621296797,6.44175365400001));
#104282=CARTESIAN_POINT('',(3.87816137631514,2.62129679507539,6.27183105529777));
#104283=CARTESIAN_POINT('Ctrl Pts',(3.90011488472912,2.6184438573276,6.11123368563928));
#104284=CARTESIAN_POINT('Ctrl Pts',(3.90745898043263,2.61987032716382,6.10652185619153));
#104285=CARTESIAN_POINT('Ctrl Pts',(3.91480307613613,2.621296797,6.10181002674376));
#104286=CARTESIAN_POINT('Ctrl Pts',(4.06296677837533,2.65007516,6.00675106734493));
#104287=CARTESIAN_POINT('Ctrl Pts',(4.20634215577609,2.678571429,5.90461297703037));
#104288=CARTESIAN_POINT('Ctrl Pts',(4.3920866264194,2.71548867704315,5.77229189108124));
#104289=CARTESIAN_POINT('Ctrl Pts',(4.5691470888706,2.75286253737571,5.62855786246398));
#104290=CARTESIAN_POINT('Ctrl Pts',(4.24023213436743,2.6184438573276,6.18633634586204));
#104291=CARTESIAN_POINT('Ctrl Pts',(4.24766563718371,2.61987032716382,6.18121493843102));
#104292=CARTESIAN_POINT('Ctrl Pts',(4.25509914,2.621296797,6.176093531));
#104293=CARTESIAN_POINT('Ctrl Pts',(4.405066589,2.65007516,6.072771527));
#104294=CARTESIAN_POINT('Ctrl Pts',(4.549842538,2.678571429,5.962292586));
#104295=CARTESIAN_POINT('Ctrl Pts',(4.7374014663965,2.71548867704315,5.81916583099209));
#104296=CARTESIAN_POINT('Ctrl Pts',(4.91559363147713,2.75286253737572,5.66453345430643));
#104297=CARTESIAN_POINT('',(4.25509913306813,2.62129679728565,6.17609353496064));
#104298=CARTESIAN_POINT('',(4.71261370775416,2.71105259867233,5.83448986989362));
#104299=CARTESIAN_POINT('Ctrl Pts',(4.25509913278686,2.62129679564643,6.17609353582486));
#104300=CARTESIAN_POINT('Ctrl Pts',(4.35529189432767,2.64052352569895,6.107064443424));
#104301=CARTESIAN_POINT('Ctrl Pts',(4.45358858142186,2.65962575012078,6.0357442557464));
#104302=CARTESIAN_POINT('Ctrl Pts',(4.54984253890747,2.67857142917862,5.9622925853075));
#104303=CARTESIAN_POINT('Ctrl Pts',(4.60460226774719,2.68934979366353,5.92050527950756));
#104304=CARTESIAN_POINT('Ctrl Pts',(4.65887125227467,2.70017879533289,5.8778985378832));
#104305=CARTESIAN_POINT('Ctrl Pts',(4.71261371105953,2.71105259956698,5.83448986743041));
#104306=CARTESIAN_POINT('Ctrl Pts',(4.55602864061065,2.74999999872861,5.63960132741109));
#104307=CARTESIAN_POINT('Ctrl Pts',(4.58217502072053,2.74318451267426,5.67196617370914));
#104308=CARTESIAN_POINT('Ctrl Pts',(4.60830916400747,2.73653622822078,5.70441009965228));
#104309=CARTESIAN_POINT('Ctrl Pts',(4.66049235264123,2.72356457274487,5.76936355819353));
#104310=CARTESIAN_POINT('Ctrl Pts',(4.68657244090915,2.71723348320718,5.80191173891234));
#104311=CARTESIAN_POINT('Ctrl Pts',(4.71261370641489,2.71105259867639,5.83448987095173));
#104312=CARTESIAN_POINT('',(4.08347730449991,2.62129679787124,6.13863006502524));
#104313=CARTESIAN_POINT('Origin',(-5.5120838449163E-13,2.71213386200022,
-7.7715611723761E-13));
#104314=CARTESIAN_POINT('',(4.706936069564,2.53084202106156,5.8390712305403));
#104315=CARTESIAN_POINT('Origin',(-0.118283871844512,2.55357148116036,-0.152541779600568));
#104316=CARTESIAN_POINT('',(5.1360534000227,2.62129679635372,5.46543277858561));
#104317=CARTESIAN_POINT('Origin',(-0.102213261879857,2.41079127246662,-0.157402635827827));
#104318=CARTESIAN_POINT('Origin',(-0.138231744102897,2.55359539255566,-0.131221323923163));
#104319=CARTESIAN_POINT('Ctrl Pts',(4.552398626,2.750764179,5.642531945));
#104320=CARTESIAN_POINT('Ctrl Pts',(4.858145424,2.686419405,5.39585522));
#104321=CARTESIAN_POINT('Ctrl Pts',(5.135447414,2.621296797,5.117585355));
#104322=CARTESIAN_POINT('Ctrl Pts',(4.51541444,2.750764179,5.988408172));
#104323=CARTESIAN_POINT('Ctrl Pts',(4.839902922,2.686419405,5.743735475));
#104324=CARTESIAN_POINT('Ctrl Pts',(5.136053407,2.621296797,5.465432773));
#104325=CARTESIAN_POINT('',(5.13575040190729,2.62129679507543,5.29150907233978));
#104326=CARTESIAN_POINT('Ctrl Pts',(5.12266696414755,2.6184438576685,5.12994702347875));
#104327=CARTESIAN_POINT('Ctrl Pts',(5.12882645412125,2.61987032733427,5.12376659120871));
#104328=CARTESIAN_POINT('Ctrl Pts',(5.13498594409497,2.621296797,5.11758615893868));
#104329=CARTESIAN_POINT('Ctrl Pts',(5.25925079361522,2.65007516,4.99289880831642));
#104330=CARTESIAN_POINT('Ctrl Pts',(5.37731746396822,2.678571429,4.86232718154151));
#104331=CARTESIAN_POINT('Ctrl Pts',(5.53027420987107,2.71548867689151,4.69317011968511));
#104332=CARTESIAN_POINT('Ctrl Pts',(5.67229652933867,2.75286253706899,4.51473374810968));
#104333=CARTESIAN_POINT('Ctrl Pts',(5.47097731265819,2.6184438576685,5.13017866966202));
#104334=CARTESIAN_POINT('Ctrl Pts',(5.47713607232912,2.61987032733427,5.12357901533102));
#104335=CARTESIAN_POINT('Ctrl Pts',(5.483294832,2.621296797,5.11697936100001));
#104336=CARTESIAN_POINT('Ctrl Pts',(5.607544948,2.65007516,4.9838344));
#104337=CARTESIAN_POINT('Ctrl Pts',(5.72518641,2.678571429,4.844815845));
#104338=CARTESIAN_POINT('Ctrl Pts',(5.87759229249829,2.71548867689151,4.66471569004545));
#104339=CARTESIAN_POINT('Ctrl Pts',(6.01837703291872,2.75286253706899,4.47539248510704));
#104340=CARTESIAN_POINT('',(5.48329482857351,2.62129679727529,5.11697936459));
#104341=CARTESIAN_POINT('',(5.8566782740463,2.71105259871343,4.68501009565352));
#104342=CARTESIAN_POINT('Ctrl Pts',(5.48329482599272,2.62129679564642,5.11697936726269));
#104343=CARTESIAN_POINT('Ctrl Pts',(5.56630592160011,2.64052352569898,5.02802565495659));
#104344=CARTESIAN_POINT('Ctrl Pts',(5.64697275466975,2.65962575012044,4.93724201144345));
#104345=CARTESIAN_POINT('Ctrl Pts',(5.72518641047971,2.6785714291162,4.84481584443312));
#104346=CARTESIAN_POINT('Ctrl Pts',(5.76968285161177,2.68934979357867,4.79223377992844));
#104347=CARTESIAN_POINT('Ctrl Pts',(5.8135238678287,2.70017879536078,4.73895693236883));
#104348=CARTESIAN_POINT('Ctrl Pts',(5.85667827678894,2.71105259961095,4.68501009253177));
#104349=CARTESIAN_POINT('Ctrl Pts',(5.66185880256267,2.74999999874769,4.52833910004848));
#104350=CARTESIAN_POINT('Ctrl Pts',(5.69435138006959,2.74318451271068,4.55432657530881));
#104351=CARTESIAN_POINT('Ctrl Pts',(5.72684900677654,2.73653622824737,4.58039391203204));
#104352=CARTESIAN_POINT('Ctrl Pts',(5.79177555439265,2.72356451299752,4.63261119234889));
#104353=CARTESIAN_POINT('Ctrl Pts',(5.82424314025865,2.71723336167496,4.6587922416216));
#104354=CARTESIAN_POINT('Ctrl Pts',(5.85667827296397,2.711052598716,4.68501009699311));
#104355=CARTESIAN_POINT('',(5.30763188220032,2.62129679787124,5.11728539181767));
#104356=CARTESIAN_POINT('Origin',(1.64928834478495E-12,2.71213386199944,
1.26157764790413E-12));
#104357=CARTESIAN_POINT('',(5.85211823264317,2.53084202101063,4.69070487109297));
#104358=CARTESIAN_POINT('Origin',(-0.148310339986101,2.5535715273533,-0.123547826992701));
#104359=CARTESIAN_POINT('',(6.19088181638272,2.62129679635371,4.23355433693757));
#104360=CARTESIAN_POINT('Origin',(-0.133660426319354,2.4107913065854,-0.131749774071899));
#104361=CARTESIAN_POINT('Origin',(-0.163208568664093,2.55359543573746,-0.0984376405150228));
#104362=CARTESIAN_POINT('Ctrl Pts',(5.658943652,2.750764179,4.531981548));
#104363=CARTESIAN_POINT('Ctrl Pts',(5.90451405500001,2.686419405,4.225345463));
#104364=CARTESIAN_POINT('Ctrl Pts',(6.115513083,2.621296797,3.893969662));
#104365=CARTESIAN_POINT('Ctrl Pts',(5.69717730100001,2.750764179,4.877721886));
#104366=CARTESIAN_POINT('Ctrl Pts',(5.961482025,2.686419405,4.56901407));
#104367=CARTESIAN_POINT('Ctrl Pts',(6.190881822,2.621296797,4.23355433));
#104368=CARTESIAN_POINT('',(6.15319744590099,2.62129679507543,4.06376200599198));
#104369=CARTESIAN_POINT('Ctrl Pts',(6.10568883044446,2.61844385890977,3.908789733995));
#104370=CARTESIAN_POINT('Ctrl Pts',(6.11037570273752,2.61987032795487,3.90142969174084));
#104371=CARTESIAN_POINT('Ctrl Pts',(6.11506257503053,2.621296797,3.89406964948668));
#104372=CARTESIAN_POINT('Ctrl Pts',(6.20961808792042,2.65007516,3.74558415068812));
#104373=CARTESIAN_POINT('Ctrl Pts',(6.29685538488361,2.678571429,3.5926843721594));
#104374=CARTESIAN_POINT('Ctrl Pts',(6.40987231768519,2.71548867633322,3.39460093130149));
#104375=CARTESIAN_POINT('Ctrl Pts',(6.51021568666705,2.75286253593971,3.18980570664055));
#104376=CARTESIAN_POINT('Ctrl Pts',(6.44590567465352,2.61844385890977,3.83413953496176));
#104377=CARTESIAN_POINT('Ctrl Pts',(6.45050171332678,2.61987032795487,3.82637022898089));
#104378=CARTESIAN_POINT('Ctrl Pts',(6.455097752,2.621296797,3.818600923));
#104379=CARTESIAN_POINT('Ctrl Pts',(6.54782073800001,2.65007516,3.661858715));
#104380=CARTESIAN_POINT('Ctrl Pts',(6.632826928,2.678571429,3.5008009));
#104381=CARTESIAN_POINT('Ctrl Pts',(6.74295343410217,2.71548867633322,3.29214863009078));
#104382=CARTESIAN_POINT('Ctrl Pts',(6.83974781229092,2.75286253593971,3.07698714219965));
#104383=CARTESIAN_POINT('',(6.45509774941754,2.62129679727529,3.81860092724444));
#104384=CARTESIAN_POINT('',(6.72689107318539,2.71105259873439,3.31646445626091));
#104385=CARTESIAN_POINT('Ctrl Pts',(6.45509774747939,2.62129679564641,3.81860093040773));
#104386=CARTESIAN_POINT('Ctrl Pts',(6.51704567080351,2.6405235256991,3.71388197465405));
#104387=CARTESIAN_POINT('Ctrl Pts',(6.57631075817407,2.65962575012053,3.60787981774369));
#104388=CARTESIAN_POINT('Ctrl Pts',(6.63282692833652,2.67857142913362,3.50080089926179));
#104389=CARTESIAN_POINT('Ctrl Pts',(6.66497947777494,2.68934979361287,3.43988275458253));
#104390=CARTESIAN_POINT('Ctrl Pts',(6.69634256801951,2.7001787953686,3.37842696767933));
#104391=CARTESIAN_POINT('Ctrl Pts',(6.72689107500102,2.71105259961325,3.31646445271963));
#104392=CARTESIAN_POINT('Ctrl Pts',(6.50294674033191,2.74999999863963,3.20533676975677));
#104393=CARTESIAN_POINT('Ctrl Pts',(6.54026619870976,2.74318451256571,3.22373172851576));
#104394=CARTESIAN_POINT('Ctrl Pts',(6.57760775536954,2.73653622819314,3.24220359592826));
#104395=CARTESIAN_POINT('Ctrl Pts',(6.65224119207437,2.7235645713651,3.27924260980075));
#104396=CARTESIAN_POINT('Ctrl Pts',(6.68957747437631,2.71723348043905,3.29783179808093));
#104397=CARTESIAN_POINT('Ctrl Pts',(6.72689107244661,2.71105259873694,3.31646445774123));
#104398=CARTESIAN_POINT('',(6.28360749135913,2.62129679787126,3.85666214075026));
#104399=CARTESIAN_POINT('Origin',(7.74987712892639E-13,2.71213386200022,
3.90746462963776E-13));
#104400=CARTESIAN_POINT('',(6.72366185127617,2.53084202102611,3.32300636522807));
#104401=CARTESIAN_POINT('Origin',(-0.171402024182553,2.55357154600533,-0.0887769892027829));
#104402=CARTESIAN_POINT('',(6.9562314790131,2.62129679635372,2.80371959999944));
#104403=CARTESIAN_POINT('Origin',(-0.158857905554866,2.41079127488136,-0.0999365371658045));
#104404=CARTESIAN_POINT('Origin',(-0.18055420549716,2.55359536942784,-0.0610512706728089));
#104405=CARTESIAN_POINT('Ctrl Pts',(6.500882762,2.750764179,3.209520729));
#104406=CARTESIAN_POINT('Ctrl Pts',(6.674794172,2.686419405,2.857263248));
#104407=CARTESIAN_POINT('Ctrl Pts',(6.809624158,2.621296797,2.488276275));
#104408=CARTESIAN_POINT('Ctrl Pts',(6.612546483,2.750764179,3.538958747));
#104409=CARTESIAN_POINT('Ctrl Pts',(6.804308854,2.686419405,3.180650644));
#104410=CARTESIAN_POINT('Ctrl Pts',(6.956231483,2.621296797,2.803719592));
#104411=CARTESIAN_POINT('',(6.88292781620325,2.62129679507543,2.64599794467697));
#104412=CARTESIAN_POINT('Ctrl Pts',(6.80321546550788,2.61844385762072,2.50486179331884));
#104413=CARTESIAN_POINT('Ctrl Pts',(6.80621057117267,2.61987032731036,2.496666282065));
#104414=CARTESIAN_POINT('Ctrl Pts',(6.8092056768374,2.621296797,2.48847077081115));
#104415=CARTESIAN_POINT('Ctrl Pts',(6.86963054157133,2.65007516,2.3231301403394));
#104416=CARTESIAN_POINT('Ctrl Pts',(6.9219593459294,2.678571429,2.15505163367438));
#104417=CARTESIAN_POINT('Ctrl Pts',(6.98975192156349,2.71548867687936,1.93730397120084));
#104418=CARTESIAN_POINT('Ctrl Pts',(7.04372440045867,2.75286253704441,1.71572588267085));
#104419=CARTESIAN_POINT('Ctrl Pts',(7.11943064298699,2.61844385762072,2.35882031047265));
#104420=CARTESIAN_POINT('Ctrl Pts',(7.12224905899349,2.61987032731036,2.35024463023634));
#104421=CARTESIAN_POINT('Ctrl Pts',(7.125067475,2.621296797,2.34166895));
#104422=CARTESIAN_POINT('Ctrl Pts',(7.181927708,2.65007516,2.168658587));
#104423=CARTESIAN_POINT('Ctrl Pts',(7.230323831,2.678571429,1.993092396));
#104424=CARTESIAN_POINT('Ctrl Pts',(7.29302157140247,2.71548867687936,1.76564435329171));
#104425=CARTESIAN_POINT('Ctrl Pts',(7.34129959039367,2.75286253704441,1.53470528735004));
#104426=CARTESIAN_POINT('',(7.12506747340202,2.62129679727527,2.34166895469459));
#104427=CARTESIAN_POINT('',(7.28256192199589,2.71105259871254,1.79284462519801));
#104428=CARTESIAN_POINT('Ctrl Pts',(7.12506747217799,2.62129679564649,2.34166895820572));
#104429=CARTESIAN_POINT('Ctrl Pts',(7.1630556076896,2.64052352569902,2.22608130136333));
#104430=CARTESIAN_POINT('Ctrl Pts',(7.19814777998631,2.65962575012048,2.10981717414423));
#104431=CARTESIAN_POINT('Ctrl Pts',(7.23032383120981,2.67857142912354,1.99309239523888));
#104432=CARTESIAN_POINT('Ctrl Pts',(7.24862907160098,2.68934979359008,1.92668663526634));
#104433=CARTESIAN_POINT('Ctrl Pts',(7.26604773257138,2.70017879536209,1.85992551309353));
#104434=CARTESIAN_POINT('Ctrl Pts',(7.28256192321581,2.7110525996155,1.79284462117634));
#104435=CARTESIAN_POINT('Ctrl Pts',(7.03996411563262,2.74999999865509,1.73245645342098));
#104436=CARTESIAN_POINT('Ctrl Pts',(7.08036543800852,2.74318451258415,1.74239876792937));
#104437=CARTESIAN_POINT('Ctrl Pts',(7.12080487551331,2.73653622815888,1.75241144266083));
#104438=CARTESIAN_POINT('Ctrl Pts',(7.20165608093836,2.72356451293218,1.7725406130909));
#104439=CARTESIAN_POINT('Ctrl Pts',(7.2421160008973,2.71723336163673,1.78266910448064));
#104440=CARTESIAN_POINT('Ctrl Pts',(7.28256192157163,2.71105259871514,1.79284462688592));
#104441=CARTESIAN_POINT('',(6.96576859816398,2.62129679787115,2.41570565417414));
#104442=CARTESIAN_POINT('Origin',(-7.2251232774434E-13,2.71213386199956,
-9.75781955236954E-14));
#104443=CARTESIAN_POINT('',(7.28081451506275,2.53084202101684,1.79992777426825));
#104444=CARTESIAN_POINT('Origin',(-0.18647930638377,2.55357153497555,-0.0498551051272444));
#104445=CARTESIAN_POINT('',(7.39631548980067,2.62129679635372,1.24278605063635));
#104446=CARTESIAN_POINT('Origin',(-0.176627145807934,2.41079128197683,-0.0634502949292973));
#104447=CARTESIAN_POINT('Origin',(-0.189457227616135,2.55359537483203,-0.0208101339617175));
#104448=CARTESIAN_POINT('Ctrl Pts',(7.03884782,2.750764179,1.736986289));
#104449=CARTESIAN_POINT('Ctrl Pts',(7.132968332,2.686419405,1.35557858));
#104450=CARTESIAN_POINT('Ctrl Pts',(7.185324776,2.621296797,0.966233856));
#104451=CARTESIAN_POINT('Ctrl Pts',(7.21872034000001,2.750764179,2.03471783));
#104452=CARTESIAN_POINT('Ctrl Pts',(7.328973763,2.686419405,1.64356353));
#104453=CARTESIAN_POINT('Ctrl Pts',(7.396315492,2.621296797,1.242786042));
#104454=CARTESIAN_POINT('',(7.29082013220642,2.62129679507543,1.10450996083933));
#104455=CARTESIAN_POINT('Ctrl Pts',(7.18263131216403,2.61844385838297,0.983809288891911));
#104456=CARTESIAN_POINT('Ctrl Pts',(7.18379460089475,2.61987032769149,0.97516152725879));
#104457=CARTESIAN_POINT('Ctrl Pts',(7.18495788962543,2.621296797,0.96651376562567));
#104458=CARTESIAN_POINT('Ctrl Pts',(7.20842670536899,2.65007516,0.792049147333845));
#104459=CARTESIAN_POINT('Ctrl Pts',(7.22340018149012,2.678571429,0.616651075659592));
#104460=CARTESIAN_POINT('Ctrl Pts',(7.24279849383286,2.71548867651787,0.389420835413089));
#104461=CARTESIAN_POINT('Ctrl Pts',(7.24787638617303,2.75286253631321,0.161420634597048));
#104462=CARTESIAN_POINT('Ctrl Pts',(7.46005895192977,2.61844385838297,0.773205258737892));
#104463=CARTESIAN_POINT('Ctrl Pts',(7.46096795696486,2.61987032769149,0.764224199368948));
#104464=CARTESIAN_POINT('Ctrl Pts',(7.461876962,2.621296797,0.75524314));
#104465=CARTESIAN_POINT('Ctrl Pts',(7.480215721,2.65007516,0.574054393));
#104466=CARTESIAN_POINT('Ctrl Pts',(7.489738828,2.678571429,0.392189107));
#104467=CARTESIAN_POINT('Ctrl Pts',(7.50207612295756,2.71548867651787,0.15658051345081));
#104468=CARTESIAN_POINT('Ctrl Pts',(7.4995803569868,2.75286253631321,-0.0793376696427069));
#104469=CARTESIAN_POINT('Ctrl Pts',(7.24780059325685,2.7499999986265,0.178568399451582));
#104470=CARTESIAN_POINT('Ctrl Pts',(7.28939465910201,2.7431845125398,0.179593178039138));
#104471=CARTESIAN_POINT('Ctrl Pts',(7.33104107381993,2.73653622816585,0.180678478153405));
#104472=CARTESIAN_POINT('Ctrl Pts',(7.41432882964981,2.7235645705627,0.182956410170129));
#104473=CARTESIAN_POINT('Ctrl Pts',(7.45601972471698,2.71723347887198,0.184150402700255));
#104474=CARTESIAN_POINT('Ctrl Pts',(7.49770826955607,2.71105259871467,0.185393373255831));
#104475=CARTESIAN_POINT('',(7.32221810744534,2.62129679787114,0.861793456887462));
#104476=CARTESIAN_POINT('Ctrl Pts',(7.247684177,2.750764179,0.183232301));
#104477=CARTESIAN_POINT('Ctrl Pts',(7.25761282,2.686419405,-0.209491436));
#104478=CARTESIAN_POINT('Ctrl Pts',(7.22504759300001,2.621296797,-0.600988584999999));
#104479=CARTESIAN_POINT('Ctrl Pts',(7.487354858,2.750764179,0.435335768));
#104480=CARTESIAN_POINT('Ctrl Pts',(7.510944005,2.686419405,0.029625212));
#104481=CARTESIAN_POINT('Ctrl Pts',(7.490556008,2.621296797,-0.376258802));
#104482=CARTESIAN_POINT('',(7.35780180129346,2.62129679507543,-0.488623681551902));
#104483=CARTESIAN_POINT('Ctrl Pts',(7.22619529940868,2.61844385851179,-0.583245041761979));
#104484=CARTESIAN_POINT('Ctrl Pts',(7.22547237799634,2.61987032775589,-0.591940695809489));
#104485=CARTESIAN_POINT('Ctrl Pts',(7.22474945658406,2.621296797,-0.600636349857002));
#104486=CARTESIAN_POINT('Ctrl Pts',(7.21016484853215,2.65007516,-0.776067183529233));
#104487=CARTESIAN_POINT('Ctrl Pts',(7.18708285276207,2.678571429,-0.95058339985461));
#104488=CARTESIAN_POINT('Ctrl Pts',(7.15717985904099,2.71548867646293,-1.17667118689306));
#104489=CARTESIAN_POINT('Ctrl Pts',(7.11312572913838,2.75286253620207,-1.4004324670367));
#104490=CARTESIAN_POINT('Ctrl Pts',(7.45186319460198,2.61844385851179,-0.848564007989048));
#104491=CARTESIAN_POINT('Ctrl Pts',(7.45082028530099,2.61987032775589,-0.857530503994525));
#104492=CARTESIAN_POINT('Ctrl Pts',(7.44977737600001,2.621296797,-0.866497));
#104493=CARTESIAN_POINT('Ctrl Pts',(7.428737159,2.65007516,-1.047391946));
#104494=CARTESIAN_POINT('Ctrl Pts',(7.398941961,2.678571429,-1.227052509));
#104495=CARTESIAN_POINT('Ctrl Pts',(7.36034193449132,2.71548867646293,-1.45980485781117));
#104496=CARTESIAN_POINT('Ctrl Pts',(7.30718908296341,2.75286253620207,-1.6896708892753));
#104497=CARTESIAN_POINT('',(7.4497773762241,2.62129679728562,-0.866496991987696));
#104498=CARTESIAN_POINT('',(7.36227011168024,2.71105259872532,-1.43072666945356));
#104499=CARTESIAN_POINT('Ctrl Pts',(7.44977737688415,2.62129679564651,-0.866496991367734));
#104500=CARTESIAN_POINT('Ctrl Pts',(7.43572047689793,2.64052352569903,-0.987352312322432));
#104501=CARTESIAN_POINT('Ctrl Pts',(7.41875122985605,2.65962575012099,-1.10760559706222));
#104502=CARTESIAN_POINT('Ctrl Pts',(7.39894196064008,2.67857142921625,-1.22705251018873));
#104503=CARTESIAN_POINT('Ctrl Pts',(7.38767229163384,2.68934979373988,-1.29500691707787));
#104504=CARTESIAN_POINT('Ctrl Pts',(7.37544877285651,2.70017879536303,-1.36291157598306));
#104505=CARTESIAN_POINT('Ctrl Pts',(7.36227011098551,2.7110525996053,-1.43072667338086));
#104506=CARTESIAN_POINT('Ctrl Pts',(7.11673797052314,2.74999999867813,-1.38366931491681));
#104507=CARTESIAN_POINT('Ctrl Pts',(7.15757988738069,2.74318451260325,-1.39160998948805));
#104508=CARTESIAN_POINT('Ctrl Pts',(7.19848593954936,2.73653622822845,-1.39950281104339));
#104509=CARTESIAN_POINT('Ctrl Pts',(7.28031615690217,2.72356457142187,-1.41518254019115));
#104510=CARTESIAN_POINT('Ctrl Pts',(7.32128900927842,2.71723348055737,-1.4229787714934));
#104511=CARTESIAN_POINT('Ctrl Pts',(7.36227011198849,2.71105259872787,-1.43072666782516));
#104512=CARTESIAN_POINT('',(7.33628883611589,2.62129679787115,-0.732415245107293));
#104513=CARTESIAN_POINT('Origin',(3.75133951679985E-13,2.71213386199922,
-5.10659223240673E-14));
#104514=CARTESIAN_POINT('',(7.36365834535768,2.5308420210249,-1.42356445975565));
#104515=CARTESIAN_POINT('Origin',(-0.190177539396756,2.55357151332881,0.0330533513936276));
#104516=CARTESIAN_POINT('',(7.23454645265237,2.62129679635372,-1.97771019422671));
#104517=CARTESIAN_POINT('Origin',(-0.186944872904844,2.410791282204,0.0165779686647455));
#104518=CARTESIAN_POINT('Origin',(-0.180684632637054,2.55359539647965,0.0606642551306097));
#104519=CARTESIAN_POINT('Ctrl Pts',(7.117626877,2.750764179,-1.379089427));
#104520=CARTESIAN_POINT('Ctrl Pts',(7.042899399,2.686419405,-1.764765866));
#104521=CARTESIAN_POINT('Ctrl Pts',(6.926935215,2.621296797,-2.140109468));
#104522=CARTESIAN_POINT('Ctrl Pts',(7.405888984,2.750764179,-1.18440211));
#104523=CARTESIAN_POINT('Ctrl Pts',(7.341710853,2.686419405,-1.585698348));
#104524=CARTESIAN_POINT('Ctrl Pts',(7.234546451,2.621296797,-1.977710203));
#104525=CARTESIAN_POINT('',(7.0807408363434,2.62129679507543,-2.05890982400181));
#104526=CARTESIAN_POINT('Ctrl Pts',(6.9318704271471,2.61844385782496,-2.12302747772819));
#104527=CARTESIAN_POINT('Ctrl Pts',(6.92929509802686,2.61987032741248,-2.13136442748401));
#104528=CARTESIAN_POINT('Ctrl Pts',(6.92671976890657,2.621296797,-2.13970137723984));
#104529=CARTESIAN_POINT('Ctrl Pts',(6.87476369713584,2.65007516,-2.3078954757923));
#104530=CARTESIAN_POINT('Ctrl Pts',(6.81470551759715,2.678571429,-2.47336965345944));
#104531=CARTESIAN_POINT('Ctrl Pts',(6.7368994466319,2.71548867677546,-2.68774337481691));
#104532=CARTESIAN_POINT('Ctrl Pts',(6.64577321665464,2.75286253683425,-2.89680290696358));
#104533=CARTESIAN_POINT('Ctrl Pts',(7.09522659686887,2.61844385782496,-2.43065536060913));
#104534=CARTESIAN_POINT('Ctrl Pts',(7.09228053793441,2.61987032741248,-2.43918803230456));
#104535=CARTESIAN_POINT('Ctrl Pts',(7.089334479,2.621296797,-2.447720704));
#104536=CARTESIAN_POINT('Ctrl Pts',(7.029899105,2.65007516,-2.619863402));
#104537=CARTESIAN_POINT('Ctrl Pts',(6.962178791,2.678571429,-2.788918514));
#104538=CARTESIAN_POINT('Ctrl Pts',(6.87444633631865,2.71548867677546,-3.00793137901318));
#104539=CARTESIAN_POINT('Ctrl Pts',(6.77312176552132,2.75286253683425,-3.2209969797396));
#104540=CARTESIAN_POINT('',(7.08933448094888,2.62129679728562,-2.4477206962377));
#104541=CARTESIAN_POINT('',(6.88258038540553,2.71105259873557,-2.97994752197314));
#104542=CARTESIAN_POINT('Ctrl Pts',(7.08933448171907,2.62129679564653,-2.44772069575958));
#104543=CARTESIAN_POINT('Ctrl Pts',(7.04962590309123,2.64052352569907,-2.56272866850804));
#104544=CARTESIAN_POINT('Ctrl Pts',(7.00720248596634,2.65962575012069,-2.67652261175817));
#104545=CARTESIAN_POINT('Ctrl Pts',(6.9621787906131,2.67857142916281,-2.78891851496585));
#104546=CARTESIAN_POINT('Ctrl Pts',(6.93656441164756,2.68934979365771,-2.85286153970963));
#104547=CARTESIAN_POINT('Ctrl Pts',(6.910029177234,2.70017879535824,-2.91655093023377));
#104548=CARTESIAN_POINT('Ctrl Pts',(6.88258038384324,2.71105259958446,-2.97994752537253));
#104549=CARTESIAN_POINT('Ctrl Pts',(6.65290458943671,2.74999999865438,-2.88120818907132));
#104550=CARTESIAN_POINT('Ctrl Pts',(6.69108463438367,2.74318451262851,-2.89774302008144));
#104551=CARTESIAN_POINT('Ctrl Pts',(6.72933760273026,2.73653622821457,-2.91424490416687));
#104552=CARTESIAN_POINT('Ctrl Pts',(6.80588401007471,2.72356456917387,-2.94714913373006));
#104553=CARTESIAN_POINT('Ctrl Pts',(6.84422299606672,2.71723347594592,-2.96357105219085));
#104554=CARTESIAN_POINT('Ctrl Pts',(6.8825803860209,2.71105259873809,-2.97994752053274));
#104555=CARTESIAN_POINT('',(7.00732285234163,2.62129679787115,-2.29237702474075));
#104556=CARTESIAN_POINT('Origin',(5.00901403688303E-13,2.71213386200067,
-1.29453739394769E-13));
#104557=CARTESIAN_POINT('',(6.88547582676816,2.53084202099543,-2.97325118946033));
#104558=CARTESIAN_POINT('Origin',(-0.178625804802862,2.55357152389825,0.0731631300769686));
#104559=CARTESIAN_POINT('',(6.64025754551519,2.62129679635372,-3.48668606478277));
#104560=CARTESIAN_POINT('Origin',(-0.179010305405579,2.41079133936449,0.0563779573340922));
#104561=CARTESIAN_POINT('Origin',(-0.163419285777804,2.55359539665695,0.0980878048727796));
#104562=CARTESIAN_POINT('Ctrl Pts',(6.654757254,2.750764179,-2.876926465));
#104563=CARTESIAN_POINT('Ctrl Pts',(6.49886783,2.686419405,-3.237521805));
#104564=CARTESIAN_POINT('Ctrl Pts',(6.304927044,2.621296797,-3.57916121));
#104565=CARTESIAN_POINT('Ctrl Pts',(6.978131972,2.750764179,-2.748758662));
#104566=CARTESIAN_POINT('Ctrl Pts',(6.829187461,2.686419405,-3.126876416));
#104567=CARTESIAN_POINT('Ctrl Pts',(6.640257542,2.621296797,-3.486686073));
#104568=CARTESIAN_POINT('',(6.472592298737,2.62129679507543,-3.53292363098937));
#104569=CARTESIAN_POINT('Ctrl Pts',(6.31341899261438,2.61844385915646,-3.56353951913638));
#104570=CARTESIAN_POINT('Ctrl Pts',(6.30911167752144,2.61987032807824,-3.57112793249725));
#104571=CARTESIAN_POINT('Ctrl Pts',(6.3048043624285,2.621296797,-3.57871634585811));
#104572=CARTESIAN_POINT('Ctrl Pts',(6.21790623558622,2.65007516,-3.73180914091384));
#104573=CARTESIAN_POINT('Ctrl Pts',(6.12368012659908,2.678571429,-3.88050389076422));
#104574=CARTESIAN_POINT('Ctrl Pts',(6.00160910777752,2.71548867610496,-4.07313966510681));
#104575=CARTESIAN_POINT('Ctrl Pts',(5.86767174108176,2.75286253547799,-4.25772205181901));
#104576=CARTESIAN_POINT('Ctrl Pts',(6.40682508435585,2.61844385915646,-3.89909198129979));
#104577=CARTESIAN_POINT('Ctrl Pts',(6.40211363267789,2.61987032807824,-3.90679184464988));
#104578=CARTESIAN_POINT('Ctrl Pts',(6.397402181,2.621296797,-3.914491708));
#104579=CARTESIAN_POINT('Ctrl Pts',(6.302350782,2.65007516,-4.069832956));
#104580=CARTESIAN_POINT('Ctrl Pts',(6.199871879,2.678571429,-4.220377789));
#104581=CARTESIAN_POINT('Ctrl Pts',(6.06710927111963,2.71548867610496,-4.41541036735175));
#104582=CARTESIAN_POINT('Ctrl Pts',(5.92235080998031,2.75286253547799,-4.60171282101012));
#104583=CARTESIAN_POINT('',(6.39740218457622,2.62129679728566,-3.91449170085054));
#104584=CARTESIAN_POINT('',(6.08106885043357,2.71105259869766,-4.3898293404743));
#104585=CARTESIAN_POINT('Ctrl Pts',(6.39740218542778,2.62129679564633,-3.91449170053633));
#104586=CARTESIAN_POINT('Ctrl Pts',(6.33389865714133,2.64052352569892,-4.01827467958564));
#104587=CARTESIAN_POINT('Ctrl Pts',(6.26800474188442,2.65962575012044,-4.1202884031626));
#104588=CARTESIAN_POINT('Ctrl Pts',(6.1998718785814,2.6785714291164,-4.22037778961493));
#104589=CARTESIAN_POINT('Ctrl Pts',(6.16111048962537,2.68934979357377,-4.27731952756113));
#104590=CARTESIAN_POINT('Ctrl Pts',(6.12150429781491,2.70017879533987,-4.33381560487414));
#104591=CARTESIAN_POINT('Ctrl Pts',(6.08106884815002,2.7110525995626,-4.38982934357438));
#104592=CARTESIAN_POINT('Ctrl Pts',(5.87798878527351,2.7499999985941,-4.24402497176462));
#104593=CARTESIAN_POINT('Ctrl Pts',(5.91172170248899,2.7431845125011,-4.26838080871113));
#104594=CARTESIAN_POINT('Ctrl Pts',(5.94553291982931,2.73653622819684,-4.29272014485459));
#104595=CARTESIAN_POINT('Ctrl Pts',(6.0132162752591,2.72356456965486,-4.34131030473907));
#104596=CARTESIAN_POINT('Ctrl Pts',(6.04712868651706,2.71723347701746,-4.36559003416882));
#104597=CARTESIAN_POINT('Ctrl Pts',(6.08106885136474,2.71105259870017,-4.3898293391711));
#104598=CARTESIAN_POINT('',(6.35070223953008,2.62129679787127,-3.74514980190602));
#104599=CARTESIAN_POINT('Origin',(-4.18935719448399E-13,2.71213386200033,
3.29163779566599E-13));
#104600=CARTESIAN_POINT('',(6.0853361110207,2.53084202103016,-4.38391199843598));
#104601=CARTESIAN_POINT('Origin',(-0.158721868614637,2.55357153612414,0.10985197956607));
#104602=CARTESIAN_POINT('',(5.7354775761899,2.62129679635372,-4.83262836973105));
#104603=CARTESIAN_POINT('Origin',(-0.162705727064962,2.41079129892709,0.0935419213495575));
#104604=CARTESIAN_POINT('Origin',(-0.138512605094451,2.55359539186379,0.130924849469142));
#104605=CARTESIAN_POINT('Ctrl Pts',(5.880718579,2.750764179,-4.24024162));
#104606=CARTESIAN_POINT('Ctrl Pts',(5.650956424,2.686419405,-4.558894822));
#104607=CARTESIAN_POINT('Ctrl Pts',(5.388107493,2.621296797,-4.850855352));
#104608=CARTESIAN_POINT('Ctrl Pts',(6.224085265,2.750764179,-4.184586314));
#104609=CARTESIAN_POINT('Ctrl Pts',(5.997338854,2.686419405,-4.521845218));
#104610=CARTESIAN_POINT('Ctrl Pts',(5.735477571,2.621296797,-4.832628377));
#104611=CARTESIAN_POINT('',(5.56179253986235,2.62129679507543,-4.84174185546838));
#104612=CARTESIAN_POINT('Ctrl Pts',(5.39975910663828,2.61844385907082,-4.83742440510579));
#104613=CARTESIAN_POINT('Ctrl Pts',(5.39392120946597,2.61987032803543,-4.84390946034449));
#104614=CARTESIAN_POINT('Ctrl Pts',(5.38808331229366,2.621296797,-4.85039451558319));
#104615=CARTESIAN_POINT('Ctrl Pts',(5.27030639029006,2.65007516,-4.98122755742915));
#104616=CARTESIAN_POINT('Ctrl Pts',(5.14631825859592,2.678571429,-5.10619007807575));
#104617=CARTESIAN_POINT('Ctrl Pts',(4.98569019364608,2.71548867628975,-5.26808047573109));
#104618=CARTESIAN_POINT('Ctrl Pts',(4.81520445166271,2.75286253585177,-5.41955485476044));
#104619=CARTESIAN_POINT('Ctrl Pts',(5.41884755555708,2.61844385907083,-5.18521138563031));
#104620=CARTESIAN_POINT('Ctrl Pts',(5.41259101177851,2.61987032803543,-5.19171840781515));
#104621=CARTESIAN_POINT('Ctrl Pts',(5.406334468,2.621296797,-5.19822543));
#104622=CARTESIAN_POINT('Ctrl Pts',(5.280111541,2.65007516,-5.329501645));
#104623=CARTESIAN_POINT('Ctrl Pts',(5.147665849,2.678571429,-5.454496888));
#104624=CARTESIAN_POINT('Ctrl Pts',(4.97608091710626,2.71548867628975,-5.6164296779869));
#104625=CARTESIAN_POINT('Ctrl Pts',(4.79465730568439,2.75286253585177,-5.76725769523455));
#104626=CARTESIAN_POINT('',(5.40633447302854,2.62129679728566,-5.19822542376748));
#104627=CARTESIAN_POINT('',(4.99521329427887,2.71105259871137,-5.59444761728836));
#104628=CARTESIAN_POINT('Ctrl Pts',(5.40633447392874,2.62129679564632,-5.19822542366268));
#104629=CARTESIAN_POINT('Ctrl Pts',(5.32200534986941,2.64052352569893,-5.28593063299743));
#104630=CARTESIAN_POINT('Ctrl Pts',(5.23572206260184,2.65962575012048,-5.37139408829185));
#104631=CARTESIAN_POINT('Ctrl Pts',(5.14766584842139,2.67857142912449,-5.45449688854606));
#104632=CARTESIAN_POINT('Ctrl Pts',(5.09756988870475,2.68934979359114,-5.50177480760766));
#104633=CARTESIAN_POINT('Ctrl Pts',(5.04674468096891,2.70017879535905,-5.54843587768945));
#104634=CARTESIAN_POINT('Ctrl Pts',(4.99521329131249,2.71105259960729,-5.59444762016897));
#104635=CARTESIAN_POINT('Ctrl Pts',(4.82822475769958,2.7499999986702,-5.40839586282795));
#104636=CARTESIAN_POINT('Ctrl Pts',(4.85593323273153,2.74318451255374,-5.43943385389486));
#104637=CARTESIAN_POINT('Ctrl Pts',(4.88372172491011,2.73653622818544,-5.47047256236182));
#104638=CARTESIAN_POINT('Ctrl Pts',(4.9393774763658,2.72356451292338,-5.53247690297572));
#104639=CARTESIAN_POINT('Ctrl Pts',(4.96727788841002,2.71723336162852,-5.56347945870885));
#104640=CARTESIAN_POINT('Ctrl Pts',(4.99521329555192,2.71105259871396,-5.5944476161405));
#104641=CARTESIAN_POINT('',(5.39712984926632,2.62129679787127,-5.02280353669731));
#104642=CARTESIAN_POINT('Origin',(1.99493199737333E-14,2.71213386199978,
1.91253263226443E-13));
#104643=CARTESIAN_POINT('',(5.0006528418571,2.53084202098007,-5.58958595540413));
#104644=CARTESIAN_POINT('Origin',(-0.131396091024157,2.55357151509916,0.141404195937408));
#104645=CARTESIAN_POINT('',(4.56251304987736,2.62129679634652,-5.95260234279302));
#104646=CARTESIAN_POINT('Origin',(-0.138792725172361,2.4107913116991,0.126331557680013));
#104647=CARTESIAN_POINT('Origin',(-0.107129219609613,2.55359538161478,0.157639934758409));
#104648=CARTESIAN_POINT('Ctrl Pts',(4.83170403900001,2.750764179,-5.405287789));
#104649=CARTESIAN_POINT('Ctrl Pts',(4.538812577,2.686419405,-5.667098985));
#104650=CARTESIAN_POINT('Ctrl Pts',(4.219346023,2.621296797,-5.895728889));
#104651=CARTESIAN_POINT('Ctrl Pts',(5.179007248,2.750764179,-5.42474736));
#104652=CARTESIAN_POINT('Ctrl Pts',(4.88506134700001,2.686419405,-5.705377563));
#104653=CARTESIAN_POINT('Ctrl Pts',(4.562513043,2.621296797,-5.952602349));
#104654=CARTESIAN_POINT('',(4.39092954262006,2.62129679507543,-5.92416561186972));
#104655=CARTESIAN_POINT('Ctrl Pts',(4.23361250166653,2.61844385572301,-5.88511669028191));
#104656=CARTESIAN_POINT('Ctrl Pts',(4.22651698779161,2.61987032636152,-5.8901951591589));
#104657=CARTESIAN_POINT('Ctrl Pts',(4.21942147391668,2.621296797,-5.89527362803587));
#104658=CARTESIAN_POINT('Ctrl Pts',(4.0762728745308,2.65007516,-5.99772930912924));
#104659=CARTESIAN_POINT('Ctrl Pts',(3.92832026919488,2.678571429,-6.09311649260205));
#104660=CARTESIAN_POINT('Ctrl Pts',(3.73664594067155,2.71548867784011,-6.21669170275015));
#104661=CARTESIAN_POINT('Ctrl Pts',(3.53758353723714,2.75286253898775,-6.32797530411712));
#104662=CARTESIAN_POINT('Ctrl Pts',(4.17749075401,2.61844385572301,-6.22887605792468));
#104663=CARTESIAN_POINT('Ctrl Pts',(4.16998165850501,2.61987032636152,-6.23388598346234));
#104664=CARTESIAN_POINT('Ctrl Pts',(4.162472563,2.621296797,-6.238895909));
#104665=CARTESIAN_POINT('Ctrl Pts',(4.010980152,2.65007516,-6.339968761));
#104666=CARTESIAN_POINT('Ctrl Pts',(3.854760685,2.678571429,-6.433569776));
#104667=CARTESIAN_POINT('Ctrl Pts',(3.65237654195466,2.71548867784011,-6.55483098381374));
#104668=CARTESIAN_POINT('Ctrl Pts',(3.44277094001505,2.75286253898775,-6.6631320152788));
#104669=CARTESIAN_POINT('',(4.16247256710208,2.6212967972753,-6.23889590617043));
#104670=CARTESIAN_POINT('',(3.67578711654018,2.71105259872685,-6.53747574191002));
#104671=CARTESIAN_POINT('Ctrl Pts',(4.16247257015249,2.62129679564632,-6.2388959040854));
#104672=CARTESIAN_POINT('Ctrl Pts',(4.06126098658328,2.64052352569889,-6.30642234553461));
#104673=CARTESIAN_POINT('Ctrl Pts',(3.95862283821071,2.65962575012066,-6.37133935655009));
#104674=CARTESIAN_POINT('Ctrl Pts',(3.85476068413728,2.67857142915737,-6.43356977651691));
#104675=CARTESIAN_POINT('Ctrl Pts',(3.79567258495783,2.68934979364761,-6.46897321358428));
#104676=CARTESIAN_POINT('Ctrl Pts',(3.73600489189462,2.70017879536733,-6.5036174562153));
#104677=CARTESIAN_POINT('Ctrl Pts',(3.67578711304722,2.71105259961759,-6.5374757440446));
#104678=CARTESIAN_POINT('Ctrl Pts',(3.55269830572751,2.74999999880152,-6.31987617340038));
#104679=CARTESIAN_POINT('Ctrl Pts',(3.57308672129151,2.7431845127979,-6.35614501628686));
#104680=CARTESIAN_POINT('Ctrl Pts',(3.59355312983288,2.73653622825198,-6.3924317625532));
#104681=CARTESIAN_POINT('Ctrl Pts',(3.63457839142501,2.72356457278339,-6.46495048348133));
#104682=CARTESIAN_POINT('Ctrl Pts',(3.65516165798572,2.71723348319677,-6.50122560227696));
#104683=CARTESIAN_POINT('Ctrl Pts',(3.67578711801596,2.71105259872974,-6.5374757410682));
#104684=CARTESIAN_POINT('',(4.1911936646973,2.62129679787127,-6.06559656086156));
#104685=CARTESIAN_POINT('Origin',(-1.70002900645727E-13,2.71213386200011,
3.17454396103756E-13));
#104686=CARTESIAN_POINT('',(3.6821446043708,2.53084202104383,-6.53389708421412));
#104687=CARTESIAN_POINT('Origin',(-0.0979263329305657,2.55357153666071,
0.166344406806528));
#104688=CARTESIAN_POINT('',(3.17621048374422,2.62129679635372,-6.79423924757478));
#104689=CARTESIAN_POINT('Origin',(-0.108390380534508,2.41079129001318,0.153214497356897));
#104690=CARTESIAN_POINT('Origin',(-0.0707368488802823,2.55359538285412,
0.176984352893484));
#104691=CARTESIAN_POINT('Ctrl Pts',(3.556764388,2.750764179,-6.317588708));
#104692=CARTESIAN_POINT('Ctrl Pts',(3.214438897,2.686419405,-6.510315898));
#104693=CARTESIAN_POINT('Ctrl Pts',(2.853292624,2.621296797,-6.664924696));
#104694=CARTESIAN_POINT('Ctrl Pts',(3.891764609,2.750764179,-6.41125325));
#104695=CARTESIAN_POINT('Ctrl Pts',(3.544363801,2.686419405,-6.622132794));
#104696=CARTESIAN_POINT('Ctrl Pts',(3.176210476,2.621296797,-6.794239252));
#104697=CARTESIAN_POINT('',(3.01475156092796,2.62129679507543,-6.72958196910444));
#104698=CARTESIAN_POINT('Ctrl Pts',(2.86950685216909,2.61844385876436,-6.65762748361419));
#104699=CARTESIAN_POINT('Ctrl Pts',(2.86148551526963,2.6198703278822,-6.66106189130307));
#104700=CARTESIAN_POINT('Ctrl Pts',(2.85346417837015,2.621296797,-6.664496298992));
#104701=CARTESIAN_POINT('Ctrl Pts',(2.69163736967406,2.65007516,-6.73378390566189));
#104702=CARTESIAN_POINT('Ctrl Pts',(2.5266383885379,2.678571429,-6.79513555330274));
#104703=CARTESIAN_POINT('Ctrl Pts',(2.31288029197869,2.7154886763067,-6.87461732503512));
#104704=CARTESIAN_POINT('Ctrl Pts',(2.09454918097776,2.75286253588607,-6.94050664340249));
#104705=CARTESIAN_POINT('Ctrl Pts',(2.74079909590421,2.61844385876436,-6.98128543055836));
#104706=CARTESIAN_POINT('Ctrl Pts',(2.73238858195209,2.6198703278822,-6.98456398977921));
#104707=CARTESIAN_POINT('Ctrl Pts',(2.723978068,2.621296797,-6.987842549));
#104708=CARTESIAN_POINT('Ctrl Pts',(2.55429979,2.65007516,-7.053985984));
#104709=CARTESIAN_POINT('Ctrl Pts',(2.381611195,2.678571429,-7.111816091));
#104710=CARTESIAN_POINT('Ctrl Pts',(2.15789111477469,2.7154886763067,-7.18673566706576));
#104711=CARTESIAN_POINT('Ctrl Pts',(1.92990446456554,2.75286253588607,-7.24744567082467));
#104712=CARTESIAN_POINT('',(2.72397807518795,2.62129679728566,-6.98784254543705));
#104713=CARTESIAN_POINT('',(2.18448521775642,2.71105259874109,-7.17481876632998));
#104714=CARTESIAN_POINT('Ctrl Pts',(2.72397807604177,2.62129679564632,-6.98784254573787));
#104715=CARTESIAN_POINT('Ctrl Pts',(2.61061657427771,2.6405235256989,-7.03203275809993));
#104716=CARTESIAN_POINT('Ctrl Pts',(2.4964228100649,2.65962575012042,-7.07336787742856));
#104717=CARTESIAN_POINT('Ctrl Pts',(2.38161119431193,2.67857142911354,-7.11181609123042));
#104718=CARTESIAN_POINT('Ctrl Pts',(2.31629384972667,2.6893497935814,-7.13368962068548));
#104719=CARTESIAN_POINT('Ctrl Pts',(2.2505736657156,2.70017879535968,-7.15469710993931));
#104720=CARTESIAN_POINT('Ctrl Pts',(2.18448521418065,2.71105259958509,-7.17481876732073));
#104721=CARTESIAN_POINT('Ctrl Pts',(2.11105163103631,2.74999999854399,-6.93584610049946));
#104722=CARTESIAN_POINT('Ctrl Pts',(2.123166647636,2.74318451250202,-6.97564990496104));
#104723=CARTESIAN_POINT('Ctrl Pts',(2.13535398462692,2.73653622814086,-7.01548795905045));
#104724=CARTESIAN_POINT('Ctrl Pts',(2.15983072381233,2.72356456894578,-7.09513047405887));
#104725=CARTESIAN_POINT('Ctrl Pts',(2.17213469463377,2.71723347557679,-7.13498232014607));
#104726=CARTESIAN_POINT('Ctrl Pts',(2.18448521924304,2.71105259874358,-7.17481876586947));
#104727=CARTESIAN_POINT('',(2.78928192372766,2.62129679787127,-6.82476903121289));
#104728=CARTESIAN_POINT('Origin',(-4.74988971765899E-13,2.71213386200044,
1.59984872571961E-12));
#104729=CARTESIAN_POINT('',(2.19146337730603,2.53084202100558,-7.17269044818231));
#104730=CARTESIAN_POINT('Origin',(-0.0598777747865242,2.55357151181406,
0.183506744246429));
#104731=CARTESIAN_POINT('',(1.64139184552713,2.62129679635372,-7.31818507535165));
#104732=CARTESIAN_POINT('Origin',(-0.0729196359695544,2.41079129102837,
0.172932995350268));
#104733=CARTESIAN_POINT('Origin',(-0.0310366278976987,2.5535954019215,0.188052770169909));
#104734=CARTESIAN_POINT('Ctrl Pts',(2.115514388,2.750764179,-6.934486201));
#104735=CARTESIAN_POINT('Ctrl Pts',(1.739761628,2.686419405,-7.049117675));
#104736=CARTESIAN_POINT('Ctrl Pts',(1.353822432,2.621296797,-7.12247603199999));
#104737=CARTESIAN_POINT('Ctrl Pts',(2.422547381,2.750764179,-7.097976063));
#104738=CARTESIAN_POINT('Ctrl Pts',(2.037935743,2.686419405,-7.229244456));
#104739=CARTESIAN_POINT('Ctrl Pts',(1.641391837,2.621296797,-7.318185078));
#104740=CARTESIAN_POINT('',(1.49760714622486,2.62129679507543,-7.22033055256809));
#104741=CARTESIAN_POINT('Ctrl Pts',(1.37122627115081,2.61844385784376,-7.11883500295392));
#104742=CARTESIAN_POINT('Ctrl Pts',(1.36265416973951,2.61987032742189,-7.12046476629346));
#104743=CARTESIAN_POINT('Ctrl Pts',(1.35408206832823,2.621296797,-7.12209452963294));
#104744=CARTESIAN_POINT('Ctrl Pts',(1.1811438929391,2.65007516,-7.15497425010359));
#104745=CARTESIAN_POINT('Ctrl Pts',(1.00681370664644,2.678571429,-7.17942162675545));
#104746=CARTESIAN_POINT('Ctrl Pts',(0.780966920247157,2.71548867679214,
-7.21109348723412));
#104747=CARTESIAN_POINT('Ctrl Pts',(0.553576011372223,2.75286253686799,
-7.2285076148007));
#104748=CARTESIAN_POINT('Ctrl Pts',(1.1759507389645,2.61844385784376,-7.40725764432955));
#104749=CARTESIAN_POINT('Ctrl Pts',(1.16703206198225,2.61987032742189,-7.40865154116478));
#104750=CARTESIAN_POINT('Ctrl Pts',(1.158113385,2.621296797,-7.410045438));
#104751=CARTESIAN_POINT('Ctrl Pts',(0.978183208000001,2.65007516,-7.438166661));
#104752=CARTESIAN_POINT('Ctrl Pts',(0.797100213,2.678571429,-7.45752179));
#104753=CARTESIAN_POINT('Ctrl Pts',(0.562505086185012,2.71548867679214,
-7.48259658469367));
#104754=CARTESIAN_POINT('Ctrl Pts',(0.326797777798836,2.75286253686799,
-7.49287683126911));
#104755=CARTESIAN_POINT('',(1.15811338992526,2.6212967972753,-7.41004543713347));
#104756=CARTESIAN_POINT('',(0.591039218777014,2.71105259868594,-7.47667523986537));
#104757=CARTESIAN_POINT('Ctrl Pts',(1.15811339355499,2.62129679564632,-7.4100454365429));
#104758=CARTESIAN_POINT('Ctrl Pts',(1.03790263162981,2.64052352569889,-7.42883313360447));
#104759=CARTESIAN_POINT('Ctrl Pts',(0.917492825588274,2.65962575012064,
-7.44465357703255));
#104760=CARTESIAN_POINT('Ctrl Pts',(0.797100212035308,2.67857142915303,
-7.45752179009368));
#104761=CARTESIAN_POINT('Ctrl Pts',(0.728607788260009,2.68934979362689,
-7.46484263040351));
#104762=CARTESIAN_POINT('Ctrl Pts',(0.65990811678701,2.70017879532997,-7.47123107939918));
#104763=CARTESIAN_POINT('Ctrl Pts',(0.591039214965599,2.71105259954616,
-7.47667524011723));
#104764=CARTESIAN_POINT('Ctrl Pts',(0.570694527564471,2.74999999866232,
-7.22750357125241));
#104765=CARTESIAN_POINT('Ctrl Pts',(0.573969660404782,2.74318451258878,
-7.26898115529249));
#104766=CARTESIAN_POINT('Ctrl Pts',(0.577308060245781,2.73653622816014,
-7.31050773529034));
#104767=CARTESIAN_POINT('Ctrl Pts',(0.584091760165737,2.72356456942296,
-7.39355002482758));
#104768=CARTESIAN_POINT('Ctrl Pts',(0.587541101836548,2.71723347653185,
-7.43511514350048));
#104769=CARTESIAN_POINT('Ctrl Pts',(0.591039220362404,2.71105259868844,
-7.4766752397323));
#104770=CARTESIAN_POINT('',(1.25694645900164,2.62129679787127,-7.26482288705877));
#104771=CARTESIAN_POINT('Origin',(2.18398975120049E-13,2.71213386199911,
-2.48499137933678E-12));
#104772=CARTESIAN_POINT('',(0.598311757139466,2.53084202105362,-7.47609677821526));
#104773=CARTESIAN_POINT('Origin',(-0.0190293522278347,2.55357152284122,
0.192088535853675));
#104774=CARTESIAN_POINT('',(0.0298235498648649,2.62129679635372,-7.49994070321252));
#104775=CARTESIAN_POINT('Origin',(-0.0340393366185852,2.41079133825631,
0.184565482644015));
#104776=CARTESIAN_POINT('Origin',(0.0101147754415452,2.55359537888983,0.190328199564994));
#104777=CARTESIAN_POINT('Ctrl Pts',(0.575345286,2.750764179,-7.227134827));
#104778=CARTESIAN_POINT('Ctrl Pts',(0.183735038,2.686419405,-7.25831054400001));
#104779=CARTESIAN_POINT('Ctrl Pts',(-0.208950992,2.621296797,-7.246988304));
#104780=CARTESIAN_POINT('Ctrl Pts',(0.840054531,2.750764179,-7.452805404));
#104781=CARTESIAN_POINT('Ctrl Pts',(0.436216075,2.686419405,-7.498324682));
#104782=CARTESIAN_POINT('Ctrl Pts',(0.029823541,2.621296797,-7.499940704));
#104783=CARTESIAN_POINT('',(-0.089563713526468,2.62129679507543,-7.37346450414545));
#104784=CARTESIAN_POINT('Ctrl Pts',(-0.191171332133358,2.61844385795941,
-7.24717371104007));
#104785=CARTESIAN_POINT('Ctrl Pts',(-0.199893373131833,2.61987032747972,
-7.24692262307867));
#104786=CARTESIAN_POINT('Ctrl Pts',(-0.208615414130308,2.621296797,-7.24667153511732));
#104787=CARTESIAN_POINT('Ctrl Pts',(-0.384578558372457,2.65007516,-7.24160595159503));
#104788=CARTESIAN_POINT('Ctrl Pts',(-0.560088466166838,2.678571429,-7.22800592478954));
#104789=CARTESIAN_POINT('Ctrl Pts',(-0.787463593391741,2.71548867672983,
-7.2103869318697));
#104790=CARTESIAN_POINT('Ctrl Pts',(-1.01328175149655,2.75286253674194,
-7.17851160256953));
#104791=CARTESIAN_POINT('Ctrl Pts',(-0.443883772970446,2.61844385795941,
-7.48687472409367));
#104792=CARTESIAN_POINT('Ctrl Pts',(-0.452893582485223,2.61987032747972,
-7.48631878054684));
#104793=CARTESIAN_POINT('Ctrl Pts',(-0.461903392,2.621296797,-7.485762837));
#104794=CARTESIAN_POINT('Ctrl Pts',(-0.643672133,2.65007516,-7.474546933));
#104795=CARTESIAN_POINT('Ctrl Pts',(-0.824682289,2.678571429,-7.454522059));
#104796=CARTESIAN_POINT('Ctrl Pts',(-1.05918305066926,2.71548867672983,
-7.42857960078149));
#104797=CARTESIAN_POINT('Ctrl Pts',(-1.29158960267233,2.75286253674194,
-7.38794939696055));
#104798=CARTESIAN_POINT('',(-0.461903384016568,2.62129679728565,-7.48576283681868));
#104799=CARTESIAN_POINT('',(-1.03004311690273,2.71105259869645,-7.42893068869823));
#104800=CARTESIAN_POINT('Ctrl Pts',(-0.461903383331764,2.62129679564632,
-7.48576283741603));
#104801=CARTESIAN_POINT('Ctrl Pts',(-0.58334248386094,2.64052352569891,
-7.47826952876861));
#104802=CARTESIAN_POINT('Ctrl Pts',(-0.704338103259426,2.65962575012065,
-7.46783555041797));
#104803=CARTESIAN_POINT('Ctrl Pts',(-0.824682289784371,2.67857142915571,
-7.45452205871534));
#104804=CARTESIAN_POINT('Ctrl Pts',(-0.893147162736126,2.68934979363534,
-7.44694789511135));
#104805=CARTESIAN_POINT('Ctrl Pts',(-0.96161400199659,2.70017879534504,
-7.43841858722724));
#104806=CARTESIAN_POINT('Ctrl Pts',(-1.03004312088585,2.7110525995794,-7.42893068822571));
#104807=CARTESIAN_POINT('Ctrl Pts',(-0.996347617439242,2.74999999863268,
-7.18121100780128));
#104808=CARTESIAN_POINT('Ctrl Pts',(-1.00206550981139,2.74318451257133,
-7.22242292571251));
#104809=CARTESIAN_POINT('Ctrl Pts',(-1.00773214704197,2.7365362281456,-7.2636962946843));
#104810=CARTESIAN_POINT('Ctrl Pts',(-1.0189586819062,2.72356457151075,-7.34625538337394));
#104811=CARTESIAN_POINT('Ctrl Pts',(-1.02452525378015,2.71723348077225,
-7.38759022418198));
#104812=CARTESIAN_POINT('Ctrl Pts',(-1.03004311525274,2.711052598699,-7.42893068891884));
#104813=CARTESIAN_POINT('',(-0.334162424660559,2.62129679787127,-7.36518169807725));
#104814=CARTESIAN_POINT('Origin',(-1.67834496300756E-13,2.71213386199978,
-1.13537651502682E-12));
#104815=CARTESIAN_POINT('',(-1.02281625401732,2.53084202103967,-7.42992913193524));
#104816=CARTESIAN_POINT('Origin',(0.0227088632592475,2.55357152724356,0.191688081250765));
#104817=CARTESIAN_POINT('',(-1.58313926314193,2.62129679635372,-7.33100743818864));
#104818=CARTESIAN_POINT('Origin',(0.00643263499767649,2.41079132162034,
0.187568015178931));
#104819=CARTESIAN_POINT('Origin',(0.0507931682393102,2.55359540981668,0.18370366215818));
#104820=CARTESIAN_POINT('Ctrl Pts',(-0.991726322,2.750764179,-7.18185066));
#104821=CARTESIAN_POINT('Ctrl Pts',(-1.380882798,2.686419405,-7.128112879));
#104822=CARTESIAN_POINT('Ctrl Pts',(-1.7619541,2.621296797,-7.032639458));
#104823=CARTESIAN_POINT('Ctrl Pts',(-0.781718335,2.750764179,-7.45914984700001));
#104824=CARTESIAN_POINT('Ctrl Pts',(-1.185900572,2.686419405,-7.41679158));
#104825=CARTESIAN_POINT('Ctrl Pts',(-1.583139272,2.621296797,-7.33100743700001));
#104826=CARTESIAN_POINT('',(-1.67254667433767,2.62129679507543,-7.181823450216));
#104827=CARTESIAN_POINT('Ctrl Pts',(-1.74462997673912,2.61844385812637,
-7.0366426313749));
#104828=CARTESIAN_POINT('Ctrl Pts',(-1.75309412426899,2.6198703275632,-7.03452243284389));
#104829=CARTESIAN_POINT('Ctrl Pts',(-1.76155827179887,2.621296797,-7.03240223431287));
#104830=CARTESIAN_POINT('Ctrl Pts',(-1.93231854455011,2.65007516,-6.98962820678504));
#104831=CARTESIAN_POINT('Ctrl Pts',(-2.10080152458572,2.678571429,-6.93861669850337));
#104832=CARTESIAN_POINT('Ctrl Pts',(-2.31907318411729,2.71548867663121,
-6.87253069719649));
#104833=CARTESIAN_POINT('Ctrl Pts',(-2.53275958572269,2.75286253654245,
-6.79285636614659));
#104834=CARTESIAN_POINT('Ctrl Pts',(-2.042962772427,2.61844385812637,-7.21641386396929));
#104835=CARTESIAN_POINT('Ctrl Pts',(-2.0516424257135,2.6198703275632,-7.21393407548468));
#104836=CARTESIAN_POINT('Ctrl Pts',(-2.060322079,2.621296797,-7.211454287));
#104837=CARTESIAN_POINT('Ctrl Pts',(-2.235430081,2.65007516,-7.161425698));
#104838=CARTESIAN_POINT('Ctrl Pts',(-2.407903564,2.678571429,-7.102957161));
#104839=CARTESIAN_POINT('Ctrl Pts',(-2.631344966097,2.71548867663121,-7.02721049162782));
#104840=CARTESIAN_POINT('Ctrl Pts',(-2.84958368863575,2.75286253654245,
-6.93756966110655));
#104841=CARTESIAN_POINT('',(-2.06032207113013,2.62129679728566,-7.21145428851868));
#104842=CARTESIAN_POINT('',(-2.60296178177509,2.71105259870812,-7.03381759525322));
#104843=CARTESIAN_POINT('Ctrl Pts',(-2.06032207062386,2.62129679564632,
-7.21145428926972));
#104844=CARTESIAN_POINT('Ctrl Pts',(-2.17731115325981,2.64052352569889,
-7.17803035289206));
#104845=CARTESIAN_POINT('Ctrl Pts',(-2.29323496566152,2.6596257501205,-7.14182983331167));
#104846=CARTESIAN_POINT('Ctrl Pts',(-2.40790356477931,2.67857142912876,
-7.10295716073582));
#104847=CARTESIAN_POINT('Ctrl Pts',(-2.47313954588311,2.68934979359667,
-7.08084215318911));
#104848=CARTESIAN_POINT('Ctrl Pts',(-2.53817211940977,2.70017879536063,
-7.05779390899266));
#104849=CARTESIAN_POINT('Ctrl Pts',(-2.60296178584741,2.71105259961602,
-7.03381759402564));
#104850=CARTESIAN_POINT('Ctrl Pts',(-2.51680165573333,2.74999999864878,
-6.7991329985847));
#104851=CARTESIAN_POINT('Ctrl Pts',(-2.5312452108601,2.74318451262334,-6.83815222697435));
#104852=CARTESIAN_POINT('Ctrl Pts',(-2.54565191943021,2.73653622822029,
-6.87724248802998));
#104853=CARTESIAN_POINT('Ctrl Pts',(-2.57436387743132,2.72356451297556,
-6.95545837152627));
#104854=CARTESIAN_POINT('Ctrl Pts',(-2.58868622039588,2.71723336167073,
-6.99463058052567));
#104855=CARTESIAN_POINT('Ctrl Pts',(-2.60296178012173,2.71105259871072,
-7.03381759585593));
#104856=CARTESIAN_POINT('',(-1.90964624444247,2.62129679787127,-7.12115279973941));
#104857=CARTESIAN_POINT('Origin',(3.33500588256541E-13,2.71213386200044,
9.0726037793587E-13));
#104858=CARTESIAN_POINT('',(-2.59611851412711,2.53084202105566,-7.03634625720979));
#104859=CARTESIAN_POINT('Origin',(0.06338529817835,2.55357150892421,0.18232500043781));
#104860=CARTESIAN_POINT('',(-3.12207624230095,2.62129679634651,-6.81928441416267));
#104861=CARTESIAN_POINT('Origin',(0.0466038476729902,2.41079129955947,0.181800031907738));
#104862=CARTESIAN_POINT('Origin',(0.0890965167551067,2.55359536994261,0.168489747675488));
#104863=CARTESIAN_POINT('Ctrl Pts',(-2.51242591,2.750764179,-6.800751138));
#104864=CARTESIAN_POINT('Ctrl Pts',(-2.880932089,2.686419405,-6.664612578));
#104865=CARTESIAN_POINT('Ctrl Pts',(-3.232570193,2.621296797,-6.489452207));
#104866=CARTESIAN_POINT('Ctrl Pts',(-2.366938921,2.750764179,-7.116712734));
#104867=CARTESIAN_POINT('Ctrl Pts',(-2.752565827,2.686419405,-6.98845754600001));
#104868=CARTESIAN_POINT('Ctrl Pts',(-3.122076251,2.621296797,-6.819284411));
#104869=CARTESIAN_POINT('',(-3.17732321119419,2.62129679507543,-6.65436831415955));
#104870=CARTESIAN_POINT('Ctrl Pts',(-3.21651165857331,2.61844385750139,
-6.49708596452346));
#104871=CARTESIAN_POINT('Ctrl Pts',(-3.22432214072034,2.61987032725071,
-6.49319579266259));
#104872=CARTESIAN_POINT('Ctrl Pts',(-3.2321326228674,2.621296797,-6.48930562080173));
#104873=CARTESIAN_POINT('Ctrl Pts',(-3.38970546347181,2.65007516,-6.41082321484841));
#104874=CARTESIAN_POINT('Ctrl Pts',(-3.54328343796041,2.678571429,-6.32478546712723));
#104875=CARTESIAN_POINT('Ctrl Pts',(-3.74224549214338,2.71548867696324,
-6.21332256371282));
#104876=CARTESIAN_POINT('Ctrl Pts',(-3.93380839988302,2.75286253721407,
-6.08957471433534));
#104877=CARTESIAN_POINT('Ctrl Pts',(-3.54651510037374,2.61844385750139,
-6.60852151350342));
#104878=CARTESIAN_POINT('Ctrl Pts',(-3.55445874868688,2.61987032725071,
-6.60423383125171));
#104879=CARTESIAN_POINT('Ctrl Pts',(-3.562402397,2.621296797,-6.599946149));
#104880=CARTESIAN_POINT('Ctrl Pts',(-3.722661803,2.65007516,-6.513444156));
#104881=CARTESIAN_POINT('Ctrl Pts',(-3.878533944,2.678571429,-6.419265881));
#104882=CARTESIAN_POINT('Ctrl Pts',(-4.08046811734263,2.71548867696324,
-6.29725682832218));
#104883=CARTESIAN_POINT('Ctrl Pts',(-4.27433441331535,2.75286253721407,
-6.16279687550622));
#104884=CARTESIAN_POINT('',(-3.56240238961421,2.62129679728566,-6.59994615216608));
#104885=CARTESIAN_POINT('',(-4.05416884645219,2.71105259871873,-6.30981100856601));
#104886=CARTESIAN_POINT('Ctrl Pts',(-3.5624023893076,2.62129679564632,-6.59994615301723));
#104887=CARTESIAN_POINT('Ctrl Pts',(-3.6694711736048,2.6405235256989,-6.54215445488011));
#104888=CARTESIAN_POINT('Ctrl Pts',(-3.77490270970122,2.65962575012087,
-6.4818800904607));
#104889=CARTESIAN_POINT('Ctrl Pts',(-3.87853394488343,2.6785714291951,-6.41926588030341));
#104890=CARTESIAN_POINT('Ctrl Pts',(-3.93749067224208,2.68934979370444,
-6.38364410140354));
#104891=CARTESIAN_POINT('Ctrl Pts',(-3.99604812892601,2.70017879536494,
-6.34715463168932));
#104892=CARTESIAN_POINT('Ctrl Pts',(-4.05416885006854,2.71105259961824,
-6.30981100648448));
#104893=CARTESIAN_POINT('Ctrl Pts',(-3.91957284471539,2.74999999874113,
-6.09913508762071));
#104894=CARTESIAN_POINT('Ctrl Pts',(-3.94206669846907,2.74318451268703,
-6.13413713061112));
#104895=CARTESIAN_POINT('Ctrl Pts',(-3.96453983709032,2.73653622822721,
-6.16921646674623));
#104896=CARTESIAN_POINT('Ctrl Pts',(-4.0093946284799,2.72356451297479,-6.23943148399764));
#104897=CARTESIAN_POINT('Ctrl Pts',(-4.03180299005541,2.71723336166631,
-6.27460898817795));
#104898=CARTESIAN_POINT('Ctrl Pts',(-4.05416884499283,2.71105259872132,
-6.30981100949368));
#104899=CARTESIAN_POINT('',(-3.39583712923581,2.62129679787127,-6.54414671075182));
#104900=CARTESIAN_POINT('Origin',(-1.84531209757033E-13,2.71213386199944,
-1.73038666728687E-13));
#104901=CARTESIAN_POINT('',(-4.04802915911569,2.53084202100993,-6.31375165200503));
#104902=CARTESIAN_POINT('Origin',(0.101097921576143,2.55357153451447,0.164436471716356));
#104903=CARTESIAN_POINT('',(-4.51502840745966,2.62129679635372,-5.9886992297988));
#104904=CARTESIAN_POINT('Origin',(0.0845957595437319,2.41079130381635,0.167530973877907));
#104905=CARTESIAN_POINT('Origin',(0.123233812183939,2.55359542229066,0.145397460344019));
#104906=CARTESIAN_POINT('Ctrl Pts',(-3.915647254,2.750764179,-6.101656052));
#104907=CARTESIAN_POINT('Ctrl Pts',(-4.246272197,2.686419405,-5.8894824));
#104908=CARTESIAN_POINT('Ctrl Pts',(-4.552034896,2.621296797,-5.642825383));
#104909=CARTESIAN_POINT('Ctrl Pts',(-3.841484074,2.750764179,-6.44150604300001));
#104910=CARTESIAN_POINT('Ctrl Pts',(-4.190524162,2.686419405,-6.233351005));
#104911=CARTESIAN_POINT('Ctrl Pts',(-4.515028415,2.621296797,-5.988699225));
#104912=CARTESIAN_POINT('',(-4.53353164605597,2.62129679507543,-5.81576231136186));
#104913=CARTESIAN_POINT('Ctrl Pts',(-4.53799284712549,2.61844386027133,
-5.65373276708909));
#104914=CARTESIAN_POINT('Ctrl Pts',(-4.54478444599355,2.61987032863568,
-5.64825452784854));
#104915=CARTESIAN_POINT('Ctrl Pts',(-4.55157604486155,2.621296797,-5.64277628860798));
#104916=CARTESIAN_POINT('Ctrl Pts',(-4.68859352275467,2.65007516,-5.53225525539869));
#104917=CARTESIAN_POINT('Ctrl Pts',(-4.82008535682161,2.678571429,-5.41521429691583));
#104918=CARTESIAN_POINT('Ctrl Pts',(-4.99043455325611,2.71548867555358,
-5.26358637970675));
#104919=CARTESIAN_POINT('Ctrl Pts',(-5.15091669160818,2.75286253436271,
-5.10155133003253));
#104920=CARTESIAN_POINT('Ctrl Pts',(-4.88423633966056,2.61844386027133,
-5.69162202889658));
#104921=CARTESIAN_POINT('Ctrl Pts',(-4.89107253833026,2.61987032863568,
-5.68572694644828));
#104922=CARTESIAN_POINT('Ctrl Pts',(-4.897908737,2.621296797,-5.679831864));
#104923=CARTESIAN_POINT('Ctrl Pts',(-5.035825996,2.65007516,-5.560901205));
#104924=CARTESIAN_POINT('Ctrl Pts',(-5.167808388,2.678571429,-5.435416862));
#104925=CARTESIAN_POINT('Ctrl Pts',(-5.33879310681165,2.71548867555358,
-5.27285044207639));
#104926=CARTESIAN_POINT('Ctrl Pts',(-5.49922199451123,2.75286253436271,
-5.09985857233358));
#104927=CARTESIAN_POINT('',(-4.89790873051315,2.62129679728566,-5.67983186868445));
#104928=CARTESIAN_POINT('',(-5.31580748222907,2.71105259874511,-5.29076467184931));
#104929=CARTESIAN_POINT('Ctrl Pts',(-4.89790873035063,2.6212967956464,-5.67983186957653));
#104930=CARTESIAN_POINT('Ctrl Pts',(-4.99005079942674,2.64052352569892,
-5.60037468588713));
#104931=CARTESIAN_POINT('Ctrl Pts',(-5.08006019835419,2.65962575012044,
-5.51884483873591));
#104932=CARTESIAN_POINT('Ctrl Pts',(-5.16780838853741,2.67857142911603,
-5.43541686148905));
#104933=CARTESIAN_POINT('Ctrl Pts',(-5.21772911097534,2.68934979358859,
-5.38795394676343));
#104934=CARTESIAN_POINT('Ctrl Pts',(-5.26707336984754,2.70017879537978,
-5.33972945793456));
#104935=CARTESIAN_POINT('Ctrl Pts',(-5.3158074852467,2.71105259963722,-5.29076466905523));
#104936=CARTESIAN_POINT('Ctrl Pts',(-5.13906916553877,2.74999999856141,
-5.11394839909537));
#104937=CARTESIAN_POINT('Ctrl Pts',(-5.16856153009576,2.74318451249827,
-5.14329660033381));
#104938=CARTESIAN_POINT('Ctrl Pts',(-5.1980502790435,2.736536228155,-5.17272474019524));
#104939=CARTESIAN_POINT('Ctrl Pts',(-5.25695027066359,2.72356457300384,
-5.23165544222286));
#104940=CARTESIAN_POINT('Ctrl Pts',(-5.28639655221916,2.71723348380006,
-5.26119306894966));
#104941=CARTESIAN_POINT('Ctrl Pts',(-5.31580748100938,2.71105259874964,
-5.29076467304409));
#104942=CARTESIAN_POINT('',(-4.72324244319091,2.62129679787127,-5.66114359451915));
#104943=CARTESIAN_POINT('Origin',(-4.76615275024628E-13,2.71213386199922,
-4.74446870679657E-13));
#104944=CARTESIAN_POINT('',(-5.31065845856635,2.5308420210107,-5.29593303699472));
#104945=CARTESIAN_POINT('Origin',(0.134083019446607,2.55357153242441,0.138858695162986));
#104946=CARTESIAN_POINT('',(-5.6968628626643,2.62129679635371,-4.87808912527821));
#104947=CARTESIAN_POINT('Origin',(0.11863234393832,2.41079130577976,0.14542877855957));
#104948=CARTESIAN_POINT('Origin',(0.151608896027703,2.55359538524557,0.115506578058185));
#104949=CARTESIAN_POINT('Ctrl Pts',(-5.135777285,2.750764179,-5.11725431));
#104950=CARTESIAN_POINT('Ctrl Pts',(-5.413061337,2.686419405,-4.838966571));
#104951=CARTESIAN_POINT('Ctrl Pts',(-5.658651506,2.621296797,-4.532346316));
#104952=CARTESIAN_POINT('Ctrl Pts',(-5.136405701,2.750764179,-5.465101689));
#104953=CARTESIAN_POINT('Ctrl Pts',(-5.432538246,2.686419405,-5.186779898));
#104954=CARTESIAN_POINT('Ctrl Pts',(-5.696862869,2.621296797,-4.878089119));
#104955=CARTESIAN_POINT('',(-5.67775717985935,2.62129679507543,-4.70521772671993));
#104956=CARTESIAN_POINT('Ctrl Pts',(-5.64728250819685,2.6184438579262,-4.54601732828464));
#104957=CARTESIAN_POINT('Ctrl Pts',(-5.65273766822465,2.61987032746311,
-4.5392071685867));
#104958=CARTESIAN_POINT('Ctrl Pts',(-5.65819282825249,2.621296797,-4.53239700888875));
#104959=CARTESIAN_POINT('Ctrl Pts',(-5.76824815817284,2.65007516,-4.39500518746768));
#104960=CARTESIAN_POINT('Ctrl Pts',(-5.87150544120964,2.678571429,-4.25243372517932));
#104961=CARTESIAN_POINT('Ctrl Pts',(-6.0052764513976,2.71548867669054,-4.06773073697445));
#104962=CARTESIAN_POINT('Ctrl Pts',(-6.12717386396559,2.75286253666248,
-3.87498505535434));
#104963=CARTESIAN_POINT('Ctrl Pts',(-5.99357609275843,2.6184438579262,-4.50858864453285));
#104964=CARTESIAN_POINT('Ctrl Pts',(-5.99898520087922,2.61987032746311,
-4.50136179926641));
#104965=CARTESIAN_POINT('Ctrl Pts',(-6.004394309,2.621296797,-4.494134954));
#104966=CARTESIAN_POINT('Ctrl Pts',(-6.113520563,2.65007516,-4.348336694));
#104967=CARTESIAN_POINT('Ctrl Pts',(-6.215441855,2.678571429,-4.197413792));
#104968=CARTESIAN_POINT('Ctrl Pts',(-6.34748207552619,2.71548867669054,
-4.00189141849574));
#104969=CARTESIAN_POINT('Ctrl Pts',(-6.466972089439,2.75286253666248,-3.7984565275671));
#104970=CARTESIAN_POINT('',(-6.00439430365377,2.62129679728566,-4.49413495997162));
#104971=CARTESIAN_POINT('',(-6.32888486767079,2.71105259873234,-4.02432805943173));
#104972=CARTESIAN_POINT('Ctrl Pts',(-6.00439430370528,2.62129679564633,
-4.49413496087588));
#104973=CARTESIAN_POINT('Ctrl Pts',(-6.07730119665115,2.64052352569891,
-4.39672762094362));
#104974=CARTESIAN_POINT('Ctrl Pts',(-6.14767971852342,2.65962575012029,
-4.29775453615439));
#104975=CARTESIAN_POINT('Ctrl Pts',(-6.21544185532184,2.67857142908998,
-4.19741379152342));
#104976=CARTESIAN_POINT('Ctrl Pts',(-6.25399233533359,2.68934979354362,
-4.14032905383643));
#104977=CARTESIAN_POINT('Ctrl Pts',(-6.29181611341531,2.70017879537231,
-4.08262446955145));
#104978=CARTESIAN_POINT('Ctrl Pts',(-6.32888487002719,2.71105259962688,
-4.02432805604451));
#104979=CARTESIAN_POINT('Ctrl Pts',(-6.11826832263678,2.74999999864412,
-3.88963916710401));
#104980=CARTESIAN_POINT('Ctrl Pts',(-6.15338016777334,2.74318451258122,
-3.91196123685969));
#104981=CARTESIAN_POINT('Ctrl Pts',(-6.18850566656794,2.73653622817913,
-3.93436215385672));
#104982=CARTESIAN_POINT('Ctrl Pts',(-6.25869729295971,2.72356451295359,
-3.97925353934956));
#104983=CARTESIAN_POINT('Ctrl Pts',(-6.29380522164525,2.71723336165523,
-4.00177075055494));
#104984=CARTESIAN_POINT('Ctrl Pts',(-6.32888486674516,2.71105259873492,
-4.02432806087192));
#104985=CARTESIAN_POINT('',(-5.82979419021296,2.62129679787127,-4.51343169603635));
#104986=CARTESIAN_POINT('Origin',(-5.78096598369271E-13,2.71213386199944,
-3.45209971719385E-13));
#104987=CARTESIAN_POINT('',(-6.32496727096945,2.53084202101589,-4.03048247922101));
#104988=CARTESIAN_POINT('Origin',(0.160798984945445,2.55357150552199,0.106788523341716));
#104989=CARTESIAN_POINT('',(-6.61231834116049,2.62129679635372,-3.53938499548876));
#104990=CARTESIAN_POINT('Origin',(0.147121763757694,2.41079132245498,0.116526339602698));
#104991=CARTESIAN_POINT('Origin',(0.172895077899152,2.55359537142438,0.0802147940364417));
#104992=CARTESIAN_POINT('Ctrl Pts',(-6.115764078,2.750764179,-3.893575445));
#104993=CARTESIAN_POINT('Ctrl Pts',(-6.326741745,2.686419405,-3.562186043));
#104994=CARTESIAN_POINT('Ctrl Pts',(-6.500675861,2.621296797,-3.209939773));
#104995=CARTESIAN_POINT('Ctrl Pts',(-6.191154706,2.750764179,-4.233155254));
#104996=CARTESIAN_POINT('Ctrl Pts',(-6.420532878,2.686419405,-3.897680728));
#104997=CARTESIAN_POINT('Ctrl Pts',(-6.612318346,2.621296797,-3.539384988));
#104998=CARTESIAN_POINT('',(-6.55649709801999,2.62129679507543,-3.37466239114689));
#104999=CARTESIAN_POINT('Ctrl Pts',(-6.49251152790548,2.61844385805783,
-3.22573516232869));
#105000=CARTESIAN_POINT('Ctrl Pts',(-6.49637516612974,2.61987032752893,
-3.2179115226025));
#105001=CARTESIAN_POINT('Ctrl Pts',(-6.500238804354,2.621296797,-3.21008788287631));
#105002=CARTESIAN_POINT('Ctrl Pts',(-6.57818592174632,2.65007516,-3.05224956345433));
#105003=CARTESIAN_POINT('Ctrl Pts',(-6.64838045698693,2.678571429,-2.89081407897152));
#105004=CARTESIAN_POINT('Ctrl Pts',(-6.73931829222693,2.71548867670329,
-2.68167253086331));
#105005=CARTESIAN_POINT('Ctrl Pts',(-6.8169311873176,2.75286253668826,-2.46722879455499));
#105006=CARTESIAN_POINT('Ctrl Pts',(-6.82266290017222,2.61844385805783,
-3.11473865527265));
#105007=CARTESIAN_POINT('Ctrl Pts',(-6.82639198808613,2.61987032752893,
-3.10651797163632));
#105008=CARTESIAN_POINT('Ctrl Pts',(-6.830121076,2.621296797,-3.098297288));
#105009=CARTESIAN_POINT('Ctrl Pts',(-6.905353703,2.65007516,-2.932448791));
#105010=CARTESIAN_POINT('Ctrl Pts',(-6.972448169,2.678571429,-2.763144319));
#105011=CARTESIAN_POINT('Ctrl Pts',(-7.05936983164764,2.71548867670329,
-2.54380840441185));
#105012=CARTESIAN_POINT('Ctrl Pts',(-7.13233374779166,2.75286253668826,
-2.31944288760547));
#105013=CARTESIAN_POINT('',(-6.83012107208854,2.62129679728566,-3.09829729497249));
#105014=CARTESIAN_POINT('',(-7.04603063111164,2.7110525987244,-2.56971833966129));
#105015=CARTESIAN_POINT('Ctrl Pts',(-6.8301210723073,2.62129679564632,-3.09829729585335));
#105016=CARTESIAN_POINT('Ctrl Pts',(-6.8803837440735,2.64052352569889,-2.98749445823591));
#105017=CARTESIAN_POINT('Ctrl Pts',(-6.927840567671,2.65962575012087,-2.87570600767742));
#105018=CARTESIAN_POINT('Ctrl Pts',(-6.97244816946066,2.67857142919565,
-2.76314431783758));
#105019=CARTESIAN_POINT('Ctrl Pts',(-6.99782582954319,2.68934979370559,
-2.69910697527566));
#105020=CARTESIAN_POINT('Ctrl Pts',(-7.02236052837708,2.7001787953517,-2.6346204987359));
#105021=CARTESIAN_POINT('Ctrl Pts',(-7.04603063233495,2.71105259957602,
-2.56971833610226));
#105022=CARTESIAN_POINT('Ctrl Pts',(-6.81138405351766,2.74999999863303,
-2.48345472967256));
#105023=CARTESIAN_POINT('Ctrl Pts',(-6.85047358844989,2.74318451256408,
-2.49770691327413));
#105024=CARTESIAN_POINT('Ctrl Pts',(-6.8895934074537,2.73653622818423,-2.51203316538098));
#105025=CARTESIAN_POINT('Ctrl Pts',(-6.96779397439078,2.72356456920812,
-2.54078576580119));
#105026=CARTESIAN_POINT('Ctrl Pts',(-7.00692124906745,2.71723347608493,
-2.55522922667391));
#105027=CARTESIAN_POINT('Ctrl Pts',(-7.04603063056539,2.71105259872689,
-2.56971834113679));
#105028=CARTESIAN_POINT('',(-6.66375124013802,2.62129679787127,-3.1546767477559));
#105029=CARTESIAN_POINT('Origin',(-1.63324215263216E-12,2.71213386200011,
-5.73976630113826E-13));
#105030=CARTESIAN_POINT('',(-7.04352764417412,2.53084202101217,-2.57657103907726));
#105031=CARTESIAN_POINT('Origin',(0.179995935634774,2.55357153834234,0.06972483404799));
#105032=CARTESIAN_POINT('',(-7.21858916277932,2.62129679634651,-2.03518315668438));
#105033=CARTESIAN_POINT('Origin',(0.168731710674025,2.41079132945112,0.0821751309787647));
#105034=CARTESIAN_POINT('Origin',(0.18609630974445,2.55359540305191,0.0411719527489995));
#105035=CARTESIAN_POINT('Ctrl Pts',(-6.80978454,2.750764179,-2.487837318));
#105036=CARTESIAN_POINT('Ctrl Pts',(-6.944590741,2.686419405,-2.118841655));
#105037=CARTESIAN_POINT('Ctrl Pts',(-7.038735838,2.621296797,-1.737440013));
#105038=CARTESIAN_POINT('Ctrl Pts',(-6.956412198,2.750764179,-2.803271184));
#105039=CARTESIAN_POINT('Ctrl Pts',(-7.10831053000001,2.686419405,-2.42633034));
#105040=CARTESIAN_POINT('Ctrl Pts',(-7.218589166,2.621296797,-2.035183148));
#105041=CARTESIAN_POINT('',(-7.12866249893688,2.62129679507543,-1.88631159207601));
#105042=CARTESIAN_POINT('Ctrl Pts',(-7.03415792518274,2.61844385865813,
-1.7546212015925));
#105043=CARTESIAN_POINT('Ctrl Pts',(-7.03624938200634,2.61987032782908,
-1.74614990797347));
#105044=CARTESIAN_POINT('Ctrl Pts',(-7.03834083882998,2.621296797,-1.73767861435444));
#105045=CARTESIAN_POINT('Ctrl Pts',(-7.08053502353146,2.65007516,-1.56677414069536));
#105046=CARTESIAN_POINT('Ctrl Pts',(-7.11438459092148,2.678571429,-1.39402317853381));
#105047=CARTESIAN_POINT('Ctrl Pts',(-7.15823710012756,2.7154886763785,-1.17022229926958));
#105048=CARTESIAN_POINT('Ctrl Pts',(-7.18793638372117,2.7528625360313,-0.944107662566128));
#105049=CARTESIAN_POINT('Ctrl Pts',(-7.33272957398523,2.61844385865813,
-1.57524694584273));
#105050=CARTESIAN_POINT('Ctrl Pts',(-7.3346042734926,2.61987032782908,-1.56641681542136));
#105051=CARTESIAN_POINT('Ctrl Pts',(-7.336478973,2.621296797,-1.557586685));
#105052=CARTESIAN_POINT('Ctrl Pts',(-7.374300178,2.65007516,-1.379442843));
#105053=CARTESIAN_POINT('Ctrl Pts',(-7.403430556,2.678571429,-1.199673288));
#105054=CARTESIAN_POINT('Ctrl Pts',(-7.44116929989033,2.7154886763785,-0.966779739269926));
#105055=CARTESIAN_POINT('Ctrl Pts',(-7.46419540639517,2.7528625360313,-0.731974680503638));
#105056=CARTESIAN_POINT('',(-7.33647897188281,2.6212967972753,-1.55758668986226));
#105057=CARTESIAN_POINT('',(-7.43371183306277,2.71105259873374,-0.994951446310446));
#105058=CARTESIAN_POINT('Ctrl Pts',(-7.33647897108187,2.62129679564632,
-1.55758669346358));
#105059=CARTESIAN_POINT('Ctrl Pts',(-7.36174719434701,2.64052352569893,
-1.43856937610547));
#105060=CARTESIAN_POINT('Ctrl Pts',(-7.38406329122853,2.65962575012077,
-1.31919266302739));
#105061=CARTESIAN_POINT('Ctrl Pts',(-7.4034305561815,2.67857142917754,-1.19967328687996));
#105062=CARTESIAN_POINT('Ctrl Pts',(-7.4144487649051,2.6893497936799,-1.1316776551174));
#105063=CARTESIAN_POINT('Ctrl Pts',(-7.42454716987242,2.70017879535656,
-1.06342460138614));
#105064=CARTESIAN_POINT('Ctrl Pts',(-7.43371183347961,2.71105259958219,
-0.994951442592408));
#105065=CARTESIAN_POINT('Ctrl Pts',(-7.18600703533534,2.74999999872123,
-0.961146710006495));
#105066=CARTESIAN_POINT('Ctrl Pts',(-7.22724647673893,2.74318451266386,
-0.966662590906057));
#105067=CARTESIAN_POINT('Ctrl Pts',(-7.26853141705599,2.73653622824394,
-0.972244298447054));
#105068=CARTESIAN_POINT('Ctrl Pts',(-7.35108465813915,2.72356456914425,
-0.98351386869375));
#105069=CARTESIAN_POINT('Ctrl Pts',(-7.39240207692326,2.71723347589383,
-0.989208442053305));
#105070=CARTESIAN_POINT('Ctrl Pts',(-7.43371183284747,2.71105259873624,
-0.994951447861807));
#105071=CARTESIAN_POINT('',(-7.18611868862997,2.62129679787127,-1.64841262084963));
#105072=CARTESIAN_POINT('Origin',(1.28282801048485E-12,2.712133862001,2.74303149638833E-13));
#105073=CARTESIAN_POINT('',(-7.43274049270506,2.53084202102667,-1.00218200151022));
#105074=CARTESIAN_POINT('Origin',(0.190776648901901,2.55357153535686,0.0294009220419665));
#105075=CARTESIAN_POINT('',(-7.48732677872139,2.62129679634651,-0.435818415173266));
#105076=CARTESIAN_POINT('Origin',(0.182451887431564,2.41079132038099,0.0439815725696998));
#105077=CARTESIAN_POINT('Origin',(0.190596324983798,2.55359539930593,0.00020417990560892));
#105078=CARTESIAN_POINT('Ctrl Pts',(-7.185387045,2.750764179,-0.965770684));
#105079=CARTESIAN_POINT('Ctrl Pts',(-7.237718391,2.686419405,-0.576422586));
#105080=CARTESIAN_POINT('Ctrl Pts',(-7.24767235000001,2.621296797,-0.18369949));
#105081=CARTESIAN_POINT('Ctrl Pts',(-7.396395587,2.750764179,-1.242309269));
#105082=CARTESIAN_POINT('Ctrl Pts',(-7.463711481,2.686419405,-0.841527441));
#105083=CARTESIAN_POINT('Ctrl Pts',(-7.48732678,2.621296797,-0.435818406));
#105084=CARTESIAN_POINT('',(-7.36749956449699,2.62129679507543,-0.309758959963846));
#105085=CARTESIAN_POINT('Ctrl Pts',(-7.24689491401017,2.61844385892813,
-0.201463106179223));
#105086=CARTESIAN_POINT('Ctrl Pts',(-7.24711639599255,2.61987032796408,
-0.192740266134972));
#105087=CARTESIAN_POINT('Ctrl Pts',(-7.24733787797487,2.621296797,-0.184017426090723));
#105088=CARTESIAN_POINT('Ctrl Pts',(-7.25180617607661,2.65007516,-0.00803810171583814));
#105089=CARTESIAN_POINT('Ctrl Pts',(-7.24772800926328,2.678571429,0.167950695928088));
#105090=CARTESIAN_POINT('Ctrl Pts',(-7.24244469784854,2.71548867625678,
0.395946228542094));
#105091=CARTESIAN_POINT('Ctrl Pts',(-7.22284166571237,2.75286253578508,
0.623158897767339));
#105092=CARTESIAN_POINT('Ctrl Pts',(-7.49992596089625,2.61844385892813,
0.0379015589993896));
#105093=CARTESIAN_POINT('Ctrl Pts',(-7.49985861394813,2.61987032796408,
0.0469282499996948));
#105094=CARTESIAN_POINT('Ctrl Pts',(-7.499791267,2.621296797,0.055954941));
#105095=CARTESIAN_POINT('Ctrl Pts',(-7.498432573,2.65007516,0.23806432));
#105096=CARTESIAN_POINT('Ctrl Pts',(-7.488236759,2.678571429,0.419893133));
#105097=CARTESIAN_POINT('Ctrl Pts',(-7.47502796352101,2.71548867625678,
0.655454472556969));
#105098=CARTESIAN_POINT('Ctrl Pts',(-7.44703958575088,2.75286253578508,
0.889719851663243));
#105099=CARTESIAN_POINT('',(-7.49979126766924,2.6212967972884,0.0559549390073793));
#105100=CARTESIAN_POINT('',(-7.47380093222409,2.71105259872497,0.62633827058748));
#105101=CARTESIAN_POINT('Ctrl Pts',(-7.49979126689562,2.62129679671618,
0.0559549390920314));
#105102=CARTESIAN_POINT('Ctrl Pts',(-7.49888352787154,2.64052352640753,
0.177621616481776));
#105103=CARTESIAN_POINT('Ctrl Pts',(-7.49501542236969,2.65962575047207,
0.29900466727516));
#105104=CARTESIAN_POINT('Ctrl Pts',(-7.48823675894358,2.67857142915768,
0.419893134006151));
#105105=CARTESIAN_POINT('Ctrl Pts',(-7.48438031722435,2.68934979364746,
0.488667654481343));
#105106=CARTESIAN_POINT('Ctrl Pts',(-7.47957023810782,2.70017879535944,
0.557495848336267));
#105107=CARTESIAN_POINT('Ctrl Pts',(-7.47380093223093,2.71105259897497,
0.626338270548561));
#105108=CARTESIAN_POINT('Ctrl Pts',(-7.22462031598099,2.74999999861703,
0.606103461913437));
#105109=CARTESIAN_POINT('Ctrl Pts',(-7.26608135359757,2.74318451256247,
0.609581800086605));
#105110=CARTESIAN_POINT('Ctrl Pts',(-7.30760097709695,2.73653622816163,
0.613005631471987));
#105111=CARTESIAN_POINT('Ctrl Pts',(-7.39064678583536,2.72356457033612,
0.6197460432713));
#105112=CARTESIAN_POINT('Ctrl Pts',(-7.43222238227318,2.71723347837816,
0.623066628800585));
#105113=CARTESIAN_POINT('Ctrl Pts',(-7.47380093235173,2.71105259872747,
0.626338268970032));
#105114=CARTESIAN_POINT('',(-7.37247121386783,2.62129679787127,-0.065070551999726));
#105115=CARTESIAN_POINT('Origin',(9.15066633577766E-14,2.71213386199933,
1.52838625002566E-14));
#105116=CARTESIAN_POINT('',(-7.4744066564856,2.53084202101296,0.619067951245984));
#105117=CARTESIAN_POINT('Origin',(0.192636453794941,2.55357154185465,-0.0122977839903749));
#105118=CARTESIAN_POINT('',(-7.40596531666914,2.62129679635372,1.18392471111636));
#105119=CARTESIAN_POINT('Origin',(0.187641356349404,2.4107912956149,0.00373151825628901));
#105120=CARTESIAN_POINT('Origin',(0.186184210808453,2.55359535292823,-0.040773175267849));
#105121=CARTESIAN_POINT('Ctrl Pts',(-7.225008838,2.750764179,0.601454314));
#105122=CARTESIAN_POINT('Ctrl Pts',(-7.192418375,2.686419405,0.992949363));
#105123=CARTESIAN_POINT('Ctrl Pts',(-7.117715759,2.621296797,1.378630618));
#105124=CARTESIAN_POINT('Ctrl Pts',(-7.490531739,2.750764179,0.376741646));
#105125=CARTESIAN_POINT('Ctrl Pts',(-7.470117579,2.686419405,0.782624346));
#105126=CARTESIAN_POINT('Ctrl Pts',(-7.40596531600001,2.621296797,1.18392472));
#105127=CARTESIAN_POINT('',(-7.26184053958062,2.62129679507543,1.28127765720773));
#105128=CARTESIAN_POINT('Ctrl Pts',(-7.12077515222738,2.61844385828202,
1.36111517550213));
#105129=CARTESIAN_POINT('Ctrl Pts',(-7.11911630287345,2.61987032764103,
1.36968169442626));
#105130=CARTESIAN_POINT('Ctrl Pts',(-7.11745745351951,2.621296797,1.37824821335038));
#105131=CARTESIAN_POINT('Ctrl Pts',(-7.08399093103904,2.65007516,1.55107379119606));
#105132=CARTESIAN_POINT('Ctrl Pts',(-7.04217572103884,2.678571429,1.72207138310816));
#105133=CARTESIAN_POINT('Ctrl Pts',(-6.9880036296484,2.71548867665875,1.94360075211794));
#105134=CARTESIAN_POINT('Ctrl Pts',(-6.92001489751408,2.75286253659817,
2.16128724597702));
#105135=CARTESIAN_POINT('Ctrl Pts',(-7.31643414512728,2.61844385828202,
1.64927782224517));
#105136=CARTESIAN_POINT('Ctrl Pts',(-7.31442790056365,2.61987032764103,
1.6580789986226));
#105137=CARTESIAN_POINT('Ctrl Pts',(-7.312421656,2.621296797,1.666880175));
#105138=CARTESIAN_POINT('Ctrl Pts',(-7.271946595,2.65007516,1.844439859));
#105139=CARTESIAN_POINT('Ctrl Pts',(-7.222901333,2.678571429,2.019825817));
#105140=CARTESIAN_POINT('Ctrl Pts',(-7.15936262624074,2.71548867665875,
2.2470403659787));
#105141=CARTESIAN_POINT('Ctrl Pts',(-7.08166846786064,2.75286253659817,
2.46981207901721));
#105142=CARTESIAN_POINT('',(-7.31242165711993,2.62129679728566,1.66688016710317));
#105143=CARTESIAN_POINT('',(-7.16442340568091,2.71105259871166,2.21834110639597));
#105144=CARTESIAN_POINT('Ctrl Pts',(-7.31242165781292,2.62129679564631,
1.66688016651325));
#105145=CARTESIAN_POINT('Ctrl Pts',(-7.28538040220296,2.6405235256989,1.78550720985933));
#105146=CARTESIAN_POINT('Ctrl Pts',(-7.25550896261107,2.6596257501206,1.90322086635885));
#105147=CARTESIAN_POINT('Ctrl Pts',(-7.22290133274773,2.67857142914657,
2.0198258179021));
#105148=CARTESIAN_POINT('Ctrl Pts',(-7.2043505635659,2.68934979362375,2.0861634074725));
#105149=CARTESIAN_POINT('Ctrl Pts',(-7.18485691423706,2.70017879534133,
2.15234841177172));
#105150=CARTESIAN_POINT('Ctrl Pts',(-7.16442340449928,2.71105259955887,
2.21834110993971));
#105151=CARTESIAN_POINT('Ctrl Pts',(-6.9254183801212,2.74999999862198,2.14501290959327));
#105152=CARTESIAN_POINT('Ctrl Pts',(-6.96516234178542,2.74318451253604,
2.15732282371328));
#105153=CARTESIAN_POINT('Ctrl Pts',(-7.00497523682302,2.73653622813951,
2.16959209955852));
#105154=CARTESIAN_POINT('Ctrl Pts',(-7.08463049941604,2.7235645689707,2.19402732086462));
#105155=CARTESIAN_POINT('Ctrl Pts',(-7.12452026293017,2.71723347564953,
2.2062077999943));
#105156=CARTESIAN_POINT('Ctrl Pts',(-7.16442340613617,2.71105259871414,
2.21834110489999));
#105157=CARTESIAN_POINT('',(-7.21409517911789,2.62129679787127,1.52131414348509));
#105158=CARTESIAN_POINT('Origin',(2.80157841370254E-13,2.71213386200022,
-6.41847686111419E-14));
#105159=CARTESIAN_POINT('',(-7.16657787235504,2.5308420210297,2.21137097685949));
#105160=CARTESIAN_POINT('Origin',(0.185489065332484,2.55357149766622,-0.0534214076825659));
#105161=CARTESIAN_POINT('',(-6.97830914658419,2.62129679635372,2.74830883345958));
#105162=CARTESIAN_POINT('Origin',(0.184056299553969,2.41079131761793,-0.03669298340372));
#105163=CARTESIAN_POINT('Origin',(0.173066248691005,2.55359536109132,-0.0798440052102473));
#105164=CARTESIAN_POINT('Ctrl Pts',(-6.926797248,2.750764179,2.140555977));
#105165=CARTESIAN_POINT('Ctrl Pts',(-6.810808868,2.686419405,2.515892103));
#105166=CARTESIAN_POINT('Ctrl Pts',(-6.65494268900001,2.621296797,2.87649749));
#105167=CARTESIAN_POINT('Ctrl Pts',(-7.234418952,2.750764179,1.978176541));
#105168=CARTESIAN_POINT('Ctrl Pts',(-7.127229281,2.686419405,2.370181488));
#105169=CARTESIAN_POINT('Ctrl Pts',(-6.978309144,2.621296797,2.748308842));
#105170=CARTESIAN_POINT('',(-6.81662592106697,2.62129679507543,2.8124031549307));
#105171=CARTESIAN_POINT('Ctrl Pts',(-6.66169585821932,2.6184438580596,2.86004922667223));
#105172=CARTESIAN_POINT('Ctrl Pts',(-6.65823424323192,2.61987032752981,
2.86805886218263));
#105173=CARTESIAN_POINT('Ctrl Pts',(-6.65477262824444,2.621296797,2.87606849769305));
#105174=CARTESIAN_POINT('Ctrl Pts',(-6.58493614400342,2.65007516,3.03765919629072));
#105175=CARTESIAN_POINT('Ctrl Pts',(-6.50733912290844,2.678571429,3.19566992533473));
#105176=CARTESIAN_POINT('Ctrl Pts',(-6.40681127817498,2.71548867668329,
3.40037466356505));
#105177=CARTESIAN_POINT('Ctrl Pts',(-6.2936159231953,2.7528625366478,3.59835620000264));
#105178=CARTESIAN_POINT('Ctrl Pts',(-6.79083400258147,2.6184438580596,3.18353569180921));
#105179=CARTESIAN_POINT('Ctrl Pts',(-6.78698266979072,2.61987032752981,
3.19169981890462));
#105180=CARTESIAN_POINT('Ctrl Pts',(-6.783131337,2.621296797,3.199863946));
#105181=CARTESIAN_POINT('Ctrl Pts',(-6.705432476,2.65007516,3.364571441));
#105182=CARTESIAN_POINT('Ctrl Pts',(-6.619831069,2.678571429,3.525313691));
#105183=CARTESIAN_POINT('Ctrl Pts',(-6.50893345005424,2.71548867668329,
3.73355714601356));
#105184=CARTESIAN_POINT('Ctrl Pts',(-6.38516640466118,2.7528625366478,3.93441863305437));
#105185=CARTESIAN_POINT('',(-6.78313133976152,2.62129679728566,3.19986393845337));
#105186=CARTESIAN_POINT('',(-6.52004540355434,2.71105259878431,3.70661677728345));
#105187=CARTESIAN_POINT('Ctrl Pts',(-6.78313134020659,2.62129679579015,
3.19986393892462));
#105188=CARTESIAN_POINT('Ctrl Pts',(-6.73122098611652,2.64052352569892,
3.30990447608709));
#105189=CARTESIAN_POINT('Ctrl Pts',(-6.6767429675063,2.65962575012078,3.41844457593528));
#105190=CARTESIAN_POINT('Ctrl Pts',(-6.61983106845008,2.67857142917906,
3.52531369197484));
#105191=CARTESIAN_POINT('Ctrl Pts',(-6.58745338552236,2.68934979350172,
3.58611247752341));
#105192=CARTESIAN_POINT('Ctrl Pts',(-6.55418766809202,2.70017879498377,
3.64655955347962));
#105193=CARTESIAN_POINT('Ctrl Pts',(-6.52004540370745,2.71105259900381,
3.70661677733075));
#105194=CARTESIAN_POINT('Ctrl Pts',(-6.30239157675153,2.74999999863007,
3.58362393733051));
#105195=CARTESIAN_POINT('Ctrl Pts',(-6.33856007909119,2.7431845125664,3.60418982947076));
#105196=CARTESIAN_POINT('Ctrl Pts',(-6.37480463932049,2.73653622817309,
3.624730852095));
#105197=CARTESIAN_POINT('Ctrl Pts',(-6.44734506632474,2.72356451355148,
3.66571849367625));
#105198=CARTESIAN_POINT('Ctrl Pts',(-6.48368414002074,2.71723336288666,
3.68618951759012));
#105199=CARTESIAN_POINT('Ctrl Pts',(-6.5200454043226,2.71105259878665,3.70661677591662));
#105200=CARTESIAN_POINT('',(-6.71839607196138,2.62129679787127,3.03656388084945));
#105201=CARTESIAN_POINT('Ctrl Pts',(-6.304696317,2.750764179,3.579567621));
#105202=CARTESIAN_POINT('Ctrl Pts',(-6.110733509,2.686419405,3.921194524));
#105203=CARTESIAN_POINT('Ctrl Pts',(-5.880991895,2.621296797,4.239862537));
#105204=CARTESIAN_POINT('Ctrl Pts',(-6.640032775,2.750764179,3.4871141));
#105205=CARTESIAN_POINT('Ctrl Pts',(-6.451079663,2.686419405,3.846911578));
#105206=CARTESIAN_POINT('Ctrl Pts',(-6.224354992,2.621296797,4.184185097));
#105207=CARTESIAN_POINT('',(-6.22435498239899,2.62129679632898,4.18418508963427));
#105208=CARTESIAN_POINT('Origin',(0.151852228411307,2.55359611104798,-0.115179169971752));
#105209=CARTESIAN_POINT('',(-6.05267345033977,2.62129679507543,4.21202380717125));
#105210=CARTESIAN_POINT('Origin',(-7.40293243373102E-13,2.71213386200011,
4.58617518961368E-13));
#105211=CARTESIAN_POINT('',(-6.52364787172068,2.53084202044609,3.70027275230428));
#105212=CARTESIAN_POINT('Origin',(0.169668428985089,2.55357152054945,-0.0920471349585866));
#105213=CARTESIAN_POINT('Origin',(0.171861648752537,2.410790211888,-0.0753995501951926));
#105214=CARTESIAN_POINT('Ctrl Pts',(-5.89112306978218,2.61844385790313,
4.22525055585264));
#105215=CARTESIAN_POINT('Ctrl Pts',(-5.88602055030678,2.61987032745155,
4.23232878604296));
#105216=CARTESIAN_POINT('Ctrl Pts',(-5.88091803083135,2.621296797,4.23940701623327));
#105217=CARTESIAN_POINT('Ctrl Pts',(-5.77797706175249,2.65007516,4.38220703466827));
#105218=CARTESIAN_POINT('Ctrl Pts',(-5.66822657968978,2.678571429,4.51984249406189));
#105219=CARTESIAN_POINT('Ctrl Pts',(-5.52604355212437,2.71548867684756,
4.69815083468151));
#105220=CARTESIAN_POINT('Ctrl Pts',(-5.37293446337063,2.75286253698008,
4.86717001809344));
#105221=CARTESIAN_POINT('Ctrl Pts',(-5.94770200808611,2.6184438579031,4.5689349698406));
#105222=CARTESIAN_POINT('Ctrl Pts',(-5.94218567104306,2.61987032745156,
4.5760803019203));
#105223=CARTESIAN_POINT('Ctrl Pts',(-5.93666933400001,2.621296797,4.583225634));
#105224=CARTESIAN_POINT('Ctrl Pts',(-5.825379787,2.65007516,4.727379402));
#105225=CARTESIAN_POINT('Ctrl Pts',(-5.707224861,2.678571429,4.865961815));
#105226=CARTESIAN_POINT('Ctrl Pts',(-5.55415377879304,2.71548867684756,
5.04549694470018));
#105227=CARTESIAN_POINT('Ctrl Pts',(-5.39010105545041,2.75286253698008,
5.21505614693326));
#105228=CARTESIAN_POINT('',(-5.93666933833169,2.62129679728565,4.58322562730095));
#105229=CARTESIAN_POINT('',(-5.90855223050183,2.62129679787124,4.4098272657317));
#105230=CARTESIAN_POINT('',(-5.57079732493823,2.71105259873791,5.02157516776287));
#105231=CARTESIAN_POINT('Ctrl Pts',(-5.93666933920874,2.62129679564635,
4.58322562705902));
#105232=CARTESIAN_POINT('Ctrl Pts',(-5.86231715742261,2.64052352569896,
4.67953428736928));
#105233=CARTESIAN_POINT('Ctrl Pts',(-5.78577989171214,2.65962575012079,
4.77382561658219));
#105234=CARTESIAN_POINT('Ctrl Pts',(-5.70722486025002,2.67857142918088,
4.86596181587965));
#105235=CARTESIAN_POINT('Ctrl Pts',(-5.66253420708315,2.68934979368581,
4.91837891579501));
#105236=CARTESIAN_POINT('Ctrl Pts',(-5.6170518883089,2.70017879535638,4.97026162768578));
#105237=CARTESIAN_POINT('Ctrl Pts',(-5.57079732239259,2.71105259957952,
5.02157517044642));
#105238=CARTESIAN_POINT('Ctrl Pts',(-5.38467194878181,2.74999999876017,
4.85466869228265));
#105239=CARTESIAN_POINT('Ctrl Pts',(-5.4155737925532,2.74318451268803,4.88252892416039));
#105240=CARTESIAN_POINT('Ctrl Pts',(-5.4465552624774,2.73653622823916,4.91038121837523));
#105241=CARTESIAN_POINT('Ctrl Pts',(-5.50858833841322,2.72356456892389,
4.96600440205996));
#105242=CARTESIAN_POINT('Ctrl Pts',(-5.53967685772086,2.71723347543569,
4.99380838334581));
#105243=CARTESIAN_POINT('Ctrl Pts',(-5.57079732597209,2.71105259874038,
5.02157516660469));
#105244=CARTESIAN_POINT('Origin',(5.79397640976254E-13,2.71213386199956,
-3.17454396103756E-13));
#105245=CARTESIAN_POINT('',(-5.17935692493163,2.62129679635372,5.42441350133401));
#105246=CARTESIAN_POINT('Origin',(0.123545161789753,2.55359537855859,-0.145133198604221));
#105247=CARTESIAN_POINT('',(-5.57567934709768,2.53084202101785,5.01615388628296));
#105248=CARTESIAN_POINT('Origin',(0.145914194189911,2.55357152512524,-0.126368749652749));
#105249=CARTESIAN_POINT('Origin',(0.151637948404064,2.41079127387234,-0.110584830266146));
#105250=CARTESIAN_POINT('Ctrl Pts',(-5.387794793,2.750764179,4.851202662));
#105251=CARTESIAN_POINT('Ctrl Pts',(-5.124927042,2.686419405,5.143146247));
#105252=CARTESIAN_POINT('Ctrl Pts',(-4.832052457,2.621296797,5.404976323));
#105253=CARTESIAN_POINT('Ctrl Pts',(-5.73516604600001,2.750764179,4.832998079));
#105254=CARTESIAN_POINT('Ctrl Pts',(-5.47328473,2.686419405,5.143764358));
#105255=CARTESIAN_POINT('Ctrl Pts',(-5.179356919,2.621296797,5.424413508));
#105256=CARTESIAN_POINT('',(-5.00570469679279,2.62129679507542,5.41469490737137));
#105257=CARTESIAN_POINT('Ctrl Pts',(-4.84508791585569,2.61844385761768,
5.39288386372956));
#105258=CARTESIAN_POINT('Ctrl Pts',(-4.8385830795463,2.61987032730884,5.39869971856641));
#105259=CARTESIAN_POINT('Ctrl Pts',(-4.83207824323687,2.621296797,5.40451557340326));
#105260=CARTESIAN_POINT('Ctrl Pts',(-4.70084619412413,2.65007516,5.5218477415437));
#105261=CARTESIAN_POINT('Ctrl Pts',(-4.56407406143641,2.678571429,5.63267225195145));
#105262=CARTESIAN_POINT('Ctrl Pts',(-4.38688417180961,2.71548867690094,
5.7762466942276));
#105263=CARTESIAN_POINT('Ctrl Pts',(-4.20102055862152,2.75286253708806,
5.90840037550124));
#105264=CARTESIAN_POINT('Ctrl Pts',(-4.82646208002768,2.61844385761768,
5.74069592738241));
#105265=CARTESIAN_POINT('Ctrl Pts',(-4.81953867601382,2.61987032730884,
5.7464883566912));
#105266=CARTESIAN_POINT('Ctrl Pts',(-4.812615272,2.621296797,5.752280786));
#105267=CARTESIAN_POINT('Ctrl Pts',(-4.672938814,2.65007516,5.86914035499999));
#105268=CARTESIAN_POINT('Ctrl Pts',(-4.527755162,2.678571429,5.979082973));
#105269=CARTESIAN_POINT('Ctrl Pts',(-4.33966805013464,2.71548867690094,
6.12151491333678));
#105270=CARTESIAN_POINT('Ctrl Pts',(-4.1430005717275,2.75286253708806,6.25184342861707));
#105271=CARTESIAN_POINT('',(-4.81261527767175,2.62129679728565,5.75228078036772));
#105272=CARTESIAN_POINT('',(-4.36106495481695,2.71105259870975,6.10173028400751));
#105273=CARTESIAN_POINT('Ctrl Pts',(-4.81261527857913,2.62129679564633,
5.75228078034081));
#105274=CARTESIAN_POINT('Ctrl Pts',(-4.71929789451606,2.64052352569892,
5.83035427570691));
#105275=CARTESIAN_POINT('Ctrl Pts',(-4.62428017899786,2.65962575012086,
5.90598787639623));
#105276=CARTESIAN_POINT('Ctrl Pts',(-4.52775516105093,2.67857142919243,
5.97908297344371));
#105277=CARTESIAN_POINT('Ctrl Pts',(-4.47284122339138,2.68934979369743,
6.02066742111355));
#105278=CARTESIAN_POINT('Ctrl Pts',(-4.41726900647831,2.70017879535494,
6.06155979027765));
#105279=CARTESIAN_POINT('Ctrl Pts',(-4.36106495158897,2.71105259959617,
6.10173028644538));
#105280=CARTESIAN_POINT('Ctrl Pts',(-4.21517104455419,2.74999999871542,
5.89871453534225));
#105281=CARTESIAN_POINT('Ctrl Pts',(-4.23936129417448,2.74318451269066,
5.93256639331657));
#105282=CARTESIAN_POINT('Ctrl Pts',(-4.26363101473255,2.73653622824346,
5.96642761659724));
#105283=CARTESIAN_POINT('Ctrl Pts',(-4.31225643993011,2.72356457207071,
6.03408562230802));
#105284=CARTESIAN_POINT('Ctrl Pts',(-4.33664107949827,2.71723348180313,
6.06792265611851));
#105285=CARTESIAN_POINT('Ctrl Pts',(-4.36106495617808,2.71105259871231,
6.10173028302464));
#105286=CARTESIAN_POINT('',(-4.82243105446794,2.62129679787126,5.57689202868901));
#105287=CARTESIAN_POINT('Origin',(6.75457953458469E-13,2.71213386199944,
-9.74914593498966E-13));
#105288=CARTESIAN_POINT('',(-4.36699825425421,2.53084202105883,6.09748523951929));
#105289=CARTESIAN_POINT('Origin',(0.115337245586927,2.55357151413217,-0.154781541207575));
#105290=CARTESIAN_POINT('',(-3.89217788024747,2.62129679635372,6.41100236577101));
#105291=CARTESIAN_POINT('Origin',(0.124320393779957,2.41079130932435,-0.140597308762092));
#105292=CARTESIAN_POINT('Origin',(0.0894574468630682,2.55359537224088,-0.168298698688354));
#105293=CARTESIAN_POINT('Ctrl Pts',(-4.218965973,2.750764179,5.896000858));
#105294=CARTESIAN_POINT('Ctrl Pts',(-3.899484683,2.686419405,6.12461016899999));
#105295=CARTESIAN_POINT('Ctrl Pts',(-3.557171616,2.621296797,6.317359424));
#105296=CARTESIAN_POINT('Ctrl Pts',(-4.562129326,2.750764179,5.95289643900001));
#105297=CARTESIAN_POINT('Ctrl Pts',(-4.239565086,2.686419405,6.200100433));
#105298=CARTESIAN_POINT('Ctrl Pts',(-3.892177873,2.621296797,6.411002371));
#105299=CARTESIAN_POINT('',(-3.72467475483459,2.62129679507543,6.36418089145162));
#105300=CARTESIAN_POINT('Ctrl Pts',(-3.57250182821409,2.61844385875657,
6.3083519216686));
#105301=CARTESIAN_POINT('Ctrl Pts',(-3.56489883753746,2.6198703278783,6.31263345580127));
#105302=CARTESIAN_POINT('Ctrl Pts',(-3.55729584686083,2.621296797,6.31691498993395));
#105303=CARTESIAN_POINT('Ctrl Pts',(-3.40390898257575,2.65007516,6.40329298549838));
#105304=CARTESIAN_POINT('Ctrl Pts',(-3.24651051216236,2.678571429,6.48212451528638));
#105305=CARTESIAN_POINT('Ctrl Pts',(-3.04259896514593,2.71548867637279,
6.58425167726325));
#105306=CARTESIAN_POINT('Ctrl Pts',(-2.83267160933287,2.75286253601974,
6.67336049472692));
#105307=CARTESIAN_POINT('Ctrl Pts',(-3.47954214211268,2.61844385875657,
6.64402832764031));
#105308=CARTESIAN_POINT('Ctrl Pts',(-3.47153540555634,2.6198703278783,6.64819700432017));
#105309=CARTESIAN_POINT('Ctrl Pts',(-3.463528669,2.621296797,6.652365681));
#105310=CARTESIAN_POINT('Ctrl Pts',(-3.301996416,2.65007516,6.736466829));
#105311=CARTESIAN_POINT('Ctrl Pts',(-3.136572664,2.678571429,6.812628856));
#105312=CARTESIAN_POINT('Ctrl Pts',(-2.9222642706896,2.71548867637279,6.9112976463071));
#105313=CARTESIAN_POINT('Ctrl Pts',(-2.70217799339193,2.75286253601974,
6.99630145831613));
#105314=CARTESIAN_POINT('',(-3.46352867574623,2.62129679728566,6.65236567673181));
#105315=CARTESIAN_POINT('',(-2.94741403486585,2.71105259872076,6.89657527394903));
#105316=CARTESIAN_POINT('Ctrl Pts',(-3.46352867664184,2.62129679564635,
6.65236567688735));
#105317=CARTESIAN_POINT('Ctrl Pts',(-3.35560950750809,2.6405235256989,6.7085533784849));
#105318=CARTESIAN_POINT('Ctrl Pts',(-3.24655426491184,2.65962575012075,
6.76199270759947));
#105319=CARTESIAN_POINT('Ctrl Pts',(-3.13657266304808,2.67857142917358,
6.81262885629644));
#105320=CARTESIAN_POINT('Ctrl Pts',(-3.07400315580616,2.68934979367116,
6.84143620945174));
#105321=CARTESIAN_POINT('Ctrl Pts',(-3.01093953572748,2.70017879536706,
6.86942615381242));
#105322=CARTESIAN_POINT('Ctrl Pts',(-2.9474140310964,2.71105259962305,6.89657527580879));
#105323=CARTESIAN_POINT('Ctrl Pts',(-2.84857342825316,2.74999999861341,
6.66694304341797));
#105324=CARTESIAN_POINT('Ctrl Pts',(-2.86492097448018,2.7431845125352,6.70520365250962));
#105325=CARTESIAN_POINT('Ctrl Pts',(-2.88134412019263,2.73653622816043,
6.74349049123379));
#105326=CARTESIAN_POINT('Ctrl Pts',(-2.91428838878775,2.72356451291915,
6.82002006788017));
#105327=CARTESIAN_POINT('Ctrl Pts',(-2.93082913926675,2.71723336163927,
6.85830838235346));
#105328=CARTESIAN_POINT('Ctrl Pts',(-2.94741403646363,2.71105259872334,
6.89657527325697));
#105329=CARTESIAN_POINT('',(-3.51081836193504,2.62129679787127,6.48318751866981));
#105330=CARTESIAN_POINT('Origin',(-2.53052787058117E-13,2.71213386199933,
6.99093560818653E-13));
#105331=CARTESIAN_POINT('',(-2.95412117554163,2.53084202101381,6.89370496034607));
#105332=CARTESIAN_POINT('Origin',(0.079367334413924,2.55357147941704,-0.175957076628545));
#105333=CARTESIAN_POINT('',(-2.42300492349163,2.62129679634651,7.09781988531365));
#105334=CARTESIAN_POINT('Origin',(0.0911895360214926,2.41079130469772,-0.164035304077856));
#105335=CARTESIAN_POINT('Origin',(0.0511867591664122,2.55359538632789,-0.183594736051459));
#105336=CARTESIAN_POINT('Ctrl Pts',(-2.852862993,2.750764179,6.665108607));
#105337=CARTESIAN_POINT('Ctrl Pts',(-2.491706754,2.686419405,6.819694125));
#105338=CARTESIAN_POINT('Ctrl Pts',(-2.115961384,2.621296797,6.93434982));
#105339=CARTESIAN_POINT('Ctrl Pts',(-3.17577251,2.750764179,6.79444397800001));
#105340=CARTESIAN_POINT('Ctrl Pts',(-2.807608091,2.686419405,6.966526703));
#105341=CARTESIAN_POINT('Ctrl Pts',(-2.423004915,2.621296797,7.097819889));
#105342=CARTESIAN_POINT('',(-2.26948316089319,2.62129679507543,7.01608485081466));
#105343=CARTESIAN_POINT('Ctrl Pts',(-2.13286953419124,2.61844385824803,
6.92884844960035));
#105344=CARTESIAN_POINT('Ctrl Pts',(-2.12452389241223,2.61987032762403,
6.93139546602818));
#105345=CARTESIAN_POINT('Ctrl Pts',(-2.11617825063324,2.621296797,6.93394248245604));
#105346=CARTESIAN_POINT('Ctrl Pts',(-1.94780876957162,2.65007516,6.98532736639538));
#105347=CARTESIAN_POINT('Ctrl Pts',(-1.7771437402721,2.678571429,7.02847984018819));
#105348=CARTESIAN_POINT('Ctrl Pts',(-1.55604521013484,2.71548867650565,
7.08438437089874));
#105349=CARTESIAN_POINT('Ctrl Pts',(-1.33187007596143,2.75286253628849,
7.12628169757759));
#105350=CARTESIAN_POINT('Ctrl Pts',(-1.96992268858995,2.61844385824803,
7.23669334289097));
#105351=CARTESIAN_POINT('Ctrl Pts',(-1.96120700129498,2.61987032762403,
7.23904334694548));
#105352=CARTESIAN_POINT('Ctrl Pts',(-1.952491314,2.621296797,7.241393351));
#105353=CARTESIAN_POINT('Ctrl Pts',(-1.776656335,2.65007516,7.288803601));
#105354=CARTESIAN_POINT('Ctrl Pts',(-1.598727514,2.678571429,7.327623785));
#105355=CARTESIAN_POINT('Ctrl Pts',(-1.36821865771831,2.71548867650565,
7.37791578420156));
#105356=CARTESIAN_POINT('Ctrl Pts',(-1.13500456736235,2.75286253628849,
7.41362021130129));
#105357=CARTESIAN_POINT('',(-1.95249132150711,2.62129679728565,7.24139334827985));
#105358=CARTESIAN_POINT('',(-1.39594530977112,2.71105259875627,7.36894406900818));
#105359=CARTESIAN_POINT('Ctrl Pts',(-1.95249132234728,2.62129679564634,
7.24139334862629));
#105360=CARTESIAN_POINT('Ctrl Pts',(-1.83501654880178,2.64052352569891,
7.27306798144823));
#105361=CARTESIAN_POINT('Ctrl Pts',(-1.71702308126209,2.65962575012074,
7.30181427500216));
#105362=CARTESIAN_POINT('Ctrl Pts',(-1.59872751298808,2.67857142917097,
7.32762378513971));
#105363=CARTESIAN_POINT('Ctrl Pts',(-1.53142811659933,2.68934979367611,
7.34230704387087));
#105364=CARTESIAN_POINT('Ctrl Pts',(-1.46382187832016,2.70017879536824,
7.35608578463689));
#105365=CARTESIAN_POINT('Ctrl Pts',(-1.3959453061231,2.71105259959742,7.36894406960316));
#105366=CARTESIAN_POINT('Ctrl Pts',(-1.34877968348022,2.74999999856131,
7.12343270341778));
#105367=CARTESIAN_POINT('Ctrl Pts',(-1.35652013322406,2.74318451250953,
7.16431304003367));
#105368=CARTESIAN_POINT('Ctrl Pts',(-1.36432877629888,2.73653622815752,
7.20523524465526));
#105369=CARTESIAN_POINT('Ctrl Pts',(-1.38005116146527,2.7235645688885,7.2870572934719));
#105370=CARTESIAN_POINT('Ctrl Pts',(-1.3879742635373,2.71723347545156,7.32800582015948));
#105371=CARTESIAN_POINT('Ctrl Pts',(-1.39594531129452,2.71105259875875,
7.36894406871193));
#105372=CARTESIAN_POINT('',(-2.03504370448729,2.62129679787127,7.08633636636968));
#105373=CARTESIAN_POINT('Origin',(-1.04083408558608E-14,2.71213386200022,
7.84528692010511E-13));
#105374=CARTESIAN_POINT('',(-1.40311267351609,2.53084202107002,7.36758269877174));
#105375=CARTESIAN_POINT('Origin',(0.0396862191300584,2.55357152508889,-0.188904991491554));
#105376=CARTESIAN_POINT('',(-0.84053494974635,2.62129679635371,7.45275123627453));
#105377=CARTESIAN_POINT('Origin',(0.0537948407454188,2.41079129773833,-0.179803285552214));
#105378=CARTESIAN_POINT('Origin',(0.0105225792016134,2.55359538998345,-0.190305860738225));
#105379=CARTESIAN_POINT('Ctrl Pts',(-1.353363311,2.750764179,7.122563285));
#105380=CARTESIAN_POINT('Ctrl Pts',(-0.967419387,2.686419405,7.195896764));
#105381=CARTESIAN_POINT('Ctrl Pts',(-0.575811149000001,2.621296797,7.227097725));
#105382=CARTESIAN_POINT('Ctrl Pts',(-1.6409201,2.750764179,7.318290868));
#105383=CARTESIAN_POINT('Ctrl Pts',(-1.244370462,2.686419405,7.407205928));
#105384=CARTESIAN_POINT('Ctrl Pts',(-0.840534941,2.621296797,7.452751238));
#105385=CARTESIAN_POINT('',(-0.708173056919068,2.62129679507543,7.33992448035002));
#105386=CARTESIAN_POINT('Origin',(-4.32596666821716E-14,2.71213386200078,
-8.20090523268036E-13));
#105387=CARTESIAN_POINT('',(0.213503817067297,2.53084202106192,7.49696045860213));
#105388=CARTESIAN_POINT('',(-0.350157640963255,2.62129679727531,7.49182151570119));
#105389=CARTESIAN_POINT('Origin',(-0.00185061631064444,2.55357152007291,
-0.193019680036474));
#105390=CARTESIAN_POINT('Origin',(0.0138847566166005,2.41079128748424,-0.18716392002421));
#105391=CARTESIAN_POINT('Ctrl Pts',(-0.350157644662314,2.62129679564685,
7.49182151547269));
#105392=CARTESIAN_POINT('Ctrl Pts',(-0.228620255756217,2.64052352569912,
7.49750200929352));
#105393=CARTESIAN_POINT('Ctrl Pts',(-0.107205806305265,2.65962575012073,
7.500211122968));
#105394=CARTESIAN_POINT('Ctrl Pts',(0.013872358933994,2.67857142917026,
7.49998717083406));
#105395=CARTESIAN_POINT('Ctrl Pts',(0.0827547991821888,2.68934979367005,
7.49985976220329));
#105396=CARTESIAN_POINT('Ctrl Pts',(0.151742463241413,2.70017879538175,
7.49878302093725));
#105397=CARTESIAN_POINT('Ctrl Pts',(0.220796270213227,2.71105259965551,
7.49674922963173));
#105398=CARTESIAN_POINT('Ctrl Pts',(-0.593506707015565,2.61844384550212,
7.2253597183345));
#105399=CARTESIAN_POINT('Ctrl Pts',(-0.584808609650274,2.61987032125107,
7.2260531237281));
#105400=CARTESIAN_POINT('Ctrl Pts',(-0.576110512284988,2.621296797,7.22674652912171));
#105401=CARTESIAN_POINT('Ctrl Pts',(-0.400631185997974,2.65007516,7.24073560123764));
#105402=CARTESIAN_POINT('Ctrl Pts',(-0.224679703852224,2.678571429,7.24619125768236));
#105403=CARTESIAN_POINT('Ctrl Pts',(0.0032675322255622,2.71548868380392,
7.25325912441818));
#105404=CARTESIAN_POINT('Ctrl Pts',(0.231208307768356,2.75286255105096,
7.24598588434386));
#105405=CARTESIAN_POINT('Ctrl Pts',(-0.368191918198986,2.61844384550211,
7.4909786179583));
#105406=CARTESIAN_POINT('Ctrl Pts',(-0.359174777099492,2.61987032125107,
7.49140006697913));
#105407=CARTESIAN_POINT('Ctrl Pts',(-0.350157636,2.621296797,7.491821516));
#105408=CARTESIAN_POINT('Ctrl Pts',(-0.168241778,2.65007516,7.500324018));
#105409=CARTESIAN_POINT('Ctrl Pts',(0.013872358,2.678571429,7.499987171));
#105410=CARTESIAN_POINT('Ctrl Pts',(0.249803384602647,2.71548868380392,
7.49955078075478));
#105411=CARTESIAN_POINT('Ctrl Pts',(0.48524050162808,2.75286255105096,7.48428631606375));
#105412=CARTESIAN_POINT('',(-0.464112665399334,2.62129679787127,7.35813600120854));
#105413=CARTESIAN_POINT('Ctrl Pts',(-1.16100722477529,3.26861999521842,
7.40959699727959));
#105414=CARTESIAN_POINT('Ctrl Pts',(-1.15701056188764,3.26797796010921,
7.41021881713979));
#105415=CARTESIAN_POINT('Ctrl Pts',(-1.153013899,3.267335925,7.410840637));
#105416=CARTESIAN_POINT('Ctrl Pts',(-0.751738269,3.202873885,7.473273012));
#105417=CARTESIAN_POINT('Ctrl Pts',(-0.346067467,3.137747733,7.492011566));
#105418=CARTESIAN_POINT('Ctrl Pts',(-1.35660408902388,3.26861999521842,
7.12195103128405));
#105419=CARTESIAN_POINT('Ctrl Pts',(-1.35276243951194,3.26797796010921,
7.12267850364203));
#105420=CARTESIAN_POINT('Ctrl Pts',(-1.34892079,3.267335925,7.123405976));
#105421=CARTESIAN_POINT('Ctrl Pts',(-0.963208917,3.202873885,7.196446144));
#105422=CARTESIAN_POINT('Ctrl Pts',(-0.571865472,3.137747733,7.227411008));
#105423=CARTESIAN_POINT('',(-0.594693634847874,3.1776659463463,7.47638545564978));
#105424=CARTESIAN_POINT('Ctrl Pts',(-0.594693636545437,3.17766594630611,
7.47638545543473));
#105425=CARTESIAN_POINT('Ctrl Pts',(-0.591699897737181,3.17146450644349,
7.43478416571922));
#105426=CARTESIAN_POINT('Ctrl Pts',(-0.588689435224447,3.16510742592506,
7.39318254135156));
#105427=CARTESIAN_POINT('Ctrl Pts',(-0.582639747481574,3.15207191348099,
7.31008139669812));
#105428=CARTESIAN_POINT('Ctrl Pts',(-0.579596922089708,3.14538572802115,
7.2685323944097));
#105429=CARTESIAN_POINT('Ctrl Pts',(-0.576538527513735,3.13852541804481,
7.22703973443035));
#105430=CARTESIAN_POINT('',(-1.1530138984719,3.26733592582627,7.41084061853901));
#105431=CARTESIAN_POINT('Origin',(0.000867139836089673,3.08932518850483,
-0.18957817087375));
#105432=CARTESIAN_POINT('',(-1.25096733006107,3.2673359273533,7.26712330898553));
#105433=CARTESIAN_POINT('Ctrl Pts',(-2.428381113,3.13774478,7.095982326));
#105434=CARTESIAN_POINT('Ctrl Pts',(-2.198434563,3.176256335,7.174674441));
#105435=CARTESIAN_POINT('Ctrl Pts',(-1.963875725,3.214285714,7.238314178));
#105436=CARTESIAN_POINT('Ctrl Pts',(-1.80102675,3.240688665,7.282497829));
#105437=CARTESIAN_POINT('Ctrl Pts',(-1.63635545,3.267335925,7.319312867));
#105438=CARTESIAN_POINT('Ctrl Pts',(-1.63233139552941,3.26798710116569,
7.32021251203984));
#105439=CARTESIAN_POINT('Ctrl Pts',(-1.62830734105882,3.26863827733136,
7.32111215707968));
#105440=CARTESIAN_POINT('Ctrl Pts',(-2.121213834,3.13774478,6.932744901));
#105441=CARTESIAN_POINT('Ctrl Pts',(-1.896557022,3.176256335,7.001483207));
#105442=CARTESIAN_POINT('Ctrl Pts',(-1.667921256,3.214285714,7.055532488));
#105443=CARTESIAN_POINT('Ctrl Pts',(-1.509184538,3.240688665,7.093057699));
#105444=CARTESIAN_POINT('Ctrl Pts',(-1.34892079,3.267335925,7.123405976));
#105445=CARTESIAN_POINT('Ctrl Pts',(-1.34500444239351,3.26798710116569,
7.12414759351159));
#105446=CARTESIAN_POINT('Ctrl Pts',(-1.34108809478702,3.26863827733136,
7.12488921102319));
#105447=CARTESIAN_POINT('',(-1.63635545054765,3.26733592550877,7.31931286465442));
#105448=CARTESIAN_POINT('',(-1.49263812863747,3.26733592642396,7.22135941971466));
#105449=CARTESIAN_POINT('',(-2.18799190370241,3.17766594629541,7.17375016484504));
#105450=CARTESIAN_POINT('Ctrl Pts',(-1.636355450892,3.26733592483458,7.31931286668268));
#105451=CARTESIAN_POINT('Ctrl Pts',(-1.74635892260571,3.24953506265028,
7.29471974078576));
#105452=CARTESIAN_POINT('Ctrl Pts',(-1.85558425339799,3.23184317427157,
7.26769546538249));
#105453=CARTESIAN_POINT('Ctrl Pts',(-1.96387572495971,3.2142857139293,7.23831417758749));
#105454=CARTESIAN_POINT('Ctrl Pts',(-2.03878453707537,3.20214063496436,
7.21799016354287));
#105455=CARTESIAN_POINT('Ctrl Pts',(-2.1135088847609,3.18993125792355,7.19646746595664));
#105456=CARTESIAN_POINT('Ctrl Pts',(-2.18799190370039,3.1776659461067,7.17375016494029));
#105457=CARTESIAN_POINT('Ctrl Pts',(-2.11665929066702,3.1385254181032,6.93413682049357));
#105458=CARTESIAN_POINT('Ctrl Pts',(-2.12856581114192,3.1453856901219,6.97400172021665));
#105459=CARTESIAN_POINT('Ctrl Pts',(-2.14046922882565,3.15207183606137,
7.01392495842331));
#105460=CARTESIAN_POINT('Ctrl Pts',(-2.1642418900651,3.16510741554023,7.09378315124004));
#105461=CARTESIAN_POINT('Ctrl Pts',(-2.17612506755813,3.17146448527804,
7.13376491949633));
#105462=CARTESIAN_POINT('Ctrl Pts',(-2.18799190244371,3.17766594628736,
7.17375016518307));
#105463=CARTESIAN_POINT('Ctrl Pts',(-2.72670784948992,3.26861999521842,
6.98678250313633));
#105464=CARTESIAN_POINT('Ctrl Pts',(-2.72293829924496,3.26797796010921,
6.98824894956816));
#105465=CARTESIAN_POINT('Ctrl Pts',(-2.719168749,3.267335925,6.989715396));
#105466=CARTESIAN_POINT('Ctrl Pts',(-2.340695835,3.202873885,7.136950535));
#105467=CARTESIAN_POINT('Ctrl Pts',(-1.948537627,3.137747733,7.242458223));
#105468=CARTESIAN_POINT('Ctrl Pts',(-2.85589638766259,3.26861999521842,
6.6638139959214));
#105469=CARTESIAN_POINT('Ctrl Pts',(-2.85230093883129,3.26797796010921,
6.66535030146071));
#105470=CARTESIAN_POINT('Ctrl Pts',(-2.84870549,3.267335925,6.666886607));
#105471=CARTESIAN_POINT('Ctrl Pts',(-2.487712823,3.202873885,6.821135787));
#105472=CARTESIAN_POINT('Ctrl Pts',(-2.112175301,3.137747733,6.935503983));
#105473=CARTESIAN_POINT('',(-2.71916874452873,3.26733592582611,6.9897153780778));
#105474=CARTESIAN_POINT('Origin',(0.0416006174824163,3.08932515708654,-0.184959702196723));
#105475=CARTESIAN_POINT('',(-2.78393710593565,3.26733592735283,6.82830100703027));
#105476=CARTESIAN_POINT('Origin',(-5.48606299277665E-14,3.35806380000056,
2.30284541435921E-13));
#105477=CARTESIAN_POINT('',(-2.18598964806097,3.35698786818065,7.17436054673024));
#105478=CARTESIAN_POINT('Origin',(0.0119076089957454,3.08947598352193,-0.182881204940006));
#105479=CARTESIAN_POINT('Origin',(0.0351660334599163,3.48205906984505,-0.184035505550071));
#105480=CARTESIAN_POINT('Ctrl Pts',(-3.897033357,3.13774478,6.40805204500001));
#105481=CARTESIAN_POINT('Ctrl Pts',(-3.689379308,3.176256335,6.534336094));
#105482=CARTESIAN_POINT('Ctrl Pts',(-3.473984987,3.214285714,6.646911186));
#105483=CARTESIAN_POINT('Ctrl Pts',(-3.324441509,3.240688665,6.725069564));
#105484=CARTESIAN_POINT('Ctrl Pts',(-3.171534278,3.267335925,6.79642334800001));
#105485=CARTESIAN_POINT('Ctrl Pts',(-3.16779770079139,3.26798710116568,
6.7981670125821));
#105486=CARTESIAN_POINT('Ctrl Pts',(-3.16406112358279,3.26863827733137,
6.79991067716421));
#105487=CARTESIAN_POINT('Ctrl Pts',(-3.561956257,3.13774478,6.314662906));
#105488=CARTESIAN_POINT('Ctrl Pts',(-3.3573285,3.176256335,6.43008872300001));
#105489=CARTESIAN_POINT('Ctrl Pts',(-3.145657109,3.214285714,6.532024292));
#105490=CARTESIAN_POINT('Ctrl Pts',(-2.998698378,3.240688665,6.602795887));
#105491=CARTESIAN_POINT('Ctrl Pts',(-2.84870549,3.267335925,6.666886607));
#105492=CARTESIAN_POINT('Ctrl Pts',(-2.84504013027117,3.26798710116568,
6.66845278488491));
#105493=CARTESIAN_POINT('Ctrl Pts',(-2.84137477054235,3.26863827733137,
6.67001896276982));
#105494=CARTESIAN_POINT('',(-3.17153427803867,3.26733592550877,6.79642334559096));
#105495=CARTESIAN_POINT('',(-3.01011989205177,3.26733592642396,6.73165497389958));
#105496=CARTESIAN_POINT('',(-3.67898209978803,3.17766594630002,6.53567828967424));
#105497=CARTESIAN_POINT('Ctrl Pts',(-3.17153427880971,3.26733592483345,
6.79642334749546));
#105498=CARTESIAN_POINT('Ctrl Pts',(-3.27367913498392,3.24953506265028,
6.74875770096114));
#105499=CARTESIAN_POINT('Ctrl Pts',(-3.37454141781148,3.23184317427167,
6.6988850207741));
#105500=CARTESIAN_POINT('Ctrl Pts',(-3.47398498685941,3.21428571394846,
6.64691118569608));
#105501=CARTESIAN_POINT('Ctrl Pts',(-3.54277341033584,3.20214063502602,
6.61095915563011));
#105502=CARTESIAN_POINT('Ctrl Pts',(-3.6111240004649,3.18993125796488,6.57387612060236));
#105503=CARTESIAN_POINT('Ctrl Pts',(-3.6789820999354,3.17766594614085,6.53567828998717));
#105504=CARTESIAN_POINT('Ctrl Pts',(-3.55780741732562,3.13852541817353,
6.31700137554185));
#105505=CARTESIAN_POINT('Ctrl Pts',(-3.57800534213567,3.14538568922323,
6.35337470099805));
#105506=CARTESIAN_POINT('Ctrl Pts',(-3.59821277736713,3.1520718341465,6.38980566719298));
#105507=CARTESIAN_POINT('Ctrl Pts',(-3.63859680666803,3.16510741642552,
6.46268641610141));
#105508=CARTESIAN_POINT('Ctrl Pts',(-3.65879706345997,3.17146448703467,
6.49917890637104));
#105509=CARTESIAN_POINT('Ctrl Pts',(-3.67898209852761,3.17766594627311,
6.53567829018584));
#105510=CARTESIAN_POINT('Ctrl Pts',(-4.16491064522116,3.26861999521842,
6.23727382379452));
#105511=CARTESIAN_POINT('Ctrl Pts',(-4.16154446761058,3.26797796010921,
6.23951632739726));
#105512=CARTESIAN_POINT('Ctrl Pts',(-4.15817829,3.267335925,6.241758831));
#105513=CARTESIAN_POINT('Ctrl Pts',(-3.820205066,3.202873885,6.466912183));
#105514=CARTESIAN_POINT('Ctrl Pts',(-3.459896332,3.137747733,6.654255583));
#105515=CARTESIAN_POINT('Ctrl Pts',(-4.2216501449166,3.26861999521842,5.8940844244334));
#105516=CARTESIAN_POINT('Ctrl Pts',(-4.2184690159583,3.26797796010921,5.89635772721671));
#105517=CARTESIAN_POINT('Ctrl Pts',(-4.215287887,3.267335925,5.89863103000001));
#105518=CARTESIAN_POINT('Ctrl Pts',(-3.895894042,3.202873885,6.126876702));
#105519=CARTESIAN_POINT('Ctrl Pts',(-3.55372216,3.137747733,6.3193005));
#105520=CARTESIAN_POINT('',(-4.15817828176499,3.26733592582611,6.24175881447829));
#105521=CARTESIAN_POINT('Origin',(0.0803888520133322,3.08932521734779,-0.171692463230565));
#105522=CARTESIAN_POINT('',(-4.18673307644162,3.26733592735283,6.07019493881691));
#105523=CARTESIAN_POINT('Origin',(-3.03576608295941E-14,3.35806380000022,
6.24500451351651E-14));
#105524=CARTESIAN_POINT('',(-3.67715786962144,3.35698786820061,6.53670482762012));
#105525=CARTESIAN_POINT('Origin',(0.050943447341012,3.08947602065486,-0.17604612105504));
#105526=CARTESIAN_POINT('Origin',(0.0739062462862405,3.48205903813151,-0.172173467210209));
#105527=CARTESIAN_POINT('Ctrl Pts',(-5.183464652,3.13774478,5.42048837300001));
#105528=CARTESIAN_POINT('Ctrl Pts',(-5.007812776,3.176256335,5.588459453));
#105529=CARTESIAN_POINT('Ctrl Pts',(-4.821654572,3.214285714,5.744706014));
#105530=CARTESIAN_POINT('Ctrl Pts',(-4.692409079,3.240688665,5.85318452000001));
#105531=CARTESIAN_POINT('Ctrl Pts',(-4.55841568800001,3.267335925,5.955740627));
#105532=CARTESIAN_POINT('Ctrl Pts',(-4.55514130622198,3.26798710116568,
5.95824677932199));
#105533=CARTESIAN_POINT('Ctrl Pts',(-4.55186692444395,3.26863827733137,
5.96075293164398));
#105534=CARTESIAN_POINT('Ctrl Pts',(-4.836145564,3.13774478,5.401314292));
#105535=CARTESIAN_POINT('Ctrl Pts',(-4.661115028,3.176256335,5.558030436));
#105536=CARTESIAN_POINT('Ctrl Pts',(-4.476305531,3.214285714,5.703085901));
#105537=CARTESIAN_POINT('Ctrl Pts',(-4.347996415,3.240688665,5.803794678));
#105538=CARTESIAN_POINT('Ctrl Pts',(-4.215287887,3.267335925,5.89863103));
#105539=CARTESIAN_POINT('Ctrl Pts',(-4.21204490327798,3.26798710116568,
5.900948535517));
#105540=CARTESIAN_POINT('Ctrl Pts',(-4.20880191955596,3.26863827733137,
5.90326604103398));
#105541=CARTESIAN_POINT('',(-4.55841568752333,3.26733592550877,5.95574062463764));
#105542=CARTESIAN_POINT('',(-4.38685179458955,3.26733592642396,5.92718582325287));
#105543=CARTESIAN_POINT('',(-4.99794718194148,3.17766594632365,5.59200536169395));
#105544=CARTESIAN_POINT('Ctrl Pts',(-4.55841568868483,3.26733592483286,
5.9557406263308));
#105545=CARTESIAN_POINT('Ctrl Pts',(-4.64792575016103,3.24953506265028,
5.88723125139043));
#105546=CARTESIAN_POINT('Ctrl Pts',(-4.73570877677773,3.23184317427168,
5.81684215734397));
#105547=CARTESIAN_POINT('Ctrl Pts',(-4.8216545719038,3.21428571395066,5.74470601375657));
#105548=CARTESIAN_POINT('Ctrl Pts',(-4.88110613673947,3.20214063497804,
5.69480704427308));
#105549=CARTESIAN_POINT('Ctrl Pts',(-4.93988697182446,3.18993125790122,
5.64389763349253));
#105550=CARTESIAN_POINT('Ctrl Pts',(-4.99794718179529,3.17766594611035,
5.59200536158081));
#105551=CARTESIAN_POINT('Ctrl Pts',(-4.83259642346465,3.13852541816698,
5.40448996726233));
#105552=CARTESIAN_POINT('Ctrl Pts',(-4.86014133022803,3.14538569126172,
5.4356709569915));
#105553=CARTESIAN_POINT('Ctrl Pts',(-4.88770791728529,3.15207183832862,
5.46690619692211));
#105554=CARTESIAN_POINT('Ctrl Pts',(-4.94281497972511,3.16510741648527,
5.52940164199938));
#105555=CARTESIAN_POINT('Ctrl Pts',(-4.97038777257657,3.17146448713464,
5.56069850019475));
#105556=CARTESIAN_POINT('Ctrl Pts',(-4.99794718103561,3.17766594632074,
5.59200536249196));
#105557=CARTESIAN_POINT('Ctrl Pts',(-5.40836684853112,3.26861999521842,
5.19611715339498));
#105558=CARTESIAN_POINT('Ctrl Pts',(-5.40556144226556,3.26797796010921,
5.19903085719749));
#105559=CARTESIAN_POINT('Ctrl Pts',(-5.402756036,3.267335925,5.201944561));
#105560=CARTESIAN_POINT('Ctrl Pts',(-5.121085753,3.202873885,5.49448820600001));
#105561=CARTESIAN_POINT('Ctrl Pts',(-4.809474131,3.137747733,5.754907348));
#105562=CARTESIAN_POINT('Ctrl Pts',(-5.39000423404587,3.26861999521842,
4.84875401616961));
#105563=CARTESIAN_POINT('Ctrl Pts',(-5.38738617102293,3.26797796010921,
4.8516580190848));
#105564=CARTESIAN_POINT('Ctrl Pts',(-5.384768108,3.267335925,4.854562022));
#105565=CARTESIAN_POINT('Ctrl Pts',(-5.121907587,3.202873885,5.146131672));
#105566=CARTESIAN_POINT('Ctrl Pts',(-4.829100921,3.137747733,5.407613549));
#105567=CARTESIAN_POINT('',(-5.40275602441283,3.26733592582611,5.20194454661871));
#105568=CARTESIAN_POINT('Origin',(0.1154182138976,3.08932517228882,-0.150397172527648));
#105569=CARTESIAN_POINT('',(-5.39376206201143,3.26733592735283,5.02825330221466));
#105570=CARTESIAN_POINT('Origin',(3.30898503042576E-13,3.35806380000056,
-3.24826970876657E-13));
#105571=CARTESIAN_POINT('',(-4.99638627664651,3.35698786819216,5.5934000550976));
#105572=CARTESIAN_POINT('Origin',(0.0875969833521245,3.08947602033563,-0.160978744650947));
#105573=CARTESIAN_POINT('Origin',(0.109190386965071,3.48205905117618,-0.152260312179363));
#105574=CARTESIAN_POINT('Ctrl Pts',(-6.2275229,3.13774478,4.17946869));
#105575=CARTESIAN_POINT('Ctrl Pts',(-6.092086485,3.176256335,4.38127266));
#105576=CARTESIAN_POINT('Ctrl Pts',(-5.943868948,3.214285714,4.573884774));
#105577=CARTESIAN_POINT('Ctrl Pts',(-5.840964815,3.240688665,4.707611073));
#105578=CARTESIAN_POINT('Ctrl Pts',(-5.732150647,3.267335925,4.836574093));
#105579=CARTESIAN_POINT('Ctrl Pts',(-5.72949156712874,3.26798710116569,
4.83972554815443));
#105580=CARTESIAN_POINT('Ctrl Pts',(-5.72683248725748,3.26863827733136,
4.84287700330887));
#105581=CARTESIAN_POINT('Ctrl Pts',(-5.884202079,3.13774478,4.235406225));
#105582=CARTESIAN_POINT('Ctrl Pts',(-5.746952999,3.176256335,4.426084824));
#105583=CARTESIAN_POINT('Ctrl Pts',(-5.597646882,3.214285714,4.607477551));
#105584=CARTESIAN_POINT('Ctrl Pts',(-5.493986972,3.240688665,4.73341448));
#105585=CARTESIAN_POINT('Ctrl Pts',(-5.384768108,3.267335925,4.854562022));
#105586=CARTESIAN_POINT('Ctrl Pts',(-5.38209913861705,3.26798710116569,
4.857522491177));
#105587=CARTESIAN_POINT('Ctrl Pts',(-5.37943016923408,3.26863827733136,
4.860482960354));
#105588=CARTESIAN_POINT('',(-5.73215064603959,3.26733592550878,4.83657409078814));
#105589=CARTESIAN_POINT('',(-5.55845938329581,3.26733592642396,4.84556805085149));
#105590=CARTESIAN_POINT('',(-6.08321380816663,3.17766594627907,4.38685647820771));
#105591=CARTESIAN_POINT('Ctrl Pts',(-5.73215064753397,3.26733592483077,
4.83657409218913));
#105592=CARTESIAN_POINT('Ctrl Pts',(-5.80484052267461,3.24953506265028,
4.75042441136096));
#105593=CARTESIAN_POINT('Ctrl Pts',(-5.87543965620554,3.23184317427165,
4.6628102196089));
#105594=CARTESIAN_POINT('Ctrl Pts',(-5.94386894792444,3.21428571394464,
4.5738847737479));
#105595=CARTESIAN_POINT('Ctrl Pts',(-5.99120376486707,3.20214063498633,
4.51237208554023));
#105596=CARTESIAN_POINT('Ctrl Pts',(-6.03766631805085,3.18993125791425,
4.45001676666744));
#105597=CARTESIAN_POINT('Ctrl Pts',(-6.08321380823861,3.17766594609085,
4.38685647829616));
#105598=CARTESIAN_POINT('Ctrl Pts',(-5.88141859146557,3.138525418069,4.23927061465614));
#105599=CARTESIAN_POINT('Ctrl Pts',(-5.91502250643536,3.14538569154247,
4.26380127091827));
#105600=CARTESIAN_POINT('Ctrl Pts',(-5.94865925736818,3.1520718390077,4.28838024855296));
#105601=CARTESIAN_POINT('Ctrl Pts',(-6.01591261206742,3.16510741550992,
4.33756818912958));
#105602=CARTESIAN_POINT('Ctrl Pts',(-6.04956866250469,3.17146448523722,
4.36220600486341));
#105603=CARTESIAN_POINT('Ctrl Pts',(-6.08321380735238,3.17766594626958,
4.3868564792451));
#105604=CARTESIAN_POINT('Ctrl Pts',(-6.39893382949064,3.26861999521842,
3.91199581910429));
#105605=CARTESIAN_POINT('Ctrl Pts',(-6.39682037224532,3.26797796010921,
3.91544448155214));
#105606=CARTESIAN_POINT('Ctrl Pts',(-6.394706915,3.267335925,3.918893144));
#105607=CARTESIAN_POINT('Ctrl Pts',(-6.182510162,3.202873885,4.265148066));
#105608=CARTESIAN_POINT('Ctrl Pts',(-5.934166264,3.137747733,4.586466041));
#105609=CARTESIAN_POINT('Ctrl Pts',(-6.30632771577689,3.26861999521842,
3.5767012587878));
#105610=CARTESIAN_POINT('Ctrl Pts',(-6.30439513638845,3.26797796010921,
3.5801001738939));
#105611=CARTESIAN_POINT('Ctrl Pts',(-6.302462557,3.267335925,3.583499089));
#105612=CARTESIAN_POINT('Ctrl Pts',(-6.108426424,3.202873885,3.924759245));
#105613=CARTESIAN_POINT('Ctrl Pts',(-5.87867629,3.137747733,4.243072598));
#105614=CARTESIAN_POINT('',(-6.39470690059427,3.26733592582611,3.91889313243628));
#105615=CARTESIAN_POINT('Origin',(0.145050850507895,3.08932516225572,-0.122069546710017));
#105616=CARTESIAN_POINT('',(-6.34858472854829,3.26733592735283,3.7511961291114));
#105617=CARTESIAN_POINT('Origin',(6.59194920871187E-14,3.35806379999989,
-5.20417042793042E-14));
#105618=CARTESIAN_POINT('',(-6.08198921396976,3.35698786820903,4.38855411234819));
#105619=CARTESIAN_POINT('Origin',(0.120154476295529,3.08947602866354,-0.138384219053677));
#105620=CARTESIAN_POINT('Origin',(0.139369057992483,3.48205902309301,-0.12522785802636));
#105621=CARTESIAN_POINT('Ctrl Pts',(-6.9803891,3.13774478,2.743021695));
#105622=CARTESIAN_POINT('Ctrl Pts',(-6.891501001,3.176256335,2.969222426));
#105623=CARTESIAN_POINT('Ctrl Pts',(-6.788154619,3.214285714,3.189193765));
#105624=CARTESIAN_POINT('Ctrl Pts',(-6.716403528,3.240688665,3.341914965));
#105625=CARTESIAN_POINT('Ctrl Pts',(-6.63785661200001,3.267335925,3.491254731));
#105626=CARTESIAN_POINT('Ctrl Pts',(-6.63593716964131,3.26798710116568,
3.49490413045825));
#105627=CARTESIAN_POINT('Ctrl Pts',(-6.63401772728262,3.26863827733137,
3.4985535299165));
#105628=CARTESIAN_POINT('Ctrl Pts',(-6.657119845,3.13774478,2.87145527));
#105629=CARTESIAN_POINT('Ctrl Pts',(-6.564069834,3.176256335,3.087180404));
#105630=CARTESIAN_POINT('Ctrl Pts',(-6.457248486,3.214285714,3.296428672));
#105631=CARTESIAN_POINT('Ctrl Pts',(-6.383084804,3.240688665,3.441705082));
#105632=CARTESIAN_POINT('Ctrl Pts',(-6.30246255700001,3.267335925,3.583499089));
#105633=CARTESIAN_POINT('Ctrl Pts',(-6.30049240000562,3.26798710116568,
3.58696409357439));
#105634=CARTESIAN_POINT('Ctrl Pts',(-6.29852224301123,3.26863827733137,
3.59042909814879));
#105635=CARTESIAN_POINT('',(-6.63785661058304,3.26733592550878,3.4912547290495));
#105636=CARTESIAN_POINT('',(-6.47015958873108,3.26733592642396,3.53737690226101));
#105637=CARTESIAN_POINT('',(-6.88403611863456,3.17766594631347,2.97658306108282));
#105638=CARTESIAN_POINT('Ctrl Pts',(-6.63785661234512,3.26733592483146,
3.49125473009715));
#105639=CARTESIAN_POINT('Ctrl Pts',(-6.69032740376243,3.24953506265028,
3.39149300637368));
#105640=CARTESIAN_POINT('Ctrl Pts',(-6.74044150766843,3.23184317427177,
3.29075045860683));
#105641=CARTESIAN_POINT('Ctrl Pts',(-6.78815461857239,3.21428571396706,
3.18919376497703));
#105642=CARTESIAN_POINT('Ctrl Pts',(-6.82115936383275,3.20214063501202,
3.1189436228721));
#105643=CARTESIAN_POINT('Ctrl Pts',(-6.853131098539,3.18993125790658,3.0480580608225));
#105644=CARTESIAN_POINT('Ctrl Pts',(-6.88403611852835,3.17766594610698,
2.97658306107234));
#105645=CARTESIAN_POINT('Ctrl Pts',(-6.65523216405864,3.13852541811756,
2.87582767986541));
#105646=CARTESIAN_POINT('Ctrl Pts',(-6.69332378757033,3.14538568860475,
2.89256096718071));
#105647=CARTESIAN_POINT('Ctrl Pts',(-6.73145786445602,3.15207183294835,
2.90933438629054));
#105648=CARTESIAN_POINT('Ctrl Pts',(-6.80771286730689,3.16510741645553,
2.94291487484572));
#105649=CARTESIAN_POINT('Ctrl Pts',(-6.84587846600961,3.1714644871039,2.9597416187823));
#105650=CARTESIAN_POINT('Ctrl Pts',(-6.88403611813504,3.17766594631055,
2.97658306221566));
#105651=CARTESIAN_POINT('Ctrl Pts',(-7.0902937755932,3.26861999521842,2.44495390907349));
#105652=CARTESIAN_POINT('Ctrl Pts',(-7.0889710902966,3.26797796010921,2.44877627453674));
#105653=CARTESIAN_POINT('Ctrl Pts',(-7.08764840500001,3.267335925,2.45259864));
#105654=CARTESIAN_POINT('Ctrl Pts',(-6.95484726800001,3.202873885,2.836374343));
#105655=CARTESIAN_POINT('Ctrl Pts',(-6.781383379,3.137747733,3.20356668));
#105656=CARTESIAN_POINT('Ctrl Pts',(-6.92777432193795,3.26861999521842,
2.13740592539923));
#105657=CARTESIAN_POINT('Ctrl Pts',(-6.92661759146898,3.26797796010921,
2.14114082319961));
#105658=CARTESIAN_POINT('Ctrl Pts',(-6.925460861,3.267335925,2.144875721));
#105659=CARTESIAN_POINT('Ctrl Pts',(-6.809322032,3.202873885,2.519869437));
#105660=CARTESIAN_POINT('Ctrl Pts',(-6.65337129,3.137747733,2.880130289));
#105661=CARTESIAN_POINT('',(-7.08764838844522,3.26733592582611,2.45259863180721));
#105662=CARTESIAN_POINT('Origin',(0.16790095296493,3.08932520347122,-0.0880339539605168));
#105663=CARTESIAN_POINT('',(-7.0065546284336,3.26733592735283,2.29873719441841));
#105664=CARTESIAN_POINT('Origin',(-4.16333634234434E-14,3.35806379999989,
4.74880551548651E-14));
#105665=CARTESIAN_POINT('',(-6.8832050954752,3.35698786817884,2.97850425767523));
#105666=CARTESIAN_POINT('Origin',(0.147094092923507,3.08947605737589,-0.109319328977385));
#105667=CARTESIAN_POINT('Origin',(0.163031056593049,3.48205907567582,-0.0923399100765862));
#105668=CARTESIAN_POINT('Ctrl Pts',(-7.406860063,3.13774478,1.178314054));
#105669=CARTESIAN_POINT('Ctrl Pts',(-7.368676589,3.176256335,1.418334652));
#105670=CARTESIAN_POINT('Ctrl Pts',(-7.315033724,3.214285714,1.655379601));
#105671=CARTESIAN_POINT('Ctrl Pts',(-7.277790677,3.240688665,1.819954627));
#105672=CARTESIAN_POINT('Ctrl Pts',(-7.23318378,3.267335925,1.982688177));
#105673=CARTESIAN_POINT('Ctrl Pts',(-7.23209372615764,3.26798710116569,
1.98666487888668));
#105674=CARTESIAN_POINT('Ctrl Pts',(-7.23100367231527,3.26863827733136,
1.99064158077337));
#105675=CARTESIAN_POINT('Ctrl Pts',(-7.118758086,3.13774478,1.373238257));
#105676=CARTESIAN_POINT('Ctrl Pts',(-7.07425806000001,3.176256335,1.60392286));
#105677=CARTESIAN_POINT('Ctrl Pts',(-7.014916327,3.214285714,1.831242452));
#105678=CARTESIAN_POINT('Ctrl Pts',(-6.973716685,3.240688665,1.98906538));
#105679=CARTESIAN_POINT('Ctrl Pts',(-6.925460861,3.267335925,2.144875721));
#105680=CARTESIAN_POINT('Ctrl Pts',(-6.92428163872934,3.26798710116569,
2.1486832411888));
#105681=CARTESIAN_POINT('Ctrl Pts',(-6.92310241645868,3.26863827733136,
2.15249076137759));
#105682=CARTESIAN_POINT('',(-7.23318377818696,3.26733592550877,1.9826881754134));
#105683=CARTESIAN_POINT('',(-7.07932232296849,3.26733592642396,2.06378194053243));
#105684=CARTESIAN_POINT('',(-7.36296855048892,3.17766594632392,1.42712792863381));
#105685=CARTESIAN_POINT('Ctrl Pts',(-7.23318378013855,3.26733592483385,
1.98268817605887));
#105686=CARTESIAN_POINT('Ctrl Pts',(-7.2629820116059,3.24953506265028,1.87397915710101));
#105687=CARTESIAN_POINT('Ctrl Pts',(-7.29026780568012,3.23184317427141,
1.76481886353824));
#105688=CARTESIAN_POINT('Ctrl Pts',(-7.31503372343932,3.21428571389762,
1.65537960077499));
#105689=CARTESIAN_POINT('Ctrl Pts',(-7.33216513187329,3.20214063490214,
1.57967682304382));
#105690=CARTESIAN_POINT('Ctrl Pts',(-7.34815108484028,3.18993125791942,
1.50357554853497));
#105691=CARTESIAN_POINT('Ctrl Pts',(-7.36296855041346,3.1776659461216,1.42712792865164));
#105692=CARTESIAN_POINT('Ctrl Pts',(-7.11785447610388,3.13852541812603,
1.37791423853735));
#105693=CARTESIAN_POINT('Ctrl Pts',(-7.1586527173248,3.14538569137985,1.38606774128126));
#105694=CARTESIAN_POINT('Ctrl Pts',(-7.19950104905351,3.15207183861513,
1.39425131180269));
#105695=CARTESIAN_POINT('Ctrl Pts',(-7.281192024112,3.16510741562126,1.41065412762892));
#105696=CARTESIAN_POINT('Ctrl Pts',(-7.32208257888771,3.1714644853935,1.41888299491582));
#105697=CARTESIAN_POINT('Ctrl Pts',(-7.3629685502442,3.17766594632102,1.42712792984957));
#105698=CARTESIAN_POINT('Ctrl Pts',(-7.45011946511826,3.26861999521842,
0.86358867113768));
#105699=CARTESIAN_POINT('Ctrl Pts',(-7.44964939905913,3.26797796010921,
0.867606010068841));
#105700=CARTESIAN_POINT('Ctrl Pts',(-7.449179333,3.267335925,0.871623349000001));
#105701=CARTESIAN_POINT('Ctrl Pts',(-7.401983445,3.202873885,1.274974909));
#105702=CARTESIAN_POINT('Ctrl Pts',(-7.311510543,3.137747733,1.670872101));
#105703=CARTESIAN_POINT('Ctrl Pts',(-7.22528590126796,3.26861999521842,
0.598167867343195));
#105704=CARTESIAN_POINT('Ctrl Pts',(-7.22495910713398,3.26797796010921,
0.602064108171597));
#105705=CARTESIAN_POINT('Ctrl Pts',(-7.224632313,3.267335925,0.605960349000001));
#105706=CARTESIAN_POINT('Ctrl Pts',(-7.191821309,3.202873885,0.997153336));
#105707=CARTESIAN_POINT('Ctrl Pts',(-7.116962042,3.137747733,1.382516288));
#105708=CARTESIAN_POINT('',(-7.44917931507457,3.2673359258261,0.871623344572886));
#105709=CARTESIAN_POINT('Origin',(0.182900004317507,3.08932517287314,-0.0498819972482253));
#105710=CARTESIAN_POINT('',(-7.3369058215324,3.26733592735283,0.738791863574644));
#105711=CARTESIAN_POINT('Origin',(1.23468943402649E-12,3.35806380000078,
-2.36193443275967E-13));
#105712=CARTESIAN_POINT('',(-7.36256995659096,3.35698786820896,1.42918285405513));
#105713=CARTESIAN_POINT('Origin',(0.167155057817885,3.08947599877084,-0.0751425101531752));
#105714=CARTESIAN_POINT('Origin',(0.179069849303855,3.48205904621345,-0.0551341927314677));
#105715=CARTESIAN_POINT('Ctrl Pts',(-7.48699448200001,3.13774478,-0.441490242));
#105716=CARTESIAN_POINT('Ctrl Pts',(-7.50130105,3.176256335,-0.198872874));
#105717=CARTESIAN_POINT('Ctrl Pts',(-7.499869982,3.214285714,0.044161726));
#105718=CARTESIAN_POINT('Ctrl Pts',(-7.498876423,3.240688665,0.212895234));
#105719=CARTESIAN_POINT('Ctrl Pts',(-7.490295313,3.267335925,0.381413328));
#105720=CARTESIAN_POINT('Ctrl Pts',(-7.49008561735748,3.26798710116569,
0.385531386153037));
#105721=CARTESIAN_POINT('Ctrl Pts',(-7.48987592171496,3.26863827733136,
0.389649444306074));
#105722=CARTESIAN_POINT('Ctrl Pts',(-7.247531111,3.13774478,-0.189189849));
#105723=CARTESIAN_POINT('Ctrl Pts',(-7.253661841,3.176256335,0.045667665));
#105724=CARTESIAN_POINT('Ctrl Pts',(-7.244574478,3.214285714,0.28042937));
#105725=CARTESIAN_POINT('Ctrl Pts',(-7.238265325,3.240688665,0.443419191));
#105726=CARTESIAN_POINT('Ctrl Pts',(-7.224632313,3.267335925,0.605960349000001));
#105727=CARTESIAN_POINT('Ctrl Pts',(-7.22429916458321,3.26798710116569,
0.609932349424512));
#105728=CARTESIAN_POINT('Ctrl Pts',(-7.22396601616642,3.26863827733136,
0.613904349849024));
#105729=CARTESIAN_POINT('',(-7.49029531088823,3.26733592550878,0.381413326840878));
#105730=CARTESIAN_POINT('',(-7.3574638135905,3.26733592642396,0.493686829699741));
#105731=CARTESIAN_POINT('',(-7.4976167564852,3.17766594630478,-0.189058119747558));
#105732=CARTESIAN_POINT('Ctrl Pts',(-7.4902953129333,3.26733592483399,0.381413327051709));
#105733=CARTESIAN_POINT('Ctrl Pts',(-7.49602765287763,3.24953506265028,
0.268840125822009));
#105734=CARTESIAN_POINT('Ctrl Pts',(-7.49920928384314,3.23184317427167,
0.156366300058196));
#105735=CARTESIAN_POINT('Ctrl Pts',(-7.49986998160241,3.21428571394786,
0.044161726036576));
#105736=CARTESIAN_POINT('Ctrl Pts',(-7.50032700804195,3.20214063500503,
-0.0334539089873134));
#105737=CARTESIAN_POINT('Ctrl Pts',(-7.49957969348547,3.18993125793839,
-0.111212485413614));
#105738=CARTESIAN_POINT('Ctrl Pts',(-7.49761675662906,3.17766594612312,
-0.189058119722564));
#105739=CARTESIAN_POINT('Ctrl Pts',(-7.24765382489753,3.13852541804203,
-0.184428940551483));
#105740=CARTESIAN_POINT('Ctrl Pts',(-7.28925098650911,3.14538569110661,
-0.185236478160081));
#105741=CARTESIAN_POINT('Ctrl Pts',(-7.33090353108689,3.15207183813376,
-0.186025418823179));
#105742=CARTESIAN_POINT('Ctrl Pts',(-7.41421074489788,3.1651074164085,-0.1875672367013));
#105743=CARTESIAN_POINT('Ctrl Pts',(-7.45591427041447,3.17146448703968,
-0.188321016362887));
#105744=CARTESIAN_POINT('Ctrl Pts',(-7.4976167564466,3.17766594629268,-0.189058118439964));
#105745=CARTESIAN_POINT('Ctrl Pts',(-7.46158584913562,3.26861999521842,
-0.758157013164344));
#105746=CARTESIAN_POINT('Ctrl Pts',(-7.46199038206781,3.26797796010921,
-0.754132547082172));
#105747=CARTESIAN_POINT('Ctrl Pts',(-7.462394915,3.267335925,-0.750108081));
#105748=CARTESIAN_POINT('Ctrl Pts',(-7.503011102,3.202873885,-0.346040936));
#105749=CARTESIAN_POINT('Ctrl Pts',(-7.499759601,3.137747733,0.0600494));
#105750=CARTESIAN_POINT('Ctrl Pts',(-7.18495114151865,3.26861999521842,
-0.969039855917186));
#105751=CARTESIAN_POINT('Ctrl Pts',(-7.18546956425932,3.26797796010921,
-0.965164455958594));
#105752=CARTESIAN_POINT('Ctrl Pts',(-7.18598798700001,3.267335925,-0.961289056));
#105753=CARTESIAN_POINT('Ctrl Pts',(-7.238039015,3.202873885,-0.572188548));
#105754=CARTESIAN_POINT('Ctrl Pts',(-7.24777156,3.137747733,-0.179742638));
#105755=CARTESIAN_POINT('',(-7.46239489653727,3.2673359258261,-0.750108081480122));
#105756=CARTESIAN_POINT('Origin',(0.189347432826993,3.08932519891378,-0.00939766698610588));
#105757=CARTESIAN_POINT('',(-7.32419145269983,3.26733592735283,-0.855698553950613));
#105758=CARTESIAN_POINT('Origin',(-7.41160605111091E-13,3.35806379999989,
2.81350463759988E-14));
#105759=CARTESIAN_POINT('',(-7.49766922987128,3.35698786824895,-0.186965551550327));
#105760=CARTESIAN_POINT('Origin',(0.179400584072857,3.08947606338236,-0.0374523169333984));
#105761=CARTESIAN_POINT('Origin',(0.186735398645302,3.48205900677173,-0.0153504641044341));
#105762=CARTESIAN_POINT('Ctrl Pts',(-7.21704536000001,3.13774478,-2.040650945));
#105763=CARTESIAN_POINT('Ctrl Pts',(-7.283173011,3.176256335,-1.806781326));
#105764=CARTESIAN_POINT('Ctrl Pts',(-7.334020655,3.214285714,-1.569121102));
#105765=CARTESIAN_POINT('Ctrl Pts',(-7.36932304100001,3.240688665,-1.404118904));
#105766=CARTESIAN_POINT('Ctrl Pts',(-7.397168962,3.267335925,-1.237695984));
#105767=CARTESIAN_POINT('Ctrl Pts',(-7.39784942971288,3.26798710116569,
-1.23362912538387));
#105768=CARTESIAN_POINT('Ctrl Pts',(-7.39852989742575,3.26863827733136,
-1.22956226676773));
#105769=CARTESIAN_POINT('Ctrl Pts',(-7.037417636,3.13774478,-1.742771649));
#105770=CARTESIAN_POINT('Ctrl Pts',(-7.09389245600001,3.176256335,-1.514722898));
#105771=CARTESIAN_POINT('Ctrl Pts',(-7.135484378,3.214285714,-1.283496277));
#105772=CARTESIAN_POINT('Ctrl Pts',(-7.164360722,3.240688665,-1.122960787));
#105773=CARTESIAN_POINT('Ctrl Pts',(-7.185987987,3.267335925,-0.961289056000001));
#105774=CARTESIAN_POINT('Ctrl Pts',(-7.18651649009927,3.26798710116569,
-0.957338301667589));
#105775=CARTESIAN_POINT('Ctrl Pts',(-7.18704499319853,3.26863827733136,
-0.953387547335178));
#105776=CARTESIAN_POINT('',(-7.3971689596895,3.26733592550878,-1.23769598468391));
#105777=CARTESIAN_POINT('',(-7.2915784731849,3.26733592642396,-1.09949252872145));
#105778=CARTESIAN_POINT('',(-7.28168473605635,3.17766594628575,-1.79640402091834));
#105779=CARTESIAN_POINT('Ctrl Pts',(-7.3971689617301,3.26733592483313,-1.23769598491716));
#105780=CARTESIAN_POINT('Ctrl Pts',(-7.37856737175047,3.24953506265028,
-1.34886957116081));
#105781=CARTESIAN_POINT('Ctrl Pts',(-7.35749607004708,3.23184317427158,
-1.45939777806657));
#105782=CARTESIAN_POINT('Ctrl Pts',(-7.33402065462609,3.21428571393052,
-1.5691211020299));
#105783=CARTESIAN_POINT('Ctrl Pts',(-7.31778192897064,3.20214063496634,
-1.64502037415957));
#105784=CARTESIAN_POINT('Ctrl Pts',(-7.30033629090686,3.18993125792124,
-1.72080034764459));
#105785=CARTESIAN_POINT('Ctrl Pts',(-7.2816847361835,3.17766594609984,-1.79640402091955));
#105786=CARTESIAN_POINT('Ctrl Pts',(-7.03856093581467,3.13852541814607,
-1.73814842744475));
#105787=CARTESIAN_POINT('Ctrl Pts',(-7.07901199899998,3.14538569403019,
-1.74787924951643));
#105788=CARTESIAN_POINT('Ctrl Pts',(-7.11952115065935,3.15207184400054,
-1.75760381572493));
#105789=CARTESIAN_POINT('Ctrl Pts',(-7.20054920654423,3.16510741640785,
-1.77701816666527));
#105790=CARTESIAN_POINT('Ctrl Pts',(-7.24111568642906,3.17146448702765,
-1.78671934870936));
#105791=CARTESIAN_POINT('Ctrl Pts',(-7.28168473631141,3.17766594627506,
-1.79640401962634));
#105792=CARTESIAN_POINT('Ctrl Pts',(-7.12415677113848,3.26861999521842,
-2.3444521183563));
#105793=CARTESIAN_POINT('Ctrl Pts',(-7.12541698756924,3.26797796010921,
-2.34060870467815));
#105794=CARTESIAN_POINT('Ctrl Pts',(-7.126677204,3.267335925,-2.336765291));
#105795=CARTESIAN_POINT('Ctrl Pts',(-7.2532063,3.202873885,-1.950876291));
#105796=CARTESIAN_POINT('Ctrl Pts',(-7.337328235,3.137747733,-1.553581145));
#105797=CARTESIAN_POINT('Ctrl Pts',(-6.80865605252724,3.26861999521842,
-2.49093635239381));
#105798=CARTESIAN_POINT('Ctrl Pts',(-6.80999545126362,3.26797796010921,
-2.4872630026969));
#105799=CARTESIAN_POINT('Ctrl Pts',(-6.81133485,3.267335925,-2.483589653));
#105800=CARTESIAN_POINT('Ctrl Pts',(-6.945814061,3.202873885,-2.114775531));
#105801=CARTESIAN_POINT('Ctrl Pts',(-7.039683335,3.137747733,-1.733596997));
#105802=CARTESIAN_POINT('',(-7.1266771859077,3.26733592582622,-2.33676528743656));
#105803=CARTESIAN_POINT('Origin',(0.186940587355398,3.08932519213192,0.0315260866611503));
#105804=CARTESIAN_POINT('',(-6.96900603178777,3.26733592735283,-2.41017745815618));
#105805=CARTESIAN_POINT('Origin',(-1.4363510381088E-12,3.35806379999989,
-3.13984949151802E-13));
#105806=CARTESIAN_POINT('',(-7.28218582271254,3.35698786820963,-1.79437165603226));
#105807=CARTESIAN_POINT('Origin',(0.183257870511054,3.08947605308055,0.00198920916088918));
#105808=CARTESIAN_POINT('Origin',(0.18566933249872,3.48205906573847,0.0251509524794924));
#105809=CARTESIAN_POINT('Ctrl Pts',(-6.609635218,3.13774478,-3.544393078));
#105810=CARTESIAN_POINT('Ctrl Pts',(-6.724491896,3.176256335,-3.330206691));
#105811=CARTESIAN_POINT('Ctrl Pts',(-6.825240674,3.214285714,-3.109033571));
#105812=CARTESIAN_POINT('Ctrl Pts',(-6.895188305,3.240688665,-2.955478003));
#105813=CARTESIAN_POINT('Ctrl Pts',(-6.958159212,3.267335925,-2.798932008));
#105814=CARTESIAN_POINT('Ctrl Pts',(-6.95969802513763,3.26798710116569,
-2.79510651071521));
#105815=CARTESIAN_POINT('Ctrl Pts',(-6.96123683827525,3.26863827733136,
-2.79128101343042));
#105816=CARTESIAN_POINT('Ctrl Pts',(-6.498242333,3.13774478,-3.214863384));
#105817=CARTESIAN_POINT('Ctrl Pts',(-6.602420544,3.176256335,-3.004286703));
#105818=CARTESIAN_POINT('Ctrl Pts',(-6.692746959,3.214285714,-2.787407065));
#105819=CARTESIAN_POINT('Ctrl Pts',(-6.755458575,3.240688665,-2.636832366));
#105820=CARTESIAN_POINT('Ctrl Pts',(-6.81133485,3.267335925,-2.483589653));
#105821=CARTESIAN_POINT('Ctrl Pts',(-6.81270029239472,3.26798710116569,
-2.47984487765461));
#105822=CARTESIAN_POINT('Ctrl Pts',(-6.81406573478944,3.26863827733136,
-2.47610010230922));
#105823=CARTESIAN_POINT('',(-6.95815920959683,3.26733592550877,-2.79893200815632));
#105824=CARTESIAN_POINT('',(-6.88474702784079,3.26733592642396,-2.64126083873485));
#105825=CARTESIAN_POINT('',(-6.72526923023681,3.17766594630029,-3.31975206625678));
#105826=CARTESIAN_POINT('Ctrl Pts',(-6.95815921154404,3.26733592483523,
-2.79893200882494));
#105827=CARTESIAN_POINT('Ctrl Pts',(-6.91609348176499,3.24953506265028,
-2.90350762661683));
#105828=CARTESIAN_POINT('Ctrl Pts',(-6.8717545181582,3.23184317427134,-3.00692203827643));
#105829=CARTESIAN_POINT('Ctrl Pts',(-6.82524067351529,3.2142857138838,-3.10903357124645));
#105830=CARTESIAN_POINT('Ctrl Pts',(-6.7930655000057,3.20214063488939,-3.17966751488298));
#105831=CARTESIAN_POINT('Ctrl Pts',(-6.75973727706754,3.18993125792766,
-3.24992549778636));
#105832=CARTESIAN_POINT('Ctrl Pts',(-6.725269230334,3.17766594611253,-3.31975206627177));
#105833=CARTESIAN_POINT('Ctrl Pts',(-6.50035275888917,3.13852541814596,
-3.21059402588742));
#105834=CARTESIAN_POINT('Ctrl Pts',(-6.53776626148371,3.14538569432647,
-3.22879313049195));
#105835=CARTESIAN_POINT('Ctrl Pts',(-6.5752378395886,3.15207184462724,-3.24699861289385));
#105836=CARTESIAN_POINT('Ctrl Pts',(-6.65019798960515,3.16510741639772,
-3.283377702109));
#105837=CARTESIAN_POINT('Ctrl Pts',(-6.68773058054202,3.17146448703241,
-3.30157266991739));
#105838=CARTESIAN_POINT('Ctrl Pts',(-6.72526923077001,3.17766594629182,
-3.31975206507072));
#105839=CARTESIAN_POINT('Ctrl Pts',(-6.45361004080255,3.26861999521842,
-3.82112324805941));
#105840=CARTESIAN_POINT('Ctrl Pts',(-6.45566701440128,3.26797796010921,
-3.8176406005297));
#105841=CARTESIAN_POINT('Ctrl Pts',(-6.457723988,3.267335925,-3.814157953));
#105842=CARTESIAN_POINT('Ctrl Pts',(-6.664249632,3.202873885,-3.464490838));
#105843=CARTESIAN_POINT('Ctrl Pts',(-6.831811556,3.137747733,-3.094567962));
#105844=CARTESIAN_POINT('Ctrl Pts',(-6.11399577311955,3.26861999521842,
-3.89635943336084));
#105845=CARTESIAN_POINT('Ctrl Pts',(-6.11609351905978,3.26797796010921,
-3.89305989568042));
#105846=CARTESIAN_POINT('Ctrl Pts',(-6.118191265,3.267335925,-3.889760358));
#105847=CARTESIAN_POINT('Ctrl Pts',(-6.328810561,3.202873885,-3.558477961));
#105848=CARTESIAN_POINT('Ctrl Pts',(-6.50242734,3.137747733,-3.206390288));
#105849=CARTESIAN_POINT('',(-6.45772397105701,3.2673359258261,-3.81415794567119));
#105850=CARTESIAN_POINT('Origin',(0.175793103684657,3.08932515318603,0.0709758570261609));
#105851=CARTESIAN_POINT('',(-6.28795763415186,3.26733592735283,-3.85195914300908));
#105852=CARTESIAN_POINT('Origin',(-3.19189119579733E-13,3.35806379999956,
-4.5102810375397E-14));
#105853=CARTESIAN_POINT('',(-6.72619550069598,3.35698786820417,-3.31787493563951));
#105854=CARTESIAN_POINT('Origin',(0.178546055844735,3.08947598647104,0.0413378320615154));
#105855=CARTESIAN_POINT('Origin',(0.175921893134506,3.48205906426425,0.0644764226566241));
#105856=CARTESIAN_POINT('Ctrl Pts',(-5.69316587900001,3.13774478,-4.88240333000001));
#105857=CARTESIAN_POINT('Ctrl Pts',(-5.851381014,3.176256335,-4.697915292));
#105858=CARTESIAN_POINT('Ctrl Pts',(-5.997320024,3.214285714,-4.503571086));
#105859=CARTESIAN_POINT('Ctrl Pts',(-6.09864222700001,3.240688665,-4.368642235));
#105860=CARTESIAN_POINT('Ctrl Pts',(-6.19379367,3.267335925,-4.229293082));
#105861=CARTESIAN_POINT('Ctrl Pts',(-6.19611887536115,3.26798710116569,
-4.22588782205426));
#105862=CARTESIAN_POINT('Ctrl Pts',(-6.1984440807223,3.26863827733136,-4.22248256210852));
#105863=CARTESIAN_POINT('Ctrl Pts',(-5.655216442,3.13774478,-4.536631679));
#105864=CARTESIAN_POINT('Ctrl Pts',(-5.802226786,3.176256335,-4.3533734));
#105865=CARTESIAN_POINT('Ctrl Pts',(-5.93706413,3.214285714,-4.160981797));
#105866=CARTESIAN_POINT('Ctrl Pts',(-6.030678693,3.240688665,-4.027408594));
#105867=CARTESIAN_POINT('Ctrl Pts',(-6.118191265,3.267335925,-3.889760358));
#105868=CARTESIAN_POINT('Ctrl Pts',(-6.12032980010958,3.26798710116569,
-3.88639666317616));
#105869=CARTESIAN_POINT('Ctrl Pts',(-6.12246833521915,3.26863827733136,
-3.88303296835232));
#105870=CARTESIAN_POINT('',(-6.19379366761472,3.26733592550878,-4.22929308165504));
#105871=CARTESIAN_POINT('',(-6.1559924626444,3.26733592642396,-4.05952672736318));
#105872=CARTESIAN_POINT('',(-5.8543876097621,3.17766594631067,-4.68787219476722));
#105873=CARTESIAN_POINT('Ctrl Pts',(-6.19379366936754,3.26733592483246,
-4.22929308272258));
#105874=CARTESIAN_POINT('Ctrl Pts',(-6.13023074682398,3.24953506265028,
-4.32238089219935));
#105875=CARTESIAN_POINT('Ctrl Pts',(-6.06469736193084,3.23184317427164,
-4.41384596580043));
#105876=CARTESIAN_POINT('Ctrl Pts',(-5.99732002374697,3.21428571394204,
-4.50357108612209));
#105877=CARTESIAN_POINT('Ctrl Pts',(-5.9507128782345,3.20214063496735,-4.56563693622809));
#105878=CARTESIAN_POINT('Ctrl Pts',(-5.90306046074902,3.18993125790292,
-4.62708774391578));
#105879=CARTESIAN_POINT('Ctrl Pts',(-5.85438760969563,3.17766594610292,
-4.68787219467207));
#105880=CARTESIAN_POINT('Ctrl Pts',(-5.65819531310952,3.13852541812815,
-4.53291581612997));
#105881=CARTESIAN_POINT('Ctrl Pts',(-5.69082182373513,3.14538569108329,
-4.55873222060614));
#105882=CARTESIAN_POINT('Ctrl Pts',(-5.72350367863138,3.15207183800177,
-4.58456733645385));
#105883=CARTESIAN_POINT('Ctrl Pts',(-5.78889090646855,3.1651074164587,-4.63621014562947));
#105884=CARTESIAN_POINT('Ctrl Pts',(-5.82163462603071,3.17146448710556,
-4.66204812285444));
#105885=CARTESIAN_POINT('Ctrl Pts',(-5.85438761052842,3.17766594630774,
-4.68787219379599));
#105886=CARTESIAN_POINT('Ctrl Pts',(-5.48129967805377,3.26861999521842,
-5.11912290128042));
#105887=CARTESIAN_POINT('Ctrl Pts',(-5.48405722702689,3.26797796010921,
-5.11616386464021));
#105888=CARTESIAN_POINT('Ctrl Pts',(-5.48681477600001,3.267335925,-5.113204828));
#105889=CARTESIAN_POINT('Ctrl Pts',(-5.763680059,3.202873885,-4.816109645));
#105890=CARTESIAN_POINT('Ctrl Pts',(-6.006846961,3.137747733,-4.49085622));
#105891=CARTESIAN_POINT('Ctrl Pts',(-5.13345184724536,3.26861999521842,
-5.11959307791208));
#105892=CARTESIAN_POINT('Ctrl Pts',(-5.13620985212268,3.26797796010921,
-5.11682163495604));
#105893=CARTESIAN_POINT('Ctrl Pts',(-5.138967857,3.267335925,-5.114050192));
#105894=CARTESIAN_POINT('Ctrl Pts',(-5.415878914,3.202873885,-4.835789916));
#105895=CARTESIAN_POINT('Ctrl Pts',(-5.66112507100001,3.137747733,-4.529256333));
#105896=CARTESIAN_POINT('',(-5.48681476101586,3.2673359258261,-5.11320481720661));
#105897=CARTESIAN_POINT('Origin',(0.156425222198522,3.08932517488456,0.107106609688186));
#105898=CARTESIAN_POINT('',(-5.31289132665814,3.26733592735283,-5.11362749944603));
#105899=CARTESIAN_POINT('Origin',(-9.06393016197882E-14,3.35806380000078,
-5.85469173142172E-14));
#105900=CARTESIAN_POINT('',(-5.85569575173381,3.35698786820111,-4.68623807111382));
#105901=CARTESIAN_POINT('Origin',(0.165484884337215,3.08947604107569,0.0787531823238918));
#105902=CARTESIAN_POINT('Origin',(0.157948508963864,3.48205905793563,0.100787081180135));
#105903=CARTESIAN_POINT('Ctrl Pts',(-4.510490432,3.13774478,-5.992117828));
#105904=CARTESIAN_POINT('Ctrl Pts',(-4.704666059,3.176256335,-5.845954596));
#105905=CARTESIAN_POINT('Ctrl Pts',(-4.888971356,3.214285714,-5.687526623));
#105906=CARTESIAN_POINT('Ctrl Pts',(-5.016930416,3.240688665,-5.577533611));
#105907=CARTESIAN_POINT('Ctrl Pts',(-5.139813221,3.267335925,-5.461897111));
#105908=CARTESIAN_POINT('Ctrl Pts',(-5.14281609460832,3.26798710116569,
-5.45907131455102));
#105909=CARTESIAN_POINT('Ctrl Pts',(-5.14581896821665,3.26863827733136,
-5.45624551810205));
#105910=CARTESIAN_POINT('Ctrl Pts',(-4.547758915,3.13774478,-5.64627212));
#105911=CARTESIAN_POINT('Ctrl Pts',(-4.730727352,3.176256335,-5.498901196));
#105912=CARTESIAN_POINT('Ctrl Pts',(-4.903770781,3.214285714,-5.339993645));
#105913=CARTESIAN_POINT('Ctrl Pts',(-5.023910978,3.240688665,-5.229667673));
#105914=CARTESIAN_POINT('Ctrl Pts',(-5.138967857,3.267335925,-5.114050192));
#105915=CARTESIAN_POINT('Ctrl Pts',(-5.14177948931427,3.26798710116569,
-5.11122486031624));
#105916=CARTESIAN_POINT('Ctrl Pts',(-5.14459112162854,3.26863827733136,
-5.10839952863248));
#105917=CARTESIAN_POINT('',(-5.13981321874104,3.26733592550878,-5.46189711015752));
#105918=CARTESIAN_POINT('',(-5.13939053267506,3.26733592642396,-5.28797365764722));
#105919=CARTESIAN_POINT('',(-4.70976133171338,3.17766594633946,-5.83679262966929));
#105920=CARTESIAN_POINT('Ctrl Pts',(-5.13981322022166,3.2673359248313,-5.4618971115748));
#105921=CARTESIAN_POINT('Ctrl Pts',(-5.05772523537544,3.24953506265028,
-5.53914443058292));
#105922=CARTESIAN_POINT('Ctrl Pts',(-4.97406169733098,3.23184317427134,
-5.61438336149303));
#105923=CARTESIAN_POINT('Ctrl Pts',(-4.88897135546675,3.21428571388327,
-5.68752662272347));
#105924=CARTESIAN_POINT('Ctrl Pts',(-4.83011153576288,3.20214063488469,
-5.73812224877108));
#105925=CARTESIAN_POINT('Ctrl Pts',(-4.77036309859118,3.18993125793235,
-5.78789250995639));
#105926=CARTESIAN_POINT('Ctrl Pts',(-4.70976133169848,3.17766594613959,
-5.83679262960069));
#105927=CARTESIAN_POINT('Ctrl Pts',(-4.55146694246914,3.13852541813341,
-5.6432835011122));
#105928=CARTESIAN_POINT('Ctrl Pts',(-4.57778088596039,3.14538568749849,
-5.67551005078106));
#105929=CARTESIAN_POINT('Ctrl Pts',(-4.60414485520672,3.15207183068127,
-5.707766769236));
#105930=CARTESIAN_POINT('Ctrl Pts',(-4.656901714923,3.16510741563564,-5.77225855134485));
#105931=CARTESIAN_POINT('Ctrl Pts',(-4.68332549931054,3.17146448541837,
-5.80453137803275));
#105932=CARTESIAN_POINT('Ctrl Pts',(-4.70976133266641,3.17766594633659,
-5.8367926288889));
#105933=CARTESIAN_POINT('Ctrl Pts',(-4.25268983415697,3.26861999521842,
-6.17775805698345));
#105934=CARTESIAN_POINT('Ctrl Pts',(-4.25601901857848,3.26797796010921,
-6.17546099249173));
#105935=CARTESIAN_POINT('Ctrl Pts',(-4.259348203,3.267335925,-6.173163928));
#105936=CARTESIAN_POINT('Ctrl Pts',(-4.593607212,3.202873885,-5.942532517));
#105937=CARTESIAN_POINT('Ctrl Pts',(-4.901008879,3.137747733,-5.677157033));
#105938=CARTESIAN_POINT('Ctrl Pts',(-3.91287341787142,3.26861999521842,
-6.10344024028336));
#105939=CARTESIAN_POINT('Ctrl Pts',(-3.91616272043571,3.26797796010921,
-6.10132648164168));
#105940=CARTESIAN_POINT('Ctrl Pts',(-3.919452023,3.267335925,-6.09921272300001));
#105941=CARTESIAN_POINT('Ctrl Pts',(-4.249706787,3.202873885,-5.886985709));
#105942=CARTESIAN_POINT('Ctrl Pts',(-4.555114885,3.137747733,-5.640339386));
#105943=CARTESIAN_POINT('',(-4.25934819074955,3.26733592582622,-6.17316391421539));
#105944=CARTESIAN_POINT('Origin',(0.129743386737614,3.08932515652023,0.138229392214959));
#105945=CARTESIAN_POINT('',(-4.08940012518944,3.26733592735283,-6.13618831737648));
#105946=CARTESIAN_POINT('Origin',(1.05644659686988E-12,3.35806379999967,
1.36652841820073E-12));
#105947=CARTESIAN_POINT('',(-4.71139017780269,3.3569878681991,-5.83547792255985));
#105948=CARTESIAN_POINT('Origin',(0.144686138641019,3.08947604254338,0.112486115523743));
#105949=CARTESIAN_POINT('Origin',(0.132589486939138,3.48205905601155,0.132384954758726));
#105950=CARTESIAN_POINT('Ctrl Pts',(-3.116909465,3.13774478,-6.821647557));
#105951=CARTESIAN_POINT('Ctrl Pts',(-3.337966148,3.176256335,-6.72064355999999));
#105952=CARTESIAN_POINT('Ctrl Pts',(-3.55201982,3.214285714,-6.605539735));
#105953=CARTESIAN_POINT('Ctrl Pts',(-3.700632515,3.240688665,-6.525625715));
#105954=CARTESIAN_POINT('Ctrl Pts',(-3.845500817,3.267335925,-6.439108903));
#105955=CARTESIAN_POINT('Ctrl Pts',(-3.84904094778363,3.26798710116569,
-6.43699470116816));
#105956=CARTESIAN_POINT('Ctrl Pts',(-3.85258107856726,3.26863827733136,
-6.43488049933635));
#105957=CARTESIAN_POINT('Ctrl Pts',(-3.227653236,3.13774478,-6.491899151));
#105958=CARTESIAN_POINT('Ctrl Pts',(-3.438024365,3.176256335,-6.387306483));
#105959=CARTESIAN_POINT('Ctrl Pts',(-3.641182561,3.214285714,-6.269313324));
#105960=CARTESIAN_POINT('Ctrl Pts',(-3.78223077,3.240688665,-6.187393303));
#105961=CARTESIAN_POINT('Ctrl Pts',(-3.919452023,3.267335925,-6.09921272300001));
#105962=CARTESIAN_POINT('Ctrl Pts',(-3.92280528368717,3.26798710116569,
-6.09705786385231));
#105963=CARTESIAN_POINT('Ctrl Pts',(-3.92615854437433,3.26863827733136,
-6.09490300470461));
#105964=CARTESIAN_POINT('',(-3.84550081497584,3.26733592550878,-6.43910890169017));
#105965=CARTESIAN_POINT('',(-3.88247641250146,3.26733592642396,-6.26916081764383));
#105966=CARTESIAN_POINT('',(-3.34491184766582,3.17766594631022,-6.71279112817122));
#105967=CARTESIAN_POINT('Ctrl Pts',(-3.84550081611735,3.26733592483148,
-6.43910890339299));
#105968=CARTESIAN_POINT('Ctrl Pts',(-3.74872611297783,3.24953506265028,
-6.4969037326349));
#105969=CARTESIAN_POINT('Ctrl Pts',(-3.65084443590249,3.23184317427172,
-6.55239843112517));
#105970=CARTESIAN_POINT('Ctrl Pts',(-3.55201981981194,3.21428571395853,
-6.6055397349545));
#105971=CARTESIAN_POINT('Ctrl Pts',(-3.48365954638371,3.20214063501282,
-6.64229934251993));
#105972=CARTESIAN_POINT('Ctrl Pts',(-3.41460885920532,3.18993125792547,
-6.67806185439175));
#105973=CARTESIAN_POINT('Ctrl Pts',(-3.34491184770643,3.17766594611633,
-6.71279112818426));
#105974=CARTESIAN_POINT('Ctrl Pts',(-3.23191703662374,3.13852541813812,
-6.4897775205516));
#105975=CARTESIAN_POINT('Ctrl Pts',(-3.25068803514173,3.14538569335125,
-6.52690738312565));
#105976=CARTESIAN_POINT('Ctrl Pts',(-3.26950140689733,3.15207184262519,
-6.56407746803246));
#105977=CARTESIAN_POINT('Ctrl Pts',(-3.30716098130688,3.16510741642107,
-6.63840257006474));
#105978=CARTESIAN_POINT('Ctrl Pts',(-3.32602929113069,3.17146448706224,
-6.67560121406347));
#105979=CARTESIAN_POINT('Ctrl Pts',(-3.34491184880586,3.17766594630695,
-6.7127911275902));
#105980=CARTESIAN_POINT('Ctrl Pts',(-2.82522894021175,3.26861999521842,
-6.94752811231027));
#105981=CARTESIAN_POINT('Ctrl Pts',(-2.82897409110587,3.26797796010921,
-6.94600042815513));
#105982=CARTESIAN_POINT('Ctrl Pts',(-2.832719242,3.267335925,-6.944472744));
#105983=CARTESIAN_POINT('Ctrl Pts',(-3.208742396,3.202873885,-6.791089174));
#105984=CARTESIAN_POINT('Ctrl Pts',(-3.566005068,3.137747733,-6.598000292));
#105985=CARTESIAN_POINT('Ctrl Pts',(-2.5093333767475,3.26861999521842,-6.80189732065103));
#105986=CARTESIAN_POINT('Ctrl Pts',(-2.51300017287375,3.26797796010921,
-6.80054008332552));
#105987=CARTESIAN_POINT('Ctrl Pts',(-2.516666969,3.267335925,-6.799182846));
#105988=CARTESIAN_POINT('Ctrl Pts',(-2.884823095,3.202873885,-6.662912593));
#105989=CARTESIAN_POINT('Ctrl Pts',(-3.23611259,3.137747733,-6.487686437));
#105990=CARTESIAN_POINT('',(-2.83271923294473,3.2673359258261,-6.9444727279121));
#105991=CARTESIAN_POINT('Origin',(0.0969947647447311,3.08932521811194,0.162888536788507));
#105992=CARTESIAN_POINT('',(-2.67469311915078,3.26733592735283,-6.87182778968677));
#105993=CARTESIAN_POINT('Origin',(-5.73109268375838E-13,3.358063799999,
-1.16746889933239E-12));
#105994=CARTESIAN_POINT('',(-3.34678523580795,3.35698786818467,-6.71185731223826));
#105995=CARTESIAN_POINT('Origin',(0.117122493434923,3.08947601560677,0.140959894909082));
#105996=CARTESIAN_POINT('Origin',(0.101030779572149,3.48205907864295,0.15779271281936));
#105997=CARTESIAN_POINT('Ctrl Pts',(-1.577585275,3.13774478,-7.332204628));
#105998=CARTESIAN_POINT('Ctrl Pts',(-1.81518665,3.176256335,-7.2810827));
#105999=CARTESIAN_POINT('Ctrl Pts',(-2.048979786,3.214285714,-7.214685152));
#106000=CARTESIAN_POINT('Ctrl Pts',(-2.211297151,3.240688665,-7.16858681300001));
#106001=CARTESIAN_POINT('Ctrl Pts',(-2.37137707,3.267335925,-7.115235119));
#106002=CARTESIAN_POINT('Ctrl Pts',(-2.37528892539741,3.26798710116569,
-7.11393136951387));
#106003=CARTESIAN_POINT('Ctrl Pts',(-2.37920078079482,3.26863827733136,
-7.11262762002775));
#106004=CARTESIAN_POINT('Ctrl Pts',(-1.756626078,3.13774478,-7.033972194));
#106005=CARTESIAN_POINT('Ctrl Pts',(-1.984563179,3.176256335,-6.977048418));
#106006=CARTESIAN_POINT('Ctrl Pts',(-2.208336691,3.214285714,-6.905486881));
#106007=CARTESIAN_POINT('Ctrl Pts',(-2.363697654,3.240688665,-6.8558033));
#106008=CARTESIAN_POINT('Ctrl Pts',(-2.516666969,3.267335925,-6.79918284600001));
#106009=CARTESIAN_POINT('Ctrl Pts',(-2.52040506334849,3.26798710116569,
-6.7977992181848));
#106010=CARTESIAN_POINT('Ctrl Pts',(-2.52414315769698,3.26863827733136,
-6.79641559036959));
#106011=CARTESIAN_POINT('',(-2.37137706833076,3.26733592550877,-7.11523511726489));
#106012=CARTESIAN_POINT('',(-2.44402201117849,3.26733592642396,-6.9572089854233));
#106013=CARTESIAN_POINT('',(-1.82365800373359,3.17766594632019,-7.27490697422542));
#106014=CARTESIAN_POINT('Ctrl Pts',(-2.37137706908236,3.26733592483625,
-7.11523511918416));
#106015=CARTESIAN_POINT('Ctrl Pts',(-2.26444072465427,3.24953506265028,
-7.15087503666887));
#106016=CARTESIAN_POINT('Ctrl Pts',(-2.15691774689163,3.23184317427153,
-7.18403063290066));
#106017=CARTESIAN_POINT('Ctrl Pts',(-2.0489797858413,3.21428571392076,-7.21468515150108));
#106018=CARTESIAN_POINT('Ctrl Pts',(-1.97431550870438,3.20214063496236,
-7.23588990102936));
#106019=CARTESIAN_POINT('Ctrl Pts',(-1.89919130530067,3.18993125794642,
-7.25597244897035));
#106020=CARTESIAN_POINT('Ctrl Pts',(-1.8236580037907,3.17766594613755,-7.27490697433494));
#106021=CARTESIAN_POINT('Ctrl Pts',(-1.76124628115218,3.13852541813551,
-7.03281675718453));
#106022=CARTESIAN_POINT('Ctrl Pts',(-1.77159658622382,3.14538568332313,
-7.07311369491504));
#106023=CARTESIAN_POINT('Ctrl Pts',(-1.78197962487405,3.15207182215019,
-7.11345901470548));
#106024=CARTESIAN_POINT('Ctrl Pts',(-1.80278107244631,3.16510741643744,
-7.19414225903988));
#106025=CARTESIAN_POINT('Ctrl Pts',(-1.81321164292256,3.17146448706018,
-7.2345273480934));
#106026=CARTESIAN_POINT('Ctrl Pts',(-1.82365800497128,3.17766594630979,
-7.27490697385328));
#106027=CARTESIAN_POINT('Ctrl Pts',(-1.26566348041818,3.26861999521842,
-7.39243947503579));
#106028=CARTESIAN_POINT('Ctrl Pts',(-1.26964947870909,3.26797796010921,
-7.3917526040179));
#106029=CARTESIAN_POINT('Ctrl Pts',(-1.273635477,3.267335925,-7.391065733));
#106030=CARTESIAN_POINT('Ctrl Pts',(-1.673840353,3.202873885,-7.322102048));
#106031=CARTESIAN_POINT('Ctrl Pts',(-2.064258824,3.137747733,-7.210328391));
#106032=CARTESIAN_POINT('Ctrl Pts',(-0.988459695241115,3.26861999521842,
-7.18230524117258));
#106033=CARTESIAN_POINT('Ctrl Pts',(-0.992332529620557,3.26797796010921,
-7.18176798808629));
#106034=CARTESIAN_POINT('Ctrl Pts',(-0.996205364,3.267335925,-7.181230735));
#106035=CARTESIAN_POINT('Ctrl Pts',(-1.385048281,3.202873885,-7.12728909));
#106036=CARTESIAN_POINT('Ctrl Pts',(-1.765793266,3.137747733,-7.031676482));
#106037=CARTESIAN_POINT('',(-1.27363547160765,3.2673359258261,-7.39106571533973));
#106038=CARTESIAN_POINT('Origin',(0.0597108984205369,3.08932518088346,0.179931436801557));
#106039=CARTESIAN_POINT('',(-1.13492043497381,3.26733592735283,-7.28614823174549));
#106040=CARTESIAN_POINT('Origin',(1.57751416096641E-13,3.35806379999978,
5.0263612716428E-13));
#106041=CARTESIAN_POINT('',(-1.82568833597157,3.3569878682181,-7.27439771350992));
#106042=CARTESIAN_POINT('Origin',(0.0840819809147508,3.08947608719351,0.162842126678377));
#106043=CARTESIAN_POINT('Origin',(0.064747991376177,3.4820590220708,0.175822390860044));
#106044=CARTESIAN_POINT('Ctrl Pts',(0.035505048,3.13774478,-7.49991595900001));
#106045=CARTESIAN_POINT('Ctrl Pts',(-0.207531042,3.176256335,-7.501066506));
#106046=CARTESIAN_POINT('Ctrl Pts',(-0.450131734,3.214285714,-7.486479909));
#106047=CARTESIAN_POINT('Ctrl Pts',(-0.618563989,3.240688665,-7.476352759));
#106048=CARTESIAN_POINT('Ctrl Pts',(-0.786370366,3.267335925,-7.458660848));
#106049=CARTESIAN_POINT('Ctrl Pts',(-0.790471032002883,3.26798710116569,
-7.45822851271418));
#106050=CARTESIAN_POINT('Ctrl Pts',(-0.794571698005766,3.26863827733136,
-7.45779617742834));
#106051=CARTESIAN_POINT('Ctrl Pts',(-0.203461038,3.13774478,-7.24714451400001));
#106052=CARTESIAN_POINT('Ctrl Pts',(-0.438306025,3.176256335,-7.240551323));
#106053=CARTESIAN_POINT('Ctrl Pts',(-0.672231452,3.214285714,-7.218767545));
#106054=CARTESIAN_POINT('Ctrl Pts',(-0.834640663,3.240688665,-7.203643554));
#106055=CARTESIAN_POINT('Ctrl Pts',(-0.996205363999999,3.267335925,-7.181230735));
#106056=CARTESIAN_POINT('Ctrl Pts',(-1.00015350285206,3.26798710116569,
-7.18068303540392));
#106057=CARTESIAN_POINT('Ctrl Pts',(-1.00410164170411,3.26863827733136,
-7.18013533580784));
#106058=CARTESIAN_POINT('',(-0.891287856244616,3.26733592642396,-7.31994579256607));
#106059=CARTESIAN_POINT('Ctrl Pts',(-0.208221607850335,3.13852541811002,
-7.24700929788454));
#106060=CARTESIAN_POINT('Ctrl Pts',(-0.209667279556549,3.14538569103608,
-7.28858917220968));
#106061=CARTESIAN_POINT('Ctrl Pts',(-0.211134519267141,3.15207183792157,
-7.33022334130803));
#106062=CARTESIAN_POINT('Ctrl Pts',(-0.214105124329206,3.16510741640027,
-7.41349185170254));
#106063=CARTESIAN_POINT('Ctrl Pts',(-0.215610233503705,3.17146448703367,
-7.4551750242645));
#106064=CARTESIAN_POINT('Ctrl Pts',(-0.217131939498219,3.17766594626658,
-7.49685625577675));
#106065=CARTESIAN_POINT('Ctrl Pts',(0.35308299665963,3.26861999521842,-7.49168858409584));
#106066=CARTESIAN_POINT('Ctrl Pts',(0.349042531829815,3.26797796010921,
-7.49187464354792));
#106067=CARTESIAN_POINT('Ctrl Pts',(0.345002067,3.267335925,-7.49206070300001));
#106068=CARTESIAN_POINT('Ctrl Pts',(-0.060671395,3.202873885,-7.510741569));
#106069=CARTESIAN_POINT('Ctrl Pts',(-0.465990131,3.137747733,-7.485509548));
#106070=CARTESIAN_POINT('Ctrl Pts',(0.578633262375529,3.26861999521842,
-7.22687655198706));
#106071=CARTESIAN_POINT('Ctrl Pts',(0.574735479187765,3.26797796010921,
-7.22718440449353));
#106072=CARTESIAN_POINT('Ctrl Pts',(0.570837696,3.267335925,-7.227492257));
#106073=CARTESIAN_POINT('Ctrl Pts',(0.179489852,3.202873885,-7.258401471));
#106074=CARTESIAN_POINT('Ctrl Pts',(-0.212907412,3.137747733,-7.246873149));
#106075=CARTESIAN_POINT('',(0.457919866872506,3.26733592735402,-7.35977648091011));
#106076=CARTESIAN_POINT('Ctrl Pts',(1.646935195,3.13774478,-7.316939556));
#106077=CARTESIAN_POINT('Ctrl Pts',(1.409828488,3.176256335,-7.370308779));
#106078=CARTESIAN_POINT('Ctrl Pts',(1.169763977,3.214285714,-7.408215186));
#106079=CARTESIAN_POINT('Ctrl Pts',(1.003092537,3.240688665,-7.434532759));
#106080=CARTESIAN_POINT('Ctrl Pts',(0.835406142,3.267335925,-7.453327886));
#106081=CARTESIAN_POINT('Ctrl Pts',(0.831308407984072,3.26798710116569,
-7.45378718045404));
#106082=CARTESIAN_POINT('Ctrl Pts',(0.827210673968144,3.26863827733136,
-7.45424647490808));
#106083=CARTESIAN_POINT('Ctrl Pts',(1.359217614,3.13774478,-7.121448411));
#106084=CARTESIAN_POINT('Ctrl Pts',(1.128445831,3.176256335,-7.16549409600001));
#106085=CARTESIAN_POINT('Ctrl Pts',(0.895306583,3.214285714,-7.194506663));
#106086=CARTESIAN_POINT('Ctrl Pts',(0.733443198,3.240688665,-7.214649441));
#106087=CARTESIAN_POINT('Ctrl Pts',(0.570837696,3.267335925,-7.227492257));
#106088=CARTESIAN_POINT('Ctrl Pts',(0.566864123208228,3.26798710116569,
-7.22780609548393));
#106089=CARTESIAN_POINT('Ctrl Pts',(0.562890550416455,3.26863827733136,
-7.22811993396787));
#106090=CARTESIAN_POINT('',(0.835406142818811,3.26733592550878,-7.45332788373253));
#106091=CARTESIAN_POINT('',(0.703121927779861,3.26733592642396,-7.340410070659));
#106092=CARTESIAN_POINT('',(1.39954697555713,3.17766594628976,-7.3682608711216));
#106093=CARTESIAN_POINT('Ctrl Pts',(0.835406142940577,3.26733592483152,
-7.45332788577904));
#106094=CARTESIAN_POINT('Ctrl Pts',(0.94742375383149,3.24953506265028,-7.44077239346166));
#106095=CARTESIAN_POINT('Ctrl Pts',(1.05893063889937,3.23184317427131,-7.42571587126418));
#106096=CARTESIAN_POINT('Ctrl Pts',(1.16976397728219,3.21428571387816,-7.4082151854994));
#106097=CARTESIAN_POINT('Ctrl Pts',(1.24643108382801,3.20214063485909,-7.3961093787905));
#106098=CARTESIAN_POINT('Ctrl Pts',(1.32304440699507,3.18993125789757,-7.38279197147513));
#106099=CARTESIAN_POINT('Ctrl Pts',(1.39954697551669,3.17766594608606,-7.36826087108064));
#106100=CARTESIAN_POINT('Ctrl Pts',(1.3545392766959,3.13852541811858,-7.12233973838241));
#106101=CARTESIAN_POINT('Ctrl Pts',(1.36206584354755,3.14538568717469,-7.16325825206757));
#106102=CARTESIAN_POINT('Ctrl Pts',(1.36958301790223,3.1520718300302,-7.20423442404044));
#106103=CARTESIAN_POINT('Ctrl Pts',(1.38458214145238,3.16510741642671,-7.28619480500098));
#106104=CARTESIAN_POINT('Ctrl Pts',(1.39207287092915,3.17146448706813,-7.32722700216388));
#106105=CARTESIAN_POINT('Ctrl Pts',(1.39954697430732,3.17766594628681,-7.3682608713497));
#106106=CARTESIAN_POINT('Ctrl Pts',(1.95531970545204,3.26861999521842,-7.24063466103159));
#106107=CARTESIAN_POINT('Ctrl Pts',(1.95141370172602,3.26797796010921,-7.2416849510158));
#106108=CARTESIAN_POINT('Ctrl Pts',(1.947507698,3.267335925,-7.242735241));
#106109=CARTESIAN_POINT('Ctrl Pts',(1.55533449,3.202873885,-7.348187161));
#106110=CARTESIAN_POINT('Ctrl Pts',(1.154067742,3.137747733,-7.410676599));
#106111=CARTESIAN_POINT('Ctrl Pts',(2.11866997199718,3.26861999521842,-6.93352714751366));
#106112=CARTESIAN_POINT('Ctrl Pts',(2.11492949599859,3.26797796010921,-6.93466571075683));
#106113=CARTESIAN_POINT('Ctrl Pts',(2.11118902,3.267335925,-6.93580427400001));
#106114=CARTESIAN_POINT('Ctrl Pts',(1.735635238,3.202873885,-7.050119065));
#106115=CARTESIAN_POINT('Ctrl Pts',(1.349933756,3.137747733,-7.123214082));
#106116=CARTESIAN_POINT('',(1.94750769550073,3.26733592582611,-7.2427352226932));
#106117=CARTESIAN_POINT('Origin',(-0.0213591459166254,3.08932517974553,
0.188373488840997));
#106118=CARTESIAN_POINT('',(2.02934834491728,3.26733592735283,-7.08926976153127));
#106119=CARTESIAN_POINT('Origin',(-1.20996962449382E-13,3.3580638,4.05491612509579E-13));
#106120=CARTESIAN_POINT('',(1.39749046265521,3.35698786822937,-7.36865119336134));
#106121=CARTESIAN_POINT('Origin',(0.00793508467649223,3.08947604551196,
0.183096902086818));
#106122=CARTESIAN_POINT('Origin',(-0.0150621914402294,3.48205902360382,
0.186758929055496));
#106123=CARTESIAN_POINT('Ctrl Pts',(3.181356483,3.13774478,-6.791831191));
#106124=CARTESIAN_POINT('Ctrl Pts',(2.961266004,3.176256335,-6.894923605));
#106125=CARTESIAN_POINT('Ctrl Pts',(2.734962825,3.214285714,-6.983550554));
#106126=CARTESIAN_POINT('Ctrl Pts',(2.577845571,3.240688665,-7.04508227100001));
#106127=CARTESIAN_POINT('Ctrl Pts',(2.418119987,3.267335925,-7.099485596));
#106128=CARTESIAN_POINT('Ctrl Pts',(2.41421679044806,3.26798710116569,-7.10081504407736));
#106129=CARTESIAN_POINT('Ctrl Pts',(2.41031359389613,3.26863827733136,-7.10214449215472));
#106130=CARTESIAN_POINT('Ctrl Pts',(2.858340762,3.13774478,-6.662761296));
#106131=CARTESIAN_POINT('Ctrl Pts',(2.642432815,3.176256335,-6.755386329));
#106132=CARTESIAN_POINT('Ctrl Pts',(2.420981077,3.214285714,-6.833838645));
#106133=CARTESIAN_POINT('Ctrl Pts',(2.26723207,3.240688665,-6.88830634));
#106134=CARTESIAN_POINT('Ctrl Pts',(2.11118902,3.267335925,-6.935804274));
#106135=CARTESIAN_POINT('Ctrl Pts',(2.10737581312693,3.26798710116569,-6.93696497579598));
#106136=CARTESIAN_POINT('Ctrl Pts',(2.10356260625386,3.26863827733136,-6.93812567759196));
#106137=CARTESIAN_POINT('',(2.41811998730806,3.26733592550877,-7.09948559360933));
#106138=CARTESIAN_POINT('',(2.2646545118938,3.26733592642396,-7.01764493229125));
#106139=CARTESIAN_POINT('',(2.95078462776239,3.17766594632317,-6.89513379697716));
#106140=CARTESIAN_POINT('Ctrl Pts',(2.41811998786744,3.26733592483209,-7.09948559558307));
#106141=CARTESIAN_POINT('Ctrl Pts',(2.52481962986193,3.24953506265028,-7.0631431689244));
#106142=CARTESIAN_POINT('Ctrl Pts',(2.63048283882753,3.23184317427183,-7.02446797538068));
#106143=CARTESIAN_POINT('Ctrl Pts',(2.73496282496311,3.21428571397938,-6.98355055387583));
#106144=CARTESIAN_POINT('Ctrl Pts',(2.80723510623411,3.20214063505568,-6.95524661319201));
#106145=CARTESIAN_POINT('Ctrl Pts',(2.87919440373112,3.18993125793867,-6.9257709591031));
#106146=CARTESIAN_POINT('Ctrl Pts',(2.95078462775552,3.1776659461331,-6.89513379703719));
#106147=CARTESIAN_POINT('Ctrl Pts',(2.85396340915401,3.1385254181184,-6.66463748826854));
#106148=CARTESIAN_POINT('Ctrl Pts',(2.87011029021384,3.14538569143452,-6.70298138426603));
#106149=CARTESIAN_POINT('Ctrl Pts',(2.88626039462627,3.15207183875374,-6.74138361346276));
#106150=CARTESIAN_POINT('Ctrl Pts',(2.91852788258014,3.16510741556512,-6.81820338161874));
#106151=CARTESIAN_POINT('Ctrl Pts',(2.93466419007876,3.17146448533258,-6.85666597771207));
#106152=CARTESIAN_POINT('Ctrl Pts',(2.95078462657957,3.17766594631795,-6.89513379745628));
#106153=CARTESIAN_POINT('Ctrl Pts',(3.46612783746513,3.26861999521842,-6.65101670874053));
#106154=CARTESIAN_POINT('Ctrl Pts',(3.46253893523256,3.26797796010921,-6.65288211887026));
#106155=CARTESIAN_POINT('Ctrl Pts',(3.458950033,3.267335925,-6.654747529));
#106156=CARTESIAN_POINT('Ctrl Pts',(3.098614662,3.202873885,-6.842039689));
#106157=CARTESIAN_POINT('Ctrl Pts',(2.72016269,3.137747733,-6.989328647));
#106158=CARTESIAN_POINT('Ctrl Pts',(3.55964002860692,3.26861999521842,-6.31597371891253));
#106159=CARTESIAN_POINT('Ctrl Pts',(3.55623176030346,3.26797796010921,-6.31788975495627));
#106160=CARTESIAN_POINT('Ctrl Pts',(3.552823492,3.267335925,-6.319805791));
#106161=CARTESIAN_POINT('Ctrl Pts',(3.21062425,3.202873885,-6.512180928));
#106162=CARTESIAN_POINT('Ctrl Pts',(2.849653521,3.137747733,-6.666481441));
#106163=CARTESIAN_POINT('',(3.45895002662524,3.26733592582611,-6.65474751165654));
#106164=CARTESIAN_POINT('Origin',(-0.0613544418924655,3.08932515244115,
0.179377709456058));
#106165=CARTESIAN_POINT('',(3.50588674961313,3.26733592735283,-6.48727666696439));
#106166=CARTESIAN_POINT('Origin',(-1.83013326715553E-13,3.35806380000067,
3.60822483003176E-13));
#106167=CARTESIAN_POINT('',(2.94886010292606,3.35698786820659,-6.89595708331305));
#106168=CARTESIAN_POINT('Origin',(-0.0316109121111718,3.08947599794032,
0.18052218025897));
#106169=CARTESIAN_POINT('Origin',(-0.0548577581699217,3.48205904643279,
0.179154830677182));
#106170=CARTESIAN_POINT('Ctrl Pts',(4.567021077,3.13774478,-5.949144349));
#106171=CARTESIAN_POINT('Ctrl Pts',(4.374238013,3.176256335,-6.097139466));
#106172=CARTESIAN_POINT('Ctrl Pts',(4.172277851,3.214285714,-6.232342861));
#106173=CARTESIAN_POINT('Ctrl Pts',(4.032061411,3.240688665,-6.326211565));
#106174=CARTESIAN_POINT('Ctrl Pts',(3.88776523,3.267335925,-6.41367925));
#106175=CARTESIAN_POINT('Ctrl Pts',(3.88423908007441,3.26798710116569,-6.41581668821089));
#106176=CARTESIAN_POINT('Ctrl Pts',(3.88071293014881,3.26863827733136,-6.41795412642177));
#106177=CARTESIAN_POINT('Ctrl Pts',(4.223811072,3.13774478,-5.89253086800001));
#106178=CARTESIAN_POINT('Ctrl Pts',(4.032862577,3.176256335,-6.029404205));
#106179=CARTESIAN_POINT('Ctrl Pts',(3.833453187,3.214285714,-6.153627927));
#106180=CARTESIAN_POINT('Ctrl Pts',(3.69500769,3.240688665,-6.239873689));
#106181=CARTESIAN_POINT('Ctrl Pts',(3.552823492,3.267335925,-6.319805791));
#106182=CARTESIAN_POINT('Ctrl Pts',(3.549348952371,3.26798710116569,-6.32175908299683));
#106183=CARTESIAN_POINT('Ctrl Pts',(3.54587441274199,3.26863827733136,-6.32371237499365));
#106184=CARTESIAN_POINT('',(3.88776522976391,3.26733592550877,-6.41367924760373));
#106185=CARTESIAN_POINT('',(3.72029436861526,3.26733592642396,-6.36674251605016));
#106186=CARTESIAN_POINT('',(4.36404687056657,3.17766594631752,-6.09959793024141));
#106187=CARTESIAN_POINT('Ctrl Pts',(3.88776523073915,3.26733592483553,-6.41367924941769));
#106188=CARTESIAN_POINT('Ctrl Pts',(3.9841577463695,3.24953506265028,-6.35524921920966));
#106189=CARTESIAN_POINT('Ctrl Pts',(4.07903658468512,3.23184317427146,-6.29476376382527));
#106190=CARTESIAN_POINT('Ctrl Pts',(4.17227785102703,3.21428571390619,-6.23234286055702));
#106191=CARTESIAN_POINT('Ctrl Pts',(4.23677593593141,3.20214063493194,-6.18916424567221));
#106192=CARTESIAN_POINT('Ctrl Pts',(4.30071647048087,3.18993125793788,-6.14490859455356));
#106193=CARTESIAN_POINT('Ctrl Pts',(4.36404687058658,3.17766594612954,-6.09959793032027));
#106194=CARTESIAN_POINT('Ctrl Pts',(4.21993938588018,3.13852541808793,-5.89530419738614));
#106195=CARTESIAN_POINT('Ctrl Pts',(4.24395154840076,3.14538568641129,-5.92928050744133));
#106196=CARTESIAN_POINT('Ctrl Pts',(4.26797939619281,3.15207182851426,-5.9633130900975));
#106197=CARTESIAN_POINT('Ctrl Pts',(4.31600650821998,3.16510741641384,-6.03140035644281));
#106198=CARTESIAN_POINT('Ctrl Pts',(4.3400338824849,3.17146448705569,-6.06549489429013));
#106199=CARTESIAN_POINT('Ctrl Pts',(4.36404686950019,3.17766594631037,-6.09959793095783));
#106200=CARTESIAN_POINT('Ctrl Pts',(4.81486368430831,3.26861999521842,-5.75040460645348));
#106201=CARTESIAN_POINT('Ctrl Pts',(4.81175969665416,3.26797796010921,-5.75299791222674));
#106202=CARTESIAN_POINT('Ctrl Pts',(4.808655709,3.267335925,-5.755591218));
#106203=CARTESIAN_POINT('Ctrl Pts',(4.497007057,3.202873885,-6.015966045));
#106204=CARTESIAN_POINT('Ctrl Pts',(4.159065854,3.137747733,-6.241167457));
#106205=CARTESIAN_POINT('Ctrl Pts',(4.83416527354552,3.26861999521842,-5.40309237873128));
#106206=CARTESIAN_POINT('Ctrl Pts',(4.83124857977277,3.26797796010921,-5.40569629586564));
#106207=CARTESIAN_POINT('Ctrl Pts',(4.828331886,3.267335925,-5.40830021300001));
#106208=CARTESIAN_POINT('Ctrl Pts',(4.53548804,3.202873885,-5.669740449));
#106209=CARTESIAN_POINT('Ctrl Pts',(4.216126656,3.137747733,-5.898031538));
#106210=CARTESIAN_POINT('',(4.80865569902819,3.26733592582611,-5.75559120246355));
#106211=CARTESIAN_POINT('Origin',(-0.0984809776797785,3.08932516186255,
0.161994630856843));
#106212=CARTESIAN_POINT('',(4.81849378641155,3.26733592735283,-5.58194572507186));
#106213=CARTESIAN_POINT('Origin',(-1.25051878574478E-12,3.35806380000044,
1.72258041164497E-12));
#106214=CARTESIAN_POINT('',(4.36234432258694,3.35698786820303,-6.10081568391773));
#106215=CARTESIAN_POINT('Origin',(-0.0696785071250122,3.08947601273034,
0.169505791713984));
#106216=CARTESIAN_POINT('Origin',(-0.09208796268315,3.48205902148428,0.163173162085032));
#106217=CARTESIAN_POINT('Ctrl Pts',(5.739136842,3.13774478,-4.828282128));
#106218=CARTESIAN_POINT('Ctrl Pts',(5.58267551400001,3.176256335,-5.014259863));
#106219=CARTESIAN_POINT('Ctrl Pts',(5.414501802,3.214285714,-5.189717742));
#106220=CARTESIAN_POINT('Ctrl Pts',(5.29774254,3.240688665,-5.311534238));
#106221=CARTESIAN_POINT('Ctrl Pts',(5.175622891,3.267335925,-5.42797639000001));
#106222=CARTESIAN_POINT('Ctrl Pts',(5.17263866655102,3.26798710116569,-5.43082187407841));
#106223=CARTESIAN_POINT('Ctrl Pts',(5.16965444210204,3.26863827733136,-5.43366735815682));
#106224=CARTESIAN_POINT('Ctrl Pts',(5.391780671,3.13774478,-4.846772245));
#106225=CARTESIAN_POINT('Ctrl Pts',(5.234720168,3.176256335,-5.021493842));
#106226=CARTESIAN_POINT('Ctrl Pts',(5.066677286,3.214285714,-5.185680407));
#106227=CARTESIAN_POINT('Ctrl Pts',(4.950008857,3.240688665,-5.29967148));
#106228=CARTESIAN_POINT('Ctrl Pts',(4.828331886,3.267335925,-5.408300213));
#106229=CARTESIAN_POINT('Ctrl Pts',(4.82535847922468,3.26798710116569,-5.41095476141654));
#106230=CARTESIAN_POINT('Ctrl Pts',(4.82238507244937,3.26863827733136,-5.41360930983306));
#106231=CARTESIAN_POINT('',(5.17562289027218,3.26733592550877,-5.4279763877023));
#106232=CARTESIAN_POINT('',(5.00197739498063,3.26733592642396,-5.41813829551714));
#106233=CARTESIAN_POINT('',(5.57325113228991,3.17766594629067,-5.01885164342991));
#106234=CARTESIAN_POINT('Ctrl Pts',(5.17562289160948,3.26733592483259,-5.42797638925954));
#106235=CARTESIAN_POINT('Ctrl Pts',(5.25720107397617,3.24953506265028,-5.35019087963773));
#106236=CARTESIAN_POINT('Ctrl Pts',(5.33685911291995,3.23184317427168,-5.27072339506802));
#106237=CARTESIAN_POINT('Ctrl Pts',(5.41450180158225,3.21428571395063,-5.18971774176483));
#106238=CARTESIAN_POINT('Ctrl Pts',(5.46820983098211,3.20214063499304,-5.13368343749541));
#106239=CARTESIAN_POINT('Ctrl Pts',(5.52114181517994,3.1899312579122,-5.07671713370057));
#106240=CARTESIAN_POINT('Ctrl Pts',(5.57325113229803,3.17766594609559,-5.01885164347858));
#106241=CARTESIAN_POINT('Ctrl Pts',(5.38859568690581,3.13852541812473,-4.85031303370965));
#106242=CARTESIAN_POINT('Ctrl Pts',(5.41935036615269,3.14538568767711,-4.87833309643387));
#106243=CARTESIAN_POINT('Ctrl Pts',(5.45013246174096,3.15207183104302,-4.90640474502264));
#106244=CARTESIAN_POINT('Ctrl Pts',(5.5116734644145,3.16510741642622,-4.96257574886785));
#106245=CARTESIAN_POINT('Ctrl Pts',(5.54246840988429,3.17146448705763,-4.99070800020555));
#106246=CARTESIAN_POINT('Ctrl Pts',(5.57325113140873,3.17766594628625,-5.01885164437964));
#106247=CARTESIAN_POINT('Ctrl Pts',(5.93846185711766,3.26861999521842,-4.58090997634739));
#106248=CARTESIAN_POINT('Ctrl Pts',(5.93598792305883,3.26797796010921,-4.5841099176737));
#106249=CARTESIAN_POINT('Ctrl Pts',(5.933513989,3.267335925,-4.587309859));
#106250=CARTESIAN_POINT('Ctrl Pts',(5.685124401,3.202873885,-4.908592516));
#106251=CARTESIAN_POINT('Ctrl Pts',(5.403495721,3.137747733,-5.201176212));
#106252=CARTESIAN_POINT('Ctrl Pts',(5.88265032276119,3.26861999521842,-4.23756844513487));
#106253=CARTESIAN_POINT('Ctrl Pts',(5.8803615848806,3.26797796010921,-4.24073848706743));
#106254=CARTESIAN_POINT('Ctrl Pts',(5.878072847,3.267335925,-4.243908529));
#106255=CARTESIAN_POINT('Ctrl Pts',(5.64827745,3.202873885,-4.562189207));
#106256=CARTESIAN_POINT('Ctrl Pts',(5.385458394,3.137747733,-4.853796235));
#106257=CARTESIAN_POINT('',(5.93351397592557,3.2673359258261,-4.58730984595519));
#106258=CARTESIAN_POINT('Origin',(-0.13100224346366,3.08932516317078,0.137036486033113));
#106259=CARTESIAN_POINT('',(5.90579340922846,3.26733592735283,-4.41560920573176));
#106260=CARTESIAN_POINT('Origin',(5.63785129692462E-15,3.35806379999922,
1.34441069388203E-13));
#106261=CARTESIAN_POINT('',(5.57185016983664,3.35698786820608,-5.02040692449348));
#106262=CARTESIAN_POINT('Origin',(-0.104488342131043,3.08947596006111,0.150564189048316));
#106263=CARTESIAN_POINT('Origin',(-0.125012668882279,3.48205909152955,0.139562309966013));
#106264=CARTESIAN_POINT('Ctrl Pts',(6.642896946,3.13774478,-3.481654802));
#106265=CARTESIAN_POINT('Ctrl Pts',(6.530073313,3.176256335,-3.696919041));
#106266=CARTESIAN_POINT('Ctrl Pts',(6.403549666,3.214285714,-3.904427189));
#106267=CARTESIAN_POINT('Ctrl Pts',(6.315707117,3.240688665,-4.048495473));
#106268=CARTESIAN_POINT('Ctrl Pts',(6.221474178,3.267335925,-4.188467387));
#106269=CARTESIAN_POINT('Ctrl Pts',(6.21917141802021,3.26798710116569,-4.19188786528789));
#106270=CARTESIAN_POINT('Ctrl Pts',(6.21686865804042,3.26863827733136,-4.19530834357579));
#106271=CARTESIAN_POINT('Ctrl Pts',(6.307636598,3.13774478,-3.574383939));
#106272=CARTESIAN_POINT('Ctrl Pts',(6.191808061,3.176256335,-3.778784008));
#106273=CARTESIAN_POINT('Ctrl Pts',(6.062989186,3.214285714,-3.975256234));
#106274=CARTESIAN_POINT('Ctrl Pts',(5.973553112,3.240688665,-4.111662523));
#106275=CARTESIAN_POINT('Ctrl Pts',(5.878072847,3.267335925,-4.243908529));
#106276=CARTESIAN_POINT('Ctrl Pts',(5.87573960625175,3.26798710116569,-4.24714021012271));
#106277=CARTESIAN_POINT('Ctrl Pts',(5.87340636550352,3.26863827733136,-4.25037189124542));
#106278=CARTESIAN_POINT('',(6.22147417679744,3.26733592550878,-4.18846738491078));
#106279=CARTESIAN_POINT('',(6.04977351754298,3.26733592642396,-4.21618795076387));
#106280=CARTESIAN_POINT('',(6.52185636487934,3.177665946289,-3.70342943169034));
#106281=CARTESIAN_POINT('Ctrl Pts',(6.22147417843737,3.26733592483217,-4.18846738614363));
#106282=CARTESIAN_POINT('Ctrl Pts',(6.28442352312444,3.24953506265028,-4.09496356066983));
#106283=CARTESIAN_POINT('Ctrl Pts',(6.34513604112105,3.23184317427178,-4.00022985798987));
#106284=CARTESIAN_POINT('Ctrl Pts',(6.40354966577435,3.21428571396938,-3.90442718890104));
#106285=CARTESIAN_POINT('Ctrl Pts',(6.44395631252021,3.20214063502836,-3.83815729691068));
#106286=CARTESIAN_POINT('Ctrl Pts',(6.4834047045776,3.18993125791671,-3.77114402172454));
#106287=CARTESIAN_POINT('Ctrl Pts',(6.52185636493112,3.17766594609818,-3.70342943175431));
#106288=CARTESIAN_POINT('Ctrl Pts',(6.30528724149941,3.13852541814473,-3.57852662369783));
#106289=CARTESIAN_POINT('Ctrl Pts',(6.34134639814436,3.14538569135369,-3.59928025709094));
#106290=CARTESIAN_POINT('Ctrl Pts',(6.37744342249335,3.15207183854731,-3.62007837831597));
#106291=CARTESIAN_POINT('Ctrl Pts',(6.44962069464325,3.16510741639835,-3.6617066147144));
#106292=CARTESIAN_POINT('Ctrl Pts',(6.48574327389207,3.1714644870305,-3.68256114658771));
#106293=CARTESIAN_POINT('Ctrl Pts',(6.52185636420256,3.17766594628177,-3.70342943280469));
#106294=CARTESIAN_POINT('Ctrl Pts',(6.78438415313431,3.26861999521842,-3.1972170876818));
#106295=CARTESIAN_POINT('Ctrl Pts',(6.78265595106716,3.26797796010921,-3.2008740388409));
#106296=CARTESIAN_POINT('Ctrl Pts',(6.780927749,3.267335925,-3.20453099));
#106297=CARTESIAN_POINT('Ctrl Pts',(6.607411645,3.202873885,-3.571698655));
#106298=CARTESIAN_POINT('Ctrl Pts',(6.395264134,3.137747733,-3.917983749));
#106299=CARTESIAN_POINT('Ctrl Pts',(6.65606918130502,3.26861999521842,-2.87390051977844));
#106300=CARTESIAN_POINT('Ctrl Pts',(6.65451541815251,3.26797796010921,-2.87748845888922));
#106301=CARTESIAN_POINT('Ctrl Pts',(6.652961655,3.267335925,-2.881076398));
#106302=CARTESIAN_POINT('Ctrl Pts',(6.49695968400001,3.202873885,-3.241315069));
#106303=CARTESIAN_POINT('Ctrl Pts',(6.302972082,3.137747733,-3.582602815));
#106304=CARTESIAN_POINT('',(6.78092773340377,3.26733592582742,-3.20453098004515));
#106305=CARTESIAN_POINT('Origin',(-0.157398646388475,3.0893251739778,0.105671234425524));
#106306=CARTESIAN_POINT('',(6.71694469594588,3.26733592735657,-3.04280370736438));
#106307=CARTESIAN_POINT('Origin',(-2.13804668414141E-13,3.35806379999933,
1.2338220722885E-13));
#106308=CARTESIAN_POINT('',(6.52082249528588,3.35698786822526,-3.70524951664081));
#106309=CARTESIAN_POINT('Origin',(-0.134411997813779,3.08947603517803,0.124581958717571));
#106310=CARTESIAN_POINT('Origin',(-0.152091470713358,3.48205903068806,0.109425263944726));
#106311=CARTESIAN_POINT('Ctrl Pts',(7.236042573,3.13774478,-1.972229166));
#106312=CARTESIAN_POINT('Ctrl Pts',(7.172132141,3.176256335,-2.206714393));
#106313=CARTESIAN_POINT('Ctrl Pts',(7.093174665,3.214285714,-2.436569961));
#106314=CARTESIAN_POINT('Ctrl Pts',(7.038356248,3.240688665,-2.596153559));
#106315=CARTESIAN_POINT('Ctrl Pts',(6.976416247,3.267335925,-2.753110305));
#106316=CARTESIAN_POINT('Ctrl Pts',(6.97490262599906,3.26798710116569,-2.75694583976186));
#106317=CARTESIAN_POINT('Ctrl Pts',(6.97338900499812,3.26863827733136,-2.76078137452372));
#106318=CARTESIAN_POINT('Ctrl Pts',(6.92855444900001,3.13774478,-2.134861413));
#106319=CARTESIAN_POINT('Ctrl Pts',(6.859373891,3.176256335,-2.359382433));
#106320=CARTESIAN_POINT('Ctrl Pts',(6.775802451,3.214285714,-2.578953498));
#106321=CARTESIAN_POINT('Ctrl Pts',(6.717780663,3.240688665,-2.731396796));
#106322=CARTESIAN_POINT('Ctrl Pts',(6.65296165500001,3.267335925,-2.881076398));
#106323=CARTESIAN_POINT('Ctrl Pts',(6.65137768002123,3.26798710116569,-2.88473410199325));
#106324=CARTESIAN_POINT('Ctrl Pts',(6.64979370504246,3.26863827733136,-2.88839180598651));
#106325=CARTESIAN_POINT('',(6.97641624536787,3.26733592550877,-2.75311030322799));
#106326=CARTESIAN_POINT('',(6.81468895436952,3.26733592642396,-2.81709334334895));
#106327=CARTESIAN_POINT('',(7.16550684269047,3.17766594629366,-2.21483897554283));
#106328=CARTESIAN_POINT('Ctrl Pts',(6.97641624723878,3.26733592483409,-2.75311030408086));
#106329=CARTESIAN_POINT('Ctrl Pts',(7.01779331252057,3.24953506265028,-2.64826029694357));
#106330=CARTESIAN_POINT('Ctrl Pts',(7.05672145986858,3.23184317427123,-2.54269001880757));
#106331=CARTESIAN_POINT('Ctrl Pts',(7.09317466455715,3.21428571386188,-2.43656996049252));
#106332=CARTESIAN_POINT('Ctrl Pts',(7.1183905582333,3.20214063482658,-2.36316318632796));
#106333=CARTESIAN_POINT('Ctrl Pts',(7.14251079594586,3.18993125789227,-2.28923640648229));
#106334=CARTESIAN_POINT('Ctrl Pts',(7.16550684258656,3.17766594608544,-2.21483897554504));
#106335=CARTESIAN_POINT('Ctrl Pts',(6.92715057363297,3.13852541810399,-2.13941228615809));
#106336=CARTESIAN_POINT('Ctrl Pts',(6.96682809446975,3.14538568954085,-2.15192905489883));
#106337=CARTESIAN_POINT('Ctrl Pts',(7.00655215970945,3.15207183487632,-2.16448113043638));
#106338=CARTESIAN_POINT('Ctrl Pts',(7.0859908302513,3.1651074164565,-2.18962014877943));
#106339=CARTESIAN_POINT('Ctrl Pts',(7.12575199162475,3.17146448709542,-2.20222182647878));
#106340=CARTESIAN_POINT('Ctrl Pts',(7.16550684231213,3.17766594629071,-2.21483897673639));
#106341=CARTESIAN_POINT('Ctrl Pts',(7.3130761865187,3.26861999521842,-1.6640258809411));
#106342=CARTESIAN_POINT('Ctrl Pts',(7.31217452525935,3.26797796010921,-1.66796884697055));
#106343=CARTESIAN_POINT('Ctrl Pts',(7.311272864,3.267335925,-1.671911813));
#106344=CARTESIAN_POINT('Ctrl Pts',(7.220743665,3.202873885,-2.067796135));
#106345=CARTESIAN_POINT('Ctrl Pts',(7.087997104,3.137747733,-2.45159072));
#106346=CARTESIAN_POINT('Ctrl Pts',(7.11825764338814,3.26861999521842,-1.37585220051464));
#106347=CARTESIAN_POINT('Ctrl Pts',(7.11751150719407,3.26797796010921,-1.37969026875732));
#106348=CARTESIAN_POINT('Ctrl Pts',(7.116765371,3.267335925,-1.383528337));
#106349=CARTESIAN_POINT('Ctrl Pts',(7.041851304,3.202873885,-1.768880641));
#106350=CARTESIAN_POINT('Ctrl Pts',(6.925765802,3.137747733,-2.143890869));
#106351=CARTESIAN_POINT('',(7.311272846636,3.26733592582707,-1.67191180663589));
#106352=CARTESIAN_POINT('Origin',(-0.176434910672402,3.08932519130311,0.0693646279067664));
#106353=CARTESIAN_POINT('',(7.21401911446167,3.26733592735558,-1.52772008934729));
#106354=CARTESIAN_POINT('Origin',(2.17274115366095E-13,3.3580638,2.1467203015213E-14));
#106355=CARTESIAN_POINT('',(7.16488840922633,3.35698786819358,-2.2168387593173));
#106356=CARTESIAN_POINT('Origin',(-0.15805117081004,3.08947605520507,0.0927747698938322));
#106357=CARTESIAN_POINT('Origin',(-0.172058993564836,3.48205904216641,0.0741718257471044));
#106358=CARTESIAN_POINT('Ctrl Pts',(7.490838891,3.13774478,-0.370584287));
#106359=CARTESIAN_POINT('Ctrl Pts',(7.47883004200001,3.176256335,-0.613326232999999));
#106360=CARTESIAN_POINT('Ctrl Pts',(7.4511307,3.214285714,-0.854781429));
#106361=CARTESIAN_POINT('Ctrl Pts',(7.43189966400001,3.240688665,-1.022418391));
#106362=CARTESIAN_POINT('Ctrl Pts',(7.405148846,3.267335925,-1.189020844));
#106363=CARTESIAN_POINT('Ctrl Pts',(7.40449513919885,3.26798710116569,-1.19309208984433));
#106364=CARTESIAN_POINT('Ctrl Pts',(7.40384143239769,3.26863827733136,-1.19716333568867));
#106365=CARTESIAN_POINT('Ctrl Pts',(7.225500794,3.13774478,-0.595515139));
#106366=CARTESIAN_POINT('Ctrl Pts',(7.206203021,3.176256335,-0.829658758));
#106367=CARTESIAN_POINT('Ctrl Pts',(7.171786724,3.214285714,-1.062061763));
#106368=CARTESIAN_POINT('Ctrl Pts',(7.147892255,3.240688665,-1.22341399));
#106369=CARTESIAN_POINT('Ctrl Pts',(7.11676537100001,3.267335925,-1.383528337));
#106370=CARTESIAN_POINT('Ctrl Pts',(7.11600472675467,3.26798710116569,-1.38744103371067));
#106371=CARTESIAN_POINT('Ctrl Pts',(7.11524408250935,3.26863827733136,-1.39135373042133));
#106372=CARTESIAN_POINT('',(7.40514884403296,3.26733592550877,-1.18902084260647));
#106373=CARTESIAN_POINT('',(7.26095711003851,3.26733592642396,-1.28627458181517));
#106374=CARTESIAN_POINT('',(7.4741061843029,3.17766594634252,-0.62268511109573));
#106375=CARTESIAN_POINT('Ctrl Pts',(7.40514884603819,3.26733592483184,-1.18902084303671));
#106376=CARTESIAN_POINT('Ctrl Pts',(7.42301888672541,3.24953506265028,-1.07772732539843));
#106377=CARTESIAN_POINT('Ctrl Pts',(7.4383424264611,3.23184317427152,-0.966256820788148));
#106378=CARTESIAN_POINT('Ctrl Pts',(7.45113069970839,3.21428571391797,-0.854781428739896));
#106379=CARTESIAN_POINT('Ctrl Pts',(7.45997677357733,3.20214063494684,-0.777670192630329));
#106380=CARTESIAN_POINT('Ctrl Pts',(7.46764102080474,3.18993125793742,-0.700286641611116));
#106381=CARTESIAN_POINT('Ctrl Pts',(7.47410618425492,3.17766594614465,-0.622685111123001));
#106382=CARTESIAN_POINT('Ctrl Pts',(7.22510804351791,3.13852541809212,-0.600261407040693));
#106383=CARTESIAN_POINT('Ctrl Pts',(7.26654866655655,3.14538569039346,-0.603956047166329));
#106384=CARTESIAN_POINT('Ctrl Pts',(7.30804233656729,3.15207183664629,-0.607675163076698));
#106385=CARTESIAN_POINT('Ctrl Pts',(7.39102790432093,3.16510741562122,-0.615149477954107));
#106386=CARTESIAN_POINT('Ctrl Pts',(7.43256845399471,3.1714644854126,-0.618909060646346));
#106387=CARTESIAN_POINT('Ctrl Pts',(7.47410618419153,3.17766594633965,-0.622685112325538));
#106388=CARTESIAN_POINT('Ctrl Pts',(7.49981690556088,3.26861999521842,-0.0530266736009007));
#106389=CARTESIAN_POINT('Ctrl Pts',(7.49978394578045,3.26797796010921,-0.0570712858004503));
#106390=CARTESIAN_POINT('Ctrl Pts',(7.49975098600001,3.267335925,-0.061115898));
#106391=CARTESIAN_POINT('Ctrl Pts',(7.496441736,3.202873885,-0.467205767));
#106392=CARTESIAN_POINT('Ctrl Pts',(7.449303207,3.137747733,-0.870564034));
#106393=CARTESIAN_POINT('Ctrl Pts',(7.24760428844329,3.26861999521842,0.186529438107579));
#106394=CARTESIAN_POINT('Ctrl Pts',(7.24770066772165,3.26797796010921,0.182620704553789));
#106395=CARTESIAN_POINT('Ctrl Pts',(7.247797047,3.267335925,0.178711971));
#106396=CARTESIAN_POINT('Ctrl Pts',(7.257473784,3.202873885,-0.213735319));
#106397=CARTESIAN_POINT('Ctrl Pts',(7.22471841,3.137747733,-0.604932968));
#106398=CARTESIAN_POINT('',(7.49975096769167,3.26733592582611,-0.0611158955104157));
#106399=CARTESIAN_POINT('Origin',(-0.187221419669709,3.08932515470111,0.0298146441256785));
#106400=CARTESIAN_POINT('',(7.3737740166168,3.26733592735283,0.0587980218521181));
#106401=CARTESIAN_POINT('Origin',(-3.85108611666851E-13,3.35806379999967,
-2.54651985262533E-14));
#106402=CARTESIAN_POINT('',(7.4739321038036,3.35698786820595,-0.624771086166611));
#106403=CARTESIAN_POINT('Origin',(-0.174300000169229,3.08947598391187,0.0566294523323047));
#106404=CARTESIAN_POINT('Origin',(-0.183981315399253,3.48205904876804,0.0354501451864496));
#106405=CARTESIAN_POINT('Ctrl Pts',(7.39537190800001,3.13774478,1.248388701));
#106406=CARTESIAN_POINT('Ctrl Pts',(7.435826162,3.176256335,1.008740379));
#106407=CARTESIAN_POINT('Ctrl Pts',(7.460680145,3.214285714,0.766975733));
#106408=CARTESIAN_POINT('Ctrl Pts',(7.477935712,3.240688665,0.599123926));
#106409=CARTESIAN_POINT('Ctrl Pts',(7.487624915,3.267335925,0.43066591));
#106410=CARTESIAN_POINT('Ctrl Pts',(7.48786168898945,3.26798710116569,0.42654931996645));
#106411=CARTESIAN_POINT('Ctrl Pts',(7.4880984629789,3.26863827733136,0.4224327299329));
#106412=CARTESIAN_POINT('Ctrl Pts',(7.184590752,3.13774478,0.971676760000001));
#106413=CARTESIAN_POINT('Ctrl Pts',(7.21607810799999,3.176256335,0.738858839));
#106414=CARTESIAN_POINT('Ctrl Pts',(7.23242622,3.214285714,0.5044908));
#106415=CARTESIAN_POINT('Ctrl Pts',(7.243776351,3.240688665,0.341774293));
#106416=CARTESIAN_POINT('Ctrl Pts',(7.247797047,3.267335925,0.178711971));
#106417=CARTESIAN_POINT('Ctrl Pts',(7.24789530030652,3.26798710116569,0.174727234948065));
#106418=CARTESIAN_POINT('Ctrl Pts',(7.24799355361303,3.26863827733136,0.170742498896129));
#106419=CARTESIAN_POINT('',(7.48762491278461,3.26733592550878,0.430665910956628));
#106420=CARTESIAN_POINT('',(7.36771098063556,3.26733592642396,0.304688949312516));
#106421=CARTESIAN_POINT('',(7.43322462765509,3.17766594627913,0.998584817437513));
#106422=CARTESIAN_POINT('Ctrl Pts',(7.48762491482875,3.26733592482897,0.430665910966661));
#106423=CARTESIAN_POINT('Ctrl Pts',(7.48115234803168,3.24953506265028,0.543198978936239));
#106424=CARTESIAN_POINT('Ctrl Pts',(7.47215476859609,3.23184317427177,0.655357473301201));
#106425=CARTESIAN_POINT('Ctrl Pts',(7.46068014479904,3.21428571396803,0.766975732996196));
#106426=CARTESIAN_POINT('Ctrl Pts',(7.45274276608358,3.20214063500042,0.844185795256662));
#106427=CARTESIAN_POINT('Ctrl Pts',(7.443592651207,3.18993125788061,0.921407748626982));
#106428=CARTESIAN_POINT('Ctrl Pts',(7.43322462755758,3.17766594606887,0.998584817391001));
#106429=CARTESIAN_POINT('Ctrl Pts',(7.18522749154915,3.1385254181464,0.966957027476661));
#106430=CARTESIAN_POINT('Ctrl Pts',(7.22649349814379,3.14538569106813,0.972257275447814));
#106431=CARTESIAN_POINT('Ctrl Pts',(7.26781657356803,3.15207183795633,0.977545023491235));
#106432=CARTESIAN_POINT('Ctrl Pts',(7.35046873326897,3.16510741557627,0.988084897019536));
#106433=CARTESIAN_POINT('Ctrl Pts',(7.39184628693084,3.17146448532406,0.993343201591113));
#106434=CARTESIAN_POINT('Ctrl Pts',(7.43322462781404,3.17766594627615,0.998584816186248));
#106435=CARTESIAN_POINT('Ctrl Pts',(7.3358745212548,3.26861999521842,1.56045200257577));
#106436=CARTESIAN_POINT('Ctrl Pts',(7.3367118041274,3.26797796010921,1.55649486578788));
#106437=CARTESIAN_POINT('Ctrl Pts',(7.337549087,3.267335925,1.552537729));
#106438=CARTESIAN_POINT('Ctrl Pts',(7.421614524,3.202873885,1.155230625));
#106439=CARTESIAN_POINT('Ctrl Pts',(7.462288171,3.137747733,0.751169259));
#106440=CARTESIAN_POINT('Ctrl Pts',(7.03806101166501,3.26861999521842,1.74018916767838));
#106441=CARTESIAN_POINT('Ctrl Pts',(7.0389953998325,3.26797796010921,1.73639253683919));
#106442=CARTESIAN_POINT('Ctrl Pts',(7.039929788,3.267335925,1.732595906));
#106443=CARTESIAN_POINT('Ctrl Pts',(7.133744856,3.202873885,1.351404028));
#106444=CARTESIAN_POINT('Ctrl Pts',(7.185851215,3.137747733,0.962310925));
#106445=CARTESIAN_POINT('',(7.33754906858522,3.26733592582611,1.55253772749335));
#106446=CARTESIAN_POINT('Origin',(-0.189253261452819,3.08932519143167,-0.0111294346502501));
#106447=CARTESIAN_POINT('',(7.18873944076293,3.26733592735283,1.64256680321968));
#106448=CARTESIAN_POINT('Origin',(6.80878964320897E-14,3.35806379999933,
7.99057001121817E-14));
#106449=CARTESIAN_POINT('',(7.43350303965737,3.35698786821069,0.996510189375122));
#106450=CARTESIAN_POINT('Origin',(-0.18239831389786,3.08947604963738,0.0178361568675284));
#106451=CARTESIAN_POINT('Origin',(-0.187300472847888,3.48205906456362,-0.0049291658198608));
#106452=CARTESIAN_POINT('Ctrl Pts',(6.954105553,3.13774478,2.808988422));
#106453=CARTESIAN_POINT('Ctrl Pts',(7.045131315,3.176256335,2.583639413));
#106454=CARTESIAN_POINT('Ctrl Pts',(7.121376478,3.214285714,2.352869961));
#106455=CARTESIAN_POINT('Ctrl Pts',(7.174311796,3.240688665,2.192651873));
#106456=CARTESIAN_POINT('Ctrl Pts',(7.219987966,3.267335925,2.030215204));
#106457=CARTESIAN_POINT('Ctrl Pts',(7.22110414954922,3.26798710116569,2.0262457569617));
#106458=CARTESIAN_POINT('Ctrl Pts',(7.22222033309843,3.26863827733136,2.02227630992341));
#106459=CARTESIAN_POINT('Ctrl Pts',(6.807737232,3.13774478,2.493434134));
#106460=CARTESIAN_POINT('Ctrl Pts',(6.888537402,3.176256335,2.272828217));
#106461=CARTESIAN_POINT('Ctrl Pts',(6.954885505,3.214285714,2.047453934));
#106462=CARTESIAN_POINT('Ctrl Pts',(7.000949515,3.240688665,1.890981591));
#106463=CARTESIAN_POINT('Ctrl Pts',(7.039929788,3.267335925,1.732595906));
#106464=CARTESIAN_POINT('Ctrl Pts',(7.0408823446497,3.26798710116569,1.72872545241275));
#106465=CARTESIAN_POINT('Ctrl Pts',(7.04183490129941,3.26863827733136,1.7248549988255));
#106466=CARTESIAN_POINT('',(7.21998796362802,3.26733592550877,2.03021520441968));
#106467=CARTESIAN_POINT('',(7.12995887474965,3.26733592642396,1.88140556352814));
#106468=CARTESIAN_POINT('',(7.04477374845227,3.17766594629653,2.57316202957168));
#106469=CARTESIAN_POINT('Ctrl Pts',(7.2199879656346,3.26733592483455,2.03021520487331));
#106470=CARTESIAN_POINT('Ctrl Pts',(7.18947543979791,3.24953506265028,2.13872590177304));
#106471=CARTESIAN_POINT('Ctrl Pts',(7.15657745751694,3.23184317427162,2.24632797920249));
#106472=CARTESIAN_POINT('Ctrl Pts',(7.12137647774863,3.21428571393803,2.35286996114285));
#106473=CARTESIAN_POINT('Ctrl Pts',(7.09702678946891,3.20214063496177,2.42656859355009));
#106474=CARTESIAN_POINT('Ctrl Pts',(7.07149016196026,3.18993125790088,2.50001813618026));
#106475=CARTESIAN_POINT('Ctrl Pts',(7.04477374840842,3.17766594609248,2.57316202952145));
#106476=CARTESIAN_POINT('Ctrl Pts',(6.80937368739756,3.13852541803299,2.48896162643405));
#106477=CARTESIAN_POINT('Ctrl Pts',(6.84853550984038,3.14538568902674,2.50300892517016));
#106478=CARTESIAN_POINT('Ctrl Pts',(6.88775575239195,3.1520718339132,2.51705628372973));
#106479=CARTESIAN_POINT('Ctrl Pts',(6.96620981330809,3.16510741556216,2.54511752053223));
#106480=CARTESIAN_POINT('Ctrl Pts',(7.00548960277271,3.17146448533082,2.5591478397402));
#106481=CARTESIAN_POINT('Ctrl Pts',(7.04477374887695,3.17766594629358,2.57316202838253));
#106482=CARTESIAN_POINT('Ctrl Pts',(6.82891479781365,3.26861999521842,3.10096567712822));
#106483=CARTESIAN_POINT('Ctrl Pts',(6.83058317290683,3.26797796010921,3.09728104706411));
#106484=CARTESIAN_POINT('Ctrl Pts',(6.832251548,3.267335925,3.093596417));
#106485=CARTESIAN_POINT('Ctrl Pts',(6.999760864,3.202873885,2.723649716));
#106486=CARTESIAN_POINT('Ctrl Pts',(7.126344834,3.137747733,2.337778712));
#106487=CARTESIAN_POINT('Ctrl Pts',(6.49942582582478,3.26861999521842,3.21247958576346));
#106488=CARTESIAN_POINT('Ctrl Pts',(6.5011545319124,3.26797796010921,3.20897258388173));
#106489=CARTESIAN_POINT('Ctrl Pts',(6.502883238,3.267335925,3.205465582));
#106490=CARTESIAN_POINT('Ctrl Pts',(6.676449947,3.202873885,2.853353225));
#106491=CARTESIAN_POINT('Ctrl Pts',(6.810981603,3.137747733,2.48455823));
#106492=CARTESIAN_POINT('',(6.83225153036765,3.26733592582623,3.09359641153269));
#106493=CARTESIAN_POINT('Origin',(-0.182436357475877,3.08932519069727,-0.0515531776573969));
#106494=CARTESIAN_POINT('',(6.66756739925649,3.26733592735283,3.14953098625499));
#106495=CARTESIAN_POINT('Origin',(8.76035355368288E-14,3.35806379999989,
1.7130394325271E-14));
#106496=CARTESIAN_POINT('',(7.04549163559553,3.35698786820739,2.57119575562601));
#106497=CARTESIAN_POINT('Origin',(-0.181968764875183,3.08947600358288,-0.0217912721665592));
#106498=CARTESIAN_POINT('Origin',(-0.181861914083051,3.48205904784782,-0.0450780114584393));
#106499=CARTESIAN_POINT('Ctrl Pts',(6.187672952,3.13774478,4.238242965));
#106500=CARTESIAN_POINT('Ctrl Pts',(6.325013958,3.176256335,4.03773034));
#106501=CARTESIAN_POINT('Ctrl Pts',(6.449085162,3.214285714,3.828746606));
#106502=CARTESIAN_POINT('Ctrl Pts',(6.53522503500001,3.240688665,3.683653856));
#106503=CARTESIAN_POINT('Ctrl Pts',(6.614752403,3.267335925,3.534833892));
#106504=CARTESIAN_POINT('Ctrl Pts',(6.61669580455652,3.26798710116569,3.53119719488613));
#106505=CARTESIAN_POINT('Ctrl Pts',(6.61863920611304,3.26863827733136,3.52756049777226));
#106506=CARTESIAN_POINT('Ctrl Pts',(6.112561485,3.13774478,3.898601299));
#106507=CARTESIAN_POINT('Ctrl Pts',(6.238896343,3.176256335,3.700522674));
#106508=CARTESIAN_POINT('Ctrl Pts',(6.352142073,3.214285714,3.494680397));
#106509=CARTESIAN_POINT('Ctrl Pts',(6.43076606,3.240688665,3.351768692));
#106510=CARTESIAN_POINT('Ctrl Pts',(6.502883238,3.267335925,3.205465582));
#106511=CARTESIAN_POINT('Ctrl Pts',(6.50464555755743,3.26798710116569,3.20189038897088));
#106512=CARTESIAN_POINT('Ctrl Pts',(6.50640787711486,3.26863827733136,3.19831519594175));
#106513=CARTESIAN_POINT('',(6.61475240058954,3.26733592550878,3.53483389192562));
#106514=CARTESIAN_POINT('',(6.55881781646897,3.26733592642396,3.370149744845));
#106515=CARTESIAN_POINT('',(6.32691707896555,3.17766594633841,4.02742104519011));
#106516=CARTESIAN_POINT('Ctrl Pts',(6.61475240244418,3.2673359248308,3.53483389279533));
#106517=CARTESIAN_POINT('Ctrl Pts',(6.56162665075058,3.24953506265028,3.63424837905445));
#106518=CARTESIAN_POINT('Ctrl Pts',(6.50636653917648,3.23184317427181,3.73226268627465));
#106519=CARTESIAN_POINT('Ctrl Pts',(6.44908516185502,3.21428571397487,3.82874660592103));
#106520=CARTESIAN_POINT('Ctrl Pts',(6.40946172851625,3.20214063504681,3.89548774174869));
#106521=CARTESIAN_POINT('Ctrl Pts',(6.36873265250859,3.18993125794093,3.96173045481968));
#106522=CARTESIAN_POINT('Ctrl Pts',(6.32691707897758,3.17766594614415,4.02742104516149));
#106523=CARTESIAN_POINT('Ctrl Pts',(6.11512113831487,3.13852541809098,3.89458514643187));
#106524=CARTESIAN_POINT('Ctrl Pts',(6.15034763687084,3.14538569136909,3.91672266857401));
#106525=CARTESIAN_POINT('Ctrl Pts',(6.18563117853984,3.15207183861718,3.9388728088184));
#106526=CARTESIAN_POINT('Ctrl Pts',(6.25621867002753,3.16510741645027,3.98314328041782));
#106527=CARTESIAN_POINT('Ctrl Pts',(6.2915640212103,3.17146448710136,4.0052895754468));
#106528=CARTESIAN_POINT('Ctrl Pts',(6.3269170796288,3.17766594633554,4.02742104413145));
#106529=CARTESIAN_POINT('Ctrl Pts',(6.00264260807393,3.26861999521841,4.49648164327883));
#106530=CARTESIAN_POINT('Ctrl Pts',(6.00506406403696,3.26797796010921,4.49324180913942));
#106531=CARTESIAN_POINT('Ctrl Pts',(6.00748552,3.267335925,4.490001975));
#106532=CARTESIAN_POINT('Ctrl Pts',(6.250606167,3.202873885,4.164713973));
#106533=CARTESIAN_POINT('Ctrl Pts',(6.457181533,3.137747733,3.815076231));
#106534=CARTESIAN_POINT('Ctrl Pts',(5.65688471072712,3.26861999521841,4.53455802985732));
#106535=CARTESIAN_POINT('Ctrl Pts',(5.65932690236356,3.26797796010921,4.53150464042866));
#106536=CARTESIAN_POINT('Ctrl Pts',(5.66176909400001,3.267335925,4.528451251));
#106537=CARTESIAN_POINT('Ctrl Pts',(5.906971658,3.202873885,4.221882796));
#106538=CARTESIAN_POINT('Ctrl Pts',(6.117638062,3.137747733,3.890630353));
#106539=CARTESIAN_POINT('',(6.00748550389026,3.26733592582694,4.49000196590072));
#106540=CARTESIAN_POINT('Origin',(-0.167088647873811,3.08932514333194,-0.0895662798971653));
#106541=CARTESIAN_POINT('',(5.8346273159664,3.26733592735517,4.50922660139811));
#106542=CARTESIAN_POINT('Origin',(-8.46545056276682E-13,3.35806380000011,
-5.56846235788555E-13));
#106543=CARTESIAN_POINT('',(6.32804087305524,3.35698786821253,4.0256550662547));
#106544=CARTESIAN_POINT('Origin',(-0.173029777855969,3.08947603555603,-0.0603996013206703));
#106545=CARTESIAN_POINT('Origin',(-0.167919645100388,3.48205903152799,-0.0831190532386661));
#106546=CARTESIAN_POINT('Ctrl Pts',(5.131911641,3.13774478,5.469321979));
#106547=CARTESIAN_POINT('Ctrl Pts',(5.30914597800001,3.176256335,5.303021483));
#106548=CARTESIAN_POINT('Ctrl Pts',(5.475241792,3.214285714,5.125595314));
#106549=CARTESIAN_POINT('Ctrl Pts',(5.59055841400001,3.240688665,5.002412278));
#106550=CARTESIAN_POINT('Ctrl Pts',(5.70021837,3.267335925,4.874167676));
#106551=CARTESIAN_POINT('Ctrl Pts',(5.70289811829972,3.26798710116569,4.87103377674732));
#106552=CARTESIAN_POINT('Ctrl Pts',(5.70557786659942,3.26863827733136,4.86789987749465));
#106553=CARTESIAN_POINT('Ctrl Pts',(5.131569157,3.13774478,5.121474201));
#106554=CARTESIAN_POINT('Ctrl Pts',(5.297531425,3.176256335,4.95518480299999));
#106555=CARTESIAN_POINT('Ctrl Pts',(5.452379538,3.214285714,4.77849949));
#106556=CARTESIAN_POINT('Ctrl Pts',(5.559887133,3.240688665,4.655830813));
#106557=CARTESIAN_POINT('Ctrl Pts',(5.661769094,3.267335925,4.52845125000001));
#106558=CARTESIAN_POINT('Ctrl Pts',(5.66425877229023,3.26798710116569,4.52533848961035));
#106559=CARTESIAN_POINT('Ctrl Pts',(5.66674845058047,3.26863827733136,4.5222257292207));
#106560=CARTESIAN_POINT('',(5.7002183676652,3.26733592550878,4.87416767540058));
#106561=CARTESIAN_POINT('',(5.68099372637676,3.26733592642396,4.70130946979503));
#106562=CARTESIAN_POINT('',(5.31322079860285,3.17766594630138,5.2933623289354));
#106563=CARTESIAN_POINT('Ctrl Pts',(5.7002183692918,3.26733592483215,4.87416767665088));
#106564=CARTESIAN_POINT('Ctrl Pts',(5.62696349193861,3.24953506265028,4.95983744082131));
#106565=CARTESIAN_POINT('Ctrl Pts',(5.55192515245494,3.23184317427144,5.04368093738522));
#106566=CARTESIAN_POINT('Ctrl Pts',(5.47524179152958,3.21428571390225,5.12559531379616));
#106567=CARTESIAN_POINT('Ctrl Pts',(5.4221973602718,3.2021406349187,5.18225821197392));
#106568=CARTESIAN_POINT('Ctrl Pts',(5.3681802826392,3.18993125792519,5.23819666005832));
#106569=CARTESIAN_POINT('Ctrl Pts',(5.3132207986748,3.17766594611117,5.29336232896479));
#106570=CARTESIAN_POINT('Ctrl Pts',(5.13493232101444,3.13852541806714,5.11810219227241));
#106571=CARTESIAN_POINT('Ctrl Pts',(5.16457633453219,3.14538569225177,5.1472948114721));
#106572=CARTESIAN_POINT('Ctrl Pts',(5.19427334580649,3.15207184046988,5.17651201696921));
#106573=CARTESIAN_POINT('Ctrl Pts',(5.25369368567045,3.1651074155469,5.23492168157518));
#106574=CARTESIAN_POINT('Ctrl Pts',(5.28345187892572,3.17146448529656,5.26414840986732));
#106575=CARTESIAN_POINT('Ctrl Pts',(5.31322079949224,3.17766594629473,5.29336232799384));
#106576=CARTESIAN_POINT('Ctrl Pts',(4.89569352152841,3.26861999521842,5.68174712431132));
#106577=CARTESIAN_POINT('Ctrl Pts',(4.89875483376421,3.26797796010921,5.67910357715566));
#106578=CARTESIAN_POINT('Ctrl Pts',(4.901816146,3.267335925,5.67646003));
#106579=CARTESIAN_POINT('Ctrl Pts',(5.209180072,3.202873885,5.411040834));
#106580=CARTESIAN_POINT('Ctrl Pts',(5.4860876,3.137747733,5.113985026));
#106581=CARTESIAN_POINT('Ctrl Pts',(4.54983395395533,3.26861999521842,5.64460557872374));
#106582=CARTESIAN_POINT('Ctrl Pts',(4.55287543697766,3.26797796010921,5.64214857486187));
#106583=CARTESIAN_POINT('Ctrl Pts',(4.55591692,3.267335925,5.639691571));
#106584=CARTESIAN_POINT('Ctrl Pts',(4.86128994,3.202873885,5.39300182));
#106585=CARTESIAN_POINT('Ctrl Pts',(5.138240564,3.137747733,5.114780924));
#106586=CARTESIAN_POINT('',(4.90181613226231,3.26733592582611,5.67646001765269));
#106587=CARTESIAN_POINT('Origin',(-0.143928092233303,3.08932515400138,-0.123391387392208));
#106588=CARTESIAN_POINT('',(4.72886654423971,3.26733592735283,5.65807579110616));
#106589=CARTESIAN_POINT('Origin',(2.1987620058006E-13,3.35806380000022,
2.23345647532014E-13));
#106590=CARTESIAN_POINT('',(5.31469795204853,3.35698786817063,5.29187921992739));
#106591=CARTESIAN_POINT('Origin',(-0.156000037174683,3.0894760332274,-0.0961835375372055));
#106592=CARTESIAN_POINT('Origin',(-0.146125483290186,3.48205904005493,-0.117273373961345));
#106593=CARTESIAN_POINT('Ctrl Pts',(3.836187846,3.13774478,6.444661575));
#106594=CARTESIAN_POINT('Ctrl Pts',(4.045028233,3.176256335,6.320349236));
#106595=CARTESIAN_POINT('Ctrl Pts',(4.2453822,3.214285714,6.182776882));
#106596=CARTESIAN_POINT('Ctrl Pts',(4.384483496,3.240688665,6.087263462));
#106597=CARTESIAN_POINT('Ctrl Pts',(4.519148461,3.267335925,5.985590797));
#106598=CARTESIAN_POINT('Ctrl Pts',(4.52243925395809,3.26798710116569,5.98310623325313));
#106599=CARTESIAN_POINT('Ctrl Pts',(4.52573004691619,3.26863827733136,5.98062166950626));
#106600=CARTESIAN_POINT('Ctrl Pts',(3.910630358,3.13774478,6.104872661));
#106601=CARTESIAN_POINT('Ctrl Pts',(4.108459826,3.176256335,5.978147999));
#106602=CARTESIAN_POINT('Ctrl Pts',(4.297669796,3.214285714,5.838881257));
#106603=CARTESIAN_POINT('Ctrl Pts',(4.429034062,3.240688665,5.74219146));
#106604=CARTESIAN_POINT('Ctrl Pts',(4.55591692,3.267335925,5.639691571));
#106605=CARTESIAN_POINT('Ctrl Pts',(4.55901754246412,3.26798710116569,5.6371867924711));
#106606=CARTESIAN_POINT('Ctrl Pts',(4.56211816492825,3.26863827733136,5.63468201394221));
#106607=CARTESIAN_POINT('',(4.5191484588534,3.26733592550877,5.9855907959051));
#106608=CARTESIAN_POINT('',(4.5375326835475,3.26733592642396,5.81264118942734));
#106609=CARTESIAN_POINT('',(4.05108421901788,3.17766594629334,6.31179187331946));
#106610=CARTESIAN_POINT('Ctrl Pts',(4.51914846017482,3.26733592483341,5.9855907974783));
#106611=CARTESIAN_POINT('Ctrl Pts',(4.42918977470013,3.24953506265028,6.05351001663708));
#106612=CARTESIAN_POINT('Ctrl Pts',(4.33788191641198,3.23184317427191,6.11926227378783));
#106613=CARTESIAN_POINT('Ctrl Pts',(4.24538220000967,3.2142857139959,6.18277688180928));
#106614=CARTESIAN_POINT('Ctrl Pts',(4.18139707048148,3.20214063507977,6.22671204840464));
#106615=CARTESIAN_POINT('Ctrl Pts',(4.11661776882006,3.18993125792659,6.26973061157319));
#106616=CARTESIAN_POINT('Ctrl Pts',(4.05108421910799,3.17766594610806,6.31179187340583));
#106617=CARTESIAN_POINT('Ctrl Pts',(3.91463977526643,3.13852541808699,6.10230246946549));
#106618=CARTESIAN_POINT('Ctrl Pts',(3.93731515698753,3.14538568580912,6.13718513501166));
#106619=CARTESIAN_POINT('Ctrl Pts',(3.96003700862289,3.15207182728962,6.17210320009783));
#106620=CARTESIAN_POINT('Ctrl Pts',(4.00551183172567,3.16510741638777,6.24192097074481));
#106621=CARTESIAN_POINT('Ctrl Pts',(4.02829141568943,3.17146448702112,6.2768615314487));
#106622=CARTESIAN_POINT('Ctrl Pts',(4.05108422008695,3.17766594628283,6.31179187256125));
#106623=CARTESIAN_POINT('Ctrl Pts',(3.55982724710696,3.26861999521842,6.60134042570219));
#106624=CARTESIAN_POINT('Ctrl Pts',(3.56338527205348,3.26797796010921,6.5994167748511));
#106625=CARTESIAN_POINT('Ctrl Pts',(3.566943297,3.267335925,6.597493124));
#106626=CARTESIAN_POINT('Ctrl Pts',(3.924178506,3.202873885,6.40435344));
#106627=CARTESIAN_POINT('Ctrl Pts',(4.258470309,3.137747733,6.173769564));
#106628=CARTESIAN_POINT('Ctrl Pts',(3.2300380178948,3.26861999521842,6.49071764506209));
#106629=CARTESIAN_POINT('Ctrl Pts',(3.2335365759474,3.26797796010921,6.48897191353104));
#106630=CARTESIAN_POINT('Ctrl Pts',(3.237035134,3.267335925,6.487226182));
#106631=CARTESIAN_POINT('Ctrl Pts',(3.588299708,3.202873885,6.311950073));
#106632=CARTESIAN_POINT('Ctrl Pts',(3.918584648,3.137747733,6.099770025));
#106633=CARTESIAN_POINT('',(3.56694328621157,3.26733592582706,6.59749310897334));
#106634=CARTESIAN_POINT('Origin',(-0.114037627145149,3.08932521420518,-0.151446856230543));
#106635=CARTESIAN_POINT('',(3.40198922851141,3.26733592735556,6.54235964623415));
#106636=CARTESIAN_POINT('Origin',(-6.21464685268691E-13,3.35806379999967,
-9.96598636948676E-13));
#106637=CARTESIAN_POINT('',(4.05284566209122,3.35698786818625,6.31066098278468));
#106638=CARTESIAN_POINT('Origin',(-0.131676465737328,3.08947593480512,-0.127470530566424));
#106639=CARTESIAN_POINT('Origin',(-0.117498977325006,3.48205908444918,-0.145944454804838));
#106640=CARTESIAN_POINT('Ctrl Pts',(2.36108817,3.13774478,7.118655958));
#106641=CARTESIAN_POINT('Ctrl Pts',(2.591769463,3.176256335,7.042144483));
#106642=CARTESIAN_POINT('Ctrl Pts',(2.817013256,3.214285714,6.950858675));
#106643=CARTESIAN_POINT('Ctrl Pts',(2.973395002,3.240688665,6.887480972));
#106644=CARTESIAN_POINT('Ctrl Pts',(3.126768193,3.267335925,6.817134344));
#106645=CARTESIAN_POINT('Ctrl Pts',(3.13051615682195,3.26798710116569,6.81541529117844));
#106646=CARTESIAN_POINT('Ctrl Pts',(3.13426412064389,3.26863827733136,6.81369623835689));
#106647=CARTESIAN_POINT('Ctrl Pts',(2.50683483,3.13774478,6.80281406));
#106648=CARTESIAN_POINT('Ctrl Pts',(2.727281211,3.176256335,6.721579638));
#106649=CARTESIAN_POINT('Ctrl Pts',(2.94200579,3.214285714,6.626243425));
#106650=CARTESIAN_POINT('Ctrl Pts',(3.09108428,3.240688665,6.560053617));
#106651=CARTESIAN_POINT('Ctrl Pts',(3.237035134,3.267335925,6.487226182));
#106652=CARTESIAN_POINT('Ctrl Pts',(3.24060171898795,3.26798710116569,6.48544650597028));
#106653=CARTESIAN_POINT('Ctrl Pts',(3.24416830397589,3.26863827733136,6.48366682994055));
#106654=CARTESIAN_POINT('',(3.12676819112568,3.26733592550878,6.81713434248249));
#106655=CARTESIAN_POINT('',(3.18190165554333,3.26733592642396,6.65218026680587));
#106656=CARTESIAN_POINT('',(2.59952344355989,3.17766594625804,7.03508904441724));
#106657=CARTESIAN_POINT('Ctrl Pts',(3.12676819207577,3.26733592483072,6.81713434429708));
#106658=CARTESIAN_POINT('Ctrl Pts',(3.02431206592027,3.24953506265028,6.86412719177397));
#106659=CARTESIAN_POINT('Ctrl Pts',(2.92100414310148,3.23184317427142,6.90871370745156));
#106660=CARTESIAN_POINT('Ctrl Pts',(2.81701325564168,3.21428571389909,6.95085867462062));
#106661=CARTESIAN_POINT('Ctrl Pts',(2.74507930028266,3.20214063492807,6.98001174970034));
#106662=CARTESIAN_POINT('Ctrl Pts',(2.67256678374785,3.18993125793566,7.0080989278413));
#106663=CARTESIAN_POINT('Ctrl Pts',(2.59952344370808,3.17766594609591,7.03508904474461));
#106664=CARTESIAN_POINT('Ctrl Pts',(2.51130302491627,3.13852541819266,6.8011658645337));
#106665=CARTESIAN_POINT('Ctrl Pts',(2.5259495383277,3.1453856913761,6.84010756067898));
#106666=CARTESIAN_POINT('Ctrl Pts',(2.54063382725774,3.15207183853582,6.87909382298944));
#106667=CARTESIAN_POINT('Ctrl Pts',(2.57003669000114,3.16510741550788,6.95705496333845));
#106668=CARTESIAN_POINT('Ctrl Pts',(2.58477250992851,3.17146448518842,6.99607556414552));
#106669=CARTESIAN_POINT('Ctrl Pts',(2.59952344479365,3.17766594623031,7.03508904377181));
#106670=CARTESIAN_POINT('Ctrl Pts',(2.05750740624301,3.26861999521841,7.21226238556067));
#106671=CARTESIAN_POINT('Ctrl Pts',(2.06139577462151,3.26797796010921,7.21114857878034));
#106672=CARTESIAN_POINT('Ctrl Pts',(2.065284143,3.267335925,7.21003477200001));
#106673=CARTESIAN_POINT('Ctrl Pts',(2.455686715,3.202873885,7.098205596));
#106674=CARTESIAN_POINT('Ctrl Pts',(2.831731678,3.137747733,6.944875499));
#106675=CARTESIAN_POINT('Ctrl Pts',(1.7592090952449,3.26861999521841,7.03333096846917));
#106676=CARTESIAN_POINT('Ctrl Pts',(1.76300113962245,3.26797796010921,7.03237813773459));
#106677=CARTESIAN_POINT('Ctrl Pts',(1.766793184,3.267335925,7.031425307));
#106678=CARTESIAN_POINT('Ctrl Pts',(2.147524569,3.202873885,6.935758556));
#106679=CARTESIAN_POINT('Ctrl Pts',(2.51570007,3.137747733,6.799540658));
#106680=CARTESIAN_POINT('',(2.0652841356999,3.26733592582647,7.21003475501715));
#106681=CARTESIAN_POINT('Origin',(-0.0788149208579259,3.08932516908768,
-0.172420872875289));
#106682=CARTESIAN_POINT('',(1.91603867765137,3.26733592735385,7.12073003569217));
#106683=CARTESIAN_POINT('Origin',(2.68665298341908E-13,3.35806380000067,
6.44449771325384E-13));
#106684=CARTESIAN_POINT('',(2.6014868129463,3.35698786818497,7.03436325179611));
#106685=CARTESIAN_POINT('Origin',(-0.101195453104435,3.08947598274281,-0.1527966907843));
#106686=CARTESIAN_POINT('Origin',(-0.0833780850768881,3.48205905312549,
-0.167790905124618));
#106687=CARTESIAN_POINT('Ctrl Pts',(0.775586635,3.13774478,7.459789901));
#106688=CARTESIAN_POINT('Ctrl Pts',(1.017322434,3.176256335,7.43465688100001));
#106689=CARTESIAN_POINT('Ctrl Pts',(1.256923902,3.214285714,7.393926041));
#106690=CARTESIAN_POINT('Ctrl Pts',(1.423273863,3.240688665,7.365647527));
#106691=CARTESIAN_POINT('Ctrl Pts',(1.588183719,3.267335925,7.329916267));
#106692=CARTESIAN_POINT('Ctrl Pts',(1.59221360303736,3.26798710116569,7.3290431061241));
#106693=CARTESIAN_POINT('Ctrl Pts',(1.59624348707472,3.26863827733136,7.32816994524821));
#106694=CARTESIAN_POINT('Ctrl Pts',(0.985822492000001,3.13774478,7.182663435));
#106695=CARTESIAN_POINT('Ctrl Pts',(1.218577958,3.176256335,7.15071768400001));
#106696=CARTESIAN_POINT('Ctrl Pts',(1.448776863,3.214285714,7.103769816));
#106697=CARTESIAN_POINT('Ctrl Pts',(1.608598834,3.240688665,7.071174957));
#106698=CARTESIAN_POINT('Ctrl Pts',(1.766793184,3.267335925,7.031425307));
#106699=CARTESIAN_POINT('Ctrl Pts',(1.77065896195487,3.26798710116569,7.03045394916905));
#106700=CARTESIAN_POINT('Ctrl Pts',(1.77452473990974,3.26863827733136,7.02948259133811));
#106701=CARTESIAN_POINT('',(1.58818371752725,3.26733592550877,7.32991626509525));
#106702=CARTESIAN_POINT('',(1.6774884429112,3.26733592642396,7.18067078900645));
#106703=CARTESIAN_POINT('',(1.02641184128338,3.17766594629658,7.42943327122658));
#106704=CARTESIAN_POINT('Ctrl Pts',(1.58818371806689,3.26733592483612,7.32991626708421));
#106705=CARTESIAN_POINT('Ctrl Pts',(1.4780208864729,3.24953506265028,7.35378540900346));
#106706=CARTESIAN_POINT('Ctrl Pts',(1.3675434625844,3.23184317427187,7.3751213666415));
#106707=CARTESIAN_POINT('Ctrl Pts',(1.25692390201705,3.21428571398719,7.39392604086586));
#106708=CARTESIAN_POINT('Ctrl Pts',(1.18040467351101,3.20214063506812,7.40693385968585));
#106709=CARTESIAN_POINT('Ctrl Pts',(1.10354954581301,3.1899312579316,7.41877632737252));
#106710=CARTESIAN_POINT('Ctrl Pts',(1.02641184133089,3.17766594611356,7.42943327135974));
#106711=CARTESIAN_POINT('Ctrl Pts',(0.990540536095495,3.13852541801635,
7.18201430225601));
#106712=CARTESIAN_POINT('Ctrl Pts',(0.996473310127783,3.14538569321089,
7.2231941425004));
#106713=CARTESIAN_POINT('Ctrl Pts',(1.00243339650977,3.15207184247826,7.2644256295697));
#106714=CARTESIAN_POINT('Ctrl Pts',(1.01438949230819,3.16510741552789,7.34688480317291));
#106715=CARTESIAN_POINT('Ctrl Pts',(1.02039252128369,3.17146448527065,7.38816089009443));
#106716=CARTESIAN_POINT('Ctrl Pts',(1.0264118425723,3.17766594628502,7.42943327098007));
#106717=CARTESIAN_POINT('Ctrl Pts',(0.458980806959232,3.26861999521842,
7.48594697166454));
#106718=CARTESIAN_POINT('Ctrl Pts',(0.463017702979616,3.26797796010921,
7.48569508933226));
#106719=CARTESIAN_POINT('Ctrl Pts',(0.467054599,3.267335925,7.485443207));
#106720=CARTESIAN_POINT('Ctrl Pts',(0.872369743,3.202873885,7.460153548));
#106721=CARTESIAN_POINT('Ctrl Pts',(1.272584422,3.137747733,7.391246775));
#106722=CARTESIAN_POINT('Ctrl Pts',(0.206121509127987,3.26861999521842,
7.24707355226296));
#106723=CARTESIAN_POINT('Ctrl Pts',(0.210029728063993,3.26797796010921,
7.24695817563147));
#106724=CARTESIAN_POINT('Ctrl Pts',(0.213937947,3.267335925,7.246842799));
#106725=CARTESIAN_POINT('Ctrl Pts',(0.606333568,3.202873885,7.235258677));
#106726=CARTESIAN_POINT('Ctrl Pts',(0.995184151,3.137747733,7.181372327));
#106727=CARTESIAN_POINT('',(0.467054595523074,3.26733592582729,7.48544318882912));
#106728=CARTESIAN_POINT('Origin',(-0.0399068760955543,3.0893251625822,-0.185332644120294));
#106729=CARTESIAN_POINT('',(0.340496287653564,3.26733592735618,7.36614300232264));
#106730=CARTESIAN_POINT('Origin',(1.97107954957865E-13,3.35806379999933,
7.19476561661381E-13));
#106731=CARTESIAN_POINT('',(1.02848533195528,3.356987868206,7.42914651327288));
#106732=CARTESIAN_POINT('Origin',(-0.0659827140366118,3.08947603214728,
-0.170978110658462));
#106733=CARTESIAN_POINT('Origin',(-0.0453586688464361,3.48205903721848,
-0.181791902684507));
#106734=CARTESIAN_POINT('Origin',(-1.17935785378005E-13,3.35806379999978,
1.91860416443035E-12));
#106735=CARTESIAN_POINT('',(-0.0246624610395199,3.26733592550877,7.49995944882694));
#106736=CARTESIAN_POINT('Ctrl Pts',(-0.0246624565254798,3.26733592553159,
7.49995945089605));
#106737=CARTESIAN_POINT('Ctrl Pts',(-0.137380907419657,3.24953506265028,
7.49958879335285));
#106738=CARTESIAN_POINT('Ctrl Pts',(-0.249862030784193,3.23184317427147,
7.49667654792688));
#106739=CARTESIAN_POINT('Ctrl Pts',(-0.361937816335415,3.21428571390813,
7.49126164372827));
#106740=CARTESIAN_POINT('Ctrl Pts',(-0.439464363273653,3.20214063517061,
7.48751597453169));
#106741=CARTESIAN_POINT('Ctrl Pts',(-0.517068439202277,3.18993125839334,
7.48255999142523));
#106742=CARTESIAN_POINT('Ctrl Pts',(-0.594693633718237,3.17766594678636,
7.47638545586979));
#106743=CARTESIAN_POINT('',(-0.592606979416598,3.3569878682049,7.47655114140618));
#106744=CARTESIAN_POINT('Origin',(-0.027684826236559,3.08947596084301,-0.181165925910972));
#106745=CARTESIAN_POINT('Origin',(-0.00521827043682879,3.48205907355581,
-0.187292892979214));
#106746=CARTESIAN_POINT('Ctrl Pts',(-0.846180468000001,3.13774478,7.452112359));
#106747=CARTESIAN_POINT('Ctrl Pts',(-0.604693462,3.176256335,7.479532986));
#106748=CARTESIAN_POINT('Ctrl Pts',(-0.361937816,3.214285714,7.491261644));
#106749=CARTESIAN_POINT('Ctrl Pts',(-0.193397981,3.240688665,7.49940459));
#106750=CARTESIAN_POINT('Ctrl Pts',(-0.02466246,3.267335925,7.499959451));
#106751=CARTESIAN_POINT('Ctrl Pts',(-0.0205390886072463,3.26798710116569,
7.49997301007732));
#106752=CARTESIAN_POINT('Ctrl Pts',(-0.0164157172144926,3.26863827733136,
7.49998656915463));
#106753=CARTESIAN_POINT('Ctrl Pts',(-0.58128581,3.13774478,7.22665945000001));
#106754=CARTESIAN_POINT('Ctrl Pts',(-0.347104645,3.176256335,7.245496119));
#106755=CARTESIAN_POINT('Ctrl Pts',(-0.112195259,3.214285714,7.249131826));
#106756=CARTESIAN_POINT('Ctrl Pts',(0.050897094,3.240688665,7.251656016));
#106757=CARTESIAN_POINT('Ctrl Pts',(0.213937947,3.267335925,7.246842799));
#106758=CARTESIAN_POINT('Ctrl Pts',(0.21792215841634,3.26798710116569,7.24672517894485));
#106759=CARTESIAN_POINT('Ctrl Pts',(0.221906369832681,3.26863827733136,
7.24660755888971));
#106760=CARTESIAN_POINT('',(0.0946377346806782,3.26733592642396,7.3734011251132));
#106761=CARTESIAN_POINT('Ctrl Pts',(-0.037736949,2.490655005,7.49990506100001));
#106762=CARTESIAN_POINT('Ctrl Pts',(0.372864527,2.556411293,7.501971067));
#106763=CARTESIAN_POINT('Ctrl Pts',(0.781237513,2.621296797,7.459200222));
#106764=CARTESIAN_POINT('Ctrl Pts',(0.201304349,2.490655005,7.247204741));
#106765=CARTESIAN_POINT('Ctrl Pts',(0.598071101,2.556411293,7.23618382));
#106766=CARTESIAN_POINT('Ctrl Pts',(0.991263374999999,2.621296797,7.181914572));
#106767=CARTESIAN_POINT('',(0.206045683893195,2.49144077928712,7.2470715026123));
#106768=CARTESIAN_POINT('Origin',(0.0078834845902781,2.41076923579639,-0.195169088968804));
#106769=CARTESIAN_POINT('Ctrl Pts',(0.206045688489983,2.49144078088258,
7.24707150221496));
#106770=CARTESIAN_POINT('Ctrl Pts',(0.207247253803597,2.49833629958132,
7.28865974208964));
#106771=CARTESIAN_POINT('Ctrl Pts',(0.208471474059975,2.50506214895585,
7.33030086491627));
#106772=CARTESIAN_POINT('Ctrl Pts',(0.210958287707542,2.51818504852657,
7.41358339843687));
#106773=CARTESIAN_POINT('Ctrl Pts',(0.212222310116712,2.52458961896209,
7.45527257747634));
#106774=CARTESIAN_POINT('Ctrl Pts',(0.213503815207118,2.53084202106317,
7.49696045865912));
#106775=CARTESIAN_POINT('Ctrl Pts',(1.24150092168421,2.62578637474627,7.39711075669431));
#106776=CARTESIAN_POINT('Ctrl Pts',(1.25530842931597,2.62354158587314,7.39474029520798));
#106777=CARTESIAN_POINT('Ctrl Pts',(1.26911593694773,2.621296797,7.39236983372176));
#106778=CARTESIAN_POINT('Ctrl Pts',(1.67083202238252,2.555986835,7.32340354854394));
#106779=CARTESIAN_POINT('Ctrl Pts',(2.06270905602151,2.49066265,7.21131183416782));
#106780=CARTESIAN_POINT('Ctrl Pts',(0.9644345386314,2.62578637474628,7.18561754598309));
#106781=CARTESIAN_POINT('Ctrl Pts',(0.977848956815707,2.62354158587314,
7.18376605899156));
#106782=CARTESIAN_POINT('Ctrl Pts',(0.991263375,2.621296797,7.181914572));
#106783=CARTESIAN_POINT('Ctrl Pts',(1.381542903,2.555986835,7.128047348));
#106784=CARTESIAN_POINT('Ctrl Pts',(1.763686919,2.49066265,7.032205092));
#106785=CARTESIAN_POINT('Ctrl Pts',(0.961669527889655,2.62578637474628,
7.18350692905078));
#106786=CARTESIAN_POINT('Ctrl Pts',(0.97508002319983,2.62354158587314,7.18166062121545));
#106787=CARTESIAN_POINT('Ctrl Pts',(0.988490518509999,2.621296797,7.17981431338));
#106788=CARTESIAN_POINT('Ctrl Pts',(1.37865591428,2.555986835,7.12609777192));
#106789=CARTESIAN_POINT('Ctrl Pts',(1.76070279869,2.49066265,7.03041767896));
#106790=CARTESIAN_POINT('',(1.75913460167848,2.49144077991026,7.03334526603423));
#106791=CARTESIAN_POINT('Origin',(-0.038363327590185,2.5535712699457,-0.19584155044322));
#106792=CARTESIAN_POINT('Ctrl Pts',(1.82013710423508,2.53084202099787,7.2757886802893));
#106793=CARTESIAN_POINT('Ctrl Pts',(1.80992389783541,2.52458961887095,7.23535092406327));
#106794=CARTESIAN_POINT('Ctrl Pts',(1.79972748647046,2.51818504845322,7.1949081423779));
#106795=CARTESIAN_POINT('Ctrl Pts',(1.77939553036727,2.50506214886567,7.11410729951541));
#106796=CARTESIAN_POINT('Ctrl Pts',(1.76924832116017,2.49833629940387,7.07370289367457));
#106797=CARTESIAN_POINT('Ctrl Pts',(1.75913460568594,2.49144078071445,7.03334526489254));
#106798=CARTESIAN_POINT('Ctrl Pts',(1.575403212,2.490655005,7.332673777));
#106799=CARTESIAN_POINT('Ctrl Pts',(1.976849185,2.556411293,7.2464243));
#106800=CARTESIAN_POINT('Ctrl Pts',(2.36648017,2.621296797,7.11686529400001));
#106801=CARTESIAN_POINT('Ctrl Pts',(1.754532759,2.490655005,7.034494637));
#106802=CARTESIAN_POINT('Ctrl Pts',(2.139654152,2.556411293,6.93843825600001));
#106803=CARTESIAN_POINT('Ctrl Pts',(2.511987525,2.621296797,6.800913077));
#106804=CARTESIAN_POINT('Origin',(-0.0342563549590419,2.41076920033269,
-0.192300740412121));
#106805=CARTESIAN_POINT('Ctrl Pts',(2.80263547683302,2.62578637456442,6.95728441748718));
#106806=CARTESIAN_POINT('Ctrl Pts',(2.81561059294644,2.62354158578221,6.95200117027106));
#106807=CARTESIAN_POINT('Ctrl Pts',(2.82858570905987,2.621296797,6.94671792305479));
#106808=CARTESIAN_POINT('Ctrl Pts',(3.20608418331737,2.555986835,6.79300694691972));
#106809=CARTESIAN_POINT('Ctrl Pts',(3.56470294445959,2.49066265,6.59929389665742));
#106810=CARTESIAN_POINT('Ctrl Pts',(2.48658196293848,2.62578637456442,6.81029688395013));
#106811=CARTESIAN_POINT('Ctrl Pts',(2.49928474396925,2.62354158578221,6.80560498047508));
#106812=CARTESIAN_POINT('Ctrl Pts',(2.511987525,2.621296797,6.800913077));
#106813=CARTESIAN_POINT('Ctrl Pts',(2.881562673,2.555986835,6.664406676));
#106814=CARTESIAN_POINT('Ctrl Pts',(3.234169123,2.49066265,6.488655491));
#106815=CARTESIAN_POINT('Ctrl Pts',(2.48342787635703,2.62578637456442,6.80883000765624));
#106816=CARTESIAN_POINT('Ctrl Pts',(2.49612793959352,2.62354158578221,6.80414400555304));
#106817=CARTESIAN_POINT('Ctrl Pts',(2.50882800283,2.621296797,6.79945800345));
#106818=CARTESIAN_POINT('Ctrl Pts',(2.87832407923,2.555986835,6.66312329717));
#106819=CARTESIAN_POINT('Ctrl Pts',(3.23087052879,2.49066265,6.48755136434));
#106820=CARTESIAN_POINT('',(3.22996834025018,2.49144077989572,6.49074762261724));
#106821=CARTESIAN_POINT('Origin',(-0.079566625270621,2.55357127829657,-0.183016063847826));
#106822=CARTESIAN_POINT('Ctrl Pts',(3.34166280629982,2.53084202104486,6.71440910928901));
#106823=CARTESIAN_POINT('Ctrl Pts',(3.32299542484375,2.5245896082431,6.6771122392648));
#106824=CARTESIAN_POINT('Ctrl Pts',(3.30434341444964,2.51818504331344,6.63980694869523));
#106825=CARTESIAN_POINT('Ctrl Pts',(3.26711702995851,2.50506214888135,6.56526598359231));
#106826=CARTESIAN_POINT('Ctrl Pts',(3.24852130392302,2.49833629942832,6.52798756039885));
#106827=CARTESIAN_POINT('Ctrl Pts',(3.22996834425851,2.49144078075648,6.4907476204609));
#106828=CARTESIAN_POINT('Ctrl Pts',(3.114879271,2.490655005,6.822574817));
#106829=CARTESIAN_POINT('Ctrl Pts',(3.488398571,2.556411293,6.652042788));
#106830=CARTESIAN_POINT('Ctrl Pts',(3.841068843,2.621296797,6.441753654));
#106831=CARTESIAN_POINT('Ctrl Pts',(3.225721167,2.490655005,6.492859382));
#106832=CARTESIAN_POINT('Ctrl Pts',(3.581189353,2.556411293,6.31625903));
#106833=CARTESIAN_POINT('Ctrl Pts',(3.91525393,2.621296797,6.101908444));
#106834=CARTESIAN_POINT('Origin',(-0.0747944090379393,2.41076919092955,
-0.180440693997387));
#106835=CARTESIAN_POINT('Ctrl Pts',(4.23272190964437,2.62578637467355,6.19214319192852));
#106836=CARTESIAN_POINT('Ctrl Pts',(4.24425793307671,2.62354158583678,6.18419419749439));
#106837=CARTESIAN_POINT('Ctrl Pts',(4.25579395650908,2.621296797,6.17624520306028));
#106838=CARTESIAN_POINT('Ctrl Pts',(4.59142341067218,2.555986835,5.94497689134849));
#106839=CARTESIAN_POINT('Ctrl Pts',(4.9000152847214,2.49066265,5.6787003118293));
#106840=CARTESIAN_POINT('Ctrl Pts',(3.89245957637013,2.62578637467355,6.11653430794237));
#106841=CARTESIAN_POINT('Ctrl Pts',(3.9038567531851,2.62354158583678,6.10922137597126));
#106842=CARTESIAN_POINT('Ctrl Pts',(3.91525393,2.621296797,6.101908444));
#106843=CARTESIAN_POINT('Ctrl Pts',(4.246843776,2.555986835,5.889145755));
#106844=CARTESIAN_POINT('Ctrl Pts',(4.553425174,2.49066265,5.641703571));
#106845=CARTESIAN_POINT('Ctrl Pts',(3.88906389553661,2.62578637467355,6.11577976177873));
#106846=CARTESIAN_POINT('Ctrl Pts',(3.90045968671834,2.62354158583678,6.10847317745445));
#106847=CARTESIAN_POINT('Ctrl Pts',(3.9118554779,2.621296797,6.10116659312999));
#106848=CARTESIAN_POINT('Ctrl Pts',(4.24340501024,2.555986835,5.88858858277999));
#106849=CARTESIAN_POINT('Ctrl Pts',(4.5499663445,2.49066265,5.64133435845));
#106850=CARTESIAN_POINT('',(4.54977234856427,2.49144077987894,5.64464983369171));
#106851=CARTESIAN_POINT('Origin',(-0.117049403437909,2.55357126053773,-0.161632706015022));
#106852=CARTESIAN_POINT('Ctrl Pts',(4.70693606860209,2.53084202106238,5.83907123131914));
#106853=CARTESIAN_POINT('Ctrl Pts',(4.68068744031113,2.52458961891124,5.80665933175817));
#106854=CARTESIAN_POINT('Ctrl Pts',(4.65445194454156,2.51818504844758,5.77423581901437));
#106855=CARTESIAN_POINT('Ctrl Pts',(4.60207176775531,2.50506214889181,5.70944012703404));
#106856=CARTESIAN_POINT('Ctrl Pts',(4.5758970400296,2.49833629932961,5.6770307834315));
#106857=CARTESIAN_POINT('Ctrl Pts',(4.54977235220718,2.49144078070503,5.64464983057672));
#106858=CARTESIAN_POINT('Ctrl Pts',(4.508707036,2.490655005,5.99345984100001));
#106859=CARTESIAN_POINT('Ctrl Pts',(4.83683431699999,2.556411293,5.746619148));
#106860=CARTESIAN_POINT('Ctrl Pts',(5.136053407,2.621296797,5.465432773));
#106861=CARTESIAN_POINT('Ctrl Pts',(4.546078438,2.490655005,5.647625239));
#106862=CARTESIAN_POINT('Ctrl Pts',(4.85527212,2.556411293,5.398738552));
#106863=CARTESIAN_POINT('Ctrl Pts',(5.135447414,2.621296797,5.117585355));
#106864=CARTESIAN_POINT('Origin',(-0.111835230384976,2.41076916224554,-0.160143598903905));
#106865=CARTESIAN_POINT('Ctrl Pts',(5.46489097127033,2.6257863747464,5.13746423310914));
#106866=CARTESIAN_POINT('Ctrl Pts',(5.47444849018765,2.6235415858732,5.1272211775746));
#106867=CARTESIAN_POINT('Ctrl Pts',(5.48400600910498,2.621296797,5.11697812203994));
#106868=CARTESIAN_POINT('Ctrl Pts',(5.7620727817793,2.555986835,4.81896632426268));
#106869=CARTESIAN_POINT('Ctrl Pts',(6.00620835592956,2.49066265,4.49257701135858));
#106870=CARTESIAN_POINT('Ctrl Pts',(5.1163301078429,2.6257863747464,5.1367693869352));
#106871=CARTESIAN_POINT('Ctrl Pts',(5.12588876092139,2.6235415858732,5.12717737096759));
#106872=CARTESIAN_POINT('Ctrl Pts',(5.135447414,2.621296797,5.117585355));
#106873=CARTESIAN_POINT('Ctrl Pts',(5.413547184,2.555986835,4.838514924));
#106874=CARTESIAN_POINT('Ctrl Pts',(5.659768124,2.49066265,4.530951863));
#106875=CARTESIAN_POINT('Ctrl Pts',(5.11285161102587,2.6257863747464,5.13676245265066));
#106876=CARTESIAN_POINT('Ctrl Pts',(5.12241027542293,2.6235415858732,5.12717693379532));
#106877=CARTESIAN_POINT('Ctrl Pts',(5.13196893981999,2.621296797,5.11759141494));
#106878=CARTESIAN_POINT('Ctrl Pts',(5.41006903912,2.555986835,4.83871001114));
#106879=CARTESIAN_POINT('Ctrl Pts',(5.65631079023,2.49066265,4.53133482854));
#106880=CARTESIAN_POINT('',(5.65683405948763,2.49144077991402,4.53461449353211));
#106881=CARTESIAN_POINT('Origin',(-0.149059046435998,2.55357125054164,-0.13269161056075));
#106882=CARTESIAN_POINT('Ctrl Pts',(5.85211823186666,2.53084202101146,4.69070487206605));
#106883=CARTESIAN_POINT('Ctrl Pts',(5.81951568170992,2.52458961890036,4.66469342404254));
#106884=CARTESIAN_POINT('Ctrl Pts',(5.78692346058046,2.51818504847848,4.63866781124984));
#106885=CARTESIAN_POINT('Ctrl Pts',(5.72183874466787,2.5050621489152,4.5866471962267));
#106886=CARTESIAN_POINT('Ctrl Pts',(5.6893089173677,2.49833629949945,4.56062235843184));
#106887=CARTESIAN_POINT('Ctrl Pts',(5.65683406228975,2.49144078081474,4.53461448979442));
#106888=CARTESIAN_POINT('Ctrl Pts',(5.691712671,2.490655005,4.884097344));
#106889=CARTESIAN_POINT('Ctrl Pts',(5.959105067,2.556411293,4.572489983));
#106890=CARTESIAN_POINT('Ctrl Pts',(6.19088182200001,2.621296797,4.23355433));
#106891=CARTESIAN_POINT('Ctrl Pts',(5.653866134,2.490655005,4.538314416));
#106892=CARTESIAN_POINT('Ctrl Pts',(5.902327759,2.556411293,4.22877906));
#106893=CARTESIAN_POINT('Ctrl Pts',(6.115513083,2.621296797,3.893969662));
#106894=CARTESIAN_POINT('Origin',(-0.143646806777386,2.41076920669575,-0.132358290931466));
#106895=CARTESIAN_POINT('Ctrl Pts',(6.44152780532351,2.62578637474175,3.84256315617851));
#106896=CARTESIAN_POINT('Ctrl Pts',(6.44865992058243,2.62354158587088,3.83050499356447));
#106897=CARTESIAN_POINT('Ctrl Pts',(6.45579203584126,2.621296797,3.8184468309505));
#106898=CARTESIAN_POINT('Ctrl Pts',(6.66329403417114,2.555986835,3.46762624718635));
#106899=CARTESIAN_POINT('Ctrl Pts',(6.83155779937354,2.49066265,3.09638580299899));
#106900=CARTESIAN_POINT('Ctrl Pts',(6.10096672854028,2.62578637474176,3.91681483759952));
#106901=CARTESIAN_POINT('Ctrl Pts',(6.10823990577019,2.62354158587088,3.90539224979975));
#106902=CARTESIAN_POINT('Ctrl Pts',(6.115513083,2.621296797,3.893969662));
#106903=CARTESIAN_POINT('Ctrl Pts',(6.32711914299999,2.555986835,3.561640513));
#106904=CARTESIAN_POINT('Ctrl Pts',(6.501466607,2.49066265,3.208337881));
#106905=CARTESIAN_POINT('Ctrl Pts',(6.09756806636723,2.62578637474176,3.91755583942896));
#106906=CARTESIAN_POINT('Ctrl Pts',(6.1048426513386,2.62354158587088,3.90613959440948));
#106907=CARTESIAN_POINT('Ctrl Pts',(6.11211723631001,2.621296797,3.89472334939));
#106908=CARTESIAN_POINT('Ctrl Pts',(6.32376425318999,2.555986835,3.56257873745));
#106909=CARTESIAN_POINT('Ctrl Pts',(6.49817243005,2.49066265,3.20945511758));
#106910=CARTESIAN_POINT('',(6.49938849676083,2.49144077990629,3.21254561858896));
#106911=CARTESIAN_POINT('Origin',(-0.174099247004624,2.55357123366904,-0.0975462565322924));
#106912=CARTESIAN_POINT('Ctrl Pts',(6.72366185073863,2.53084202102691,3.32300636632164));
#106913=CARTESIAN_POINT('Ctrl Pts',(6.68622983778571,2.52458961891645,3.30461163604301));
#106914=CARTESIAN_POINT('Ctrl Pts',(6.6488048672343,2.51818504847267,3.28620085165096));
#106915=CARTESIAN_POINT('Ctrl Pts',(6.57405890157978,2.50506214891626,3.24938773966147));
#106916=CARTESIAN_POINT('Ctrl Pts',(6.53669503270045,2.49833629947486,3.23096429927423));
#106917=CARTESIAN_POINT('Ctrl Pts',(6.49938849887346,2.49144078080004,3.21254561397528));
#106918=CARTESIAN_POINT('Ctrl Pts',(6.608580148,2.490655005,3.546359884));
#106919=CARTESIAN_POINT('Ctrl Pts',(6.802734686,2.556411293,3.184556269));
#106920=CARTESIAN_POINT('Ctrl Pts',(6.956231483,2.621296797,2.803719592));
#106921=CARTESIAN_POINT('Ctrl Pts',(6.497285334,2.490655005,3.216797055));
#106922=CARTESIAN_POINT('Ctrl Pts',(6.673397112,2.556411293,2.861086559));
#106923=CARTESIAN_POINT('Ctrl Pts',(6.809624158,2.621296797,2.488276275));
#106924=CARTESIAN_POINT('Origin',(-0.1687414122409,2.41076915116035,-0.0983839597344316));
#106925=CARTESIAN_POINT('Ctrl Pts',(7.11696595813061,2.62578637464404,2.36798809633568));
#106926=CARTESIAN_POINT('Ctrl Pts',(7.1213391798758,2.62354158582205,2.35467865318869));
#106927=CARTESIAN_POINT('Ctrl Pts',(7.12571240162084,2.621296797,2.34136921004164));
#106928=CARTESIAN_POINT('Ctrl Pts',(7.2529470631546,2.555986835,1.95414382044684));
#106929=CARTESIAN_POINT('Ctrl Pts',(7.33747119381903,2.49066265,1.55541103631253));
#106930=CARTESIAN_POINT('Ctrl Pts',(6.80032892691287,2.62578637464404,2.51371437875452));
#106931=CARTESIAN_POINT('Ctrl Pts',(6.80497654245637,2.62354158582205,2.50099532687726));
#106932=CARTESIAN_POINT('Ctrl Pts',(6.809624158,2.621296797,2.488276275));
#106933=CARTESIAN_POINT('Ctrl Pts',(6.944842042,2.555986835,2.118227749));
#106934=CARTESIAN_POINT('Ctrl Pts',(7.039163737,2.49066265,1.735705586));
#106935=CARTESIAN_POINT('Ctrl Pts',(6.79716901706411,2.62578637464404,2.51516866827108));
#106936=CARTESIAN_POINT('Ctrl Pts',(6.80181937094693,2.62354158582205,2.50245550826054));
#106937=CARTESIAN_POINT('Ctrl Pts',(6.80646972483,2.621296797,2.48974234825));
#106938=CARTESIAN_POINT('Ctrl Pts',(6.94176727817,2.555986835,2.11986524042));
#106939=CARTESIAN_POINT('Ctrl Pts',(7.03618674890999,2.49066265,1.73750485288));
#106940=CARTESIAN_POINT('',(7.03803875113731,2.49144077992003,1.74026168046717));
#106941=CARTESIAN_POINT('Origin',(-0.190998271340511,2.55357130199046,-0.0578394435494334));
#106942=CARTESIAN_POINT('Ctrl Pts',(7.28081451460901,2.5308420210154,1.79992777604475));
#106943=CARTESIAN_POINT('Ctrl Pts',(7.24030324971045,2.52458960837035,1.79000986396438));
#106944=CARTESIAN_POINT('Ctrl Pts',(7.19979551660118,2.51818504338184,1.78007478494001));
#106945=CARTESIAN_POINT('Ctrl Pts',(7.11888337027677,2.5050621488933,1.76019052401277));
#106946=CARTESIAN_POINT('Ctrl Pts',(7.07843255283466,2.49833629947179,1.75022994088429));
#106947=CARTESIAN_POINT('Ctrl Pts',(7.03803875201506,2.49144078078745,1.74026167631028));
#106948=CARTESIAN_POINT('Ctrl Pts',(7.216437762,2.490655005,2.042798577));
#106949=CARTESIAN_POINT('Ctrl Pts',(7.328275993,2.556411293,1.647716243));
#106950=CARTESIAN_POINT('Ctrl Pts',(7.396315492,2.621296797,1.242786042));
#106951=CARTESIAN_POINT('Ctrl Pts',(7.036898692,2.490655005,1.744865839));
#106952=CARTESIAN_POINT('Ctrl Pts',(7.132425833,2.556411293,1.35961283));
#106953=CARTESIAN_POINT('Ctrl Pts',(7.185324776,2.621296797,0.966233856));
#106954=CARTESIAN_POINT('Origin',(-0.185946087418248,2.41076918789427,-0.0598094055549393));
#106955=CARTESIAN_POINT('Ctrl Pts',(7.45962269256189,2.62578637465542,0.782688546059122));
#106956=CARTESIAN_POINT('Ctrl Pts',(7.46103253396334,2.62354158582774,0.768750156846797));
#106957=CARTESIAN_POINT('Ctrl Pts',(7.46244237536476,2.621296797,0.754811767634472));
#106958=CARTESIAN_POINT('Ctrl Pts',(7.50346034873277,2.555986835,0.349287800947316));
#106959=CARTESIAN_POINT('Ctrl Pts',(7.50029259058375,2.49066265,-0.0582930225763819));
#106960=CARTESIAN_POINT('Ctrl Pts',(7.18171530263629,2.62578637465542,0.993075431001356));
#106961=CARTESIAN_POINT('Ctrl Pts',(7.18352003931813,2.62354158582774,0.979654643500677));
#106962=CARTESIAN_POINT('Ctrl Pts',(7.185324776,2.621296797,0.966233856));
#106963=CARTESIAN_POINT('Ctrl Pts',(7.237831846,2.555986835,0.575769011));
#106964=CARTESIAN_POINT('Ctrl Pts',(7.247717395,2.49066265,0.181913626));
#106965=CARTESIAN_POINT('Ctrl Pts',(7.17894189898503,2.62578637465542,0.99517500724877));
#106966=CARTESIAN_POINT('Ctrl Pts',(7.18075057656252,2.62354158582774,0.98175938520438));
#106967=CARTESIAN_POINT('Ctrl Pts',(7.18255925414001,2.621296797,0.968343763159999));
#106968=CARTESIAN_POINT('Ctrl Pts',(7.23518098069,2.555986835,0.578029202120001));
#106969=CARTESIAN_POINT('Ctrl Pts',(7.24519679643001,2.49066265,0.18431079146));
#106970=CARTESIAN_POINT('',(7.24759813578468,2.49144077987902,0.186605041169715));
#106971=CARTESIAN_POINT('Origin',(-0.198966747438476,2.55357127314528,-0.0154282146168049));
#106972=CARTESIAN_POINT('Ctrl Pts',(7.49752438372847,2.53084202102278,0.19268656358911));
#106973=CARTESIAN_POINT('Ctrl Pts',(7.4558282619199,2.52458961889093,0.191709252839032));
#106974=CARTESIAN_POINT('Ctrl Pts',(7.41413179084399,2.51818504845344,0.19071441476443));
#106975=CARTESIAN_POINT('Ctrl Pts',(7.33083676504294,2.50506214889565,0.188688755670287));
#106976=CARTESIAN_POINT('Ctrl Pts',(7.28919043403217,2.4983362994351,0.187656775431307));
#106977=CARTESIAN_POINT('Ctrl Pts',(7.24759813575377,2.49144078078428,0.186605036456807));
#106978=CARTESIAN_POINT('Ctrl Pts',(7.48686276700001,2.490655005,0.443718279));
#106979=CARTESIAN_POINT('Ctrl Pts',(7.511155258,2.556411293,0.033830836));
#106980=CARTESIAN_POINT('Ctrl Pts',(7.490556008,2.621296797,-0.376258802));
#106981=CARTESIAN_POINT('Ctrl Pts',(7.247474489,2.490655005,0.191346636));
#106982=CARTESIAN_POINT('Ctrl Pts',(7.25795025,2.556411293,-0.205434883));
#106983=CARTESIAN_POINT('Ctrl Pts',(7.22504759300001,2.621296797,-0.600988585));
#106984=CARTESIAN_POINT('Origin',(-0.194455944157425,2.41076918068398,-0.018438186900226));
#106985=CARTESIAN_POINT('Ctrl Pts',(7.45347576122951,2.62578637474903,-0.839208650378814));
#106986=CARTESIAN_POINT('Ctrl Pts',(7.45185629962364,2.62354158587455,-0.853124242334209));
#106987=CARTESIAN_POINT('Ctrl Pts',(7.45023683801784,2.621296797,-0.867039834289613));
#106988=CARTESIAN_POINT('Ctrl Pts',(7.40312016832359,2.555986835,-1.27190052837077));
#106989=CARTESIAN_POINT('Ctrl Pts',(7.31240864069535,2.49066265,-1.66927136382544));
#106990=CARTESIAN_POINT('Ctrl Pts',(7.22729265237664,2.62578637474904,-0.573998620455721));
#106991=CARTESIAN_POINT('Ctrl Pts',(7.22617012268838,2.62354158587455,-0.587493602727866));
#106992=CARTESIAN_POINT('Ctrl Pts',(7.225047593,2.621296797,-0.600988585));
#106993=CARTESIAN_POINT('Ctrl Pts',(7.192388677,2.555986835,-0.993612047));
#106994=CARTESIAN_POINT('Ctrl Pts',(7.117375842,2.49066265,-1.380384412));
#106995=CARTESIAN_POINT('Ctrl Pts',(7.22503543618639,2.62578637474904,-0.571351931335677));
#106996=CARTESIAN_POINT('Ctrl Pts',(7.22391786567831,2.62354158587455,-0.584842716092841));
#106997=CARTESIAN_POINT('Ctrl Pts',(7.22280029517,2.621296797,-0.59833350085));
#106998=CARTESIAN_POINT('Ctrl Pts',(7.19028566172001,2.555986835,-0.99083484021));
#106999=CARTESIAN_POINT('Ctrl Pts',(7.11542949334,2.49066265,-1.37750143675));
#107000=CARTESIAN_POINT('',(7.11826788656464,2.4914407799091,-1.37577704263276));
#107001=CARTESIAN_POINT('Origin',(-0.197631358335422,2.55357126158124,0.0277044275792105));
#107002=CARTESIAN_POINT('Ctrl Pts',(7.36365834559444,2.53084202102572,-1.42356445854499));
#107003=CARTESIAN_POINT('Ctrl Pts',(7.32272696298888,2.52458961890017,-1.41555548667759));
#107004=CARTESIAN_POINT('Ctrl Pts',(7.28179147137135,2.51818504846001,-1.40756355721964));
#107005=CARTESIAN_POINT('Ctrl Pts',(7.20000837997913,2.50506214889318,-1.3916358889752));
#107006=CARTESIAN_POINT('Ctrl Pts',(7.15911387198551,2.49833629947242,-1.38369101187184));
#107007=CARTESIAN_POINT('Ctrl Pts',(7.1182678855985,2.49144078080531,-1.37577704683838));
#107008=CARTESIAN_POINT('Ctrl Pts',(7.40721039,2.490655005,-1.176109793));
#107009=CARTESIAN_POINT('Ctrl Pts',(7.342821252,2.556411293,-1.581636462));
#107010=CARTESIAN_POINT('Ctrl Pts',(7.234546451,2.621296797,-1.977710203));
#107011=CARTESIAN_POINT('Ctrl Pts',(7.11916643300001,2.490655005,-1.371119723));
#107012=CARTESIAN_POINT('Ctrl Pts',(7.044100979,2.556411293,-1.76087669));
#107013=CARTESIAN_POINT('Ctrl Pts',(6.926935215,2.621296797,-2.140109468));
#107014=CARTESIAN_POINT('Origin',(-0.19387335622159,2.4107691791716,0.0237951653835827));
#107015=CARTESIAN_POINT('Ctrl Pts',(7.09881258653112,2.62578637474301,-2.42186538442023));
#107016=CARTESIAN_POINT('Ctrl Pts',(7.09423954612711,2.62354158587153,-2.4351075011484));
#107017=CARTESIAN_POINT('Ctrl Pts',(7.0896665057231,2.621296797,-2.4483496178766));
#107018=CARTESIAN_POINT('Ctrl Pts',(6.95661831629296,2.555986835,-2.83361620186909));
#107019=CARTESIAN_POINT('Ctrl Pts',(6.78260459090735,2.49066265,-3.20219643111982));
#107020=CARTESIAN_POINT('Ctrl Pts',(6.93492983067391,2.625786374743,-2.1142331352719));
#107021=CARTESIAN_POINT('Ctrl Pts',(6.93093252283703,2.62354158587153,-2.12717130163598));
#107022=CARTESIAN_POINT('Ctrl Pts',(6.926935215,2.621296797,-2.140109468));
#107023=CARTESIAN_POINT('Ctrl Pts',(6.810637408,2.555986835,-2.51653291));
#107024=CARTESIAN_POINT('Ctrl Pts',(6.654233705,2.49066265,-2.878137209));
#107025=CARTESIAN_POINT('Ctrl Pts',(6.93329434687637,2.625786374743,-2.11116308951596));
#107026=CARTESIAN_POINT('Ctrl Pts',(6.92930278461823,2.62354158587153,-2.12409822257802));
#107027=CARTESIAN_POINT('Ctrl Pts',(6.92531122236,2.621296797,-2.13703335564));
#107028=CARTESIAN_POINT('Ctrl Pts',(6.80918057742,2.555986835,-2.51336854665));
#107029=CARTESIAN_POINT('Ctrl Pts',(6.65295261534,2.49066265,-2.87490322868));
#107030=CARTESIAN_POINT('',(6.65609534290415,2.49144077992861,-2.87382932098846));
#107031=CARTESIAN_POINT('Origin',(-0.187055439915538,2.55357125199513,0.0695416967133695));
#107032=CARTESIAN_POINT('Ctrl Pts',(6.88547582727293,2.53084202099626,-2.9732511882983));
#107033=CARTESIAN_POINT('Ctrl Pts',(6.8472230899018,2.52458961887946,-2.95663042439173));
#107034=CARTESIAN_POINT('Ctrl Pts',(6.80896267611096,2.51818504847444,-2.94002542125642));
#107035=CARTESIAN_POINT('Ctrl Pts',(6.73251560584466,2.50506214892888,-2.90688918613168));
#107036=CARTESIAN_POINT('Ctrl Pts',(6.69428510228322,2.49833629948875,-2.89033894558378));
#107037=CARTESIAN_POINT('Ctrl Pts',(6.65609534087841,2.49144078083071,-2.8738293252976));
#107038=CARTESIAN_POINT('Ctrl Pts',(6.981205087,2.490655005,-2.740944277));
#107039=CARTESIAN_POINT('Ctrl Pts',(6.831145085,2.556411293,-3.123148198));
#107040=CARTESIAN_POINT('Ctrl Pts',(6.640257542,2.621296797,-3.486686073));
#107041=CARTESIAN_POINT('Ctrl Pts',(6.657974068,2.490655005,-2.869474048));
#107042=CARTESIAN_POINT('Ctrl Pts',(6.500877375,2.556411293,-3.23398186));
#107043=CARTESIAN_POINT('Ctrl Pts',(6.304927044,2.621296797,-3.57916121));
#107044=CARTESIAN_POINT('Origin',(-0.184225460090732,2.410769191445,0.0649159095010382));
#107045=CARTESIAN_POINT('Ctrl Pts',(6.41221682473796,2.62578637463497,-3.89127838495056));
#107046=CARTESIAN_POINT('Ctrl Pts',(6.40490403598196,2.62354158581749,-3.90322783954274));
#107047=CARTESIAN_POINT('Ctrl Pts',(6.39759124722611,2.621296797,-3.91517729413494));
#107048=CARTESIAN_POINT('Ctrl Pts',(6.18483272311034,2.555986835,-4.26283513136997));
#107049=CARTESIAN_POINT('Ctrl Pts',(5.93565348803106,2.49066265,-4.58539035288199));
#107050=CARTESIAN_POINT('Ctrl Pts',(6.31829739625385,2.62578637463497,-3.55560845819269));
#107051=CARTESIAN_POINT('Ctrl Pts',(6.31161222012691,2.62354158581749,-3.56738483409634));
#107052=CARTESIAN_POINT('Ctrl Pts',(6.304927044,2.621296797,-3.57916121));
#107053=CARTESIAN_POINT('Ctrl Pts',(6.110428303,2.555986835,-3.92178349));
#107054=CARTESIAN_POINT('Ctrl Pts',(5.879946996,2.49066265,-4.24131151));
#107055=CARTESIAN_POINT('Ctrl Pts',(6.31736011824208,2.62578637463497,-3.5522586077237));
#107056=CARTESIAN_POINT('Ctrl Pts',(6.31068120543602,2.62354158581749,-3.56403325637183));
#107057=CARTESIAN_POINT('Ctrl Pts',(6.30400229263001,2.621296797,-3.57580790502));
#107058=CARTESIAN_POINT('Ctrl Pts',(6.1096857769,2.555986835,-3.91837993219));
#107059=CARTESIAN_POINT('Ctrl Pts',(5.87939106768,2.49066265,-4.23787774194));
#107060=CARTESIAN_POINT('',(5.88269117803411,2.49144077925192,-4.23750453416556));
#107061=CARTESIAN_POINT('Origin',(-0.167732537891393,2.55357122438483,0.108127094189924));
#107062=CARTESIAN_POINT('Ctrl Pts',(6.08533611175123,2.53084202103098,-4.38391199742654));
#107063=CARTESIAN_POINT('Ctrl Pts',(6.05155067503814,2.52458961889364,-4.35945660995114));
#107064=CARTESIAN_POINT('Ctrl Pts',(6.01775435318723,2.51818504845103,-4.33501496450926));
#107065=CARTESIAN_POINT('Ctrl Pts',(5.95021788409655,2.50506214889897,-4.2862195759487));
#107066=CARTESIAN_POINT('Ctrl Pts',(5.91643900043463,2.49833629934497,-4.26183784232312));
#107067=CARTESIAN_POINT('Ctrl Pts',(5.8826911748804,2.49144078071014,-4.2375045381262));
#107068=CARTESIAN_POINT('Ctrl Pts',(6.228766394,2.490655005,-4.177615254));
#107069=CARTESIAN_POINT('Ctrl Pts',(6.000052166,2.556411293,-4.518624994));
#107070=CARTESIAN_POINT('Ctrl Pts',(5.735477571,2.621296797,-4.832628377));
#107071=CARTESIAN_POINT('Ctrl Pts',(5.885462235,2.490655005,-4.233654956));
#107072=CARTESIAN_POINT('Ctrl Pts',(5.653679971,2.556411293,-4.555869632));
#107073=CARTESIAN_POINT('Ctrl Pts',(5.388107493,2.621296797,-4.850855352));
#107074=CARTESIAN_POINT('Origin',(-0.165963364033447,2.41076915419993,0.103001217880749));
#107075=CARTESIAN_POINT('Ctrl Pts',(5.42579293193456,2.62578637464283,-5.17873953196371));
#107076=CARTESIAN_POINT('Ctrl Pts',(5.41608233257228,2.62354158582141,-5.18883758156318));
#107077=CARTESIAN_POINT('Ctrl Pts',(5.40637173320981,2.621296797,-5.19893563116276));
#107078=CARTESIAN_POINT('Ctrl Pts',(5.12385122646595,2.555986835,-5.49272862822822));
#107079=CARTESIAN_POINT('Ctrl Pts',(4.81115782554438,2.49066265,-5.75417651719663));
#107080=CARTESIAN_POINT('Ctrl Pts',(5.40622839938115,2.62578637464282,-4.83072748088294));
#107081=CARTESIAN_POINT('Ctrl Pts',(5.3971679461906,2.62354158582141,-4.84079141644148));
#107082=CARTESIAN_POINT('Ctrl Pts',(5.388107493,2.621296797,-4.850855352));
#107083=CARTESIAN_POINT('Ctrl Pts',(5.124502361,2.555986835,-5.143655834));
#107084=CARTESIAN_POINT('Ctrl Pts',(4.830720501,2.49066265,-5.406166798));
#107085=CARTESIAN_POINT('Ctrl Pts',(5.40603315323804,2.62578637464282,-4.82725446099159));
#107086=CARTESIAN_POINT('Ctrl Pts',(5.39697918824405,2.62354158582141,-4.83731805610587));
#107087=CARTESIAN_POINT('Ctrl Pts',(5.38792522325,2.621296797,-4.84738165122));
#107088=CARTESIAN_POINT('Ctrl Pts',(5.12450885906,2.555986835,-5.14017222832));
#107089=CARTESIAN_POINT('Ctrl Pts',(4.83091572861001,2.49066265,-5.40269380138));
#107090=CARTESIAN_POINT('',(4.83421891288047,2.49144077990264,-5.40303874585956));
#107091=CARTESIAN_POINT('Origin',(-0.140567026918504,2.55357128902595,0.141656766217955));
#107092=CARTESIAN_POINT('Ctrl Pts',(5.00065284321323,2.53084202097844,-5.58958595417019));
#107093=CARTESIAN_POINT('Ctrl Pts',(4.97291443011114,2.52458960835985,-5.55843939754943));
#107094=CARTESIAN_POINT('Ctrl Pts',(4.9451625040527,2.51818504337976,-5.52730400233));
#107095=CARTESIAN_POINT('Ctrl Pts',(4.88969458781793,2.50506214891053,-5.4651311021405));
#107096=CARTESIAN_POINT('Ctrl Pts',(4.86194678848643,2.49833629952378,-5.43405793901533));
#107097=CARTESIAN_POINT('Ctrl Pts',(4.83421890948478,2.4914407808494,-5.40303874868449));
#107098=CARTESIAN_POINT('Ctrl Pts',(5.185077507,2.490655005,-5.418945585));
#107099=CARTESIAN_POINT('Ctrl Pts',(4.888403477,2.556411293,-5.702815909));
#107100=CARTESIAN_POINT('Ctrl Pts',(4.562513043,2.621296797,-5.952602349));
#107101=CARTESIAN_POINT('Ctrl Pts',(4.837752729,2.490655005,-5.399874863));
#107102=CARTESIAN_POINT('Ctrl Pts',(4.542122774,2.556411293,-5.664730004));
#107103=CARTESIAN_POINT('Ctrl Pts',(4.219346023,2.621296797,-5.895728889));
#107104=CARTESIAN_POINT('Origin',(-0.139941037339313,2.41076919133494,0.136270381714059));
#107105=CARTESIAN_POINT('Ctrl Pts',(4.18566499123835,2.62578637470629,-6.2240485747905));
#107106=CARTESIAN_POINT('Ctrl Pts',(4.17401063797517,2.62354158585314,-6.23182304588717));
#107107=CARTESIAN_POINT('Ctrl Pts',(4.16235628471194,2.621296797,-6.23959751698383));
#107108=CARTESIAN_POINT('Ctrl Pts',(3.82328414093743,2.555986835,-6.46578823919025));
#107109=CARTESIAN_POINT('Ctrl Pts',(3.46169776941117,2.49066265,-6.65390378403682));
#107110=CARTESIAN_POINT('Ctrl Pts',(4.24137017021633,2.62578637470629,-5.87996705533536));
#107111=CARTESIAN_POINT('Ctrl Pts',(4.23035809660814,2.62354158585314,-5.88784797216773));
#107112=CARTESIAN_POINT('Ctrl Pts',(4.219346023,2.621296797,-5.895728889));
#107113=CARTESIAN_POINT('Ctrl Pts',(3.898960385,2.555986835,-6.125016547));
#107114=CARTESIAN_POINT('Ctrl Pts',(3.555614883,2.49066265,-6.31823573500001));
#107115=CARTESIAN_POINT('Ctrl Pts',(4.24192608543249,2.62578637470629,-5.87653326056434));
#107116=CARTESIAN_POINT('Ctrl Pts',(4.23092042151628,2.62354158585314,-5.88441523968222));
#107117=CARTESIAN_POINT('Ctrl Pts',(4.2199147576,2.621296797,-5.8922972188));
#107118=CARTESIAN_POINT('Ctrl Pts',(3.89971560339,2.555986835,-6.12161578297));
#107119=CARTESIAN_POINT('Ctrl Pts',(3.55655213791,2.49066265,-6.31488590327));
#107120=CARTESIAN_POINT('',(3.55970394316432,2.49144077994426,-6.31593287016467));
#107121=CARTESIAN_POINT('Origin',(-0.106828722370003,2.55357124591186,0.168562830045095));
#107122=CARTESIAN_POINT('Ctrl Pts',(3.68214460546017,2.53084202104465,-6.53389708360331));
#107123=CARTESIAN_POINT('Ctrl Pts',(3.66175032427548,2.52458961893437,-6.49751583846893));
#107124=CARTESIAN_POINT('Ctrl Pts',(3.64134039390339,2.51818504852252,-6.4611424947273));
#107125=CARTESIAN_POINT('Ctrl Pts',(3.60053460648105,2.5050621489647,-6.38849917192798));
#107126=CARTESIAN_POINT('Ctrl Pts',(3.58011534677004,2.49833629958865,-6.35218752553789));
#107127=CARTESIAN_POINT('Ctrl Pts',(3.55970393905361,2.49144078091802,-6.3159328722938));
#107128=CARTESIAN_POINT('Ctrl Pts',(3.898940158,2.490655005,-6.406892042));
#107129=CARTESIAN_POINT('Ctrl Pts',(3.548178474,2.556411293,-6.620349489));
#107130=CARTESIAN_POINT('Ctrl Pts',(3.176210476,2.621296797,-6.794239252));
#107131=CARTESIAN_POINT('Ctrl Pts',(3.563835282,2.490655005,-6.313602623));
#107132=CARTESIAN_POINT('Ctrl Pts',(3.218180965,2.556411293,-6.508713897));
#107133=CARTESIAN_POINT('Ctrl Pts',(2.853292624,2.621296797,-6.664924696));
#107134=CARTESIAN_POINT('Origin',(-0.10737519180722,2.41076923273296,0.163167647018698));
#107135=CARTESIAN_POINT('Ctrl Pts',(2.74982000782157,2.62578637464853,-6.97832802384387));
#107136=CARTESIAN_POINT('Ctrl Pts',(2.73676684554022,2.62354158582426,-6.9834153906098));
#107137=CARTESIAN_POINT('Ctrl Pts',(2.72371368325887,2.621296797,-6.98850275737571));
#107138=CARTESIAN_POINT('Ctrl Pts',(2.34394453822343,2.555986835,-7.13651477818134));
#107139=CARTESIAN_POINT('Ctrl Pts',(1.95037257434254,2.49066265,-7.24250190481632));
#107140=CARTESIAN_POINT('Ctrl Pts',(2.87819018699071,2.62578637464852,-6.65426590596132));
#107141=CARTESIAN_POINT('Ctrl Pts',(2.86574140549535,2.62354158582426,-6.65959530098065));
#107142=CARTESIAN_POINT('Ctrl Pts',(2.853292624,2.621296797,-6.664924696));
#107143=CARTESIAN_POINT('Ctrl Pts',(2.491107354,2.555986835,-6.819978295));
#107144=CARTESIAN_POINT('Ctrl Pts',(2.114252666,2.49066265,-6.934870991));
#107145=CARTESIAN_POINT('Ctrl Pts',(2.8794712695978,2.62578637464852,-6.65103189674261));
#107146=CARTESIAN_POINT('Ctrl Pts',(2.8670285195789,2.62354158582426,-6.65636370710631));
#107147=CARTESIAN_POINT('Ctrl Pts',(2.85458576956,2.621296797,-6.66169551747));
#107148=CARTESIAN_POINT('Ctrl Pts',(2.49257597954,2.555986835,-6.81681938857999));
#107149=CARTESIAN_POINT('Ctrl Pts',(2.11588812321,2.49066265,-6.93180095857));
#107150=CARTESIAN_POINT('',(2.11874117385913,2.49144077990718,-6.93350099308308));
#107151=CARTESIAN_POINT('Origin',(-0.0680950929919488,2.55357123368024,
0.187586940969906));
#107152=CARTESIAN_POINT('Ctrl Pts',(2.19146337849108,2.5308420210064,-7.17269044782304));
#107153=CARTESIAN_POINT('Ctrl Pts',(2.17936679654677,2.52458961889286,-7.13277560835312));
#107154=CARTESIAN_POINT('Ctrl Pts',(2.16725323268617,2.51818504846641,-7.09286512135973));
#107155=CARTESIAN_POINT('Ctrl Pts',(2.14301762893445,2.5050621489118,-7.01314812101274));
#107156=CARTESIAN_POINT('Ctrl Pts',(2.13088169066015,2.49833629949416,-6.97329588324911));
#107157=CARTESIAN_POINT('Ctrl Pts',(2.11874116901779,2.49144078082763,-6.93350099440057));
#107158=CARTESIAN_POINT('Ctrl Pts',(2.430492701,2.490655005,-7.095259349));
#107159=CARTESIAN_POINT('Ctrl Pts',(2.042044589,2.556411293,-7.228322886));
#107160=CARTESIAN_POINT('Ctrl Pts',(1.641391837,2.621296797,-7.318185078));
#107161=CARTESIAN_POINT('Ctrl Pts',(2.123276858,2.490655005,-6.932113342));
#107162=CARTESIAN_POINT('Ctrl Pts',(1.743760591,2.556411293,-7.048357562));
#107163=CARTESIAN_POINT('Ctrl Pts',(1.353822432,2.621296797,-7.122476032));
#107164=CARTESIAN_POINT('Origin',(-0.06978859721431,2.41076920475297,0.182435340521501));
#107165=CARTESIAN_POINT('Ctrl Pts',(1.185396495819,2.62578637457119,-7.40630861043433));
#107166=CARTESIAN_POINT('Ctrl Pts',(1.17155487598352,2.6235415857856,-7.40847099329535));
#107167=CARTESIAN_POINT('Ctrl Pts',(1.15771325614802,2.621296797,-7.41063337615642));
#107168=CARTESIAN_POINT('Ctrl Pts',(0.755004693420207,2.555986835,-7.4735458173585));
#107169=CARTESIAN_POINT('Ctrl Pts',(0.347850124077357,2.49066265,-7.49244868540235));
#107170=CARTESIAN_POINT('Ctrl Pts',(1.38042922812604,2.6257863745712,-7.1174186787875));
#107171=CARTESIAN_POINT('Ctrl Pts',(1.36712583006301,2.6235415857856,-7.11994735539381));
#107172=CARTESIAN_POINT('Ctrl Pts',(1.353822432,2.621296797,-7.12247603199999));
#107173=CARTESIAN_POINT('Ctrl Pts',(0.966772911999999,2.555986835,-7.196045436));
#107174=CARTESIAN_POINT('Ctrl Pts',(0.574030344,2.49066265,-7.227239388));
#107175=CARTESIAN_POINT('Ctrl Pts',(1.38237557612367,2.6257863745712,-7.11453567379976));
#107176=CARTESIAN_POINT('Ctrl Pts',(1.36907754929682,2.6235415857856,-7.11706800587));
#107177=CARTESIAN_POINT('Ctrl Pts',(1.35577952247,2.621296797,-7.11960033794));
#107178=CARTESIAN_POINT('Ctrl Pts',(0.968886273399999,2.555986835,-7.19327609412999));
#107179=CARTESIAN_POINT('Ctrl Pts',(0.57628753136,2.49066265,-7.22459270619));
#107180=CARTESIAN_POINT('',(0.578708421721061,2.49144077986087,-7.22686631479657));
#107181=CARTESIAN_POINT('Origin',(-0.0261773973728766,2.55357124537482,
0.197839503071522));
#107182=CARTESIAN_POINT('Ctrl Pts',(0.598311758986545,2.53084202105489,
-7.47609677807153));
#107183=CARTESIAN_POINT('Ctrl Pts',(0.595078493574171,2.52458960821832,
-7.43451464653647));
#107184=CARTESIAN_POINT('Ctrl Pts',(0.591827716122453,2.51818504328756,
-7.39293322468143));
#107185=CARTESIAN_POINT('Ctrl Pts',(0.585295528807562,2.50506214885077,
-7.30987005778724));
#107186=CARTESIAN_POINT('Ctrl Pts',(0.582010375225292,2.49833629930322,
-7.26834067461977));
#107187=CARTESIAN_POINT('Ctrl Pts',(0.578708417200044,2.49144078060891,
-7.22686631503214));
#107188=CARTESIAN_POINT('Ctrl Pts',(0.848398107,2.490655005,-7.45186021400001));
#107189=CARTESIAN_POINT('Ctrl Pts',(0.440426968,2.556411293,-7.498307938));
#107190=CARTESIAN_POINT('Ctrl Pts',(0.029823541,2.621296797,-7.499940704));
#107191=CARTESIAN_POINT('Ctrl Pts',(0.583436368,2.490655005,-7.226486145));
#107192=CARTESIAN_POINT('Ctrl Pts',(0.18780391,2.556411293,-7.258427861));
#107193=CARTESIAN_POINT('Ctrl Pts',(-0.208950992,2.621296797,-7.246988304));
#107194=CARTESIAN_POINT('Origin',(-0.0289387772614658,2.4107691699622,0.193172334428261));
#107195=CARTESIAN_POINT('Ctrl Pts',(-0.434454836636775,2.62578637474255,
-7.48797843674285));
#107196=CARTESIAN_POINT('Ctrl Pts',(-0.448437696021263,2.62354158587127,
-7.48711472518744));
#107197=CARTESIAN_POINT('Ctrl Pts',(-0.46242055540574,2.621296797,-7.486251013632));
#107198=CARTESIAN_POINT('Ctrl Pts',(-0.869238330894812,2.555986835,-7.46112216094296));
#107199=CARTESIAN_POINT('Ctrl Pts',(-1.27093741073832,2.49066265,-7.39205689301602));
#107200=CARTESIAN_POINT('Ctrl Pts',(-0.181879065534724,2.62578637474254,
-7.24776886349915));
#107201=CARTESIAN_POINT('Ctrl Pts',(-0.195415028767364,2.62354158587127,
-7.24737858374956));
#107202=CARTESIAN_POINT('Ctrl Pts',(-0.208950992,2.621296797,-7.246988304));
#107203=CARTESIAN_POINT('Ctrl Pts',(-0.602766756,2.555986835,-7.235633492));
#107204=CARTESIAN_POINT('Ctrl Pts',(-0.993032999,2.49066265,-7.181670103));
#107205=CARTESIAN_POINT('Ctrl Pts',(-0.179358461221376,2.62578637474254,
-7.24537166885228));
#107206=CARTESIAN_POINT('Ctrl Pts',(-0.192889964610694,2.62354158587127,
-7.24498611376109));
#107207=CARTESIAN_POINT('Ctrl Pts',(-0.206421468,2.621296797,-7.24460055867));
#107208=CARTESIAN_POINT('Ctrl Pts',(-0.60010747717,2.555986835,-7.23338320603999));
#107209=CARTESIAN_POINT('Ctrl Pts',(-0.990259625069999,2.49066265,-7.1795705277));
#107210=CARTESIAN_POINT('',(-0.988384093003052,2.4914407799151,-7.18231140161213));
#107211=CARTESIAN_POINT('Origin',(0.0169642529078204,2.55357128339156,0.198841623721516));
#107212=CARTESIAN_POINT('Ctrl Pts',(-1.02281625280334,2.53084202104047,
-7.42992913210504));
#107213=CARTESIAN_POINT('Ctrl Pts',(-1.0170350070352,2.52458961892557,-7.38862418208833));
#107214=CARTESIAN_POINT('Ctrl Pts',(-1.01127100116621,2.51818504848532,
-7.34731605168382));
#107215=CARTESIAN_POINT('Ctrl Pts',(-0.999794339433034,2.5050621489194,
-7.26479059594511));
#107216=CARTESIAN_POINT('Ctrl Pts',(-0.994075098219575,2.49833629950665,
-7.22352593649113));
#107217=CARTESIAN_POINT('Ctrl Pts',(-0.988384096897287,2.49144078082864,
-7.18231140092156));
#107218=CARTESIAN_POINT('Ctrl Pts',(-0.773366640000001,2.490655005,-7.46002037800001));
#107219=CARTESIAN_POINT('Ctrl Pts',(-1.181784528,2.556411293,-7.417680444));
#107220=CARTESIAN_POINT('Ctrl Pts',(-1.583139272,2.621296797,-7.331007437));
#107221=CARTESIAN_POINT('Ctrl Pts',(-0.983684957,2.490655005,-7.182956488));
#107222=CARTESIAN_POINT('Ctrl Pts',(-1.376934274,2.556411293,-7.12910214));
#107223=CARTESIAN_POINT('Ctrl Pts',(-1.7619541,2.621296797,-7.032639458));
#107224=CARTESIAN_POINT('Origin',(0.0132641981247958,2.41076921905478,0.194877278076248));
#107225=CARTESIAN_POINT('Ctrl Pts',(-2.03399154486877,2.62578637460005,
-7.21951871510429));
#107226=CARTESIAN_POINT('Ctrl Pts',(-2.04746181990288,2.62354158580003,
-7.21566929529137));
#107227=CARTESIAN_POINT('Ctrl Pts',(-2.06093209493694,2.621296797,-7.21181987547841));
#107228=CARTESIAN_POINT('Ctrl Pts',(-2.45283673674309,2.555986835,-7.09982472399587));
#107229=CARTESIAN_POINT('Ctrl Pts',(-2.83029732434835,2.49066265,-6.94602073587784));
#107230=CARTESIAN_POINT('Ctrl Pts',(-1.73568289820837,2.62578637460005,
-7.03922143219571));
#107231=CARTESIAN_POINT('Ctrl Pts',(-1.74881849910419,2.62354158580002,
-7.0359304450978));
#107232=CARTESIAN_POINT('Ctrl Pts',(-1.7619541,2.621296797,-7.032639458));
#107233=CARTESIAN_POINT('Ctrl Pts',(-2.144121721,2.555986835,-6.936891367));
#107234=CARTESIAN_POINT('Ctrl Pts',(-2.513663223,2.49066265,-6.80029390600001));
#107235=CARTESIAN_POINT('Ctrl Pts',(-1.73270589824414,2.62578637460005,
-7.03742213803926));
#107236=CARTESIAN_POINT('Ctrl Pts',(-1.7458381592271,2.62354158580002,-7.03413672387456));
#107237=CARTESIAN_POINT('Ctrl Pts',(-1.75897042021,2.621296797,-7.03085130971));
#107238=CARTESIAN_POINT('Ctrl Pts',(-2.14104086967,2.555986835,-6.93526535782));
#107239=CARTESIAN_POINT('Ctrl Pts',(-2.51050334239,2.49066265,-6.79883961102));
#107240=CARTESIAN_POINT('',(-2.50926086557921,2.49144077988688,-6.80191958859535));
#107241=CARTESIAN_POINT('Origin',(0.0593126565459542,2.55357125085242,0.190545812164162));
#107242=CARTESIAN_POINT('Ctrl Pts',(-2.59611851297963,2.53084202105645,
-7.03634625763598));
#107243=CARTESIAN_POINT('Ctrl Pts',(-2.58159308632968,2.52458961892987,
-6.99724979130256));
#107244=CARTESIAN_POINT('Ctrl Pts',(-2.56708381281763,2.51818504847661,
-6.95814651287555));
#107245=CARTESIAN_POINT('Ctrl Pts',(-2.53813493563216,2.5050621488739,-6.88001759932194));
#107246=CARTESIAN_POINT('Ctrl Pts',(-2.52367872523227,2.49833629948252,
-6.84094715263981));
#107247=CARTESIAN_POINT('Ctrl Pts',(-2.50926086955057,2.49144078078428,
-6.80191958696967));
#107248=CARTESIAN_POINT('Ctrl Pts',(-2.358969622,2.490655005,-7.11935828));
#107249=CARTESIAN_POINT('Ctrl Pts',(-2.748737092,2.556411293,-6.990210457));
#107250=CARTESIAN_POINT('Ctrl Pts',(-3.122076251,2.621296797,-6.819284411));
#107251=CARTESIAN_POINT('Ctrl Pts',(-2.504810268,2.490655005,-6.803559768));
#107252=CARTESIAN_POINT('Ctrl Pts',(-2.877288541,2.556411293,-6.666427527));
#107253=CARTESIAN_POINT('Ctrl Pts',(-3.232570193,2.621296797,-6.48945220700001));
#107254=CARTESIAN_POINT('Origin',(0.0548469433709137,2.41076919432706,0.187469768850078));
#107255=CARTESIAN_POINT('Ctrl Pts',(-3.53842107017982,2.62578637453734,
-6.61348232156691));
#107256=CARTESIAN_POINT('Ctrl Pts',(-3.55074890599494,2.62354158576867,
-6.60682718819617));
#107257=CARTESIAN_POINT('Ctrl Pts',(-3.56307674181012,2.621296797,-6.60017205482555));
#107258=CARTESIAN_POINT('Ctrl Pts',(-3.92174322298082,2.555986835,-6.40654737458525));
#107259=CARTESIAN_POINT('Ctrl Pts',(-4.25731568083912,2.49066265,-6.17519636984647));
#107260=CARTESIAN_POINT('Ctrl Pts',(-3.2083281275445,2.62578637453734,-6.50152782997209));
#107261=CARTESIAN_POINT('Ctrl Pts',(-3.22044916027223,2.62354158576867,
-6.49549001848606));
#107262=CARTESIAN_POINT('Ctrl Pts',(-3.232570193,2.621296797,-6.489452207));
#107263=CARTESIAN_POINT('Ctrl Pts',(-3.585219938,2.555986835,-6.313787911));
#107264=CARTESIAN_POINT('Ctrl Pts',(-3.916757348,2.49066265,-6.100943523));
#107265=CARTESIAN_POINT('Ctrl Pts',(-3.20503393312735,2.62578637453734,
-6.50041056930515));
#107266=CARTESIAN_POINT('Ctrl Pts',(-3.21715290204361,2.62354158576867,
-6.49437891844269));
#107267=CARTESIAN_POINT('Ctrl Pts',(-3.22927187096,2.621296797,-6.48834726758));
#107268=CARTESIAN_POINT('Ctrl Pts',(-3.58186157136,2.555986835,-6.31286220897));
#107269=CARTESIAN_POINT('Ctrl Pts',(-3.91335871321,2.49066265,-6.10020250954));
#107270=CARTESIAN_POINT('',(-3.91280738900435,2.49144077992664,-6.10347757543066));
#107271=CARTESIAN_POINT('Origin',(0.0988877438209256,2.55357123314395,0.173340571503654));
#107272=CARTESIAN_POINT('Ctrl Pts',(-4.04802915756938,2.5308420210067,-6.31375165296533));
#107273=CARTESIAN_POINT('Ctrl Pts',(-4.02543870508658,2.52458960847576,
-6.27869171914355));
#107274=CARTESIAN_POINT('Ctrl Pts',(-4.00286262173711,2.51818504343692,
-6.24362175005694));
#107275=CARTESIAN_POINT('Ctrl Pts',(-3.95779516364708,2.50506214893107,
-6.17354262673062));
#107276=CARTESIAN_POINT('Ctrl Pts',(-3.93527794006458,2.49833629948923,
-6.13849328278224));
#107277=CARTESIAN_POINT('Ctrl Pts',(-3.91280739300335,2.49144078084299,
-6.10347757268393));
#107278=CARTESIAN_POINT('Ctrl Pts',(-3.834269807,2.490655005,-6.445802902));
#107279=CARTESIAN_POINT('Ctrl Pts',(-4.187161766,2.556411293,-6.235885999));
#107280=CARTESIAN_POINT('Ctrl Pts',(-4.515028415,2.621296797,-5.98869922500001));
#107281=CARTESIAN_POINT('Ctrl Pts',(-3.908813434,2.490655005,-6.106036156));
#107282=CARTESIAN_POINT('Ctrl Pts',(-4.243103994,2.556411293,-5.892038171));
#107283=CARTESIAN_POINT('Ctrl Pts',(-4.55203489600001,2.621296797,-5.642825383));
#107284=CARTESIAN_POINT('Origin',(0.0938651415814157,2.41076919440569,0.171296399202997));
#107285=CARTESIAN_POINT('Ctrl Pts',(-4.87739795608349,2.62578637477553,
-5.69820684568798));
#107286=CARTESIAN_POINT('Ctrl Pts',(-4.88800691759883,2.62354158588777,
-5.68905718488216));
#107287=CARTESIAN_POINT('Ctrl Pts',(-4.89861587911403,2.621296797,-5.67990752407633));
#107288=CARTESIAN_POINT('Ctrl Pts',(-5.20727335563351,2.555986835,-5.41370699056624));
#107289=CARTESIAN_POINT('Ctrl Pts',(-5.48526668878452,2.49066265,-5.11562668380304));
#107290=CARTESIAN_POINT('Ctrl Pts',(-4.5309554974236,2.62578637477554,-5.65983001298165));
#107291=CARTESIAN_POINT('Ctrl Pts',(-4.54149519671181,2.62354158588777,
-5.65132769799085));
#107292=CARTESIAN_POINT('Ctrl Pts',(-4.552034896,2.621296797,-5.642825383));
#107293=CARTESIAN_POINT('Ctrl Pts',(-4.858677255,2.555986835,-5.39545875));
#107294=CARTESIAN_POINT('Ctrl Pts',(-5.136708253,2.49066265,-5.116319803));
#107295=CARTESIAN_POINT('Ctrl Pts',(-4.52749814143179,2.62578637477554,
-5.65944702767146));
#107296=CARTESIAN_POINT('Ctrl Pts',(-4.53803714951089,2.62354158588777,
-5.65095117293073));
#107297=CARTESIAN_POINT('Ctrl Pts',(-4.54857615759,2.621296797,-5.64245531819));
#107298=CARTESIAN_POINT('Ctrl Pts',(-4.85519840653001,2.555986835,-5.39527663992));
#107299=CARTESIAN_POINT('Ctrl Pts',(-5.13322978040999,2.49066265,-5.11632672005));
#107300=CARTESIAN_POINT('',(-5.13339538778399,2.49144077986205,-5.11964373418254));
#107301=CARTESIAN_POINT('Origin',(0.133838830789741,2.55357128992126,0.148029969099299));
#107302=CARTESIAN_POINT('Ctrl Pts',(-5.31065845768252,2.53084202101153,
-5.29593303788484));
#107303=CARTESIAN_POINT('Ctrl Pts',(-5.28105935724433,2.52458961887591,
-5.26654911421029));
#107304=CARTESIAN_POINT('Ctrl Pts',(-5.2514720567994,2.51818504843525,-5.23715222562454));
#107305=CARTESIAN_POINT('Ctrl Pts',(-5.19239328821142,2.50506214886337,
-5.17839966207316));
#107306=CARTESIAN_POINT('Ctrl Pts',(-5.1628679316371,2.49833629933328,-5.14901028953704));
#107307=CARTESIAN_POINT('Ctrl Pts',(-5.13339539093447,2.49144078066965,
-5.11964373083106));
#107308=CARTESIAN_POINT('Ctrl Pts',(-5.130283797,2.490655005,-5.470848943));
#107309=CARTESIAN_POINT('Ctrl Pts',(-5.429799409,2.556411293,-5.189978441));
#107310=CARTESIAN_POINT('Ctrl Pts',(-5.696862869,2.621296797,-4.878089119));
#107311=CARTESIAN_POINT('Ctrl Pts',(-5.130044829,2.490655005,-5.123001079));
#107312=CARTESIAN_POINT('Ctrl Pts',(-5.41051662,2.556411293,-4.84214366));
#107313=CARTESIAN_POINT('Ctrl Pts',(-5.658651506,2.621296797,-4.532346316));
#107314=CARTESIAN_POINT('Origin',(0.128494115922295,2.41076916488146,0.147113210000817));
#107315=CARTESIAN_POINT('Ctrl Pts',(-5.98831313732953,2.62578637459952,
-4.51648954957938));
#107316=CARTESIAN_POINT('Ctrl Pts',(-5.99670716025373,2.62354158579976,
-4.50527319005812));
#107317=CARTESIAN_POINT('Ctrl Pts',(-6.00510118317796,2.621296797,-4.49405683053693));
#107318=CARTESIAN_POINT('Ctrl Pts',(-6.2493171727924,2.555986835,-4.1677276835873));
#107319=CARTESIAN_POINT('Ctrl Pts',(-6.4567327218282,2.49066265,-3.81685598088725));
#107320=CARTESIAN_POINT('Ctrl Pts',(-5.64172042550917,2.62578637459952,
-4.55348483398021));
#107321=CARTESIAN_POINT('Ctrl Pts',(-5.65018596575455,2.62354158579976,
-4.54291557499014));
#107322=CARTESIAN_POINT('Ctrl Pts',(-5.658651506,2.621296797,-4.532346316));
#107323=CARTESIAN_POINT('Ctrl Pts',(-5.904948223,2.555986835,-4.224843934));
#107324=CARTESIAN_POINT('Ctrl Pts',(-6.116472389,2.49066265,-3.892462655));
#107325=CARTESIAN_POINT('Ctrl Pts',(-5.63826157005114,2.62578637459952,
-4.5538540319957));
#107326=CARTESIAN_POINT('Ctrl Pts',(-5.64672782401051,2.62354158579976,
-4.54329123080786));
#107327=CARTESIAN_POINT('Ctrl Pts',(-5.65519407797001,2.621296797,-4.53272842962));
#107328=CARTESIAN_POINT('Ctrl Pts',(-5.90151155978999,2.555986835,-4.22541393114));
#107329=CARTESIAN_POINT('Ctrl Pts',(-6.11307672812999,2.49066265,-3.89321717911));
#107330=CARTESIAN_POINT('',(-6.11395152353538,2.49144077987698,-3.89642104262899));
#107331=CARTESIAN_POINT('Origin',(0.162531914113915,2.55357126815225,0.115797771320377));
#107332=CARTESIAN_POINT('Ctrl Pts',(-6.3249672702921,2.53084202101672,-4.03048248028905));
#107333=CARTESIAN_POINT('Ctrl Pts',(-6.28974350540492,2.52458961887847,
-4.00814846808179));
#107334=CARTESIAN_POINT('Ctrl Pts',(-6.25452847761627,2.51818504844432,
-3.98579925744782));
#107335=CARTESIAN_POINT('Ctrl Pts',(-6.18420087352717,2.50506214887975,
-3.94112048507921));
#107336=CARTESIAN_POINT('Ctrl Pts',(-6.14904795691205,2.49833629931285,
-3.91876529849178));
#107337=CARTESIAN_POINT('Ctrl Pts',(-6.11395152592254,2.49144078066012,
-3.89642103863775));
#107338=CARTESIAN_POINT('Ctrl Pts',(-6.186411418,2.490655005,-4.240084169));
#107339=CARTESIAN_POINT('Ctrl Pts',(-6.418545666,2.556411293,-3.90139326));
#107340=CARTESIAN_POINT('Ctrl Pts',(-6.612318346,2.621296797,-3.539384988));
#107341=CARTESIAN_POINT('Ctrl Pts',(-6.111401029,2.490655005,-3.900420166));
#107342=CARTESIAN_POINT('Ctrl Pts',(-6.32493950200001,2.556411293,-3.565835892));
#107343=CARTESIAN_POINT('Ctrl Pts',(-6.500675861,2.621296797,-3.209939773));
#107344=CARTESIAN_POINT('Origin',(0.157115078729169,2.410769176666,0.116051396770692));
#107345=CARTESIAN_POINT('Ctrl Pts',(-6.81922145039121,2.62578637461624,
-3.12358622217615));
#107346=CARTESIAN_POINT('Ctrl Pts',(-6.8250080400054,2.62354158580812,-3.11082762807019));
#107347=CARTESIAN_POINT('Ctrl Pts',(-6.83079462961958,2.621296797,-3.09806903396429));
#107348=CARTESIAN_POINT('Ctrl Pts',(-6.99914986484065,2.555986835,-2.72687006272141));
#107349=CARTESIAN_POINT('Ctrl Pts',(-7.1262891087385,2.49066265,-2.3396133331402));
#107350=CARTESIAN_POINT('Ctrl Pts',(-6.48868477624709,2.62578637461624,
-3.23422376610269));
#107351=CARTESIAN_POINT('Ctrl Pts',(-6.49468031862353,2.62354158580812,
-3.22208176955133));
#107352=CARTESIAN_POINT('Ctrl Pts',(-6.500675861,2.621296797,-3.209939773));
#107353=CARTESIAN_POINT('Ctrl Pts',(-6.675110375,2.555986835,-2.856680112));
#107354=CARTESIAN_POINT('Ctrl Pts',(-6.810237074,2.49066265,-2.486598279));
#107355=CARTESIAN_POINT('Ctrl Pts',(-6.48538615356852,2.62578637461624,
-3.23532788416292));
#107356=CARTESIAN_POINT('Ctrl Pts',(-6.49138378120926,2.62354158580812,
-3.22319204100645));
#107357=CARTESIAN_POINT('Ctrl Pts',(-6.49738140885,2.621296797,-3.21105619785));
#107358=CARTESIAN_POINT('Ctrl Pts',(-6.6718765916,2.555986835,-2.85797556393));
#107359=CARTESIAN_POINT('Ctrl Pts',(-6.80708300218,2.49066265,-2.48806512947));
#107360=CARTESIAN_POINT('',(-6.80862608162008,2.4914407798974,-2.49100603347877));
#107361=CARTESIAN_POINT('Origin',(0.183624911732442,2.55357125500911,0.078150840754438));
#107362=CARTESIAN_POINT('Ctrl Pts',(-7.04352764352837,2.53084202101004,
-2.57657104078789));
#107363=CARTESIAN_POINT('Ctrl Pts',(-7.0043261726185,2.52458960840355,-2.56233122981495));
#107364=CARTESIAN_POINT('Ctrl Pts',(-6.96513006845,2.51818504338796,-2.54807473423963));
#107365=CARTESIAN_POINT('Ctrl Pts',(-6.88684209941904,2.50506214888574,
-2.51955889384003));
#107366=CARTESIAN_POINT('Ctrl Pts',(-6.8477053345953,2.4983362994034,-2.50528319728224));
#107367=CARTESIAN_POINT('Ctrl Pts',(-6.80862608309262,2.49144078072764,
-2.49100602904715));
#107368=CARTESIAN_POINT('Ctrl Pts',(-6.953269318,2.490655005,-2.811057772));
#107369=CARTESIAN_POINT('Ctrl Pts',(-7.107167862,2.556411293,-2.430383266));
#107370=CARTESIAN_POINT('Ctrl Pts',(-7.218589166,2.621296797,-2.035183148));
#107371=CARTESIAN_POINT('Ctrl Pts',(-6.806994909,2.490655005,-2.49545994));
#107372=CARTESIAN_POINT('Ctrl Pts',(-6.943615243,2.556411293,-2.122793602));
#107373=CARTESIAN_POINT('Ctrl Pts',(-7.038735838,2.621296797,-1.737440013));
#107374=CARTESIAN_POINT('Origin',(0.178389307057937,2.41076914731909,0.0795630440553063));
#107375=CARTESIAN_POINT('Ctrl Pts',(-7.33127054800828,2.6257863745359,-1.5846274748125));
#107376=CARTESIAN_POINT('Ctrl Pts',(-7.33417912971875,2.62354158576795,
-1.57092322405954));
#107377=CARTESIAN_POINT('Ctrl Pts',(-7.33708771142923,2.621296797,-1.55721897330657));
#107378=CARTESIAN_POINT('Ctrl Pts',(-7.42171008824151,2.555986835,-1.15850702824784));
#107379=CARTESIAN_POINT('Ctrl Pts',(-7.46262813804136,2.49066265,-0.752972966339287));
#107380=CARTESIAN_POINT('Ctrl Pts',(-7.03224543889095,2.6257863745359,-1.76373398808824));
#107381=CARTESIAN_POINT('Ctrl Pts',(-7.03549063844555,2.62354158576795,
-1.75058700054412));
#107382=CARTESIAN_POINT('Ctrl Pts',(-7.038735838,2.621296797,-1.737440013));
#107383=CARTESIAN_POINT('Ctrl Pts',(-7.133151786,2.555986835,-1.354941103));
#107384=CARTESIAN_POINT('Ctrl Pts',(-7.18556264200001,2.49066265,-0.964463331));
#107385=CARTESIAN_POINT('Ctrl Pts',(-7.0292612889204,2.6257863745359,-1.76552139884411));
#107386=CARTESIAN_POINT('Ctrl Pts',(-7.03250984778524,2.62354158576795,
-1.75237997256209));
#107387=CARTESIAN_POINT('Ctrl Pts',(-7.03575840664999,2.621296797,-1.73923854628));
#107388=CARTESIAN_POINT('Ctrl Pts',(-7.13027209054,2.555986835,-1.35690143583));
#107389=CARTESIAN_POINT('Ctrl Pts',(-7.18279764011001,2.49066265,-0.96657391953));
#107390=CARTESIAN_POINT('',(-7.1849368512499,2.49144077995398,-0.969114350955572));
#107391=CARTESIAN_POINT('Origin',(0.196132190812308,2.55357125277221,0.036849830138366));
#107392=CARTESIAN_POINT('Ctrl Pts',(-7.43274049243919,2.53084202102401,
-1.0021820033146));
#107393=CARTESIAN_POINT('Ctrl Pts',(-7.39139439192935,2.52458960846359,
-0.996702268783386));
#107394=CARTESIAN_POINT('Ctrl Pts',(-7.35004994567745,2.51818504345243,
-0.991205086004076));
#107395=CARTESIAN_POINT('Ctrl Pts',(-7.26746224275289,2.50506214895304,
-0.980185529411156));
#107396=CARTESIAN_POINT('Ctrl Pts',(-7.22617162141718,2.49833629958382,
-0.97465683841716));
#107397=CARTESIAN_POINT('Ctrl Pts',(-7.18493685170376,2.49144078092553,
-0.969114346370235));
#107398=CARTESIAN_POINT('Ctrl Pts',(-7.39500007200001,2.490655005,-1.250589437));
#107399=CARTESIAN_POINT('Ctrl Pts',(-7.463466788,2.556411293,-0.845731252));
#107400=CARTESIAN_POINT('Ctrl Pts',(-7.48732678,2.621296797,-0.435818406));
#107401=CARTESIAN_POINT('Ctrl Pts',(-7.184301272,2.490655005,-0.973814782));
#107402=CARTESIAN_POINT('Ctrl Pts',(-7.237615252,2.556411293,-0.580491841));
#107403=CARTESIAN_POINT('Ctrl Pts',(-7.24767235,2.621296797,-0.18369949));
#107404=CARTESIAN_POINT('Origin',(0.191322602224666,2.4107692487785,0.0393544752637704));
#107405=CARTESIAN_POINT('Ctrl Pts',(-7.50051758257422,2.62578637468215,
0.0284266915779838));
#107406=CARTESIAN_POINT('Ctrl Pts',(-7.50041215445485,2.62354158584108,
0.0424358040812995));
#107407=CARTESIAN_POINT('Ctrl Pts',(-7.50030672633549,2.621296797,0.0564449165846143));
#107408=CARTESIAN_POINT('Ctrl Pts',(-7.49723939708654,2.555986835,0.464026506667262));
#107409=CARTESIAN_POINT('Ctrl Pts',(-7.4500229692408,2.49066265,0.86887557847777));
#107410=CARTESIAN_POINT('Ctrl Pts',(-7.24698612022987,2.62578637468215,
-0.210773971470443));
#107411=CARTESIAN_POINT('Ctrl Pts',(-7.24732923511492,2.62354158584108,
-0.197236730735224));
#107412=CARTESIAN_POINT('Ctrl Pts',(-7.24767235000001,2.621296797,-0.18369949));
#107413=CARTESIAN_POINT('Ctrl Pts',(-7.257654946,2.555986835,0.210153447));
#107414=CARTESIAN_POINT('Ctrl Pts',(-7.224899287,2.49066265,0.60276885));
#107415=CARTESIAN_POINT('Ctrl Pts',(-7.24445597850344,2.62578637468215,
-0.213161097600633));
#107416=CARTESIAN_POINT('Ctrl Pts',(-7.24480356966667,2.62354158584108,
-0.199628565955319));
#107417=CARTESIAN_POINT('Ctrl Pts',(-7.24515116083001,2.621296797,-0.18609603431));
#107418=CARTESIAN_POINT('Ctrl Pts',(-7.25526398982,2.555986835,0.20761989627));
#107419=CARTESIAN_POINT('Ctrl Pts',(-7.22265264346,2.49066265,0.60011321219));
#107420=CARTESIAN_POINT('',(-7.22528795887604,2.49144077931082,0.598092041708296));
#107421=CARTESIAN_POINT('Origin',(0.199468459704493,2.55357127355161,-0.00617432263186217));
#107422=CARTESIAN_POINT('Ctrl Pts',(-7.4744066565912,2.53084202101378,0.619067950003639));
#107423=CARTESIAN_POINT('Ctrl Pts',(-7.43284929343279,2.52458961890745,
0.615531388015672));
#107424=CARTESIAN_POINT('Ctrl Pts',(-7.3912896880179,2.51818504849757,0.612012212856936));
#107425=CARTESIAN_POINT('Ctrl Pts',(-7.30826392881563,2.50506214895256,
0.605020221165677));
#107426=CARTESIAN_POINT('Ctrl Pts',(-7.26675015383567,2.49833629953379,
0.60154339156249));
#107427=CARTESIAN_POINT('Ctrl Pts',(-7.22528795819245,2.49144078086637,
0.598092046812624));
#107428=CARTESIAN_POINT('Ctrl Pts',(-7.490948841,2.490655005,0.36835507));
#107429=CARTESIAN_POINT('Ctrl Pts',(-7.470782301,2.556411293,0.778466215));
#107430=CARTESIAN_POINT('Ctrl Pts',(-7.405965316,2.621296797,1.18392472));
#107431=CARTESIAN_POINT('Ctrl Pts',(-7.225677693,2.490655005,0.593364874000001));
#107432=CARTESIAN_POINT('Ctrl Pts',(-7.19319241600001,2.556411293,0.988953072));
#107433=CARTESIAN_POINT('Ctrl Pts',(-7.117715759,2.621296797,1.378630618));
#107434=CARTESIAN_POINT('Origin',(0.19530968465359,2.41076918195982,-0.00269430202695181));
#107435=CARTESIAN_POINT('Ctrl Pts',(-7.31904875066757,2.6257863747346,1.64015165671534));
#107436=CARTESIAN_POINT('Ctrl Pts',(-7.31593424229251,2.6235415858673,1.65381058023396));
#107437=CARTESIAN_POINT('Ctrl Pts',(-7.31281973391756,2.621296797,1.66746950375251));
#107438=CARTESIAN_POINT('Ctrl Pts',(-7.2222061236215,2.555986835,2.06486267909892));
#107439=CARTESIAN_POINT('Ctrl Pts',(-7.08906300674665,2.49066265,2.45009646767005));
#107440=CARTESIAN_POINT('Ctrl Pts',(-7.12286578617508,2.6257863747346,1.35204160345207));
#107441=CARTESIAN_POINT('Ctrl Pts',(-7.1202907725876,2.6235415858673,1.36533611072604));
#107442=CARTESIAN_POINT('Ctrl Pts',(-7.117715759,2.621296797,1.378630618));
#107443=CARTESIAN_POINT('Ctrl Pts',(-7.04279822799999,2.555986835,1.765421455));
#107444=CARTESIAN_POINT('Ctrl Pts',(-6.926407672,2.49066265,2.141816229));
#107445=CARTESIAN_POINT('Ctrl Pts',(-7.12090795932432,2.6257863747346,1.34916638133631));
#107446=CARTESIAN_POINT('Ctrl Pts',(-7.11833832967726,2.6235415858673,1.36245725188317));
#107447=CARTESIAN_POINT('Ctrl Pts',(-7.11576870003,2.621296797,1.37574812243));
#107448=CARTESIAN_POINT('Ctrl Pts',(-7.04100780956999,2.555986835,1.76243315237));
#107449=CARTESIAN_POINT('Ctrl Pts',(-6.92478443737,2.49066265,2.13873971657));
#107450=CARTESIAN_POINT('',(-6.9277926318589,2.49144077988269,2.137332315355));
#107451=CARTESIAN_POINT('Origin',(0.193477601861138,2.55357126352284,-0.048909767983537));
#107452=CARTESIAN_POINT('Ctrl Pts',(-7.16657787288143,2.5308420210282,2.2113709751042));
#107453=CARTESIAN_POINT('Ctrl Pts',(-7.12675228698287,2.52458960837003,
2.19898347034696));
#107454=CARTESIAN_POINT('Ctrl Pts',(-7.08692087679801,2.51818504336427,
2.18661249604038));
#107455=CARTESIAN_POINT('Ctrl Pts',(-7.00733931618786,2.5050621488743,2.16193589866133));
#107456=CARTESIAN_POINT('Ctrl Pts',(-6.96754352551645,2.49833629938396,
2.14961612077613));
#107457=CARTESIAN_POINT('Ctrl Pts',(-6.92779263023784,2.49144078071947,
2.13733232013111));
#107458=CARTESIAN_POINT('Ctrl Pts',(-7.236629169,2.490655005,1.970075703));
#107459=CARTESIAN_POINT('Ctrl Pts',(-7.128772338,2.556411293,2.366263468));
#107460=CARTESIAN_POINT('Ctrl Pts',(-6.978309144,2.621296797,2.748308842));
#107461=CARTESIAN_POINT('Ctrl Pts',(-6.929189456,2.490655005,2.132799448));
#107462=CARTESIAN_POINT('Ctrl Pts',(-6.812423898,2.556411293,2.512155639));
#107463=CARTESIAN_POINT('Ctrl Pts',(-6.654942689,2.621296797,2.87649749));
#107464=CARTESIAN_POINT('Origin',(0.190164101466889,2.41076917337337,-0.0446170585626998));
#107465=CARTESIAN_POINT('Ctrl Pts',(-6.79534933510274,2.62578637467629,
3.17518495546536));
#107466=CARTESIAN_POINT('Ctrl Pts',(-6.78937137745835,2.62354158583815,
3.18785501350895));
#107467=CARTESIAN_POINT('Ctrl Pts',(-6.78339341981399,2.621296797,3.20052507155255));
#107468=CARTESIAN_POINT('Ctrl Pts',(-6.60947051893525,2.555986835,3.56914816665374));
#107469=CARTESIAN_POINT('Ctrl Pts',(-6.39662633629009,2.49066265,3.91675356870698));
#107470=CARTESIAN_POINT('Ctrl Pts',(-6.66568816340674,2.62578637467629,
2.85163721580644));
#107471=CARTESIAN_POINT('Ctrl Pts',(-6.6603154262033,2.62354158583815,2.86406735290325));
#107472=CARTESIAN_POINT('Ctrl Pts',(-6.65494268900001,2.621296797,2.87649749));
#107473=CARTESIAN_POINT('Ctrl Pts',(-6.498628092,2.555986835,3.238140317));
#107474=CARTESIAN_POINT('Ctrl Pts',(-6.304044932,2.49066265,3.580714662));
#107475=CARTESIAN_POINT('Ctrl Pts',(-6.66439419721497,2.62578637467629,
2.84840833987498));
#107476=CARTESIAN_POINT('Ctrl Pts',(-6.65902749986742,2.62354158583815,
2.86083608265752));
#107477=CARTESIAN_POINT('Ctrl Pts',(-6.65366080252,2.621296797,2.87326382544));
#107478=CARTESIAN_POINT('Ctrl Pts',(-6.49752192928999,2.555986835,3.23483699218));
#107479=CARTESIAN_POINT('Ctrl Pts',(-6.30312100693,2.49066265,3.57736112926));
#107480=CARTESIAN_POINT('',(-6.30636142167443,2.49144077994544,3.57663330547932));
#107481=CARTESIAN_POINT('Origin',(0.178440093734786,2.55357123951412,-0.0893582737754317));
#107482=CARTESIAN_POINT('Ctrl Pts',(-6.52364787265427,2.53084202104553,
3.70027275048277));
#107483=CARTESIAN_POINT('Ctrl Pts',(-6.48741633343293,2.5245896082618,3.67961353455242));
#107484=CARTESIAN_POINT('Ctrl Pts',(-6.45117555386211,2.5181850433564,3.65896921127779));
#107485=CARTESIAN_POINT('Ctrl Pts',(-6.37875930532489,2.5050621489458,3.61776185602896));
#107486=CARTESIAN_POINT('Ctrl Pts',(-6.34254230674421,2.4983362995596,3.59717518928135));
#107487=CARTESIAN_POINT('Ctrl Pts',(-6.30636141925216,2.49144078088254,
3.57663330943117));
#107488=CARTESIAN_POINT('Ctrl Pts',(-6.643932759,2.490655005,3.479677786));
#107489=CARTESIAN_POINT('Ctrl Pts',(-6.453428903,2.556411293,3.84341687));
#107490=CARTESIAN_POINT('Ctrl Pts',(-6.224354992,2.621296797,4.184185097));
#107491=CARTESIAN_POINT('Ctrl Pts',(-6.308700021,2.490655005,3.572506689));
#107492=CARTESIAN_POINT('Ctrl Pts',(-6.113114009,2.556411293,3.9178926));
#107493=CARTESIAN_POINT('Ctrl Pts',(-5.880991895,2.621296797,4.239862537));
#107494=CARTESIAN_POINT('Origin',(0.176126986800866,2.41076917395093,-0.0844537108595922));
#107495=CARTESIAN_POINT('Ctrl Pts',(-5.95390693584867,2.62578637476293,
4.56175013253003));
#107496=CARTESIAN_POINT('Ctrl Pts',(-5.94534505143132,2.62354158588146,
4.57283888770188));
#107497=CARTESIAN_POINT('Ctrl Pts',(-5.93678316701407,2.621296797,4.58392764287384));
#107498=CARTESIAN_POINT('Ctrl Pts',(-5.68768341845483,2.555986835,4.90654425278669));
#107499=CARTESIAN_POINT('Ctrl Pts',(-5.40509052821108,2.49066265,5.20026762634116));
#107500=CARTESIAN_POINT('Ctrl Pts',(-5.89683037055794,2.62578637476292,
4.2178934411378));
#107501=CARTESIAN_POINT('Ctrl Pts',(-5.88891113277903,2.62354158588146,
4.22887798906888));
#107502=CARTESIAN_POINT('Ctrl Pts',(-5.880991895,2.621296797,4.239862537));
#107503=CARTESIAN_POINT('Ctrl Pts',(-5.650589329,2.555986835,4.559447338));
#107504=CARTESIAN_POINT('Ctrl Pts',(-5.386912058,2.49066265,4.852182858));
#107505=CARTESIAN_POINT('Ctrl Pts',(-5.89626076945952,2.62578637476292,
4.21446189006023));
#107506=CARTESIAN_POINT('Ctrl Pts',(-5.88834794503479,2.62354158588146,
4.22544539804511));
#107507=CARTESIAN_POINT('Ctrl Pts',(-5.88043512061,2.621296797,4.23642890603));
#107508=CARTESIAN_POINT('Ctrl Pts',(-5.65021914495,2.555986835,4.5559834508));
#107509=CARTESIAN_POINT('Ctrl Pts',(-5.38673064420001,2.49066265,4.84870911242));
#107510=CARTESIAN_POINT('',(-5.39005175947313,2.49144077988329,4.848694897278));
#107511=CARTESIAN_POINT('Origin',(0.155058782873332,2.55357125459944,-0.125628383699805));
#107512=CARTESIAN_POINT('Ctrl Pts',(-5.57567934822786,2.53084202100795,
5.01615388492042));
#107513=CARTESIAN_POINT('Ctrl Pts',(-5.54473600627949,2.52458960887614,
4.98818896292234));
#107514=CARTESIAN_POINT('Ctrl Pts',(-5.51378043344695,2.51818504360533,
4.96023659441289));
#107515=CARTESIAN_POINT('Ctrl Pts',(-5.45191559857526,2.50506214888001,
4.90442529013533));
#107516=CARTESIAN_POINT('Ctrl Pts',(-5.42097085769936,2.49833629937661,
4.8765343436698));
#107517=CARTESIAN_POINT('Ctrl Pts',(-5.39005175646082,2.49144078071805,
4.84869490041678));
#107518=CARTESIAN_POINT('Ctrl Pts',(-5.740573438,2.490655005,4.826574003));
#107519=CARTESIAN_POINT('Ctrl Pts',(-5.476330305,2.556411293,5.140856372));
#107520=CARTESIAN_POINT('Ctrl Pts',(-5.179356919,2.621296797,5.424413508));
#107521=CARTESIAN_POINT('Ctrl Pts',(-5.393222785,2.490655005,4.845167489));
#107522=CARTESIAN_POINT('Ctrl Pts',(-5.12796170400001,2.556411293,5.140433258));
#107523=CARTESIAN_POINT('Ctrl Pts',(-4.832052457,2.621296797,5.404976323));
#107524=CARTESIAN_POINT('Origin',(0.153854054401565,2.41076917057774,-0.120341188345526));
#107525=CARTESIAN_POINT('Ctrl Pts',(-4.83406646628012,2.62578637475954,
5.73501294467684));
#107526=CARTESIAN_POINT('Ctrl Pts',(-4.82332099939218,2.62354158587977,
5.74400189885379));
#107527=CARTESIAN_POINT('Ctrl Pts',(-4.81257553250423,2.621296797,5.75299085303078));
#107528=CARTESIAN_POINT('Ctrl Pts',(-4.49994656305008,2.555986835,6.01451578350814));
#107529=CARTESIAN_POINT('Ctrl Pts',(-4.16081869483508,2.49066265,6.24062295031996));
#107530=CARTESIAN_POINT('Ctrl Pts',(-4.8522433440357,2.62578637475954,5.38692565646089));
#107531=CARTESIAN_POINT('Ctrl Pts',(-4.84214790051785,2.62354158587977,
5.39595098973051));
#107532=CARTESIAN_POINT('Ctrl Pts',(-4.832052457,2.621296797,5.404976323));
#107533=CARTESIAN_POINT('Ctrl Pts',(-4.538335289,2.555986835,5.667559668));
#107534=CARTESIAN_POINT('Ctrl Pts',(-4.217893162,2.49066265,5.896768375));
#107535=CARTESIAN_POINT('Ctrl Pts',(-4.85242474194361,2.62578637475954,
5.38345188573355));
#107536=CARTESIAN_POINT('Ctrl Pts',(-4.84233578539682,2.62354158587977,
5.39247758205185));
#107537=CARTESIAN_POINT('Ctrl Pts',(-4.83224682884999,2.621296797,5.40150327837001));
#107538=CARTESIAN_POINT('Ctrl Pts',(-4.538718393,2.555986835,5.66409718592));
#107539=CARTESIAN_POINT('Ctrl Pts',(-4.21846274216001,2.49066265,5.89333684504));
#107540=CARTESIAN_POINT('',(-4.22170926802651,2.49144077988097,5.89403690448083));
#107541=CARTESIAN_POINT('Origin',(0.1244271772488,2.55357125499674,-0.156024291756064));
#107542=CARTESIAN_POINT('Ctrl Pts',(-4.36699825526782,2.53084202105966,
6.09748523879666));
#107543=CARTESIAN_POINT('Ctrl Pts',(-4.34279002162134,2.52458961891928,
6.06352227161413));
#107544=CARTESIAN_POINT('Ctrl Pts',(-4.318567084774,2.5181850484725,6.02956885146575));
#107545=CARTESIAN_POINT('Ctrl Pts',(-4.27014637778942,2.50506214891138,
5.96176324873251));
#107546=CARTESIAN_POINT('Ctrl Pts',(-4.24592083658121,2.49833629941155,
5.92787217255079));
#107547=CARTESIAN_POINT('Ctrl Pts',(-4.22170926388744,2.49144078076664,
5.89403690726214));
#107548=CARTESIAN_POINT('Ctrl Pts',(-4.568791283,2.490655005,5.947784984));
#107549=CARTESIAN_POINT('Ctrl Pts',(-4.243164588,2.556411293,6.197915143));
#107550=CARTESIAN_POINT('Ctrl Pts',(-3.892177873,2.621296797,6.411002371));
#107551=CARTESIAN_POINT('Ctrl Pts',(-4.225564445,2.490655005,5.891273642));
#107552=CARTESIAN_POINT('Ctrl Pts',(-3.903031608,2.556411293,6.12261297));
#107553=CARTESIAN_POINT('Ctrl Pts',(-3.557171616,2.621296797,6.317359424));
#107554=CARTESIAN_POINT('Origin',(0.124387267833697,2.41076918495438,-0.150601809272185));
#107555=CARTESIAN_POINT('Ctrl Pts',(-3.48819042137609,2.6257863746852,6.64011292507194));
#107556=CARTESIAN_POINT('Ctrl Pts',(-3.47576381827505,2.6235415858426,6.64658176465048));
#107557=CARTESIAN_POINT('Ctrl Pts',(-3.463337215174,2.621296797,6.65305060422905));
#107558=CARTESIAN_POINT('Ctrl Pts',(-3.10179720708206,2.555986835,6.84125524024733));
#107559=CARTESIAN_POINT('Ctrl Pts',(-2.72199160358742,2.49066265,6.98917368021648));
#107560=CARTESIAN_POINT('Ctrl Pts',(-3.58077081065142,2.62578637468521,
6.30407121606756));
#107561=CARTESIAN_POINT('Ctrl Pts',(-3.56897121332571,2.6235415858426,6.31071532003383));
#107562=CARTESIAN_POINT('Ctrl Pts',(-3.557171616,2.621296797,6.317359424));
#107563=CARTESIAN_POINT('Ctrl Pts',(-3.213873735,2.555986835,6.51066320800001));
#107564=CARTESIAN_POINT('Ctrl Pts',(-2.851650271,2.49066265,6.66562755700001));
#107565=CARTESIAN_POINT('Ctrl Pts',(-3.58169472559192,2.62578637468521,
6.30071765536171));
#107566=CARTESIAN_POINT('Ctrl Pts',(-3.56990138553099,2.6235415858426,6.30736350839596));
#107567=CARTESIAN_POINT('Ctrl Pts',(-3.55810804547,2.621296797,6.31400936143));
#107568=CARTESIAN_POINT('Ctrl Pts',(-3.21499221354,2.555986835,6.50736403287));
#107569=CARTESIAN_POINT('Ctrl Pts',(-2.8529442122,2.49066265,6.6623986972));
#107570=CARTESIAN_POINT('',(-2.85596434332632,2.49144077993471,6.66378029754127));
#107571=CARTESIAN_POINT('Origin',(0.0879774927781977,2.55357123324615,-0.17912462577321));
#107572=CARTESIAN_POINT('Ctrl Pts',(-2.9541211766701,2.53084202101462,6.89370495986537));
#107573=CARTESIAN_POINT('Ctrl Pts',(-2.93777995225721,2.52458961891118,
6.85533197352984));
#107574=CARTESIAN_POINT('Ctrl Pts',(-2.9214223160308,2.51818504848243,6.81696515014835));
#107575=CARTESIAN_POINT('Ctrl Pts',(-2.88870985871748,2.50506214891889,
6.74033578394755));
#107576=CARTESIAN_POINT('Ctrl Pts',(-2.87233627702697,2.49833629948779,
6.70202928740089));
#107577=CARTESIAN_POINT('Ctrl Pts',(-2.85596433928416,2.49144078079788,
6.66378029911584));
#107578=CARTESIAN_POINT('Ctrl Pts',(-3.183377525,2.490655005,6.79088415));
#107579=CARTESIAN_POINT('Ctrl Pts',(-2.811593211,2.556411293,6.965166291));
#107580=CARTESIAN_POINT('Ctrl Pts',(-2.423004915,2.621296797,7.097819889));
#107581=CARTESIAN_POINT('Ctrl Pts',(-2.860323408,2.490655005,6.661910387));
#107582=CARTESIAN_POINT('Ctrl Pts',(-2.495600093,2.556411293,6.818506104));
#107583=CARTESIAN_POINT('Ctrl Pts',(-2.115961384,2.621296797,6.93434982));
#107584=CARTESIAN_POINT('Origin',(0.0891042866592537,2.41076916744523,-0.173820589646979));
#107585=CARTESIAN_POINT('Ctrl Pts',(-1.9792104682936,2.6257863746344,7.23472860556905));
#107586=CARTESIAN_POINT('Ctrl Pts',(-1.96568378315313,2.6235415858172,7.2383748548763));
#107587=CARTESIAN_POINT('Ctrl Pts',(-1.95215709801272,2.621296797,7.24202110418352));
#107588=CARTESIAN_POINT('Ctrl Pts',(-1.5586112616565,2.555986835,7.34810520522353));
#107589=CARTESIAN_POINT('Ctrl Pts',(-1.15588720928485,2.49066265,7.41091841655395));
#107590=CARTESIAN_POINT('Ctrl Pts',(-2.14186541422032,2.6257863746344,6.92644541242964));
#107591=CARTESIAN_POINT('Ctrl Pts',(-2.12891339911013,2.6235415858172,6.93039761621488));
#107592=CARTESIAN_POINT('Ctrl Pts',(-2.115961384,2.621296797,6.93434982));
#107593=CARTESIAN_POINT('Ctrl Pts',(-1.739135017,2.555986835,7.049335371));
#107594=CARTESIAN_POINT('Ctrl Pts',(-1.352067382,2.49066265,7.122809403));
#107595=CARTESIAN_POINT('Ctrl Pts',(-2.14348864497014,2.6257863746344,6.92336887051507));
#107596=CARTESIAN_POINT('Ctrl Pts',(-2.13054236483504,2.6235415858172,6.9273241276026));
#107597=CARTESIAN_POINT('Ctrl Pts',(-2.1175960847,2.621296797,6.93127938469));
#107598=CARTESIAN_POINT('Ctrl Pts',(-1.74093657126,2.555986835,7.04635376857));
#107599=CARTESIAN_POINT('Ctrl Pts',(-1.35402518099,2.49066265,7.11993419126));
#107600=CARTESIAN_POINT('',(-1.35667770051763,2.49144077987293,7.1219327287485));
#107601=CARTESIAN_POINT('Origin',(0.0474141679670559,2.5535712289894,-0.19384950688544));
#107602=CARTESIAN_POINT('Ctrl Pts',(-1.40311267532108,2.53084202106957,
7.36758269842034));
#107603=CARTESIAN_POINT('Ctrl Pts',(-1.39540254430667,2.52458960834639,
7.32659390134295));
#107604=CARTESIAN_POINT('Ctrl Pts',(-1.38767508043641,2.51818504337406,
7.2856077020964));
#107605=CARTESIAN_POINT('Ctrl Pts',(-1.37220047685122,2.50506214890662,
7.2037377083547));
#107606=CARTESIAN_POINT('Ctrl Pts',(-1.36444446486421,2.49833629945179,
7.16280696022082));
#107607=CARTESIAN_POINT('Ctrl Pts',(-1.35667769591991,2.49144078077239,
7.1219327294704));
#107608=CARTESIAN_POINT('Ctrl Pts',(-1.649112573,2.490655005,7.31644912000001));
#107609=CARTESIAN_POINT('Ctrl Pts',(-1.248554861,2.556411293,7.406734004));
#107610=CARTESIAN_POINT('Ctrl Pts',(-0.840534941,2.621296797,7.45275123800001));
#107611=CARTESIAN_POINT('Ctrl Pts',(-1.361336828,2.490655005,7.121043606));
#107612=CARTESIAN_POINT('Ctrl Pts',(-0.971477090999999,2.556411293,7.195573471));
#107613=CARTESIAN_POINT('Ctrl Pts',(-0.575811149,2.621296797,7.227097725));
#107614=CARTESIAN_POINT('Origin',(0.0496547889975075,2.4107691558232,-0.188911435488969));
#107615=CARTESIAN_POINT('Ctrl Pts',(-0.377684835313728,2.62578637475243,
7.49105641693586));
#107616=CARTESIAN_POINT('Ctrl Pts',(-0.363690560360698,2.62354158587621,
7.49170958152756));
#107617=CARTESIAN_POINT('Ctrl Pts',(-0.349696285407675,2.621296797,7.49236274611938));
#107618=CARTESIAN_POINT('Ctrl Pts',(0.0574536141148712,2.555986835,7.51136593841204));
#107619=CARTESIAN_POINT('Ctrl Pts',(0.464265185679254,2.49066265,7.48613684418663));
#107620=CARTESIAN_POINT('Ctrl Pts',(-0.602808772041866,2.62578637475243,
7.22494671878989));
#107621=CARTESIAN_POINT('Ctrl Pts',(-0.589309960520928,2.62354158587621,
7.226022221895));
#107622=CARTESIAN_POINT('Ctrl Pts',(-0.575811149000001,2.621296797,7.227097725));
#107623=CARTESIAN_POINT('Ctrl Pts',(-0.183076279,2.555986835,7.258388448));
#107624=CARTESIAN_POINT('Ctrl Pts',(0.210736675,2.49066265,7.246936598));
#107625=CARTESIAN_POINT('Ctrl Pts',(-0.60505541812148,2.62578637475243,
7.2222910513438));
#107626=CARTESIAN_POINT('Ctrl Pts',(-0.591561551125732,2.62354158587621,
7.22337076921702));
#107627=CARTESIAN_POINT('Ctrl Pts',(-0.57806768413,2.621296797,7.22445048709));
#107628=CARTESIAN_POINT('Ctrl Pts',(-0.18547667031,2.555986835,7.25586383469));
#107629=CARTESIAN_POINT('Ctrl Pts',(0.20820656273,2.49066265,7.24454947603));
#107630=CARTESIAN_POINT('Origin',(0.00463374273099309,2.55357126605449,
-0.199509935815785));
#107631=CARTESIAN_POINT('Ctrl Pts',(-1.34892079,3.267335925,7.123405976));
#107632=CARTESIAN_POINT('Ctrl Pts',(-0.962430673,3.331598135,7.19659351500001));
#107633=CARTESIAN_POINT('Ctrl Pts',(-0.57029087,3.396744076,7.227535425));
#107634=CARTESIAN_POINT('Ctrl Pts',(-1.153013899,3.267335925,7.410840637));
#107635=CARTESIAN_POINT('Ctrl Pts',(-0.750928622000001,3.331598135,7.47339898));
#107636=CARTESIAN_POINT('Ctrl Pts',(-0.344435225,3.396744076,7.492086784));
#107637=CARTESIAN_POINT('',(-0.574977342003353,3.39596551435623,7.22716410679017));
#107638=CARTESIAN_POINT('Ctrl Pts',(-0.574977341341557,3.39596551348928,
7.22716410851735));
#107639=CARTESIAN_POINT('Ctrl Pts',(-0.577947813433749,3.3891302450623,
7.26866336228872));
#107640=CARTESIAN_POINT('Ctrl Pts',(-0.580902909912182,3.38247027236386,
7.3102192791635));
#107641=CARTESIAN_POINT('Ctrl Pts',(-0.586879657064628,3.36926348332785,
7.39477921946042));
#107642=CARTESIAN_POINT('Ctrl Pts',(-0.589803775723335,3.36293886744668,
7.43643676797683));
#107643=CARTESIAN_POINT('Ctrl Pts',(-0.592606977972659,3.35698786876839,
7.47655114138138));
#107644=CARTESIAN_POINT('Origin',(0.001144562001206,3.48208295609875,-0.19502964771908));
#107645=CARTESIAN_POINT('Ctrl Pts',(-2.119693429,3.396737969,6.933209918));
#107646=CARTESIAN_POINT('Ctrl Pts',(-2.003146542,3.376870318,6.968841851));
#107647=CARTESIAN_POINT('Ctrl Pts',(-1.885467899,3.357142857,7.000536465));
#107648=CARTESIAN_POINT('Ctrl Pts',(-1.619528158,3.312561141,7.072162525));
#107649=CARTESIAN_POINT('Ctrl Pts',(-1.34892079,3.267335925,7.123405976));
#107650=CARTESIAN_POINT('Ctrl Pts',(-2.426824903,3.396737969,7.0965147));
#107651=CARTESIAN_POINT('Ctrl Pts',(-2.307532871,3.376870318,7.137309497));
#107652=CARTESIAN_POINT('Ctrl Pts',(-2.186937109,3.357142857,7.174071792));
#107653=CARTESIAN_POINT('Ctrl Pts',(-1.914405023,3.312561141,7.25715021));
#107654=CARTESIAN_POINT('Ctrl Pts',(-1.63635545,3.267335925,7.31931286700001));
#107655=CARTESIAN_POINT('',(-2.1151613392112,3.39596551386392,6.93459389680009));
#107656=CARTESIAN_POINT('Ctrl Pts',(-2.11516133429227,3.39596551252257,
6.93459389798702));
#107657=CARTESIAN_POINT('Ctrl Pts',(-2.03883838298854,3.38295904388416,
6.95787361101831));
#107658=CARTESIAN_POINT('Ctrl Pts',(-1.96225208742926,3.37001483652073,
6.97985603265297));
#107659=CARTESIAN_POINT('Ctrl Pts',(-1.88546790027978,3.35714285716407,
7.0005364649097));
#107660=CARTESIAN_POINT('Ctrl Pts',(-1.7428577927959,3.33323592504676,7.03894591890685));
#107661=CARTESIAN_POINT('Ctrl Pts',(-1.59858079503118,3.30907960191736,
7.07312617265287));
#107662=CARTESIAN_POINT('Ctrl Pts',(-1.45302067817422,3.2847386775838,7.1029029922699));
#107663=CARTESIAN_POINT('Ctrl Pts',(-1.41839143496263,3.27894788950982,
7.1099869981834));
#107664=CARTESIAN_POINT('Ctrl Pts',(-1.38368968313904,3.2731466708905,7.11682198006919));
#107665=CARTESIAN_POINT('Ctrl Pts',(-1.34892079120537,3.267335925,7.12340597682154));
#107666=CARTESIAN_POINT('Ctrl Pts',(-2.18598964688771,3.35698786872379,
7.17436054715959));
#107667=CARTESIAN_POINT('Ctrl Pts',(-2.174628554927,3.36293887920927,7.13578655462272));
#107668=CARTESIAN_POINT('Ctrl Pts',(-2.16281771494842,3.369263464767,7.09573172665881));
#107669=CARTESIAN_POINT('Ctrl Pts',(-2.13880288145924,3.38247021625705,
7.01443380632259));
#107670=CARTESIAN_POINT('Ctrl Pts',(-2.12698352521173,3.38913021761768,
6.97448451705911));
#107671=CARTESIAN_POINT('Ctrl Pts',(-2.11516134064853,3.3959655135504,6.93459389632039));
#107672=CARTESIAN_POINT('Ctrl Pts',(-2.84870549,3.267335925,6.666886607));
#107673=CARTESIAN_POINT('Ctrl Pts',(-2.486984455,3.331598135,6.821447013));
#107674=CARTESIAN_POINT('Ctrl Pts',(-2.110664259,3.396744076,6.935963984));
#107675=CARTESIAN_POINT('Ctrl Pts',(-2.719168749,3.267335925,6.989715396));
#107676=CARTESIAN_POINT('Ctrl Pts',(-2.339932197,3.331598135,7.137247609));
#107677=CARTESIAN_POINT('Ctrl Pts',(-1.946959715,3.396744076,7.242882566));
#107678=CARTESIAN_POINT('Origin',(0.0430438123304711,3.48208225451749,-0.190224481412699));
#107679=CARTESIAN_POINT('Ctrl Pts',(-3.560571363,3.396737969,6.315443893));
#107680=CARTESIAN_POINT('Ctrl Pts',(-3.45440909,3.376870318,6.375296907));
#107681=CARTESIAN_POINT('Ctrl Pts',(-3.346295113,3.357142857,6.431547949));
#107682=CARTESIAN_POINT('Ctrl Pts',(-3.101970381,3.312561141,6.558668615));
#107683=CARTESIAN_POINT('Ctrl Pts',(-2.84870549,3.267335925,6.666886607));
#107684=CARTESIAN_POINT('Ctrl Pts',(-3.895627974,3.396737969,6.408906513));
#107685=CARTESIAN_POINT('Ctrl Pts',(-3.787894599,3.376870318,6.47439181));
#107686=CARTESIAN_POINT('Ctrl Pts',(-3.678021106,3.357142857,6.536219148));
#107687=CARTESIAN_POINT('Ctrl Pts',(-3.429720073,3.312561141,6.67594158));
#107688=CARTESIAN_POINT('Ctrl Pts',(-3.171534278,3.267335925,6.796423348));
#107689=CARTESIAN_POINT('',(-3.55644274497419,3.39596551373282,6.31776978094853));
#107690=CARTESIAN_POINT('Ctrl Pts',(-3.55644274019271,3.39596551234443,
6.31776978329846));
#107691=CARTESIAN_POINT('Ctrl Pts',(-3.48690862792311,3.38295904375008,
6.35691240809697));
#107692=CARTESIAN_POINT('Ctrl Pts',(-3.41683844837133,3.37001483645008,
6.39484468269108));
#107693=CARTESIAN_POINT('Ctrl Pts',(-3.34629511471059,3.35714285726472,
6.43154794832714));
#107694=CARTESIAN_POINT('Ctrl Pts',(-3.21527588556531,3.3332358953807,6.49971645300047));
#107695=CARTESIAN_POINT('Ctrl Pts',(-3.08171957845639,3.30907954184599,
6.56411295660272));
#107696=CARTESIAN_POINT('Ctrl Pts',(-2.94596353678932,3.28473858662282,
6.62448479822373));
#107697=CARTESIAN_POINT('Ctrl Pts',(-2.91366692831899,3.27894782923934,
6.63884736881376));
#107698=CARTESIAN_POINT('Ctrl Pts',(-2.88124597494332,3.27314664142021,
6.65298232703042));
#107699=CARTESIAN_POINT('Ctrl Pts',(-2.84870549797431,3.26733592642396,
6.66688660359265));
#107700=CARTESIAN_POINT('Ctrl Pts',(-3.67715786822643,3.35698786876754,
6.53670482815668));
#107701=CARTESIAN_POINT('Ctrl Pts',(-3.65777016219896,3.36293886754113,
6.50147504251046));
#107702=CARTESIAN_POINT('Ctrl Pts',(-3.63762475105133,3.36926348416743,
6.4648954769089));
#107703=CARTESIAN_POINT('Ctrl Pts',(-3.59669478159549,3.38247021621516,
6.39066084503493));
#107704=CARTESIAN_POINT('Ctrl Pts',(-3.57656383913318,3.38913021755435,
6.35418636013907));
#107705=CARTESIAN_POINT('Ctrl Pts',(-3.55644274658362,3.3959655134553,6.31776978008172));
#107706=CARTESIAN_POINT('Ctrl Pts',(-4.215287887,3.267335925,5.89863103));
#107707=CARTESIAN_POINT('Ctrl Pts',(-3.895249607,3.331598135,6.127337229));
#107708=CARTESIAN_POINT('Ctrl Pts',(-3.552345332,3.396744076,6.320074576));
#107709=CARTESIAN_POINT('Ctrl Pts',(-4.15817829,3.267335925,6.241758831));
#107710=CARTESIAN_POINT('Ctrl Pts',(-3.819523143,3.331598135,6.467366471));
#107711=CARTESIAN_POINT('Ctrl Pts',(-3.458446532,3.396744076,6.65500921));
#107712=CARTESIAN_POINT('Origin',(0.082930151739517,3.48208255747605,-0.176524157443751));
#107713=CARTESIAN_POINT('Ctrl Pts',(-4.834960937,3.396737969,5.402374731));
#107714=CARTESIAN_POINT('Ctrl Pts',(-4.744147307,3.376870318,5.483650165));
#107715=CARTESIAN_POINT('Ctrl Pts',(-4.650653287,3.357142857,5.561827398));
#107716=CARTESIAN_POINT('Ctrl Pts',(-4.439367916,3.312561141,5.738498649));
#107717=CARTESIAN_POINT('Ctrl Pts',(-4.215287887,3.267335925,5.89863103000001));
#107718=CARTESIAN_POINT('Ctrl Pts',(-5.182275811,3.396737969,5.421624979));
#107719=CARTESIAN_POINT('Ctrl Pts',(-5.091138586,3.376870318,5.508738758));
#107720=CARTESIAN_POINT('Ctrl Pts',(-4.997124924,3.357142857,5.59274016));
#107721=CARTESIAN_POINT('Ctrl Pts',(-4.784665224,3.312561141,5.782573342));
#107722=CARTESIAN_POINT('Ctrl Pts',(-4.558415688,3.267335925,5.955740627));
#107723=CARTESIAN_POINT('',(-4.83142884097952,3.39596551373665,5.40553377166376));
#107724=CARTESIAN_POINT('Ctrl Pts',(-4.83142883691769,3.39596551243094,
5.40553377475887));
#107725=CARTESIAN_POINT('Ctrl Pts',(-4.77193490002935,3.38295904377871,
5.45870904546908));
#107726=CARTESIAN_POINT('Ctrl Pts',(-4.71165724017725,3.37001483644787,
5.51081750187918));
#107727=CARTESIAN_POINT('Ctrl Pts',(-4.65065328796363,3.35714285717796,
5.56182739730548));
#107728=CARTESIAN_POINT('Ctrl Pts',(-4.53735147580372,3.33323590524741,
5.65656738232091));
#107729=CARTESIAN_POINT('Ctrl Pts',(-4.42076103529562,3.30907956178187,
5.74816895335652));
#107730=CARTESIAN_POINT('Ctrl Pts',(-4.30115710773929,3.28473861678128,
5.83631283751082));
#107731=CARTESIAN_POINT('Ctrl Pts',(-4.27270305300004,3.27894784890599,
5.8572824741766));
#107732=CARTESIAN_POINT('Ctrl Pts',(-4.24407862990798,3.27314665055719,
5.87805654968572));
#107733=CARTESIAN_POINT('Ctrl Pts',(-4.21528788727099,3.267335925,5.89863103004511));
#107734=CARTESIAN_POINT('Ctrl Pts',(-4.99638627566226,3.3569878687369,5.59340005602189));
#107735=CARTESIAN_POINT('Ctrl Pts',(-4.96987847846357,3.36293886806068,
5.56316170399128));
#107736=CARTESIAN_POINT('Ctrl Pts',(-4.9423405379198,3.36926348296273,5.5317680247819));
#107737=CARTESIAN_POINT('Ctrl Pts',(-4.88640923164213,3.38247021622749,
5.46806768500484));
#107738=CARTESIAN_POINT('Ctrl Pts',(-4.85890800332103,3.38913021754945,
5.43677351095003));
#107739=CARTESIAN_POINT('Ctrl Pts',(-4.83142884220982,3.39596551347391,
5.40553377052408));
#107740=CARTESIAN_POINT('Ctrl Pts',(-5.38476810800001,3.267335925,4.854562022));
#107741=CARTESIAN_POINT('Ctrl Pts',(-5.121377218,3.331598135,5.14671996700001));
#107742=CARTESIAN_POINT('Ctrl Pts',(-4.827922686,3.396744076,5.408665504));
#107743=CARTESIAN_POINT('Ctrl Pts',(-5.402756036,3.267335925,5.201944561));
#107744=CARTESIAN_POINT('Ctrl Pts',(-5.120517432,3.331598135,5.49507846600001));
#107745=CARTESIAN_POINT('Ctrl Pts',(-4.808220234,3.396744076,5.755955019));
#107746=CARTESIAN_POINT('Origin',(0.11893884844377,3.48208255706764,-0.154569677558902));
#107747=CARTESIAN_POINT('Ctrl Pts',(-5.883273111,3.396737969,4.236696531));
#107748=CARTESIAN_POINT('Ctrl Pts',(-5.81205447,3.376870318,4.335594037));
#107749=CARTESIAN_POINT('Ctrl Pts',(-5.737552082,3.357142857,4.43204198));
#107750=CARTESIAN_POINT('Ctrl Pts',(-5.569185542,3.312561141,4.650002864));
#107751=CARTESIAN_POINT('Ctrl Pts',(-5.384768108,3.267335925,4.854562022));
#107752=CARTESIAN_POINT('Ctrl Pts',(-6.226606191,3.396737969,4.180834288));
#107753=CARTESIAN_POINT('Ctrl Pts',(-6.156326591,3.376870318,4.285503204));
#107754=CARTESIAN_POINT('Ctrl Pts',(-6.082568734,3.357142857,4.387750858));
#107755=CARTESIAN_POINT('Ctrl Pts',(-5.915884747,3.312561141,4.618818401));
#107756=CARTESIAN_POINT('Ctrl Pts',(-5.732150647,3.267335925,4.836574093));
#107757=CARTESIAN_POINT('',(-5.88050269384339,3.3959655137552,4.240541011126));
#107758=CARTESIAN_POINT('Ctrl Pts',(-5.88050269069937,3.39596551248106,
4.24054101494916));
#107759=CARTESIAN_POINT('Ctrl Pts',(-5.83383080093294,3.38295904381877,
4.30526251552692));
#107760=CARTESIAN_POINT('Ctrl Pts',(-5.78616417724815,3.37001483647222,
4.36911062035155));
#107761=CARTESIAN_POINT('Ctrl Pts',(-5.73755208286525,3.35714285718789,
4.43204197906141));
#107762=CARTESIAN_POINT('Ctrl Pts',(-5.64726547606571,3.33323589884546,
4.54892356737364));
#107763=CARTESIAN_POINT('Ctrl Pts',(-5.55309245898912,3.30907954889413,
4.66344707267108));
#107764=CARTESIAN_POINT('Ctrl Pts',(-5.45523310639709,3.28473859731843,
4.77524153924819));
#107765=CARTESIAN_POINT('Ctrl Pts',(-5.43195216929584,3.27894783590822,
4.8018376680362));
#107766=CARTESIAN_POINT('Ctrl Pts',(-5.40846280757583,3.27314664404836,
4.82827943229482));
#107767=CARTESIAN_POINT('Ctrl Pts',(-5.38476810818828,3.267335925,4.85456202199025));
#107768=CARTESIAN_POINT('Ctrl Pts',(-6.08198921329168,3.35698786876477,
4.38855411340845));
#107769=CARTESIAN_POINT('Ctrl Pts',(-6.04960074080444,3.36293887928365,
4.36472106532315));
#107770=CARTESIAN_POINT('Ctrl Pts',(-6.01595806662991,3.36926346429008,
4.33998131233127));
#107771=CARTESIAN_POINT('Ctrl Pts',(-5.9476406162827,3.38247021628422,4.28979375773227));
#107772=CARTESIAN_POINT('Ctrl Pts',(-5.91405502901164,3.38913021762073,
4.26514317521011));
#107773=CARTESIAN_POINT('Ctrl Pts',(-5.88050269485365,3.39596551352586,
4.2405410096845));
#107774=CARTESIAN_POINT('Ctrl Pts',(-6.30246255700001,3.267335925,3.583499089));
#107775=CARTESIAN_POINT('Ctrl Pts',(-6.108034921,3.331598135,3.9254478));
#107776=CARTESIAN_POINT('Ctrl Pts',(-5.877751741,3.396744076,4.244353245));
#107777=CARTESIAN_POINT('Ctrl Pts',(-6.39470691500001,3.267335925,3.918893144));
#107778=CARTESIAN_POINT('Ctrl Pts',(-6.182082017,3.331598135,4.265846698));
#107779=CARTESIAN_POINT('Ctrl Pts',(-5.933166901,3.396744076,4.58775876899999));
#107780=CARTESIAN_POINT('Origin',(0.149385868638626,3.48208259248333,-0.125387490683405));
#107781=CARTESIAN_POINT('Ctrl Pts',(-6.656489974,3.396737969,2.87291511));
#107782=CARTESIAN_POINT('Ctrl Pts',(-6.608196425,3.376870318,2.98481035));
#107783=CARTESIAN_POINT('Ctrl Pts',(-6.556169318,3.357142857,3.095019205));
#107784=CARTESIAN_POINT('Ctrl Pts',(-6.438594242,3.312561141,3.344078114));
#107785=CARTESIAN_POINT('Ctrl Pts',(-6.302462557,3.267335925,3.583499089));
#107786=CARTESIAN_POINT('Ctrl Pts',(-6.979787386,3.396737969,2.744552431));
#107787=CARTESIAN_POINT('Ctrl Pts',(-6.933651607,3.376870318,2.861882283));
#107788=CARTESIAN_POINT('Ctrl Pts',(-6.883598391,3.357142857,2.977595203));
#107789=CARTESIAN_POINT('Ctrl Pts',(-6.770484074,3.312561141,3.239092645));
#107790=CARTESIAN_POINT('Ctrl Pts',(-6.63785661200001,3.267335925,3.491254731));
#107791=CARTESIAN_POINT('',(-6.65461077676593,3.39596551374942,2.87726526625745));
#107792=CARTESIAN_POINT('Ctrl Pts',(-6.65461077492331,3.3959655124626,2.87726527063129));
#107793=CARTESIAN_POINT('Ctrl Pts',(-6.62294325708987,3.3829590439033,2.9505066947672));
#107794=CARTESIAN_POINT('Ctrl Pts',(-6.59011650753996,3.37001483656461,
3.02310898150559));
#107795=CARTESIAN_POINT('Ctrl Pts',(-6.55616931878919,3.35714285729924,
3.09501920332825));
#107796=CARTESIAN_POINT('Ctrl Pts',(-6.49311964373262,3.33323589670651,
3.228577129268));
#107797=CARTESIAN_POINT('Ctrl Pts',(-6.42576750106537,3.30907954446892,
3.36066756582076));
#107798=CARTESIAN_POINT('Ctrl Pts',(-6.35422854380943,3.28473859052526,
3.49088521988956));
#107799=CARTESIAN_POINT('Ctrl Pts',(-6.33720929007269,3.27894783137455,
3.52186424699044));
#107800=CARTESIAN_POINT('Ctrl Pts',(-6.31995330093824,3.27314664177974,
3.55273732373537));
#107801=CARTESIAN_POINT('Ctrl Pts',(-6.30246255717339,3.267335925,3.58349908895232));
#107802=CARTESIAN_POINT('Ctrl Pts',(-6.8832050949221,3.35698786871989,2.97850425893303));
#107803=CARTESIAN_POINT('Ctrl Pts',(-6.84645051598102,3.36293886794177,
2.96219100945032));
#107804=CARTESIAN_POINT('Ctrl Pts',(-6.80827589352812,3.3692634829752,2.94526175870117));
#107805=CARTESIAN_POINT('Ctrl Pts',(-6.73076693640478,3.38247021625307,
2.91093384222089));
#107806=CARTESIAN_POINT('Ctrl Pts',(-6.69266741499193,3.38913021757927,
2.89407948518823));
#107807=CARTESIAN_POINT('Ctrl Pts',(-6.65461077733531,3.39596551349355,
2.87726526486472));
#107808=CARTESIAN_POINT('Ctrl Pts',(-6.925460861,3.267335925,2.144875721));
#107809=CARTESIAN_POINT('Ctrl Pts',(-6.809087701,3.331598135,2.520626056));
#107810=CARTESIAN_POINT('Ctrl Pts',(-6.652743657,3.396744076,2.881579746));
#107811=CARTESIAN_POINT('Ctrl Pts',(-7.087648405,3.267335925,2.45259864));
#107812=CARTESIAN_POINT('Ctrl Pts',(-6.954579317,3.331598135,2.837148681));
#107813=CARTESIAN_POINT('Ctrl Pts',(-6.780685278,3.396744076,3.205044018));
#107814=CARTESIAN_POINT('Origin',(0.172847961265036,3.48208254856463,-0.0903424629903771));
#107815=CARTESIAN_POINT('Ctrl Pts',(-7.118456763,3.396737969,1.374799371));
#107816=CARTESIAN_POINT('Ctrl Pts',(-7.095346459,3.376870318,1.494460248));
#107817=CARTESIAN_POINT('Ctrl Pts',(-7.068227363,3.357142857,1.613276771));
#107818=CARTESIAN_POINT('Ctrl Pts',(-7.00694143000001,3.312561141,1.881787987));
#107819=CARTESIAN_POINT('Ctrl Pts',(-6.925460861,3.267335925,2.144875721));
#107820=CARTESIAN_POINT('Ctrl Pts',(-7.40660148,3.396737969,1.179938354));
#107821=CARTESIAN_POINT('Ctrl Pts',(-7.386766779,3.376870318,1.304442928));
#107822=CARTESIAN_POINT('Ctrl Pts',(-7.362758637,3.357142857,1.428210506));
#107823=CARTESIAN_POINT('Ctrl Pts',(-7.308503091,3.312561141,1.707910518));
#107824=CARTESIAN_POINT('Ctrl Pts',(-7.23318378,3.267335925,1.982688177));
#107825=CARTESIAN_POINT('',(-7.11755665579964,3.39596551374277,1.37945179519918));
#107826=CARTESIAN_POINT('Ctrl Pts',(-7.11755665457148,3.39596551231891,
1.37945180024207));
#107827=CARTESIAN_POINT('Ctrl Pts',(-7.10237424704946,3.38295904372266,
1.45778846079517));
#107828=CARTESIAN_POINT('Ctrl Pts',(-7.08592231402127,3.3700148364319,1.53575012695171));
#107829=CARTESIAN_POINT('Ctrl Pts',(-7.06822736368685,3.3571428571178,1.61327676996068));
#107830=CARTESIAN_POINT('Ctrl Pts',(-7.0353627534341,3.33323589104236,1.75726603526585));
#107831=CARTESIAN_POINT('Ctrl Pts',(-6.99798079655694,3.30907953327899,
1.90074702277125));
#107832=CARTESIAN_POINT('Ctrl Pts',(-6.95610731559513,3.28473857385227,
2.04329905286339));
#107833=CARTESIAN_POINT('Ctrl Pts',(-6.94614554674343,3.27894782023285,
2.07721241140201));
#107834=CARTESIAN_POINT('Ctrl Pts',(-6.93592980152675,3.27314663619637,
2.11107318782929));
#107835=CARTESIAN_POINT('Ctrl Pts',(-6.92546086189945,3.267335925,2.14487572052594));
#107836=CARTESIAN_POINT('Ctrl Pts',(-7.36256995641699,3.35698786876322,
1.42918285531943));
#107837=CARTESIAN_POINT('Ctrl Pts',(-7.32316781100546,3.36293886821889,
1.42115214801801));
#107838=CARTESIAN_POINT('Ctrl Pts',(-7.28224641027146,3.36926348187864,
1.41282511087487));
#107839=CARTESIAN_POINT('Ctrl Pts',(-7.19917007545255,3.38247021622246,
1.3959618950794));
#107840=CARTESIAN_POINT('Ctrl Pts',(-7.158338111131,3.38913021755116,1.38769185434494));
#107841=CARTESIAN_POINT('Ctrl Pts',(-7.11755665616871,3.39596551346862,
1.37945179314519));
#107842=CARTESIAN_POINT('Ctrl Pts',(-7.224632313,3.267335925,0.605960349000001));
#107843=CARTESIAN_POINT('Ctrl Pts',(-7.191755107,3.331598135,0.997942639));
#107844=CARTESIAN_POINT('Ctrl Pts',(-7.116660674,3.396744076,1.38406678));
#107845=CARTESIAN_POINT('Ctrl Pts',(-7.449179333,3.267335925,0.871623349000001));
#107846=CARTESIAN_POINT('Ctrl Pts',(-7.401888218,3.331598135,1.275788744));
#107847=CARTESIAN_POINT('Ctrl Pts',(-7.311146348,3.396744076,1.672464971));
#107848=CARTESIAN_POINT('Origin',(0.188227844185853,3.48208256576102,-0.0510731071993649));
#107849=CARTESIAN_POINT('Ctrl Pts',(-7.247572426,3.396737969,-0.187600458));
#107850=CARTESIAN_POINT('Ctrl Pts',(-7.25072598,3.376870318,-0.065769154));
#107851=CARTESIAN_POINT('Ctrl Pts',(-7.249782953,3.357142857,0.056099309));
#107852=CARTESIAN_POINT('Ctrl Pts',(-7.247651826,3.312561141,0.331507546));
#107853=CARTESIAN_POINT('Ctrl Pts',(-7.224632313,3.267335925,0.605960349000001));
#107854=CARTESIAN_POINT('Ctrl Pts',(-7.487091121,3.396737969,-0.43984833));
#107855=CARTESIAN_POINT('Ctrl Pts',(-7.494484947,3.376870318,-0.313990729));
#107856=CARTESIAN_POINT('Ctrl Pts',(-7.497644473,3.357142857,-0.187955727));
#107857=CARTESIAN_POINT('Ctrl Pts',(-7.504784626,3.312561141,0.0968683920000001));
#107858=CARTESIAN_POINT('Ctrl Pts',(-7.490295313,3.267335925,0.381413328));
#107859=CARTESIAN_POINT('',(-7.24769349608873,3.39596551376398,-0.182863309139555));
#107860=CARTESIAN_POINT('Ctrl Pts',(-7.2476934961534,3.39596551248093,-0.182863304051593));
#107861=CARTESIAN_POINT('Ctrl Pts',(-7.2497061112786,3.38295904386738,-0.103094342054963));
#107862=CARTESIAN_POINT('Ctrl Pts',(-7.25039826907839,3.37001483651852,
-0.0234186968749169));
#107863=CARTESIAN_POINT('Ctrl Pts',(-7.24978295327409,3.35714285717451,
0.0560993076602942));
#107864=CARTESIAN_POINT('Ctrl Pts',(-7.24864013544803,3.33323588073399,
0.203787167236864));
#107865=CARTESIAN_POINT('Ctrl Pts',(-7.24297631397189,3.30907951252702,
0.35194972910359));
#107866=CARTESIAN_POINT('Ctrl Pts',(-7.23272627583705,3.28473854237686,
0.500170597084882));
#107867=CARTESIAN_POINT('Ctrl Pts',(-7.23028778066582,3.27894779922121,
0.535432502074355));
#107868=CARTESIAN_POINT('Ctrl Pts',(-7.22758994432299,3.27314662567951,
0.570697651697861));
#107869=CARTESIAN_POINT('Ctrl Pts',(-7.22463231342918,3.267335925,0.605960348637243));
#107870=CARTESIAN_POINT('Ctrl Pts',(-7.49766922997614,3.35698786881975,
-0.186965550244216));
#107871=CARTESIAN_POINT('Ctrl Pts',(-7.4574619215761,3.3629388680623,-0.186338207434659));
#107872=CARTESIAN_POINT('Ctrl Pts',(-7.41570717295739,3.36926348177469,
-0.185673671628998));
#107873=CARTESIAN_POINT('Ctrl Pts',(-7.33094802269087,3.38247021627394,
-0.184283678323024));
#107874=CARTESIAN_POINT('Ctrl Pts',(-7.28929287292059,3.38913021757036,
-0.183582704619095));
#107875=CARTESIAN_POINT('Ctrl Pts',(-7.24769349602485,3.39596551350206,
-0.182863310345163));
#107876=CARTESIAN_POINT('Ctrl Pts',(-7.185987987,3.267335925,-0.961289056000001));
#107877=CARTESIAN_POINT('Ctrl Pts',(-7.238144037,3.331598135,-0.571403467));
#107878=CARTESIAN_POINT('Ctrl Pts',(-7.247810547,3.396744076,-0.17816361));
#107879=CARTESIAN_POINT('Ctrl Pts',(-7.462394915,3.267335925,-0.750108081));
#107880=CARTESIAN_POINT('Ctrl Pts',(-7.503093053,3.331598135,-0.345225657));
#107881=CARTESIAN_POINT('Ctrl Pts',(-7.49974634,3.396744076,0.0616833200000001));
#107882=CARTESIAN_POINT('Origin',(0.194806496690273,3.48208256695309,-0.0094156120496422));
#107883=CARTESIAN_POINT('Ctrl Pts',(-7.03779965700001,3.396737969,-1.741228298));
#107884=CARTESIAN_POINT('Ctrl Pts',(-7.067069611,3.376870318,-1.622923263));
#107885=CARTESIAN_POINT('Ctrl Pts',(-7.09234675,3.357142857,-1.503701295));
#107886=CARTESIAN_POINT('Ctrl Pts',(-7.149470077,3.312561141,-1.234273819));
#107887=CARTESIAN_POINT('Ctrl Pts',(-7.18598798700001,3.267335925,-0.961289056));
#107888=CARTESIAN_POINT('Ctrl Pts',(-7.217492702,3.396737969,-2.039068194));
#107889=CARTESIAN_POINT('Ctrl Pts',(-7.251769329,3.376870318,-1.917742529));
#107890=CARTESIAN_POINT('Ctrl Pts',(-7.281948786,3.357142857,-1.79533336));
#107891=CARTESIAN_POINT('Ctrl Pts',(-7.350150772,3.312561141,-1.518703192));
#107892=CARTESIAN_POINT('Ctrl Pts',(-7.397168962,3.267335925,-1.237695984));
#107893=CARTESIAN_POINT('',(-7.03893624368007,3.39596551376467,-1.73662792753749));
#107894=CARTESIAN_POINT('Ctrl Pts',(-7.03893624466455,3.39596551246643,
-1.73662792249366));
#107895=CARTESIAN_POINT('Ctrl Pts',(-7.05804977456909,3.38295904384934,
-1.65915656746975));
#107896=CARTESIAN_POINT('Ctrl Pts',(-7.07585365883465,3.37001483650869,
-1.58149248836743));
#107897=CARTESIAN_POINT('Ctrl Pts',(-7.09234674982968,3.35714285721031,
-1.50370129642354));
#107898=CARTESIAN_POINT('Ctrl Pts',(-7.1229791605006,3.33323589123215,-1.35922068675125));
#107899=CARTESIAN_POINT('Ctrl Pts',(-7.14929831789834,3.30907953349491,
-1.21330459259));
#107900=CARTESIAN_POINT('Ctrl Pts',(-7.17115101956385,3.28473857395464,
-1.06634565525889));
#107901=CARTESIAN_POINT('Ctrl Pts',(-7.17634981263611,3.27894782030931,
-1.03138388636658));
#107902=CARTESIAN_POINT('Ctrl Pts',(-7.1812960243595,3.27314663623902,-0.99636319779376));
#107903=CARTESIAN_POINT('Ctrl Pts',(-7.18598798717056,3.267335925,-0.961289056223232));
#107904=CARTESIAN_POINT('Ctrl Pts',(-7.28218582307141,3.35698786876996,
-1.79437165487534));
#107905=CARTESIAN_POINT('Ctrl Pts',(-7.24305332634517,3.36293887913784,
-1.78511557887735));
#107906=CARTESIAN_POINT('Ctrl Pts',(-7.20241782122286,3.36926346384614,
-1.77549058655937));
#107907=CARTESIAN_POINT('Ctrl Pts',(-7.11993850864496,3.38247029310111,
-1.75591223833854));
#107908=CARTESIAN_POINT('Ctrl Pts',(-7.07940817845462,3.38913025525282,
-1.74627308796842));
#107909=CARTESIAN_POINT('Ctrl Pts',(-7.0389362434003,3.39596551355439,-1.73662792952758));
#107910=CARTESIAN_POINT('Ctrl Pts',(-6.81133485,3.267335925,-2.483589653));
#107911=CARTESIAN_POINT('Ctrl Pts',(-6.946085397,3.331598135,-2.114031381));
#107912=CARTESIAN_POINT('Ctrl Pts',(-7.040060855,3.396744076,-1.732063268));
#107913=CARTESIAN_POINT('Ctrl Pts',(-7.126677204,3.267335925,-2.336765291));
#107914=CARTESIAN_POINT('Ctrl Pts',(-7.253461596,3.331598135,-1.950097689));
#107915=CARTESIAN_POINT('Ctrl Pts',(-7.337666529,3.396744076,-1.551982574));
#107916=CARTESIAN_POINT('Origin',(0.192275901926948,3.48208255376959,0.0326820931064098));
#107917=CARTESIAN_POINT('Ctrl Pts',(-6.498947198,3.396737969,-3.213438239));
#107918=CARTESIAN_POINT('Ctrl Pts',(-6.552964923,3.376870318,-3.104191285));
#107919=CARTESIAN_POINT('Ctrl Pts',(-6.603280295,3.357142857,-2.993190497));
#107920=CARTESIAN_POINT('Ctrl Pts',(-6.716987053,3.312561141,-2.742341913));
#107921=CARTESIAN_POINT('Ctrl Pts',(-6.81133485,3.267335925,-2.483589653));
#107922=CARTESIAN_POINT('Ctrl Pts',(-6.610412346,3.396737969,-3.542943496));
#107923=CARTESIAN_POINT('Ctrl Pts',(-6.669969036,3.376870318,-3.431822819));
#107924=CARTESIAN_POINT('Ctrl Pts',(-6.725757268,3.357142857,-3.3187632));
#107925=CARTESIAN_POINT('Ctrl Pts',(-6.851832038,3.312561141,-3.063261902));
#107926=CARTESIAN_POINT('Ctrl Pts',(-6.95815921200001,3.267335925,-2.798932008));
#107927=CARTESIAN_POINT('',(-6.50104615569751,3.39596551372471,-3.2091897545298));
#107928=CARTESIAN_POINT('Ctrl Pts',(-6.50104615793014,3.39596551236517,
-3.20918974991457));
#107929=CARTESIAN_POINT('Ctrl Pts',(-6.53636687541928,3.38295904389764,
-3.13763847664817));
#107930=CARTESIAN_POINT('Ctrl Pts',(-6.5704499960716,3.37001483658892,-3.06561744931968));
#107931=CARTESIAN_POINT('Ctrl Pts',(-6.60328029421643,3.35714285730722,
-2.99319049872864));
#107932=CARTESIAN_POINT('Ctrl Pts',(-6.66425557433981,3.33323589990589,
-2.85867287694132));
#107933=CARTESIAN_POINT('Ctrl Pts',(-6.72132703253208,3.30907955088029,
-2.72182611067045));
#107934=CARTESIAN_POINT('Ctrl Pts',(-6.77426064199191,3.28473860015761,
-2.5830007274313));
#107935=CARTESIAN_POINT('Ctrl Pts',(-6.78685365678872,3.27894783780932,
-2.54997388261299));
#107936=CARTESIAN_POINT('Ctrl Pts',(-6.79921266075128,3.27314664500316,
-2.51683519774265));
#107937=CARTESIAN_POINT('Ctrl Pts',(-6.81133485011412,3.267335925,-2.48358965324511));
#107938=CARTESIAN_POINT('Ctrl Pts',(-6.72619550123133,3.35698786876473,
-3.31787493432137));
#107939=CARTESIAN_POINT('Ctrl Pts',(-6.68996775206939,3.3629388678247,-3.30042296335432));
#107940=CARTESIAN_POINT('Ctrl Pts',(-6.65235119061501,3.36926348312789,
-3.28228747871531));
#107941=CARTESIAN_POINT('Ctrl Pts',(-6.57600906312393,3.38247029531356,
-3.24543629492914));
#107942=CARTESIAN_POINT('Ctrl Pts',(-6.53849844885975,3.38913025630653,
-3.22730968299859));
#107943=CARTESIAN_POINT('Ctrl Pts',(-6.50104615482508,3.39596551351214,
-3.20918975625285));
#107944=CARTESIAN_POINT('Ctrl Pts',(-6.118191265,3.267335925,-3.889760358));
#107945=CARTESIAN_POINT('Ctrl Pts',(-6.329235524,3.331598135,-3.557809538));
#107946=CARTESIAN_POINT('Ctrl Pts',(-6.503125741,3.396744076,-3.204973572));
#107947=CARTESIAN_POINT('Ctrl Pts',(-6.45772398800001,3.267335925,-3.814157953));
#107948=CARTESIAN_POINT('Ctrl Pts',(-6.664666336,3.331598135,-3.463785321));
#107949=CARTESIAN_POINT('Ctrl Pts',(-6.832485586,3.396744076,-3.093079487));
#107950=CARTESIAN_POINT('Origin',(0.180754990267068,3.48208253270065,0.0732516867238425));
#107951=CARTESIAN_POINT('Ctrl Pts',(-5.656211191,3.396737969,-4.535391379));
#107952=CARTESIAN_POINT('Ctrl Pts',(-5.732450877,3.376870318,-4.440310772));
#107953=CARTESIAN_POINT('Ctrl Pts',(-5.805451792,3.357142857,-4.342721438));
#107954=CARTESIAN_POINT('Ctrl Pts',(-5.97042518,3.312561141,-4.122181147));
#107955=CARTESIAN_POINT('Ctrl Pts',(-6.118191265,3.267335925,-3.889760358));
#107956=CARTESIAN_POINT('Ctrl Pts',(-5.694236456,3.396737969,-4.881154698));
#107957=CARTESIAN_POINT('Ctrl Pts',(-5.776288404,3.376870318,-4.785434889));
#107958=CARTESIAN_POINT('Ctrl Pts',(-5.855076814,3.357142857,-4.687011361));
#107959=CARTESIAN_POINT('Ctrl Pts',(-6.033129253,3.312561141,-4.464585891));
#107960=CARTESIAN_POINT('Ctrl Pts',(-6.19379367,3.267335925,-4.229293082));
#107961=CARTESIAN_POINT('',(-5.65917437486607,3.39596551372921,-4.5316934355077));
#107962=CARTESIAN_POINT('Ctrl Pts',(-5.6591743779949,3.39596551235788,-4.53169343152599));
#107963=CARTESIAN_POINT('Ctrl Pts',(-5.70905072577702,3.38295904374474,
-4.469407896851));
#107964=CARTESIAN_POINT('Ctrl Pts',(-5.75781939387318,3.37001483644105,
-4.40639754447334));
#107965=CARTESIAN_POINT('Ctrl Pts',(-5.80545179132042,3.35714285719604,
-4.34272143928784));
#107966=CARTESIAN_POINT('Ctrl Pts',(-5.89391873234071,3.33323592234731,
-4.22445675947104));
#107967=CARTESIAN_POINT('Ctrl Pts',(-5.97907382423562,3.3090795962726,-4.1030781881729));
#107968=CARTESIAN_POINT('Ctrl Pts',(-6.06061315891376,3.28473866884692,
-3.97887774869767));
#107969=CARTESIAN_POINT('Ctrl Pts',(-6.08001162970604,3.27894788368063,
-3.94933006343559));
#107970=CARTESIAN_POINT('Ctrl Pts',(-6.09920560139156,3.27314666797384,
-3.91962284618732));
#107971=CARTESIAN_POINT('Ctrl Pts',(-6.11819126506037,3.267335925,-3.88976035827113));
#107972=CARTESIAN_POINT('Ctrl Pts',(-5.85569575257732,3.35698786875252,
-4.68623807017156));
#107973=CARTESIAN_POINT('Ctrl Pts',(-5.82406658291608,3.36293887966387,
-4.66140617195981));
#107974=CARTESIAN_POINT('Ctrl Pts',(-5.79122822973608,3.36926346374271,
-4.63560836239597));
#107975=CARTESIAN_POINT('Ctrl Pts',(-5.72459315521993,3.38247021623446,
-4.58320767478909));
#107976=CARTESIAN_POINT('Ctrl Pts',(-5.69185599036889,3.38913021755001,
-4.5574410118512));
#107977=CARTESIAN_POINT('Ctrl Pts',(-5.65917437376494,3.3959655134616,-4.53169343683433));
#107978=CARTESIAN_POINT('Ctrl Pts',(-5.138967857,3.267335925,-5.114050192));
#107979=CARTESIAN_POINT('Ctrl Pts',(-5.416437632,3.331598135,-4.835228475));
#107980=CARTESIAN_POINT('Ctrl Pts',(-5.662111695,3.396744076,-4.528022874));
#107981=CARTESIAN_POINT('Ctrl Pts',(-5.486814776,3.267335925,-5.11320482800001));
#107982=CARTESIAN_POINT('Ctrl Pts',(-5.764238685,3.331598135,-4.815510201));
#107983=CARTESIAN_POINT('Ctrl Pts',(-6.007825211,3.396744076,-4.489547442));
#107984=CARTESIAN_POINT('Origin',(0.160782004737559,3.48208256640899,0.110395990657645));
#107985=CARTESIAN_POINT('Ctrl Pts',(-4.548997036,3.396737969,-5.64527465800001));
#107986=CARTESIAN_POINT('Ctrl Pts',(-4.6438938,3.376870318,-5.568806262));
#107987=CARTESIAN_POINT('Ctrl Pts',(-4.736166816,3.357142857,-5.489191552));
#107988=CARTESIAN_POINT('Ctrl Pts',(-4.944692861,3.312561141,-5.309271772));
#107989=CARTESIAN_POINT('Ctrl Pts',(-5.138967857,3.267335925,-5.114050192));
#107990=CARTESIAN_POINT('Ctrl Pts',(-4.511804397,3.396737969,-5.991128531));
#107991=CARTESIAN_POINT('Ctrl Pts',(-4.612514947,3.376870318,-5.915285341));
#107992=CARTESIAN_POINT('Ctrl Pts',(-4.710619476,3.357142857,-5.83610008));
#107993=CARTESIAN_POINT('Ctrl Pts',(-4.93232405,3.312561141,-5.657150805));
#107994=CARTESIAN_POINT('Ctrl Pts',(-5.139813221,3.267335925,-5.461897111));
#107995=CARTESIAN_POINT('',(-4.55268589075781,3.39596551376344,-5.64230016798178));
#107996=CARTESIAN_POINT('Ctrl Pts',(-4.55268589439774,3.39596551241353,
-5.64230016474708));
#107997=CARTESIAN_POINT('Ctrl Pts',(-4.61478570966965,3.38295904375274,
-5.59219277144712));
#107998=CARTESIAN_POINT('Ctrl Pts',(-4.67595955649415,3.37001483642585,
-5.54113938813364));
#107999=CARTESIAN_POINT('Ctrl Pts',(-4.73616681521636,3.35714285716618,
-5.48919155275715));
#108000=CARTESIAN_POINT('Ctrl Pts',(-4.84798885387433,3.33323592329174,
-5.39270961640222));
#108001=CARTESIAN_POINT('Ctrl Pts',(-4.95724586759288,3.30907959821499,
-5.29247464058025));
#108002=CARTESIAN_POINT('Ctrl Pts',(-5.06357827707533,3.28473867183283,
-5.18870648985122));
#108003=CARTESIAN_POINT('Ctrl Pts',(-5.0888751057795,3.27894788567283,-5.16401970670844));
#108004=CARTESIAN_POINT('Ctrl Pts',(-5.11400651106192,3.27314666897044,
-5.13913316002725));
#108005=CARTESIAN_POINT('Ctrl Pts',(-5.13896785700169,3.267335925,-5.114050192696));
#108006=CARTESIAN_POINT('Ctrl Pts',(-4.71139017880485,3.35698786875269,
-5.83547792184127));
#108007=CARTESIAN_POINT('Ctrl Pts',(-4.68583860689359,3.36293887935722,
-5.80442724467471));
#108008=CARTESIAN_POINT('Ctrl Pts',(-4.65931375765883,3.36926346474903,
-5.77217329178179));
#108009=CARTESIAN_POINT('Ctrl Pts',(-4.60550117740311,3.38247021619481,
-5.70667313699998));
#108010=CARTESIAN_POINT('Ctrl Pts',(-4.57906846021727,3.3891302175044,-5.67447136160083));
#108011=CARTESIAN_POINT('Ctrl Pts',(-4.55268588945475,3.39596551344277,
-5.64230016898225));
#108012=CARTESIAN_POINT('Ctrl Pts',(-3.919452023,3.267335925,-6.09921272300001));
#108013=CARTESIAN_POINT('Ctrl Pts',(-4.250373136,3.331598135,-5.886557502));
#108014=CARTESIAN_POINT('Ctrl Pts',(-4.5563436,3.396744076,-5.639346859));
#108015=CARTESIAN_POINT('Ctrl Pts',(-4.259348203,3.267335925,-6.173163928));
#108016=CARTESIAN_POINT('Ctrl Pts',(-4.59428164,3.331598135,-5.942067176));
#108017=CARTESIAN_POINT('Ctrl Pts',(-4.902245606,3.396744076,-5.676089148));
#108018=CARTESIAN_POINT('Origin',(0.133291327431939,3.48208259557583,0.142378644240245));
#108019=CARTESIAN_POINT('Ctrl Pts',(-3.229076835,3.396737969,-6.49119116900001));
#108020=CARTESIAN_POINT('Ctrl Pts',(-3.33819341,3.376870318,-6.436910561));
#108021=CARTESIAN_POINT('Ctrl Pts',(-3.445423944,3.357142857,-6.378993169));
#108022=CARTESIAN_POINT('Ctrl Pts',(-3.6877522,3.312561141,-6.248106749));
#108023=CARTESIAN_POINT('Ctrl Pts',(-3.919452023,3.267335925,-6.09921272300001));
#108024=CARTESIAN_POINT('Ctrl Pts',(-3.11840538,3.396737969,-6.820963853));
#108025=CARTESIAN_POINT('Ctrl Pts',(-3.233065417,3.376870318,-6.768543626));
#108026=CARTESIAN_POINT('Ctrl Pts',(-3.345898807,3.357142857,-6.712299246));
#108027=CARTESIAN_POINT('Ctrl Pts',(-3.600888855,3.312561141,-6.585193635));
#108028=CARTESIAN_POINT('Ctrl Pts',(-3.845500817,3.267335925,-6.439108903));
#108029=CARTESIAN_POINT('',(-3.23331887358448,3.39596551379113,-6.48907921538511));
#108030=CARTESIAN_POINT('Ctrl Pts',(-3.23331887791266,3.39596551246019,
-6.48907921306364));
#108031=CARTESIAN_POINT('Ctrl Pts',(-3.30473844184022,3.38295904388523,
-6.45349292782824));
#108032=CARTESIAN_POINT('Ctrl Pts',(-3.37545704658702,3.37001483654186,
-6.41678371308469));
#108033=CARTESIAN_POINT('Ctrl Pts',(-3.44542394259196,3.35714285725904,
-6.37899316976051));
#108034=CARTESIAN_POINT('Ctrl Pts',(-3.57537225490592,3.33323595160592,
-6.3088054431801));
#108035=CARTESIAN_POINT('Ctrl Pts',(-3.70362230820437,3.30907965522593,
-6.23440102649535));
#108036=CARTESIAN_POINT('Ctrl Pts',(-3.82977566596386,3.28473875800089,
-6.15591734453168));
#108037=CARTESIAN_POINT('Ctrl Pts',(-3.85978814753651,3.2789479432148,-6.13724570470757));
#108038=CARTESIAN_POINT('Ctrl Pts',(-3.88968201527148,3.27314669778425,
-6.11834340825996));
#108039=CARTESIAN_POINT('Ctrl Pts',(-3.91945202291905,3.267335925,-6.09921272337206));
#108040=CARTESIAN_POINT('Ctrl Pts',(-3.34678523697663,3.3569878687276,-6.71185731173205));
#108041=CARTESIAN_POINT('Ctrl Pts',(-3.32850605734561,3.36293886864128,
-6.67603981394387));
#108042=CARTESIAN_POINT('Ctrl Pts',(-3.30953490584486,3.36926348259368,
-6.63883771552335));
#108043=CARTESIAN_POINT('Ctrl Pts',(-3.27106108269111,3.38247021625425,
-6.56330090580448));
#108044=CARTESIAN_POINT('Ctrl Pts',(-3.25216877742182,3.38913021759946,
-6.52616973707086));
#108045=CARTESIAN_POINT('Ctrl Pts',(-3.23331887183457,3.39596551355691,
-6.48907921623128));
#108046=CARTESIAN_POINT('Ctrl Pts',(-2.516666969,3.267335925,-6.79918284600001));
#108047=CARTESIAN_POINT('Ctrl Pts',(-2.885565917,3.331598135,-6.662637643));
#108048=CARTESIAN_POINT('Ctrl Pts',(-3.237525941,3.396744076,-6.486981253));
#108049=CARTESIAN_POINT('Ctrl Pts',(-2.832719242,3.267335925,-6.94447274400001));
#108050=CARTESIAN_POINT('Ctrl Pts',(-3.209501092,3.331598135,-6.790779694));
#108051=CARTESIAN_POINT('Ctrl Pts',(-3.567442445,3.396744076,-6.597223234));
#108052=CARTESIAN_POINT('Origin',(0.099567748023463,3.48208258641656,0.167703371500352));
#108053=CARTESIAN_POINT('Ctrl Pts',(-1.758168589,3.396737969,-7.033586796));
#108054=CARTESIAN_POINT('Ctrl Pts',(-1.876402807,3.376870318,-7.004032076));
#108055=CARTESIAN_POINT('Ctrl Pts',(-1.993576877,3.357142857,-6.970520155));
#108056=CARTESIAN_POINT('Ctrl Pts',(-2.258376345,3.312561141,-6.894787199));
#108057=CARTESIAN_POINT('Ctrl Pts',(-2.516666969,3.267335925,-6.799182846));
#108058=CARTESIAN_POINT('Ctrl Pts',(-1.579193193,3.396737969,-7.331858486));
#108059=CARTESIAN_POINT('Ctrl Pts',(-1.702441341,3.376870318,-7.305312333));
#108060=CARTESIAN_POINT('Ctrl Pts',(-1.824727629,3.357142857,-7.274638759));
#108061=CARTESIAN_POINT('Ctrl Pts',(-2.1010801,3.312561141,-7.20532013));
#108062=CARTESIAN_POINT('Ctrl Pts',(-2.37137707,3.267335925,-7.115235119));
#108063=CARTESIAN_POINT('',(-1.76276545951291,3.39596551375301,-7.0324361311284));
#108064=CARTESIAN_POINT('Ctrl Pts',(-1.76276546417588,3.39596551234759,
-7.03243612999851));
#108065=CARTESIAN_POINT('Ctrl Pts',(-1.84016527804476,3.38295904390363,
-7.01303492728227));
#108066=CARTESIAN_POINT('Ctrl Pts',(-1.91712191713628,3.37001483660174,
-6.99238636288139));
#108067=CARTESIAN_POINT('Ctrl Pts',(-1.99357687556294,3.35714285721626,
-6.97052015564213));
#108068=CARTESIAN_POINT('Ctrl Pts',(-2.13557595262986,3.33323585096109,
-6.92990825481634));
#108069=CARTESIAN_POINT('Ctrl Pts',(-2.27682293005017,3.30907945238249,
-6.88481313408911));
#108070=CARTESIAN_POINT('Ctrl Pts',(-2.41689914240186,3.28473845141959,
-6.83528335471055));
#108071=CARTESIAN_POINT('Ctrl Pts',(-2.45022320893918,3.27894773847801,
-6.82350024296103));
#108072=CARTESIAN_POINT('Ctrl Pts',(-2.48348102141939,3.27314659526071,
-6.81146637762032));
#108073=CARTESIAN_POINT('Ctrl Pts',(-2.516666969,3.267335925,-6.799182846));
#108074=CARTESIAN_POINT('Ctrl Pts',(-1.82568833719241,3.35698786877967,
-7.27439771327727));
#108075=CARTESIAN_POINT('Ctrl Pts',(-1.81553619967536,3.36293887933007,
-7.23548805576183));
#108076=CARTESIAN_POINT('Ctrl Pts',(-1.80500598344178,3.36926346353021,
-7.19507767308363));
#108077=CARTESIAN_POINT('Ctrl Pts',(-1.78366980731412,3.38247021627563,
-7.11303601874255));
#108078=CARTESIAN_POINT('Ctrl Pts',(-1.77320129741808,3.38913021757011,
-7.07271166924245));
#108079=CARTESIAN_POINT('Ctrl Pts',(-1.76276545739149,3.39596551349533,
-7.03243613163435));
#108080=CARTESIAN_POINT('Ctrl Pts',(-0.996205363999999,3.267335925,-7.181230735));
#108081=CARTESIAN_POINT('Ctrl Pts',(-1.385832842,3.331598135,-7.127180253));
#108082=CARTESIAN_POINT('Ctrl Pts',(-1.767325168,3.396744076,-7.031291613));
#108083=CARTESIAN_POINT('Ctrl Pts',(-1.273635477,3.267335925,-7.391065733));
#108084=CARTESIAN_POINT('Ctrl Pts',(-1.674647839,3.331598135,-7.321962901));
#108085=CARTESIAN_POINT('Ctrl Pts',(-2.065829641,3.396744076,-7.209878494));
#108086=CARTESIAN_POINT('Origin',(0.0611886336607825,3.48208255128803,0.185186683605522));
#108087=CARTESIAN_POINT('Ctrl Pts',(-0.205050335,3.396737969,-7.247099721));
#108088=CARTESIAN_POINT('Ctrl Pts',(-0.326873693,3.376870318,-7.243652835));
#108089=CARTESIAN_POINT('Ctrl Pts',(-0.448512371,3.357142857,-7.236113367));
#108090=CARTESIAN_POINT('Ctrl Pts',(-0.723401321,3.312561141,-7.21907506300001));
#108091=CARTESIAN_POINT('Ctrl Pts',(-0.996205364,3.267335925,-7.181230735));
#108092=CARTESIAN_POINT('Ctrl Pts',(0.033860313,3.396737969,-7.499923565));
#108093=CARTESIAN_POINT('Ctrl Pts',(-0.092213001,3.376870318,-7.500492755));
#108094=CARTESIAN_POINT('Ctrl Pts',(-0.218234215,3.357142857,-7.496824249));
#108095=CARTESIAN_POINT('Ctrl Pts',(-0.503027175,3.312561141,-7.488533863));
#108096=CARTESIAN_POINT('Ctrl Pts',(-0.786370366,3.267335925,-7.458660848));
#108097=CARTESIAN_POINT('',(-0.209787091585121,3.39596551378162,-7.24696414902478));
#108098=CARTESIAN_POINT('Ctrl Pts',(-0.209787096109259,3.39596551248188,
-7.24696414920313));
#108099=CARTESIAN_POINT('Ctrl Pts',(-0.28954803098352,3.38295904384088,
-7.24465520746408));
#108100=CARTESIAN_POINT('Ctrl Pts',(-0.369144297527101,3.37001483649756,
-7.24103279796689));
#108101=CARTESIAN_POINT('Ctrl Pts',(-0.448512369281491,3.35714285725138,
-7.23611336728682));
#108102=CARTESIAN_POINT('Ctrl Pts',(-0.595921292197588,3.33323595691704,
-7.22697659379603));
#108103=CARTESIAN_POINT('Ctrl Pts',(-0.743559459221487,3.30907966593021,
-7.21329977761382));
#108104=CARTESIAN_POINT('Ctrl Pts',(-0.891007556090164,3.2847387741694,
-7.19504034292312));
#108105=CARTESIAN_POINT('Ctrl Pts',(-0.926086197406635,3.27894795401279,
-7.19069633188629));
#108106=CARTESIAN_POINT('Ctrl Pts',(-0.961154037905286,3.27314670319171,
-7.18609317742572));
#108107=CARTESIAN_POINT('Ctrl Pts',(-0.996205363815112,3.267335925,-7.18123073524444));
#108108=CARTESIAN_POINT('Ctrl Pts',(-0.219224279818265,3.35698786879476,
-7.49679536283724));
#108109=CARTESIAN_POINT('Ctrl Pts',(-0.217673919736165,3.36293888004325,
-7.45661297729563));
#108110=CARTESIAN_POINT('Ctrl Pts',(-0.216076931763992,3.36926346459429,
-7.41488367955715));
#108111=CARTESIAN_POINT('Ctrl Pts',(-0.212876114293901,3.38247021622806,
-7.33017347319156));
#108112=CARTESIAN_POINT('Ctrl Pts',(-0.211320895472024,3.38913021760024,
-7.28854146381554));
#108113=CARTESIAN_POINT('Ctrl Pts',(-0.209787090011592,3.39596551352973,
-7.24696414904142));
#108114=CARTESIAN_POINT('Ctrl Pts',(0.570837696,3.267335925,-7.227492257));
#108115=CARTESIAN_POINT('Ctrl Pts',(0.178700236,3.331598135,-7.258463836));
#108116=CARTESIAN_POINT('Ctrl Pts',(-0.214486235,3.396744076,-7.246826592));
#108117=CARTESIAN_POINT('Ctrl Pts',(0.345002067,3.267335925,-7.492060703));
#108118=CARTESIAN_POINT('Ctrl Pts',(-0.061489915,3.331598135,-7.510779261));
#108119=CARTESIAN_POINT('Ctrl Pts',(-0.467620938,3.396744076,-7.485407848));
#108120=CARTESIAN_POINT('Origin',(0.0199484237424318,3.48208257448395,0.19401088831975));
#108121=CARTESIAN_POINT('Ctrl Pts',(1.357655845,3.396737969,-7.121746317));
#108122=CARTESIAN_POINT('Ctrl Pts',(1.237939671,3.376870318,-7.14456843900001));
#108123=CARTESIAN_POINT('Ctrl Pts',(1.117524075,3.357142857,-7.163353959));
#108124=CARTESIAN_POINT('Ctrl Pts',(0.845399144,3.312561141,-7.205807));
#108125=CARTESIAN_POINT('Ctrl Pts',(0.570837696,3.267335925,-7.227492257));
#108126=CARTESIAN_POINT('Ctrl Pts',(1.645330548,3.396737969,-7.317300553));
#108127=CARTESIAN_POINT('Ctrl Pts',(1.522327117,3.376870318,-7.344958472));
#108128=CARTESIAN_POINT('Ctrl Pts',(1.398463589,3.357142857,-7.36846657));
#108129=CARTESIAN_POINT('Ctrl Pts',(1.118546742,3.312561141,-7.421592076));
#108130=CARTESIAN_POINT('Ctrl Pts',(0.835406142,3.267335925,-7.45332788600001));
#108131=CARTESIAN_POINT('',(1.35300068757869,3.39596551374153,-7.12263217768761));
#108132=CARTESIAN_POINT('Ctrl Pts',(1.35300068233051,3.39596551240205,-7.12263217854008));
#108133=CARTESIAN_POINT('Ctrl Pts',(1.2746081595671,3.38295904372139,-7.13752346249768));
#108134=CARTESIAN_POINT('Ctrl Pts',(1.19609409861221,3.37001483640097,-7.15109658726971));
#108135=CARTESIAN_POINT('Ctrl Pts',(1.11752407593566,3.35714285712236,-7.1633539590213));
#108136=CARTESIAN_POINT('Ctrl Pts',(0.97159705154719,3.33323590700525,-7.18611940684339));
#108137=CARTESIAN_POINT('Ctrl Pts',(0.824470163904568,3.30907956542225,
-7.20450021779076));
#108138=CARTESIAN_POINT('Ctrl Pts',(0.676543772340042,3.28473862232611,
-7.21836467120363));
#108139=CARTESIAN_POINT('Ctrl Pts',(0.641351723076271,3.27894785260945,
-7.22166305847827));
#108140=CARTESIAN_POINT('Ctrl Pts',(0.60611451475454,3.27314665241224,-7.22470604357414));
#108141=CARTESIAN_POINT('Ctrl Pts',(0.570837696373458,3.267335925,-7.22749225731879));
#108142=CARTESIAN_POINT('Ctrl Pts',(1.39749046141673,3.35698786879297,-7.36865119366902));
#108143=CARTESIAN_POINT('Ctrl Pts',(1.39036656336943,3.36293886876702,-7.32907504330461));
#108144=CARTESIAN_POINT('Ctrl Pts',(1.38295561590671,3.36926348197299,-7.28797786324346));
#108145=CARTESIAN_POINT('Ctrl Pts',(1.3678713393157,3.38247029533229,-7.20455966330532));
#108146=CARTESIAN_POINT('Ctrl Pts',(1.36044059487445,3.38913025632477,-7.16356692879642));
#108147=CARTESIAN_POINT('Ctrl Pts',(1.35300068947362,3.39596551352698,-7.12263217749919));
#108148=CARTESIAN_POINT('Ctrl Pts',(2.11118902,3.267335925,-6.935804274));
#108149=CARTESIAN_POINT('Ctrl Pts',(1.73487749,3.331598135,-7.050349716));
#108150=CARTESIAN_POINT('Ctrl Pts',(1.348381837,3.396744076,-7.123508014));
#108151=CARTESIAN_POINT('Ctrl Pts',(1.947507698,3.267335925,-7.242735241));
#108152=CARTESIAN_POINT('Ctrl Pts',(1.554543209,3.331598135,-7.34839993));
#108153=CARTESIAN_POINT('Ctrl Pts',(1.1524532,3.396744076,-7.410927852));
#108154=CARTESIAN_POINT('Origin',(-0.0222246156226963,3.48208256333927,
0.193763563776748));
#108155=CARTESIAN_POINT('Ctrl Pts',(2.856879547,3.396737969,-6.663387971));
#108156=CARTESIAN_POINT('Ctrl Pts',(2.744868352,3.376870318,-6.711411963));
#108157=CARTESIAN_POINT('Ctrl Pts',(2.631306337,3.357142857,-6.755644082));
#108158=CARTESIAN_POINT('Ctrl Pts',(2.374669684,3.312561141,-6.855603411));
#108159=CARTESIAN_POINT('Ctrl Pts',(2.11118902,3.267335925,-6.93580427400001));
#108160=CARTESIAN_POINT('Ctrl Pts',(3.179866955,3.396737969,-6.792528701));
#108161=CARTESIAN_POINT('Ctrl Pts',(3.065684911,3.376870318,-6.845982094));
#108162=CARTESIAN_POINT('Ctrl Pts',(2.94977079,3.357142857,-6.895567583));
#108163=CARTESIAN_POINT('Ctrl Pts',(2.687818656,3.312561141,-7.007624892));
#108164=CARTESIAN_POINT('Ctrl Pts',(2.418119987,3.267335925,-7.099485596));
#108165=CARTESIAN_POINT('',(2.85252365818121,3.39596551374359,-6.66525384216208));
#108166=CARTESIAN_POINT('Ctrl Pts',(2.852523653046,3.39596551231933,-6.66525384416588));
#108167=CARTESIAN_POINT('Ctrl Pts',(2.77916509043875,3.38295904377301,-6.69664905294925));
#108168=CARTESIAN_POINT('Ctrl Pts',(2.70540446510206,3.37001483648196,-6.72678304782433));
#108169=CARTESIAN_POINT('Ctrl Pts',(2.63130633853808,3.35714285723369,-6.75564408156074));
#108170=CARTESIAN_POINT('Ctrl Pts',(2.49368487690778,3.33323590224748,-6.80924729363336));
#108171=CARTESIAN_POINT('Ctrl Pts',(2.3539490363617,3.30907955566733,-6.85882631280321));
#108172=CARTESIAN_POINT('Ctrl Pts',(2.21246149976698,3.28473860750851,-6.90416643206194));
#108173=CARTESIAN_POINT('Ctrl Pts',(2.17880130540959,3.27894784271333,-6.91495294558227));
#108174=CARTESIAN_POINT('Ctrl Pts',(2.14504210403852,3.27314664745598,-6.92549973634016));
#108175=CARTESIAN_POINT('Ctrl Pts',(2.1111890205697,3.267335925,-6.93580427430381));
#108176=CARTESIAN_POINT('Ctrl Pts',(2.94886010157405,3.35698786876897,-6.89595708377018));
#108177=CARTESIAN_POINT('Ctrl Pts',(2.93339505702865,3.36293886751201,-6.85883763699597));
#108178=CARTESIAN_POINT('Ctrl Pts',(2.91732268763635,3.36926348341502,-6.82029440453799));
#108179=CARTESIAN_POINT('Ctrl Pts',(2.88465882512692,3.38247021619802,-6.74206962658919));
#108180=CARTESIAN_POINT('Ctrl Pts',(2.86858947662251,3.38913021753449,-6.70363241886973));
#108181=CARTESIAN_POINT('Ctrl Pts',(2.85252365959883,3.39596551344807,-6.66525384151601));
#108182=CARTESIAN_POINT('Ctrl Pts',(3.552823492,3.267335925,-6.319805791));
#108183=CARTESIAN_POINT('Ctrl Pts',(3.2099338,3.331598135,-6.51256908));
#108184=CARTESIAN_POINT('Ctrl Pts',(2.848201072,3.396744076,-6.667102118));
#108185=CARTESIAN_POINT('Ctrl Pts',(3.458950033,3.267335925,-6.65474752900001));
#108186=CARTESIAN_POINT('Ctrl Pts',(3.09788762,3.331598135,-6.842417585));
#108187=CARTESIAN_POINT('Ctrl Pts',(2.718639907,3.396744076,-6.989921105));
#108188=CARTESIAN_POINT('Origin',(-0.0633584572675827,3.48208260128073,
0.18445584139668));
#108189=CARTESIAN_POINT('Ctrl Pts',(4.222518736,3.396737969,-5.89345701));
#108190=CARTESIAN_POINT('Ctrl Pts',(4.123450039,3.376870318,-5.964437323));
#108191=CARTESIAN_POINT('Ctrl Pts',(4.022051639,3.357142857,-6.032047796));
#108192=CARTESIAN_POINT('Ctrl Pts',(3.79290331,3.312561141,-6.184839426));
#108193=CARTESIAN_POINT('Ctrl Pts',(3.552823492,3.267335925,-6.319805791));
#108194=CARTESIAN_POINT('Ctrl Pts',(4.565716317,3.396737969,-5.950145755));
#108195=CARTESIAN_POINT('Ctrl Pts',(4.465694686,3.376870318,-6.026895202));
#108196=CARTESIAN_POINT('Ctrl Pts',(4.363149987,3.357142857,-6.100239519));
#108197=CARTESIAN_POINT('Ctrl Pts',(4.131411158,3.312561141,-6.265988957));
#108198=CARTESIAN_POINT('Ctrl Pts',(3.88776523,3.267335925,-6.41367925));
#108199=CARTESIAN_POINT('',(4.21866579244059,3.39596551376989,-5.89621564499187));
#108200=CARTESIAN_POINT('Ctrl Pts',(4.21866578869482,3.39596551246601,-5.89621564797497));
#108201=CARTESIAN_POINT('Ctrl Pts',(4.15377134973309,3.38295904378691,-5.94264677680636));
#108202=CARTESIAN_POINT('Ctrl Pts',(4.08821312497822,3.37001483644987,-5.98793260973008));
#108203=CARTESIAN_POINT('Ctrl Pts',(4.02205164047476,3.35714285719441,-6.03204779542876));
#108204=CARTESIAN_POINT('Ctrl Pts',(3.8991708216098,3.33323590672447,-6.11398232501675));
#108205=CARTESIAN_POINT('Ctrl Pts',(3.77335997481717,3.30907956474255,-6.19244127511079));
#108206=CARTESIAN_POINT('Ctrl Pts',(3.644927148364,3.28473862118571,-6.26713699279031));
#108207=CARTESIAN_POINT('Ctrl Pts',(3.61437266836811,3.27894785185105,-6.28490728465918));
#108208=CARTESIAN_POINT('Ctrl Pts',(3.58366996254106,3.27314665203412,-6.30246474160323));
#108209=CARTESIAN_POINT('Ctrl Pts',(3.55282349211638,3.267335925,-6.31980579103262));
#108210=CARTESIAN_POINT('Ctrl Pts',(4.36234432158474,3.35698786875377,-6.10081568471984));
#108211=CARTESIAN_POINT('Ctrl Pts',(4.33926125519902,3.36293886804972,-6.06788859433876));
#108212=CARTESIAN_POINT('Ctrl Pts',(4.31527899933772,3.36926348229613,-6.03370157477921));
#108213=CARTESIAN_POINT('Ctrl Pts',(4.2665627804133,3.38247021623225,-5.96432740782836));
#108214=CARTESIAN_POINT('Ctrl Pts',(4.24260626070832,3.38913021759041,-5.93024327565408));
#108215=CARTESIAN_POINT('Ctrl Pts',(4.21866579364629,3.3959655135348,-5.89621564409636));
#108216=CARTESIAN_POINT('Ctrl Pts',(4.828331886,3.267335925,-5.408300213));
#108217=CARTESIAN_POINT('Ctrl Pts',(4.534897174,3.331598135,-5.670267952));
#108218=CARTESIAN_POINT('Ctrl Pts',(4.214841591,3.396744076,-5.89894993700001));
#108219=CARTESIAN_POINT('Ctrl Pts',(4.808655709,3.267335925,-5.755591218));
#108220=CARTESIAN_POINT('Ctrl Pts',(4.49637825,3.331598135,-6.016491399));
#108221=CARTESIAN_POINT('Ctrl Pts',(4.157706034,3.396744076,-6.242073416));
#108222=CARTESIAN_POINT('Origin',(-0.101529668806381,3.48208256172017,0.166523092993265));
#108223=CARTESIAN_POINT('Ctrl Pts',(5.39071764200001,3.396737969,-4.847954548));
#108224=CARTESIAN_POINT('Ctrl Pts',(5.309223786,3.376870318,-4.93857222300001));
#108225=CARTESIAN_POINT('Ctrl Pts',(5.224730277,3.357142857,-5.026399659));
#108226=CARTESIAN_POINT('Ctrl Pts',(5.033784992,3.312561141,-5.224879222));
#108227=CARTESIAN_POINT('Ctrl Pts',(4.828331886,3.267335925,-5.40830021300001));
#108228=CARTESIAN_POINT('Ctrl Pts',(5.73807786,3.396737969,-4.829540607));
#108229=CARTESIAN_POINT('Ctrl Pts',(5.656893541,3.376870318,-4.92599738900001));
#108230=CARTESIAN_POINT('Ctrl Pts',(5.57251314,3.357142857,-5.019671036));
#108231=CARTESIAN_POINT('Ctrl Pts',(5.38182346500001,3.312561141,-5.231362342));
#108232=CARTESIAN_POINT('Ctrl Pts',(5.17562289100001,3.267335925,-5.42797639));
#108233=CARTESIAN_POINT('',(5.38754780316155,3.39596551374977,-4.85147695721432));
#108234=CARTESIAN_POINT('Ctrl Pts',(5.38754779964328,3.39596551235192,-4.85147696088385));
#108235=CARTESIAN_POINT('Ctrl Pts',(5.33415187731936,3.38295904377502,-4.91077294193955));
#108236=CARTESIAN_POINT('Ctrl Pts',(5.27986148300074,3.37001483647243,-4.9690930976777));
#108237=CARTESIAN_POINT('Ctrl Pts',(5.22473027794813,3.35714285719587,-5.02639965812588));
#108238=CARTESIAN_POINT('Ctrl Pts',(5.12233584940433,3.33323590746412,-5.13283434396295));
#108239=CARTESIAN_POINT('Ctrl Pts',(5.01633274907877,3.30907956627202,-5.23650457710434));
#108240=CARTESIAN_POINT('Ctrl Pts',(4.90695998635107,3.28473862356702,-5.33706320852209));
#108241=CARTESIAN_POINT('Ctrl Pts',(4.88093993712966,3.27894785343848,-5.36098635422923));
#108242=CARTESIAN_POINT('Ctrl Pts',(4.85472937426329,3.27314665282757,-5.38473350510159));
#108243=CARTESIAN_POINT('Ctrl Pts',(4.82833188668483,3.267335925,-5.4083002130388));
#108244=CARTESIAN_POINT('Ctrl Pts',(5.57185016888731,3.35698786876255,-5.02040692549819));
#108245=CARTESIAN_POINT('Ctrl Pts',(5.54222842210733,3.36293886778275,-4.99321183034349));
#108246=CARTESIAN_POINT('Ctrl Pts',(5.51145765308973,3.36926348336969,-4.96497955430138));
#108247=CARTESIAN_POINT('Ctrl Pts',(5.4489666271509,3.38247029552344,-4.90769952435259));
#108248=CARTESIAN_POINT('Ctrl Pts',(5.41824331752566,3.38913025642266,-4.87956238800544));
#108249=CARTESIAN_POINT('Ctrl Pts',(5.38754780472075,3.39596551353952,-4.85147695545905));
#108250=CARTESIAN_POINT('Ctrl Pts',(5.878072847,3.267335925,-4.243908529));
#108251=CARTESIAN_POINT('Ctrl Pts',(5.647813796,3.331598135,-4.562831397));
#108252=CARTESIAN_POINT('Ctrl Pts',(5.384400802,3.396744076,-4.854969413));
#108253=CARTESIAN_POINT('Ctrl Pts',(5.933513989,3.267335925,-4.587309859));
#108254=CARTESIAN_POINT('Ctrl Pts',(5.684623229,3.331598135,-4.909240762));
#108255=CARTESIAN_POINT('Ctrl Pts',(5.402362448,3.396744076,-5.202353312));
#108256=CARTESIAN_POINT('Origin',(-0.134953372141405,3.48208259745366,0.140803901079568));
#108257=CARTESIAN_POINT('Ctrl Pts',(6.306852583,3.396737969,-3.575767121));
#108258=CARTESIAN_POINT('Ctrl Pts',(6.246744129,3.376870318,-3.681784975));
#108259=CARTESIAN_POINT('Ctrl Pts',(6.183106334,3.357142857,-3.785722661));
#108260=CARTESIAN_POINT('Ctrl Pts',(6.039292483,3.312561141,-4.020609474));
#108261=CARTESIAN_POINT('Ctrl Pts',(5.878072847,3.267335925,-4.243908529));
#108262=CARTESIAN_POINT('Ctrl Pts',(6.642133258,3.396737969,-3.483111508));
#108263=CARTESIAN_POINT('Ctrl Pts',(6.58358234,3.376870318,-3.594765413));
#108264=CARTESIAN_POINT('Ctrl Pts',(6.521311771,3.357142857,-3.704388314));
#108265=CARTESIAN_POINT('Ctrl Pts',(6.380587689,3.312561141,-3.952123038));
#108266=CARTESIAN_POINT('Ctrl Pts',(6.221474178,3.267335925,-4.188467387));
#108267=CARTESIAN_POINT('',(6.30451406690207,3.3959655137755,-3.5798885989803));
#108268=CARTESIAN_POINT('Ctrl Pts',(6.30451406510151,3.39596551257587,-3.57988860303183));
#108269=CARTESIAN_POINT('Ctrl Pts',(6.2651133921919,3.38295904390818,-3.64927682231007));
#108270=CARTESIAN_POINT('Ctrl Pts',(6.22462938630305,3.37001483653199,-3.71790431544402));
#108271=CARTESIAN_POINT('Ctrl Pts',(6.18310633484167,3.35714285725499,-3.78572265965193));
#108272=CARTESIAN_POINT('Ctrl Pts',(6.10598607637181,3.33323588697773,-3.91168084524802));
#108273=CARTESIAN_POINT('Ctrl Pts',(6.02474723190066,3.30907952487959,-4.03571496374845));
#108274=CARTESIAN_POINT('Ctrl Pts',(5.93954859646137,3.2847385609158,-4.15743460203448));
#108275=CARTESIAN_POINT('Ctrl Pts',(5.91927972212827,3.27894781160174,-4.18639187393878));
#108276=CARTESIAN_POINT('Ctrl Pts',(5.89878695617026,3.27314663187857,-4.21521822142582));
#108277=CARTESIAN_POINT('Ctrl Pts',(5.87807284737279,3.267335925,-4.24390852893982));
#108278=CARTESIAN_POINT('Ctrl Pts',(6.52082249472828,3.35698786878879,-3.70524951776723));
#108279=CARTESIAN_POINT('Ctrl Pts',(6.48604707793,3.36293887951342,-3.6850579891456));
#108280=CARTESIAN_POINT('Ctrl Pts',(6.44992678160999,3.36926346437347,-3.66410067488437));
#108281=CARTESIAN_POINT('Ctrl Pts',(6.3765835824589,3.38247021627534,-3.62159373779551));
#108282=CARTESIAN_POINT('Ctrl Pts',(6.34052967847699,3.38913021762558,-3.60071889880902));
#108283=CARTESIAN_POINT('Ctrl Pts',(6.30451406744253,3.39596551355646,-3.57988859797397));
#108284=CARTESIAN_POINT('Ctrl Pts',(6.652961655,3.267335925,-2.881076398));
#108285=CARTESIAN_POINT('Ctrl Pts',(6.496644922,3.331598135,-3.242041916));
#108286=CARTESIAN_POINT('Ctrl Pts',(6.302191415,3.396744076,-3.583975916));
#108287=CARTESIAN_POINT('Ctrl Pts',(6.780927749,3.267335925,-3.20453099));
#108288=CARTESIAN_POINT('Ctrl Pts',(6.607061545,3.331598135,-3.572439483));
#108289=CARTESIAN_POINT('Ctrl Pts',(6.394410397,3.396744076,-3.919376949));
#108290=CARTESIAN_POINT('Origin',(-0.162067079264793,3.48208259603613,0.108501079889591));
#108291=CARTESIAN_POINT('Ctrl Pts',(6.928086106,3.396737969,-2.136380796));
#108292=CARTESIAN_POINT('Ctrl Pts',(6.892173659,3.376870318,-2.252841553));
#108293=CARTESIAN_POINT('Ctrl Pts',(6.852367211,3.357142857,-2.368029478));
#108294=CARTESIAN_POINT('Ctrl Pts',(6.76240936900001,3.312561141,-2.628340495));
#108295=CARTESIAN_POINT('Ctrl Pts',(6.652961655,3.267335925,-2.881076398));
#108296=CARTESIAN_POINT('Ctrl Pts',(7.235609888,3.396737969,-1.973815986));
#108297=CARTESIAN_POINT('Ctrl Pts',(7.202430147,3.376870318,-2.095446201));
#108298=CARTESIAN_POINT('Ctrl Pts',(7.165181113,3.357142857,-2.215892511));
#108299=CARTESIAN_POINT('Ctrl Pts',(7.081002724,3.312561141,-2.488086853));
#108300=CARTESIAN_POINT('Ctrl Pts',(6.976416247,3.267335925,-2.753110305));
#108301=CARTESIAN_POINT('',(6.92668825921923,3.39596551374539,-2.14090862877695));
#108302=CARTESIAN_POINT('Ctrl Pts',(6.92668825783294,3.39596551239671,-2.14090863337104));
#108303=CARTESIAN_POINT('Ctrl Pts',(6.90312516711708,3.38295904390286,-2.21714457406198));
#108304=CARTESIAN_POINT('Ctrl Pts',(6.87834053751168,3.37001483658745,-2.29287045883608));
#108305=CARTESIAN_POINT('Ctrl Pts',(6.85236721145235,3.35714285722418,-2.36802947669104));
#108306=CARTESIAN_POINT('Ctrl Pts',(6.80412723414096,3.33323587011083,-2.50762150427388));
#108307=CARTESIAN_POINT('Ctrl Pts',(6.75145133814406,3.30907949095744,-2.64621982014326));
#108308=CARTESIAN_POINT('Ctrl Pts',(6.69441067811292,3.28473850983767,-2.78340900225841));
#108309=CARTESIAN_POINT('Ctrl Pts',(6.68084067475151,3.27894777748228,-2.81604638165472));
#108310=CARTESIAN_POINT('Ctrl Pts',(6.66702387080435,3.2731466147879,-2.84860402807476));
#108311=CARTESIAN_POINT('Ctrl Pts',(6.65296165575154,3.267335925,-2.88107639770267));
#108312=CARTESIAN_POINT('Ctrl Pts',(7.16488840890112,3.35698786873672,-2.21683876059868));
#108313=CARTESIAN_POINT('Ctrl Pts',(7.12658551330807,3.36293886811032,-2.20459500866856));
#108314=CARTESIAN_POINT('Ctrl Pts',(7.08680430148347,3.36926348261331,-2.19189240174846));
#108315=CARTESIAN_POINT('Ctrl Pts',(7.0060376629728,3.38247030444418,-2.16614573658246));
#108316=CARTESIAN_POINT('Ctrl Pts',(6.96633949484734,3.38913026076675,-2.15350955557203));
#108317=CARTESIAN_POINT('Ctrl Pts',(6.92668826046996,3.39596551347636,-2.1409086266833));
#108318=CARTESIAN_POINT('Ctrl Pts',(7.116765371,3.267335925,-1.383528337));
#108319=CARTESIAN_POINT('Ctrl Pts',(7.041700152,3.331598135,-1.769658159));
#108320=CARTESIAN_POINT('Ctrl Pts',(6.925298563,3.396744076,-2.145399688));
#108321=CARTESIAN_POINT('Ctrl Pts',(7.311272864,3.267335925,-1.671911813));
#108322=CARTESIAN_POINT('Ctrl Pts',(7.220561006,3.331598135,-2.068594904));
#108323=CARTESIAN_POINT('Ctrl Pts',(7.087462824,3.396744076,-2.453134876));
#108324=CARTESIAN_POINT('Origin',(-0.181602625130144,3.48208254599677,0.0711247740124582));
#108325=CARTESIAN_POINT('Ctrl Pts',(7.225370023,3.396737969,-0.597099681));
#108326=CARTESIAN_POINT('Ctrl Pts',(7.21533281000001,3.376870318,-0.718557763));
#108327=CARTESIAN_POINT('Ctrl Pts',(7.201219013,3.357142857,-0.839609869));
#108328=CARTESIAN_POINT('Ctrl Pts',(7.16932351,3.312561141,-1.113173236));
#108329=CARTESIAN_POINT('Ctrl Pts',(7.116765371,3.267335925,-1.383528337));
#108330=CARTESIAN_POINT('Ctrl Pts',(7.490757441,3.396737969,-0.372227023));
#108331=CARTESIAN_POINT('Ctrl Pts',(7.484500325,3.376870318,-0.498146254));
#108332=CARTESIAN_POINT('Ctrl Pts',(7.474014549,3.357142857,-0.623784038));
#108333=CARTESIAN_POINT('Ctrl Pts',(7.45031794100001,3.312561141,-0.907710493));
#108334=CARTESIAN_POINT('Ctrl Pts',(7.405148846,3.267335925,-1.189020844));
#108335=CARTESIAN_POINT('',(7.22497820777076,3.39596551374994,-0.601822150741499));
#108336=CARTESIAN_POINT('Ctrl Pts',(7.2249782070017,3.39596551246352,-0.601822155609413));
#108337=CARTESIAN_POINT('Ctrl Pts',(7.21835448240688,3.38295904386693,-0.681341109866494));
#108338=CARTESIAN_POINT('Ctrl Pts',(7.21042813046328,3.37001483652023,-0.760624528247004));
#108339=CARTESIAN_POINT('Ctrl Pts',(7.20121901317613,3.35714285724619,-0.839609867489352));
#108340=CARTESIAN_POINT('Ctrl Pts',(7.18411505685797,3.33323592201497,-0.986308161852371));
#108341=CARTESIAN_POINT('Ctrl Pts',(7.16246529151479,3.30907959556797,-1.13298957017443));
#108342=CARTESIAN_POINT('Ctrl Pts',(7.13624990595926,3.2847386677418,-1.27923308736274));
#108343=CARTESIAN_POINT('Ctrl Pts',(7.13001318165582,3.27894788294406,-1.31402488914406));
#108344=CARTESIAN_POINT('Ctrl Pts',(7.12351828192882,3.2731466676059,-1.3487918764834));
#108345=CARTESIAN_POINT('Ctrl Pts',(7.11676537203918,3.267335925,-1.38352833629909));
#108346=CARTESIAN_POINT('Ctrl Pts',(7.47393210366752,3.35698786876155,-0.624771087536086));
#108347=CARTESIAN_POINT('Ctrl Pts',(7.43389266565902,3.36293886785064,-0.621047578195738));
#108348=CARTESIAN_POINT('Ctrl Pts',(7.39231082795146,3.36926348285857,-0.617193735242564));
#108349=CARTESIAN_POINT('Ctrl Pts',(7.30789826191457,3.38247021624306,-0.609411504751938));
#108350=CARTESIAN_POINT('Ctrl Pts',(7.26641150751208,3.389130217592,-0.605604655336773));
#108351=CARTESIAN_POINT('Ctrl Pts',(7.22497820790518,3.39596551351833,-0.601822148850575));
#108352=CARTESIAN_POINT('Ctrl Pts',(7.247797047,3.267335925,0.178711971));
#108353=CARTESIAN_POINT('Ctrl Pts',(7.257493309,3.331598135,-0.214527153));
#108354=CARTESIAN_POINT('Ctrl Pts',(7.224586446,3.396744076,-0.606506955));
#108355=CARTESIAN_POINT('Ctrl Pts',(7.499750986,3.267335925,-0.061115898));
#108356=CARTESIAN_POINT('Ctrl Pts',(7.496435059,3.331598135,-0.468025127));
#108357=CARTESIAN_POINT('Ctrl Pts',(7.449113366,3.396744076,-0.872186943));
#108358=CARTESIAN_POINT('Origin',(-0.192646482398922,3.4820825457969,0.0304227050463073));
#108359=CARTESIAN_POINT('Ctrl Pts',(7.184803668,3.396737969,0.970101153));
#108360=CARTESIAN_POINT('Ctrl Pts',(7.201111017,3.376870318,0.849324988));
#108361=CARTESIAN_POINT('Ctrl Pts',(7.213349817,3.357142857,0.728068964));
#108362=CARTESIAN_POINT('Ctrl Pts',(7.241008051,3.312561141,0.454044767));
#108363=CARTESIAN_POINT('Ctrl Pts',(7.247797047,3.267335925,0.178711971));
#108364=CARTESIAN_POINT('Ctrl Pts',(7.395645502,3.396737969,1.246766863));
#108365=CARTESIAN_POINT('Ctrl Pts',(7.416603586,3.376870318,1.122446458));
#108366=CARTESIAN_POINT('Ctrl Pts',(7.433371371,3.357142857,0.997491884));
#108367=CARTESIAN_POINT('Ctrl Pts',(7.471264572,3.312561141,0.715109402));
#108368=CARTESIAN_POINT('Ctrl Pts',(7.487624915,3.267335925,0.43066591));
#108369=CARTESIAN_POINT('',(7.18543620481062,3.39596551373394,0.965404863303355));
#108370=CARTESIAN_POINT('Ctrl Pts',(7.18543620520418,3.39596551236943,0.965404858045346));
#108371=CARTESIAN_POINT('Ctrl Pts',(7.19606156435663,3.3829590437794,0.886321106970015));
#108372=CARTESIAN_POINT('Ctrl Pts',(7.20536411729142,3.37001483646942,0.807187359173183));
#108373=CARTESIAN_POINT('Ctrl Pts',(7.21334981711854,3.35714285715552,0.728068965219242));
#108374=CARTESIAN_POINT('Ctrl Pts',(7.22818155036869,3.33323590368426,0.58112343890167));
#108375=CARTESIAN_POINT('Ctrl Pts',(7.2385701157649,3.30907955877851,0.43321718806126));
#108376=CARTESIAN_POINT('Ctrl Pts',(7.24440566172763,3.28473861229339,0.284757116497334));
#108377=CARTESIAN_POINT('Ctrl Pts',(7.24579395134919,3.27894784591094,0.249438128713763));
#108378=CARTESIAN_POINT('Ctrl Pts',(7.24692476879664,3.27314664905907,0.214087875340147));
#108379=CARTESIAN_POINT('Ctrl Pts',(7.24779704733703,3.267335925,0.178711971354076));
#108380=CARTESIAN_POINT('Ctrl Pts',(7.43350303989333,3.35698786876789,0.996510188147964));
#108381=CARTESIAN_POINT('Ctrl Pts',(7.39359918051022,3.36293887930503,0.991539338669348));
#108382=CARTESIAN_POINT('Ctrl Pts',(7.35216123765737,3.36926346403428,0.98636423935489));
#108383=CARTESIAN_POINT('Ctrl Pts',(7.26804866643108,3.38247028762204,0.975818247058842));
#108384=CARTESIAN_POINT('Ctrl Pts',(7.22671373276374,3.38913025251371,0.970617699024864));
#108385=CARTESIAN_POINT('Ctrl Pts',(7.18543620457005,3.39596551344063,0.965404864874389));
#108386=CARTESIAN_POINT('Ctrl Pts',(7.039929788,3.267335925,1.732595906));
#108387=CARTESIAN_POINT('Ctrl Pts',(7.133934145,3.331598135,1.350634904));
#108388=CARTESIAN_POINT('Ctrl Pts',(7.186060697,3.396744076,0.960745369));
#108389=CARTESIAN_POINT('Ctrl Pts',(7.337549087,3.267335925,1.552537729));
#108390=CARTESIAN_POINT('Ctrl Pts',(7.421784141,3.331598135,1.154428985));
#108391=CARTESIAN_POINT('Ctrl Pts',(7.462451646,3.396744076,0.749543483));
#108392=CARTESIAN_POINT('Origin',(-0.194682376371735,3.48208258157526,-0.0117018368190408));
#108393=CARTESIAN_POINT('Ctrl Pts',(6.808283879,3.396737969,2.491941134));
#108394=CARTESIAN_POINT('Ctrl Pts',(6.850173276,3.376870318,2.377494247));
#108395=CARTESIAN_POINT('Ctrl Pts',(6.888192401,3.357142857,2.261704102));
#108396=CARTESIAN_POINT('Ctrl Pts',(6.974111103,3.312561141,2.00003214));
#108397=CARTESIAN_POINT('Ctrl Pts',(7.039929788,3.267335925,1.732595906));
#108398=CARTESIAN_POINT('Ctrl Pts',(6.954721399,3.396737969,2.807463316));
#108399=CARTESIAN_POINT('Ctrl Pts',(7.001914706,3.376870318,2.690554822));
#108400=CARTESIAN_POINT('Ctrl Pts',(7.04515201,3.357142857,2.572126194));
#108401=CARTESIAN_POINT('Ctrl Pts',(7.142863175,3.312561141,2.304491575));
#108402=CARTESIAN_POINT('Ctrl Pts',(7.219987966,3.267335925,2.030215204));
#108403=CARTESIAN_POINT('',(6.80991119073934,3.39596551375276,2.48749061769332));
#108404=CARTESIAN_POINT('Ctrl Pts',(6.80991119222407,3.39596551241334,2.48749061268678));
#108405=CARTESIAN_POINT('Ctrl Pts',(6.83728880486597,3.38295904379503,2.41253993402923));
#108406=CARTESIAN_POINT('Ctrl Pts',(6.86338528591401,3.37001483647005,2.33725606338888));
#108407=CARTESIAN_POINT('Ctrl Pts',(6.88819240069204,3.35714285718407,2.26170410317289));
#108408=CARTESIAN_POINT('Ctrl Pts',(6.93426633835587,3.3332358944779,2.12138241075397));
#108409=CARTESIAN_POINT('Ctrl Pts',(6.97620751152916,3.30907954004391,1.97916730415587));
#108410=CARTESIAN_POINT('Ctrl Pts',(7.01382116403914,3.2847385838048,1.83543255897252));
#108411=CARTESIAN_POINT('Ctrl Pts',(7.02276951907545,3.27894782689033,1.80123780666515));
#108412=CARTESIAN_POINT('Ctrl Pts',(7.03147314347654,3.27314663953617,1.76695717111046));
#108413=CARTESIAN_POINT('Ctrl Pts',(7.03992978840013,3.267335925,1.73259590666138));
#108414=CARTESIAN_POINT('Ctrl Pts',(7.045491636111,3.35698786875769,2.57119575441533));
#108415=CARTESIAN_POINT('Ctrl Pts',(7.00758936241169,3.36293886830875,2.55776299522492));
#108416=CARTESIAN_POINT('Ctrl Pts',(6.96823253199427,3.36926348165724,2.54380089152843));
#108417=CARTESIAN_POINT('Ctrl Pts',(6.88835362328747,3.38247029190796,2.51541977092196));
#108418=CARTESIAN_POINT('Ctrl Pts',(6.84910305541214,3.38913025463968,2.5014550247814));
#108419=CARTESIAN_POINT('Ctrl Pts',(6.80991119013386,3.39596551352048,2.48749061958343));
#108420=CARTESIAN_POINT('Ctrl Pts',(6.502883238,3.267335925,3.205465582));
#108421=CARTESIAN_POINT('Ctrl Pts',(6.676800149,3.331598135,2.852642774));
#108422=CARTESIAN_POINT('Ctrl Pts',(6.811522736,3.396744076,2.483074308));
#108423=CARTESIAN_POINT('Ctrl Pts',(6.832251548,3.267335925,3.093596417));
#108424=CARTESIAN_POINT('Ctrl Pts',(7.000098845,3.331598135,2.722903281));
#108425=CARTESIAN_POINT('Ctrl Pts',(7.126853981,3.396744076,2.336226088));
#108426=CARTESIAN_POINT('Origin',(-0.187615177368009,3.48208256415948,-0.0532791725642151));
#108427=CARTESIAN_POINT('Ctrl Pts',(6.113416303,3.396737969,3.897260718));
#108428=CARTESIAN_POINT('Ctrl Pts',(6.178929047,3.376870318,3.794494518));
#108429=CARTESIAN_POINT('Ctrl Pts',(6.240950764,3.357142857,3.68958447));
#108430=CARTESIAN_POINT('Ctrl Pts',(6.381112471,3.312561141,3.452500234));
#108431=CARTESIAN_POINT('Ctrl Pts',(6.502883238,3.267335925,3.205465582));
#108432=CARTESIAN_POINT('Ctrl Pts',(6.188602252,3.396737969,4.236885904));
#108433=CARTESIAN_POINT('Ctrl Pts',(6.259824077,3.376870318,4.132855832));
#108434=CARTESIAN_POINT('Ctrl Pts',(6.327509171,3.357142857,4.026490742));
#108435=CARTESIAN_POINT('Ctrl Pts',(6.480469435,3.312561141,3.786118284));
#108436=CARTESIAN_POINT('Ctrl Pts',(6.614752403,3.267335925,3.534833892));
#108437=CARTESIAN_POINT('',(6.11596229868539,3.39596551374412,3.89326407617423));
#108438=CARTESIAN_POINT('Ctrl Pts',(6.11596230129545,3.39596551235726,3.89326407151603));
#108439=CARTESIAN_POINT('Ctrl Pts',(6.15881202082059,3.3829590437766,3.82595107545144));
#108440=CARTESIAN_POINT('Ctrl Pts',(6.20048218733259,3.37001483646751,3.75803727209581));
#108441=CARTESIAN_POINT('Ctrl Pts',(6.24095076366032,3.35714285712456,3.68958447086456));
#108442=CARTESIAN_POINT('Ctrl Pts',(6.31611262983619,3.33323586399187,3.5624477948108));
#108443=CARTESIAN_POINT('Ctrl Pts',(6.38764537173352,3.30907947870888,3.43257354309568));
#108444=CARTESIAN_POINT('Ctrl Pts',(6.45527843514372,3.28473849130112,3.3002848860287));
#108445=CARTESIAN_POINT('Ctrl Pts',(6.47136835562607,3.27894776510738,3.26881338576536));
#108446=CARTESIAN_POINT('Ctrl Pts',(6.48723773182478,3.27314660859326,3.23720540176058));
#108447=CARTESIAN_POINT('Ctrl Pts',(6.502883238,3.267335925,3.205465582));
#108448=CARTESIAN_POINT('Ctrl Pts',(6.32804087382115,3.35698786876481,4.02565506518012));
#108449=CARTESIAN_POINT('Ctrl Pts',(6.29391238080765,3.36293886823552,4.00438848822485));
#108450=CARTESIAN_POINT('Ctrl Pts',(6.25847712951975,3.36926348181522,3.98229225475981));
#108451=CARTESIAN_POINT('Ctrl Pts',(6.18656726015517,3.38247021623562,3.93740332255877));
#108452=CARTESIAN_POINT('Ctrl Pts',(6.15123613580125,3.38913021753919,3.91532721514912));
#108453=CARTESIAN_POINT('Ctrl Pts',(6.11596229760619,3.39596551350274,3.89326407782484));
#108454=CARTESIAN_POINT('Ctrl Pts',(5.66176909400001,3.267335925,4.528451251));
#108455=CARTESIAN_POINT('Ctrl Pts',(5.907466399,3.331598135,4.221264238));
#108456=CARTESIAN_POINT('Ctrl Pts',(6.11848554200001,3.396744076,3.889297452));
#108457=CARTESIAN_POINT('Ctrl Pts',(6.00748552,3.267335925,4.490001975));
#108458=CARTESIAN_POINT('Ctrl Pts',(6.251096707,3.331598135,4.164057646));
#108459=CARTESIAN_POINT('Ctrl Pts',(6.458012545,3.396744076,3.813669358));
#108460=CARTESIAN_POINT('Origin',(-0.171775537985642,3.48208257530023,-0.0923653531614632));
#108461=CARTESIAN_POINT('Ctrl Pts',(5.132692175,3.396737969,5.120348722));
#108462=CARTESIAN_POINT('Ctrl Pts',(5.218764963,3.376870318,5.03406844200001));
#108463=CARTESIAN_POINT('Ctrl Pts',(5.301889206,3.357142857,4.944943968));
#108464=CARTESIAN_POINT('Ctrl Pts',(5.489740113,3.312561141,4.743533254));
#108465=CARTESIAN_POINT('Ctrl Pts',(5.661769094,3.267335925,4.52845125));
#108466=CARTESIAN_POINT('Ctrl Pts',(5.133110943,3.396737969,5.468196417));
#108467=CARTESIAN_POINT('Ctrl Pts',(5.22503103100001,3.376870318,5.381909097));
#108468=CARTESIAN_POINT('Ctrl Pts',(5.313999035,3.357142857,5.292581058));
#108469=CARTESIAN_POINT('Ctrl Pts',(5.51505614700001,3.312561141,5.09071031));
#108470=CARTESIAN_POINT('Ctrl Pts',(5.70021837,3.267335925,4.874167676));
#108471=CARTESIAN_POINT('',(5.13603780693678,3.39596551375112,5.11699283301184));
#108472=CARTESIAN_POINT('Ctrl Pts',(5.13603781027852,3.39596551232431,5.11699282926967));
#108473=CARTESIAN_POINT('Ctrl Pts',(5.19235603125485,3.38295904386035,5.06046499702263));
#108474=CARTESIAN_POINT('Ctrl Pts',(5.24765143270648,3.37001483656328,5.0030968345882));
#108475=CARTESIAN_POINT('Ctrl Pts',(5.30188920504041,3.35714285723109,4.9449439694496));
#108476=CARTESIAN_POINT('Ctrl Pts',(5.40262434824966,3.33323588965341,4.8369373737601));
#108477=CARTESIAN_POINT('Ctrl Pts',(5.50040371818527,3.30907953040397,4.72547705731968));
#108478=CARTESIAN_POINT('Ctrl Pts',(5.59489361499051,3.28473856932848,4.61082047448819));
#108479=CARTESIAN_POINT('Ctrl Pts',(5.61737290688907,3.27894781722051,4.58354349694134));
#108480=CARTESIAN_POINT('Ctrl Pts',(5.63966614902101,3.27314663469309,4.55608581445833));
#108481=CARTESIAN_POINT('Ctrl Pts',(5.6617690941662,3.267335925,4.52845125149442));
#108482=CARTESIAN_POINT('Ctrl Pts',(5.31469795297972,3.35698786870842,5.29187921908844));
#108483=CARTESIAN_POINT('Ctrl Pts',(5.28593899785827,3.36293887909632,5.26377317423017));
#108484=CARTESIAN_POINT('Ctrl Pts',(5.25608237635442,3.36926346364826,5.23457613979773));
#108485=CARTESIAN_POINT('Ctrl Pts',(5.19550343018046,3.38247021624225,5.17527810805215));
#108486=CARTESIAN_POINT('Ctrl Pts',(5.165744038557,3.38913021751788,5.14612298051144));
#108487=CARTESIAN_POINT('Ctrl Pts',(5.13603780535955,3.39596551346047,5.11699283455206));
#108488=CARTESIAN_POINT('Ctrl Pts',(4.55591692,3.267335925,5.639691571));
#108489=CARTESIAN_POINT('Ctrl Pts',(4.861906086,3.331598135,5.392504079));
#108490=CARTESIAN_POINT('Ctrl Pts',(5.139354765,3.396744076,5.113661369));
#108491=CARTESIAN_POINT('Ctrl Pts',(4.901816146,3.267335925,5.67646003));
#108492=CARTESIAN_POINT('Ctrl Pts',(5.209800235,3.331598135,5.410505303));
#108493=CARTESIAN_POINT('Ctrl Pts',(5.48720162,3.396744076,5.112789687));
#108494=CARTESIAN_POINT('Origin',(-0.147903616601148,3.48208256703089,-0.127132486034253));
#108495=CARTESIAN_POINT('Ctrl Pts',(3.911969065,3.396737969,6.104014911));
#108496=CARTESIAN_POINT('Ctrl Pts',(4.014577229,3.376870318,6.03825492));
#108497=CARTESIAN_POINT('Ctrl Pts',(4.114917201,3.357142857,5.969083383));
#108498=CARTESIAN_POINT('Ctrl Pts',(4.341673608,3.312561141,5.812763932));
#108499=CARTESIAN_POINT('Ctrl Pts',(4.55591692,3.267335925,5.639691571));
#108500=CARTESIAN_POINT('Ctrl Pts',(3.837601071,3.396737969,6.44382014200001));
#108501=CARTESIAN_POINT('Ctrl Pts',(3.945921342,3.376870318,6.379310274));
#108502=CARTESIAN_POINT('Ctrl Pts',(4.052012211,3.357142857,6.311196166));
#108503=CARTESIAN_POINT('Ctrl Pts',(4.291764963,3.312561141,6.157266379));
#108504=CARTESIAN_POINT('Ctrl Pts',(4.519148461,3.267335925,5.985590797));
#108505=CARTESIAN_POINT('',(3.91595789500395,3.39596551384657,6.10145669215797));
#108506=CARTESIAN_POINT('Ctrl Pts',(3.91595789925708,3.39596551228061,6.10145668921002));
#108507=CARTESIAN_POINT('Ctrl Pts',(3.98311124483374,3.38295904374827,6.05835719870953));
#108508=CARTESIAN_POINT('Ctrl Pts',(4.04944632971667,3.37001483646856,6.01421714884346));
#108509=CARTESIAN_POINT('Ctrl Pts',(4.11491719996409,3.35714285720156,5.9690833837649));
#108510=CARTESIAN_POINT('Ctrl Pts',(4.23651531527283,3.3332359135643,5.88525708363404));
#108511=CARTESIAN_POINT('Ctrl Pts',(4.35596921437483,3.30907957859659,5.79742241323709));
#108512=CARTESIAN_POINT('Ctrl Pts',(4.4728976542248,3.28473864218913,5.70575907122463));
#108513=CARTESIAN_POINT('Ctrl Pts',(4.50071525452162,3.27894786587584,5.68395210780971));
#108514=CARTESIAN_POINT('Ctrl Pts',(4.52838999981166,3.27314665905663,5.66192866720594));
#108515=CARTESIAN_POINT('Ctrl Pts',(4.55591691995108,3.267335925,5.63969157146022));
#108516=CARTESIAN_POINT('Ctrl Pts',(4.05284566323258,3.35698786873722,6.31066098193971));
#108517=CARTESIAN_POINT('Ctrl Pts',(4.03080108981236,3.36293886711398,6.27702978340556));
#108518=CARTESIAN_POINT('Ctrl Pts',(4.00791888511499,3.36926348337905,6.24209689463089));
#108519=CARTESIAN_POINT('Ctrl Pts',(3.96150363406496,3.38247021623708,6.17116264113993));
#108520=CARTESIAN_POINT('Ctrl Pts',(3.93870749073462,3.38913021755258,6.13629175453415));
#108521=CARTESIAN_POINT('Ctrl Pts',(3.91595789307705,3.39596551346942,6.10145669334236));
#108522=CARTESIAN_POINT('Ctrl Pts',(3.237035134,3.267335925,6.487226182));
#108523=CARTESIAN_POINT('Ctrl Pts',(3.589008448,3.331598135,6.311596421));
#108524=CARTESIAN_POINT('Ctrl Pts',(3.919913471,3.396744076,6.098916164));
#108525=CARTESIAN_POINT('Ctrl Pts',(3.566943297,3.267335925,6.597493124));
#108526=CARTESIAN_POINT('Ctrl Pts',(3.924899294,3.331598135,6.403963745));
#108527=CARTESIAN_POINT('Ctrl Pts',(4.259815245,3.396744076,6.172841653));
#108528=CARTESIAN_POINT('Origin',(-0.11711599026234,3.48208228754832,-0.155955219364179));
#108529=CARTESIAN_POINT('Ctrl Pts',(2.50832663,3.396737969,6.802264146));
#108530=CARTESIAN_POINT('Ctrl Pts',(2.622672326,3.376870318,6.76009931));
#108531=CARTESIAN_POINT('Ctrl Pts',(2.735536241,3.357142857,6.714115092));
#108532=CARTESIAN_POINT('Ctrl Pts',(2.99059527,3.312561141,6.610196228));
#108533=CARTESIAN_POINT('Ctrl Pts',(3.237035134,3.267335925,6.487226182));
#108534=CARTESIAN_POINT('Ctrl Pts',(2.362649238,3.396737969,7.118138));
#108535=CARTESIAN_POINT('Ctrl Pts',(2.482304756,3.376870318,7.078421992));
#108536=CARTESIAN_POINT('Ctrl Pts',(2.600557799,3.357142857,7.034706755));
#108537=CARTESIAN_POINT('Ctrl Pts',(2.867795619,3.312561141,6.935915516));
#108538=CARTESIAN_POINT('Ctrl Pts',(3.126768193,3.267335925,6.817134344));
#108539=CARTESIAN_POINT('',(2.51277214475068,3.39596551375339,6.80062321798605));
#108540=CARTESIAN_POINT('Ctrl Pts',(2.51277214949544,3.39596551225138,6.80062321598465));
#108541=CARTESIAN_POINT('Ctrl Pts',(2.58762060356924,3.38295904370181,6.77296735215514));
#108542=CARTESIAN_POINT('Ctrl Pts',(2.66189361690341,3.37001483643105,6.74411935425174));
#108543=CARTESIAN_POINT('Ctrl Pts',(2.73553623993914,3.3571428571487,6.71411509284571));
#108544=CARTESIAN_POINT('Ctrl Pts',(2.87231202328787,3.33323584566299,6.65838844796532));
#108545=CARTESIAN_POINT('Ctrl Pts',(3.00785539350867,3.30907944181061,6.598286178192));
#108546=CARTESIAN_POINT('Ctrl Pts',(3.1417553897474,3.28473843554526,6.53390182583033));
#108547=CARTESIAN_POINT('Ctrl Pts',(3.17361009877579,3.27894772834719,6.51858483652433));
#108548=CARTESIAN_POINT('Ctrl Pts',(3.2053718310647,3.27314659089702,6.50302572734794));
#108549=CARTESIAN_POINT('Ctrl Pts',(3.23703512624063,3.26733592642395,6.48722618587181));
#108550=CARTESIAN_POINT('Ctrl Pts',(2.60148681409268,3.35698786873481,7.03436325144702));
#108551=CARTESIAN_POINT('Ctrl Pts',(2.58718731604156,3.36293887879503,6.99677932612183));
#108552=CARTESIAN_POINT('Ctrl Pts',(2.57234969575745,3.36926346386341,6.9577443421693));
#108553=CARTESIAN_POINT('Ctrl Pts',(2.54226833099559,3.38247021621572,6.87849046822266));
#108554=CARTESIAN_POINT('Ctrl Pts',(2.52750135875675,3.38913021753285,6.83953434665205));
#108555=CARTESIAN_POINT('Ctrl Pts',(2.51277214241879,3.39596551346009,6.80062321881723));
#108556=CARTESIAN_POINT('Ctrl Pts',(1.766793184,3.267335925,7.031425307));
#108557=CARTESIAN_POINT('Ctrl Pts',(2.148292764,3.331598135,6.93556553));
#108558=CARTESIAN_POINT('Ctrl Pts',(2.51718138,3.396744076,6.798992418));
#108559=CARTESIAN_POINT('Ctrl Pts',(2.065284143,3.267335925,7.21003477200001));
#108560=CARTESIAN_POINT('Ctrl Pts',(2.456474424,3.331598135,7.097979961));
#108561=CARTESIAN_POINT('Ctrl Pts',(2.833244645,3.396744076,6.944258404));
#108562=CARTESIAN_POINT('Origin',(-0.0808521869256668,3.48208254633516,
-0.177485595265519));
#108563=CARTESIAN_POINT('Ctrl Pts',(0.98739763,3.396737969,7.182447071));
#108564=CARTESIAN_POINT('Ctrl Pts',(1.10813418,3.376870318,7.165848969));
#108565=CARTESIAN_POINT('Ctrl Pts',(1.228244647,3.357142857,7.145202243));
#108566=CARTESIAN_POINT('Ctrl Pts',(1.499680022,3.312561141,7.098543095));
#108567=CARTESIAN_POINT('Ctrl Pts',(1.766793184,3.267335925,7.031425307));
#108568=CARTESIAN_POINT('Ctrl Pts',(0.777222552,3.396737969,7.459619635));
#108569=CARTESIAN_POINT('Ctrl Pts',(0.902618358,3.376870318,7.446554566));
#108570=CARTESIAN_POINT('Ctrl Pts',(1.027504195,3.357142857,7.429282275));
#108571=CARTESIAN_POINT('Ctrl Pts',(1.309731339,3.312561141,7.390248953));
#108572=CARTESIAN_POINT('Ctrl Pts',(1.588183719,3.267335925,7.329916267));
#108573=CARTESIAN_POINT('',(0.992091960819354,3.3959655138041,7.18180016023131));
#108574=CARTESIAN_POINT('Ctrl Pts',(0.992091965201248,3.39596551263151,
7.18180016009836));
#108575=CARTESIAN_POINT('Ctrl Pts',(1.07113569834774,3.38295904380298,7.17088107956549));
#108576=CARTESIAN_POINT('Ctrl Pts',(1.14987371695153,3.37001483640952,7.15867403457068));
#108577=CARTESIAN_POINT('Ctrl Pts',(1.22824464557595,3.35714285718804,7.14520224359184));
#108578=CARTESIAN_POINT('Ctrl Pts',(1.3738017716988,3.33323592741606,7.12018129133799));
#108579=CARTESIAN_POINT('Ctrl Pts',(1.51909593195878,3.30907960644241,7.09062211347458));
#108580=CARTESIAN_POINT('Ctrl Pts',(1.663705666322,3.28473868418063,7.05652771971352));
#108581=CARTESIAN_POINT('Ctrl Pts',(1.69810882624232,3.27894789392113,7.04841654458334));
#108582=CARTESIAN_POINT('Ctrl Pts',(1.73247323072682,3.27314667310194,7.04004891557619));
#108583=CARTESIAN_POINT('Ctrl Pts',(1.766793184,3.267335925,7.031425307));
#108584=CARTESIAN_POINT('Ctrl Pts',(1.02848533315043,3.35698786876585,7.4291465131798));
#108585=CARTESIAN_POINT('Ctrl Pts',(1.02259958178645,3.36293887945333,7.38936730565414));
#108586=CARTESIAN_POINT('Ctrl Pts',(1.01650022449133,3.36926346446715,7.34805528870315));
#108587=CARTESIAN_POINT('Ctrl Pts',(1.00415932290298,3.38247028390876,7.26418729613533));
#108588=CARTESIAN_POINT('Ctrl Pts',(0.99811204299841,3.38913025079369,7.22296771414462));
#108589=CARTESIAN_POINT('Ctrl Pts',(0.992091959548617,3.39596551362997,
7.18180016038823));
#108590=CARTESIAN_POINT('Ctrl Pts',(0.213937947,3.267335925,7.246842799));
#108591=CARTESIAN_POINT('Ctrl Pts',(0.607125298,3.331598135,7.235235304));
#108592=CARTESIAN_POINT('Ctrl Pts',(0.996748685,3.396744076,7.181155343));
#108593=CARTESIAN_POINT('Ctrl Pts',(0.467054599,3.267335925,7.485443207));
#108594=CARTESIAN_POINT('Ctrl Pts',(0.87318754,3.331598135,7.460102522));
#108595=CARTESIAN_POINT('Ctrl Pts',(1.274194673,3.396744076,7.39096935));
#108596=CARTESIAN_POINT('Origin',(-0.0408077614185605,3.48208260746332,
-0.190716837355268));
#108597=CARTESIAN_POINT('Ctrl Pts',(-0.579700987,3.396737969,7.226786752));
#108598=CARTESIAN_POINT('Ctrl Pts',(-0.458219089,3.376870318,7.236531495));
#108599=CARTESIAN_POINT('Ctrl Pts',(-0.336478302,3.357142857,7.242187677));
#108600=CARTESIAN_POINT('Ctrl Pts',(-0.061358598,3.312561141,7.254969977));
#108601=CARTESIAN_POINT('Ctrl Pts',(0.213937947,3.267335925,7.24684279900001));
#108602=CARTESIAN_POINT('Ctrl Pts',(-0.844546196,3.396737969,7.452297748));
#108603=CARTESIAN_POINT('Ctrl Pts',(-0.71927347,3.376870318,7.46649452400001));
#108604=CARTESIAN_POINT('Ctrl Pts',(-0.593594363,3.357142857,7.476472814));
#108605=CARTESIAN_POINT('Ctrl Pts',(-0.309574522,3.312561141,7.499022561));
#108606=CARTESIAN_POINT('Ctrl Pts',(-0.02466246,3.267335925,7.499959451));
#108607=CARTESIAN_POINT('Ctrl Pts',(-0.574977340788912,3.39596551522583,
7.22716410353705));
#108608=CARTESIAN_POINT('Ctrl Pts',(-0.455851638000001,3.376486685,7.23664148900001));
#108609=CARTESIAN_POINT('Ctrl Pts',(-0.336478302,3.357142857,7.242187677));
#108610=CARTESIAN_POINT('Ctrl Pts',(-0.0613585965077572,3.31256114087447,
7.25496997652748));
#108611=CARTESIAN_POINT('Ctrl Pts',(0.213937950575229,3.26733592689007,
7.24684279957603));
#108612=CARTESIAN_POINT('Ctrl Pts',(0.178686009732229,2.48690656550041,
7.24784936885964));
#108613=CARTESIAN_POINT('Ctrl Pts',(0.192365848366114,2.48917367225018,
7.24746042942977));
#108614=CARTESIAN_POINT('Ctrl Pts',(0.206045687,2.491440779,7.24707149000001));
#108615=CARTESIAN_POINT('Ctrl Pts',(0.602789375,2.557191576,7.23579144));
#108616=CARTESIAN_POINT('Ctrl Pts',(0.995930671,2.622066995,7.18126883600001));
#108617=CARTESIAN_POINT('Ctrl Pts',(0.4311616098954,2.48690656550041,7.48817560011827));
#108618=CARTESIAN_POINT('Ctrl Pts',(0.445293291484062,2.48917367225018,
7.48730837266027));
#108619=CARTESIAN_POINT('Ctrl Pts',(0.459424973072718,2.491440779,7.48644114520224));
#108620=CARTESIAN_POINT('Ctrl Pts',(0.869273043739099,2.557191576,7.46128975056695));
#108621=CARTESIAN_POINT('Ctrl Pts',(1.27392616352466,2.622066995,7.39154817726272));
#108622=CARTESIAN_POINT('',(0.458902333983518,2.4914407798504,7.4859474130173));
#108623=CARTESIAN_POINT('',(1.02398864463363,2.58208164081247,7.42976765664733));
#108624=CARTESIAN_POINT('Origin',(0.001328250839037,2.41074793646468,-0.189950586860783));
#108625=CARTESIAN_POINT('Ctrl Pts',(0.991263375970751,2.62129679704272,
7.18191457174322));
#108626=CARTESIAN_POINT('Ctrl Pts',(0.996664707245066,2.61444751350223,
7.22317185246287));
#108627=CARTESIAN_POINT('Ctrl Pts',(1.00209692939513,2.60775977698502,7.26447633270777));
#108628=CARTESIAN_POINT('Ctrl Pts',(1.01300518115998,2.59469807325527,7.34708108552444));
#108629=CARTESIAN_POINT('Ctrl Pts',(1.0184871761395,2.58831697879642,7.38842649747231));
#108630=CARTESIAN_POINT('Ctrl Pts',(1.02398863945874,2.58208164077288,7.42976764544215));
#108631=CARTESIAN_POINT('',(0.332473999383933,2.49144078146678,7.36650945118224));
#108632=CARTESIAN_POINT('Origin',(2.89210929510508E-14,2.58316965300033,
2.78423117894278E-13));
#108633=CARTESIAN_POINT('',(1.02346990113142,2.40074633455656,7.42983912063183));
#108634=CARTESIAN_POINT('Origin',(-0.00170106791189131,2.55355106829602,
-0.190812554157955));
#108635=CARTESIAN_POINT('',(1.58020016870039,2.49144077881204,7.33164152797676));
#108636=CARTESIAN_POINT('Origin',(-0.0278993116906279,2.41071458311704,
-0.19085055781879));
#108637=CARTESIAN_POINT('Origin',(-0.0308560152959829,2.55357125325729,
-0.190428015594565));
#108638=CARTESIAN_POINT('Ctrl Pts',(0.9866149,2.622074631,7.182554632));
#108639=CARTESIAN_POINT('Ctrl Pts',(1.376928915,2.556767114,7.128940056));
#108640=CARTESIAN_POINT('Ctrl Pts',(1.759134602,2.491440779,7.033345253));
#108641=CARTESIAN_POINT('Ctrl Pts',(0.776409618,2.622074631,7.459704291));
#108642=CARTESIAN_POINT('Ctrl Pts',(1.181784486,2.556767114,7.417512679));
#108643=CARTESIAN_POINT('Ctrl Pts',(1.580200173,2.491440779,7.331641522));
#108644=CARTESIAN_POINT('Ctrl Pts',(0.77430756518,2.622074631,7.46247578759));
#108645=CARTESIAN_POINT('Ctrl Pts',(1.17983304171,2.556767114,7.42039840523));
#108646=CARTESIAN_POINT('Ctrl Pts',(1.57841082871,2.491440779,7.33462448469001));
#108647=CARTESIAN_POINT('',(1.6696673844688,2.49144077849314,7.18249338820464));
#108648=CARTESIAN_POINT('Ctrl Pts',(1.73258179986369,2.48690656552405,7.03998646724969));
#108649=CARTESIAN_POINT('Ctrl Pts',(1.74585820093184,2.489173672262,7.03666586012479));
#108650=CARTESIAN_POINT('Ctrl Pts',(1.759134602,2.491440779,7.033345253));
#108651=CARTESIAN_POINT('Ctrl Pts',(2.144177766,2.557191576,6.93704076));
#108652=CARTESIAN_POINT('Ctrl Pts',(2.516406889,2.622066995,6.799279107));
#108653=CARTESIAN_POINT('Ctrl Pts',(2.03081769670521,2.48690656552405,7.22041921463527));
#108654=CARTESIAN_POINT('Ctrl Pts',(2.04443255908916,2.489173672262,7.21653436867755));
#108655=CARTESIAN_POINT('Ctrl Pts',(2.05804742147311,2.491440779,7.21264952271985));
#108656=CARTESIAN_POINT('Ctrl Pts',(2.45290666554322,2.557191576,7.09998093342908));
#108657=CARTESIAN_POINT('Ctrl Pts',(2.83310684298389,2.622066995,6.94488142061167));
#108658=CARTESIAN_POINT('',(2.05743086091823,2.49144077985044,7.21227968580291));
#108659=CARTESIAN_POINT('',(2.59722878304874,2.58208164080325,7.03593652810296));
#108660=CARTESIAN_POINT('Origin',(-0.0395365885006085,2.41074795151913,
-0.185795251756038));
#108661=CARTESIAN_POINT('Ctrl Pts',(2.51198752636068,2.62129679696105,6.80091307643713));
#108662=CARTESIAN_POINT('Ctrl Pts',(2.52613167332026,2.61444751340273,6.84004465842731));
#108663=CARTESIAN_POINT('Ctrl Pts',(2.54031613545444,2.60775977687909,6.879215695743));
#108664=CARTESIAN_POINT('Ctrl Pts',(2.56872693491772,2.5946980747769,6.95754423388337));
#108665=CARTESIAN_POINT('Ctrl Pts',(2.58296880150041,2.58831698191966,6.99674453567385));
#108666=CARTESIAN_POINT('Ctrl Pts',(2.59722877560764,2.58208164077717,7.03593651817469));
#108667=CARTESIAN_POINT('',(1.908282721884,2.49144078146678,7.1228124714158));
#108668=CARTESIAN_POINT('Origin',(7.42678488152571E-13,2.58316965300044,
2.05521363816352E-12));
#108669=CARTESIAN_POINT('',(2.59673753012003,2.40074633453864,7.0361178357593));
#108670=CARTESIAN_POINT('Origin',(-0.0426803276019039,2.55355106469629,
-0.185985695722827));
#108671=CARTESIAN_POINT('',(3.119342175801,2.4914407788122,6.82053549638486));
#108672=CARTESIAN_POINT('Origin',(-0.0682743477746839,2.41071456818591,
-0.180391257391022));
#108673=CARTESIAN_POINT('Origin',(-0.071070994550492,2.55357129094536,-0.179342759647155));
#108674=CARTESIAN_POINT('Ctrl Pts',(2.507585323,2.622074631,6.802537457));
#108675=CARTESIAN_POINT('Ctrl Pts',(2.877248464,2.556767114,6.666270384));
#108676=CARTESIAN_POINT('Ctrl Pts',(3.229968338,2.491440779,6.49074761));
#108677=CARTESIAN_POINT('Ctrl Pts',(2.361873508,2.622074631,7.118395433));
#108678=CARTESIAN_POINT('Ctrl Pts',(2.748700987,2.556767114,6.990046624));
#108679=CARTESIAN_POINT('Ctrl Pts',(3.119342177,2.491440779,6.820535491));
#108680=CARTESIAN_POINT('Ctrl Pts',(2.36041638985,2.622074631,7.12155401276));
#108681=CARTESIAN_POINT('Ctrl Pts',(2.74741551223,2.556767114,6.9932843864));
#108682=CARTESIAN_POINT('Ctrl Pts',(3.11823591539,2.491440779,6.82383336981));
#108683=CARTESIAN_POINT('',(3.17465525469772,2.49144077849433,6.65564155183665));
#108684=CARTESIAN_POINT('Ctrl Pts',(3.2054639914271,2.48690656571219,6.50294162341348));
#108685=CARTESIAN_POINT('Ctrl Pts',(3.21771616471352,2.48917367235607,6.49684461670674));
#108686=CARTESIAN_POINT('Ctrl Pts',(3.229968338,2.491440779,6.49074761));
#108687=CARTESIAN_POINT('Ctrl Pts',(3.585306787,2.557191576,6.313921764));
#108688=CARTESIAN_POINT('Ctrl Pts',(3.919218717,2.622066995,6.099362643));
#108689=CARTESIAN_POINT('Ctrl Pts',(3.53551500587727,2.4869065657122,6.61504405117166));
#108690=CARTESIAN_POINT('Ctrl Pts',(3.54797643276839,2.48917367235607,6.60832323804217));
#108691=CARTESIAN_POINT('Ctrl Pts',(3.56043785965957,2.491440779,6.6016024249127));
#108692=CARTESIAN_POINT('Ctrl Pts',(3.92184509740445,2.557191576,6.40668489823342));
#108693=CARTESIAN_POINT('Ctrl Pts',(4.25981459571951,2.622066995,6.17347972708782));
#108694=CARTESIAN_POINT('',(3.55975620996069,2.49144077985043,6.60137377688286));
#108695=CARTESIAN_POINT('',(4.04902538988259,2.58208164076325,6.31311282687116));
#108696=CARTESIAN_POINT('Origin',(-0.0785528899479215,2.41074794720924,
-0.172952521176576));
#108697=CARTESIAN_POINT('Ctrl Pts',(3.91525393165237,2.62129679694602,6.10190844352683));
#108698=CARTESIAN_POINT('Ctrl Pts',(3.93747952956042,2.61444751341348,6.13708457730189));
#108699=CARTESIAN_POINT('Ctrl Pts',(3.95975298189506,2.60775977689882,6.17229057739767));
#108700=CARTESIAN_POINT('Ctrl Pts',(4.00433788126619,2.59469807234326,6.24268036890378));
#108701=CARTESIAN_POINT('Ctrl Pts',(4.02667369633177,2.5883169770036,6.27790262364398));
#108702=CARTESIAN_POINT('Ctrl Pts',(4.0490253804682,2.58208164071723,6.31311281894294));
#108703=CARTESIAN_POINT('',(3.39486226506754,2.49144078146677,6.54606069746623));
#108704=CARTESIAN_POINT('Origin',(7.0906822080552E-14,2.58316965300056,
1.24032728532342E-13));
#108705=CARTESIAN_POINT('',(4.04858459835607,2.40074633454437,6.31339550070062));
#108706=CARTESIAN_POINT('Origin',(-0.081663894348511,2.55355105428733,-0.172462402234757));
#108707=CARTESIAN_POINT('',(4.51262720696831,2.4914407788122,5.99050880554589));
#108708=CARTESIAN_POINT('Origin',(-0.105456859430594,2.41071461865303,-0.161496726585507));
#108709=CARTESIAN_POINT('Origin',(-0.10796268082271,2.55357129252955,-0.159871514079931));
#108710=CARTESIAN_POINT('Ctrl Pts',(3.911303843,2.622074631,6.104441191));
#108711=CARTESIAN_POINT('Ctrl Pts',(4.243031073,2.556767114,5.891893318));
#108712=CARTESIAN_POINT('Ctrl Pts',(4.549772344,2.491440779,5.644649822));
#108713=CARTESIAN_POINT('Ctrl Pts',(3.836898817,2.622074631,6.444238315));
#108714=CARTESIAN_POINT('Ctrl Pts',(4.187091285,2.556767114,6.235733757));
#108715=CARTESIAN_POINT('Ctrl Pts',(4.512627207,2.491440779,5.99050880000001));
#108716=CARTESIAN_POINT('Ctrl Pts',(3.83615476674,2.622074631,6.44763628624));
#108717=CARTESIAN_POINT('Ctrl Pts',(4.18653188712,2.556767114,6.23917216139));
#108718=CARTESIAN_POINT('Ctrl Pts',(4.51225575563,2.491440779,5.99396738978001));
#108719=CARTESIAN_POINT('',(4.53119977305058,2.49144077849433,5.8175793129078));
#108720=CARTESIAN_POINT('Ctrl Pts',(4.52846224709165,2.48690656555413,5.66182645693944));
#108721=CARTESIAN_POINT('Ctrl Pts',(4.53911729554583,2.48917367227704,5.6532381394697));
#108722=CARTESIAN_POINT('Ctrl Pts',(4.549772344,2.491440779,5.644649822));
#108723=CARTESIAN_POINT('Ctrl Pts',(4.85879084800001,2.557191576,5.395570803));
#108724=CARTESIAN_POINT('Ctrl Pts',(5.138772234,2.622066995,5.114246761));
#108725=CARTESIAN_POINT('Ctrl Pts',(4.87489556037499,2.48690656555413,5.70035678045006));
#108726=CARTESIAN_POINT('Ctrl Pts',(4.88562087025615,2.48917367227704,5.69111425748587));
#108727=CARTESIAN_POINT('Ctrl Pts',(4.89634618013719,2.491440779,5.68187173452161));
#108728=CARTESIAN_POINT('Ctrl Pts',(5.20740241124098,2.557191576,5.41381939934162));
#108729=CARTESIAN_POINT('Ctrl Pts',(5.48733815209132,2.622066995,5.11341298321399));
#108730=CARTESIAN_POINT('',(4.89563131445871,2.49144077985042,5.6817949666801));
#108731=CARTESIAN_POINT('',(5.31149407010535,2.58208164084134,5.29509498696339));
#108732=CARTESIAN_POINT('Origin',(-0.113895876282957,2.41074793632891,-0.15202226988008));
#108733=CARTESIAN_POINT('Ctrl Pts',(5.13544741496347,2.62129679693993,5.11758535379643));
#108734=CARTESIAN_POINT('Ctrl Pts',(5.16471521985902,2.61444751339497,5.14716124259995));
#108735=CARTESIAN_POINT('Ctrl Pts',(5.19403618067066,2.6077597768829,5.17675601218363));
#108736=CARTESIAN_POINT('Ctrl Pts',(5.25271042576565,2.59469807426784,5.23591568543397));
#108737=CARTESIAN_POINT('Ctrl Pts',(5.28209577596687,2.5883169808747,5.26551291392302));
#108738=CARTESIAN_POINT('Ctrl Pts',(5.31149405920984,2.58208164081004,5.29509498109586));
#108739=CARTESIAN_POINT('',(4.72270182137915,2.49144078146676,5.66322240019092));
#108740=CARTESIAN_POINT('Origin',(-6.40546643504436E-13,2.58316965300033,
-6.43148728718401E-13));
#108741=CARTESIAN_POINT('',(5.31112435035526,2.40074633451093,5.29546580931694));
#108742=CARTESIAN_POINT('Origin',(-0.116828924643203,2.55355111047958,-0.1508749981619));
#108743=CARTESIAN_POINT('',(5.69490680501467,2.49144077881248,4.8803725837289));
#108744=CARTESIAN_POINT('Origin',(-0.137708370212528,2.41071459951173,-0.135050933525499));
#108745=CARTESIAN_POINT('Origin',(-0.139806310418847,2.55357127476894,-0.132925095633139));
#108746=CARTESIAN_POINT('Ctrl Pts',(5.132134143,2.622074631,5.120908039));
#108747=CARTESIAN_POINT('Ctrl Pts',(5.410414265,2.556767114,4.842017869));
#108748=CARTESIAN_POINT('Ctrl Pts',(5.656834052,2.491440779,4.534614483));
#108749=CARTESIAN_POINT('Ctrl Pts',(5.132515003,2.622074631,5.468755777));
#108750=CARTESIAN_POINT('Ctrl Pts',(5.429697849,2.556767114,5.18984491));
#108751=CARTESIAN_POINT('Ctrl Pts',(5.694906805,2.491440779,4.880372576));
#108752=CARTESIAN_POINT('Ctrl Pts',(5.1325188116,2.622074631,5.47223425438));
#108753=CARTESIAN_POINT('Ctrl Pts',(5.42989068484001,2.556767114,5.19332318041001));
#108754=CARTESIAN_POINT('Ctrl Pts',(5.69528753253,2.491440779,4.88383015693));
#108755=CARTESIAN_POINT('',(5.67587042651797,2.49144077849433,4.70749353188976));
#108756=CARTESIAN_POINT('Ctrl Pts',(5.63971464197941,2.4869065655115,4.55597057888841));
#108757=CARTESIAN_POINT('Ctrl Pts',(5.64827434698972,2.48917367225572,4.54529253094417));
#108758=CARTESIAN_POINT('Ctrl Pts',(5.65683405200001,2.491440779,4.534614483));
#108759=CARTESIAN_POINT('Ctrl Pts',(5.905083248,2.557191576,4.224928949));
#108760=CARTESIAN_POINT('Ctrl Pts',(6.118042472,2.622066995,3.889994385));
#108761=CARTESIAN_POINT('Ctrl Pts',(5.98633141772411,2.4869065655115,4.51912716241547));
#108762=CARTESIAN_POINT('Ctrl Pts',(5.99481910667497,2.48917367225572,4.50779509979886));
#108763=CARTESIAN_POINT('Ctrl Pts',(6.00330679562579,2.491440779,4.49646303718222));
#108764=CARTESIAN_POINT('Ctrl Pts',(6.24946737655826,2.557191576,4.1678097214174));
#108765=CARTESIAN_POINT('Ctrl Pts',(6.45827987534397,2.622066995,3.81424873074632));
#108766=CARTESIAN_POINT('',(6.00259214027373,2.49144077985043,4.49654173912977));
#108767=CARTESIAN_POINT('',(6.32560319063832,2.5820816408139,4.02948439011544));
#108768=CARTESIAN_POINT('Origin',(-0.14391329291115,2.41074795037636,-0.123983781589465));
#108769=CARTESIAN_POINT('Ctrl Pts',(6.11551308426914,2.6212967969781,3.89396966096671));
#108770=CARTESIAN_POINT('Ctrl Pts',(6.15045456600537,2.61444751341353,3.91656236895765));
#108771=CARTESIAN_POINT('Ctrl Pts',(6.18545201972378,2.60775977688574,3.93916208936406));
#108772=CARTESIAN_POINT('Ctrl Pts',(6.25547208577829,2.59469807216963,3.98432542110109));
#108773=CARTESIAN_POINT('Ctrl Pts',(6.29053296465008,2.58831697663297,4.00691370917541));
#108774=CARTESIAN_POINT('Ctrl Pts',(6.32560317876756,2.58208164076528,4.02948438689549));
#108775=CARTESIAN_POINT('',(5.82971308973407,2.49144078146677,4.51557811846253));
#108776=CARTESIAN_POINT('Origin',(1.00527225432856E-12,2.58316965300022,
6.98876720384156E-13));
#108777=CARTESIAN_POINT('',(6.3253218305668,2.4007463345075,4.02992602189079));
#108778=CARTESIAN_POINT('Origin',(-0.146531164652753,2.553551096683,-0.122232832307339));
#108779=CARTESIAN_POINT('',(6.61089889168057,2.49144077881248,3.54203556251265));
#108780=CARTESIAN_POINT('Origin',(-0.163520847235297,2.41071460928183,-0.102290334524298));
#108781=CARTESIAN_POINT('Origin',(-0.16511287802337,2.55357127486387,-0.0997632859032118));
#108782=CARTESIAN_POINT('Ctrl Pts',(6.11299155399999,2.622074631,3.897926919));
#108783=CARTESIAN_POINT('Ctrl Pts',(6.324812498,2.556767114,3.565735045));
#108784=CARTESIAN_POINT('Ctrl Pts',(6.499388487,2.491440779,3.21254561));
#108785=CARTESIAN_POINT('Ctrl Pts',(6.188140491,2.622074631,4.237560296));
#108786=CARTESIAN_POINT('Ctrl Pts',(6.418417775,2.556767114,3.901284683));
#108787=CARTESIAN_POINT('Ctrl Pts',(6.61089889,2.491440779,3.542035555));
#108788=CARTESIAN_POINT('Ctrl Pts',(6.18889198036999,2.622074631,4.24095662977));
#108789=CARTESIAN_POINT('Ctrl Pts',(6.41935382777,2.556767114,3.90464017938));
#108790=CARTESIAN_POINT('Ctrl Pts',(6.61201399403,2.491440779,3.54533045445));
#108791=CARTESIAN_POINT('',(6.55514368707803,2.49144077849433,3.37729058525997));
#108792=CARTESIAN_POINT('Ctrl Pts',(6.48726024865665,2.48690656555131,3.23708257910937));
#108793=CARTESIAN_POINT('Ctrl Pts',(6.49332436782831,2.48917367227563,3.22481409455469));
#108794=CARTESIAN_POINT('Ctrl Pts',(6.499388487,2.491440779,3.21254561));
#108795=CARTESIAN_POINT('Ctrl Pts',(6.67526052,2.557191576,2.856734113));
#108796=CARTESIAN_POINT('Ctrl Pts',(6.81123984400001,2.622066995,2.483850194));
#108797=CARTESIAN_POINT('Ctrl Pts',(6.817853071007,2.48690656555132,3.12658818021115));
#108798=CARTESIAN_POINT('Ctrl Pts',(6.82370626395992,2.48917367227563,3.11369645281647));
#108799=CARTESIAN_POINT('Ctrl Pts',(6.829559456913,2.491440779,3.10080472542187));
#108800=CARTESIAN_POINT('Ctrl Pts',(6.99931419211015,2.557191576,2.72691789345473));
#108801=CARTESIAN_POINT('Ctrl Pts',(7.12723960977484,2.622066995,2.33673444670107));
#108802=CARTESIAN_POINT('',(6.82887843004262,2.4914407798504,3.10103521501192));
#108803=CARTESIAN_POINT('',(7.04393413620837,2.58208164078061,2.5754595818908));
#108804=CARTESIAN_POINT('Origin',(-0.1672016121272,2.41074790913348,-0.0901480503329738));
#108805=CARTESIAN_POINT('Ctrl Pts',(6.8096241586967,2.6212967969834,2.48827627384362));
#108806=CARTESIAN_POINT('Ctrl Pts',(6.84860541200244,2.61444752754034,2.50282936134758));
#108807=CARTESIAN_POINT('Ctrl Pts',(6.88764282530724,2.6077598055919,2.51737726108904));
#108808=CARTESIAN_POINT('Ctrl Pts',(6.96573480727117,2.59469807329946,2.5464325162797));
#108809=CARTESIAN_POINT('Ctrl Pts',(7.00483178883872,2.58831697892964,2.56095564735769));
#108810=CARTESIAN_POINT('Ctrl Pts',(7.04393412388175,2.58208164074236,2.57545958120439));
#108811=CARTESIAN_POINT('',(6.66413345302227,2.49144078146678,3.15679042217479));
#108812=CARTESIAN_POINT('Origin',(-1.67834496300756E-12,2.58316965299956,
-6.07586897460877E-13));
#108813=CARTESIAN_POINT('',(7.04375429213915,2.40074633454149,2.57595137240142));
#108814=CARTESIAN_POINT('Origin',(-0.169381858058412,2.55355109385969,-0.0878752584789577));
#108815=CARTESIAN_POINT('',(7.21777269325484,2.49144077881249,2.03807689497822));
#108816=CARTESIAN_POINT('Origin',(-0.181687328975315,2.41071460036769,-0.0647467316436268));
#108817=CARTESIAN_POINT('Origin',(-0.18269865670645,2.55357127027427,-0.061936443737653));
#108818=CARTESIAN_POINT('Ctrl Pts',(6.808012274,2.622074631,2.492683068));
#108819=CARTESIAN_POINT('Ctrl Pts',(6.943469529,2.556767114,2.122722415));
#108820=CARTESIAN_POINT('Ctrl Pts',(7.03803874,2.491440779,1.740261674));
#108821=CARTESIAN_POINT('Ctrl Pts',(6.954415407,2.622074631,2.808221206));
#108822=CARTESIAN_POINT('Ctrl Pts',(7.10701962,2.556767114,2.430304721));
#108823=CARTESIAN_POINT('Ctrl Pts',(7.21777269,2.491440779,2.038076888));
#108824=CARTESIAN_POINT('Ctrl Pts',(6.95587943833001,2.622074631,2.81137658738));
#108825=CARTESIAN_POINT('Ctrl Pts',(7.10865512091,2.556767114,2.43338054406));
#108826=CARTESIAN_POINT('Ctrl Pts',(7.2195700295,2.491440779,2.04105504014));
#108827=CARTESIAN_POINT('',(7.12790571420459,2.49144077849433,1.88916928400112));
#108828=CARTESIAN_POINT('Ctrl Pts',(7.03146877638639,2.48690656567176,1.76683219441741));
#108829=CARTESIAN_POINT('Ctrl Pts',(7.03475375819324,2.48917367233585,1.7535469342087));
#108830=CARTESIAN_POINT('Ctrl Pts',(7.03803874,2.491440779,1.740261674));
#108831=CARTESIAN_POINT('Ctrl Pts',(7.133310028,2.557191576,1.354961564));
#108832=CARTESIAN_POINT('Ctrl Pts',(7.18595121099999,2.622066995,0.961563929));
#108833=CARTESIAN_POINT('Ctrl Pts',(7.33057949286396,2.48690656567176,1.58785340997492));
#108834=CARTESIAN_POINT('Ctrl Pts',(7.33352450100962,2.48917367233585,1.5740048208671));
#108835=CARTESIAN_POINT('Ctrl Pts',(7.33646950915533,2.491440779,1.56015623175923));
#108836=CARTESIAN_POINT('Ctrl Pts',(7.42188085561533,2.557191576,1.15851841490154));
#108837=CARTESIAN_POINT('Ctrl Pts',(7.46293754093156,2.622066995,0.749957057554851));
#108838=CARTESIAN_POINT('',(7.33585395163772,2.49144077985043,1.56052773568837));
#108839=CARTESIAN_POINT('',(7.43289855053669,2.58208164078526,1.00100914581307));
#108840=CARTESIAN_POINT('Origin',(-0.182671872314275,2.4107479441789,-0.0520970523417763));
#108841=CARTESIAN_POINT('Ctrl Pts',(7.18532477592665,2.62129679696926,0.96623385415251));
#108842=CARTESIAN_POINT('Ctrl Pts',(7.22652323753413,2.61444751346219,0.972066893244294));
#108843=CARTESIAN_POINT('Ctrl Pts',(7.26777544245234,2.6077597769625,0.97788279460163));
#108844=CARTESIAN_POINT('Ctrl Pts',(7.35028750978922,2.59469807451361,0.989471259813259));
#108845=CARTESIAN_POINT('Ctrl Pts',(7.39159246099731,2.58831698137499,0.995250151657246));
#108846=CARTESIAN_POINT('Ctrl Pts',(7.43289853829811,2.58208164075722,1.0010091477115));
#108847=CARTESIAN_POINT('',(7.18694634311339,2.49144078146678,1.65039471424761));
#108848=CARTESIAN_POINT('Origin',(9.08995101411847E-13,2.583169653,1.07634170673498E-13));
#108849=CARTESIAN_POINT('',(7.43282863131921,2.40074633450192,1.00152810022529));
#108850=CARTESIAN_POINT('Origin',(-0.184312290055271,2.55355107458263,-0.0494086632345077));
#108851=CARTESIAN_POINT('',(7.48715146569616,2.4914407788124,0.438820016134038));
#108852=CARTESIAN_POINT('Origin',(-0.191357879378022,2.41071461740584,-0.0241755478479756));
#108853=CARTESIAN_POINT('Origin',(-0.191741974367537,2.55357130245492,-0.0212136133590121));
#108854=CARTESIAN_POINT('Ctrl Pts',(7.184697907,2.622074631,0.970884128));
#108855=CARTESIAN_POINT('Ctrl Pts',(7.237457642,2.556767114,0.580453643));
#108856=CARTESIAN_POINT('Ctrl Pts',(7.247598124,2.491440779,0.186605037));
#108857=CARTESIAN_POINT('Ctrl Pts',(7.395509589,2.622074631,1.247572813));
#108858=CARTESIAN_POINT('Ctrl Pts',(7.46330512600001,2.556767114,0.845686411));
#108859=CARTESIAN_POINT('Ctrl Pts',(7.487151461,2.491440779,0.43882001));
#108860=CARTESIAN_POINT('Ctrl Pts',(7.39761770582,2.622074631,1.25033969985));
#108861=CARTESIAN_POINT('Ctrl Pts',(7.46556360084,2.556767114,0.84833873868));
#108862=CARTESIAN_POINT('Ctrl Pts',(7.48954699437,2.491440779,0.44134215973));
#108863=CARTESIAN_POINT('',(7.36737479236834,2.49144077849433,0.312712526601943));
#108864=CARTESIAN_POINT('Ctrl Pts',(7.24689363902624,2.48690656569715,0.213966701214266));
#108865=CARTESIAN_POINT('Ctrl Pts',(7.24724588151317,2.48917367234855,0.200285869107131));
#108866=CARTESIAN_POINT('Ctrl Pts',(7.247598124,2.491440779,0.186605037));
#108867=CARTESIAN_POINT('Ctrl Pts',(7.257813887,2.557191576,-0.210167481));
#108868=CARTESIAN_POINT('Ctrl Pts',(7.224655486,2.622066995,-0.605683996));
#108869=CARTESIAN_POINT('Ctrl Pts',(7.500536164337,2.48690656569716,-0.0251276215615274));
#108870=CARTESIAN_POINT('Ctrl Pts',(7.50043528254417,2.48917367234855,-0.0392855279489237));
#108871=CARTESIAN_POINT('Ctrl Pts',(7.50033440075132,2.491440779,-0.0534434343363214));
#108872=CARTESIAN_POINT('Ctrl Pts',(7.49740861943488,2.557191576,-0.464052096364095));
#108873=CARTESIAN_POINT('Ctrl Pts',(7.44967680768896,2.622066995,-0.871887489814411));
#108874=CARTESIAN_POINT('',(7.49981309758335,2.4914407798504,-0.05294829189469));
#108875=CARTESIAN_POINT('',(7.47430888983564,2.58208164080481,-0.620247365094564));
#108876=CARTESIAN_POINT('Origin',(-0.189600407854941,2.41074793233023,-0.011610007931523));
#108877=CARTESIAN_POINT('Ctrl Pts',(7.22504759239769,2.62129679701665,-0.600988586287213));
#108878=CARTESIAN_POINT('Ctrl Pts',(7.26653670335673,2.61444752746288,-0.604148365421792));
#108879=CARTESIAN_POINT('Ctrl Pts',(7.30807460570636,2.60775980536993,-0.607336433764565));
#108880=CARTESIAN_POINT('Ctrl Pts',(7.39114895381358,2.59469807312342,-0.613756570528413));
#108881=CARTESIAN_POINT('Ctrl Pts',(7.43273051931852,2.58831697852743,-0.616992130316176));
#108882=CARTESIAN_POINT('Ctrl Pts',(7.47430887837775,2.58208164076432,-0.620247360527366));
#108883=CARTESIAN_POINT('',(7.37370560986287,2.49144078146676,0.0668283836306943));
#108884=CARTESIAN_POINT('Origin',(-5.95010152260045E-13,2.58316965300044,
1.45659173741639E-13));
#108885=CARTESIAN_POINT('',(7.47435216511153,2.40074633456696,-0.619725513626632));
#108886=CARTESIAN_POINT('Origin',(-0.190624814482888,2.55355107517748,-0.00863181457063135));
#108887=CARTESIAN_POINT('',(7.40643935690458,2.49144077881248,-1.18095559800117));
#108888=CARTESIAN_POINT('Origin',(-0.192081249505737,2.41071462784453,0.0175259825687855));
#108889=CARTESIAN_POINT('Origin',(-0.191819194414465,2.55357127695176,0.0205011828761191));
#108890=CARTESIAN_POINT('Ctrl Pts',(7.225435051,2.622074631,-0.596312275));
#108891=CARTESIAN_POINT('Ctrl Pts',(7.19303028,2.556767114,-0.988956496));
#108892=CARTESIAN_POINT('Ctrl Pts',(7.118267874,2.491440779,-1.375777044));
#108893=CARTESIAN_POINT('Ctrl Pts',(7.490797961,2.622074631,-0.371410698));
#108894=CARTESIAN_POINT('Ctrl Pts',(7.47061478,2.556767114,-0.778475256));
#108895=CARTESIAN_POINT('Ctrl Pts',(7.406439351,2.491440779,-1.180955603));
#108896=CARTESIAN_POINT('Ctrl Pts',(7.49345159010001,2.622074631,-0.36916168223));
#108897=CARTESIAN_POINT('Ctrl Pts',(7.473390625,2.556767114,-0.7763704436));
#108898=CARTESIAN_POINT('Ctrl Pts',(7.40932106577,2.491440779,-1.17900738859));
#108899=CARTESIAN_POINT('',(7.26235361303824,2.49144077849433,-1.27836632044227));
#108900=CARTESIAN_POINT('Ctrl Pts',(7.1234618085242,2.48690656562793,-1.34890363637193));
#108901=CARTESIAN_POINT('Ctrl Pts',(7.12086484126211,2.48917367231394,-1.36234034018596));
#108902=CARTESIAN_POINT('Ctrl Pts',(7.118267874,2.491440779,-1.375777044));
#108903=CARTESIAN_POINT('Ctrl Pts',(7.042950436,2.557191576,-1.765469329));
#108904=CARTESIAN_POINT('Ctrl Pts',(6.925542901,2.622066995,-2.144610811));
#108905=CARTESIAN_POINT('Ctrl Pts',(7.31977610096884,2.48690656562794,-1.63693371243211));
#108906=CARTESIAN_POINT('Ctrl Pts',(7.31663404633257,2.48917367231394,-1.65073892846223));
#108907=CARTESIAN_POINT('Ctrl Pts',(7.31349199169623,2.491440779,-1.66454414449235));
#108908=CARTESIAN_POINT('Ctrl Pts',(7.22236588906184,2.557191576,-2.06492404823634));
#108909=CARTESIAN_POINT('Ctrl Pts',(7.08807746581271,2.622066995,-2.45296354767138));
#108910=CARTESIAN_POINT('',(7.31308931728985,2.49144077985038,-1.66394851343346));
#108911=CARTESIAN_POINT('',(7.16622885233626,2.58208164074841,-2.21250179872927));
#108912=CARTESIAN_POINT('Origin',(-0.187663248092902,2.41074796270394,0.029419856961789));
#108913=CARTESIAN_POINT('Ctrl Pts',(6.92693521466089,2.62129679693166,-2.14010946824839));
#108914=CARTESIAN_POINT('Ctrl Pts',(6.96677515560324,2.6144475133313,-2.15211433059853));
#108915=CARTESIAN_POINT('Ctrl Pts',(7.00665667656492,2.60775977678319,-2.16415731290675));
#108916=CARTESIAN_POINT('Ctrl Pts',(7.08640817575413,2.59469812265093,-2.1882857354475));
#108917=CARTESIAN_POINT('Ctrl Pts',(7.12632169586457,2.58831707916653,-2.20038435307007));
#108918=CARTESIAN_POINT('Ctrl Pts',(7.16622884238419,2.58208164067141,-2.21250179179743));
#108919=CARTESIAN_POINT('',(7.21567859711874,2.49144078146676,-1.51986276769353));
#108920=CARTESIAN_POINT('Origin',(8.62157567560473E-13,2.58316965299989,
-2.5576329248933E-13));
#108921=CARTESIAN_POINT('',(7.16638329838829,2.40074633454233,-2.21200145070765));
#108922=CARTESIAN_POINT('Origin',(-0.188023568116957,2.55355108735271,0.0325486569326483));
#108923=CARTESIAN_POINT('',(6.97941037431554,2.49144077881229,-2.74551104348949));
#108924=CARTESIAN_POINT('Origin',(-0.183822865911698,2.41071459369151,0.0584079944944987));
#108925=CARTESIAN_POINT('Origin',(-0.182927537906269,2.55357125929785,0.0612573726347116));
#108926=CARTESIAN_POINT('Ctrl Pts',(6.928318882,2.622074631,-2.135625779));
#108927=CARTESIAN_POINT('Ctrl Pts',(6.812264815,2.556767114,-2.512124128));
#108928=CARTESIAN_POINT('Ctrl Pts',(6.65609533,2.491440779,-2.873829319));
#108929=CARTESIAN_POINT('Ctrl Pts',(7.235824946,2.622074631,-1.973027457));
#108930=CARTESIAN_POINT('Ctrl Pts',(7.128606789,2.556767114,-2.366236285));
#108931=CARTESIAN_POINT('Ctrl Pts',(6.979410369,2.491440779,-2.745511045));
#108932=CARTESIAN_POINT('Ctrl Pts',(7.23890000664,2.622074631,-1.97140147378));
#108933=CARTESIAN_POINT('Ctrl Pts',(7.13177020874,2.556767114,-2.36477740657));
#108934=CARTESIAN_POINT('Ctrl Pts',(6.98264351939001,2.491440779,-2.74422786226));
#108935=CARTESIAN_POINT('',(6.81775285068297,2.49144077849433,-2.80967017912947));
#108936=CARTESIAN_POINT('Ctrl Pts',(6.66694482167319,2.48690656554502,-2.848700738649));
#108937=CARTESIAN_POINT('Ctrl Pts',(6.66152007583659,2.48917367227249,-2.86126502882453));
#108938=CARTESIAN_POINT('Ctrl Pts',(6.65609533,2.491440779,-2.873829319));
#108939=CARTESIAN_POINT('Ctrl Pts',(6.49876645,2.557191576,-3.238219792));
#108940=CARTESIAN_POINT('Ctrl Pts',(6.302599626,2.622066995,-3.583258008));
#108941=CARTESIAN_POINT('Ctrl Pts',(6.79675144311513,2.48690656554502,-3.17219860169431));
#108942=CARTESIAN_POINT('Ctrl Pts',(6.79071513448913,2.48917367227249,-3.18500561081046));
#108943=CARTESIAN_POINT('Ctrl Pts',(6.78467882586311,2.491440779,-3.19781261992669));
#108944=CARTESIAN_POINT('Ctrl Pts',(6.60961335660931,2.557191576,-3.56924244559905));
#108945=CARTESIAN_POINT('Ctrl Pts',(6.39504749997121,2.622066995,-3.91934175583024));
#108946=CARTESIAN_POINT('',(6.78441360938226,2.49144077985043,-3.19714434868294));
#108947=CARTESIAN_POINT('',(6.52306391845758,2.58208164080626,-3.70130210716894));
#108948=CARTESIAN_POINT('Origin',(-0.176951405087596,2.41074795767547,0.0690740987240757));
#108949=CARTESIAN_POINT('Ctrl Pts',(6.30492704362086,2.6212967969752,-3.57916121053907));
#108950=CARTESIAN_POINT('Ctrl Pts',(6.34125478323769,2.6144475275756,-3.59944977361168));
#108951=CARTESIAN_POINT('Ctrl Pts',(6.3776149261663,2.60775980566249,-3.61978449806117));
#108952=CARTESIAN_POINT('Ctrl Pts',(6.45031541722462,2.59469807337158,-3.66049326997677));
#108953=CARTESIAN_POINT('Ctrl Pts',(6.48669524604243,2.58831697904106,-3.68088942978343));
#108954=CARTESIAN_POINT('Ctrl Pts',(6.52306390997007,2.58208164076785,-3.70130209819832));
#108955=CARTESIAN_POINT('',(6.72025447322876,2.49144078146676,-3.03548682471018));
#108956=CARTESIAN_POINT('Origin',(4.43655528981068E-13,2.583169653,-2.21610924056037E-13));
#108957=CARTESIAN_POINT('',(6.52332231405131,2.40074633455023,-3.70084665820525));
#108958=CARTESIAN_POINT('Origin',(-0.176630612761898,2.55355109588944,0.0722071555427695));
#108959=CARTESIAN_POINT('',(6.22603192246307,2.49144077881206,-4.18168943993897));
#108960=CARTESIAN_POINT('Origin',(-0.166969114515872,2.41071458448309,0.0965588810765111));
#108961=CARTESIAN_POINT('Origin',(-0.165482309762637,2.55357128393338,0.0991492473481255));
#108962=CARTESIAN_POINT('Ctrl Pts',(6.307242223,2.622074631,-3.575079795));
#108963=CARTESIAN_POINT('Ctrl Pts',(6.11296542,2.556767114,-3.917827629));
#108964=CARTESIAN_POINT('Ctrl Pts',(5.882691166,2.491440779,-4.23750453));
#108965=CARTESIAN_POINT('Ctrl Pts',(6.642512799,2.622074631,-3.482387646));
#108966=CARTESIAN_POINT('Ctrl Pts',(6.453273068,2.556767114,-3.843354735));
#108967=CARTESIAN_POINT('Ctrl Pts',(6.226031915,2.491440779,-4.181689442));
#108968=CARTESIAN_POINT('Ctrl Pts',(6.64586550476001,2.622074631,-3.48146072451));
#108969=CARTESIAN_POINT('Ctrl Pts',(6.45667614448,2.556767114,-3.84261000606));
#108970=CARTESIAN_POINT('Ctrl Pts',(6.22946532249,2.491440779,-4.18113129112));
#108971=CARTESIAN_POINT('',(6.05436154227657,2.49144077849314,-4.2095969834449));
#108972=CARTESIAN_POINT('Ctrl Pts',(5.89868890436543,2.48690656560986,-4.2152957621876));
#108973=CARTESIAN_POINT('Ctrl Pts',(5.89069003518275,2.48917367230491,-4.2264001460938));
#108974=CARTESIAN_POINT('Ctrl Pts',(5.882691166,2.491440779,-4.23750453));
#108975=CARTESIAN_POINT('Ctrl Pts',(5.650707367,2.557191576,-4.559554698));
#108976=CARTESIAN_POINT('Ctrl Pts',(5.384953798,2.622066995,-4.854356043));
#108977=CARTESIAN_POINT('Ctrl Pts',(5.95591824127479,2.48690656560986,-4.55913501163647));
#108978=CARTESIAN_POINT('Ctrl Pts',(5.94726992991814,2.48917367230491,-4.57034497191049));
#108979=CARTESIAN_POINT('Ctrl Pts',(5.9386216185615,2.491440779,-4.58155493218466));
#108980=CARTESIAN_POINT('Ctrl Pts',(5.68780264932776,2.557191576,-4.90666703386099));
#108981=CARTESIAN_POINT('Ctrl Pts',(5.4029922208282,2.622066995,-5.20245589976416));
#108982=CARTESIAN_POINT('',(5.93850626126276,2.49144077985043,-4.58084527104709));
#108983=CARTESIAN_POINT('',(5.57488776576028,2.58208164079198,-5.01703364292958));
#108984=CARTESIAN_POINT('Origin',(-0.157965533946155,2.41074797302503,0.105498548043241));
#108985=CARTESIAN_POINT('Ctrl Pts',(5.38810749188006,2.62129679706164,-4.85085535278));
#108986=CARTESIAN_POINT('Ctrl Pts',(5.41922446827193,2.61444752753297,-4.87847897090086));
#108987=CARTESIAN_POINT('Ctrl Pts',(5.4503631671097,2.60775980550092,-4.90615463707291));
#108988=CARTESIAN_POINT('Ctrl Pts',(5.51261277153886,2.59469807464639,-4.96154011084877));
#108989=CARTESIAN_POINT('Ctrl Pts',(5.54375748182496,2.58831698163702,-4.98928000146014));
#108990=CARTESIAN_POINT('Ctrl Pts',(5.57488775926951,2.58208164076488,-5.01703363236939));
#108991=CARTESIAN_POINT('',(5.91059871904757,2.49144078146676,-4.40917489237154));
#108992=CARTESIAN_POINT('Origin',(8.06646416329215E-14,2.58316965300056,
-3.07913416985883E-14));
#108993=CARTESIAN_POINT('',(5.57523802806608,2.40074633456092,-5.01664438946));
#108994=CARTESIAN_POINT('Origin',(-0.156978674655573,2.55355110431272,0.108489348300177));
#108995=CARTESIAN_POINT('',(5.18153113441456,2.49144077881227,-5.42233668988284));
#108996=CARTESIAN_POINT('Origin',(-0.142308321068101,2.41071463315435,0.130194957196538));
#108997=CARTESIAN_POINT('Origin',(-0.140299164977355,2.55357126531762,0.132404891235678));
#108998=CARTESIAN_POINT('Ctrl Pts',(5.391245927,2.622074631,-4.847367054));
#108999=CARTESIAN_POINT('Ctrl Pts',(5.127830556,2.556767114,-5.14033786300001));
#109000=CARTESIAN_POINT('Ctrl Pts',(4.834218902,2.491440779,-5.403038739));
#109001=CARTESIAN_POINT('Ctrl Pts',(5.738604136,2.622074631,-4.828915258));
#109002=CARTESIAN_POINT('Ctrl Pts',(5.476191471,2.556767114,-5.14076219));
#109003=CARTESIAN_POINT('Ctrl Pts',(5.181531129,2.491440779,-5.422336689));
#109004=CARTESIAN_POINT('Ctrl Pts',(5.74207771809,2.622074631,-4.82873074004));
#109005=CARTESIAN_POINT('Ctrl Pts',(5.47967508015,2.556767114,-5.14076643327));
#109006=CARTESIAN_POINT('Ctrl Pts',(5.18500425127001,2.491440779,-5.4225296685));
#109007=CARTESIAN_POINT('',(5.00787501777898,2.49144077849432,-5.41268771189147));
#109008=CARTESIAN_POINT('Ctrl Pts',(4.85461685026215,2.48690656571168,-5.38478824115059));
#109009=CARTESIAN_POINT('Ctrl Pts',(4.84441787613114,2.48917367235581,-5.3939134900753));
#109010=CARTESIAN_POINT('Ctrl Pts',(4.834218902,2.491440779,-5.403038739));
#109011=CARTESIAN_POINT('Ctrl Pts',(4.538427489,2.557191576,-5.667689893));
#109012=CARTESIAN_POINT('Ctrl Pts',(4.215513515,2.622066995,-5.898469785));
#109013=CARTESIAN_POINT('Ctrl Pts',(4.83659292192365,2.48690656571168,-5.73289133567628));
#109014=CARTESIAN_POINT('Ctrl Pts',(4.82573699343333,2.48917367235581,-5.74198008177738));
#109015=CARTESIAN_POINT('Ctrl Pts',(4.81488106494289,2.491440779,-5.75106882787834));
#109016=CARTESIAN_POINT('Ctrl Pts',(4.50003661232125,2.557191576,-6.01466132424542));
#109017=CARTESIAN_POINT('Ctrl Pts',(4.15829902993438,2.622066995,-6.24230898857749));
#109018=CARTESIAN_POINT('',(4.81492095921965,2.49144077985039,-5.75035096193016));
#109019=CARTESIAN_POINT('',(4.36603605687917,2.58208164081465,-6.09817426156109));
#109020=CARTESIAN_POINT('Origin',(-0.131593410693618,2.41074792150729,0.136990085206607));
#109021=CARTESIAN_POINT('Ctrl Pts',(4.21934602251979,2.62129679699324,-5.89572888979408));
#109022=CARTESIAN_POINT('Ctrl Pts',(4.2437972900956,2.61444751343298,-5.92939598223856));
#109023=CARTESIAN_POINT('Ctrl Pts',(4.26825859004058,2.60775977690531,-5.96311858498214));
#109024=CARTESIAN_POINT('Ctrl Pts',(4.31714649608614,2.59469807212449,-6.03059086746435));
#109025=CARTESIAN_POINT('Ctrl Pts',(4.34159981442992,2.58831697653239,-6.06437742162148));
#109026=CARTESIAN_POINT('Ctrl Pts',(4.36603605302416,2.58208164076558,-6.09817424988061));
#109027=CARTESIAN_POINT('',(4.82456993844327,2.49144078146676,-5.57669484260008));
#109028=CARTESIAN_POINT('Origin',(2.52185425320128E-13,2.58316965299956,
-3.40873163029443E-13));
#109029=CARTESIAN_POINT('',(4.3664618082785,2.40074633452804,-6.09786940478252));
#109030=CARTESIAN_POINT('Origin',(-0.12998675156063,2.55355109067572,0.139698914534188));
#109031=CARTESIAN_POINT('',(3.89474771260811,2.49144077881251,-6.40944149926319));
#109032=CARTESIAN_POINT('Origin',(-0.110993050041865,2.41071459137445,0.157742983199087));
#109033=CARTESIAN_POINT('Origin',(-0.108555880427218,2.55357126078289,0.159469471285793));
#109034=CARTESIAN_POINT('Ctrl Pts',(4.223160964,2.622074631,-5.892996816));
#109035=CARTESIAN_POINT('Ctrl Pts',(3.902924033,2.556767114,-6.122491612));
#109036=CARTESIAN_POINT('Ctrl Pts',(3.559703934,2.491440779,-6.315932861));
#109037=CARTESIAN_POINT('Ctrl Pts',(4.566364721,2.622074631,-5.94964816));
#109038=CARTESIAN_POINT('Ctrl Pts',(4.243049246,2.556767114,-6.197793318));
#109039=CARTESIAN_POINT('Ctrl Pts',(3.894747705,2.491440779,-6.409441498));
#109040=CARTESIAN_POINT('Ctrl Pts',(4.56979675856999,2.622074631,-5.95021467344));
#109041=CARTESIAN_POINT('Ctrl Pts',(4.24645049813,2.556767114,-6.19854633505999));
#109042=CARTESIAN_POINT('Ctrl Pts',(3.89809814271,2.491440779,-6.41037658437));
#109043=CARTESIAN_POINT('',(3.72722582217897,2.49144077849432,-6.36268717793067));
#109044=CARTESIAN_POINT('Ctrl Pts',(3.58354830709371,2.4869065657146,-6.30249400556225));
#109045=CARTESIAN_POINT('Ctrl Pts',(3.57162612054686,2.48917367235727,-6.30921343328113));
#109046=CARTESIAN_POINT('Ctrl Pts',(3.559703934,2.491440779,-6.315932861));
#109047=CARTESIAN_POINT('Ctrl Pts',(3.213935785,2.557191576,-6.510810208));
#109048=CARTESIAN_POINT('Ctrl Pts',(2.848960505,2.622066995,-6.666777635));
#109049=CARTESIAN_POINT('Ctrl Pts',(3.49111389272047,2.4869065657146,-6.63858403102125));
#109050=CARTESIAN_POINT('Ctrl Pts',(3.47855795805834,2.48917367235727,-6.64512658357427));
#109051=CARTESIAN_POINT('Ctrl Pts',(3.46600202339621,2.491440779,-6.65166913612718));
#109052=CARTESIAN_POINT('Ctrl Pts',(3.1018538639937,2.557191576,-6.84141673629003));
#109053=CARTESIAN_POINT('Ctrl Pts',(2.71916839820034,2.622066995,-6.99027864614378));
#109054=CARTESIAN_POINT('',(3.46619530490013,2.49144077985039,-6.65097662960528));
#109055=CARTESIAN_POINT('',(2.9530333546921,2.58208164077412,-6.89417102909293));
#109056=CARTESIAN_POINT('Origin',(-0.0990679971332942,2.41074794347386,
0.162075993420773));
#109057=CARTESIAN_POINT('Ctrl Pts',(2.85329262184866,2.62129679704082,-6.66492469624666));
#109058=CARTESIAN_POINT('Ctrl Pts',(2.86993476900124,2.6144475273861,-6.70306089312993));
#109059=CARTESIAN_POINT('Ctrl Pts',(2.88657477658767,2.60775980518931,-6.74125344879505));
#109060=CARTESIAN_POINT('Ctrl Pts',(2.91981523095929,2.59469807424988,-6.8176578743698));
#109061=CARTESIAN_POINT('Ctrl Pts',(2.93643372789784,2.58831698082537,-6.8559112442663));
#109062=CARTESIAN_POINT('Ctrl Pts',(2.95303335326477,2.58208164074392,-6.89417101679466));
#109063=CARTESIAN_POINT('',(3.51294962880404,2.49144078146678,-6.48345473929143));
#109064=CARTESIAN_POINT('Origin',(-5.87637577487143E-14,2.583169653,3.06178693509906E-13));
#109065=CARTESIAN_POINT('',(2.95351468760116,2.40074633455062,-6.8939648237853));
#109066=CARTESIAN_POINT('Origin',(-0.096916549270849,2.55355105557019,0.16437603281196));
#109067=CARTESIAN_POINT('',(2.42585021516617,2.49144077881249,-7.09684794887307));
#109068=CARTESIAN_POINT('Origin',(-0.0744880397869285,2.4107146057847,0.177915339574071));
#109069=CARTESIAN_POINT('Origin',(-0.0717367755555178,2.55357127143605,
0.179077716464044));
#109070=CARTESIAN_POINT('Ctrl Pts',(2.857605688,2.622074631,-6.663076597));
#109071=CARTESIAN_POINT('Ctrl Pts',(2.495521121,2.556767114,-6.818364458));
#109072=CARTESIAN_POINT('Ctrl Pts',(2.118741167,2.491440779,-6.933500982));
#109073=CARTESIAN_POINT('Ctrl Pts',(3.180607168,2.622074631,-6.792182127));
#109074=CARTESIAN_POINT('Ctrl Pts',(2.811506755,2.556767114,-6.96502251800001));
#109075=CARTESIAN_POINT('Ctrl Pts',(2.425850208,2.491440779,-7.096847946));
#109076=CARTESIAN_POINT('Ctrl Pts',(3.1838371828,2.622074631,-6.79347318230001));
#109077=CARTESIAN_POINT('Ctrl Pts',(2.81466661134,2.556767114,-6.96648909860001));
#109078=CARTESIAN_POINT('Ctrl Pts',(2.42892129841,2.491440779,-7.09848141564));
#109079=CARTESIAN_POINT('',(2.27229569045365,2.49144077849433,-7.01517446304328));
#109080=CARTESIAN_POINT('Ctrl Pts',(2.14491702998573,2.48690656547073,-6.92550215446538));
#109081=CARTESIAN_POINT('Ctrl Pts',(2.1318290984929,2.48917367223534,-6.92950156823269));
#109082=CARTESIAN_POINT('Ctrl Pts',(2.118741167,2.491440779,-6.933500982));
#109083=CARTESIAN_POINT('Ctrl Pts',(1.739164016,2.557191576,-7.049492274));
#109084=CARTESIAN_POINT('Ctrl Pts',(1.349193269,2.622066995,-7.123354373));
#109085=CARTESIAN_POINT('Ctrl Pts',(1.98239426019606,2.48690656547073,-7.23386391516343));
#109086=CARTESIAN_POINT('Ctrl Pts',(1.96872542015212,2.48917367223534,-7.23755435190902));
#109087=CARTESIAN_POINT('Ctrl Pts',(1.95505658010818,2.491440779,-7.24124478865457));
#109088=CARTESIAN_POINT('Ctrl Pts',(1.55863187661946,2.557191576,-7.34827510636233));
#109089=CARTESIAN_POINT('Ctrl Pts',(1.15289247451102,2.622066995,-7.41139064303918));
#109090=CARTESIAN_POINT('',(1.95539421362746,2.49144077968687,-7.24061002108648));
#109091=CARTESIAN_POINT('',(1.40195009493992,2.58208164075595,-7.36780402184064));
#109092=CARTESIAN_POINT('Origin',(-0.0619102066622512,2.41074799745518,
0.179583077257681));
#109093=CARTESIAN_POINT('Ctrl Pts',(1.35382243093522,2.62129679694517,-7.12247603196643));
#109094=CARTESIAN_POINT('Ctrl Pts',(1.36187735507601,2.61444751336702,-7.1632982784614));
#109095=CARTESIAN_POINT('Ctrl Pts',(1.36991807621742,2.60775977682948,-7.20417511712516));
#109096=CARTESIAN_POINT('Ctrl Pts',(1.3859566607698,2.59469807297325,-7.28593879530451));
#109097=CARTESIAN_POINT('Ctrl Pts',(1.39396328432408,2.58831697829252,-7.32687031691883));
#109098=CARTESIAN_POINT('Ctrl Pts',(1.401950096276,2.58208164071552,-7.36780400958062));
#109099=CARTESIAN_POINT('',(2.03706769954258,2.49144078146677,-7.08705549831995));
#109100=CARTESIAN_POINT('Origin',(9.30245463992563E-14,2.58316965299978,
-5.59014640133526E-13));
#109101=CARTESIAN_POINT('',(1.40246450238646,2.40074633473875,-7.36770610983971));
#109102=CARTESIAN_POINT('Origin',(-0.0593146844469267,2.55355108193507,
0.181367093158652));
#109103=CARTESIAN_POINT('',(0.843522657377911,2.49144077881244,-7.45241367635275));
#109104=CARTESIAN_POINT('Origin',(-0.0345000262588741,2.41071456861255,
0.189768554694382));
#109105=CARTESIAN_POINT('Origin',(-0.0315631804266333,2.55357129110865,
0.190312136075104));
#109106=CARTESIAN_POINT('Ctrl Pts',(1.358431946,2.622074631,-7.121598321));
#109107=CARTESIAN_POINT('Ctrl Pts',(0.971430415,2.556767114,-7.19541816));
#109108=CARTESIAN_POINT('Ctrl Pts',(0.578708417,2.491440779,-7.226866303));
#109109=CARTESIAN_POINT('Ctrl Pts',(1.646127958,2.622074631,-7.317121206));
#109110=CARTESIAN_POINT('Ctrl Pts',(1.248501333,2.556767114,-7.406575007));
#109111=CARTESIAN_POINT('Ctrl Pts',(0.843522651,2.491440779,-7.452413672));
#109112=CARTESIAN_POINT('Ctrl Pts',(1.64900491812,2.622074631,-7.31907643485));
#109113=CARTESIAN_POINT('Ctrl Pts',(1.25127204218,2.556767114,-7.40868657547001));
#109114=CARTESIAN_POINT('Ctrl Pts',(0.84617079334,2.491440779,-7.45466914569));
#109115=CARTESIAN_POINT('',(0.711115537090266,2.49144077849433,-7.33963998720059));
#109116=CARTESIAN_POINT('Ctrl Pts',(0.589268654989089,2.48968577857207,
-7.22602066694827));
#109117=CARTESIAN_POINT('Ctrl Pts',(0.583988535994544,2.49056327878603,
-7.22644348497414));
#109118=CARTESIAN_POINT('Ctrl Pts',(0.578708417,2.491440779,-7.226866303));
#109119=CARTESIAN_POINT('Ctrl Pts',(0.18307087,2.557191576,-7.258547916));
#109120=CARTESIAN_POINT('Ctrl Pts',(-0.213660746,2.622066995,-7.246850977));
#109121=CARTESIAN_POINT('Ctrl Pts',(0.363928115288176,2.48968577857207,
-7.49137659932231));
#109122=CARTESIAN_POINT('Ctrl Pts',(0.358454361982624,2.49056327878603,
-7.49163449528042));
#109123=CARTESIAN_POINT('Ctrl Pts',(0.352980608677072,2.491440779,-7.49189239123853));
#109124=CARTESIAN_POINT('Ctrl Pts',(-0.057165892363825,2.557191576,-7.51121644896398));
#109125=CARTESIAN_POINT('Ctrl Pts',(-0.466970758744476,2.622066995,-7.48565195764118));
#109126=CARTESIAN_POINT('Ctrl Pts',(-0.208950993496339,2.62129679688656,
-7.24698830400573));
#109127=CARTESIAN_POINT('Ctrl Pts',(-0.209859963272608,2.61444752746582,
-7.28858763389194));
#109128=CARTESIAN_POINT('Ctrl Pts',(-0.210794539299999,2.60775980554242,
-7.3302372148635));
#109129=CARTESIAN_POINT('Ctrl Pts',(-0.212707705721166,2.59469807423041,
-7.41353730072241));
#109130=CARTESIAN_POINT('Ctrl Pts',(-0.213687339137458,2.58831698335809,
-7.45523302806801));
#109131=CARTESIAN_POINT('Ctrl Pts',(-0.214686788682326,2.58208164328187,
-7.49692665879079));
#109132=CARTESIAN_POINT('',(0.465934748101219,2.49144078146678,-7.3592734190439));
#109133=CARTESIAN_POINT('Ctrl Pts',(-0.204260564,2.622074631,-7.247122023));
#109134=CARTESIAN_POINT('Ctrl Pts',(-0.598083297,2.556767114,-7.23602210600001));
#109135=CARTESIAN_POINT('Ctrl Pts',(-0.988384095,2.491440779,-7.182311389));
#109136=CARTESIAN_POINT('Ctrl Pts',(0.034677634,2.622074631,-7.49991983));
#109137=CARTESIAN_POINT('Ctrl Pts',(-0.372882624,2.556767114,-7.501804281));
#109138=CARTESIAN_POINT('Ctrl Pts',(-0.778247087,2.491440779,-7.459512817));
#109139=CARTESIAN_POINT('Ctrl Pts',(0.03706701598,2.622074631,-7.50244780807));
#109140=CARTESIAN_POINT('Ctrl Pts',(-0.37063061727,2.556767114,-7.50446210275));
#109141=CARTESIAN_POINT('Ctrl Pts',(-0.77614571692,2.491440779,-7.46228483128));
#109142=CARTESIAN_POINT('',(-0.88331558791762,2.49144077849433,-7.32091210337191));
#109143=CARTESIAN_POINT('Ctrl Pts',(-0.961268905873276,2.48690656566808,
-7.18604280921463));
#109144=CARTESIAN_POINT('Ctrl Pts',(-0.974826500436638,2.48917367233402,
-7.18417709910731));
#109145=CARTESIAN_POINT('Ctrl Pts',(-0.988384095,2.491440779,-7.182311389));
#109146=CARTESIAN_POINT('Ctrl Pts',(-1.381582466,2.557191576,-7.128201925));
#109147=CARTESIAN_POINT('Ctrl Pts',(-1.766524221,2.622066995,-7.031492884));
#109148=CARTESIAN_POINT('Ctrl Pts',(-1.23824831884656,2.48690656566808,
-7.39766282396809));
#109149=CARTESIAN_POINT('Ctrl Pts',(-1.2522033956195,2.48917367233402,-7.39527277674135));
#109150=CARTESIAN_POINT('Ctrl Pts',(-1.26615847239241,2.491440779,-7.39288272951463));
#109151=CARTESIAN_POINT('Ctrl Pts',(-1.67088465214717,2.557191576,-7.32356640118142));
#109152=CARTESIAN_POINT('Ctrl Pts',(-2.06562528673817,2.622066995,-7.21048295863567));
#109153=CARTESIAN_POINT('',(-1.26558551255393,2.49144077985043,-7.39244839868839));
#109154=CARTESIAN_POINT('',(-1.82128516547444,2.58208164082782,-7.27550139284704));
#109155=CARTESIAN_POINT('Origin',(0.0192168786179955,2.41074796101253,0.188980975291886));
#109156=CARTESIAN_POINT('Ctrl Pts',(-1.76195410109266,2.62129679686244,
-7.03263945803568));
#109157=CARTESIAN_POINT('Ctrl Pts',(-1.77178446640157,2.6144475132992,-7.07307090047985));
#109158=CARTESIAN_POINT('Ctrl Pts',(-1.78165064464794,2.60775977678226,
-7.11354592569115));
#109159=CARTESIAN_POINT('Ctrl Pts',(-1.80142609344871,2.59469807529347,
-7.19448704266161));
#109160=CARTESIAN_POINT('Ctrl Pts',(-1.81134617464545,2.58831698297699,
-7.23499736360396));
#109161=CARTESIAN_POINT('Ctrl Pts',(-1.82128515921039,2.58208164080564,
-7.27550138211921));
#109162=CARTESIAN_POINT('',(-1.12698479404631,2.49144078146678,-7.28737989481257));
#109163=CARTESIAN_POINT('Origin',(2.65629532258949E-13,2.58316965300011,
9.47592698752331E-13));
#109164=CARTESIAN_POINT('',(-1.82077718939072,2.40074633449375,-7.2756285243275));
#109165=CARTESIAN_POINT('Origin',(0.0223215638672389,2.55355104571884,0.189510060974852));
#109166=CARTESIAN_POINT('',(-2.36362685302965,2.49144077881259,-7.11781344061047));
#109167=CARTESIAN_POINT('Origin',(0.0483703533929128,2.41071457610894,0.186715408605023));
#109168=CARTESIAN_POINT('Origin',(0.051264056983934,2.55357123384883,0.18597571480012));
#109169=CARTESIAN_POINT('Ctrl Pts',(-1.757402077,2.622074631,-7.033778354));
#109170=CARTESIAN_POINT('Ctrl Pts',(-2.1396313,2.556767114,-6.938277701));
#109171=CARTESIAN_POINT('Ctrl Pts',(-2.509260865,2.491440779,-6.801919576));
#109172=CARTESIAN_POINT('Ctrl Pts',(-1.578394177,2.622074631,-7.332030539));
#109173=CARTESIAN_POINT('Ctrl Pts',(-1.976831005,2.556767114,-7.246257523));
#109174=CARTESIAN_POINT('Ctrl Pts',(-2.363626857,2.491440779,-7.117813434));
#109175=CARTESIAN_POINT('Ctrl Pts',(-1.576604098,2.622074631,-7.33501306085001));
#109176=CARTESIAN_POINT('Ctrl Pts',(-1.97520300205,2.556767114,-7.24933732122));
#109177=CARTESIAN_POINT('Ctrl Pts',(-2.36217051692,2.491440779,-7.12097237258));
#109178=CARTESIAN_POINT('',(-2.43644385806959,2.49144077849432,-6.95986650602585));
#109179=CARTESIAN_POINT('Ctrl Pts',(-2.48358175836414,2.48690656555699,
-6.81139272207903));
#109180=CARTESIAN_POINT('Ctrl Pts',(-2.49642131168206,2.48917367227847,
-6.80665614903953));
#109181=CARTESIAN_POINT('Ctrl Pts',(-2.509260865,2.491440779,-6.801919576));
#109182=CARTESIAN_POINT('Ctrl Pts',(-2.881634541,2.557191576,-6.664549134));
#109183=CARTESIAN_POINT('Ctrl Pts',(-3.236786987,2.622066995,-6.487349998));
#109184=CARTESIAN_POINT('Ctrl Pts',(-2.79957759473554,2.48690656555699,
-6.95852279157715));
#109185=CARTESIAN_POINT('Ctrl Pts',(-2.8126926203869,2.48917367227847,-6.95318869321943));
#109186=CARTESIAN_POINT('Ctrl Pts',(-2.82580764603826,2.491440779,-6.94785459486179));
#109187=CARTESIAN_POINT('Ctrl Pts',(-3.20617059104897,2.557191576,-6.79315467934256));
#109188=CARTESIAN_POINT('Ctrl Pts',(-3.56737281157474,2.622066995,-6.59785749653093));
#109189=CARTESIAN_POINT('',(-2.82515471339926,2.49144077985043,-6.94755358787023));
#109190=CARTESIAN_POINT('',(-3.34272226778266,2.58208164079413,-6.71388173945941));
#109191=CARTESIAN_POINT('Origin',(0.059392855570275,2.4107479566335,0.180431512122942));
#109192=CARTESIAN_POINT('Ctrl Pts',(-3.23257019409512,2.62129679699428,
-6.4894522060673));
#109193=CARTESIAN_POINT('Ctrl Pts',(-3.25086225817596,2.61444752746025,
-6.52682506928392));
#109194=CARTESIAN_POINT('Ctrl Pts',(-3.26919866182157,2.60775980540329,
-6.56423278756611));
#109195=CARTESIAN_POINT('Ctrl Pts',(-3.30591180070054,2.59469807479607,
-6.63903057594865));
#109196=CARTESIAN_POINT('Ctrl Pts',(-3.32430847897031,2.58831698194924,
-6.67646126717085));
#109197=CARTESIAN_POINT('Ctrl Pts',(-3.34272225931077,2.58208164076833,
-6.71388173038885));
#109198=CARTESIAN_POINT('',(-2.66720777989305,2.49144078146678,-6.87473658497311));
#109199=CARTESIAN_POINT('Origin',(7.11236625150491E-14,2.58316965300056,
1.9298798670242E-13));
#109200=CARTESIAN_POINT('',(-3.34225349745921,2.40074633454216,-6.71411509886202));
#109201=CARTESIAN_POINT('Origin',(0.0625387514614029,2.55355110413983,0.180280971376496));
#109202=CARTESIAN_POINT('',(-3.83848606137291,2.49144077881225,-6.44329301049446));
#109203=CARTESIAN_POINT('Origin',(0.0873777332257386,2.41071459753082,0.171951807332024));
#109204=CARTESIAN_POINT('Origin',(0.0900447143229784,2.55357127459312,0.170607277916298));
#109205=CARTESIAN_POINT('Ctrl Pts',(-3.228369423,2.622074631,-6.491543027));
#109206=CARTESIAN_POINT('Ctrl Pts',(-3.581132521,2.556767114,-6.316107141));
#109207=CARTESIAN_POINT('Ctrl Pts',(-3.912807385,2.491440779,-6.103477563));
#109208=CARTESIAN_POINT('Ctrl Pts',(-3.117662031,2.622074631,-6.821303648));
#109209=CARTESIAN_POINT('Ctrl Pts',(-3.488344964,2.556767114,-6.65188381800001));
#109210=CARTESIAN_POINT('Ctrl Pts',(-3.838486062,2.491440779,-6.44329300500001));
#109211=CARTESIAN_POINT('Ctrl Pts',(-3.11655495708,2.622074631,-6.82460125420999));
#109212=CARTESIAN_POINT('Ctrl Pts',(-3.48741708843,2.556767114,-6.65524158477));
#109213=CARTESIAN_POINT('Ctrl Pts',(-3.83774284877,2.491440779,-6.44669115942001));
#109214=CARTESIAN_POINT('',(-3.87564672085863,2.49144077849432,-6.27338528563182));
#109215=CARTESIAN_POINT('Ctrl Pts',(-3.88976508816575,2.48690656560517,
-6.11824948085734));
#109216=CARTESIAN_POINT('Ctrl Pts',(-3.90128623658284,2.48917367230256,
-6.11086352192864));
#109217=CARTESIAN_POINT('Ctrl Pts',(-3.912807385,2.491440779,-6.103477563));
#109218=CARTESIAN_POINT('Ctrl Pts',(-4.246944588,2.557191576,-5.889269433));
#109219=CARTESIAN_POINT('Ctrl Pts',(-4.555701191,2.622066995,-5.639865837));
#109220=CARTESIAN_POINT('Ctrl Pts',(-4.23000173462422,2.48690656560517,
-6.19400996793768));
#109221=CARTESIAN_POINT('Ctrl Pts',(-4.24166346466579,2.48917367230256,
-6.18598123507829));
#109222=CARTESIAN_POINT('Ctrl Pts',(-4.25332519470735,2.491440779,-6.17795250221879));
#109223=CARTESIAN_POINT('Ctrl Pts',(-4.59153955643061,2.557191576,-5.94510259488557));
#109224=CARTESIAN_POINT('Ctrl Pts',(-4.9023139484091,2.622066995,-5.67672355130975));
#109225=CARTESIAN_POINT('',(-4.25262281964114,2.49144077985043,-6.17779889382796));
#109226=CARTESIAN_POINT('',(-4.70785739189339,2.58208164078621,-5.83832843814145));
#109227=CARTESIAN_POINT('Origin',(0.0967917407034796,2.41074795623055,0.16344543293264));
#109228=CARTESIAN_POINT('Ctrl Pts',(-4.5520348968241,2.62129679694249,-5.64282538264453));
#109229=CARTESIAN_POINT('Ctrl Pts',(-4.57793341658891,2.61444751335628,
-5.67539230278681));
#109230=CARTESIAN_POINT('Ctrl Pts',(-4.60388273930677,2.60775977681687,
-5.70798374014004));
#109231=CARTESIAN_POINT('Ctrl Pts',(-4.65581675711939,2.59469807182015,
-5.77314043040226));
#109232=CARTESIAN_POINT('Ctrl Pts',(-4.68182983665765,2.58831697595684,
-5.80574128731554));
#109233=CARTESIAN_POINT('Ctrl Pts',(-4.70785738166523,2.58208164073532,
-5.83832843131991));
#109234=CARTESIAN_POINT('',(-4.08271509389942,2.49144078146678,-6.14063823337773));
#109235=CARTESIAN_POINT('Origin',(8.67361737988404E-15,2.58316965300056,
3.38271077815477E-14));
#109236=CARTESIAN_POINT('',(-4.70744974629859,2.4007463345217,-5.83865711346281));
#109237=CARTESIAN_POINT('Origin',(0.0998316725259318,2.55355109009625,0.162622053385927));
#109238=CARTESIAN_POINT('',(-5.13386192418331,2.49144077881253,-5.46749136466001));
#109239=CARTESIAN_POINT('Origin',(0.122299545908611,2.41071455200006,0.1491481746298));
#109240=CARTESIAN_POINT('Origin',(0.124615097880485,2.55357125344024,0.147261696059101));
#109241=CARTESIAN_POINT('Ctrl Pts',(-4.548381802,2.622074631,-5.645770362));
#109242=CARTESIAN_POINT('Ctrl Pts',(-4.85518396500001,2.556767114,-5.398602432));
#109243=CARTESIAN_POINT('Ctrl Pts',(-5.13339538200001,2.491440779,-5.119643723));
#109244=CARTESIAN_POINT('Ctrl Pts',(-4.511151473,2.622074631,-5.99162018));
#109245=CARTESIAN_POINT('Ctrl Pts',(-4.83674779000001,2.556767114,-5.746475418));
#109246=CARTESIAN_POINT('Ctrl Pts',(-5.133861925,2.491440779,-5.46749135700001));
#109247=CARTESIAN_POINT('Ctrl Pts',(-4.51077916970999,2.622074631,-5.99507867818));
#109248=CARTESIAN_POINT('Ctrl Pts',(-4.83656342825001,2.556767114,-5.74995414786));
#109249=CARTESIAN_POINT('Ctrl Pts',(-5.13386659043,2.491440779,-5.47096983334));
#109250=CARTESIAN_POINT('',(-5.13362865127118,2.49144077849432,-5.29356754216149));
#109251=CARTESIAN_POINT('Ctrl Pts',(-5.11406732737489,2.48690656569176,
-5.13902369391064));
#109252=CARTESIAN_POINT('Ctrl Pts',(-5.12373135468741,2.48917367234586,
-5.12933370845532));
#109253=CARTESIAN_POINT('Ctrl Pts',(-5.133395382,2.491440779,-5.119643723));
#109254=CARTESIAN_POINT('Ctrl Pts',(-5.413672226,2.557191576,-4.838614039));
#109255=CARTESIAN_POINT('Ctrl Pts',(-5.66159587,2.622066995,-4.528667818));
#109256=CARTESIAN_POINT('Ctrl Pts',(-5.46263569378407,2.48690656569176,
-5.13987212188714));
#109257=CARTESIAN_POINT('Ctrl Pts',(-5.47229883864984,2.48917367234586,
-5.12952416929416));
#109258=CARTESIAN_POINT('Ctrl Pts',(-5.4819619835156,2.491440779,-5.11917621670133));
#109259=CARTESIAN_POINT('Ctrl Pts',(-5.76221323472681,2.557191576,-4.81906412049436));
#109260=CARTESIAN_POINT('Ctrl Pts',(-6.00802833355053,2.622066995,-4.49015232227628));
#109261=CARTESIAN_POINT('',(-5.48124301056672,2.49144077985039,-5.11917718797777));
#109262=CARTESIAN_POINT('',(-5.85285833666219,2.5820816407985,-4.68978138803624));
#109263=CARTESIAN_POINT('Origin',(0.12966479496718,2.41074795964312,0.138816861836842));
#109264=CARTESIAN_POINT('Ctrl Pts',(-5.6586515066873,2.62129679699947,-4.53234631572041));
#109265=CARTESIAN_POINT('Ctrl Pts',(-5.69094539166984,2.61444752760817,
-4.55858436875302));
#109266=CARTESIAN_POINT('Ctrl Pts',(-5.72329415329283,2.60775980571505,
-4.58483543755505));
#109267=CARTESIAN_POINT('Ctrl Pts',(-5.78802088432703,2.59469807261756,
-4.63730463473079));
#109268=CARTESIAN_POINT('Ctrl Pts',(-5.82043400878806,2.58831697755227,
-4.663551255023));
#109269=CARTESIAN_POINT('Ctrl Pts',(-5.85285832520197,2.58208164075407,
-4.68978138350754));
#109270=CARTESIAN_POINT('',(-5.30731918799508,2.49144078146676,-5.11941046289051));
#109271=CARTESIAN_POINT('Origin',(7.45931094670027E-14,2.58316965299933,
4.16333634234434E-14));
#109272=CARTESIAN_POINT('',(-5.85253087724993,2.40074633455269,-4.6901900103424));
#109273=CARTESIAN_POINT('Origin',(0.132456444858018,2.55355106810776,0.137359050767329));
#109274=CARTESIAN_POINT('',(-6.18918411085228,2.49144077881255,-4.23603589763637));
#109275=CARTESIAN_POINT('Origin',(0.151502940283521,2.41071459750532,0.119370561588326));
#109276=CARTESIAN_POINT('Origin',(0.153358491952575,2.55357124787777,0.117030173352617));
#109277=CARTESIAN_POINT('Ctrl Pts',(-5.65571690300001,2.622074631,-4.536007751));
#109278=CARTESIAN_POINT('Ctrl Pts',(-5.902212403,2.556767114,-4.228665073));
#109279=CARTESIAN_POINT('Ctrl Pts',(-6.113951515,2.491440779,-3.896421033));
#109280=CARTESIAN_POINT('Ctrl Pts',(-5.693704486,2.622074631,-4.88177521199999));
#109281=CARTESIAN_POINT('Ctrl Pts',(-5.958989665,2.556767114,-4.572368215));
#109282=CARTESIAN_POINT('Ctrl Pts',(-6.18918411,2.491440779,-4.23603589));
#109283=CARTESIAN_POINT('Ctrl Pts',(-5.69408436183001,2.622074631,-4.88523288661));
#109284=CARTESIAN_POINT('Ctrl Pts',(-5.95955743762001,2.556767114,-4.57580524642));
#109285=CARTESIAN_POINT('Ctrl Pts',(-6.18993643594999,2.491440779,-4.23943203857));
#109286=CARTESIAN_POINT('',(-6.15156781078794,2.49144077849432,-4.06622846409008));
#109287=CARTESIAN_POINT('Ctrl Pts',(-6.09924145970536,2.48690656548447,
-3.91950287244791));
#109288=CARTESIAN_POINT('Ctrl Pts',(-6.10659648735274,2.48917367224221,
-3.90796195272396));
#109289=CARTESIAN_POINT('Ctrl Pts',(-6.113951515,2.491440779,-3.896421033));
#109290=CARTESIAN_POINT('Ctrl Pts',(-6.327262568,2.557191576,-3.56171043));
#109291=CARTESIAN_POINT('Ctrl Pts',(-6.502760619,2.622066995,-3.205714324));
#109292=CARTESIAN_POINT('Ctrl Pts',(-6.43984287951191,2.48690656548447,
-3.84539956878979));
#109293=CARTESIAN_POINT('Ctrl Pts',(-6.44705560182278,2.48917367224221,
-3.83321625452855));
#109294=CARTESIAN_POINT('Ctrl Pts',(-6.45426832413366,2.491440779,-3.82103294026727));
#109295=CARTESIAN_POINT('Ctrl Pts',(-6.66345222729634,2.557191576,-3.46769156362974));
#109296=CARTESIAN_POINT('Ctrl Pts',(-6.83281399032402,2.622066995,-3.09362655994177));
#109297=CARTESIAN_POINT('',(-6.45356636728458,2.49144077985042,-3.82118844870344));
#109298=CARTESIAN_POINT('',(-6.72418613066418,2.58208164076895,-3.32194537211322));
#109299=CARTESIAN_POINT('Origin',(0.156474591155465,2.4107479616494,0.107697166367046));
#109300=CARTESIAN_POINT('Ctrl Pts',(-6.5006758616883,2.62129679701399,-3.20993977145643));
#109301=CARTESIAN_POINT('Ctrl Pts',(-6.53785521611478,2.61444751350204,
-3.22862220123853));
#109302=CARTESIAN_POINT('Ctrl Pts',(-6.57509097269971,2.60775977699807,
-3.24730555074524));
#109303=CARTESIAN_POINT('Ctrl Pts',(-6.64958357449561,2.5946980755614,-3.28463362300767));
#109304=CARTESIAN_POINT('Ctrl Pts',(-6.68688112675005,2.58831698350122,
-3.30329873896052));
#109305=CARTESIAN_POINT('Ctrl Pts',(-6.72418611842758,2.58208164075017,
-3.32194536991413));
#109306=CARTESIAN_POINT('',(-6.28375893558179,2.49144078146676,-3.85880474889419));
#109307=CARTESIAN_POINT('Origin',(-1.77722420113824E-12,2.583169653,-9.55832635263221E-13));
#109308=CARTESIAN_POINT('',(-6.72395416877965,2.40074633454126,-3.32241483495408));
#109309=CARTESIAN_POINT('Origin',(0.158887903390401,2.55355108009206,0.105673490532908));
#109310=CARTESIAN_POINT('',(-6.95510692647806,2.4914407788125,-2.80650809933182));
#109311=CARTESIAN_POINT('Origin',(0.173621591640072,2.41071463550373,0.0840108764685926));
#109312=CARTESIAN_POINT('Origin',(0.174931003160467,2.55357126558374,0.0813264799573265));
#109313=CARTESIAN_POINT('Ctrl Pts',(-6.498596968,2.622074631,-3.214146458));
#109314=CARTESIAN_POINT('Ctrl Pts',(-6.67325995,2.556767114,-2.861000035));
#109315=CARTESIAN_POINT('Ctrl Pts',(-6.808626071,2.491440779,-2.491006026));
#109316=CARTESIAN_POINT('Ctrl Pts',(-6.610026206,2.622074631,-3.543663861));
#109317=CARTESIAN_POINT('Ctrl Pts',(-6.80259580600001,2.556767114,-3.184462156));
#109318=CARTESIAN_POINT('Ctrl Pts',(-6.955106924,2.491440779,-2.806508092));
#109319=CARTESIAN_POINT('Ctrl Pts',(-6.61114049838,2.622074631,-3.54695903503));
#109320=CARTESIAN_POINT('Ctrl Pts',(-6.80388916456,2.556767114,-3.18769677721));
#109321=CARTESIAN_POINT('Ctrl Pts',(-6.95657173253,2.491440779,-2.80966311266));
#109322=CARTESIAN_POINT('',(-6.88186649638476,2.49144077849432,-2.64875706189757));
#109323=CARTESIAN_POINT('Ctrl Pts',(-6.79922184204682,2.48690656561667,
-2.51671045117644));
#109324=CARTESIAN_POINT('Ctrl Pts',(-6.80392395652347,2.48917367230831,
-2.5038582385882));
#109325=CARTESIAN_POINT('Ctrl Pts',(-6.808626071,2.491440779,-2.491006026));
#109326=CARTESIAN_POINT('Ctrl Pts',(-6.944997145,2.557191576,-2.1182652));
#109327=CARTESIAN_POINT('Ctrl Pts',(-7.039863509,2.622066995,-1.732865192));
#109328=CARTESIAN_POINT('Ctrl Pts',(-7.11593016962833,2.48690656561667,
-2.37112040446412));
#109329=CARTESIAN_POINT('Ctrl Pts',(-7.12035520993026,2.48917367230831,
-2.35767140762744));
#109330=CARTESIAN_POINT('Ctrl Pts',(-7.12478025023214,2.491440779,-2.34422241079084));
#109331=CARTESIAN_POINT('Ctrl Pts',(-7.25311559839781,2.557191576,-1.9541736036031));
#109332=CARTESIAN_POINT('Ctrl Pts',(-7.33810486046178,2.622066995,-1.55244625913541));
#109333=CARTESIAN_POINT('',(-7.12412813449252,2.49144077985043,-2.34452518347534));
#109334=CARTESIAN_POINT('',(-7.28109845461218,2.58208164083062,-1.79877888269512));
#109335=CARTESIAN_POINT('Origin',(0.175968276889885,2.41074793770117,0.0715419416780225));
#109336=CARTESIAN_POINT('Ctrl Pts',(-7.03873583834957,2.62129679700212,
-1.7374400121656));
#109337=CARTESIAN_POINT('Ctrl Pts',(-7.07906204740106,2.61444752758852,
-1.74769317383412));
#109338=CARTESIAN_POINT('Ctrl Pts',(-7.11944352632008,2.60775980565941,
-1.75793510623339));
#109339=CARTESIAN_POINT('Ctrl Pts',(-7.20021915405798,2.5946980736025,-1.77837680933423));
#109340=CARTESIAN_POINT('Ctrl Pts',(-7.24065717235596,2.58831697949574,
-1.78858767743524));
#109341=CARTESIAN_POINT('Ctrl Pts',(-7.28109844228063,2.58208164079368,
-1.79877888333402));
#109342=CARTESIAN_POINT('',(-6.96637709903875,2.49144078146678,-2.41776561379499));
#109343=CARTESIAN_POINT('Origin',(-6.28837260041593E-13,2.58316965300011,
-9.69276742202041E-14));
#109344=CARTESIAN_POINT('',(-7.2809728364116,2.40074633457368,-1.79928723503158));
#109345=CARTESIAN_POINT('Origin',(0.177890141013355,2.55355108091248,0.0690467838518782));
#109346=CARTESIAN_POINT('',(-7.39581667399581,2.49144077881244,-1.24575110158275));
#109347=CARTESIAN_POINT('Origin',(0.18762263744327,2.41071458012096,0.0447233372678933));
#109348=CARTESIAN_POINT('Origin',(0.188324448607427,2.55357128732538,0.041820229100871));
#109349=CARTESIAN_POINT('Ctrl Pts',(-7.037609861,2.622074631,-1.741995249));
#109350=CARTESIAN_POINT('Ctrl Pts',(-7.132273277,2.556767114,-1.359557815));
#109351=CARTESIAN_POINT('Ctrl Pts',(-7.184936839,2.491440779,-0.969114346));
#109352=CARTESIAN_POINT('Ctrl Pts',(-7.21727044700001,2.622074631,-2.039854725));
#109353=CARTESIAN_POINT('Ctrl Pts',(-7.328120127,2.556767114,-1.647654185));
#109354=CARTESIAN_POINT('Ctrl Pts',(-7.39581667,2.491440779,-1.245751095));
#109355=CARTESIAN_POINT('Ctrl Pts',(-7.21906705286,2.622074631,-2.04283331976));
#109356=CARTESIAN_POINT('Ctrl Pts',(-7.3300785955,2.556767114,-1.6505351487));
#109357=CARTESIAN_POINT('Ctrl Pts',(-7.39792546831,2.491440779,-1.24851746249));
#109358=CARTESIAN_POINT('',(-7.29037675403372,2.49144077849432,-1.10743272356957));
#109359=CARTESIAN_POINT('Ctrl Pts',(-7.18127816726304,2.48690656553082,
-0.9962394477905));
#109360=CARTESIAN_POINT('Ctrl Pts',(-7.18310750313154,2.48917367226538,
-0.982676896895252));
#109361=CARTESIAN_POINT('Ctrl Pts',(-7.184936839,2.491440779,-0.969114346));
#109362=CARTESIAN_POINT('Ctrl Pts',(-7.237991373,2.557191576,-0.575772243));
#109363=CARTESIAN_POINT('Ctrl Pts',(-7.247790206,2.622066995,-0.178989209));
#109364=CARTESIAN_POINT('Ctrl Pts',(-7.45928447412705,2.48690656553082,
-0.785970285862701));
#109365=CARTESIAN_POINT('Ctrl Pts',(-7.46071492270005,2.48917367226538,
-0.771884465993628));
#109366=CARTESIAN_POINT('Ctrl Pts',(-7.46214537127316,2.491440779,-0.757798646124541));
#109367=CARTESIAN_POINT('Ctrl Pts',(-7.50363134646488,2.557191576,-0.349280657688787));
#109368=CARTESIAN_POINT('Ctrl Pts',(-7.50027410217251,2.622066995,0.0613247038400555));
#109369=CARTESIAN_POINT('',(-7.46157358879537,2.49144077985042,-0.758234525785307));
#109370=CARTESIAN_POINT('',(-7.49755470733861,2.58208164080026,-0.191503492201462));
#109371=CARTESIAN_POINT('Origin',(0.187233531968248,2.41074792168317,0.032041345118505));
#109372=CARTESIAN_POINT('Ctrl Pts',(-7.24767235074776,2.62129679697139,
-0.183699488456621));
#109373=CARTESIAN_POINT('Ctrl Pts',(-7.2892598818894,2.61444752755311,-0.185043994028461));
#109374=CARTESIAN_POINT('Ctrl Pts',(-7.33089897670836,2.60775980564852,
-0.186365651459866));
#109375=CARTESIAN_POINT('Ctrl Pts',(-7.41418046610708,2.59469807529747,
-0.188965066345878));
#109376=CARTESIAN_POINT('Ctrl Pts',(-7.45586808822642,2.58831698299861,
-0.19024423107201));
#109377=CARTESIAN_POINT('Ctrl Pts',(-7.49755469532192,2.58208164077877,
-0.191503495362631));
#109378=CARTESIAN_POINT('',(-7.32325521222775,2.49144078146676,-0.863674445527217));
#109379=CARTESIAN_POINT('Origin',(9.00321484031963E-13,2.58316965299956,
9.75781955236954E-16));
#109380=CARTESIAN_POINT('',(-7.49754130651673,2.40074633455664,-0.192026963734102));
#109381=CARTESIAN_POINT('Origin',(0.188574016816311,2.55355108770253,0.0291913730601223));
#109382=CARTESIAN_POINT('',(-7.49070625230964,2.49144077881258,0.373255832402669));
#109383=CARTESIAN_POINT('Origin',(0.192850144084868,2.41071460097831,0.00334440390496821));
#109384=CARTESIAN_POINT('Origin',(0.192911317040971,2.55357123636567,0.000358288584547154));
#109385=CARTESIAN_POINT('Ctrl Pts',(-7.24755193900001,2.622074631,-0.188390278));
#109386=CARTESIAN_POINT('Ctrl Pts',(-7.257789433,2.556767114,0.205455817));
#109387=CARTESIAN_POINT('Ctrl Pts',(-7.225287946,2.491440779,0.598092044));
#109388=CARTESIAN_POINT('Ctrl Pts',(-7.487043143,2.622074631,-0.440664251));
#109389=CARTESIAN_POINT('Ctrl Pts',(-7.510989697,2.556767114,-0.033803736));
#109390=CARTESIAN_POINT('Ctrl Pts',(-7.490706247,2.491440779,0.373255838));
#109391=CARTESIAN_POINT('Ctrl Pts',(-7.48943805504001,2.622074631,-0.44318699073));
#109392=CARTESIAN_POINT('Ctrl Pts',(-7.51352169964,2.556767114,-0.0361963315300001));
#109393=CARTESIAN_POINT('Ctrl Pts',(-7.49336043001,2.491440779,0.37100747594));
#109394=CARTESIAN_POINT('',(-7.35799709670449,2.49144077849432,0.485673937901959));
#109395=CARTESIAN_POINT('Ctrl Pts',(-7.22754590707776,2.48690656539367,
0.570814604899168));
#109396=CARTESIAN_POINT('Ctrl Pts',(-7.22641692653879,2.48917367219681,
0.584453324449584));
#109397=CARTESIAN_POINT('Ctrl Pts',(-7.225287946,2.491440779,0.598092044));
#109398=CARTESIAN_POINT('Ctrl Pts',(-7.19254517,2.557191576,0.993643183999999));
#109399=CARTESIAN_POINT('Ctrl Pts',(-7.116818287,2.622066995,1.38325611));
#109400=CARTESIAN_POINT('Ctrl Pts',(-7.4538509263014,2.48690656539367,0.835930928125738));
#109401=CARTESIAN_POINT('Ctrl Pts',(-7.45221989685616,2.48917367219681,
0.849994933965902));
#109402=CARTESIAN_POINT('Ctrl Pts',(-7.45058886741099,2.491440779,0.864058939806079));
#109403=CARTESIAN_POINT('Ctrl Pts',(-7.40328563237933,2.557191576,1.27194426382674));
#109404=CARTESIAN_POINT('Ctrl Pts',(-7.31173886259761,2.622066995,1.6722281922973));
#109405=CARTESIAN_POINT('',(-7.45012415412549,2.49144077985042,0.863510334451682));
#109406=CARTESIAN_POINT('',(-7.36343363451669,2.58208164079611,1.42472638913831));
#109407=CARTESIAN_POINT('Origin',(0.189743853020058,2.41074793455603,-0.00895740390180852));
#109408=CARTESIAN_POINT('Ctrl Pts',(-7.11771575797403,2.62129679704776,
1.37863061942135));
#109409=CARTESIAN_POINT('Ctrl Pts',(-7.15862010913201,2.61444751349351,
1.38625765323444));
#109410=CARTESIAN_POINT('Ctrl Pts',(-7.19956991822297,2.60775977696405,
1.39391808802037));
#109411=CARTESIAN_POINT('Ctrl Pts',(-7.28146295658397,2.59469807427698,
1.40928247184832));
#109412=CARTESIAN_POINT('Ctrl Pts',(-7.32245093530049,2.58831698089371,
1.41699482114407));
#109413=CARTESIAN_POINT('Ctrl Pts',(-7.36343362353817,2.58208164076581,
1.42472638341801));
#109414=CARTESIAN_POINT('',(-7.33770605049959,2.49144078146676,0.73080117944313));
#109415=CARTESIAN_POINT('Origin',(5.68121938382404E-13,2.583169653,-6.21247844834194E-14));
#109416=CARTESIAN_POINT('',(-7.363533078059,2.40074633454557,1.42421227530058));
#109417=CARTESIAN_POINT('Origin',(0.190440384937789,2.55355104710757,-0.0120289222636236));
#109418=CARTESIAN_POINT('',(-7.23533873239084,2.49144077881247,1.97480973969609));
#109419=CARTESIAN_POINT('Origin',(0.189060473731137,2.4107145792923,-0.0381908852372392));
#109420=CARTESIAN_POINT('Origin',(0.188478046561856,2.55357127601239,-0.041120270749862));
#109421=CARTESIAN_POINT('Ctrl Pts',(-7.118606543,2.622074631,1.374023613));
#109422=CARTESIAN_POINT('Ctrl Pts',(-7.043939422,2.556767114,1.760862564));
#109423=CARTESIAN_POINT('Ctrl Pts',(-6.927792619,2.491440779,2.137332315));
#109424=CARTESIAN_POINT('Ctrl Pts',(-7.406730022,2.622074631,1.179131195));
#109425=CARTESIAN_POINT('Ctrl Pts',(-7.342653736,2.556767114,1.581627338));
#109426=CARTESIAN_POINT('Ctrl Pts',(-7.235338726,2.491440779,1.974809744));
#109427=CARTESIAN_POINT('Ctrl Pts',(-7.40961125679,2.622074631,1.17718227082));
#109428=CARTESIAN_POINT('Ctrl Pts',(-7.34564087914,2.556767114,1.57983498574));
#109429=CARTESIAN_POINT('Ctrl Pts',(-7.23841418707,2.491440779,1.97318451829));
#109430=CARTESIAN_POINT('',(-7.08156567336569,2.49144077849432,2.05607102651835));
#109431=CARTESIAN_POINT('Ctrl Pts',(-6.93586163280649,2.48690656567579,
2.11117800379407));
#109432=CARTESIAN_POINT('Ctrl Pts',(-6.93182712590332,2.48917367233787,
2.12425515939704));
#109433=CARTESIAN_POINT('Ctrl Pts',(-6.92779261899999,2.491440779,2.137332315));
#109434=CARTESIAN_POINT('Ctrl Pts',(-6.810783548,2.557191576,2.51659696));
#109435=CARTESIAN_POINT('Ctrl Pts',(-6.653071856,2.622066995,2.880821911));
#109436=CARTESIAN_POINT('Ctrl Pts',(-7.09988359422218,2.48690656567579,
2.41874494454143));
#109437=CARTESIAN_POINT('Ctrl Pts',(-7.09526735207894,2.48917367233787,
2.43212951777117));
#109438=CARTESIAN_POINT('Ctrl Pts',(-7.09065110993579,2.491440779,2.44551409100092));
#109439=CARTESIAN_POINT('Ctrl Pts',(-6.95677050999374,2.557191576,2.83369448500872));
#109440=CARTESIAN_POINT('Ctrl Pts',(-6.78131484150381,2.622066995,3.20494014823205));
#109441=CARTESIAN_POINT('',(-7.09031519534277,2.49144077985042,2.44487841211678));
#109442=CARTESIAN_POINT('',(-6.88500658986866,2.58208164074794,2.97433764640151));
#109443=CARTESIAN_POINT('Origin',(0.183382424378213,2.41074792779091,-0.0495374053930203));
#109444=CARTESIAN_POINT('Ctrl Pts',(-6.65494268860644,2.6212967969372,2.87649749092932));
#109445=CARTESIAN_POINT('Ctrl Pts',(-6.69325113231692,2.61444751332667,
2.89273943554867));
#109446=CARTESIAN_POINT('Ctrl Pts',(-6.73159679081763,2.60775977676549,
2.90902377224826));
#109447=CARTESIAN_POINT('Ctrl Pts',(-6.80827173775859,2.59469817447579,
2.94163327719176));
#109448=CARTESIAN_POINT('Ctrl Pts',(-6.84664284917639,2.58831718441713,
2.95797623595795));
#109449=CARTESIAN_POINT('Ctrl Pts',(-6.88500658063842,2.58208164062072,
2.97433763948164));
#109450=CARTESIAN_POINT('',(-7.00905390970131,2.49144078146676,2.29110535411757));
#109451=CARTESIAN_POINT('Ctrl Pts',(-6.656803017,2.622074631,2.872189686));
#109452=CARTESIAN_POINT('Ctrl Pts',(-6.500722632,2.556767114,3.233933334));
#109453=CARTESIAN_POINT('Ctrl Pts',(-6.306361409,2.491440779,3.576633302));
#109454=CARTESIAN_POINT('Ctrl Pts',(-6.980086438,2.622074631,2.743791776));
#109455=CARTESIAN_POINT('Ctrl Pts',(-6.830983446,2.556767114,3.123103275));
#109456=CARTESIAN_POINT('Ctrl Pts',(-6.641654807,2.491440779,3.48402374));
#109457=CARTESIAN_POINT('Ctrl Pts',(-6.98331927221,2.622074631,2.7425077969));
#109458=CARTESIAN_POINT('Ctrl Pts',(-6.83428605413999,2.556767114,3.12199497441));
#109459=CARTESIAN_POINT('Ctrl Pts',(-6.64500774098,2.491440779,3.48309764438));
#109460=CARTESIAN_POINT('',(-6.6416548109875,2.49144077881208,3.48402374074511));
#109461=CARTESIAN_POINT('Origin',(0.175232140450808,2.55357127254053,-0.0806762294126564));
#109462=CARTESIAN_POINT('',(-6.4740081094864,2.49144077849433,3.5303285182742));
#109463=CARTESIAN_POINT('Origin',(-2.90999863095109E-13,2.58316965299956,
1.45283091113058E-13));
#109464=CARTESIAN_POINT('',(-6.88521422698715,2.40074633447349,2.97385693108466));
#109465=CARTESIAN_POINT('Origin',(0.183402177679237,2.55355105024397,-0.052686769679634));
#109466=CARTESIAN_POINT('Origin',(0.176430275859584,2.41071461896874,-0.0779403562094694));
#109467=CARTESIAN_POINT('Ctrl Pts',(-6.31986417766011,2.48690656564425,
3.55282506333069));
#109468=CARTESIAN_POINT('Ctrl Pts',(-6.31311279333012,2.4891736723221,3.56472918266534));
#109469=CARTESIAN_POINT('Ctrl Pts',(-6.306361409,2.491440779,3.576633302));
#109470=CARTESIAN_POINT('Ctrl Pts',(-6.110557257,2.557191576,3.921877459));
#109471=CARTESIAN_POINT('Ctrl Pts',(-5.87823517799999,2.622066995,4.243683681));
#109472=CARTESIAN_POINT('Ctrl Pts',(-6.41393359556659,2.48690656564425,
3.8884611333781));
#109473=CARTESIAN_POINT('Ctrl Pts',(-6.40654799092982,2.4891736723221,3.90054042721907));
#109474=CARTESIAN_POINT('Ctrl Pts',(-6.39916238629304,2.491440779,3.9126197210601));
#109475=CARTESIAN_POINT('Ctrl Pts',(-6.18496452964555,2.557191576,4.26294430216168));
#109476=CARTESIAN_POINT('Ctrl Pts',(-5.93380407379803,2.622066995,4.58779266501244));
#109477=CARTESIAN_POINT('',(-6.39897097736251,2.49144077985043,3.91192669229793));
#109478=CARTESIAN_POINT('',(-6.35266619768326,2.49144078146678,3.74427998846434));
#109479=CARTESIAN_POINT('',(-6.08464428739668,2.58208164078499,4.38487218380399));
#109480=CARTESIAN_POINT('Origin',(0.168445965700353,2.41074796746151,-0.0878010593493334));
#109481=CARTESIAN_POINT('Ctrl Pts',(-5.88099189403263,2.62129679694873,
4.23986253723593));
#109482=CARTESIAN_POINT('Ctrl Pts',(-5.9149131694583,2.61444751339891,4.26395993721713));
#109483=CARTESIAN_POINT('Ctrl Pts',(-5.94886167659632,2.60775977687749,
4.28810673828796));
#109484=CARTESIAN_POINT('Ctrl Pts',(-6.01673444503164,2.59469807475853,
4.33643706788972));
#109485=CARTESIAN_POINT('Ctrl Pts',(-6.05069579275439,2.58831698187106,
4.36064701015502));
#109486=CARTESIAN_POINT('Ctrl Pts',(-6.08464427979713,2.58208164075899,
4.3848721740135));
#109487=CARTESIAN_POINT('Origin',(1.04170144732407E-12,2.58316965300044,
-7.54171031180917E-13));
#109488=CARTESIAN_POINT('',(-5.73741449653065,2.49144077881202,4.83032865927712));
#109489=CARTESIAN_POINT('Origin',(0.153792080296967,2.5535713027714,-0.116459622361033));
#109490=CARTESIAN_POINT('',(-6.08495041118466,2.40074633452799,4.38444734227674));
#109491=CARTESIAN_POINT('Origin',(0.167788274850221,2.55355109662838,-0.0908810363877111));
#109492=CARTESIAN_POINT('Origin',(0.155550450071232,2.41071458854319,-0.114045366558431));
#109493=CARTESIAN_POINT('Ctrl Pts',(-5.88373478,2.622074631,4.236055362));
#109494=CARTESIAN_POINT('Ctrl Pts',(-5.653539277,2.556767114,4.555788976));
#109495=CARTESIAN_POINT('Ctrl Pts',(-5.390051748,2.491440779,4.848694892));
#109496=CARTESIAN_POINT('Ctrl Pts',(-6.22706177,2.622074631,4.180155704));
#109497=CARTESIAN_POINT('Ctrl Pts',(-5.999903964,2.556767114,4.518546375));
#109498=CARTESIAN_POINT('Ctrl Pts',(-5.737414491,2.491440779,4.830328659));
#109499=CARTESIAN_POINT('Ctrl Pts',(-6.23049503989999,2.622074631,4.17959670742));
#109500=CARTESIAN_POINT('Ctrl Pts',(-6.00336761087,2.556767114,4.51817394899));
#109501=CARTESIAN_POINT('Ctrl Pts',(-5.74088811843,2.491440779,4.83014499667));
#109502=CARTESIAN_POINT('',(-5.56373312153948,2.49144077849386,4.83951177315532));
#109503=CARTESIAN_POINT('Ctrl Pts',(-5.40835689678428,2.48690656569021,
4.82834597309885));
#109504=CARTESIAN_POINT('Ctrl Pts',(-5.39920432239215,2.48917367234508,
4.83852043254936));
#109505=CARTESIAN_POINT('Ctrl Pts',(-5.390051748,2.491440779,4.848694892));
#109506=CARTESIAN_POINT('Ctrl Pts',(-5.1246081,2.557191576,5.143775327));
#109507=CARTESIAN_POINT('Ctrl Pts',(-4.828538757,2.622066995,5.408115519));
#109508=CARTESIAN_POINT('Ctrl Pts',(-5.42807519093172,2.48690656569021,
5.17635720151946));
#109509=CARTESIAN_POINT('Ctrl Pts',(-5.41826556660759,2.48917367234508,
5.18656640138796));
#109510=CARTESIAN_POINT('Ctrl Pts',(-5.40845594228348,2.491440779,5.19677560125659));
#109511=CARTESIAN_POINT('Ctrl Pts',(-5.12395648294661,2.557191576,5.49286358046064));
#109512=CARTESIAN_POINT('Ctrl Pts',(-4.80883522364381,2.622066995,5.75612509553517));
#109513=CARTESIAN_POINT('',(-5.40841798908711,2.49144077985043,5.19605762786303));
#109514=CARTESIAN_POINT('',(-4.99977078188444,2.58208164079232,5.59037496954931));
#109515=CARTESIAN_POINT('Origin',(0.145633230011868,2.41074796083966,-0.121959297299493));
#109516=CARTESIAN_POINT('Ctrl Pts',(-4.83205245536802,2.62129679697757,
5.40497632402769));
#109517=CARTESIAN_POINT('Ctrl Pts',(-4.86000044148469,2.61444751346176,
5.43580241133959));
#109518=CARTESIAN_POINT('Ctrl Pts',(-4.88796440292578,2.60775977695734,
5.46668259888027));
#109519=CARTESIAN_POINT('Ctrl Pts',(-4.94386075122956,2.59469807493931,
5.52847363037815));
#109520=CARTESIAN_POINT('Ctrl Pts',(-4.97182367878698,2.58831698223328,
5.55941824246101));
#109521=CARTESIAN_POINT('Ctrl Pts',(-4.99977077658195,2.58208164076771,
5.590374958319));
#109522=CARTESIAN_POINT('',(-5.39923487480582,2.49144078146676,5.02237625242088));
#109523=CARTESIAN_POINT('Origin',(-3.58220397789211E-13,2.58316965299911,
3.24826970876657E-13));
#109524=CARTESIAN_POINT('',(-5.00016107681822,2.40074633453083,5.5900258682109));
#109525=CARTESIAN_POINT('Origin',(0.144328703502746,2.5535510911766,-0.124825772307806));
#109526=CARTESIAN_POINT('',(-4.56489905870438,2.49144077881237,5.95077277843231));
#109527=CARTESIAN_POINT('Origin',(0.127397609975873,2.41071461307179,-0.144818061835398));
#109528=CARTESIAN_POINT('Origin',(0.125161223023721,2.5535712640916,-0.146797725607393));
#109529=CARTESIAN_POINT('Ctrl Pts',(-4.835549645,2.622074631,5.401847798));
#109530=CARTESIAN_POINT('Ctrl Pts',(-4.542002709,2.556767114,5.664620989));
#109531=CARTESIAN_POINT('Ctrl Pts',(-4.221709258,2.491440779,5.894036897));
#109532=CARTESIAN_POINT('Ctrl Pts',(-5.182866615,2.622074631,5.421060196));
#109533=CARTESIAN_POINT('Ctrl Pts',(-4.88827564,2.556767114,5.702707268));
#109534=CARTESIAN_POINT('Ctrl Pts',(-4.564899051,2.491440779,5.95077277800001));
#109535=CARTESIAN_POINT('Ctrl Pts',(-5.1863397847,2.622074631,5.42125231998));
#109536=CARTESIAN_POINT('Ctrl Pts',(-4.89173836931,2.556767114,5.70308813079));
#109537=CARTESIAN_POINT('Ctrl Pts',(-4.56833094893,2.491440779,5.95134013681001));
#109538=CARTESIAN_POINT('',(-4.39330415699558,2.49144077849392,5.92240483564876));
#109539=CARTESIAN_POINT('Ctrl Pts',(-4.24396085842985,2.48690656573101,
5.878098790588));
#109540=CARTESIAN_POINT('Ctrl Pts',(-4.23283505821495,2.48917367236547,
5.88606784379398));
#109541=CARTESIAN_POINT('Ctrl Pts',(-4.221709258,2.491440779,5.894036897));
#109542=CARTESIAN_POINT('Ctrl Pts',(-3.899037964,2.557191576,6.125155977));
#109543=CARTESIAN_POINT('Ctrl Pts',(-3.553065231,2.622066995,6.31966988600001));
#109544=CARTESIAN_POINT('Ctrl Pts',(-4.18840602291764,2.486906565731,6.22221255992507));
#109545=CARTESIAN_POINT('Ctrl Pts',(-4.17663106608019,2.48917367236548,
6.23007429505655));
#109546=CARTESIAN_POINT('Ctrl Pts',(-4.16485610924274,2.491440779,6.23793603018786));
#109547=CARTESIAN_POINT('Ctrl Pts',(-3.82335792608898,2.557191576,6.46594266332069));
#109548=CARTESIAN_POINT('Ctrl Pts',(-3.45901058282517,2.622066995,6.65530751465221));
#109549=CARTESIAN_POINT('',(-4.16497338460572,2.49144077985039,6.23722668575043));
#109550=CARTESIAN_POINT('',(-3.6811135513713,2.58208164079298,6.53447803534407));
#109551=CARTESIAN_POINT('Origin',(0.116010728969889,2.41074796290915,-0.150414734490522));
#109552=CARTESIAN_POINT('Ctrl Pts',(-3.55717161529104,2.62129679695473,
6.31735942486863));
#109553=CARTESIAN_POINT('Ctrl Pts',(-3.57783949549941,2.61444751335948,
6.35347280667645));
#109554=CARTESIAN_POINT('Ctrl Pts',(-3.59851134755322,2.60775977681711,
6.38964245789835));
#109555=CARTESIAN_POINT('Ctrl Pts',(-3.6398176296258,2.59469807329828,6.46200492028157));
#109556=CARTESIAN_POINT('Ctrl Pts',(-3.66047462828288,2.58831697893288,
6.49823727743706));
#109557=CARTESIAN_POINT('Ctrl Pts',(-3.68111354872381,2.58208164075444,
6.53447802327984));
#109558=CARTESIAN_POINT('',(-4.19334132994659,2.49144078146676,6.06563178439533));
#109559=CARTESIAN_POINT('Origin',(-6.54858112181245E-14,2.58316965300011,
-2.73218947466347E-14));
#109560=CARTESIAN_POINT('',(-3.68156976764956,2.40074633450494,6.53422099774582));
#109561=CARTESIAN_POINT('Origin',(0.114120472869241,2.55355107061601,-0.152933734037438));
#109562=CARTESIAN_POINT('',(-3.17893401143449,2.49144077881209,6.79296537807907));
#109563=CARTESIAN_POINT('Origin',(0.0932874242503334,2.41071459168756,-0.16881882010749));
#109564=CARTESIAN_POINT('Origin',(0.0906779232206405,2.55357127085558,-0.170271772113147));
#109565=CARTESIAN_POINT('Ctrl Pts',(-3.561259582,2.622074631,6.315055834));
#109566=CARTESIAN_POINT('Ctrl Pts',(-3.218087142,2.556767114,6.50858162));
#109567=CARTESIAN_POINT('Ctrl Pts',(-2.855964336,2.491440779,6.663780287));
#109568=CARTESIAN_POINT('Ctrl Pts',(-3.896326377,2.622074631,6.408481939));
#109569=CARTESIAN_POINT('Ctrl Pts',(-3.54807698,2.556767114,6.620215907));
#109570=CARTESIAN_POINT('Ctrl Pts',(-3.178934004,2.491440779,6.792965376));
#109571=CARTESIAN_POINT('Ctrl Pts',(-3.89967704495,2.622074631,6.40941620005));
#109572=CARTESIAN_POINT('Ctrl Pts',(-3.55137687838,2.556767114,6.62133224987001));
#109573=CARTESIAN_POINT('Ctrl Pts',(-3.18216370068,2.491440779,6.79425722688999));
#109574=CARTESIAN_POINT('',(-3.01744917283955,2.49144077849314,6.72837283022655));
#109575=CARTESIAN_POINT('Ctrl Pts',(-2.88112192769865,2.48690656581069,
6.65299824113503));
#109576=CARTESIAN_POINT('Ctrl Pts',(-2.86854313184929,2.48917367240532,
6.65838926406759));
#109577=CARTESIAN_POINT('Ctrl Pts',(-2.855964336,2.491440779,6.663780287));
#109578=CARTESIAN_POINT('Ctrl Pts',(-2.491153147,2.557191576,6.820131142));
#109579=CARTESIAN_POINT('Ctrl Pts',(-2.111454323,2.622066995,6.935723513));
#109580=CARTESIAN_POINT('Ctrl Pts',(-2.75289164418675,2.48690656581069,
6.97712417427914));
#109581=CARTESIAN_POINT('Ctrl Pts',(-2.73970193885012,2.48917367240532,
6.98227083867556));
#109582=CARTESIAN_POINT('Ctrl Pts',(-2.72651223351355,2.491440779,6.98741750307182));
#109583=CARTESIAN_POINT('Ctrl Pts',(-2.34398340133904,2.557191576,7.1366814533166));
#109584=CARTESIAN_POINT('Ctrl Pts',(-1.94744645129448,2.622066995,7.24329515151907));
#109585=CARTESIAN_POINT('',(-2.72677925511041,2.49144077985039,6.9867499534755));
#109586=CARTESIAN_POINT('',(-2.1903315421454,2.58208164079196,7.17303617095425));
#109587=CARTESIAN_POINT('Origin',(0.0809637820517822,2.41074797514361,-0.171837106840123));
#109588=CARTESIAN_POINT('Ctrl Pts',(-2.11596138345152,2.62129679691413,
6.93434982023637));
#109589=CARTESIAN_POINT('Ctrl Pts',(-2.1283827246779,2.61444752758119,6.97406179194022));
#109590=CARTESIAN_POINT('Ctrl Pts',(-2.14079584527957,2.60775980576447,
7.01382956018076));
#109591=CARTESIAN_POINT('Ctrl Pts',(-2.16558067114611,2.59469807468317,
7.09338002604718));
#109592=CARTESIAN_POINT('Ctrl Pts',(-2.17796583179262,2.58831698174837,
7.13320592542989));
#109593=CARTESIAN_POINT('Ctrl Pts',(-2.1903315420636,2.58208164076534,7.17303615854577));
#109594=CARTESIAN_POINT('',(-2.7913718055054,2.49144078146677,6.82526511527213));
#109595=CARTESIAN_POINT('Origin',(4.62737487216813E-13,2.58316965300044,
-1.26721549920106E-12));
#109596=CARTESIAN_POINT('',(-2.19083234810414,2.40074633453921,7.17288321534959));
#109597=CARTESIAN_POINT('Origin',(0.0785761618095226,2.55355108003917,-0.173890731842352));
#109598=CARTESIAN_POINT('',(-1.64432554279914,2.4914407788121,7.31752646662564));
#109599=CARTESIAN_POINT('Origin',(0.0548153802276763,2.41071457910362,-0.184926017836832));
#109600=CARTESIAN_POINT('Origin',(0.0519544797054261,2.55357126758846,-0.185783815545175));
#109601=CARTESIAN_POINT('Ctrl Pts',(-2.12044898,2.622074631,6.932978878));
#109602=CARTESIAN_POINT('Ctrl Pts',(-1.743697397,2.556767114,7.048208208));
#109603=CARTESIAN_POINT('Ctrl Pts',(-1.356677695,2.491440779,7.121932718));
#109604=CARTESIAN_POINT('Ctrl Pts',(-2.427598248,2.622074631,7.096250189));
#109605=CARTESIAN_POINT('Ctrl Pts',(-2.041974184,2.556767114,7.228170609));
#109606=CARTESIAN_POINT('Ctrl Pts',(-1.644325536,2.491440779,7.317526463));
#109607=CARTESIAN_POINT('Ctrl Pts',(-2.43066974068,2.622074631,7.09788290211));
#109608=CARTESIAN_POINT('Ctrl Pts',(-2.04495695187,2.556767114,7.22997023301));
#109609=CARTESIAN_POINT('Ctrl Pts',(-1.64720201441,2.491440779,7.31948240044999));
#109610=CARTESIAN_POINT('',(-1.50050161854692,2.49144077849314,7.21972958986675));
#109611=CARTESIAN_POINT('Ctrl Pts',(-1.38356493859898,2.48690656559387,
7.1168108876931));
#109612=CARTESIAN_POINT('Ctrl Pts',(-1.37012131679948,2.48917367229691,
7.11937180234655));
#109613=CARTESIAN_POINT('Ctrl Pts',(-1.356677695,2.491440779,7.121932717));
#109614=CARTESIAN_POINT('Ctrl Pts',(-0.966784777,2.557191576,7.196204554));
#109615=CARTESIAN_POINT('Ctrl Pts',(-0.571114157,2.622066995,7.227470416));
#109616=CARTESIAN_POINT('Ctrl Pts',(-1.18865511346413,2.48690656559387,
7.40579321700299));
#109617=CARTESIAN_POINT('Ctrl Pts',(-1.17466739474133,2.48917367229691,
7.40798415859763));
#109618=CARTESIAN_POINT('Ctrl Pts',(-1.16067967601852,2.491440779,7.41017510019224));
#109619=CARTESIAN_POINT('Ctrl Pts',(-0.755006818633824,2.557191576,7.47371695105929));
#109620=CARTESIAN_POINT('Ctrl Pts',(-0.344821887789227,2.622066995,7.49259435609274));
#109621=CARTESIAN_POINT('',(-1.16108395826105,2.49144077985039,7.40958055924775));
#109622=CARTESIAN_POINT('',(-0.597132064662066,2.58208164077664,7.47619110706454));
#109623=CARTESIAN_POINT('Origin',(0.0421309546760995,2.41074796189775,-0.185224158370121));
#109624=CARTESIAN_POINT('Ctrl Pts',(-0.575811147771544,2.62129679698884,
7.22709772421984));
#109625=CARTESIAN_POINT('Ctrl Pts',(-0.579405185147711,2.61444752745383,
7.26855147446483));
#109626=CARTESIAN_POINT('Ctrl Pts',(-0.582979199524533,2.60775980541408,
7.31005794984184));
#109627=CARTESIAN_POINT('Ctrl Pts',(-0.590083571131229,2.59469807517952,
7.39307656959251));
#109628=CARTESIAN_POINT('Ctrl Pts',(-0.593617782357874,2.58831698274238,
7.43463380158057));
#109629=CARTESIAN_POINT('Ctrl Pts',(-0.597132067174118,2.58208164075448,
7.47619109490713));
#109630=CARTESIAN_POINT('',(-1.25888083740932,2.49144078146678,7.26575663541678));
#109631=CARTESIAN_POINT('Origin',(-1.6554411921138E-14,2.58316965300056,
5.00467722819309E-13));
#109632=CARTESIAN_POINT('',(-0.597654043017649,2.4007463345303,7.47614938614282));
#109633=CARTESIAN_POINT('Origin',(0.0393577243934989,2.55355107526744,-0.186716797871721));
#109634=CARTESIAN_POINT('',(-0.03283023986312,2.49144077881205,7.4999281500093));
#109635=CARTESIAN_POINT('Origin',(0.0137802080897542,2.41071457200419,-0.192386363698522));
#109636=CARTESIAN_POINT('Origin',(0.010801788896734,2.55357128359452,-0.192608996550105));
#109637=CARTESIAN_POINT('Ctrl Pts',(-0.580488539,2.622074631,7.226723535));
#109638=CARTESIAN_POINT('Ctrl Pts',(-0.1877743,2.556767114,7.258268414));
#109639=CARTESIAN_POINT('Ctrl Pts',(0.206045687,2.491440779,7.24707149));
#109640=CARTESIAN_POINT('Ctrl Pts',(-0.845358323000001,2.622074631,7.452205667));
#109641=CARTESIAN_POINT('Ctrl Pts',(-0.440390945,2.556767114,7.498144086));
#109642=CARTESIAN_POINT('Ctrl Pts',(-0.032830234,2.491440779,7.499928145));
#109643=CARTESIAN_POINT('Ctrl Pts',(-0.848007020840001,2.622074631,7.45446048832));
#109644=CARTESIAN_POINT('Ctrl Pts',(-0.44291711145,2.556767114,7.50054284272));
#109645=CARTESIAN_POINT('Ctrl Pts',(-0.03521899321,2.491440779,7.50245671154999));
#109646=CARTESIAN_POINT('',(0.086607723388183,2.49144077849314,7.37349981753655));
#109647=CARTESIAN_POINT('Ctrl Pts',(-1.641068979,3.266573167,7.318257484));
#109648=CARTESIAN_POINT('Ctrl Pts',(-1.244023089,3.330825242,7.407292298));
#109649=CARTESIAN_POINT('Ctrl Pts',(-0.839675095000001,3.395965514,7.452848163));
#109650=CARTESIAN_POINT('Ctrl Pts',(-1.353508207,3.266573167,7.122535752));
#109651=CARTESIAN_POINT('Ctrl Pts',(-0.967081035,3.330825242,7.195969198));
#109652=CARTESIAN_POINT('Ctrl Pts',(-0.574977339,3.395965514,7.227164109));
#109653=CARTESIAN_POINT('',(-0.839675102516549,3.39596551397696,7.45284816193034));
#109654=CARTESIAN_POINT('',(-0.707326224613764,3.39596551522583,7.3400061352663));
#109655=CARTESIAN_POINT('',(-1.39547228497567,3.30628897739669,7.36903366125719));
#109656=CARTESIAN_POINT('Origin',(0.00745224377008552,3.48210502434058,
-0.189556297375185));
#109657=CARTESIAN_POINT('Ctrl Pts',(-1.34892078857225,3.26733592495805,
7.12340597695071));
#109658=CARTESIAN_POINT('Ctrl Pts',(-1.35655738881502,3.27415053067158,
7.16430599565868));
#109659=CARTESIAN_POINT('Ctrl Pts',(-1.36426297460565,3.28079893120748,
7.20524768819475));
#109660=CARTESIAN_POINT('Ctrl Pts',(-1.3797808582022,3.29377261882018,7.28710885345242));
#109661=CARTESIAN_POINT('Ctrl Pts',(-1.38760239032622,3.30010561499173,
7.3280769990597));
#109662=CARTESIAN_POINT('Ctrl Pts',(-1.39547228151228,3.30628897727386,
7.36903366194122));
#109663=CARTESIAN_POINT('Ctrl Pts',(-1.95959162658564,3.39726054241129,
7.23947982964322));
#109664=CARTESIAN_POINT('Ctrl Pts',(-1.95562373629282,3.39661302820565,
7.24054919782161));
#109665=CARTESIAN_POINT('Ctrl Pts',(-1.951655846,3.395965514,7.241618566));
#109666=CARTESIAN_POINT('Ctrl Pts',(-1.832291891,3.376486685,7.273787806));
#109667=CARTESIAN_POINT('Ctrl Pts',(-1.711932572,3.357142857,7.302005674));
#109668=CARTESIAN_POINT('Ctrl Pts',(-1.432141907,3.31217565,7.367601728));
#109669=CARTESIAN_POINT('Ctrl Pts',(-1.148152096,3.266554913,7.411595426));
#109670=CARTESIAN_POINT('Ctrl Pts',(-2.12276066440802,3.39726054241129,
6.93227598202677));
#109671=CARTESIAN_POINT('Ctrl Pts',(-2.11896100170401,3.39661302820565,
6.93343493951338));
#109672=CARTESIAN_POINT('Ctrl Pts',(-2.115161339,3.395965514,6.934593897));
#109673=CARTESIAN_POINT('Ctrl Pts',(-2.000858086,3.376486685,6.969458205));
#109674=CARTESIAN_POINT('Ctrl Pts',(-1.885467899,3.357142857,7.000536465));
#109675=CARTESIAN_POINT('Ctrl Pts',(-1.617228618,3.31217565,7.072781865));
#109676=CARTESIAN_POINT('Ctrl Pts',(-1.344247503,3.266554913,7.124289344));
#109677=CARTESIAN_POINT('',(-1.95165584931786,3.39596551355058,7.24161856620618));
#109678=CARTESIAN_POINT('Ctrl Pts',(-1.39547228792016,3.30628897830869,
7.36903366077302));
#109679=CARTESIAN_POINT('Ctrl Pts',(-1.50164913379404,3.32334891375385,
7.34892697479509));
#109680=CARTESIAN_POINT('Ctrl Pts',(-1.60718233601057,3.34030767936807,
7.3265640420645));
#109681=CARTESIAN_POINT('Ctrl Pts',(-1.71193257096189,3.35714285683316,
7.30200567424338));
#109682=CARTESIAN_POINT('Ctrl Pts',(-1.79202337301739,3.37001483643651,
7.28322863481056));
#109683=CARTESIAN_POINT('Ctrl Pts',(-1.87195374174027,3.38295904433187,
7.26309871975793));
#109684=CARTESIAN_POINT('Ctrl Pts',(-1.95165584885848,3.39596551444773,
7.24161856504488));
#109685=CARTESIAN_POINT('',(-2.03340860029504,3.3959655126796,7.08810622926379));
#109686=CARTESIAN_POINT('Origin',(4.20670442924376E-14,3.48737837500078,
-6.15826833971767E-13));
#109687=CARTESIAN_POINT('',(-1.4027848099639,3.4862983196521,7.36764513069795));
#109688=CARTESIAN_POINT('Origin',(0.0563618769074783,3.62489370122117,-0.177672047855243));
#109689=CARTESIAN_POINT('Origin',(0.0367081618178045,3.48214200415296,-0.189266476659903));
#109690=CARTESIAN_POINT('Ctrl Pts',(-3.175910731,3.266573167,6.794379371));
#109691=CARTESIAN_POINT('Ctrl Pts',(-2.807287406,3.330825242,6.96668573));
#109692=CARTESIAN_POINT('Ctrl Pts',(-2.422186008,3.395965514,7.098099389));
#109693=CARTESIAN_POINT('Ctrl Pts',(-2.852998583,3.266573167,6.66505056900001));
#109694=CARTESIAN_POINT('Ctrl Pts',(-2.491391884,3.330825242,6.819837601));
#109695=CARTESIAN_POINT('Ctrl Pts',(-2.115161339,3.395965514,6.934593897));
#109696=CARTESIAN_POINT('',(-2.42218601520096,3.39596551397697,7.09809938660105));
#109697=CARTESIAN_POINT('',(-2.26867368077813,3.39596551522584,7.01634664064668));
#109698=CARTESIAN_POINT('',(-2.94697132857873,3.30628897732248,6.89676445798204));
#109699=CARTESIAN_POINT('Origin',(0.0480269488321092,3.48210505014218,-0.183522448319748));
#109700=CARTESIAN_POINT('Ctrl Pts',(-2.84870548848616,3.26733592487573,
6.6668866075392));
#109701=CARTESIAN_POINT('Ctrl Pts',(-2.86495564557713,3.27415044722697,
6.70518829485233));
#109702=CARTESIAN_POINT('Ctrl Pts',(-2.88128210332557,3.28079876150916,
6.74351578730517));
#109703=CARTESIAN_POINT('Ctrl Pts',(-2.91403550111338,3.29377268004841,
6.82012856164089));
#109704=CARTESIAN_POINT('Ctrl Pts',(-2.93048128834732,3.30010573966433,
6.85845790751624));
#109705=CARTESIAN_POINT('Ctrl Pts',(-2.94697132493218,3.30628897718608,
6.89676445955767));
#109706=CARTESIAN_POINT('Ctrl Pts',(-3.47005162939067,3.39726054241129,
6.64897053993111));
#109707=CARTESIAN_POINT('Ctrl Pts',(-3.46640638869534,3.39661302820565,
6.65086788596556));
#109708=CARTESIAN_POINT('Ctrl Pts',(-3.462761148,3.395965514,6.652765232));
#109709=CARTESIAN_POINT('Ctrl Pts',(-3.353103291,3.376486685,6.709842094));
#109710=CARTESIAN_POINT('Ctrl Pts',(-3.241623914,3.357142857,6.763273941));
#109711=CARTESIAN_POINT('Ctrl Pts',(-2.982475812,3.31217565,6.887483117));
#109712=CARTESIAN_POINT('Ctrl Pts',(-2.71458287,3.266554913,6.991497682));
#109713=CARTESIAN_POINT('Ctrl Pts',(-3.56336611914593,3.39726054241129,
6.31387242722714));
#109714=CARTESIAN_POINT('Ctrl Pts',(-3.55990443207297,3.39661302820565,
6.31582110411357));
#109715=CARTESIAN_POINT('Ctrl Pts',(-3.556442745,3.395965514,6.317769781));
#109716=CARTESIAN_POINT('Ctrl Pts',(-3.452306635,3.376486685,6.376390802));
#109717=CARTESIAN_POINT('Ctrl Pts',(-3.346295113,3.357142857,6.431547949));
#109718=CARTESIAN_POINT('Ctrl Pts',(-3.099857743,3.31217565,6.55976780700001));
#109719=CARTESIAN_POINT('Ctrl Pts',(-2.84433136,3.266554913,6.66875394));
#109720=CARTESIAN_POINT('',(-3.46276115493587,3.39596551397716,6.65276522825413));
#109721=CARTESIAN_POINT('Ctrl Pts',(-2.94697133156129,3.3062889783089,6.89676445651874));
#109722=CARTESIAN_POINT('Ctrl Pts',(-3.04634347853802,3.32334891375403,
6.85430297046257));
#109723=CARTESIAN_POINT('Ctrl Pts',(-3.14460200356063,3.34030767936782,
6.80977635198074));
#109724=CARTESIAN_POINT('Ctrl Pts',(-3.24162391269816,3.35714285675915,
6.76327394139216));
#109725=CARTESIAN_POINT('Ctrl Pts',(-3.3158057287211,3.37001483655547,6.72771874213896));
#109726=CARTESIAN_POINT('Ctrl Pts',(-3.38954003520254,3.38295904483435,
6.69087678604438));
#109727=CARTESIAN_POINT('Ctrl Pts',(-3.46276115484867,3.39596551520491,
6.652765228235));
#109728=CARTESIAN_POINT('',(-3.50960195363195,3.39596551267963,6.48526750264044));
#109729=CARTESIAN_POINT('Origin',(-2.74736830507827E-13,3.48737837500022,
8.58254439739525E-13));
#109730=CARTESIAN_POINT('',(-2.95381439771736,3.48629831963313,6.89383641367548));
#109731=CARTESIAN_POINT('Origin',(0.093238293760558,3.62489371327987,-0.161401769541824));
#109732=CARTESIAN_POINT('Origin',(0.076536543906639,3.48214199689222,-0.176950158017798));
#109733=CARTESIAN_POINT('Ctrl Pts',(-4.56225042700001,3.266573167,5.952803629));
#109734=CARTESIAN_POINT('Ctrl Pts',(-4.239286085,3.330825242,6.20032467900001));
#109735=CARTESIAN_POINT('Ctrl Pts',(-3.891438196,3.395965514,6.411451378));
#109736=CARTESIAN_POINT('Ctrl Pts',(-4.219085917,3.266573167,5.895915029));
#109737=CARTESIAN_POINT('Ctrl Pts',(-3.899208018,3.330825242,6.124817978));
#109738=CARTESIAN_POINT('Ctrl Pts',(-3.556442745,3.395965514,6.317769781));
#109739=CARTESIAN_POINT('',(-3.89143820237509,3.39596551397697,6.41145137387599));
#109740=CARTESIAN_POINT('',(-3.72394047710203,3.39596551522583,6.36461057563715));
#109741=CARTESIAN_POINT('',(-4.36067326829594,3.306288977333,6.10201021368914));
#109742=CARTESIAN_POINT('Origin',(0.0863561497287396,3.48210502566653,-0.168907609084561));
#109743=CARTESIAN_POINT('Ctrl Pts',(-4.2152878865285,3.26733592487922,5.89863103039522));
#109744=CARTESIAN_POINT('Ctrl Pts',(-4.23939214923398,3.27415053058325,
5.9325443570056));
#109745=CARTESIAN_POINT('Ctrl Pts',(-4.26357651993798,3.28079893111318,
5.96646653943243));
#109746=CARTESIAN_POINT('Ctrl Pts',(-4.31203278075909,3.29377261872553,
6.03424593089019));
#109747=CARTESIAN_POINT('Ctrl Pts',(-4.33633348893587,3.30010561490405,
6.0681434368539));
#109748=CARTESIAN_POINT('Ctrl Pts',(-4.36067326513809,3.3062889771908,6.10201021589449));
#109749=CARTESIAN_POINT('Ctrl Pts',(-4.81825587435657,3.3972605424113,5.74756277776071));
#109750=CARTESIAN_POINT('Ctrl Pts',(-4.81510373067828,3.39661302820565,
5.75019938388036));
#109751=CARTESIAN_POINT('Ctrl Pts',(-4.811951587,3.395965514,5.75283599));
#109752=CARTESIAN_POINT('Ctrl Pts',(-4.717127308,3.376486685,5.832151624));
#109753=CARTESIAN_POINT('Ctrl Pts',(-4.619740525,3.357142857,5.908299035));
#109754=CARTESIAN_POINT('Ctrl Pts',(-4.393352463,3.31217565,6.085313451));
#109755=CARTESIAN_POINT('Ctrl Pts',(-4.154082765,3.266554913,6.244485277));
#109756=CARTESIAN_POINT('Ctrl Pts',(-4.83735253472087,3.3972605424113,5.40023921543882));
#109757=CARTESIAN_POINT('Ctrl Pts',(-4.83439068786043,3.39661302820565,
5.40288649371941));
#109758=CARTESIAN_POINT('Ctrl Pts',(-4.831428841,3.395965514,5.405533772));
#109759=CARTESIAN_POINT('Ctrl Pts',(-4.742329161,3.376486685,5.485170451));
#109760=CARTESIAN_POINT('Ctrl Pts',(-4.650653287,3.357142857,5.561827398));
#109761=CARTESIAN_POINT('Ctrl Pts',(-4.437540965,3.31217565,5.740026298));
#109762=CARTESIAN_POINT('Ctrl Pts',(-4.211417444,3.266554913,5.901395014));
#109763=CARTESIAN_POINT('',(-4.81195159120568,3.39596551354713,5.7528359871114));
#109764=CARTESIAN_POINT('Ctrl Pts',(-4.36067327090021,3.30628897830886,
6.10201021177672));
#109765=CARTESIAN_POINT('Ctrl Pts',(-4.44859418812871,3.32334891375399,
6.03917937748522));
#109766=CARTESIAN_POINT('Ctrl Pts',(-4.5349835767243,3.34030767936764,5.9745710882284));
#109767=CARTESIAN_POINT('Ctrl Pts',(-4.61974052367493,3.3571428567285,5.90829903560032));
#109768=CARTESIAN_POINT('Ctrl Pts',(-4.68454469282505,3.37001483650127,
5.85762819936046));
#109769=CARTESIAN_POINT('Ctrl Pts',(-4.74863520074109,3.3829590448342,5.80579689162175));
#109770=CARTESIAN_POINT('Ctrl Pts',(-4.81195159287912,3.39596551520488,
5.75283598485012));
#109771=CARTESIAN_POINT('',(-4.82169022013556,3.39596551267962,5.57918487569748));
#109772=CARTESIAN_POINT('Origin',(-3.33283747822044E-13,3.48737837499933,
3.5301622736128E-13));
#109773=CARTESIAN_POINT('',(-4.36672690753549,3.48629831964532,6.09767956787773));
#109774=CARTESIAN_POINT('Origin',(0.125755312071149,3.62489371866856,-0.137585200598519));
#109775=CARTESIAN_POINT('Origin',(0.112786245811037,3.48214197539546,-0.156360099239026));
#109776=CARTESIAN_POINT('Ctrl Pts',(-5.735264364,3.266573167,4.832881405));
#109777=CARTESIAN_POINT('Ctrl Pts',(-5.473060458,3.330825242,5.144043338));
#109778=CARTESIAN_POINT('Ctrl Pts',(-5.178731058,3.395965514,5.425011025));
#109779=CARTESIAN_POINT('Ctrl Pts',(-5.387893482,3.266573167,4.851093055));
#109780=CARTESIAN_POINT('Ctrl Pts',(-5.124701518,3.330825242,5.143408673));
#109781=CARTESIAN_POINT('Ctrl Pts',(-4.831428841,3.395965514,5.40553377200001));
#109782=CARTESIAN_POINT('',(-5.17873106354357,3.39596551397697,5.42501101981538));
#109783=CARTESIAN_POINT('',(-5.00507995511728,3.39596551522583,5.41527239330822));
#109784=CARTESIAN_POINT('',(-5.57047497242684,3.30628897733851,5.02193275359628));
#109785=CARTESIAN_POINT('Origin',(0.120647090505832,3.4821050288845,-0.146394402571267));
#109786=CARTESIAN_POINT('Ctrl Pts',(-5.38476810741094,3.26733592498887,
4.85456202254788));
#109787=CARTESIAN_POINT('Ctrl Pts',(-5.41559918872214,3.27415053066729,
4.88250077028925));
#109788=CARTESIAN_POINT('Ctrl Pts',(-5.44651040880628,3.28079893117115,
4.91043094599988));
#109789=CARTESIAN_POINT('Ctrl Pts',(-5.50840435484866,3.2937726187527,4.96620902910849));
#109790=CARTESIAN_POINT('Ctrl Pts',(-5.5394238877264,3.30010561491808,4.99409009625292));
#109791=CARTESIAN_POINT('Ctrl Pts',(-5.57047496986067,3.30628897720077,
5.02193275641807));
#109792=CARTESIAN_POINT('Ctrl Pts',(-5.9411638298455,3.3972605424113,4.5774053670745));
#109793=CARTESIAN_POINT('Ctrl Pts',(-5.93865217392275,3.39661302820565,
4.58065794853726));
#109794=CARTESIAN_POINT('Ctrl Pts',(-5.936140518,3.395965514,4.58391053));
#109795=CARTESIAN_POINT('Ctrl Pts',(-5.860583695,3.376486685,4.681756226));
#109796=CARTESIAN_POINT('Ctrl Pts',(-5.781843203,3.357142857,4.777058632));
#109797=CARTESIAN_POINT('Ctrl Pts',(-5.598800835,3.31217565,4.998601291));
#109798=CARTESIAN_POINT('Ctrl Pts',(-5.39934236800001,3.266554913,5.205487681));
#109799=CARTESIAN_POINT('Ctrl Pts',(-5.88514972182881,3.3972605424113,4.23409681912444));
#109800=CARTESIAN_POINT('Ctrl Pts',(-5.88282620791441,3.39661302820565,
4.23731891506222));
#109801=CARTESIAN_POINT('Ctrl Pts',(-5.880502694,3.395965514,4.240541011));
#109802=CARTESIAN_POINT('Ctrl Pts',(-5.810605648,3.376486685,4.337469627));
#109803=CARTESIAN_POINT('Ctrl Pts',(-5.737552082,3.357142857,4.43204198));
#109804=CARTESIAN_POINT('Ctrl Pts',(-5.567729703,3.31217565,4.651887538));
#109805=CARTESIAN_POINT('Ctrl Pts',(-5.381582328,3.266554913,4.858093417));
#109806=CARTESIAN_POINT('',(-5.93614052278745,3.39596551397716,4.58391052373854));
#109807=CARTESIAN_POINT('Ctrl Pts',(-5.57047497456071,3.3062889783089,5.02193275120465));
#109808=CARTESIAN_POINT('Ctrl Pts',(-5.64283357730374,3.32334891375403,
4.94167046845604));
#109809=CARTESIAN_POINT('Ctrl Pts',(-5.71331435752237,3.34030767936776,
4.86000152005898));
#109810=CARTESIAN_POINT('Ctrl Pts',(-5.78184320195352,3.3571428567475,4.77705863309879));
#109811=CARTESIAN_POINT('Ctrl Pts',(-5.83423955398265,3.37001483653487,
4.71364147256023));
#109812=CARTESIAN_POINT('Ctrl Pts',(-5.88568946219912,3.38295904483425,
4.64924438689859));
#109813=CARTESIAN_POINT('Ctrl Pts',(-5.93614052263486,3.39596551520492,
4.58391052370727));
#109814=CARTESIAN_POINT('',(-5.90832161085222,3.39596551267962,4.41222576400249));
#109815=CARTESIAN_POINT('Origin',(1.10415149245924E-12,3.48737837500033,
-1.05644659686988E-12));
#109816=CARTESIAN_POINT('',(-5.5754561197949,3.48629831964252,5.01640200242548));
#109817=CARTESIAN_POINT('Origin',(0.152391677636978,3.62489374132545,-0.107334577125267));
#109818=CARTESIAN_POINT('Origin',(0.143762229393116,3.48214198317769,-0.128458831607123));
#109819=CARTESIAN_POINT('Ctrl Pts',(-6.640103713,3.266573167,3.486979019));
#109820=CARTESIAN_POINT('Ctrl Pts',(-6.450920607,3.330825242,3.847232247));
#109821=CARTESIAN_POINT('Ctrl Pts',(-6.223872212,3.395965514,4.184903187));
#109822=CARTESIAN_POINT('Ctrl Pts',(-6.304769136,3.266573167,3.579439362));
#109823=CARTESIAN_POINT('Ctrl Pts',(-6.110569671,3.330825242,3.921499296));
#109824=CARTESIAN_POINT('Ctrl Pts',(-5.880502694,3.395965514,4.240541011));
#109825=CARTESIAN_POINT('',(-6.22387221623639,3.39596551397697,4.1849031807028));
#109826=CARTESIAN_POINT('',(-6.05218745736987,3.39596551522583,4.21272209272205));
#109827=CARTESIAN_POINT('',(-6.51980745789167,3.3062889773493,3.70703529982725));
#109828=CARTESIAN_POINT('Origin',(0.149296895945722,3.48210497061754,-0.117036208815399));
#109829=CARTESIAN_POINT('Ctrl Pts',(-6.30246255588907,3.26733592487402,
3.58349908979831));
#109830=CARTESIAN_POINT('Ctrl Pts',(-6.33857882863868,3.27415053057877,
3.60415687415245));
#109831=CARTESIAN_POINT('Ctrl Pts',(-6.37477152392552,3.28079893112066,
3.62478905937302));
#109832=CARTESIAN_POINT('Ctrl Pts',(-6.4472090632051,3.29377261874503,3.66595771307224));
#109833=CARTESIAN_POINT('Ctrl Pts',(-6.48349698199461,3.30010561492302,
3.68651865366252));
#109834=CARTESIAN_POINT('Ctrl Pts',(-6.51980745608699,3.30628897722029,
3.70703530306007));
#109835=CARTESIAN_POINT('Ctrl Pts',(-6.78626956786007,3.3972605424113,3.19321356957691));
#109836=CARTESIAN_POINT('Ctrl Pts',(-6.78451584193003,3.39661302820565,
3.19693003928845));
#109837=CARTESIAN_POINT('Ctrl Pts',(-6.78276211600001,3.395965514,3.200646509));
#109838=CARTESIAN_POINT('Ctrl Pts',(-6.730005702,3.376486685,3.312447111));
#109839=CARTESIAN_POINT('Ctrl Pts',(-6.673593319,3.357142857,3.422448278));
#109840=CARTESIAN_POINT('Ctrl Pts',(-6.542455503,3.31217565,3.678160091));
#109841=CARTESIAN_POINT('Ctrl Pts',(-6.392134722,3.266554913,3.923087266));
#109842=CARTESIAN_POINT('Ctrl Pts',(-6.65776384915911,3.3972605424113,2.86997276216926));
#109843=CARTESIAN_POINT('Ctrl Pts',(-6.65618731307956,3.39661302820565,
2.87361901408463));
#109844=CARTESIAN_POINT('Ctrl Pts',(-6.65461077700001,3.395965514,2.877265266));
#109845=CARTESIAN_POINT('Ctrl Pts',(-6.60718467200001,3.376486685,2.986953543));
#109846=CARTESIAN_POINT('Ctrl Pts',(-6.556169318,3.357142857,3.095019205));
#109847=CARTESIAN_POINT('Ctrl Pts',(-6.437577588,3.31217565,3.346231687));
#109848=CARTESIAN_POINT('Ctrl Pts',(-6.300110404,3.266554913,3.58763277));
#109849=CARTESIAN_POINT('',(-6.78276211930252,3.39596551397715,3.20064650184279));
#109850=CARTESIAN_POINT('Ctrl Pts',(-6.51980745952236,3.30628897830886,
3.70703529715327));
#109851=CARTESIAN_POINT('Ctrl Pts',(-6.57322034014727,3.32334891375399,
3.61309454144891));
#109852=CARTESIAN_POINT('Ctrl Pts',(-6.62449690909045,3.34030767936783,
3.5181836834444));
#109853=CARTESIAN_POINT('Ctrl Pts',(-6.67359331829069,3.35714285676664,
3.4224482792469));
#109854=CARTESIAN_POINT('Ctrl Pts',(-6.71113185794451,3.3700148365687,3.34925010973637));
#109855=CARTESIAN_POINT('Ctrl Pts',(-6.74753542590834,3.38295904483419,
3.27529838263715));
#109856=CARTESIAN_POINT('Ctrl Pts',(-6.78276211917339,3.39596551520488,
3.20064650185762));
#109857=CARTESIAN_POINT('',(-6.71868644984201,3.39596551267962,3.03895588011132));
#109858=CARTESIAN_POINT('Origin',(-2.38090797077817E-13,3.48737837499967,
5.50774703622636E-14));
#109859=CARTESIAN_POINT('',(-6.52348320100086,3.48629831963772,3.7005630546879));
#109860=CARTESIAN_POINT('Origin',(0.171902718338477,3.62489370565627,-0.0720655235974765));
#109861=CARTESIAN_POINT('Origin',(0.168016080065133,3.48214198897817,-0.0945509470315842));
#109862=CARTESIAN_POINT('Ctrl Pts',(-7.23445919300001,3.266573167,1.978029369));
#109863=CARTESIAN_POINT('Ctrl Pts',(-7.127142877,3.330825242,2.370528853));
#109864=CARTESIAN_POINT('Ctrl Pts',(-6.97799201900001,3.395965514,2.749113927));
#109865=CARTESIAN_POINT('Ctrl Pts',(-6.926840792,3.266573167,2.140415062));
#109866=CARTESIAN_POINT('Ctrl Pts',(-6.810714378,3.330825242,2.516224969));
#109867=CARTESIAN_POINT('Ctrl Pts',(-6.654610777,3.395965514,2.877265266));
#109868=CARTESIAN_POINT('',(-6.97799202168079,3.39596551397697,2.74911391989859));
#109869=CARTESIAN_POINT('',(-6.81630140091813,3.39596551522583,2.81318958942943));
#109870=CARTESIAN_POINT('',(-7.16428099291218,3.30628897730615,2.21880099504165));
#109871=CARTESIAN_POINT('Origin',(0.170965953034417,3.48210502415779,-0.0822056236155499));
#109872=CARTESIAN_POINT('Ctrl Pts',(-6.92546086104984,3.26733592499053,
2.14487572213753));
#109873=CARTESIAN_POINT('Ctrl Pts',(-6.96517356826331,3.27415053065529,
2.15728660792526));
#109874=CARTESIAN_POINT('Ctrl Pts',(-7.00495540816731,3.28079893115101,
2.16965606448942));
#109875=CARTESIAN_POINT('Ctrl Pts',(-7.08454944149771,3.29377261873339,
2.19429028833485));
#109876=CARTESIAN_POINT('Ctrl Pts',(-7.12440896325153,3.30010561488432,
2.20656969571793));
#109877=CARTESIAN_POINT('Ctrl Pts',(-7.16428099180961,3.30628897717171,
2.21880099870381));
#109878=CARTESIAN_POINT('Ctrl Pts',(-7.3140568833428,3.39726054241129,1.65971065413928));
#109879=CARTESIAN_POINT('Ctrl Pts',(-7.31314308967141,3.39661302820565,
1.66371723406964));
#109880=CARTESIAN_POINT('Ctrl Pts',(-7.312229296,3.395965514,1.667723814));
#109881=CARTESIAN_POINT('Ctrl Pts',(-7.284740122,3.376486685,1.788251649));
#109882=CARTESIAN_POINT('Ctrl Pts',(-7.253293629,3.357142857,1.907808045));
#109883=CARTESIAN_POINT('Ctrl Pts',(-7.180192223,3.31217565,2.185732212));
#109884=CARTESIAN_POINT('Ctrl Pts',(-7.086037961,3.266554913,2.457247651));
#109885=CARTESIAN_POINT('Ctrl Pts',(-7.11906833833695,3.39726054241129,
1.37165196852683));
#109886=CARTESIAN_POINT('Ctrl Pts',(-7.11831249716847,3.39661302820565,
1.37555188176341));
#109887=CARTESIAN_POINT('Ctrl Pts',(-7.117556656,3.395965514,1.379451795));
#109888=CARTESIAN_POINT('Ctrl Pts',(-7.094819084,3.376486685,1.496770832));
#109889=CARTESIAN_POINT('Ctrl Pts',(-7.068227363,3.357142857,1.613276771));
#109890=CARTESIAN_POINT('Ctrl Pts',(-7.006411501,3.31217565,1.884109762));
#109891=CARTESIAN_POINT('Ctrl Pts',(-6.92405232,3.266554913,2.149418403));
#109892=CARTESIAN_POINT('',(-7.31222929770336,3.39596551397716,1.6677238063043));
#109893=CARTESIAN_POINT('Ctrl Pts',(-7.16428099403738,3.30628897830889,
2.21880099199275));
#109894=CARTESIAN_POINT('Ctrl Pts',(-7.19625062562276,3.32334891375402,
2.11557432831844));
#109895=CARTESIAN_POINT('Ctrl Pts',(-7.22592534802315,3.3403076793677,2.01185948673362));
#109896=CARTESIAN_POINT('Ctrl Pts',(-7.25329362833298,3.35714285673703,
1.90780804624414));
#109897=CARTESIAN_POINT('Ctrl Pts',(-7.27421909452139,3.37001483651634,
1.82825153253987));
#109898=CARTESIAN_POINT('Ctrl Pts',(-7.29387413230536,3.38295904483434,
1.74820306499536));
#109899=CARTESIAN_POINT('Ctrl Pts',(-7.31222929756424,3.39596551520491,
1.66772380634285));
#109900=CARTESIAN_POINT('',(-7.21489297767553,3.39596551267961,1.52358779656558));
#109901=CARTESIAN_POINT('Origin',(4.46257614195034E-13,3.48737837499967,
-1.83555427801796E-13));
#109902=CARTESIAN_POINT('',(-7.16647945764019,3.48629831962515,2.21168989156009));
#109903=CARTESIAN_POINT('Origin',(0.183375927394167,3.62489371453121,-0.0334267439120248));
#109904=CARTESIAN_POINT('Origin',(0.184413422376409,3.48214204626776,-0.0562218677092333));
#109905=CARTESIAN_POINT('Ctrl Pts',(-7.490539402,3.266573167,0.376589264));
#109906=CARTESIAN_POINT('Ctrl Pts',(-7.470107869,3.330825242,0.782982164));
#109907=CARTESIAN_POINT('Ctrl Pts',(-7.405828674,3.395965514,1.184779155));
#109908=CARTESIAN_POINT('Ctrl Pts',(-7.225021072,3.266573167,0.601307333));
#109909=CARTESIAN_POINT('Ctrl Pts',(-7.19239765,3.330825242,0.993294759999999));
#109910=CARTESIAN_POINT('Ctrl Pts',(-7.117556656,3.395965514,1.379451795));
#109911=CARTESIAN_POINT('',(-7.40582867522515,3.39596551397696,1.1847791475097));
#109912=CARTESIAN_POINT('',(-7.26169266632994,3.39596551522583,1.28211546746747));
#109913=CARTESIAN_POINT('',(-7.47376071103804,3.30628897732951,0.626818022433091));
#109914=CARTESIAN_POINT('Origin',(0.184640406146561,3.48210501342017,-0.0435310537882508));
#109915=CARTESIAN_POINT('Ctrl Pts',(-7.22463231302281,3.26733592498612,
0.605960349825525));
#109916=CARTESIAN_POINT('Ctrl Pts',(-7.26608453277289,3.2741505306695,0.609544017994957));
#109917=CARTESIAN_POINT('Ctrl Pts',(-7.30759536288584,3.28079893118097,
0.613072364018514));
#109918=CARTESIAN_POINT('Ctrl Pts',(-7.39062455165567,3.29377267969189,
0.620020321807375));
#109919=CARTESIAN_POINT('Ctrl Pts',(-7.43219233249536,3.30010573881294,
0.623444059561667));
#109920=CARTESIAN_POINT('Ctrl Pts',(-7.47376071072472,3.30628897719416,
0.626818026364407));
#109921=CARTESIAN_POINT('Ctrl Pts',(-7.49984702782103,3.3972605424113,0.0486015141103514));
#109922=CARTESIAN_POINT('Ctrl Pts',(-7.49981589441051,3.39661302820565,
0.0527108610551757));
#109923=CARTESIAN_POINT('Ctrl Pts',(-7.499784761,3.395965514,0.056820208));
#109924=CARTESIAN_POINT('Ctrl Pts',(-7.498848191,3.376486685,0.180439529));
#109925=CARTESIAN_POINT('Ctrl Pts',(-7.49383799,3.357142857,0.303960829));
#109926=CARTESIAN_POINT('Ctrl Pts',(-7.482191134,3.31217565,0.591101925));
#109927=CARTESIAN_POINT('Ctrl Pts',(-7.44860594,3.266554913,0.876509867));
#109928=CARTESIAN_POINT('Ctrl Pts',(-7.24749310390195,3.3972605424113,-0.190805746883935));
#109929=CARTESIAN_POINT('Ctrl Pts',(-7.24759329995098,3.39661302820565,
-0.186834527941968));
#109930=CARTESIAN_POINT('Ctrl Pts',(-7.247693496,3.395965514,-0.182863309));
#109931=CARTESIAN_POINT('Ctrl Pts',(-7.250707641,3.376486685,-0.06339922));
#109932=CARTESIAN_POINT('Ctrl Pts',(-7.249782953,3.357142857,0.056099309));
#109933=CARTESIAN_POINT('Ctrl Pts',(-7.247633398,3.31217565,0.333888958));
#109934=CARTESIAN_POINT('Ctrl Pts',(-7.224233245,3.266554913,0.61069962));
#109935=CARTESIAN_POINT('',(-7.49978476208606,3.39596551355058,0.0568202048562634));
#109936=CARTESIAN_POINT('Ctrl Pts',(-7.47376071114191,3.30628897830889,
0.626818019136488));
#109937=CARTESIAN_POINT('Ctrl Pts',(-7.48279222925345,3.32334891375402,
0.519132211709427));
#109938=CARTESIAN_POINT('Ctrl Pts',(-7.48947754816551,3.34030767936767,
0.411462977315972));
#109939=CARTESIAN_POINT('Ctrl Pts',(-7.49383798972126,3.35714285673008,
0.303960830511502));
#109940=CARTESIAN_POINT('Ctrl Pts',(-7.497171931789,3.37001483625442,0.221765949147783));
#109941=CARTESIAN_POINT('Ctrl Pts',(-7.49915939119715,3.38295904433211,
0.139363719624729));
#109942=CARTESIAN_POINT('Ctrl Pts',(-7.49978476084517,3.39596551444813,
0.0568202049882929));
#109943=CARTESIAN_POINT('',(-7.37373912843069,3.3959655126796,-0.0630215586091557));
#109944=CARTESIAN_POINT('Origin',(1.33270131041918E-12,3.48737837500044,
-9.09103521629095E-14));
#109945=CARTESIAN_POINT('',(-7.47437910004273,3.48629831962699,0.619400567520625));
#109946=CARTESIAN_POINT('Origin',(0.186274213854775,3.62489373218069,0.00677518458523894));
#109947=CARTESIAN_POINT('Origin',(0.19218808190701,3.48214199745557,-0.0152639929471668));
#109948=CARTESIAN_POINT('Ctrl Pts',(-7.396370313,3.266573167,-1.242459737));
#109949=CARTESIAN_POINT('Ctrl Pts',(-7.463778918,3.330825242,-0.841175901));
#109950=CARTESIAN_POINT('Ctrl Pts',(-7.487377012,3.395965514,-0.434954574));
#109951=CARTESIAN_POINT('Ctrl Pts',(-7.185367396,3.266573167,-0.965916859000001));
#109952=CARTESIAN_POINT('Ctrl Pts',(-7.237772401,3.330825242,-0.576080809));
#109953=CARTESIAN_POINT('Ctrl Pts',(-7.247693496,3.395965514,-0.182863309));
#109954=CARTESIAN_POINT('',(-7.48737701144181,3.39596551397696,-0.434954581569916));
#109955=CARTESIAN_POINT('',(-7.36753525367957,3.39596551522583,-0.30890894914232));
#109956=CARTESIAN_POINT('',(-7.43377568527516,3.30628897737924,-0.994474264932722));
#109957=CARTESIAN_POINT('Origin',(0.189681805221984,3.48210505004052,-0.00282106332404317));
#109958=CARTESIAN_POINT('Ctrl Pts',(-7.18598798705034,3.2673359249808,-0.961289055455298));
#109959=CARTESIAN_POINT('Ctrl Pts',(-7.22724145968924,3.27415053066413,
-0.966700173467491));
#109960=CARTESIAN_POINT('Ctrl Pts',(-7.26854027983182,3.28079893118089,
-0.972177919707717));
#109961=CARTESIAN_POINT('Ctrl Pts',(-7.35112151021921,3.29377261878279,
-0.983241170704317));
#109962=CARTESIAN_POINT('Ctrl Pts',(-7.39245302187789,3.30010561495841,
-0.988833261135669));
#109963=CARTESIAN_POINT('Ctrl Pts',(-7.43377568577855,3.30628897725429,
-0.994474261382158));
#109964=CARTESIAN_POINT('Ctrl Pts',(-7.33495266083656,3.3972605424113,-1.5647801799305));
#109965=CARTESIAN_POINT('Ctrl Pts',(-7.33580564341827,3.39661302820565,
-1.56076021446525));
#109966=CARTESIAN_POINT('Ctrl Pts',(-7.33665862600001,3.395965514,-1.556740249));
#109967=CARTESIAN_POINT('Ctrl Pts',(-7.362318452,3.376486685,-1.435809744));
#109968=CARTESIAN_POINT('Ctrl Pts',(-7.383978815,3.357142857,-1.314099258));
#109969=CARTESIAN_POINT('Ctrl Pts',(-7.43433110500001,3.31217565,-1.031167631));
#109970=CARTESIAN_POINT('Ctrl Pts',(-7.462885385,3.266554913,-0.745212545));
#109971=CARTESIAN_POINT('Ctrl Pts',(-7.03703314764056,3.3972605424113,-1.74434159666193));
#109972=CARTESIAN_POINT('Ctrl Pts',(-7.03798469582028,3.39661302820565,
-1.74048476183097));
#109973=CARTESIAN_POINT('Ctrl Pts',(-7.038936244,3.395965514,-1.736627927));
#109974=CARTESIAN_POINT('Ctrl Pts',(-7.067561167,3.376486685,-1.620604795));
#109975=CARTESIAN_POINT('Ctrl Pts',(-7.09234675,3.357142857,-1.503701295));
#109976=CARTESIAN_POINT('Ctrl Pts',(-7.149964013,3.31217565,-1.231944122));
#109977=CARTESIAN_POINT('Ctrl Pts',(-7.18661705200001,3.266554913,-0.956574799));
#109978=CARTESIAN_POINT('',(-7.33665862544624,3.39596551354713,-1.55674025405169));
#109979=CARTESIAN_POINT('Ctrl Pts',(-7.43377568496655,3.30628897830885,
-0.994474267950553));
#109980=CARTESIAN_POINT('Ctrl Pts',(-7.4194467856062,3.32334891375399,-1.1015839503658));
#109981=CARTESIAN_POINT('Ctrl Pts',(-7.40283010245738,3.34030767936774,
-1.20817308388293));
#109982=CARTESIAN_POINT('Ctrl Pts',(-7.38397881522136,3.3571428567508,-1.31409925646954));
#109983=CARTESIAN_POINT('Ctrl Pts',(-7.36956534156352,3.3700148365407,-1.39508916791251));
#109984=CARTESIAN_POINT('Ctrl Pts',(-7.35379229118658,3.3829590448342,-1.4759921258145));
#109985=CARTESIAN_POINT('Ctrl Pts',(-7.33665862420373,3.39596551520488,
-1.55674025660656));
#109986=CARTESIAN_POINT('',(-7.18779743318909,3.3959655126796,-1.64668409590467));
#109987=CARTESIAN_POINT('Origin',(-8.54351311918577E-14,3.48737837500022,
1.29291109068896E-14));
#109988=CARTESIAN_POINT('',(-7.4327850829995,3.4862983196318,-1.00185123922132));
#109989=CARTESIAN_POINT('Origin',(0.18046278988964,3.62489369570797,0.0466602352497604));
#109990=CARTESIAN_POINT('Origin',(0.190975911410668,3.48214202383925,0.0264075856926274));
#109991=CARTESIAN_POINT('Ctrl Pts',(-6.956355169,3.266573167,-2.8034127));
#109992=CARTESIAN_POINT('Ctrl Pts',(-7.108451961,3.330825242,-2.426001516));
#109993=CARTESIAN_POINT('Ctrl Pts',(-7.218823922,3.395965514,-2.03435031));
#109994=CARTESIAN_POINT('Ctrl Pts',(-6.80973392700001,3.266573167,-2.487975852));
#109995=CARTESIAN_POINT('Ctrl Pts',(-6.94471696,3.330825242,-2.118519479));
#109996=CARTESIAN_POINT('Ctrl Pts',(-7.03893624400001,3.395965514,-1.736627927));
#109997=CARTESIAN_POINT('',(-7.21882391984119,3.39596551397696,-2.03435031727704));
#109998=CARTESIAN_POINT('',(-7.12888008104419,3.39596551522583,-1.88548912589476));
#109999=CARTESIAN_POINT('',(-7.04619557022418,3.3062889773588,-2.56926604054269));
#110000=CARTESIAN_POINT('Origin',(0.185853545006802,3.48210500655179,0.0380208618339362));
#110001=CARTESIAN_POINT('Ctrl Pts',(-6.81133485030236,3.26733592504445,
-2.48358965276559));
#110002=CARTESIAN_POINT('Ctrl Pts',(-6.85046060920791,3.27415053069601,
-2.49774253882626));
#110003=CARTESIAN_POINT('Ctrl Pts',(-6.88961633227399,3.28079893118911,
-2.51197024378488));
#110004=CARTESIAN_POINT('Ctrl Pts',(-6.96788858726607,3.29377261876151,
-2.54052736533596));
#110005=CARTESIAN_POINT('Ctrl Pts',(-7.00705165692539,3.3001056149326,-2.55487376898962));
#110006=CARTESIAN_POINT('Ctrl Pts',(-7.04619557146458,3.30628897721914,
-2.56926603699822));
#110007=CARTESIAN_POINT('Ctrl Pts',(-6.82708405989074,3.39726054241129,
-3.1049944917374));
#110008=CARTESIAN_POINT('Ctrl Pts',(-6.82878127394537,3.39661302820565,
-3.1012518768687));
#110009=CARTESIAN_POINT('Ctrl Pts',(-6.830478488,3.395965514,-3.097509262));
#110010=CARTESIAN_POINT('Ctrl Pts',(-6.881534885,3.376486685,-2.984922149));
#110011=CARTESIAN_POINT('Ctrl Pts',(-6.928852998,3.357142857,-2.870713524));
#110012=CARTESIAN_POINT('Ctrl Pts',(-7.038850015,3.31217565,-2.605220935));
#110013=CARTESIAN_POINT('Ctrl Pts',(-7.128208603,3.266554913,-2.332089646));
#110014=CARTESIAN_POINT('Ctrl Pts',(-6.49752934201089,3.39726054241129,
-3.21631397286633));
#110015=CARTESIAN_POINT('Ctrl Pts',(-6.49928774900545,3.39661302820565,
-3.21275186343316));
#110016=CARTESIAN_POINT('Ctrl Pts',(-6.501046156,3.395965514,-3.209189754));
#110017=CARTESIAN_POINT('Ctrl Pts',(-6.553943388,3.376486685,-3.102032691));
#110018=CARTESIAN_POINT('Ctrl Pts',(-6.603280295,3.357142857,-2.993190497));
#110019=CARTESIAN_POINT('Ctrl Pts',(-6.71797025700001,3.31217565,-2.740172865));
#110020=CARTESIAN_POINT('Ctrl Pts',(-6.812962634,3.266554913,-2.479120843));
#110021=CARTESIAN_POINT('',(-6.83047848634386,3.39596551354713,-3.09750926682452));
#110022=CARTESIAN_POINT('Ctrl Pts',(-7.04619556909987,3.30628897830889,
-2.56926604348342));
#110023=CARTESIAN_POINT('Ctrl Pts',(-7.0091762559016,3.32334891375402,-2.67079127129904));
#110024=CARTESIAN_POINT('Ctrl Pts',(-6.97003454879645,3.34030767936774,
-2.77131631447829));
#110025=CARTESIAN_POINT('Ctrl Pts',(-6.92885299822154,3.35714285674388,
-2.87071352264016));
#110026=CARTESIAN_POINT('Ctrl Pts',(-6.89736606607387,3.37001483652846,
-2.94671146444352));
#110027=CARTESIAN_POINT('Ctrl Pts',(-6.86457003692198,3.38295904483433,
-3.02233221654559));
#110028=CARTESIAN_POINT('Ctrl Pts',(-6.83047848461137,3.39596551520491,
-3.09750926904244));
#110029=CARTESIAN_POINT('',(-6.66576231853218,3.39596551267961,-3.15334951533053));
#110030=CARTESIAN_POINT('Origin',(2.94902990916057E-14,3.48737837499956,
5.46437894932694E-14));
#110031=CARTESIAN_POINT('',(-7.04364229628584,3.48629831963653,-2.57625759529346));
#110032=CARTESIAN_POINT('Origin',(0.166213305170159,3.62489367230267,0.0843635729055464));
#110033=CARTESIAN_POINT('Origin',(0.180834155856733,3.48214200407374,0.0668443663325308));
#110034=CARTESIAN_POINT('Ctrl Pts',(-6.191068588,3.266573167,-4.233281202));
#110035=CARTESIAN_POINT('Ctrl Pts',(-6.420741691,3.330825242,-3.897389996));
#110036=CARTESIAN_POINT('Ctrl Pts',(-6.61272664900001,3.395965514,-3.538622086));
#110037=CARTESIAN_POINT('Ctrl Pts',(-6.115684868,3.266573167,-3.893699859));
#110038=CARTESIAN_POINT('Ctrl Pts',(-6.326934271,3.330825242,-3.561898533));
#110039=CARTESIAN_POINT('Ctrl Pts',(-6.501046156,3.395965514,-3.209189754));
#110040=CARTESIAN_POINT('',(-6.6127266453021,3.39596551397696,-3.5386220926291));
#110041=CARTESIAN_POINT('',(-6.55688639900026,3.39596551522583,-3.37390592680144));
#110042=CARTESIAN_POINT('',(-6.32914318155958,3.3062889773532,-4.02392179185992));
#110043=CARTESIAN_POINT('Origin',(0.173334860569169,3.48210500429325,0.0770848768754384));
#110044=CARTESIAN_POINT('Ctrl Pts',(-6.11819126530476,3.2673359249502,-3.88976035761938));
#110045=CARTESIAN_POINT('Ctrl Pts',(-6.15335983356358,3.27415053064474,
-3.91199323889897));
#110046=CARTESIAN_POINT('Ctrl Pts',(-6.18854158161075,3.28079893116152,
-3.93430563116583));
#110047=CARTESIAN_POINT('Ctrl Pts',(-6.25884493789794,3.29377261876225,
-3.9790213243313));
#110048=CARTESIAN_POINT('Ctrl Pts',(-6.29400834408267,3.30010561492991,
-4.00145121935033));
#110049=CARTESIAN_POINT('Ctrl Pts',(-6.32914318354082,3.30628897721165,
-4.02392178863842));
#110050=CARTESIAN_POINT('Ctrl Pts',(-5.99998859553901,3.39726054241129,
-4.50002271153911));
#110051=CARTESIAN_POINT('Ctrl Pts',(-6.00245068126951,3.39661302820565,
-4.49673244776956));
#110052=CARTESIAN_POINT('Ctrl Pts',(-6.004912767,3.395965514,-4.493442184));
#110053=CARTESIAN_POINT('Ctrl Pts',(-6.078978396,3.376486685,-4.394462911));
#110054=CARTESIAN_POINT('Ctrl Pts',(-6.149741715,3.357142857,-4.293096416));
#110055=CARTESIAN_POINT('Ctrl Pts',(-6.314240122,3.31217565,-4.057457004));
#110056=CARTESIAN_POINT('Ctrl Pts',(-6.460224709,3.266554913,-3.809920827));
#110057=CARTESIAN_POINT('Ctrl Pts',(-5.65420828564301,3.39726054241129,
-4.5378950825258));
#110058=CARTESIAN_POINT('Ctrl Pts',(-5.65669133032151,3.39661302820565,
-4.5347942587629));
#110059=CARTESIAN_POINT('Ctrl Pts',(-5.659174375,3.395965514,-4.53169343500001));
#110060=CARTESIAN_POINT('Ctrl Pts',(-5.733870501,3.376486685,-4.438412986));
#110061=CARTESIAN_POINT('Ctrl Pts',(-5.805451792,3.357142857,-4.342721438));
#110062=CARTESIAN_POINT('Ctrl Pts',(-5.971851679,3.31217565,-4.12027417));
#110063=CARTESIAN_POINT('Ctrl Pts',(-6.120741654,3.266554913,-3.885745952));
#110064=CARTESIAN_POINT('',(-6.00491276436094,3.39596551354713,-4.49344218835395));
#110065=CARTESIAN_POINT('Ctrl Pts',(-6.32914317981192,3.30628897830886,
-4.02392179450353));
#110066=CARTESIAN_POINT('Ctrl Pts',(-6.2711644346662,3.32334891375399,-4.11511536091147));
#110067=CARTESIAN_POINT('Ctrl Pts',(-6.21132792606103,3.3403076793678,-4.20487587433852));
#110068=CARTESIAN_POINT('Ctrl Pts',(-6.1497417158695,3.35714285676231,-4.29309641475446));
#110069=CARTESIAN_POINT('Ctrl Pts',(-6.10265362077076,3.37001483656105,
-4.3605488071224));
#110070=CARTESIAN_POINT('Ctrl Pts',(-6.05436811763914,3.38295904483433,
-4.42735141118742));
#110071=CARTESIAN_POINT('Ctrl Pts',(-6.00491276217618,3.39596551520488,
-4.49344219014927));
#110072=CARTESIAN_POINT('',(-5.8320435660374,3.39596551267961,-4.51256781591366));
#110073=CARTESIAN_POINT('Origin',(-9.02489888376934E-13,3.487378375,-6.71554825637521E-13));
#110074=CARTESIAN_POINT('',(-6.32514662437651,3.48629831963453,-4.03020100929146));
#110075=CARTESIAN_POINT('Origin',(0.144191659664066,3.62489375334973,0.118122165331142));
#110076=CARTESIAN_POINT('Origin',(0.162236844850232,3.48214202030952,0.10415561729928));
#110077=CARTESIAN_POINT('Ctrl Pts',(-5.13629452100001,3.266573167,-5.46520618000001));
#110078=CARTESIAN_POINT('Ctrl Pts',(-5.432804675,3.330825242,-5.186540851));
#110079=CARTESIAN_POINT('Ctrl Pts',(-5.697425627,3.395965514,-4.877431827));
#110080=CARTESIAN_POINT('Ctrl Pts',(-5.135673182,3.266573167,-5.117358788));
#110081=CARTESIAN_POINT('Ctrl Pts',(-5.413311169,3.330825242,-4.83872717));
#110082=CARTESIAN_POINT('Ctrl Pts',(-5.659174375,3.395965514,-4.531693435));
#110083=CARTESIAN_POINT('',(-5.69742562195829,3.39596551397696,-4.87743183267498));
#110084=CARTESIAN_POINT('',(-5.67829999611997,3.39596551522583,-4.70456263689008));
#110085=CARTESIAN_POINT('',(-5.31614709217801,3.30628897737121,-5.29042343252636));
#110086=CARTESIAN_POINT('Origin',(0.152711476053585,3.48210502425196,0.112544600522418));
#110087=CARTESIAN_POINT('Ctrl Pts',(-5.13896785745178,3.26733592494318,
-5.11405019183392));
#110088=CARTESIAN_POINT('Ctrl Pts',(-5.16853479175912,3.27415053063135,
-5.1433234832491));
#110089=CARTESIAN_POINT('Ctrl Pts',(-5.19809750522736,3.28079893115591,
-5.1726772600891));
#110090=CARTESIAN_POINT('Ctrl Pts',(-5.25714465569619,3.29377261877121,
-5.23146066871708));
#110091=CARTESIAN_POINT('Ctrl Pts',(-5.28666419646867,3.30010561494333,
-5.26092525818259));
#110092=CARTESIAN_POINT('Ctrl Pts',(-5.31614709470979,3.30628897724565,
-5.29042343002221));
#110093=CARTESIAN_POINT('Ctrl Pts',(-4.89234033307211,3.3972605424113,-5.68463487117339));
#110094=CARTESIAN_POINT('Ctrl Pts',(-4.89545216603606,3.39661302820565,
-5.6819508075867));
#110095=CARTESIAN_POINT('Ctrl Pts',(-4.898563999,3.395965514,-5.679266744));
#110096=CARTESIAN_POINT('Ctrl Pts',(-4.992175632,3.376486685,-5.598523472));
#110097=CARTESIAN_POINT('Ctrl Pts',(-5.083075345,3.357142857,-5.514738891));
#110098=CARTESIAN_POINT('Ctrl Pts',(-5.29438337900001,3.31217565,-5.319970893));
#110099=CARTESIAN_POINT('Ctrl Pts',(-5.490167888,3.266554913,-5.109604345));
#110100=CARTESIAN_POINT('Ctrl Pts',(-4.54650273517165,3.3972605424113,-5.64728926211416));
#110101=CARTESIAN_POINT('Ctrl Pts',(-4.54959431308582,3.39661302820565,
-5.64479471505708));
#110102=CARTESIAN_POINT('Ctrl Pts',(-4.552685891,3.395965514,-5.64230016800001));
#110103=CARTESIAN_POINT('Ctrl Pts',(-4.645688202,3.376486685,-5.567258022));
#110104=CARTESIAN_POINT('Ctrl Pts',(-4.736166816,3.357142857,-5.489191552));
#110105=CARTESIAN_POINT('Ctrl Pts',(-4.946495953,3.31217565,-5.30771603400001));
#110106=CARTESIAN_POINT('Ctrl Pts',(-5.142321598,3.266554913,-5.110677899));
#110107=CARTESIAN_POINT('',(-4.89856399292942,3.39596551397715,-5.67926674902997));
#110108=CARTESIAN_POINT('Ctrl Pts',(-5.31614709017629,3.30628897830889,
-5.29042343480269));
#110109=CARTESIAN_POINT('Ctrl Pts',(-5.23991993481122,3.32334891375402,
-5.3670212298921));
#110110=CARTESIAN_POINT('Ctrl Pts',(-5.16218651342885,3.340307679368,-5.44182011168093));
#110111=CARTESIAN_POINT('Ctrl Pts',(-5.08307534592634,3.35714285679733,
-5.51473889012026));
#110112=CARTESIAN_POINT('Ctrl Pts',(-5.02258787301562,3.370014836623,-5.57049173472499));
#110113=CARTESIAN_POINT('Ctrl Pts',(-4.96107067312144,3.38295904483426,
-5.62535257504625));
#110114=CARTESIAN_POINT('Ctrl Pts',(-4.89856399296705,3.39596551520491,
-5.67926674896868));
#110115=CARTESIAN_POINT('',(-4.72562493877464,3.3959655126796,-5.66078346119694));
#110116=CARTESIAN_POINT('Origin',(-1.6826817716975E-13,3.48737837500044,
-2.05131051034257E-13));
#110117=CARTESIAN_POINT('',(-5.31089412610486,3.48629831962543,-5.29569670366415));
#110118=CARTESIAN_POINT('Origin',(0.115427610360891,3.62489372344857,0.146357328935068));
#110119=CARTESIAN_POINT('Origin',(0.1360537206532,3.4821420105048,0.13659692597751));
#110120=CARTESIAN_POINT('Ctrl Pts',(-3.841353031,3.266573167,-6.441584191));
#110121=CARTESIAN_POINT('Ctrl Pts',(-4.190835751,3.330825242,-6.233174821));
#110122=CARTESIAN_POINT('Ctrl Pts',(-4.515719315,3.395965514,-5.988178277));
#110123=CARTESIAN_POINT('Ctrl Pts',(-3.915523125,3.266573167,-6.101735708));
#110124=CARTESIAN_POINT('Ctrl Pts',(-4.246567652,3.330825242,-5.889302302));
#110125=CARTESIAN_POINT('Ctrl Pts',(-4.552685891,3.395965514,-5.642300168));
#110126=CARTESIAN_POINT('',(-4.51571930876571,3.39596551397696,-5.98817828133813));
#110127=CARTESIAN_POINT('',(-4.53420259696787,3.39596551522583,-5.81523922720331));
#110128=CARTESIAN_POINT('',(-4.05457387323724,3.30628897737472,-6.30955075328127));
#110129=CARTESIAN_POINT('Origin',(0.124947428463476,3.48210504497436,0.142741857003189));
#110130=CARTESIAN_POINT('Ctrl Pts',(-3.91945202346168,3.26733592500564,
-6.09921272262872));
#110131=CARTESIAN_POINT('Ctrl Pts',(-3.9420348069806,3.27415053068454,-6.13415763776697));
#110132=CARTESIAN_POINT('Ctrl Pts',(-3.96459616635793,3.28079893119255,
-6.16918024915714));
#110133=CARTESIAN_POINT('Ctrl Pts',(-4.00962613217553,3.29377261878804,
-6.23928272632204));
#110134=CARTESIAN_POINT('Ctrl Pts',(-4.03212150681201,3.30010561495652,
-6.27440427875316));
#110135=CARTESIAN_POINT('Ctrl Pts',(-4.05457387631763,3.306288977244,-6.30955075129799));
#110136=CARTESIAN_POINT('Ctrl Pts',(-3.5559316742459,3.3972605424113,-6.60343982105814));
#110137=CARTESIAN_POINT('Ctrl Pts',(-3.55954774862295,3.39661302820565,
-6.60148746152907));
#110138=CARTESIAN_POINT('Ctrl Pts',(-3.563163823,3.395965514,-6.599535102));
#110139=CARTESIAN_POINT('Ctrl Pts',(-3.671944285,3.376486685,-6.540803298));
#110140=CARTESIAN_POINT('Ctrl Pts',(-3.778730021,3.357142857,-6.478518305));
#110141=CARTESIAN_POINT('Ctrl Pts',(-4.026967153,3.31217565,-6.333728855));
#110142=CARTESIAN_POINT('Ctrl Pts',(-4.263396918,3.266554913,-6.170368443));
#110143=CARTESIAN_POINT('Ctrl Pts',(-3.22620776921482,3.3972605424113,-6.49262247109658));
#110144=CARTESIAN_POINT('Ctrl Pts',(-3.22976332160741,3.39661302820565,
-6.4908508430483));
#110145=CARTESIAN_POINT('Ctrl Pts',(-3.233318874,3.395965514,-6.489079215));
#110146=CARTESIAN_POINT('Ctrl Pts',(-3.340278685,3.376486685,-6.435784261));
#110147=CARTESIAN_POINT('Ctrl Pts',(-3.445423944,3.357142857,-6.378993169));
#110148=CARTESIAN_POINT('Ctrl Pts',(-3.689847575,3.31217565,-6.246974995));
#110149=CARTESIAN_POINT('Ctrl Pts',(-3.923452299,3.266554913,-6.096640227));
#110150=CARTESIAN_POINT('',(-3.56316381609284,3.39596551397714,-6.59953510579764));
#110151=CARTESIAN_POINT('Ctrl Pts',(-4.05457387064305,3.30628897830886,
-6.30955075494452));
#110152=CARTESIAN_POINT('Ctrl Pts',(-3.96366260214418,3.32334891375399,
-6.36797115091668));
#110153=CARTESIAN_POINT('Ctrl Pts',(-3.87166699641581,3.34030767936791,
-6.42431088867839));
#110154=CARTESIAN_POINT('Ctrl Pts',(-3.77873002219183,3.3571428567841,-6.47851830430484));
#110155=CARTESIAN_POINT('Ctrl Pts',(-3.70767149963447,3.37001483659959,
-6.51996465985505));
#110156=CARTESIAN_POINT('Ctrl Pts',(-3.63579907860465,3.38295904483422,
-6.56031850441926));
#110157=CARTESIAN_POINT('Ctrl Pts',(-3.56316381603993,3.39596551520488,
-6.59953510555543));
#110158=CARTESIAN_POINT('',(-3.39824134130304,3.39596551267961,-6.54430716223715));
#110159=CARTESIAN_POINT('Origin',(6.85215773010839E-13,3.48737837500089,
1.19869392189997E-12));
#110160=CARTESIAN_POINT('',(-4.04831012106115,3.48629831963159,-6.31357150582533));
#110161=CARTESIAN_POINT('Origin',(0.0812663912945105,3.62489370994011,0.167748984259999));
#110162=CARTESIAN_POINT('Origin',(0.10350851005091,3.48214198135497,0.162650836534864));
#110163=CARTESIAN_POINT('Ctrl Pts',(-2.366794143,3.266573167,-7.116760884));
#110164=CARTESIAN_POINT('Ctrl Pts',(-2.752908005,3.330825242,-6.988352464));
#110165=CARTESIAN_POINT('Ctrl Pts',(-3.122862986,3.395965514,-6.81892416500001));
#110166=CARTESIAN_POINT('Ctrl Pts',(-2.512287559,3.266573167,-6.800802248));
#110167=CARTESIAN_POINT('Ctrl Pts',(-2.881259352,3.330825242,-6.664500205));
#110168=CARTESIAN_POINT('Ctrl Pts',(-3.233318874,3.395965514,-6.489079215));
#110169=CARTESIAN_POINT('',(-3.12286297908662,3.39596551397696,-6.81892416813198));
#110170=CARTESIAN_POINT('',(-3.17809092309782,3.39596551522583,-6.65400169329663));
#110171=CARTESIAN_POINT('',(-2.60341328610598,3.30628897734022,-7.03365049340117));
#110172=CARTESIAN_POINT('Origin',(0.0913408454317249,3.48210503010585,0.166264369373738));
#110173=CARTESIAN_POINT('Ctrl Pts',(-2.5166669693812,3.26733592496633,-6.79918284502861));
#110174=CARTESIAN_POINT('Ctrl Pts',(-2.53120965623776,3.27415053064923,
-6.83816539843916));
#110175=CARTESIAN_POINT('Ctrl Pts',(-2.54571471740442,3.2807989311671,-6.87721922612769));
#110176=CARTESIAN_POINT('Ctrl Pts',(-2.57462194719662,3.29377261875497,
-6.95536285802594));
#110177=CARTESIAN_POINT('Ctrl Pts',(-2.58904129683186,3.3001056149235,-6.99449912875471));
#110178=CARTESIAN_POINT('Ctrl Pts',(-2.603413289663,3.30628897720744,-7.03365049210116));
#110179=CARTESIAN_POINT('Ctrl Pts',(-2.05325160269057,3.39726054241129,
-7.21347526574445));
#110180=CARTESIAN_POINT('Ctrl Pts',(-2.05720283484529,3.39661302820565,
-7.21234590037222));
#110181=CARTESIAN_POINT('Ctrl Pts',(-2.061154067,3.395965514,-7.21121653500001));
#110182=CARTESIAN_POINT('Ctrl Pts',(-2.180016904,3.376486685,-7.177242431));
#110183=CARTESIAN_POINT('Ctrl Pts',(-2.297695481,3.357142857,-7.139369403));
#110184=CARTESIAN_POINT('Ctrl Pts',(-2.571254418,3.31217565,-7.05132869600001));
#110185=CARTESIAN_POINT('Ctrl Pts',(-2.837274247,3.266554913,-6.94261297));
#110186=CARTESIAN_POINT('Ctrl Pts',(-1.75505891355549,3.39726054241129,
-7.03436787041624));
#110187=CARTESIAN_POINT('Ctrl Pts',(-1.75891218677775,3.39661302820565,
-7.03340200070812));
#110188=CARTESIAN_POINT('Ctrl Pts',(-1.76276546,3.395965514,-7.032436131));
#110189=CARTESIAN_POINT('Ctrl Pts',(-1.87868145,3.376486685,-7.003380381));
#110190=CARTESIAN_POINT('Ctrl Pts',(-1.993576877,3.357142857,-6.970520155));
#110191=CARTESIAN_POINT('Ctrl Pts',(-2.260666024,3.31217565,-6.894132348));
#110192=CARTESIAN_POINT('Ctrl Pts',(-2.521126731,3.266554913,-6.797530434));
#110193=CARTESIAN_POINT('',(-2.0611540593741,3.39596551397715,-7.21121653699979));
#110194=CARTESIAN_POINT('Ctrl Pts',(-2.60341328311995,3.30628897830887,
-7.03365049452299));
#110195=CARTESIAN_POINT('Ctrl Pts',(-2.50206881124079,3.32334891375401,
-7.07116181866411));
#110196=CARTESIAN_POINT('Ctrl Pts',(-2.40011263349957,3.34030767936808,
-7.10640802868447));
#110197=CARTESIAN_POINT('Ctrl Pts',(-2.29769548211474,3.35714285681676,
-7.13936940264124));
#110198=CARTESIAN_POINT('Ctrl Pts',(-2.21938852700798,3.37001483665733,
-7.16457128373588));
#110199=CARTESIAN_POINT('Ctrl Pts',(-2.14052155993246,3.38295904483429,
-7.18853123205442));
#110200=CARTESIAN_POINT('Ctrl Pts',(-2.06115405943867,3.39596551520489,
-7.21121653697635));
#110201=CARTESIAN_POINT('',(-1.91195975566792,3.39596551267961,-7.12182633510264));
#110202=CARTESIAN_POINT('Origin',(-4.25657772917809E-13,3.48737837499945,
-1.36305897124878E-12));
#110203=CARTESIAN_POINT('',(-2.59643163431783,3.48629831961912,-7.03623072141385));
#110204=CARTESIAN_POINT('Origin',(0.0433053581522996,3.62489369331728,0.181296946656153));
#110205=CARTESIAN_POINT('Origin',(0.0661234053702608,3.48214199777855,0.181099351764563));
#110206=CARTESIAN_POINT('Ctrl Pts',(-0.781566591,3.266573167,-7.459165749));
#110207=CARTESIAN_POINT('Ctrl Pts',(-1.18625734,3.330825242,-7.416762512));
#110208=CARTESIAN_POINT('Ctrl Pts',(-1.583985056,3.395965514,-7.330824738));
#110209=CARTESIAN_POINT('Ctrl Pts',(-0.991580219,3.266573167,-7.181870833));
#110210=CARTESIAN_POINT('Ctrl Pts',(-1.381226566,3.330825242,-7.128073485));
#110211=CARTESIAN_POINT('Ctrl Pts',(-1.76276546,3.395965514,-7.032436131));
#110212=CARTESIAN_POINT('',(-1.58398504857742,3.39596551397696,-7.33082473958187));
#110213=CARTESIAN_POINT('',(-1.67337525055052,3.39596551522583,-7.18163043623579));
#110214=CARTESIAN_POINT('',(-1.03051998746748,3.30628897732933,-7.42886455333183));
#110215=CARTESIAN_POINT('Origin',(0.0534634752718685,3.4821050195673,0.182013100375262));
#110216=CARTESIAN_POINT('Ctrl Pts',(-0.996205364753573,3.26733592494251,
-7.18123073465414));
#110217=CARTESIAN_POINT('Ctrl Pts',(-1.00202795503195,3.27415053062055,
-7.22242814541734));
#110218=CARTESIAN_POINT('Ctrl Pts',(-1.00779847745467,3.2807989311329,-7.26368707561806));
#110219=CARTESIAN_POINT('Ctrl Pts',(-1.01923135518573,3.29377267967181,
-7.34621834033066));
#110220=CARTESIAN_POINT('Ctrl Pts',(-1.02490050608604,3.30010573880957,
-7.38753980110302));
#110221=CARTESIAN_POINT('Ctrl Pts',(-1.03051999137626,3.30628897719394,
-7.42886455280585));
#110222=CARTESIAN_POINT('Ctrl Pts',(-0.454563767573316,3.3972605424113,
-7.48621662364792));
#110223=CARTESIAN_POINT('Ctrl Pts',(-0.458665402286658,3.39661302820565,
-7.48596306032396));
#110224=CARTESIAN_POINT('Ctrl Pts',(-0.462767037,3.395965514,-7.48570949700001));
#110225=CARTESIAN_POINT('Ctrl Pts',(-0.586154355,3.376486685,-7.478081685));
#110226=CARTESIAN_POINT('Ctrl Pts',(-0.709223254,3.357142857,-7.466391523));
#110227=CARTESIAN_POINT('Ctrl Pts',(-0.995312685000001,3.31217565,-7.439216243));
#110228=CARTESIAN_POINT('Ctrl Pts',(-1.278483785,3.266554913,-7.39022863000001));
#110229=CARTESIAN_POINT('Ctrl Pts',(-0.201845453451928,3.3972605424113,
-7.24719404571963));
#110230=CARTESIAN_POINT('Ctrl Pts',(-0.205816272725964,3.39661302820565,
-7.24707909735982));
#110231=CARTESIAN_POINT('Ctrl Pts',(-0.209787092,3.395965514,-7.246964149));
#110232=CARTESIAN_POINT('Ctrl Pts',(-0.329239158,3.376486685,-7.243506218));
#110233=CARTESIAN_POINT('Ctrl Pts',(-0.448512371,3.357142857,-7.236113367));
#110234=CARTESIAN_POINT('Ctrl Pts',(-0.725778243,3.31217565,-7.21892773600001));
#110235=CARTESIAN_POINT('Ctrl Pts',(-1.000916079,3.266554913,-7.180575673));
#110236=CARTESIAN_POINT('',(-0.462767033893976,3.39596551355056,-7.48570949824636));
#110237=CARTESIAN_POINT('Ctrl Pts',(-1.03051998418126,3.30628897830881,
-7.42886455361434));
#110238=CARTESIAN_POINT('Ctrl Pts',(-0.923481063958462,3.32334891375394,
-7.44371281826105));
#110239=CARTESIAN_POINT('Ctrl Pts',(-0.816331671680277,3.3403076793679,
-7.45621742731177));
#110240=CARTESIAN_POINT('Ctrl Pts',(-0.709223255344492,3.35714285678867,
-7.46639152287229));
#110241=CARTESIAN_POINT('Ctrl Pts',(-0.627329415421036,3.37001483635925,
-7.47417051711955));
#110242=CARTESIAN_POINT('Ctrl Pts',(-0.545155634773015,3.38295904433458,
-7.48061622843096));
#110243=CARTESIAN_POINT('Ctrl Pts',(-0.462767033959746,3.39596551445183,
-7.48570949700878));
#110244=CARTESIAN_POINT('',(-0.336277056399031,3.39596551267961,-7.36633682336981));
#110245=CARTESIAN_POINT('Origin',(1.66262403150652E-13,3.48737837499922,
1.2862974574368E-12));
#110246=CARTESIAN_POINT('',(-1.02314689010349,3.48629831963628,-7.42988360835676));
#110247=CARTESIAN_POINT('Origin',(0.00331945825586336,3.62489370198345,
0.186367959974886));
#110248=CARTESIAN_POINT('Origin',(0.025646474010152,3.48214201755016,0.191079869937566));
#110249=CARTESIAN_POINT('Ctrl Pts',(0.840206145999999,3.266573167,-7.452788313));
#110250=CARTESIAN_POINT('Ctrl Pts',(0.4358614,3.330825242,-7.498372989));
#110251=CARTESIAN_POINT('Ctrl Pts',(0.028958256,3.395965514,-7.499944094));
#110252=CARTESIAN_POINT('Ctrl Pts',(0.57549231,3.266573167,-7.227123121));
#110253=CARTESIAN_POINT('Ctrl Pts',(0.183390838,3.330825242,-7.258345971));
#110254=CARTESIAN_POINT('Ctrl Pts',(-0.209787092,3.395965514,-7.246964149));
#110255=CARTESIAN_POINT('',(0.0289582635899049,3.39596551397696,-7.49994409402047));
#110256=CARTESIAN_POINT('',(-0.0904144103515404,3.39596551522583,-7.37345412159378));
#110257=CARTESIAN_POINT('',(0.590559280491092,3.30628897736223,-7.47671316417767));
#110258=CARTESIAN_POINT('Origin',(0.0130861047795402,3.48210501151378,0.189250681594911));
#110259=CARTESIAN_POINT('Ctrl Pts',(0.570837695264029,3.26733592494405,
-7.22749225733758));
#110260=CARTESIAN_POINT('Ctrl Pts',(0.574007459370702,3.2741505306344,-7.26897818017597));
#110261=CARTESIAN_POINT('Ctrl Pts',(0.577241298962552,3.28079893115661,
-7.3105129911894));
#110262=CARTESIAN_POINT('Ctrl Pts',(0.583817467099475,3.29377261875627,
-7.39357206124346));
#110263=CARTESIAN_POINT('Ctrl Pts',(0.587163713369376,3.30010561493485,
-7.43514570629488));
#110264=CARTESIAN_POINT('Ctrl Pts',(0.590559276754091,3.30628897722236,
-7.47671316441908));
#110265=CARTESIAN_POINT('Ctrl Pts',(1.16537896377315,3.3972605424113,-7.40891081180722));
#110266=CARTESIAN_POINT('Ctrl Pts',(1.16131871438658,3.39661302820565,-7.40954490690361));
#110267=CARTESIAN_POINT('Ctrl Pts',(1.157258465,3.395965514,-7.410179002));
#110268=CARTESIAN_POINT('Ctrl Pts',(1.03511612,3.376486685,-7.429254151));
#110269=CARTESIAN_POINT('Ctrl Pts',(0.912411464,3.357142857,-7.444293474));
#110270=CARTESIAN_POINT('Ctrl Pts',(0.627168763,3.31217565,-7.479254308));
#110271=CARTESIAN_POINT('Ctrl Pts',(0.340087157,3.266554913,-7.492285414));
#110272=CARTESIAN_POINT('Ctrl Pts',(1.36080607551578,3.3972605424113,-7.12114948230861));
#110273=CARTESIAN_POINT('Ctrl Pts',(1.35690338125789,3.39661302820565,-7.12189083015431));
#110274=CARTESIAN_POINT('Ctrl Pts',(1.353000687,3.395965514,-7.12263217800001));
#110275=CARTESIAN_POINT('Ctrl Pts',(1.23559799,3.376486685,-7.144933755));
#110276=CARTESIAN_POINT('Ctrl Pts',(1.117524075,3.357142857,-7.163353959));
#110277=CARTESIAN_POINT('Ctrl Pts',(0.843046122,3.31217565,-7.206174085));
#110278=CARTESIAN_POINT('Ctrl Pts',(0.566096296,3.266554913,-7.227865175));
#110279=CARTESIAN_POINT('',(1.1572584727817,3.39596551397715,-7.41017900074624));
#110280=CARTESIAN_POINT('Ctrl Pts',(0.590559283615143,3.30628897830888,
-7.47671316387715));
#110281=CARTESIAN_POINT('Ctrl Pts',(0.69828763140258,3.32334891375402,-7.46820408056629));
#110282=CARTESIAN_POINT('Ctrl Pts',(0.805620051771964,3.340307679368,-7.45738238676489));
#110283=CARTESIAN_POINT('Ctrl Pts',(0.912411462719141,3.35714285679808,
-7.44429347415699));
#110284=CARTESIAN_POINT('Ctrl Pts',(0.994062925744556,3.37001483662431,
-7.43428584474713));
#110285=CARTESIAN_POINT('Ctrl Pts',(1.07570116794024,3.3829590448342,-7.42291592453298));
#110286=CARTESIAN_POINT('Ctrl Pts',(1.15725847269244,3.39596551520491,-7.41017900061876));
#110287=CARTESIAN_POINT('',(1.25512958399112,3.3959655126796,-7.26640558861969));
#110288=CARTESIAN_POINT('Origin',(-1.14874608306628E-13,3.48737837499989,
1.91990520703733E-12));
#110289=CARTESIAN_POINT('',(0.597979065930149,3.48629831963031,-7.47612339603309));
#110290=CARTESIAN_POINT('Origin',(-0.0368217379796355,3.62489368320795,
0.18272430210277));
#110291=CARTESIAN_POINT('Origin',(-0.0160296329366373,3.48214204465331,
0.192125554458964));
#110292=CARTESIAN_POINT('Ctrl Pts',(2.422691778,3.266573167,-7.097926778));
#110293=CARTESIAN_POINT('Ctrl Pts',(2.037599744,3.330825242,-7.229367878));
#110294=CARTESIAN_POINT('Ctrl Pts',(1.640547511,3.395965514,-7.3183744));
#110295=CARTESIAN_POINT('Ctrl Pts',(2.115655458,3.266573167,-6.934443163));
#110296=CARTESIAN_POINT('Ctrl Pts',(1.739433091,3.330825242,-7.049226266));
#110297=CARTESIAN_POINT('Ctrl Pts',(1.353000687,3.395965514,-7.122632178));
#110298=CARTESIAN_POINT('',(1.64054751841347,3.39596551397696,-7.31837439837307));
#110299=CARTESIAN_POINT('',(1.4967741064898,3.39596551522583,-7.2205032874474));
#110300=CARTESIAN_POINT('',(2.18402465294681,3.30628897734932,-7.17495897641274));
#110301=CARTESIAN_POINT('Origin',(-0.0279031602769891,3.48210505020889,
0.18763928548272));
#110302=CARTESIAN_POINT('Ctrl Pts',(2.11118901980916,3.26733592496051,-6.93580427423557));
#110303=CARTESIAN_POINT('Ctrl Pts',(2.12320292378257,3.27415053065322,-6.97563887355951));
#110304=CARTESIAN_POINT('Ctrl Pts',(2.13528991457471,3.28079893116479,-7.01550744370506));
#110305=CARTESIAN_POINT('Ctrl Pts',(2.15956758027455,3.29377261876942,-7.09521095702699));
#110306=CARTESIAN_POINT('Ctrl Pts',(2.17177269778662,3.30010561493228,-7.13509328920972));
#110307=CARTESIAN_POINT('Ctrl Pts',(2.18402464941342,3.30628897722014,-7.1749589775187));
#110308=CARTESIAN_POINT('Ctrl Pts',(2.73082986964228,3.39726054241129,-6.98517256627893));
#110309=CARTESIAN_POINT('Ctrl Pts',(2.72700085832114,3.39661302820565,-6.98666467013947));
#110310=CARTESIAN_POINT('Ctrl Pts',(2.723171847,3.395965514,-6.988156774));
#110311=CARTESIAN_POINT('Ctrl Pts',(2.607985715,3.376486685,-7.03304294900001));
#110312=CARTESIAN_POINT('Ctrl Pts',(2.491382836,3.357142857,-7.074108535));
#110313=CARTESIAN_POINT('Ctrl Pts',(2.220324497,3.31217565,-7.169570753));
#110314=CARTESIAN_POINT('Ctrl Pts',(1.942756002,3.266554913,-7.244011259));
#110315=CARTESIAN_POINT('Ctrl Pts',(2.85982782510034,3.39726054241129,-6.66212788310328));
#110316=CARTESIAN_POINT('Ctrl Pts',(2.85617574155017,3.39661302820565,-6.66369086255164));
#110317=CARTESIAN_POINT('Ctrl Pts',(2.852523658,3.395965514,-6.665253842));
#110318=CARTESIAN_POINT('Ctrl Pts',(2.742659951,3.376486685,-6.71227213));
#110319=CARTESIAN_POINT('Ctrl Pts',(2.631306337,3.357142857,-6.755644082));
#110320=CARTESIAN_POINT('Ctrl Pts',(2.372450588,3.31217565,-6.856467744));
#110321=CARTESIAN_POINT('Ctrl Pts',(2.106638638,3.266554913,-6.937187734));
#110322=CARTESIAN_POINT('',(2.72317185034836,3.39596551355056,-6.9881567738227));
#110323=CARTESIAN_POINT('Ctrl Pts',(2.18402465597099,3.3062889783089,-7.17495897559197));
#110324=CARTESIAN_POINT('Ctrl Pts',(2.287405173422,3.32334891375403,-7.14349041942547));
#110325=CARTESIAN_POINT('Ctrl Pts',(2.3899018770918,3.34030767936787,-7.1098484331051));
#110326=CARTESIAN_POINT('Ctrl Pts',(2.49138283465962,3.35714285677056,-7.07410853538993));
#110327=CARTESIAN_POINT('Ctrl Pts',(2.5689739854683,3.37001483632763,-7.04678222827701));
#110328=CARTESIAN_POINT('Ctrl Pts',(2.64625937286991,3.38295904433555,-7.01812832265671));
#110329=CARTESIAN_POINT('Ctrl Pts',(2.72317184976995,3.39596551445312,-6.98815677273005));
#110330=CARTESIAN_POINT('',(2.78784776000748,3.39596551267962,-6.82670530493414));
#110331=CARTESIAN_POINT('Origin',(-4.47450236584768E-13,3.48737837500022,
1.14795326022765E-12));
#110332=CARTESIAN_POINT('',(2.19114418520372,3.48629831963248,-7.17278796251029));
#110333=CARTESIAN_POINT('Origin',(-0.0752411761832097,3.62489372401122,
0.170536642326012));
#110334=CARTESIAN_POINT('Origin',(-0.0569562512824762,3.48214202558383,
0.18418808260192));
#110335=CARTESIAN_POINT('Ctrl Pts',(3.891895034,3.266573167,-6.411174077));
#110336=CARTESIAN_POINT('Ctrl Pts',(3.54406219,3.330825242,-6.622325561));
#110337=CARTESIAN_POINT('Ctrl Pts',(3.175426589,3.395965514,-6.794605653));
#110338=CARTESIAN_POINT('Ctrl Pts',(3.556892909,3.266573167,-6.31751635));
#110339=CARTESIAN_POINT('Ctrl Pts',(3.214141385,3.330825242,-6.510492576));
#110340=CARTESIAN_POINT('Ctrl Pts',(2.852523658,3.395965514,-6.665253842));
#110341=CARTESIAN_POINT('',(3.17542659581968,3.39596551397696,-6.7946056496667));
#110342=CARTESIAN_POINT('',(3.01397513048093,3.39596551522583,-6.72992974437362));
#110343=CARTESIAN_POINT('',(3.67536745979543,3.30628897733966,-6.53771168204423));
#110344=CARTESIAN_POINT('Origin',(-0.0675876810856374,3.48210503795346,
0.177253988013014));
#110345=CARTESIAN_POINT('Ctrl Pts',(3.55282349146402,3.26733592496364,-6.31980579117285));
#110346=CARTESIAN_POINT('Ctrl Pts',(3.57311977824477,3.27415053065783,-6.35612644571022));
#110347=CARTESIAN_POINT('Ctrl Pts',(3.5934947459802,3.28079893117787,-6.39246456534641));
#110348=CARTESIAN_POINT('Ctrl Pts',(3.63433871271115,3.29377261876238,-6.46508567454925));
#110349=CARTESIAN_POINT('Ctrl Pts',(3.65483200398093,3.30010561492691,-6.5014118406284));
#110350=CARTESIAN_POINT('Ctrl Pts',(3.67536745644001,3.30628897719833,-6.53771168388222));
#110351=CARTESIAN_POINT('Ctrl Pts',(4.16859020585149,3.3972605424113,-6.2348154138769));
#110352=CARTESIAN_POINT('Ctrl Pts',(4.16517147292575,3.39661302820565,-6.23709575743844));
#110353=CARTESIAN_POINT('Ctrl Pts',(4.16175274,3.395965514,-6.239376101));
#110354=CARTESIAN_POINT('Ctrl Pts',(4.058908797,3.376486685,-6.307974476));
#110355=CARTESIAN_POINT('Ctrl Pts',(3.953859916,3.357142857,-6.373146144));
#110356=CARTESIAN_POINT('Ctrl Pts',(3.709660325,3.31217565,-6.52464603900001));
#110357=CARTESIAN_POINT('Ctrl Pts',(3.454583735,3.266554913,-6.657015188));
#110358=CARTESIAN_POINT('Ctrl Pts',(4.2251272029383,3.3972605424113,-5.89159258926902));
#110359=CARTESIAN_POINT('Ctrl Pts',(4.22189649746915,3.39661302820565,-5.89390411713451));
#110360=CARTESIAN_POINT('Ctrl Pts',(4.218665792,3.395965514,-5.896215645));
#110361=CARTESIAN_POINT('Ctrl Pts',(4.12147818,3.376486685,-5.965752121));
#110362=CARTESIAN_POINT('Ctrl Pts',(4.022051639,3.357142857,-6.032047796));
#110363=CARTESIAN_POINT('Ctrl Pts',(3.7909219,3.31217565,-6.186160591));
#110364=CARTESIAN_POINT('Ctrl Pts',(3.548676898,3.266554913,-6.322135104));
#110365=CARTESIAN_POINT('',(4.16175274448907,3.39596551354713,-6.23937609860885));
#110366=CARTESIAN_POINT('Ctrl Pts',(3.67536746257195,3.30628897830886,-6.53771168043497));
#110367=CARTESIAN_POINT('Ctrl Pts',(3.76956619177034,3.32334891375399,-6.48475508644378));
#110368=CARTESIAN_POINT('Ctrl Pts',(3.86243454701094,3.34030767936762,-6.42986586961159));
#110369=CARTESIAN_POINT('Ctrl Pts',(3.95385991457985,3.35714285672509,-6.37314614456213));
#110370=CARTESIAN_POINT('Ctrl Pts',(4.02376268007051,3.37001483649523,-6.32977890632933));
#110371=CARTESIAN_POINT('Ctrl Pts',(4.0930814367508,3.38295904483422,-6.28518083842415));
#110372=CARTESIAN_POINT('Ctrl Pts',(4.16175274640143,3.39596551520488,-6.23937609651593));
#110373=CARTESIAN_POINT('',(4.19020927267297,3.3959655126796,-6.06779586839188));
#110374=CARTESIAN_POINT('Origin',(-3.25260651745651E-14,3.48737837500033,
1.47451495458029E-14));
#110375=CARTESIAN_POINT('',(3.68185383757783,3.48629831961797,-6.53406093588961));
#110376=CARTESIAN_POINT('Origin',(-0.110142518670112,3.62489370752314,0.150375150523643));
#110377=CARTESIAN_POINT('Origin',(-0.095219468594035,3.48214199609701,0.167637657977258));
#110378=CARTESIAN_POINT('Ctrl Pts',(5.179117605,3.266573167,-5.424642001));
#110379=CARTESIAN_POINT('Ctrl Pts',(4.884808226,3.330825242,-5.70563066));
#110380=CARTESIAN_POINT('Ctrl Pts',(4.561826248,3.395965514,-5.953128697));
#110381=CARTESIAN_POINT('Ctrl Pts',(4.831814,3.266573167,-5.405189494));
#110382=CARTESIAN_POINT('Ctrl Pts',(4.538560001,3.330825242,-5.667335489));
#110383=CARTESIAN_POINT('Ctrl Pts',(4.218665792,3.395965514,-5.89621564500001));
#110384=CARTESIAN_POINT('',(4.56182625396996,3.39596551397696,-5.95312869231247));
#110385=CARTESIAN_POINT('',(4.39024602614564,3.39596551522583,-5.92467216644601));
#110386=CARTESIAN_POINT('',(4.99485416922012,3.30628897734424,-5.59476825503998));
#110387=CARTESIAN_POINT('Origin',(-0.104112042527872,3.48210506471219,0.158580729364672));
#110388=CARTESIAN_POINT('Ctrl Pts',(4.82833188523068,3.26733592501069,-5.40830021398496));
#110389=CARTESIAN_POINT('Ctrl Pts',(4.85596152334697,3.2741505306834,-5.43940860997987));
#110390=CARTESIAN_POINT('Ctrl Pts',(4.88367175730801,3.28079893118907,-5.47051714869432));
#110391=CARTESIAN_POINT('Ctrl Pts',(4.93917220669472,3.2937726187639,-5.53266017110701));
#110392=CARTESIAN_POINT('Ctrl Pts',(4.96699542809321,3.30010561492509,-5.56373159971429));
#110393=CARTESIAN_POINT('Ctrl Pts',(4.99485416633788,3.30628897720176,-5.59476825754054));
#110394=CARTESIAN_POINT('Ctrl Pts',(5.41143189778815,3.3972605424113,-5.19292522215096));
#110395=CARTESIAN_POINT('Ctrl Pts',(5.40858329939408,3.39661302820565,-5.19588717907548));
#110396=CARTESIAN_POINT('Ctrl Pts',(5.405734701,3.395965514,-5.198849136));
#110397=CARTESIAN_POINT('Ctrl Pts',(5.320041815,3.376486685,-5.28795212699999));
#110398=CARTESIAN_POINT('Ctrl Pts',(5.2314589,3.357142857,-5.374182522));
#110399=CARTESIAN_POINT('Ctrl Pts',(5.02553655899999,3.31217565,-5.574636127));
#110400=CARTESIAN_POINT('Ctrl Pts',(4.804878973,3.266554913,-5.758744486));
#110401=CARTESIAN_POINT('Ctrl Pts',(5.39286432943003,3.3972605424113,-4.84557297336042));
#110402=CARTESIAN_POINT('Ctrl Pts',(5.39020606621502,3.39661302820565,-4.84852496518022));
#110403=CARTESIAN_POINT('Ctrl Pts',(5.387547803,3.395965514,-4.851476957));
#110404=CARTESIAN_POINT('Ctrl Pts',(5.30758067,3.376486685,-4.940280173));
#110405=CARTESIAN_POINT('Ctrl Pts',(5.224730277,3.357142857,-5.026399659));
#110406=CARTESIAN_POINT('Ctrl Pts',(5.032133918,3.31217565,-5.22659544400001));
#110407=CARTESIAN_POINT('Ctrl Pts',(4.82478297,3.266554913,-5.411466464));
#110408=CARTESIAN_POINT('',(5.40573470643638,3.39596551397716,-5.19884913029323));
#110409=CARTESIAN_POINT('Ctrl Pts',(4.99485417156935,3.3062889783089,-5.59476825287003));
#110410=CARTESIAN_POINT('Ctrl Pts',(5.07546648430106,3.32334891375403,-5.52279981230656));
#110411=CARTESIAN_POINT('Ctrl Pts',(5.15436406977217,3.34030767936791,-5.44922992368464));
#110412=CARTESIAN_POINT('Ctrl Pts',(5.23145889898019,3.35714285677832,-5.3741825227477));
#110413=CARTESIAN_POINT('Ctrl Pts',(5.29040470296592,3.37001483658936,-5.31680215796539));
#110414=CARTESIAN_POINT('Ctrl Pts',(5.34851555915562,3.38295904483425,-5.25834528453235));
#110415=CARTESIAN_POINT('Ctrl Pts',(5.40573470628808,3.39596551520492,-5.19884913024567));
#110416=CARTESIAN_POINT('',(5.39664125752635,3.3959655126796,-5.02516304056512));
#110417=CARTESIAN_POINT('Origin',(-1.06512021424976E-12,3.48737837499989,
1.34874750257197E-12));
#110418=CARTESIAN_POINT('',(5.00040409668657,3.48629831962102,-5.58980848202957));
#110419=CARTESIAN_POINT('Origin',(-0.139893566805701,3.62489370874121,0.123181968684504));
#110420=CARTESIAN_POINT('Origin',(-0.129030497729903,3.48214198866982,0.143249074360335));
#110421=CARTESIAN_POINT('Ctrl Pts',(6.22417039200001,3.266573167,-4.184459694));
#110422=CARTESIAN_POINT('Ctrl Pts',(5.997146059,3.330825242,-4.522146811));
#110423=CARTESIAN_POINT('Ctrl Pts',(5.734919982,3.395965514,-4.83329006));
#110424=CARTESIAN_POINT('Ctrl Pts',(5.880804839,3.266573167,-4.240121985));
#110425=CARTESIAN_POINT('Ctrl Pts',(5.650760595,3.330825242,-4.559180094));
#110426=CARTESIAN_POINT('Ctrl Pts',(5.38754780300001,3.395965514,-4.851476957));
#110427=CARTESIAN_POINT('',(5.73491998675332,3.39596551397696,-4.83329005408083));
#110428=CARTESIAN_POINT('',(5.56123389752299,3.39596551522583,-4.84238350273135));
#110429=CARTESIAN_POINT('',(6.08078704939524,3.30628897732461,-4.39021968257402));
#110430=CARTESIAN_POINT('Origin',(-0.135768054767925,3.48210502381861,0.13249211387284));
#110431=CARTESIAN_POINT('Ctrl Pts',(5.87807284719938,3.2673359249554,-4.24390852955201));
#110432=CARTESIAN_POINT('Ctrl Pts',(5.91174390509398,3.27415053062209,-4.26835007303321));
#110433=CARTESIAN_POINT('Ctrl Pts',(5.94549370534151,3.28079893112742,-4.29277443015119));
#110434=CARTESIAN_POINT('Ctrl Pts',(6.01305549792867,3.29377261871852,-4.34153362712332));
#110435=CARTESIAN_POINT('Ctrl Pts',(6.04690766664564,3.30010561489497,-4.36589745282733));
#110436=CARTESIAN_POINT('Ctrl Pts',(6.08078704722014,3.30628897719265,-4.39021968563735));
#110437=CARTESIAN_POINT('Ctrl Pts',(6.4012410481422,3.3972605424113,-3.90821961906406));
#110438=CARTESIAN_POINT('Ctrl Pts',(6.39909578157111,3.39661302820565,-3.91172469153203));
#110439=CARTESIAN_POINT('Ctrl Pts',(6.39695051500001,3.395965514,-3.915229764));
#110440=CARTESIAN_POINT('Ctrl Pts',(6.33241559,3.376486685,-4.020671014));
#110441=CARTESIAN_POINT('Ctrl Pts',(6.264440681,3.357142857,-4.123928098));
#110442=CARTESIAN_POINT('Ctrl Pts',(6.10642429,3.31217565,-4.363962426));
#110443=CARTESIAN_POINT('Ctrl Pts',(5.93050341,3.266554913,-4.591201292));
#110444=CARTESIAN_POINT('Ctrl Pts',(6.30843711407222,3.3972605424113,-3.5729797511861));
#110445=CARTESIAN_POINT('Ctrl Pts',(6.30647559053612,3.39661302820565,-3.57643417509305));
#110446=CARTESIAN_POINT('Ctrl Pts',(6.30451406700001,3.395965514,-3.579888599));
#110447=CARTESIAN_POINT('Ctrl Pts',(6.245506587,3.376486685,-3.683806215));
#110448=CARTESIAN_POINT('Ctrl Pts',(6.183106334,3.357142857,-3.785722661));
#110449=CARTESIAN_POINT('Ctrl Pts',(6.038048947,3.31217565,-4.022640503));
#110450=CARTESIAN_POINT('Ctrl Pts',(5.875287554,3.266554913,-4.247763666));
#110451=CARTESIAN_POINT('',(6.39695051908622,3.39596551397713,-3.91522975725942));
#110452=CARTESIAN_POINT('Ctrl Pts',(6.08078705139423,3.30628897830882,-4.39021968008645));
#110453=CARTESIAN_POINT('Ctrl Pts',(6.14404360579022,3.32334891375396,-4.30260455727574));
#110454=CARTESIAN_POINT('Ctrl Pts',(6.20528125817945,3.3403076793676,-4.21379404295133));
#110455=CARTESIAN_POINT('Ctrl Pts',(6.26444067997507,3.35714285672434,-4.12392809923762));
#110456=CARTESIAN_POINT('Ctrl Pts',(6.30967328093506,3.37001483649389,-4.05521765063235));
#110457=CARTESIAN_POINT('Ctrl Pts',(6.35385903796572,3.38295904483422,-3.9856353497436));
#110458=CARTESIAN_POINT('Ctrl Pts',(6.39695051892677,3.39596551520485,-3.91522975724217));
#110459=CARTESIAN_POINT('',(6.35073229512134,3.3959655126796,-3.74755917451584));
#110460=CARTESIAN_POINT('Origin',(6.00214322687975E-13,3.48737837499989,
-4.62737487216813E-13));
#110461=CARTESIAN_POINT('',(6.08514101776744,3.48629831964224,-4.38418279619622));
#110462=CARTESIAN_POINT('Origin',(-0.163103671461469,3.62489372136745,0.0902292550734224));
#110463=CARTESIAN_POINT('Origin',(-0.156808169483224,3.48214199047778,0.112162257750512));
#110464=CARTESIAN_POINT('Ctrl Pts',(6.97818789,3.266573167,-2.748616702));
#110465=CARTESIAN_POINT('Ctrl Pts',(6.829064008,3.330825242,-3.127212403));
#110466=CARTESIAN_POINT('Ctrl Pts',(6.639855232,3.395965514,-3.487452151));
#110467=CARTESIAN_POINT('Ctrl Pts',(6.654815779,3.266573167,-2.876791084));
#110468=CARTESIAN_POINT('Ctrl Pts',(6.498737904,3.330825242,-3.237842504));
#110469=CARTESIAN_POINT('Ctrl Pts',(6.304514067,3.395965514,-3.579888599));
#110470=CARTESIAN_POINT('',(6.63985523530303,3.39596551397696,-3.48745214416228));
#110471=CARTESIAN_POINT('',(6.47218465316547,3.39596551522583,-3.53367036828643));
#110472=CARTESIAN_POINT('',(6.88238908513195,3.30628897738563,-2.98038931745279));
#110473=CARTESIAN_POINT('Origin',(-0.161075771399515,3.48210503785382,0.100208411574002));
#110474=CARTESIAN_POINT('Ctrl Pts',(6.65296165528463,3.26733592498242,-2.8810763986581));
#110475=CARTESIAN_POINT('Ctrl Pts',(6.69109971203849,3.27415053066632,-2.89770823034314));
#110476=CARTESIAN_POINT('Ctrl Pts',(6.72931097559604,3.2807989311849,-2.91430635021598));
#110477=CARTESIAN_POINT('Ctrl Pts',(6.80577499705763,3.29377261878132,-2.94740179608021));
#110478=CARTESIAN_POINT('Ctrl Pts',(6.8440732232251,3.30010561496541,-2.96391879355285));
#110479=CARTESIAN_POINT('Ctrl Pts',(6.88238908369249,3.30628897725673,-2.98038932077374));
#110480=CARTESIAN_POINT('Ctrl Pts',(7.09173528189306,3.3972605424113,-2.44077001058573));
#110481=CARTESIAN_POINT('Ctrl Pts',(7.09039365744652,3.39661302820565,-2.44465430529287));
#110482=CARTESIAN_POINT('Ctrl Pts',(7.089052033,3.395965514,-2.4485386));
#110483=CARTESIAN_POINT('Ctrl Pts',(7.048692651,3.376486685,-2.565387793));
#110484=CARTESIAN_POINT('Ctrl Pts',(7.004504177,3.357142857,-2.68084338));
#110485=CARTESIAN_POINT('Ctrl Pts',(6.901782407,3.31217565,-2.949234692));
#110486=CARTESIAN_POINT('Ctrl Pts',(6.778824099,3.266554913,-3.208978629));
#110487=CARTESIAN_POINT('Ctrl Pts',(6.92903438933913,3.3972605424113,-2.13331796710826));
#110488=CARTESIAN_POINT('Ctrl Pts',(6.92786132416957,3.39661302820565,-2.13711329805413));
#110489=CARTESIAN_POINT('Ctrl Pts',(6.926688259,3.395965514,-2.140908629));
#110490=CARTESIAN_POINT('Ctrl Pts',(6.891399557,3.376486685,-2.255081572));
#110491=CARTESIAN_POINT('Ctrl Pts',(6.852367211,3.357142857,-2.368029478));
#110492=CARTESIAN_POINT('Ctrl Pts',(6.761631518,3.31217565,-2.630591364));
#110493=CARTESIAN_POINT('Ctrl Pts',(6.651070221,3.266554913,-2.88544016));
#110494=CARTESIAN_POINT('',(7.08905203541566,3.39596551397713,-2.44853859249506));
#110495=CARTESIAN_POINT('Ctrl Pts',(6.88238908634082,3.30628897830882,-2.98038931465817));
#110496=CARTESIAN_POINT('Ctrl Pts',(6.92533207594406,3.32334891375396,-2.88122429529154));
#110497=CARTESIAN_POINT('Ctrl Pts',(6.96604639052516,3.34030767936816,-2.78132583629271));
#110498=CARTESIAN_POINT('Ctrl Pts',(7.00450417663027,3.35714285683815,-2.68084338096604));
#110499=CARTESIAN_POINT('Ctrl Pts',(7.03390855033864,3.37001483669515,-2.60401567187915));
#110500=CARTESIAN_POINT('Ctrl Pts',(7.06210313077174,3.38295904483419,-2.52656153579043));
#110501=CARTESIAN_POINT('Ctrl Pts',(7.08905203538231,3.39596551520487,-2.44853859255604));
#110502=CARTESIAN_POINT('',(7.0078701485236,3.3959655126796,-2.29472360679316));
#110503=CARTESIAN_POINT('Origin',(7.78457159844592E-13,3.48737837499967,
-3.23525928269675E-13));
#110504=CARTESIAN_POINT('',(6.88534350783937,3.48629831963854,-2.97355759564998));
#110505=CARTESIAN_POINT('Origin',(-0.178686657029109,3.62489371308647,0.0530570999432844));
#110506=CARTESIAN_POINT('Origin',(-0.177253922351563,3.48214200983984,0.0758309610416999));
#110507=CARTESIAN_POINT('Ctrl Pts',(7.405913077,3.266573167,-1.184251449));
#110508=CARTESIAN_POINT('Ctrl Pts',(7.341662513,3.330825242,-1.586053019));
#110509=CARTESIAN_POINT('Ctrl Pts',(7.23431823,3.395965514,-1.978544855));
#110510=CARTESIAN_POINT('Ctrl Pts',(7.11765493,3.266573167,-1.37894463));
#110511=CARTESIAN_POINT('Ctrl Pts',(7.042841452,3.330825242,-1.765106997));
#110512=CARTESIAN_POINT('Ctrl Pts',(6.926688259,3.395965514,-2.140908629));
#110513=CARTESIAN_POINT('',(7.23431823199865,3.39596551397695,-1.97854484767375));
#110514=CARTESIAN_POINT('',(7.08050324663787,3.39596551522658,-2.05972673465086));
#110515=CARTESIAN_POINT('',(7.36217825648022,3.30628897732936,-1.43119925979488));
#110516=CARTESIAN_POINT('Origin',(-0.17885161942905,3.48210502933222,0.0632390378060677));
#110517=CARTESIAN_POINT('Ctrl Pts',(7.1167653709526,3.26733592502957,-1.3835283382044));
#110518=CARTESIAN_POINT('Ctrl Pts',(7.15758713331703,3.27415053070575,-1.39157277193384));
#110519=CARTESIAN_POINT('Ctrl Pts',(7.19847314391143,3.28079893121671,-1.39956854473737));
#110520=CARTESIAN_POINT('Ctrl Pts',(7.28026402154608,3.29377261878572,-1.41545273291013));
#110521=CARTESIAN_POINT('Ctrl Pts',(7.32121752243622,3.3001056149233,-1.42335058548555));
#110522=CARTESIAN_POINT('Ctrl Pts',(7.36217825580228,3.30628897719839,-1.43119926343611));
#110523=CARTESIAN_POINT('Ctrl Pts',(7.45062785596414,3.3972605424113,-0.859192708687909));
#110524=CARTESIAN_POINT('Ctrl Pts',(7.45015260648208,3.39661302820565,-0.863274600343954));
#110525=CARTESIAN_POINT('Ctrl Pts',(7.449677357,3.395965514,-0.867356492));
#110526=CARTESIAN_POINT('Ctrl Pts',(7.435380677,3.376486685,-0.99014989));
#110527=CARTESIAN_POINT('Ctrl Pts',(7.417044844,3.357142857,-1.112405405));
#110528=CARTESIAN_POINT('Ctrl Pts',(7.37442085,3.31217565,-1.396604021));
#110529=CARTESIAN_POINT('Ctrl Pts',(7.310174507,3.266554913,-1.676707691));
#110530=CARTESIAN_POINT('Ctrl Pts',(7.22563771925764,3.3972605424113,-0.593904605882858));
#110531=CARTESIAN_POINT('Ctrl Pts',(7.22530796362882,3.39661302820565,-0.597863378441429));
#110532=CARTESIAN_POINT('Ctrl Pts',(7.224978208,3.395965514,-0.601822151));
#110533=CARTESIAN_POINT('Ctrl Pts',(7.215058343,3.376486685,-0.720911822));
#110534=CARTESIAN_POINT('Ctrl Pts',(7.201219013,3.357142857,-0.839609869));
#110535=CARTESIAN_POINT('Ctrl Pts',(7.16904771400001,3.31217565,-1.115538695));
#110536=CARTESIAN_POINT('Ctrl Pts',(7.115856237,3.266554913,-1.38819668));
#110537=CARTESIAN_POINT('',(7.44967735812331,3.39596551354851,-0.867356486601909));
#110538=CARTESIAN_POINT('Ctrl Pts',(7.36217825729832,3.30628897830878,-1.43119925674442));
#110539=CARTESIAN_POINT('Ctrl Pts',(7.38279971594842,3.32334891375392,-1.3251211870437));
#110540=CARTESIAN_POINT('Ctrl Pts',(7.40108693691377,3.34030767936786,-1.21880592444598));
#110541=CARTESIAN_POINT('Ctrl Pts',(7.41704484379493,3.35714285678366,-1.11240540636732));
#110542=CARTESIAN_POINT('Ctrl Pts',(7.42924607266077,3.37001483659878,-1.03105281569138));
#110543=CARTESIAN_POINT('Ctrl Pts',(7.44013112972881,3.3829590448342,-0.949348512339761));
#110544=CARTESIAN_POINT('Ctrl Pts',(7.44967735772577,3.39596551520482,-0.867356484217573));
#110545=CARTESIAN_POINT('',(7.33732778330786,3.3959655126796,-0.734589313430841));
#110546=CARTESIAN_POINT('Origin',(-6.09321620936853E-13,3.487378375,2.26056152963228E-14));
#110547=CARTESIAN_POINT('',(7.36359498823962,3.48629831963846,-1.42389214627077));
#110548=CARTESIAN_POINT('Origin',(-0.185914974277281,3.62489366151202,0.0134043705532033));
#110549=CARTESIAN_POINT('Origin',(-0.189411175297511,3.48214197762132,0.0359537120336828));
#110550=CARTESIAN_POINT('Ctrl Pts',(7.487346,3.266573167,0.435488086));
#110551=CARTESIAN_POINT('Ctrl Pts',(7.510973039,3.330825242,0.029268441));
#110552=CARTESIAN_POINT('Ctrl Pts',(7.490512549,3.395965514,-0.377123002));
#110553=CARTESIAN_POINT('Ctrl Pts',(7.247680448,3.266573167,0.183379743));
#110554=CARTESIAN_POINT('Ctrl Pts',(7.257629561,3.330825242,-0.209837049));
#110555=CARTESIAN_POINT('Ctrl Pts',(7.224978208,3.395965514,-0.601822151));
#110556=CARTESIAN_POINT('',(7.49051254917363,3.39596551397693,-0.377122994396843));
#110557=CARTESIAN_POINT('',(7.35774537900854,3.39596551522778,-0.489472568855644));
#110558=CARTESIAN_POINT('',(7.4977201548532,3.3062889773198,0.184912084007772));
#110559=CARTESIAN_POINT('Origin',(-0.188264802751972,3.48210504267805,0.0233127280800562));
#110560=CARTESIAN_POINT('Ctrl Pts',(7.24779704645756,3.26733592488707,0.178711969599105));
#110561=CARTESIAN_POINT('Ctrl Pts',(7.28939373438671,3.27415053059898,0.179631082648405));
#110562=CARTESIAN_POINT('Ctrl Pts',(7.33104270767518,3.28079893112976,0.180611530324912));
#110563=CARTESIAN_POINT('Ctrl Pts',(7.41433599124088,3.29377261874755,0.182681326643943));
#110564=CARTESIAN_POINT('Ctrl Pts',(7.45602982699191,3.30010561490455,0.183771913555003));
#110565=CARTESIAN_POINT('Ctrl Pts',(7.49772015497779,3.30628897718653,0.18491208017517));
#110566=CARTESIAN_POINT('Ctrl Pts',(7.46113735175124,3.3972605424113,0.762559489829848));
#110567=CARTESIAN_POINT('Ctrl Pts',(7.46155069937562,3.39661302820565,0.758470865914925));
#110568=CARTESIAN_POINT('Ctrl Pts',(7.461964047,3.395965514,0.754382242));
#110569=CARTESIAN_POINT('Ctrl Pts',(7.474398566,3.376486685,0.631386321));
#110570=CARTESIAN_POINT('Ctrl Pts',(7.482772737,3.357142857,0.50804741));
#110571=CARTESIAN_POINT('Ctrl Pts',(7.50223956900001,3.31217565,0.221330301));
#110572=CARTESIAN_POINT('Ctrl Pts',(7.49970928,3.266554913,-0.066035765));
#110573=CARTESIAN_POINT('Ctrl Pts',(7.18437825902062,3.3972605424113,0.973279075776289));
#110574=CARTESIAN_POINT('Ctrl Pts',(7.18490723201031,3.39661302820565,0.969341969388144));
#110575=CARTESIAN_POINT('Ctrl Pts',(7.185436205,3.395965514,0.965404863));
#110576=CARTESIAN_POINT('Ctrl Pts',(7.201349021,3.376486685,0.846966964));
#110577=CARTESIAN_POINT('Ctrl Pts',(7.213349817,3.357142857,0.728068964));
#110578=CARTESIAN_POINT('Ctrl Pts',(7.241247207,3.31217565,0.451675322));
#110579=CARTESIAN_POINT('Ctrl Pts',(7.24791272300001,3.266554913,0.173957335));
#110580=CARTESIAN_POINT('',(7.46196404772562,3.39596551355055,0.754382245272086));
#110581=CARTESIAN_POINT('Ctrl Pts',(7.49772015484195,3.30628897830888,0.184912087247228));
#110582=CARTESIAN_POINT('Ctrl Pts',(7.49505584584998,3.32334891375402,0.292943114560101));
#110583=CARTESIAN_POINT('Ctrl Pts',(7.49006088308634,3.34030767936768,0.400703997279967));
#110584=CARTESIAN_POINT('Ctrl Pts',(7.48277273681091,3.35714285673465,0.50804740855631));
#110585=CARTESIAN_POINT('Ctrl Pts',(7.4772003050315,3.37001483626404,0.590120922717139));
#110586=CARTESIAN_POINT('Ctrl Pts',(7.47026686602102,3.38295904433524,0.672254989142124));
#110587=CARTESIAN_POINT('Ctrl Pts',(7.46196404651734,3.39596551445283,0.754382245007042));
#110588=CARTESIAN_POINT('',(7.32370012505435,3.3959655126796,0.859893560554126));
#110589=CARTESIAN_POINT('Origin',(6.28837260041593E-13,3.487378375,9.13711380862159E-14));
#110590=CARTESIAN_POINT('',(7.49753295098508,3.48629831961751,0.192352916921865));
#110591=CARTESIAN_POINT('Origin',(-0.18444968183899,3.62489371393,-0.0268752585810736));
#110592=CARTESIAN_POINT('Origin',(-0.192711909498522,3.48214199176069,-0.00560467464567588));
#110593=CARTESIAN_POINT('Ctrl Pts',(7.218678946,3.266573167,2.034864682));
#110594=CARTESIAN_POINT('Ctrl Pts',(7.329078814,3.330825242,1.643221342));
#110595=CARTESIAN_POINT('Ctrl Pts',(7.39645882600001,3.395965514,1.241932705));
#110596=CARTESIAN_POINT('Ctrl Pts',(7.038812482,3.266573167,1.737129483));
#110597=CARTESIAN_POINT('Ctrl Pts',(7.133058978,3.330825242,1.355244646));
#110598=CARTESIAN_POINT('Ctrl Pts',(7.185436205,3.395965514,0.965404863000001));
#110599=CARTESIAN_POINT('',(7.39645882446883,3.39596551397696,1.24193271243835));
#110600=CARTESIAN_POINT('',(7.29094751435517,3.39596551522583,1.10366879156288));
#110601=CARTESIAN_POINT('',(7.2826769922493,3.30628897734568,1.79237714414339));
#110602=CARTESIAN_POINT('Origin',(-0.188874803198071,3.48210505377031,-0.0177036707167831));
#110603=CARTESIAN_POINT('Ctrl Pts',(7.03992978882774,3.26733592500448,1.73259590554336));
#110604=CARTESIAN_POINT('Ctrl Pts',(7.08035638700341,3.27415053067568,1.74243558812496));
#110605=CARTESIAN_POINT('Ctrl Pts',(7.12082086307071,3.2807989311798,1.75234641132533));
#110606=CARTESIAN_POINT('Ctrl Pts',(7.20172185073038,3.2937726187524,1.77227341039973));
#110607=CARTESIAN_POINT('Ctrl Pts',(7.24220646393772,3.30010561492267,1.78230144215772));
#110608=CARTESIAN_POINT('Ctrl Pts',(7.28267699309591,3.30628897720145,1.79237714041993));
#110609=CARTESIAN_POINT('Ctrl Pts',(7.1227723568037,3.3972605424113,2.34865525323209));
#110610=CARTESIAN_POINT('Ctrl Pts',(7.12405497390185,3.39661302820565,2.34475107661605));
#110611=CARTESIAN_POINT('Ctrl Pts',(7.125337591,3.395965514,2.3408469));
#110612=CARTESIAN_POINT('Ctrl Pts',(7.163921886,3.376486685,2.22339961));
#110613=CARTESIAN_POINT('Ctrl Pts',(7.198614493,3.357142857,2.104744493));
#110614=CARTESIAN_POINT('Ctrl Pts',(7.279261905,3.31217565,1.828915464));
#110615=CARTESIAN_POINT('Ctrl Pts',(7.338565982,3.266554913,1.547723919));
#110616=CARTESIAN_POINT('Ctrl Pts',(6.80718525625549,3.3972605424113,2.49495330789937));
#110617=CARTESIAN_POINT('Ctrl Pts',(6.80854822362774,3.39661302820565,2.49122196244969));
#110618=CARTESIAN_POINT('Ctrl Pts',(6.809911191,3.395965514,2.487490617));
#110619=CARTESIAN_POINT('Ctrl Pts',(6.850912621,3.376486685,2.375242516));
#110620=CARTESIAN_POINT('Ctrl Pts',(6.888192401,3.357142857,2.261704102));
#110621=CARTESIAN_POINT('Ctrl Pts',(6.974854028,3.31217565,1.997769504));
#110622=CARTESIAN_POINT('Ctrl Pts',(7.041064867,3.266554913,1.727977298));
#110623=CARTESIAN_POINT('',(7.12533759102965,3.39596551355058,2.34084690331928));
#110624=CARTESIAN_POINT('Ctrl Pts',(7.2826769914196,3.3062889783088,1.79237714723104));
#110625=CARTESIAN_POINT('Ctrl Pts',(7.25685149499618,3.32334891375393,1.89730972162753));
#110626=CARTESIAN_POINT('Ctrl Pts',(7.22880790718498,3.34030767936789,2.00147744554113));
#110627=CARTESIAN_POINT('Ctrl Pts',(7.19861449338123,3.35714285678744,2.10474449169613));
#110628=CARTESIAN_POINT('Ctrl Pts',(7.17552896304024,3.37001483635539,2.18370126497809));
#110629=CARTESIAN_POINT('Ctrl Pts',(7.15110122700862,3.38295904433124,2.26242459777464));
#110630=CARTESIAN_POINT('Ctrl Pts',(7.12533758989274,3.39596551444677,2.34084690279715));
#110631=CARTESIAN_POINT('',(6.96762438834504,3.3959655126796,2.41416876616258));
#110632=CARTESIAN_POINT('Origin',(7.45931094670027E-14,3.48737837499989,
3.07913416985883E-14));
#110633=CARTESIAN_POINT('',(7.28089460575553,3.48629831964464,1.79960377154734));
#110634=CARTESIAN_POINT('Origin',(-0.174359959206638,3.62489367356382,-0.0658981559459898));
#110635=CARTESIAN_POINT('Origin',(-0.187001520370689,3.4821419913019,-0.0469009982022248));
#110636=CARTESIAN_POINT('Ctrl Pts',(6.612474487,3.266573167,3.539093268));
#110637=CARTESIAN_POINT('Ctrl Pts',(6.804485009,3.330825242,3.180339039));
#110638=CARTESIAN_POINT('Ctrl Pts',(6.956554908,3.395965514,2.802917018));
#110639=CARTESIAN_POINT('Ctrl Pts',(6.50081746800001,3.266573167,3.209652979));
#110640=CARTESIAN_POINT('Ctrl Pts',(6.674954485,3.330825242,2.856956608));
#110641=CARTESIAN_POINT('Ctrl Pts',(6.809911191,3.395965514,2.487490617));
#110642=CARTESIAN_POINT('',(6.95655490512513,3.39596551397696,2.80291702502385));
#110643=CARTESIAN_POINT('',(6.88323304675614,3.39596551522583,2.64520382463995));
#110644=CARTESIAN_POINT('',(6.72710394729357,3.30628897734393,3.3160326417093));
#110645=CARTESIAN_POINT('Origin',(-0.180653151738133,3.48210507734314,-0.0578922113520686));
#110646=CARTESIAN_POINT('Ctrl Pts',(6.50288323813701,3.26733592504243,3.20546558201951));
#110647=CARTESIAN_POINT('Ctrl Pts',(6.54024944394122,3.27415053070218,3.22376574196963));
#110648=CARTESIAN_POINT('Ctrl Pts',(6.57763734891704,3.28079893119047,3.24214352186137));
#110649=CARTESIAN_POINT('Ctrl Pts',(6.65236354640081,3.29377267879171,3.278996130233));
#110650=CARTESIAN_POINT('Ctrl Pts',(6.68974631313084,3.30010573699289,3.29749290274777));
#110651=CARTESIAN_POINT('Ctrl Pts',(6.72710394902543,3.3062889772105,3.31603263823113));
#110652=CARTESIAN_POINT('Ctrl Pts',(6.45135444343917,3.3972605424113,3.82493050776523));
#110653=CARTESIAN_POINT('Ctrl Pts',(6.45344635621958,3.39661302820565,3.82139333338262));
#110654=CARTESIAN_POINT('Ctrl Pts',(6.455538269,3.395965514,3.817856159));
#110655=CARTESIAN_POINT('Ctrl Pts',(6.51846818000001,3.376486685,3.711449204));
#110656=CARTESIAN_POINT('Ctrl Pts',(6.577857036,3.357142857,3.603026063));
#110657=CARTESIAN_POINT('Ctrl Pts',(6.71591404400001,3.31217565,3.350982573));
#110658=CARTESIAN_POINT('Ctrl Pts',(6.834279495,3.266554913,3.089113754));
#110659=CARTESIAN_POINT('Ctrl Pts',(6.11169583714959,3.3972605424113,3.89996629798646));
#110660=CARTESIAN_POINT('Ctrl Pts',(6.1138290680748,3.39661302820565,3.89661518699323));
#110661=CARTESIAN_POINT('Ctrl Pts',(6.115962299,3.395965514,3.893264076));
#110662=CARTESIAN_POINT('Ctrl Pts',(6.180135162,3.376486685,3.792454368));
#110663=CARTESIAN_POINT('Ctrl Pts',(6.240950764,3.357142857,3.68958447));
#110664=CARTESIAN_POINT('Ctrl Pts',(6.382324428,3.31217565,3.450450204));
#110665=CARTESIAN_POINT('Ctrl Pts',(6.504984643,3.266554913,3.201198963));
#110666=CARTESIAN_POINT('',(6.45553826832072,3.39596551355059,3.81785616224398));
#110667=CARTESIAN_POINT('Ctrl Pts',(6.72710394570673,3.30628897830882,3.31603264454493));
#110668=CARTESIAN_POINT('Ctrl Pts',(6.67932483331376,3.32334891375395,3.41296023525716));
#110669=CARTESIAN_POINT('Ctrl Pts',(6.62954390754829,3.34030767936776,3.50866403323463));
#110670=CARTESIAN_POINT('Ctrl Pts',(6.5778570366183,3.35714285675868,3.60302606167889));
#110671=CARTESIAN_POINT('Ctrl Pts',(6.53833786072227,3.37001483630424,3.67517416255527));
#110672=CARTESIAN_POINT('Ctrl Pts',(6.49755804217794,3.38295904433065,3.74680574662116));
#110673=CARTESIAN_POINT('Ctrl Pts',(6.45553826732074,3.39596551444587,3.81785616148869));
#110674=CARTESIAN_POINT('',(6.28575027975988,3.3959655126796,3.8555601244127));
#110675=CARTESIAN_POINT('Origin',(-1.33703811910912E-12,3.48737837499989,
-6.96057794735694E-13));
#110676=CARTESIAN_POINT('',(6.72380972100027,3.48629831961384,3.32270715385137));
#110677=CARTESIAN_POINT('Origin',(-0.156117583026004,3.62489372625139,-0.101839827650431));
#110678=CARTESIAN_POINT('Origin',(-0.172547195397816,3.48214198959482,-0.0860042770115643));
#110679=CARTESIAN_POINT('Ctrl Pts',(5.69707807,3.266573167,4.877837785));
#110680=CARTESIAN_POINT('Ctrl Pts',(5.961721047,3.330825242,4.568747618));
#110681=CARTESIAN_POINT('Ctrl Pts',(6.191370215,3.395965514,4.232840047));
#110682=CARTESIAN_POINT('Ctrl Pts',(5.658851455,3.266573167,4.532096669));
#110683=CARTESIAN_POINT('Ctrl Pts',(5.90473653900001,3.330825242,4.225080454));
#110684=CARTESIAN_POINT('Ctrl Pts',(6.115962299,3.395965514,3.893264076));
#110685=CARTESIAN_POINT('',(6.1913702105932,3.39596551397696,4.23284005318075));
#110686=CARTESIAN_POINT('',(6.15366625278541,3.39596551522583,4.06305206788318));
#110687=CARTESIAN_POINT('',(5.85697899846951,3.30628897736477,4.68463413833494));
#110688=CARTESIAN_POINT('Origin',(-0.163984420983014,3.48210502581023,-0.0953737962201601));
#110689=CARTESIAN_POINT('Ctrl Pts',(5.66176909444807,3.2673359249139,4.52845124930181));
#110690=CARTESIAN_POINT('Ctrl Pts',(5.69432770575813,3.2741505306263,4.55435619189982));
#110691=CARTESIAN_POINT('Ctrl Pts',(5.72689082285085,3.28079893114848,4.58034160419976));
#110692=CARTESIAN_POINT('Ctrl Pts',(5.79194744092253,3.29377261878756,4.63239630226048));
#110693=CARTESIAN_POINT('Ctrl Pts',(5.8244796192849,3.30010561494795,4.65849654522998));
#110694=CARTESIAN_POINT('Ctrl Pts',(5.85697900078839,3.30628897723755,4.68463413548175));
#110695=CARTESIAN_POINT('Ctrl Pts',(5.47827836712809,3.39726054241128,5.12235626254302));
#110696=CARTESIAN_POINT('Ctrl Pts',(5.48108176006405,3.39661302820564,5.11935148477151));
#110697=CARTESIAN_POINT('Ctrl Pts',(5.483885153,3.395965514,5.116346707));
#110698=CARTESIAN_POINT('Ctrl Pts',(5.568218147,3.376486685,5.025955559));
#110699=CARTESIAN_POINT('Ctrl Pts',(5.649526295,3.357142857,4.932834139));
#110700=CARTESIAN_POINT('Ctrl Pts',(5.838537507,3.31217565,4.71636146100001));
#110701=CARTESIAN_POINT('Ctrl Pts',(6.010429695,3.266554913,4.486060063));
#110702=CARTESIAN_POINT('Ctrl Pts',(5.13043031307462,3.39726054241128,5.12262119754953));
#110703=CARTESIAN_POINT('Ctrl Pts',(5.13323406003731,3.39661302820564,5.11980701527477));
#110704=CARTESIAN_POINT('Ctrl Pts',(5.136037807,3.395965514,5.11699283300001));
#110705=CARTESIAN_POINT('Ctrl Pts',(5.220381451,3.376486685,5.032335269));
#110706=CARTESIAN_POINT('Ctrl Pts',(5.301889206,3.357142857,4.944943968));
#110707=CARTESIAN_POINT('Ctrl Pts',(5.49136443,3.31217565,4.741791688));
#110708=CARTESIAN_POINT('Ctrl Pts',(5.664738566,3.266554913,4.524736122));
#110709=CARTESIAN_POINT('',(5.48388514991963,3.39596551354712,5.11634671104307));
#110710=CARTESIAN_POINT('Ctrl Pts',(5.85697899656006,3.30628897830817,4.6846341407772));
#110711=CARTESIAN_POINT('Ctrl Pts',(5.7894803663614,3.32334891375353,4.76902452145373));
#110712=CARTESIAN_POINT('Ctrl Pts',(5.72028980334209,3.34030767936758,4.85178939038818));
#110713=CARTESIAN_POINT('Ctrl Pts',(5.64952629587156,3.35714285676466,4.93283413787115));
#110714=CARTESIAN_POINT('Ctrl Pts',(5.59542134620887,3.3700148365652,4.99480000303176));
#110715=CARTESIAN_POINT('Ctrl Pts',(5.5401962631029,3.38295904483422,5.0559904258671));
#110716=CARTESIAN_POINT('Ctrl Pts',(5.48388514753892,3.39596551520486,5.1163467125916));
#110717=CARTESIAN_POINT('',(5.30996147437299,3.3959655126796,5.11666977583958));
#110718=CARTESIAN_POINT('Origin',(-2.61509564003504E-13,3.48737837500056,
-2.7451999007333E-13));
#110719=CARTESIAN_POINT('',(5.85232696648482,3.48629831960878,4.69044444290798));
#110720=CARTESIAN_POINT('Origin',(-0.130574933793124,3.62489369821667,-0.133019419928523));
#110721=CARTESIAN_POINT('Origin',(-0.150024756310734,3.48214198979312,-0.121086082947772));
#110722=CARTESIAN_POINT('Ctrl Pts',(4.515292615,3.266573167,5.988500029));
#110723=CARTESIAN_POINT('Ctrl Pts',(4.840193635,3.330825242,5.74352663499999));
#110724=CARTESIAN_POINT('Ctrl Pts',(5.136683932,3.395965514,5.464840179));
#110725=CARTESIAN_POINT('Ctrl Pts',(4.552283837,3.266573167,5.642624555));
#110726=CARTESIAN_POINT('Ctrl Pts',(4.858419675,3.330825242,5.395644234));
#110727=CARTESIAN_POINT('Ctrl Pts',(5.136037807,3.395965514,5.116992833));
#110728=CARTESIAN_POINT('',(5.13668392641925,3.39596551397696,5.46484018414394));
#110729=CARTESIAN_POINT('',(5.13636086401175,3.39596551522583,5.29091651132793));
#110730=CARTESIAN_POINT('',(4.71298822131528,3.30628897735935,5.83418734891346));
#110731=CARTESIAN_POINT('Origin',(-0.139648144273157,3.48210502084463,-0.12839596685466));
#110732=CARTESIAN_POINT('Ctrl Pts',(4.55591692076069,3.2673359248366,5.63969156977355));
#110733=CARTESIAN_POINT('Ctrl Pts',(4.58214553288379,3.27415053054439,5.67199000816677));
#110734=CARTESIAN_POINT('Ctrl Pts',(4.6083612468954,3.28079893108282,5.70436800366454));
#110735=CARTESIAN_POINT('Ctrl Pts',(4.66070665598637,3.29377261873428,5.76919094168075));
#110736=CARTESIAN_POINT('Ctrl Pts',(4.68686746942877,3.30010561492014,5.80167443228908));
#110737=CARTESIAN_POINT('Ctrl Pts',(4.71298822421363,3.3062889772303,5.83418734660105));
#110738=CARTESIAN_POINT('Ctrl Pts',(4.24904408282165,3.3972605424113,6.18026633229042));
#110739=CARTESIAN_POINT('Ctrl Pts',(4.25242787241083,3.39661302820565,6.17793445114522));
#110740=CARTESIAN_POINT('Ctrl Pts',(4.255811662,3.395965514,6.17560257000001));
#110741=CARTESIAN_POINT('Ctrl Pts',(4.357604423,3.376486685,6.105453817));
#110742=CARTESIAN_POINT('Ctrl Pts',(4.457029984,3.357142857,6.031988372));
#110743=CARTESIAN_POINT('Ctrl Pts',(4.68815744500001,3.31217565,5.86120852900001));
#110744=CARTESIAN_POINT('Ctrl Pts',(4.905538882,3.266554913,5.673243189));
#110745=CARTESIAN_POINT('Ctrl Pts',(3.90927156911326,3.3972605424113,6.1057480230819));
#110746=CARTESIAN_POINT('Ctrl Pts',(3.91261473205663,3.39661302820565,6.10360235754095));
#110747=CARTESIAN_POINT('Ctrl Pts',(3.915957895,3.395965514,6.101456692));
#110748=CARTESIAN_POINT('Ctrl Pts',(4.016528506,3.376486685,6.036909765));
#110749=CARTESIAN_POINT('Ctrl Pts',(4.114917201,3.357142857,5.969083383));
#110750=CARTESIAN_POINT('Ctrl Pts',(4.343634335,3.31217565,5.811412262));
#110751=CARTESIAN_POINT('Ctrl Pts',(4.55961561000001,3.266554913,5.636701649));
#110752=CARTESIAN_POINT('',(4.25581165538039,3.39596551397713,6.17560257428537));
#110753=CARTESIAN_POINT('Ctrl Pts',(4.71298821889922,3.30628897830884,5.83418735089416));
#110754=CARTESIAN_POINT('Ctrl Pts',(4.6289262320271,3.32334891375397,5.90209452101998));
#110755=CARTESIAN_POINT('Ctrl Pts',(4.54356130583569,3.34030767936806,5.968050467354));
#110756=CARTESIAN_POINT('Ctrl Pts',(4.45702998493824,3.35714285681746,6.03198837130674));
#110757=CARTESIAN_POINT('Ctrl Pts',(4.39086914972084,3.37001483665857,6.08087454457559));
#110758=CARTESIAN_POINT('Ctrl Pts',(4.32378106640564,3.38295904483421,6.12876260887068));
#110759=CARTESIAN_POINT('Ctrl Pts',(4.2558116554647,3.39596551520487,6.17560257428695));
#110760=CARTESIAN_POINT('',(4.08588477174921,3.3959655126796,6.13852963549342));
#110761=CARTESIAN_POINT('Origin',(-3.0964814046186E-13,3.48737837500011,
-4.24573570745324E-13));
#110762=CARTESIAN_POINT('',(4.70719590771123,3.486298319625,5.83886176247301));
#110763=CARTESIAN_POINT('Origin',(-0.0989268748628985,3.62489373771985,
-0.15797920210728));
#110764=CARTESIAN_POINT('Origin',(-0.120487295497355,3.48214202377494,-0.150505976053753));
#110765=CARTESIAN_POINT('Ctrl Pts',(3.122377096,3.266573167,6.819146668));
#110766=CARTESIAN_POINT('Ctrl Pts',(3.492344149,3.330825242,6.649744731));
#110767=CARTESIAN_POINT('Ctrl Pts',(3.841812017,3.395965514,6.441310459));
#110768=CARTESIAN_POINT('Ctrl Pts',(3.232856486,3.266573167,6.489309589));
#110769=CARTESIAN_POINT('Ctrl Pts',(3.584928506,3.330825242,6.31391368600001));
#110770=CARTESIAN_POINT('Ctrl Pts',(3.915957895,3.395965514,6.101456692));
#110771=CARTESIAN_POINT('',(3.84181201039949,3.39596551397696,6.44131046274925));
#110772=CARTESIAN_POINT('',(3.87888494949472,3.39596551522583,6.27138357952356));
#110773=CARTESIAN_POINT('',(3.34862335342703,3.30628897733836,6.71094044364197));
#110774=CARTESIAN_POINT('Origin',(-0.1087818672081,3.48210502909658,-0.155414273976533));
#110775=CARTESIAN_POINT('Ctrl Pts',(3.23703513543889,3.26733592487956,6.4872261814177));
#110776=CARTESIAN_POINT('Ctrl Pts',(3.25570709551634,3.27415044581596,6.52440741390821));
#110777=CARTESIAN_POINT('Ctrl Pts',(3.27434932675907,3.28079875863233,6.56166350460611));
#110778=CARTESIAN_POINT('Ctrl Pts',(3.31153658116327,3.29377267903747,6.63622497162145));
#110779=CARTESIAN_POINT('Ctrl Pts',(3.33010297381103,3.30010573760448,6.67357321278013));
#110780=CARTESIAN_POINT('Ctrl Pts',(3.34862335692902,3.30628897720421,6.71094044191187));
#110781=CARTESIAN_POINT('Ctrl Pts',(2.82112921903796,3.39726054241128,6.94919401667821));
#110782=CARTESIAN_POINT('Ctrl Pts',(2.82493518301898,3.39661302820564,6.9476440683391));
#110783=CARTESIAN_POINT('Ctrl Pts',(2.828741147,3.395965514,6.94609412));
#110784=CARTESIAN_POINT('Ctrl Pts',(2.943233958,3.376486685,6.89946784));
#110785=CARTESIAN_POINT('Ctrl Pts',(3.056127904,3.357142857,6.849093534));
#110786=CARTESIAN_POINT('Ctrl Pts',(3.318564352,3.31217565,6.73199200100001));
#110787=CARTESIAN_POINT('Ctrl Pts',(3.571270523,3.266554913,6.595151768));
#110788=CARTESIAN_POINT('Ctrl Pts',(2.50531963238601,3.39726054241128,6.80337685771355));
#110789=CARTESIAN_POINT('Ctrl Pts',(2.50904588869301,3.39661302820564,6.80200003785678));
#110790=CARTESIAN_POINT('Ctrl Pts',(2.512772145,3.395965514,6.800623218));
#110791=CARTESIAN_POINT('Ctrl Pts',(2.624867152,3.376486685,6.759205071));
#110792=CARTESIAN_POINT('Ctrl Pts',(2.735536241,3.357142857,6.714115092));
#110793=CARTESIAN_POINT('Ctrl Pts',(2.992800725,3.31217565,6.609297658));
#110794=CARTESIAN_POINT('Ctrl Pts',(3.241290096,3.266554913,6.485101272));
#110795=CARTESIAN_POINT('',(2.82874113965045,3.39596551397711,6.9460941228516));
#110796=CARTESIAN_POINT('Ctrl Pts',(3.34862335043211,3.30628897830838,6.71094044494617));
#110797=CARTESIAN_POINT('Ctrl Pts',(3.25192865189507,3.32334891375364,6.75918914112259));
#110798=CARTESIAN_POINT('Ctrl Pts',(3.15438093133575,3.34030767936753,6.80525213843028));
#110799=CARTESIAN_POINT('Ctrl Pts',(3.05612790517976,3.35714285674499,6.849093533206));
#110800=CARTESIAN_POINT('Ctrl Pts',(2.9810047912196,3.37001483653036,6.88261415006091));
#110801=CARTESIAN_POINT('Ctrl Pts',(2.90519067147907,3.38295904483422,6.91496066358033));
#110802=CARTESIAN_POINT('Ctrl Pts',(2.82874113969565,3.39596551520471,6.94609412278089));
#110803=CARTESIAN_POINT('',(2.67075663844161,3.39596551267969,6.87335867193694));
#110804=CARTESIAN_POINT('Origin',(-1.02999206386123E-13,3.487378375,-1.96023752785379E-13));
#110805=CARTESIAN_POINT('',(3.34196159990722,3.48629831963972,6.71426039577534));
#110806=CARTESIAN_POINT('Origin',(-0.0626532617245851,3.62489367964053,
-0.175552255267503));
#110807=CARTESIAN_POINT('Origin',(-0.085315925288148,3.48214200458338,-0.172888223368134));
#110808=CARTESIAN_POINT('Ctrl Pts',(1.583462693,3.266573167,7.330937587));
#110809=CARTESIAN_POINT('Ctrl Pts',(1.981196531,3.330825242,7.24502815300001));
#110810=CARTESIAN_POINT('Ctrl Pts',(2.367301242,3.395965514,7.11659222000001));
#110811=CARTESIAN_POINT('Ctrl Pts',(1.762264358,3.266573167,7.032561719));
#110812=CARTESIAN_POINT('Ctrl Pts',(2.143810065,3.330825242,6.93695155199999));
#110813=CARTESIAN_POINT('Ctrl Pts',(2.512772145,3.395965514,6.800623218));
#110814=CARTESIAN_POINT('',(2.36730123479723,3.39596551397696,7.11659222239137));
#110815=CARTESIAN_POINT('',(2.44003668628186,3.39596551522583,6.95860772153104));
#110816=CARTESIAN_POINT('',(1.82768057874502,3.30628897738304,7.27389742193992));
#110817=CARTESIAN_POINT('Origin',(-0.0728291577683449,3.48210502662294,
-0.175165736868625));
#110818=CARTESIAN_POINT('Ctrl Pts',(1.76679318450052,3.26733592499019,7.03142530652031));
#110819=CARTESIAN_POINT('Ctrl Pts',(1.77703586598406,3.27415053065561,7.07175168348233));
#110820=CARTESIAN_POINT('Ctrl Pts',(1.78723343627441,3.28079893115732,7.11214484880847));
#110821=CARTESIAN_POINT('Ctrl Pts',(1.80752239786033,3.2937726187693,7.1929558207359));
#110822=CARTESIAN_POINT('Ctrl Pts',(1.81762584548155,3.30010561494277,7.23342167884843));
#110823=CARTESIAN_POINT('Ctrl Pts',(1.82768058216335,3.30628897725914,7.27389742110968));
#110824=CARTESIAN_POINT('Ctrl Pts',(1.26130148850622,3.3972605424113,7.39318511227826));
#110825=CARTESIAN_POINT('Ctrl Pts',(1.26535166425311,3.39661302820565,7.39248957063913));
#110826=CARTESIAN_POINT('Ctrl Pts',(1.26940184,3.395965514,7.39179402900001));
#110827=CARTESIAN_POINT('Ctrl Pts',(1.391241145,3.376486685,7.370870416));
#110828=CARTESIAN_POINT('Ctrl Pts',(1.51232468,3.357142857,7.345942694));
#110829=CARTESIAN_POINT('Ctrl Pts',(1.793798878,3.31217565,7.28799500900001));
#110830=CARTESIAN_POINT('Ctrl Pts',(2.070013524,3.266554913,7.208678382));
#110831=CARTESIAN_POINT('Ctrl Pts',(0.98422173280296,3.3972605424113,7.18288735118082));
#110832=CARTESIAN_POINT('Ctrl Pts',(0.98815684690148,3.39661302820565,7.18234375559041));
#110833=CARTESIAN_POINT('Ctrl Pts',(0.992091961000001,3.395965514,7.18180016));
#110834=CARTESIAN_POINT('Ctrl Pts',(1.110469927,3.376486685,7.16544746));
#110835=CARTESIAN_POINT('Ctrl Pts',(1.228244647,3.357142857,7.145202243));
#110836=CARTESIAN_POINT('Ctrl Pts',(1.502027081,3.31217565,7.09813964100001));
#110837=CARTESIAN_POINT('Ctrl Pts',(1.77140546,3.266554913,7.030264767));
#110838=CARTESIAN_POINT('',(1.26940183221709,3.39596551397713,7.39179403025101));
#110839=CARTESIAN_POINT('Ctrl Pts',(1.82768057589193,3.30628897830882,7.27389742284408));
#110840=CARTESIAN_POINT('Ctrl Pts',(1.72287450224015,3.32334891375395,7.30023158920542));
#110841=CARTESIAN_POINT('Ctrl Pts',(1.61770521034536,3.34030767936791,7.32424778261358));
#110842=CARTESIAN_POINT('Ctrl Pts',(1.51232468132775,3.35714285678788,7.34594269372665));
#110843=CARTESIAN_POINT('Ctrl Pts',(1.4317519622742,3.37001483660626,7.36253036886505));
#110844=CARTESIAN_POINT('Ctrl Pts',(1.35075679015301,3.38295904483418,7.37782284375787));
#110845=CARTESIAN_POINT('Ctrl Pts',(1.26940183226868,3.39596551520485,7.39179403014655));
#110846=CARTESIAN_POINT('',(1.13074689248646,3.3959655126796,7.28679709574352));
#110847=CARTESIAN_POINT('Origin',(-3.19622800448727E-13,3.48737837500067,
-1.20606649667288E-12));
#110848=CARTESIAN_POINT('',(1.82046088170413,3.48629831962542,7.27570767520948));
#110849=CARTESIAN_POINT('Origin',(-0.0234499208463798,3.6248937128969,-0.184916550395832));
#110850=CARTESIAN_POINT('Origin',(-0.0461554583641602,3.48214200263419,
-0.187186741471569));
#110851=CARTESIAN_POINT('Ctrl Pts',(-0.029492665,3.266573167,7.499942012));
#110852=CARTESIAN_POINT('Ctrl Pts',(0.377410366,3.330825242,7.501542112));
#110853=CARTESIAN_POINT('Ctrl Pts',(0.782098092,3.395965514,7.45911003900001));
#110854=CARTESIAN_POINT('Ctrl Pts',(0.209270708,3.266573167,7.246979079));
#110855=CARTESIAN_POINT('Ctrl Pts',(0.602449449000001,3.330825242,7.235625273));
#110856=CARTESIAN_POINT('Ctrl Pts',(0.992091961,3.395965514,7.18180016));
#110857=CARTESIAN_POINT('',(0.782098084443958,3.39596551397696,7.45911003971456));
#110858=CARTESIAN_POINT('',(0.887095018906516,3.39596551522583,7.32045510042018));
#110859=CARTESIAN_POINT('',(0.221277491332775,3.3062889773396,7.49673504102568));
#110860=CARTESIAN_POINT('Origin',(-0.0334709849852924,3.48210504334308,
-0.186726363592657));
#110861=CARTESIAN_POINT('Ctrl Pts',(0.213937948288746,3.26733592498261,
7.24684279884774));
#110862=CARTESIAN_POINT('Ctrl Pts',(0.215272182578208,3.27415053065561,
7.28842824134559));
#110863=CARTESIAN_POINT('Ctrl Pts',(0.21654800280224,3.28079893116271,7.33006921317212));
#110864=CARTESIAN_POINT('Ctrl Pts',(0.21899064948497,3.29377261875098,7.41335239647561));
#110865=CARTESIAN_POINT('Ctrl Pts',(0.220158920749398,3.30010561492063,
7.45504412795859));
#110866=CARTESIAN_POINT('Ctrl Pts',(0.221277495101919,3.3062889772091,7.49673504094391));
#110867=CARTESIAN_POINT('Ctrl Pts',(-0.357503297558374,3.39726054241128,
7.49147908942938));
#110868=CARTESIAN_POINT('Ctrl Pts',(-0.353398291779187,3.39661302820564,
7.49167047721469));
#110869=CARTESIAN_POINT('Ctrl Pts',(-0.349293286,3.395965514,7.491861865));
#110870=CARTESIAN_POINT('Ctrl Pts',(-0.225804558,3.376486685,7.497619283));
#110871=CARTESIAN_POINT('Ctrl Pts',(-0.102193166,3.357142857,7.499303738));
#110872=CARTESIAN_POINT('Ctrl Pts',(0.185157361,3.31217565,7.50321947));
#110873=CARTESIAN_POINT('Ctrl Pts',(0.471964993000001,3.266554913,7.48513520600001));
#110874=CARTESIAN_POINT('Ctrl Pts',(-0.582897279531815,3.39726054241128,
7.2265340158684));
#110875=CARTESIAN_POINT('Ctrl Pts',(-0.578937309265908,3.39661302820564,
7.2268490624342));
#110876=CARTESIAN_POINT('Ctrl Pts',(-0.574977339,3.395965514,7.227164109));
#110877=CARTESIAN_POINT('Ctrl Pts',(-0.455851638000001,3.376486685,7.236641489));
#110878=CARTESIAN_POINT('Ctrl Pts',(-0.336478302,3.357142857,7.242187677));
#110879=CARTESIAN_POINT('Ctrl Pts',(-0.058979681,3.31217565,7.25508050300001));
#110880=CARTESIAN_POINT('Ctrl Pts',(0.218691873,3.266554913,7.246700895));
#110881=CARTESIAN_POINT('',(-0.349293289221942,3.39596551355055,7.49186186590368));
#110882=CARTESIAN_POINT('Ctrl Pts',(0.221277488156341,3.3062889783084,7.49673504116422));
#110883=CARTESIAN_POINT('Ctrl Pts',(0.113260654782681,3.32334891375368,
7.49992332148587));
#110884=CARTESIAN_POINT('Ctrl Pts',(0.00538739075076868,3.34030767936764,
7.50076974060923));
#110885=CARTESIAN_POINT('Ctrl Pts',(-0.102193164471641,3.35714285676083,
7.49930373802083));
#110886=CARTESIAN_POINT('Ctrl Pts',(-0.184447995828977,3.37001483630999,
7.49818284974637));
#110887=CARTESIAN_POINT('Ctrl Pts',(-0.266836974385724,3.38295904433457,
7.49570622753082));
#110888=CARTESIAN_POINT('Ctrl Pts',(-0.349293289022749,3.39596551445177,
7.49186186468031));
#110889=CARTESIAN_POINT('',(-0.462135320593511,3.3959655126796,7.35951298649177));
#110890=CARTESIAN_POINT('Origin',(4.30970363562988E-15,3.48737837499922,
3.37403716077489E-13));
#110891=CARTESIAN_POINT('',(0.213837435912931,3.48629831963484,7.49695095004132));
#110892=CARTESIAN_POINT('Origin',(0.0168499294855356,3.62489369157933,-0.185634169748569));
#110893=CARTESIAN_POINT('Origin',(-0.00483675567923905,3.48214198196337,
-0.192732463258353));
#110894=CARTESIAN_POINT('Ctrl Pts',(0.431186334568378,2.49597508212359,
7.48817336585162));
#110895=CARTESIAN_POINT('Ctrl Pts',(0.445305298725013,2.4937079305618,7.48730692006504));
#110896=CARTESIAN_POINT('Ctrl Pts',(0.459424262881653,2.491440779,7.48644047427845));
#110897=CARTESIAN_POINT('Ctrl Pts',(0.868893215852792,2.425690334,7.46131238094947));
#110898=CARTESIAN_POINT('Ctrl Pts',(1.27317905959915,2.360702725,7.39167617769089));
#110899=CARTESIAN_POINT('Ctrl Pts',(0.178710628942825,2.4959750821236,7.24784866891599));
#110900=CARTESIAN_POINT('Ctrl Pts',(0.192378157971412,2.4937079305618,7.24746007945792));
#110901=CARTESIAN_POINT('Ctrl Pts',(0.206045687,2.491440779,7.24707149000001));
#110902=CARTESIAN_POINT('Ctrl Pts',(0.602422414,2.425690334,7.235801873));
#110903=CARTESIAN_POINT('Ctrl Pts',(0.99520558,2.360702725,7.181369358));
#110904=CARTESIAN_POINT('',(0.990540537957771,2.36147458141303,7.18201430105441));
#110905=CARTESIAN_POINT('Origin',(0.00477268321056754,2.55353552148333,
-0.196313054014068));
#110906=CARTESIAN_POINT('Ctrl Pts',(1.02346990277171,2.40074633455827,7.42983912041194));
#110907=CARTESIAN_POINT('Ctrl Pts',(1.01793509438388,2.3945034694007,7.38850162286635));
#110908=CARTESIAN_POINT('Ctrl Pts',(1.01241952112976,2.38811405787387,7.34716093692049));
#110909=CARTESIAN_POINT('Ctrl Pts',(1.00144325721363,2.37503353899324,7.26456531650046));
#110910=CARTESIAN_POINT('Ctrl Pts',(0.995976668043135,2.36833540947472,
7.2232660213906));
#110911=CARTESIAN_POINT('Ctrl Pts',(0.990540535864242,2.36147458185979,
7.18201430276513));
#110912=CARTESIAN_POINT('Ctrl Pts',(0.775652296,2.36069511,7.459783074));
#110913=CARTESIAN_POINT('Ctrl Pts',(1.181411227,2.42611337,7.41759312800001));
#110914=CARTESIAN_POINT('Ctrl Pts',(1.580200173,2.491440779,7.331641522));
#110915=CARTESIAN_POINT('Ctrl Pts',(0.985885713,2.36069511,7.182654757));
#110916=CARTESIAN_POINT('Ctrl Pts',(1.376570843,2.42611337,7.129029614));
#110917=CARTESIAN_POINT('Ctrl Pts',(1.759134602,2.491440779,7.033345253));
#110918=CARTESIAN_POINT('Origin',(-0.0353484116106306,2.41071388899553,
-0.196509256623171));
#110919=CARTESIAN_POINT('Ctrl Pts',(2.03084136166895,2.4959750823296,7.22041171789993));
#110920=CARTESIAN_POINT('Ctrl Pts',(2.04444397266669,2.4937079306648,7.21653036902814));
#110921=CARTESIAN_POINT('Ctrl Pts',(2.0580465836644,2.491440779,7.21264902015633));
#110922=CARTESIAN_POINT('Ctrl Pts',(2.45254058252075,2.425690334,7.10008468690785));
#110923=CARTESIAN_POINT('Ctrl Pts',(2.83240472203601,2.360702725,6.9451670333772));
#110924=CARTESIAN_POINT('Ctrl Pts',(1.73260569168895,2.4959750823296,7.03998049159346));
#110925=CARTESIAN_POINT('Ctrl Pts',(1.74587014684451,2.4937079306648,7.03666287229668));
#110926=CARTESIAN_POINT('Ctrl Pts',(1.759134602,2.491440779,7.033345253));
#110927=CARTESIAN_POINT('Ctrl Pts',(2.143821627,2.425690334,6.93712983500001));
#110928=CARTESIAN_POINT('Ctrl Pts',(2.515720358,2.360702725,6.79953315100001));
#110929=CARTESIAN_POINT('',(2.51130302647691,2.36147458139038,6.80116586227588));
#110930=CARTESIAN_POINT('Origin',(-0.037539604168903,2.55353595096111,-0.192746987546534));
#110931=CARTESIAN_POINT('Ctrl Pts',(2.59673753170465,2.40074633454041,7.03611783518101));
#110932=CARTESIAN_POINT('Ctrl Pts',(2.58244578398888,2.3945034693668,6.99693660543367));
#110933=CARTESIAN_POINT('Ctrl Pts',(2.56817213626816,2.38811405780995,6.95774812676184));
#110934=CARTESIAN_POINT('Ctrl Pts',(2.53969690108746,2.37503355114849,6.87944319142751));
#110935=CARTESIAN_POINT('Ctrl Pts',(2.52547997584348,2.36833541537222,6.84028456675752));
#110936=CARTESIAN_POINT('Ctrl Pts',(2.51130302489948,2.36147458172356,6.80116586364809));
#110937=CARTESIAN_POINT('Ctrl Pts',(2.361150828,2.36069511,7.118635176));
#110938=CARTESIAN_POINT('Ctrl Pts',(2.748353749,2.42611337,6.990205431));
#110939=CARTESIAN_POINT('Ctrl Pts',(3.119342177,2.491440779,6.820535491));
#110940=CARTESIAN_POINT('Ctrl Pts',(2.506894708,2.36069511,6.802791995));
#110941=CARTESIAN_POINT('Ctrl Pts',(2.876918016,2.42611337,6.666434823));
#110942=CARTESIAN_POINT('Ctrl Pts',(3.229968338,2.491440779,6.49074761));
#110943=CARTESIAN_POINT('Origin',(-0.0767657578313008,2.4107138892903,-0.184316315788779));
#110944=CARTESIAN_POINT('Ctrl Pts',(3.53553650424483,2.49597508246236,6.61503164336028));
#110945=CARTESIAN_POINT('Ctrl Pts',(3.54798671884754,2.49370793073122,6.60831687878963));
#110946=CARTESIAN_POINT('Ctrl Pts',(3.56043693345028,2.491440779,6.60160211421911));
#110947=CARTESIAN_POINT('Ctrl Pts',(3.92150987762511,2.425690334,6.40686492371389));
#110948=CARTESIAN_POINT('Ctrl Pts',(4.25919028771019,2.360702725,6.17390959719505));
#110949=CARTESIAN_POINT('Ctrl Pts',(3.20548603833938,2.49597508246235,6.50293065227997));
#110950=CARTESIAN_POINT('Ctrl Pts',(3.21772718816967,2.49370793073122,6.49683913113996));
#110951=CARTESIAN_POINT('Ctrl Pts',(3.229968338,2.491440779,6.49074761));
#110952=CARTESIAN_POINT('Ctrl Pts',(3.584978123,2.425690334,6.31408531600001));
#110953=CARTESIAN_POINT('Ctrl Pts',(3.918602849,2.360702725,6.099758332));
#110954=CARTESIAN_POINT('',(3.91463977674166,2.36147458139229,6.10230246674701));
#110955=CARTESIAN_POINT('Origin',(-0.0780968644945962,2.55353597351477,
-0.18017079869992));
#110956=CARTESIAN_POINT('Ctrl Pts',(4.04858459986332,2.40074633454433,6.31339549972611));
#110957=CARTESIAN_POINT('Ctrl Pts',(4.02620398823041,2.39450341615075,6.27820230870856));
#110958=CARTESIAN_POINT('Ctrl Pts',(4.00383978725195,2.38811403160265,6.24299860634402));
#110959=CARTESIAN_POINT('Ctrl Pts',(3.95919710097473,2.3750335425731,6.17264582572751));
#110960=CARTESIAN_POINT('Ctrl Pts',(3.93689462839103,2.36833541116663,6.13745895128617));
#110961=CARTESIAN_POINT('Ctrl Pts',(3.9146397755647,2.3614745817329,6.10230246879974));
#110962=CARTESIAN_POINT('Ctrl Pts',(3.836244571,2.36069511,6.444627809));
#110963=CARTESIAN_POINT('Ctrl Pts',(4.186786305,2.42611337,6.235963497));
#110964=CARTESIAN_POINT('Ctrl Pts',(4.512627207,2.491440779,5.99050879999999));
#110965=CARTESIAN_POINT('Ctrl Pts',(3.910684093,2.36069511,6.104838239));
#110966=CARTESIAN_POINT('Ctrl Pts',(4.2427437,2.42611337,5.89212495));
#110967=CARTESIAN_POINT('Ctrl Pts',(4.549772344,2.491440779,5.644649822));
#110968=CARTESIAN_POINT('Origin',(-0.114593353872106,2.41071384020386,-0.163504429967748));
#110969=CARTESIAN_POINT('Ctrl Pts',(4.87491388932696,2.49597508251598,5.70034004077986));
#110970=CARTESIAN_POINT('Ctrl Pts',(4.88562954905136,2.49370793075803,5.6911058354888));
#110971=CARTESIAN_POINT('Ctrl Pts',(4.89634520877575,2.491440779,5.68187163019773));
#110972=CARTESIAN_POINT('Ctrl Pts',(5.20711372828778,2.425690334,5.41406727834382));
#110973=CARTESIAN_POINT('Ctrl Pts',(5.48682085031788,2.360702725,5.11396701104611));
#110974=CARTESIAN_POINT('Ctrl Pts',(4.52848142063812,2.49597508251598,5.66181100249455));
#110975=CARTESIAN_POINT('Ctrl Pts',(4.53912688231906,2.49370793075803,5.65323041224728));
#110976=CARTESIAN_POINT('Ctrl Pts',(4.549772344,2.491440779,5.644649822));
#110977=CARTESIAN_POINT('Ctrl Pts',(4.858505026,2.425690334,5.395801184));
#110978=CARTESIAN_POINT('Ctrl Pts',(5.138255826,2.360702725,5.114765592));
#110979=CARTESIAN_POINT('',(5.13493232112417,2.36147458135829,5.11810219084302));
#110980=CARTESIAN_POINT('Origin',(-0.115002567746854,2.55353598996265,-0.159170189430652));
#110981=CARTESIAN_POINT('Ctrl Pts',(5.31112435157405,2.40074633451179,5.2954658080937));
#110982=CARTESIAN_POINT('Ctrl Pts',(5.2817017413302,2.39450346936203,5.26590683617229));
#110983=CARTESIAN_POINT('Ctrl Pts',(5.25229251438714,2.38811405780908,5.23633368521848));
#110984=CARTESIAN_POINT('Ctrl Pts',(5.19356970548814,2.37503355193669,5.17722249497532));
#110985=CARTESIAN_POINT('Ctrl Pts',(5.16422449208846,2.36833541577011,5.14765261981391));
#110986=CARTESIAN_POINT('Ctrl Pts',(5.13493232125685,2.36147458173208,5.11810219192745));
#110987=CARTESIAN_POINT('Ctrl Pts',(5.131959782,2.36069511,5.469276808));
#110988=CARTESIAN_POINT('Ctrl Pts',(5.429449386,2.42611337,5.190134841));
#110989=CARTESIAN_POINT('Ctrl Pts',(5.694906805,2.491440779,4.880372576));
#110990=CARTESIAN_POINT('Ctrl Pts',(5.131614236,2.36069511,5.121429033));
#110991=CARTESIAN_POINT('Ctrl Pts',(5.410183404,2.42611337,4.842305862));
#110992=CARTESIAN_POINT('Ctrl Pts',(5.65683405200001,2.491440779,4.534614483));
#110993=CARTESIAN_POINT('Origin',(-0.1470630375133,2.410713851561,-0.135047780565773));
#110994=CARTESIAN_POINT('Ctrl Pts',(5.98634572009426,2.49597508243042,4.51910687327443));
#110995=CARTESIAN_POINT('Ctrl Pts',(5.9948257723109,2.49370793071522,4.50778500869404));
#110996=CARTESIAN_POINT('Ctrl Pts',(6.00330582452749,2.491440779,4.4964631441136));
#110997=CARTESIAN_POINT('Ctrl Pts',(6.24923872929147,2.425690334,4.16811386365014));
#110998=CARTESIAN_POINT('Ctrl Pts',(6.45789376747328,2.360702725,3.81490101081275));
#110999=CARTESIAN_POINT('Ctrl Pts',(5.63973004538815,2.49597508243039,4.55595136341759));
#111000=CARTESIAN_POINT('Ctrl Pts',(5.64828204869408,2.49370793071524,4.54528292320879));
#111001=CARTESIAN_POINT('Ctrl Pts',(5.656834052,2.491440779,4.534614483));
#111002=CARTESIAN_POINT('Ctrl Pts',(5.904853635,2.425690334,4.225215387));
#111003=CARTESIAN_POINT('Ctrl Pts',(6.117649671,2.360702725,3.890612098));
#111004=CARTESIAN_POINT('',(6.11512113791658,2.36147458135708,3.89458514479899));
#111005=CARTESIAN_POINT('Origin',(-0.146530587764919,2.55353595661026,-0.130726585502198));
#111006=CARTESIAN_POINT('Ctrl Pts',(6.3253218314692,2.40074633450931,4.02992602048566));
#111007=CARTESIAN_POINT('Ctrl Pts',(6.29023280025013,2.39450346934649,4.00738311236295));
#111008=CARTESIAN_POINT('Ctrl Pts',(6.25515379150861,2.38811405781194,3.98482347979215));
#111009=CARTESIAN_POINT('Ctrl Pts',(6.18509674548874,2.37503355473301,3.93971795405276));
#111010=CARTESIAN_POINT('Ctrl Pts',(6.15008094986346,2.36833541717758,3.91714775456561));
#111011=CARTESIAN_POINT('Ctrl Pts',(6.11512113812636,2.36147458179299,3.89458514566824));
#111012=CARTESIAN_POINT('Ctrl Pts',(6.18771025700001,2.36069511,4.238188502));
#111013=CARTESIAN_POINT('Ctrl Pts',(6.418237448,2.42611337,3.901621248));
#111014=CARTESIAN_POINT('Ctrl Pts',(6.61089889,2.491440779,3.542035555));
#111015=CARTESIAN_POINT('Ctrl Pts',(6.1125958,2.36069511,3.898547497));
#111016=CARTESIAN_POINT('Ctrl Pts',(6.324648946,2.42611337,3.566065933));
#111017=CARTESIAN_POINT('Ctrl Pts',(6.499388487,2.491440779,3.21254561));
#111018=CARTESIAN_POINT('Origin',(-0.172655948842431,2.41071392620491,-0.100276158910808));
#111019=CARTESIAN_POINT('Ctrl Pts',(6.81786267752745,2.49597508234954,3.12656529063839));
#111020=CARTESIAN_POINT('Ctrl Pts',(6.82371060452681,2.49370793067477,3.11368516462101));
#111021=CARTESIAN_POINT('Ctrl Pts',(6.82955853152627,2.491440779,3.10080503860365));
#111022=CARTESIAN_POINT('Ctrl Pts',(6.99915627252464,2.425690334,2.72726407673456));
#111023=CARTESIAN_POINT('Ctrl Pts',(7.12700274970052,2.360702725,2.33745447875269));
#111024=CARTESIAN_POINT('Ctrl Pts',(6.4872711613576,2.49597508234954,3.23706050140318));
#111025=CARTESIAN_POINT('Ctrl Pts',(6.49332982417881,2.49370793067477,3.22480305570161));
#111026=CARTESIAN_POINT('Ctrl Pts',(6.499388487,2.491440779,3.21254561));
#111027=CARTESIAN_POINT('Ctrl Pts',(6.67509785,2.425690334,2.857063214));
#111028=CARTESIAN_POINT('Ctrl Pts',(6.810989017,2.360702725,2.484537907));
#111029=CARTESIAN_POINT('',(6.80937368675615,2.36147458134305,2.48896162520109));
#111030=CARTESIAN_POINT('Origin',(-0.171207237284685,2.55353595066915,-0.0961705711236122));
#111031=CARTESIAN_POINT('Ctrl Pts',(7.04375429273431,2.40074633454334,2.57595137079213));
#111032=CARTESIAN_POINT('Ctrl Pts',(7.00463956477323,2.39450346938452,2.56147860793005));
#111033=CARTESIAN_POINT('Ctrl Pts',(6.96553102956395,2.3881140578281,2.54698735705099));
#111034=CARTESIAN_POINT('Ctrl Pts',(6.88741540060877,2.37503353410922,2.51799652197757));
#111035=CARTESIAN_POINT('Ctrl Pts',(6.84836639463092,2.36833540700786,2.50348138654198));
#111036=CARTESIAN_POINT('Ctrl Pts',(6.80937368765278,2.36147458174416,2.48896162659278));
#111037=CARTESIAN_POINT('Ctrl Pts',(6.954130278,2.36069511,2.808927212));
#111038=CARTESIAN_POINT('Ctrl Pts',(7.10691586000001,2.42611337,2.430672182));
#111039=CARTESIAN_POINT('Ctrl Pts',(7.21777269,2.491440779,2.038076888));
#111040=CARTESIAN_POINT('Ctrl Pts',(6.807759179,2.36069511,2.493374213));
#111041=CARTESIAN_POINT('Ctrl Pts',(6.943380931,2.42611337,2.123080726));
#111042=CARTESIAN_POINT('Ctrl Pts',(7.03803874,2.491440779,1.740261674));
#111043=CARTESIAN_POINT('Origin',(-0.190175948612856,2.41071383979128,-0.0608158988614296));
#111044=CARTESIAN_POINT('Ctrl Pts',(7.33058395393016,2.49597508242676,1.58782899156932));
#111045=CARTESIAN_POINT('Ctrl Pts',(7.33352631333063,2.49370793071342,1.57399286405882));
#111046=CARTESIAN_POINT('Ctrl Pts',(7.33646867273096,2.491440779,1.56015673654826));
#111047=CARTESIAN_POINT('Ctrl Pts',(7.42180104761325,2.425690334,1.1588904536096));
#111048=CARTESIAN_POINT('Ctrl Pts',(7.46286100361699,2.360702725,0.750711174245291));
#111049=CARTESIAN_POINT('Ctrl Pts',(7.03147468762232,2.4959750824268,1.76680828812868));
#111050=CARTESIAN_POINT('Ctrl Pts',(7.03475671381116,2.4937079307134,1.75353498106434));
#111051=CARTESIAN_POINT('Ctrl Pts',(7.03803874,2.491440779,1.740261674));
#111052=CARTESIAN_POINT('Ctrl Pts',(7.133221908,2.425690334,1.35531794));
#111053=CARTESIAN_POINT('Ctrl Pts',(7.185854086,2.360702725,0.962289484));
#111054=CARTESIAN_POINT('',(7.18522749011262,2.36147458135454,0.966957026736748));
#111055=CARTESIAN_POINT('Origin',(-0.187878458689477,2.55353595748085,-0.0571176862103746));
#111056=CARTESIAN_POINT('Ctrl Pts',(7.43282863154981,2.40074633450367,1.00152809855962));
#111057=CARTESIAN_POINT('Ctrl Pts',(7.39151716795935,2.3945034693615,0.995802211064734));
#111058=CARTESIAN_POINT('Ctrl Pts',(7.35020777802992,2.38811405783215,0.9900569365596));
#111059=CARTESIAN_POINT('Ctrl Pts',(7.26768633535209,2.37503354348097,0.978536450388198));
#111060=CARTESIAN_POINT('Ctrl Pts',(7.22642991707173,2.36833541165497,0.972755048399386));
#111061=CARTESIAN_POINT('Ctrl Pts',(7.18522749108296,2.36147458180083,0.966957027865269));
#111062=CARTESIAN_POINT('Ctrl Pts',(7.395382895,2.36069511,1.248323608));
#111063=CARTESIAN_POINT('Ctrl Pts',(7.463282786,2.42611337,0.846067586));
#111064=CARTESIAN_POINT('Ctrl Pts',(7.487151461,2.491440779,0.43882001));
#111065=CARTESIAN_POINT('Ctrl Pts',(7.184599304,2.36069511,0.971613522));
#111066=CARTESIAN_POINT('Ctrl Pts',(7.237448142,2.42611337,0.580822623));
#111067=CARTESIAN_POINT('Ctrl Pts',(7.247598124,2.491440779,0.186605037));
#111068=CARTESIAN_POINT('Origin',(-0.198803195775803,2.41071385645573,-0.0185118389587539));
#111069=CARTESIAN_POINT('Ctrl Pts',(7.50053527191827,2.4959750822797,-0.0251524287664814));
#111070=CARTESIAN_POINT('Ctrl Pts',(7.50043448216075,2.49370793063989,-0.0392975951575152));
#111071=CARTESIAN_POINT('Ctrl Pts',(7.50033369240322,2.491440779,-0.0534427615485497));
#111072=CARTESIAN_POINT('Ctrl Pts',(7.49741065395632,2.425690334,-0.463671600436942));
#111073=CARTESIAN_POINT('Ctrl Pts',(7.4497641723792,2.360702725,-0.87113455191811));
#111074=CARTESIAN_POINT('Ctrl Pts',(7.24689427289999,2.4959750822797,0.213942082389185));
#111075=CARTESIAN_POINT('Ctrl Pts',(7.24724619844996,2.49370793063989,0.200273559694589));
#111076=CARTESIAN_POINT('Ctrl Pts',(7.247598124,2.491440779,0.186605037));
#111077=CARTESIAN_POINT('Ctrl Pts',(7.257804438,2.425690334,-0.209800494));
#111078=CARTESIAN_POINT('Ctrl Pts',(7.22471660500001,2.360702725,-0.604954526));
#111079=CARTESIAN_POINT('',(7.2251080422661,2.36147458140569,-0.600261409189046));
#111080=CARTESIAN_POINT('Origin',(-0.195764717093502,2.55353597250716,-0.0153939945248779));
#111081=CARTESIAN_POINT('Ctrl Pts',(7.47435216496847,2.4007463345685,-0.619725515399625));
#111082=CARTESIAN_POINT('Ctrl Pts',(7.43277529405746,2.39450341687222,-0.616436763641023));
#111083=CARTESIAN_POINT('Ctrl Pts',(7.39119681606624,2.38811403197589,-0.613167433927704));
#111084=CARTESIAN_POINT('Ctrl Pts',(7.30812833342854,2.37503355199203,-0.606678923770133));
#111085=CARTESIAN_POINT('Ctrl Pts',(7.26659360799277,2.36833541581745,-0.60345624713839));
#111086=CARTESIAN_POINT('Ctrl Pts',(7.22510804348048,2.36147458176016,-0.60026140759842));
#111087=CARTESIAN_POINT('Ctrl Pts',(7.490835629,2.36069511,-0.370650221));
#111088=CARTESIAN_POINT('Ctrl Pts',(7.470674903,2.42611337,-0.77809819));
#111089=CARTESIAN_POINT('Ctrl Pts',(7.406439351,2.491440779,-1.180955603));
#111090=CARTESIAN_POINT('Ctrl Pts',(7.225495552,2.36069511,-0.595578738));
#111091=CARTESIAN_POINT('Ctrl Pts',(7.19310032100001,2.42611337,-0.988594101));
#111092=CARTESIAN_POINT('Ctrl Pts',(7.118267874,2.491440779,-1.375777044));
#111093=CARTESIAN_POINT('Origin',(-0.198134895535887,2.41071388758876,0.0246577965306941));
#111094=CARTESIAN_POINT('Ctrl Pts',(7.31976989665382,2.49597508238335,-1.63695774767015));
#111095=CARTESIAN_POINT('Ctrl Pts',(7.31663067059766,2.49370793069171,-1.65075054141746));
#111096=CARTESIAN_POINT('Ctrl Pts',(7.31349144454157,2.491440779,-1.66454333516476));
#111097=CARTESIAN_POINT('Ctrl Pts',(7.22244967133344,2.425690334,-2.06455288459223));
#111098=CARTESIAN_POINT('Ctrl Pts',(7.08832464740652,2.360702725,-2.45224699364326));
#111099=CARTESIAN_POINT('Ctrl Pts',(7.12345713531641,2.49597508238334,-1.34892781573121));
#111100=CARTESIAN_POINT('Ctrl Pts',(7.12086250465821,2.49370793069171,-1.36235242986561));
#111101=CARTESIAN_POINT('Ctrl Pts',(7.118267874,2.491440779,-1.375777044));
#111102=CARTESIAN_POINT('Ctrl Pts',(7.043020099,2.425690334,-1.76510889));
#111103=CARTESIAN_POINT('Ctrl Pts',(6.925759405,2.360702725,-2.143911534));
#111104=CARTESIAN_POINT('',(6.92715057170216,2.36147458141132,-2.13941228764283));
#111105=CARTESIAN_POINT('Origin',(-0.19449701381967,2.55353595734725,0.0270495149301808));
#111106=CARTESIAN_POINT('Ctrl Pts',(7.1663832978545,2.4007463345425,-2.21200145241878));
#111107=CARTESIAN_POINT('Ctrl Pts',(7.12648545170843,2.39450341625723,-2.19985179039366));
#111108=CARTESIAN_POINT('Ctrl Pts',(7.08658186676122,2.38811403167542,-2.18772075264125));
#111109=CARTESIAN_POINT('Ctrl Pts',(7.0068502209734,2.37503353593916,-2.16352664264567));
#111110=CARTESIAN_POINT('Ctrl Pts',(6.96697938663502,2.36833540792811,-2.15145058793241));
#111111=CARTESIAN_POINT('Ctrl Pts',(6.92715057360104,2.36147458177965,-2.13941228563727));
#111112=CARTESIAN_POINT('Ctrl Pts',(7.236025213,2.36069511,-1.972292858));
#111113=CARTESIAN_POINT('Ctrl Pts',(7.128746565,2.42611337,-2.365880959));
#111114=CARTESIAN_POINT('Ctrl Pts',(6.979410369,2.491440779,-2.745511045));
#111115=CARTESIAN_POINT('Ctrl Pts',(6.928535658,2.36069511,-2.134922397));
#111116=CARTESIAN_POINT('Ctrl Pts',(6.812411124,2.42611337,-2.511785262));
#111117=CARTESIAN_POINT('Ctrl Pts',(6.65609533,2.491440779,-2.873829319));
#111118=CARTESIAN_POINT('Origin',(-0.188201868405449,2.41071387521461,0.0666744331180874));
#111119=CARTESIAN_POINT('Ctrl Pts',(6.79674021710689,2.49597508252471,-3.17222074089898));
#111120=CARTESIAN_POINT('Ctrl Pts',(6.79070934129096,2.49370793076239,-3.18501622638997));
#111121=CARTESIAN_POINT('Ctrl Pts',(6.78467846547508,2.491440779,-3.19781171188092));
#111122=CARTESIAN_POINT('Ctrl Pts',(6.60977496972601,2.425690334,-3.56889797041118));
#111123=CARTESIAN_POINT('Ctrl Pts',(6.3954429407611,2.360702725,-3.91869509163868));
#111124=CARTESIAN_POINT('Ctrl Pts',(6.66693506001777,2.49597508252471,-2.84872334773867));
#111125=CARTESIAN_POINT('Ctrl Pts',(6.6615151950089,2.49370793076239,-2.86127633336936));
#111126=CARTESIAN_POINT('Ctrl Pts',(6.65609533,2.491440779,-2.873829319));
#111127=CARTESIAN_POINT('Ctrl Pts',(6.498911968,2.425690334,-3.237882756));
#111128=CARTESIAN_POINT('Ctrl Pts',(6.302961392,2.360702725,-3.582621622));
#111129=CARTESIAN_POINT('',(6.30528724043917,2.36147458137357,-3.57852662396335));
#111130=CARTESIAN_POINT('Origin',(-0.184134812498761,2.55353595767753,0.0682281691905767));
#111131=CARTESIAN_POINT('Ctrl Pts',(6.52332231319455,2.40074633455067,-3.70084665970845));
#111132=CARTESIAN_POINT('Ctrl Pts',(6.48696938400318,2.3945034693982,-3.68040436650925));
#111133=CARTESIAN_POINT('Ctrl Pts',(6.45060637304175,2.38811405784751,-3.65997876206446));
#111134=CARTESIAN_POINT('Ctrl Pts',(6.37793976229787,2.37503355046822,-3.61921031372038));
#111135=CARTESIAN_POINT('Ctrl Pts',(6.34159703770279,2.36833541508829,-3.59884551561224));
#111136=CARTESIAN_POINT('Ctrl Pts',(6.30528724136624,2.3614745818094,-3.57852662358162));
#111137=CARTESIAN_POINT('Ctrl Pts',(6.64286630100001,2.36069511,-3.481713272));
#111138=CARTESIAN_POINT('Ctrl Pts',(6.45348596100001,2.42611337,-3.843037764));
#111139=CARTESIAN_POINT('Ctrl Pts',(6.226031915,2.491440779,-4.181689442));
#111140=CARTESIAN_POINT('Ctrl Pts',(6.307605137,2.36069511,-3.574439458));
#111141=CARTESIAN_POINT('Ctrl Pts',(6.11318115400001,2.42611337,-3.917528137));
#111142=CARTESIAN_POINT('Ctrl Pts',(5.882691166,2.491440779,-4.23750453));
#111143=CARTESIAN_POINT('Origin',(-0.169468734258499,2.41071389137068,0.105573437157334));
#111144=CARTESIAN_POINT('Ctrl Pts',(5.95590251870123,2.49597508252968,-4.55915421965815));
#111145=CARTESIAN_POINT('Ctrl Pts',(5.94726199025258,2.49370793076488,-4.57035409378245));
#111146=CARTESIAN_POINT('Ctrl Pts',(5.93862146180392,2.491440779,-4.58155396790664));
#111147=CARTESIAN_POINT('Ctrl Pts',(5.6880345362443,2.425690334,-4.90636535416808));
#111148=CARTESIAN_POINT('Ctrl Pts',(5.40351742966767,2.360702725,-5.20190936238205));
#111149=CARTESIAN_POINT('Ctrl Pts',(5.89867451079924,2.49597508252968,-4.21531574393402));
#111150=CARTESIAN_POINT('Ctrl Pts',(5.8906828383996,2.49370793076488,-4.22641013696702));
#111151=CARTESIAN_POINT('Ctrl Pts',(5.882691166,2.491440779,-4.23750453));
#111152=CARTESIAN_POINT('Ctrl Pts',(5.650921937,2.425690334,-4.559256823));
#111153=CARTESIAN_POINT('Ctrl Pts',(5.385443911,2.360702725,-4.853812304));
#111154=CARTESIAN_POINT('',(5.38859568422889,2.36147458137419,-4.8503130343453));
#111155=CARTESIAN_POINT('Origin',(-0.165164502110791,2.55353553498122,0.10621801655163));
#111156=CARTESIAN_POINT('Ctrl Pts',(5.57523802689835,2.4007463345603,-5.0166443907419));
#111157=CARTESIAN_POINT('Ctrl Pts',(5.54412949788782,2.39450346940797,-4.98886522176393));
#111158=CARTESIAN_POINT('Ctrl Pts',(5.5130075352218,2.38811405785102,-4.96110018408175));
#111159=CARTESIAN_POINT('Ctrl Pts',(5.45080379357579,2.37503354047566,-4.90566366378113));
#111160=CARTESIAN_POINT('Ctrl Pts',(5.41968859661357,2.3683354101439,-4.87796239430515));
#111161=CARTESIAN_POINT('Ctrl Pts',(5.3885956866165,2.3614745817378,-4.85031303352163));
#111162=CARTESIAN_POINT('Ctrl Pts',(5.739094344,2.36069511,-4.828332643));
#111163=CARTESIAN_POINT('Ctrl Pts',(5.476467525,2.42611337,-5.140498395));
#111164=CARTESIAN_POINT('Ctrl Pts',(5.181531129,2.491440779,-5.42233668900001));
#111165=CARTESIAN_POINT('Ctrl Pts',(5.39173801,2.36069511,-4.846819703));
#111166=CARTESIAN_POINT('Ctrl Pts',(5.128105628,2.42611337,-5.14009175));
#111167=CARTESIAN_POINT('Ctrl Pts',(4.834218902,2.491440779,-5.403038739));
#111168=CARTESIAN_POINT('Origin',(-0.142811494539211,2.41071387228298,0.139535953330484));
#111169=CARTESIAN_POINT('Ctrl Pts',(4.83657343703978,2.4959750822612,-5.73290671538372));
#111170=CARTESIAN_POINT('Ctrl Pts',(4.82572727809061,2.49370793063064,-5.74198728391551));
#111171=CARTESIAN_POINT('Ctrl Pts',(4.81488111914144,2.491440779,-5.75106785244731));
#111172=CARTESIAN_POINT('Ctrl Pts',(4.50032792921937,2.425690334,-6.01441654679815));
#111173=CARTESIAN_POINT('Ctrl Pts',(4.15892944980332,2.360702725,-6.24188813278773));
#111174=CARTESIAN_POINT('Ctrl Pts',(4.85459849703071,2.4959750822612,-5.38480466216928));
#111175=CARTESIAN_POINT('Ctrl Pts',(4.84440869951533,2.49370793063064,-5.39392170058464));
#111176=CARTESIAN_POINT('Ctrl Pts',(4.83421890200001,2.491440779,-5.403038739));
#111177=CARTESIAN_POINT('Ctrl Pts',(4.538701076,2.425690334,-5.667445109));
#111178=CARTESIAN_POINT('Ctrl Pts',(4.216109057,2.360702725,-5.898044118));
#111179=CARTESIAN_POINT('',(4.21993938413277,2.36147458134235,-5.89530419657684));
#111180=CARTESIAN_POINT('Origin',(-0.138467891967822,2.55353595480635,0.13923832245939));
#111181=CARTESIAN_POINT('Ctrl Pts',(4.36646180685913,2.40074633452991,-6.09786940580669));
#111182=CARTESIAN_POINT('Ctrl Pts',(4.34205207570985,2.39450341760044,-6.06405200370533));
#111183=CARTESIAN_POINT('Ctrl Pts',(4.3176264968511,2.38811403232265,-6.03024594398858));
#111184=CARTESIAN_POINT('Ctrl Pts',(4.26879433193897,2.3750335349705,-5.96273363615639));
#111185=CARTESIAN_POINT('Ctrl Pts',(4.24436155596373,2.3683354074509,-5.9289911744189));
#111186=CARTESIAN_POINT('Ctrl Pts',(4.21993938576903,2.36147458177666,-5.89530419695903));
#111187=CARTESIAN_POINT('Ctrl Pts',(4.566968713,2.36069511,-5.94918454700001));
#111188=CARTESIAN_POINT('Ctrl Pts',(4.243375555,2.42611337,-6.19759503400001));
#111189=CARTESIAN_POINT('Ctrl Pts',(3.894747705,2.491440779,-6.409441498));
#111190=CARTESIAN_POINT('Ctrl Pts',(4.223759206,2.36069511,-5.892568045));
#111191=CARTESIAN_POINT('Ctrl Pts',(3.903245582,2.42611337,-6.122310386));
#111192=CARTESIAN_POINT('Ctrl Pts',(3.559703934,2.491440779,-6.315932861));
#111193=CARTESIAN_POINT('Origin',(-0.109476389224066,2.41071387441741,0.166973696340317));
#111194=CARTESIAN_POINT('Ctrl Pts',(3.49109155737623,2.49597508229257,-6.63859486236934));
#111195=CARTESIAN_POINT('Ctrl Pts',(3.47854692169554,2.49370793064629,-6.64513152876386));
#111196=CARTESIAN_POINT('Ctrl Pts',(3.46600228601477,2.491440779,-6.65166819515836));
#111197=CARTESIAN_POINT('Ctrl Pts',(3.10219099014338,2.425690334,-6.84124030647186));
#111198=CARTESIAN_POINT('Ctrl Pts',(2.71987455125237,2.360702725,-6.99000315145689));
#111199=CARTESIAN_POINT('Ctrl Pts',(3.58352685309772,2.49597508229257,-6.30250609716514));
#111200=CARTESIAN_POINT('Ctrl Pts',(3.57161539354887,2.49370793064629,-6.30921947908256));
#111201=CARTESIAN_POINT('Ctrl Pts',(3.559703934,2.491440779,-6.315932861));
#111202=CARTESIAN_POINT('Ctrl Pts',(3.214255597,2.425690334,-6.51062996));
#111203=CARTESIAN_POINT('Ctrl Pts',(2.84963363,2.360702725,-6.666489944));
#111204=CARTESIAN_POINT('',(2.85396340807876,2.36147458133375,-6.66463748776735));
#111205=CARTESIAN_POINT('Origin',(-0.105298459875244,2.55353594867096,0.165749496562412));
#111206=CARTESIAN_POINT('Ctrl Pts',(2.95351468598881,2.4007463345525,-6.893964824483));
#111207=CARTESIAN_POINT('Ctrl Pts',(2.93694538232913,2.39450341751036,-6.8556906831616));
#111208=CARTESIAN_POINT('Ctrl Pts',(2.92035816359941,2.38811403227426,-6.8174242132272));
#111209=CARTESIAN_POINT('Ctrl Pts',(2.88718082282725,2.375033536788,-6.74099284469345));
#111210=CARTESIAN_POINT('Ctrl Pts',(2.87057290089408,2.36833540831626,-6.70278693262186));
#111211=CARTESIAN_POINT('Ctrl Pts',(2.85396340960552,2.36147458173546,-6.66463748835739));
#111212=CARTESIAN_POINT('Ctrl Pts',(3.181296702,2.36069511,-6.79185919300001));
#111213=CARTESIAN_POINT('Ctrl Pts',(2.81186806,2.42611337,-6.964899017));
#111214=CARTESIAN_POINT('Ctrl Pts',(2.425850208,2.491440779,-7.096847946));
#111215=CARTESIAN_POINT('Ctrl Pts',(2.858282117,2.36069511,-6.662786455));
#111216=CARTESIAN_POINT('Ctrl Pts',(2.49587411,2.42611337,-6.81825659200001));
#111217=CARTESIAN_POINT('Ctrl Pts',(2.118741167,2.491440779,-6.933500982));
#111218=CARTESIAN_POINT('Origin',(-0.071022573616687,2.41071391683862,0.186604418640867));
#111219=CARTESIAN_POINT('Ctrl Pts',(1.98237012011077,2.49597508279149,-7.23386969147354));
#111220=CARTESIAN_POINT('Ctrl Pts',(1.96871357948591,2.49370793089575,-7.23755680881284));
#111221=CARTESIAN_POINT('Ctrl Pts',(1.95505703886105,2.491440779,-7.24124392615215));
#111222=CARTESIAN_POINT('Ctrl Pts',(1.55899904868913,2.425690334,-7.34817527304667));
#111223=CARTESIAN_POINT('Ctrl Pts',(1.15364134058453,2.360702725,-7.41127339159409));
#111224=CARTESIAN_POINT('Ctrl Pts',(2.14489347970249,2.49597508279145,-6.9255093509647));
#111225=CARTESIAN_POINT('Ctrl Pts',(2.13181732335125,2.49370793089577,-6.92950516648233));
#111226=CARTESIAN_POINT('Ctrl Pts',(2.118741167,2.491440779,-6.933500982));
#111227=CARTESIAN_POINT('Ctrl Pts',(1.739515099,2.425690334,-7.04938499));
#111228=CARTESIAN_POINT('Ctrl Pts',(1.349912501,2.360702725,-7.12321811));
#111229=CARTESIAN_POINT('',(1.35453927523772,2.36147458134696,-7.12233973723395));
#111230=CARTESIAN_POINT('Origin',(-0.0672054225599605,2.55353596763685,
0.184510496211542));
#111231=CARTESIAN_POINT('Ctrl Pts',(1.40246450071486,2.40074633455926,-7.36770611019184));
#111232=CARTESIAN_POINT('Ctrl Pts',(1.39451038722834,2.39450341760035,-7.32676488706728));
#111233=CARTESIAN_POINT('Ctrl Pts',(1.38653712826532,2.38811403233655,-7.28582730402155));
#111234=CARTESIAN_POINT('Ctrl Pts',(1.37056594056082,2.37503353713036,-7.20405071257824));
#111235=CARTESIAN_POINT('Ctrl Pts',(1.36255944421315,2.36833540852492,-7.16316782030079));
#111236=CARTESIAN_POINT('Ctrl Pts',(1.35453927636171,2.36147458179984,-7.12233973828936));
#111237=CARTESIAN_POINT('Ctrl Pts',(1.646870792,2.36069511,-7.316954052));
#111238=CARTESIAN_POINT('Ctrl Pts',(1.24888074,2.42611337,-7.40653206300001));
#111239=CARTESIAN_POINT('Ctrl Pts',(0.843522651,2.491440779,-7.45241367199999));
#111240=CARTESIAN_POINT('Ctrl Pts',(1.359154932,2.36069511,-7.121460375));
#111241=CARTESIAN_POINT('Ctrl Pts',(0.971798339000001,2.42611337,-7.195388698));
#111242=CARTESIAN_POINT('Ctrl Pts',(0.578708417,2.491440779,-7.226866303));
#111243=CARTESIAN_POINT('Origin',(-0.0292476493498572,2.4107139102224,0.197509355480732));
#111244=CARTESIAN_POINT('Ctrl Pts',(0.363937711287557,2.49319894677753,
-7.49137623344886));
#111245=CARTESIAN_POINT('Ctrl Pts',(0.358459121765824,2.49231986288877,
-7.49163435721352));
#111246=CARTESIAN_POINT('Ctrl Pts',(0.352980532244091,2.491440779,-7.49189248097817));
#111247=CARTESIAN_POINT('Ctrl Pts',(-0.0567866169785492,2.425690334,-7.51119866166007));
#111248=CARTESIAN_POINT('Ctrl Pts',(-0.466215022234156,2.360702725,-7.48569914995376));
#111249=CARTESIAN_POINT('Ctrl Pts',(0.589277985104296,2.49319894677753,
-7.22601991980783));
#111250=CARTESIAN_POINT('Ctrl Pts',(0.583993201052148,2.49231986288877,
-7.22644311140391));
#111251=CARTESIAN_POINT('Ctrl Pts',(0.578708417,2.491440779,-7.226866303));
#111252=CARTESIAN_POINT('Ctrl Pts',(0.183436808,2.425690334,-7.258518613));
#111253=CARTESIAN_POINT('Ctrl Pts',(-0.212929036,2.360702725,-7.246872513));
#111254=CARTESIAN_POINT('',(-0.208221609147027,2.36147458135266,-7.24700929638663));
#111255=CARTESIAN_POINT('Origin',(-0.0259698947458284,2.55353597210639,
0.194643709376892));
#111256=CARTESIAN_POINT('Ctrl Pts',(-0.214163364830837,2.40074633010132,
-7.49694161690444));
#111257=CARTESIAN_POINT('Ctrl Pts',(-0.213130371432346,2.39450346485659,
-7.4552480234001));
#111258=CARTESIAN_POINT('Ctrl Pts',(-0.212116845861083,2.38811405782144,
-7.41355336951517));
#111259=CARTESIAN_POINT('Ctrl Pts',(-0.210135085308225,2.37503355527668,
-7.33025528930787));
#111260=CARTESIAN_POINT('Ctrl Pts',(-0.209165779495856,2.36833541741468,
-7.28860699457912));
#111261=CARTESIAN_POINT('Ctrl Pts',(-0.208221608534118,2.3614745817406,
-7.2470092971132));
#111262=CARTESIAN_POINT('Ctrl Pts',(0.035439035,2.36069511,-7.499916271));
#111263=CARTESIAN_POINT('Ctrl Pts',(-0.372502856,2.42611337,-7.50184390200001));
#111264=CARTESIAN_POINT('Ctrl Pts',(-0.778247087,2.491440779,-7.459512817));
#111265=CARTESIAN_POINT('Ctrl Pts',(-0.203524827,2.36069511,-7.24714272300001));
#111266=CARTESIAN_POINT('Ctrl Pts',(-0.597717642,2.42611337,-7.236072426));
#111267=CARTESIAN_POINT('Ctrl Pts',(-0.988384095,2.491440779,-7.182311389));
#111268=CARTESIAN_POINT('Origin',(0.0138950876763513,2.41071430159107,0.199181670296006));
#111269=CARTESIAN_POINT('Ctrl Pts',(-1.2382726553927,2.49597508222491,-7.39765792981161));
#111270=CARTESIAN_POINT('Ctrl Pts',(-1.25221517461467,2.49370793061246,
-7.39527003456471));
#111271=CARTESIAN_POINT('Ctrl Pts',(-1.26615769383664,2.491440779,-7.39288213931789));
#111272=CARTESIAN_POINT('Ctrl Pts',(-1.67050949731884,2.425690334,-7.32362996657868));
#111273=CARTESIAN_POINT('Ctrl Pts',(-2.06489640117708,2.360702725,-7.21069098516172));
#111274=CARTESIAN_POINT('Ctrl Pts',(-0.961293303489874,2.49597508222487,
-7.18603945174254));
#111275=CARTESIAN_POINT('Ctrl Pts',(-0.974838699244942,2.49370793061248,
-7.18417542037124));
#111276=CARTESIAN_POINT('Ctrl Pts',(-0.988384094999999,2.491440779,-7.182311389));
#111277=CARTESIAN_POINT('Ctrl Pts',(-1.381218784,2.425690334,-7.128251973));
#111278=CARTESIAN_POINT('Ctrl Pts',(-1.765814248,2.360702725,-7.031671213));
#111279=CARTESIAN_POINT('',(-1.76124628360346,2.36147458140683,-7.03281675504062));
#111280=CARTESIAN_POINT('Origin',(0.0164799599871354,2.55353599730958,0.195676067966756));
#111281=CARTESIAN_POINT('Ctrl Pts',(-1.82077719099447,2.40074633449545,
-7.27562852393234));
#111282=CARTESIAN_POINT('Ctrl Pts',(-1.81080545823754,2.39450346933559,
-7.23513176665407));
#111283=CARTESIAN_POINT('Ctrl Pts',(-1.8008525031392,2.38811405780701,-7.1946297599833));
#111284=CARTESIAN_POINT('Ctrl Pts',(-1.78101041491868,2.37503353213395,
-7.11370501954481));
#111285=CARTESIAN_POINT('Ctrl Pts',(-1.77111063743132,2.36833540606227,
-7.07323888724965));
#111286=CARTESIAN_POINT('Ctrl Pts',(-1.76124628168249,2.36147458179985,
-7.03281675696655));
#111287=CARTESIAN_POINT('Ctrl Pts',(-1.577649813,2.36069511,-7.332190741));
#111288=CARTESIAN_POINT('Ctrl Pts',(-1.976468632,2.42611337,-7.24637785700001));
#111289=CARTESIAN_POINT('Ctrl Pts',(-2.363626857,2.491440779,-7.11781343400001));
#111290=CARTESIAN_POINT('Ctrl Pts',(-1.756687991,2.36069511,-7.033956732));
#111291=CARTESIAN_POINT('Ctrl Pts',(-2.13928501,2.42611337,-6.93840544900001));
#111292=CARTESIAN_POINT('Ctrl Pts',(-2.509260865,2.491440779,-6.801919576));
#111293=CARTESIAN_POINT('Origin',(0.0563876163794358,2.41071387880783,0.191535565088941));
#111294=CARTESIAN_POINT('Ctrl Pts',(-2.7996003098369,2.49597508240935,-6.95851278037652));
#111295=CARTESIAN_POINT('Ctrl Pts',(-2.81270353432863,2.49370793070468,
-6.95318348310568));
#111296=CARTESIAN_POINT('Ctrl Pts',(-2.82580675882035,2.491440779,-6.94785418583485));
#111297=CARTESIAN_POINT('Ctrl Pts',(-3.20581787121601,2.425690334,-6.79329740590194));
#111298=CARTESIAN_POINT('Ctrl Pts',(-3.56670568702239,2.360702725,-6.5982173485554));
#111299=CARTESIAN_POINT('Ctrl Pts',(-2.48360486337345,2.49597508240936,
-6.81138419847442));
#111300=CARTESIAN_POINT('Ctrl Pts',(-2.49643286418676,2.49370793070468,
-6.8066518872372));
#111301=CARTESIAN_POINT('Ctrl Pts',(-2.509260865,2.491440779,-6.801919576));
#111302=CARTESIAN_POINT('Ctrl Pts',(-2.881290121,2.425690334,-6.664676193));
#111303=CARTESIAN_POINT('Ctrl Pts',(-3.236131948,2.360702725,-6.487676781));
#111304=CARTESIAN_POINT('',(-3.23191703699043,2.36147458135554,-6.48977751941193));
#111305=CARTESIAN_POINT('Origin',(0.058159215223072,2.55353598666095,0.187558505738186));
#111306=CARTESIAN_POINT('Ctrl Pts',(-3.34225349900583,2.40074633454303,
-6.7141150980915));
#111307=CARTESIAN_POINT('Ctrl Pts',(-3.32380929400625,2.39450346938553,
-6.67670876023693));
#111308=CARTESIAN_POINT('Ctrl Pts',(-3.30538229912372,2.38811405783145,
-6.63929325890826));
#111309=CARTESIAN_POINT('Ctrl Pts',(-3.26860772365964,2.37503354743692,
-6.56452604360058));
#111310=CARTESIAN_POINT('Ctrl Pts',(-3.2502403522527,2.36833541359946,-6.52713410004322));
#111311=CARTESIAN_POINT('Ctrl Pts',(-3.23191703633811,2.36147458180118,
-6.48977752054085));
#111312=CARTESIAN_POINT('Ctrl Pts',(-3.116969508,2.36069511,-6.821620122));
#111313=CARTESIAN_POINT('Ctrl Pts',(-3.488016932,2.42611337,-6.652079238));
#111314=CARTESIAN_POINT('Ctrl Pts',(-3.838486062,2.491440779,-6.443293005));
#111315=CARTESIAN_POINT('Ctrl Pts',(-3.227710377,2.36069511,-6.491870741));
#111316=CARTESIAN_POINT('Ctrl Pts',(-3.580821789,2.42611337,-6.316306345));
#111317=CARTESIAN_POINT('Ctrl Pts',(-3.912807385,2.491440779,-6.103477563));
#111318=CARTESIAN_POINT('Origin',(0.0962436524464921,2.41071388612422,0.174935665357462));
#111319=CARTESIAN_POINT('Ctrl Pts',(-4.23002176612037,2.49597508244881,
-6.19399530803162));
#111320=CARTESIAN_POINT('Ctrl Pts',(-4.2416730032187,2.49370793072441,-6.18597380075739));
#111321=CARTESIAN_POINT('Ctrl Pts',(-4.25332424031696,2.491440779,-6.17795229348326));
#111322=CARTESIAN_POINT('Ctrl Pts',(-4.59122576484367,2.425690334,-5.94531780891545));
#111323=CARTESIAN_POINT('Ctrl Pts',(-4.90173977726586,2.360702725,-5.67721840209496));
#111324=CARTESIAN_POINT('Ctrl Pts',(-3.88978582024371,2.49597508244882,
-6.11823618995914));
#111325=CARTESIAN_POINT('Ctrl Pts',(-3.90129660262183,2.49370793072441,
-6.11085687647957));
#111326=CARTESIAN_POINT('Ctrl Pts',(-3.912807385,2.491440779,-6.103477563));
#111327=CARTESIAN_POINT('Ctrl Pts',(-4.246635534,2.425690334,-5.889467561));
#111328=CARTESIAN_POINT('Ctrl Pts',(-4.55513171500001,2.360702725,-5.640325794));
#111329=CARTESIAN_POINT('',(-4.55146694340284,2.3614745814012,-5.64328349840463));
#111330=CARTESIAN_POINT('Origin',(0.0971190746755296,2.55353596056757,0.170671054071678));
#111331=CARTESIAN_POINT('Ctrl Pts',(-4.70744974767337,2.40074633452359,
-5.8386571123626));
#111332=CARTESIAN_POINT('Ctrl Pts',(-4.68139528364874,2.39450341726951,
-5.80609000094193));
#111333=CARTESIAN_POINT('Ctrl Pts',(-4.65535599040997,2.38811403216799,
-5.77351065652692));
#111334=CARTESIAN_POINT('Ctrl Pts',(-4.60336851064569,2.37503353882064,
-5.70839698870585));
#111335=CARTESIAN_POINT('Ctrl Pts',(-4.57739241382645,2.36833540936728,
-5.67582771278331));
#111336=CARTESIAN_POINT('Ctrl Pts',(-4.55146694245506,2.36147458181044,
-5.64328350085495));
#111337=CARTESIAN_POINT('Ctrl Pts',(-4.510543174,2.36069511,-5.992078127));
#111338=CARTESIAN_POINT('Ctrl Pts',(-4.83646943600001,2.42611337,-5.746736787));
#111339=CARTESIAN_POINT('Ctrl Pts',(-5.133861925,2.491440779,-5.46749135700001));
#111340=CARTESIAN_POINT('Ctrl Pts',(-4.547808613,2.36069511,-5.64623209));
#111341=CARTESIAN_POINT('Ctrl Pts',(-4.854923321,2.42611337,-5.398863776));
#111342=CARTESIAN_POINT('Ctrl Pts',(-5.133395382,2.491440779,-5.119643723));
#111343=CARTESIAN_POINT('Origin',(0.131599621200214,2.41071388183387,0.150156326072586));
#111344=CARTESIAN_POINT('Ctrl Pts',(-5.46265210513852,2.49597508244516,
-5.13985349893491));
#111345=CARTESIAN_POINT('Ctrl Pts',(-5.47230655587297,2.49370793072262,
-5.12951485847333));
#111346=CARTESIAN_POINT('Ctrl Pts',(-5.48196100660741,2.491440779,-5.11917621801159));
#111347=CARTESIAN_POINT('Ctrl Pts',(-5.76195304493989,2.425690334,-4.81934175864285));
#111348=CARTESIAN_POINT('Ctrl Pts',(-6.00757396462814,2.360702725,-4.49075903227299));
#111349=CARTESIAN_POINT('Ctrl Pts',(-5.1140847172565,2.49597508244516,-5.13900625734142));
#111350=CARTESIAN_POINT('Ctrl Pts',(-5.12374004962819,2.49370793072262,
-5.12932499017063));
#111351=CARTESIAN_POINT('Ctrl Pts',(-5.133395382,2.491440779,-5.119643723));
#111352=CARTESIAN_POINT('Ctrl Pts',(-5.413412989,2.425690334,-4.838873972));
#111353=CARTESIAN_POINT('Ctrl Pts',(-5.661138586,2.360702725,-4.529239441));
#111354=CARTESIAN_POINT('',(-5.65819531292125,2.36147458136162,-4.53291581459397));
#111355=CARTESIAN_POINT('Origin',(0.131537820879867,2.55353600730791,0.145803241101173));
#111356=CARTESIAN_POINT('Ctrl Pts',(-5.85253087835358,2.40074633455458,
-4.69019000897543));
#111357=CARTESIAN_POINT('Ctrl Pts',(-5.82008458820373,2.39450341754668,
-4.66398523911349));
#111358=CARTESIAN_POINT('Ctrl Pts',(-5.78765048252088,2.38811403232733,
-4.6377652594527));
#111359=CARTESIAN_POINT('Ctrl Pts',(-5.72288093750899,2.37503354102958,
-4.58534969261362));
#111360=CARTESIAN_POINT('Ctrl Pts',(-5.69051071011439,2.36833541046703,
-4.5591259566022));
#111361=CARTESIAN_POINT('Ctrl Pts',(-5.65819531327409,2.36147458182936,
-4.5329158161715));
#111362=CARTESIAN_POINT('Ctrl Pts',(-5.693208854,2.36069511,-4.882353219));
#111363=CARTESIAN_POINT('Ctrl Pts',(-5.95877400500001,2.42611337,-4.57268331000001));
#111364=CARTESIAN_POINT('Ctrl Pts',(-6.18918411,2.491440779,-4.23603589));
#111365=CARTESIAN_POINT('Ctrl Pts',(-5.655256373,2.36069511,-4.536581902));
#111366=CARTESIAN_POINT('Ctrl Pts',(-5.902014034,2.42611337,-4.228976338));
#111367=CARTESIAN_POINT('Ctrl Pts',(-6.113951515,2.491440779,-3.896421033));
#111368=CARTESIAN_POINT('Origin',(0.160802047155614,2.41071386843307,0.11835571462205));
#111369=CARTESIAN_POINT('Ctrl Pts',(-6.43985490420489,2.49597508252274,
-3.84537785260529));
#111370=CARTESIAN_POINT('Ctrl Pts',(-6.44706113725208,2.49370793076141,
-3.83320550208452));
#111371=CARTESIAN_POINT('Ctrl Pts',(-6.45426737029939,2.491440779,-3.82103315156376));
#111372=CARTESIAN_POINT('Ctrl Pts',(-6.66325780389173,2.425690334,-3.46801864364053));
#111373=CARTESIAN_POINT('Ctrl Pts',(-6.83250066956373,2.360702725,-3.09431676174519));
#111374=CARTESIAN_POINT('Ctrl Pts',(-6.09925469507655,2.49597508252274,
-3.91948210457872));
#111375=CARTESIAN_POINT('Ctrl Pts',(-6.10660310503828,2.49370793076141,
-3.90795156878934));
#111376=CARTESIAN_POINT('Ctrl Pts',(-6.113951515,2.491440779,-3.896421033));
#111377=CARTESIAN_POINT('Ctrl Pts',(-6.32706527000001,2.425690334,-3.562020014));
#111378=CARTESIAN_POINT('Ctrl Pts',(-6.50243690800001,2.360702725,-3.206370886));
#111379=CARTESIAN_POINT('',(-6.5003527587057,2.36147458134442,-3.21059402478539));
#111380=CARTESIAN_POINT('Origin',(0.159805770113787,2.55353595460724,0.114117596466036));
#111381=CARTESIAN_POINT('Ctrl Pts',(-6.72395416956975,2.40074633454225,
-3.32241483335559));
#111382=CARTESIAN_POINT('Ctrl Pts',(-6.68663319934288,2.39450341663434,
-3.30379770709918));
#111383=CARTESIAN_POINT('Ctrl Pts',(-6.64932086725947,2.38811403186844,
-3.28516311144202));
#111384=CARTESIAN_POINT('Ctrl Pts',(-6.57479782539573,2.37503354490892,
-3.24789654151664));
#111385=CARTESIAN_POINT('Ctrl Pts',(-6.53754705603456,2.36833541236912,
-3.22924453809376));
#111386=CARTESIAN_POINT('Ctrl Pts',(-6.50035275940381,2.36147458181569,
-3.21059402611262));
#111387=CARTESIAN_POINT('Ctrl Pts',(-6.609666415,2.36069511,-3.5443349));
#111388=CARTESIAN_POINT('Ctrl Pts',(-6.802452925,2.42611337,-3.184816244));
#111389=CARTESIAN_POINT('Ctrl Pts',(-6.955106924,2.491440779,-2.806508092));
#111390=CARTESIAN_POINT('Ctrl Pts',(-6.49827063,2.36069511,-3.214806186));
#111391=CARTESIAN_POINT('Ctrl Pts',(-6.673133131,2.42611337,-2.861346666));
#111392=CARTESIAN_POINT('Ctrl Pts',(-6.808626071,2.491440779,-2.491006026));
#111393=CARTESIAN_POINT('Origin',(0.182487905438553,2.41071429564125,0.0810218689469716));
#111394=CARTESIAN_POINT('Ctrl Pts',(-7.11593724508701,2.49597508225771,
-2.37109661029227));
#111395=CARTESIAN_POINT('Ctrl Pts',(-7.12035830459428,2.49370793062889,
-2.35765971624731));
#111396=CARTESIAN_POINT('Ctrl Pts',(-7.12477936410143,2.491440779,-2.34422282220235));
#111397=CARTESIAN_POINT('Ctrl Pts',(-7.25299603309939,2.425690334,-1.95453483150014));
#111398=CARTESIAN_POINT('Ctrl Pts',(-7.33794723805909,2.360702725,-1.55318767885172));
#111399=CARTESIAN_POINT('Ctrl Pts',(-6.79923030378816,2.49597508225771,
-2.51668732283746));
#111400=CARTESIAN_POINT('Ctrl Pts',(-6.80392818739409,2.49370793062889,
-2.50384667441869));
#111401=CARTESIAN_POINT('Ctrl Pts',(-6.80862607100001,2.491440779,-2.491006026));
#111402=CARTESIAN_POINT('Ctrl Pts',(-6.944871011,2.425690334,-2.11860996));
#111403=CARTESIAN_POINT('Ctrl Pts',(-7.039688507,2.360702725,-1.733575992));
#111404=CARTESIAN_POINT('',(-7.03856093436333,2.36147458134285,-1.73814842650295));
#111405=CARTESIAN_POINT('Origin',(0.180601220225389,2.55353597284607,0.0770959809789962));
#111406=CARTESIAN_POINT('Ctrl Pts',(-7.28097283682833,2.40074633457552,
-1.79928723337112));
#111407=CARTESIAN_POINT('Ctrl Pts',(-7.24052262012437,2.39450346940029,
-1.78912835643461));
#111408=CARTESIAN_POINT('Ctrl Pts',(-7.20007656101851,2.38811405783542,
-1.77895043030641));
#111409=CARTESIAN_POINT('Ctrl Pts',(-7.11928449131764,2.37503355074156,
-1.75857535170139));
#111410=CARTESIAN_POINT('Ctrl Pts',(-7.07889497548673,2.36833541519939,
-1.74836723103845));
#111411=CARTESIAN_POINT('Ctrl Pts',(-7.03856093503845,2.36147458176162,
-1.73814842746186));
#111412=CARTESIAN_POINT('Ctrl Pts',(-7.217063321,2.36069511,-2.040587421));
#111413=CARTESIAN_POINT('Ctrl Pts',(-7.328056705,2.42611337,-1.648030711));
#111414=CARTESIAN_POINT('Ctrl Pts',(-7.39581666999999,2.491440779,-1.245751095));
#111415=CARTESIAN_POINT('Ctrl Pts',(-7.03743297500001,2.36069511,-1.742709706));
#111416=CARTESIAN_POINT('Ctrl Pts',(-7.132223939,2.42611337,-1.359923604));
#111417=CARTESIAN_POINT('Ctrl Pts',(-7.184936839,2.491440779,-0.969114346));
#111418=CARTESIAN_POINT('Origin',(0.195638787465489,2.41071431194102,0.0398981238600597));
#111419=CARTESIAN_POINT('Ctrl Pts',(-7.45928626917492,2.49597508222446,
-0.785945526233097));
#111420=CARTESIAN_POINT('Ctrl Pts',(-7.46071543173044,2.49370793061227,
-0.771872382326965));
#111421=CARTESIAN_POINT('Ctrl Pts',(-7.462144594286,2.491440779,-0.757799238420837));
#111422=CARTESIAN_POINT('Ctrl Pts',(-7.50359222994364,2.425690334,-0.349659143433354));
#111423=CARTESIAN_POINT('Ctrl Pts',(-7.50027954846603,2.360702725,0.0605667337499607));
#111424=CARTESIAN_POINT('Ctrl Pts',(-7.18128145937083,2.49597508222447,
-0.996215040427868));
#111425=CARTESIAN_POINT('Ctrl Pts',(-7.18310914918541,2.49370793061227,
-0.982664693213935));
#111426=CARTESIAN_POINT('Ctrl Pts',(-7.184936839,2.491440779,-0.969114346));
#111427=CARTESIAN_POINT('Ctrl Pts',(-7.237942301,2.425690334,-0.576136058));
#111428=CARTESIAN_POINT('Ctrl Pts',(-7.24777209600001,2.360702725,-0.179721011));
#111429=CARTESIAN_POINT('',(-7.24765382360903,2.36147458135816,-0.184428939767084));
#111430=CARTESIAN_POINT('Origin',(0.192952530454964,2.55353598637138,0.0364696205559954));
#111431=CARTESIAN_POINT('Ctrl Pts',(-7.49754130656375,2.40074633455833,
-0.192026962126391));
#111432=CARTESIAN_POINT('Ctrl Pts',(-7.45585293515902,2.39450346937786,
-0.190801194864945));
#111433=CARTESIAN_POINT('Ctrl Pts',(-7.41416452940256,2.38811405784962,
-0.189555930013006));
#111434=CARTESIAN_POINT('Ctrl Pts',(-7.33088131199388,2.37503355361642,
-0.187025116539651));
#111435=CARTESIAN_POINT('Ctrl Pts',(-7.28924162669139,2.36833541661307,
-0.185738207668953));
#111436=CARTESIAN_POINT('Ctrl Pts',(-7.24765382450455,2.36147458176434,
-0.184428940115875));
#111437=CARTESIAN_POINT('Ctrl Pts',(-7.486998367,2.36069511,-0.441424342));
#111438=CARTESIAN_POINT('Ctrl Pts',(-7.511008699,2.42611337,-0.034185093));
#111439=CARTESIAN_POINT('Ctrl Pts',(-7.490706247,2.491440779,0.373255838));
#111440=CARTESIAN_POINT('Ctrl Pts',(-7.247532776,2.36069511,-0.189126057));
#111441=CARTESIAN_POINT('Ctrl Pts',(-7.257819883,2.42611337,0.205087974));
#111442=CARTESIAN_POINT('Ctrl Pts',(-7.225287946,2.491440779,0.598092044));
#111443=CARTESIAN_POINT('Origin',(0.199639167737231,2.41071391476071,-0.00309109376033817));
#111444=CARTESIAN_POINT('Ctrl Pts',(-7.45384735693224,2.49597508251434,
0.835955493822569));
#111445=CARTESIAN_POINT('Ctrl Pts',(-7.45221779643163,2.49370793075721,
0.850006844084534));
#111446=CARTESIAN_POINT('Ctrl Pts',(-7.45058823593115,2.491440779,0.864058194346502));
#111447=CARTESIAN_POINT('Ctrl Pts',(-7.40332879345145,2.425690334,1.27156621829887));
#111448=CARTESIAN_POINT('Ctrl Pts',(-7.31190712236696,2.360702725,1.67148911281306));
#111449=CARTESIAN_POINT('Ctrl Pts',(-7.22754387548367,2.49597508251434,
0.570839148403493));
#111450=CARTESIAN_POINT('Ctrl Pts',(-7.22641591074183,2.49370793075721,
0.584465596201748));
#111451=CARTESIAN_POINT('Ctrl Pts',(-7.225287946,2.491440779,0.598092044));
#111452=CARTESIAN_POINT('Ctrl Pts',(-7.192575454,2.425690334,0.993277326));
#111453=CARTESIAN_POINT('Ctrl Pts',(-7.116957917,2.360702725,1.382537524));
#111454=CARTESIAN_POINT('',(-7.11785447482644,2.36147458139012,1.37791424072264));
#111455=CARTESIAN_POINT('Origin',(0.196281286854487,2.5535358133817,-0.00586212603583963));
#111456=CARTESIAN_POINT('Ctrl Pts',(-7.36353307773095,2.40074633454747,
1.42421227703032));
#111457=CARTESIAN_POINT('Ctrl Pts',(-7.32255551225088,2.39450341737561,
1.41644755423288));
#111458=CARTESIAN_POINT('Ctrl Pts',(-7.28157424400633,2.38811403222071,
1.40870196489122));
#111459=CARTESIAN_POINT('Ctrl Pts',(-7.19969419612551,2.3750335446404,1.39327019884403));
#111460=CARTESIAN_POINT('Ctrl Pts',(-7.1587514060899,2.36833541220006,1.38557572453513));
#111461=CARTESIAN_POINT('Ctrl Pts',(-7.11785447620099,2.36147458176668,
1.37791423874306));
#111462=CARTESIAN_POINT('Ctrl Pts',(-7.406849691,2.36069511,1.178379249));
#111463=CARTESIAN_POINT('Ctrl Pts',(-7.342754274,2.42611337,1.581258982));
#111464=CARTESIAN_POINT('Ctrl Pts',(-7.235338726,2.491440779,1.974809744));
#111465=CARTESIAN_POINT('Ctrl Pts',(-7.118745999,2.36069511,1.373300916));
#111466=CARTESIAN_POINT('Ctrl Pts',(-7.044048235,2.42611337,1.760509866));
#111467=CARTESIAN_POINT('Ctrl Pts',(-6.92779261899999,2.491440779,2.137332315));
#111468=CARTESIAN_POINT('Origin',(0.194307367130044,2.41071390558892,-0.0459353841191443));
#111469=CARTESIAN_POINT('Ctrl Pts',(-7.09987482744547,2.49597508226345,
2.41876816842104));
#111470=CARTESIAN_POINT('Ctrl Pts',(-7.09526274045952,2.49370793063177,
2.43214069782287));
#111471=CARTESIAN_POINT('Ctrl Pts',(-7.09065065347373,2.491440779,2.4455132272247));
#111472=CARTESIAN_POINT('Ctrl Pts',(-6.95689393096362,2.425690334,2.83333455625786));
#111473=CARTESIAN_POINT('Ctrl Pts',(-6.78163804747186,2.360702725,3.2042545191125));
#111474=CARTESIAN_POINT('Ctrl Pts',(-6.93585437261289,2.49597508226346,
2.11120153655164));
#111475=CARTESIAN_POINT('Ctrl Pts',(-6.9318234958064,2.49370793063177,2.12426692577582));
#111476=CARTESIAN_POINT('Ctrl Pts',(-6.92779261900001,2.491440779,2.137332315));
#111477=CARTESIAN_POINT('Ctrl Pts',(-6.810891773,2.425690334,2.516246166));
#111478=CARTESIAN_POINT('Ctrl Pts',(-6.653362696,2.360702725,2.880150141));
#111479=CARTESIAN_POINT('',(-6.65523216194324,2.36147458138726,2.87582768139692));
#111480=CARTESIAN_POINT('Origin',(0.190432156601331,2.55353592875688,-0.0479197318352048));
#111481=CARTESIAN_POINT('Ctrl Pts',(-6.88521422635454,2.40074633447517,
2.97385693256405));
#111482=CARTESIAN_POINT('Ctrl Pts',(-6.84686419893038,2.39450346931693,
2.95746491590463));
#111483=CARTESIAN_POINT('Ctrl Pts',(-6.80850595347635,2.38811405780224,
2.94109058031555));
#111484=CARTESIAN_POINT('Ctrl Pts',(-6.73185741844179,2.37503354110023,
2.90841773763505));
#111485=CARTESIAN_POINT('Ctrl Pts',(-6.69352594351825,2.36833541044172,
2.89210167091586));
#111486=CARTESIAN_POINT('Ctrl Pts',(-6.65523216371794,2.36147458173047,
2.87582767950765));
#111487=CARTESIAN_POINT('Ctrl Pts',(-6.980364955,2.36069511,2.743083136));
#111488=CARTESIAN_POINT('Ctrl Pts',(-6.83116082000001,2.42611337,3.122765145));
#111489=CARTESIAN_POINT('Ctrl Pts',(-6.641654807,2.491440779,3.48402374));
#111490=CARTESIAN_POINT('Ctrl Pts',(-6.65709457100001,2.36069511,2.871513865));
#111491=CARTESIAN_POINT('Ctrl Pts',(-6.500904721,2.42611337,3.233612273));
#111492=CARTESIAN_POINT('Ctrl Pts',(-6.306361409,2.491440779,3.576633302));
#111493=CARTESIAN_POINT('Origin',(0.17988987011895,2.41071387449181,-0.0866317942443601));
#111494=CARTESIAN_POINT('Ctrl Pts',(-6.41392004192706,2.49597508250466,
3.88848192866056));
#111495=CARTESIAN_POINT('Ctrl Pts',(-6.4065410840626,2.49370793075237,3.9005503540226));
#111496=CARTESIAN_POINT('Ctrl Pts',(-6.39916212619799,2.491440779,3.91261877938463));
#111497=CARTESIAN_POINT('Ctrl Pts',(-6.18516244014714,2.425690334,4.26261931956866));
#111498=CARTESIAN_POINT('Ctrl Pts',(-5.93426711362043,2.360702725,4.58719254601069));
#111499=CARTESIAN_POINT('Ctrl Pts',(-6.31985202892025,2.49597508250466,
3.55284648411619));
#111500=CARTESIAN_POINT('Ctrl Pts',(-6.31310671896012,2.49370793075237,
3.56473989305809));
#111501=CARTESIAN_POINT('Ctrl Pts',(-6.306361409,2.491440779,3.576633302));
#111502=CARTESIAN_POINT('Ctrl Pts',(-6.110738363,2.425690334,3.921558131));
#111503=CARTESIAN_POINT('Ctrl Pts',(-5.87866363,2.360702725,4.243090139));
#111504=CARTESIAN_POINT('',(-5.88141858947572,2.36147458139205,4.23927061567419));
#111505=CARTESIAN_POINT('Origin',(0.17567859128798,2.55353596923167,-0.0877366492651954));
#111506=CARTESIAN_POINT('Ctrl Pts',(-6.0849504101184,2.400746334527,4.38444734373401));
#111507=CARTESIAN_POINT('Ctrl Pts',(-6.05102049224245,2.39450341566143,
4.36019423236533));
#111508=CARTESIAN_POINT('Ctrl Pts',(-6.01707919396739,2.3881140313641,4.33595694134223));
#111509=CARTESIAN_POINT('Ctrl Pts',(-5.94924644971532,2.37503353301049,
4.28757086998339));
#111510=CARTESIAN_POINT('Ctrl Pts',(-5.91531863784454,2.36833540648173,
4.26339614570779));
#111511=CARTESIAN_POINT('Ctrl Pts',(-5.88141859215414,2.36147458175874,
4.23927061437437));
#111512=CARTESIAN_POINT('Ctrl Pts',(-6.227486113,2.36069511,4.179523504));
#111513=CARTESIAN_POINT('Ctrl Pts',(-6.000149879,2.42611337,4.51825428));
#111514=CARTESIAN_POINT('Ctrl Pts',(-5.737414491,2.491440779,4.83032865900001));
#111515=CARTESIAN_POINT('Ctrl Pts',(-5.884164799,2.36069511,4.235458017));
#111516=CARTESIAN_POINT('Ctrl Pts',(-5.653786127,2.42611337,4.555514565));
#111517=CARTESIAN_POINT('Ctrl Pts',(-5.390051748,2.491440779,4.848694892));
#111518=CARTESIAN_POINT('Origin',(0.157060863459541,2.41071387183971,-0.123277390313924));
#111519=CARTESIAN_POINT('Ctrl Pts',(-5.42805748376532,2.49597508245143,
5.17637459698762));
#111520=CARTESIAN_POINT('Ctrl Pts',(-5.41825668723348,2.49370793072575,
5.18657461133535));
#111521=CARTESIAN_POINT('Ctrl Pts',(-5.40845589070163,2.491440779,5.19677462568309));
#111522=CARTESIAN_POINT('Ctrl Pts',(-5.12421962807833,2.425690334,5.49258874114573));
#111523=CARTESIAN_POINT('Ctrl Pts',(-4.80941644524494,2.360702725,5.75563854725621));
#111524=CARTESIAN_POINT('Ctrl Pts',(-5.40834042720503,2.49597508245143,
4.82836428150074));
#111525=CARTESIAN_POINT('Ctrl Pts',(-5.39919608760243,2.49370793072576,
4.83852958675043));
#111526=CARTESIAN_POINT('Ctrl Pts',(-5.390051748,2.491440779,4.848694892));
#111527=CARTESIAN_POINT('Ctrl Pts',(-5.124853618,2.425690334,5.143502397));
#111528=CARTESIAN_POINT('Ctrl Pts',(-4.829084786,2.360702725,5.407627958));
#111529=CARTESIAN_POINT('',(-4.83259642189076,2.36147458135634,5.40448996696835));
#111530=CARTESIAN_POINT('Origin',(0.152710607699905,2.55353599870726,-0.123451173809973));
#111531=CARTESIAN_POINT('Ctrl Pts',(-5.00016107556259,2.40074633453265,
5.59002586934225));
#111532=CARTESIAN_POINT('Ctrl Pts',(-4.97223836249954,2.39450346937479,
5.55904611943058));
#111533=CARTESIAN_POINT('Ctrl Pts',(-4.94430076676404,2.38811405783615,
5.52807896560669));
#111534=CARTESIAN_POINT('Ctrl Pts',(-4.8884553877854,2.37503353569015,5.46624198633146));
#111535=CARTESIAN_POINT('Ctrl Pts',(-4.86051763445355,2.36833540783023,
5.4353389703849));
#111536=CARTESIAN_POINT('Ctrl Pts',(-4.83259642383872,2.36147458182015,
5.40448996692274));
#111537=CARTESIAN_POINT('Ctrl Pts',(-5.183416941,2.36069511,5.42053399799999));
#111538=CARTESIAN_POINT('Ctrl Pts',(-4.888578597,2.42611337,5.702474866));
#111539=CARTESIAN_POINT('Ctrl Pts',(-4.564899051,2.491440779,5.950772778));
#111540=CARTESIAN_POINT('Ctrl Pts',(-4.836098022,2.36069511,5.401356859));
#111541=CARTESIAN_POINT('Ctrl Pts',(-4.542302778,2.42611337,5.664406059));
#111542=CARTESIAN_POINT('Ctrl Pts',(-4.221709258,2.491440779,5.894036897));
#111543=CARTESIAN_POINT('Origin',(0.12688778706036,2.41071389289739,-0.154158578376882));
#111544=CARTESIAN_POINT('Ctrl Pts',(-4.1883849903721,2.49597508243633,6.22222574211514));
#111545=CARTESIAN_POINT('Ctrl Pts',(-4.17662062947665,2.4937079307182,6.23008040424037));
#111546=CARTESIAN_POINT('Ctrl Pts',(-4.16485626858112,2.491440779,6.23793506636559));
#111547=CARTESIAN_POINT('Ctrl Pts',(-3.82367400106207,2.425690334,6.4657308181516));
#111548=CARTESIAN_POINT('Ctrl Pts',(-3.45968280923341,2.360702725,6.65495728654121));
#111549=CARTESIAN_POINT('Ctrl Pts',(-4.24394083831678,2.49597508243633,
5.87811313032217));
#111550=CARTESIAN_POINT('Ctrl Pts',(-4.23282504815834,2.4937079307182,5.88607501366108));
#111551=CARTESIAN_POINT('Ctrl Pts',(-4.221709258,2.491440779,5.894036897));
#111552=CARTESIAN_POINT('Ctrl Pts',(-3.899336413,2.425690334,6.124942208));
#111553=CARTESIAN_POINT('Ctrl Pts',(-3.553703304,2.360702725,6.319311104));
#111554=CARTESIAN_POINT('',(-3.55780741590456,2.36147458136437,6.31700137503095));
#111555=CARTESIAN_POINT('Origin',(0.122601975477235,2.55353596932925,-0.153393243284287));
#111556=CARTESIAN_POINT('Ctrl Pts',(-3.68156976613605,2.40074633450448,
6.53422099858764));
#111557=CARTESIAN_POINT('Ctrl Pts',(-3.6609596010483,2.39450346936461,6.49796298013453));
#111558=CARTESIAN_POINT('Ctrl Pts',(-3.6403321933983,2.38811405783015,6.46171406386962));
#111559=CARTESIAN_POINT('Ctrl Pts',(-3.59908559050729,2.37503354191843,
6.38931772749768));
#111560=CARTESIAN_POINT('Ctrl Pts',(-3.57844423085058,2.36833541091996,
6.3531313975145));
#111561=CARTESIAN_POINT('Ctrl Pts',(-3.55780741727867,2.36147458187027,
6.31700137561664));
#111562=CARTESIAN_POINT('Ctrl Pts',(-3.896976953,2.36069511,6.408086347));
#111563=CARTESIAN_POINT('Ctrl Pts',(-3.548422814,2.42611337,6.62005406600001));
#111564=CARTESIAN_POINT('Ctrl Pts',(-3.178934004,2.491440779,6.792965376));
#111565=CARTESIAN_POINT('Ctrl Pts',(-3.561900676,2.36069511,6.314694258));
#111566=CARTESIAN_POINT('Ctrl Pts',(-3.218426399,2.42611337,6.508436221));
#111567=CARTESIAN_POINT('Ctrl Pts',(-2.855964336,2.491440779,6.663780287));
#111568=CARTESIAN_POINT('Origin',(0.0907828019592194,2.41071434575424,-0.177833967379083));
#111569=CARTESIAN_POINT('Ctrl Pts',(-2.75286827051218,2.49597508252244,
6.97713252655705));
#111570=CARTESIAN_POINT('Ctrl Pts',(-2.73969043341109,2.49370793076126,
6.982274561309));
#111571=CARTESIAN_POINT('Ctrl Pts',(-2.72651259631005,2.491440779,6.98741659606107));
#111572=CARTESIAN_POINT('Ctrl Pts',(-2.34433762754852,2.425690334,7.13654250767061));
#111573=CARTESIAN_POINT('Ctrl Pts',(-1.94817824990591,2.360702725,7.24309761964013));
#111574=CARTESIAN_POINT('Ctrl Pts',(-2.88109929397571,2.49597508252244,
6.65300794152305));
#111575=CARTESIAN_POINT('Ctrl Pts',(-2.86853181498786,2.49370793076126,
6.65839411426155));
#111576=CARTESIAN_POINT('Ctrl Pts',(-2.855964336,2.491440779,6.663780287));
#111577=CARTESIAN_POINT('Ctrl Pts',(-2.491490572,2.425690334,6.819986528));
#111578=CARTESIAN_POINT('Ctrl Pts',(-2.112154606,2.360702725,6.935510285));
#111579=CARTESIAN_POINT('',(-2.11665928906527,2.36147458134173,6.93413681942433));
#111580=CARTESIAN_POINT('Origin',(0.0867605426048537,2.55353593756859,-0.17616271679774));
#111581=CARTESIAN_POINT('Ctrl Pts',(-2.19083234638043,2.40074633453881,
7.17288321586643));
#111582=CARTESIAN_POINT('Ctrl Pts',(-2.17849833213471,2.39450341596068,
7.1330419724508));
#111583=CARTESIAN_POINT('Ctrl Pts',(-2.16614568309511,2.38811403152101,
7.09320643362084));
#111584=CARTESIAN_POINT('Ctrl Pts',(-2.14142653374841,2.37503354663782,
7.01363607193964));
#111585=CARTESIAN_POINT('Ctrl Pts',(-2.12904674398792,2.36833541317278,
6.9738584605462));
#111586=CARTESIAN_POINT('Ctrl Pts',(-2.11665928997783,2.3614745817451,6.9341368200675));
#111587=CARTESIAN_POINT('Ctrl Pts',(-2.428318655,2.36069511,7.0960037));
#111588=CARTESIAN_POINT('Ctrl Pts',(-2.042346724,2.42611337,7.22808689500001));
#111589=CARTESIAN_POINT('Ctrl Pts',(-1.644325536,2.491440779,7.317526463));
#111590=CARTESIAN_POINT('Ctrl Pts',(-2.121152813,2.36069511,6.932763572));
#111591=CARTESIAN_POINT('Ctrl Pts',(-1.744059979,2.42611337,7.048139138));
#111592=CARTESIAN_POINT('Ctrl Pts',(-1.356677695,2.491440779,7.121932718));
#111593=CARTESIAN_POINT('Origin',(0.0504308075600973,2.41071389512704,-0.193189663991771));
#111594=CARTESIAN_POINT('Ctrl Pts',(-1.18863048790655,2.49597508226724,
7.40579634977361));
#111595=CARTESIAN_POINT('Ctrl Pts',(-1.17465535663115,2.49370793063366,
7.40798532104452));
#111596=CARTESIAN_POINT('Ctrl Pts',(-1.16068022535578,2.491440779,7.4101742923153));
#111597=CARTESIAN_POINT('Ctrl Pts',(-0.755382632264268,2.425690334,7.47365740169885));
#111598=CARTESIAN_POINT('Ctrl Pts',(-0.345579041176663,2.360702725,7.49255875907289));
#111599=CARTESIAN_POINT('Ctrl Pts',(-1.38354074594054,2.49597508226724,
7.11681549620122));
#111600=CARTESIAN_POINT('Ctrl Pts',(-1.37010922047026,2.49370793063366,
7.11937410660064));
#111601=CARTESIAN_POINT('Ctrl Pts',(-1.356677695,2.491440779,7.12193271700001));
#111602=CARTESIAN_POINT('Ctrl Pts',(-0.967145401,2.425690334,7.196135858));
#111603=CARTESIAN_POINT('Ctrl Pts',(-0.571843906,2.360702725,7.227412715));
#111604=CARTESIAN_POINT('',(-0.57653852648969,2.36147458135925,7.22703973357806));
#111605=CARTESIAN_POINT('Origin',(0.0468623792659997,2.55353595236423,-0.190695107929225));
#111606=CARTESIAN_POINT('Ctrl Pts',(-0.597654041416066,2.400746334532,7.4761493862767));
#111607=CARTESIAN_POINT('Ctrl Pts',(-0.594173108960324,2.39450346937549,
7.43458851622998));
#111608=CARTESIAN_POINT('Ctrl Pts',(-0.590672705689646,2.38811405787017,
7.39302866746393));
#111609=CARTESIAN_POINT('Ctrl Pts',(-0.583636731008162,2.37503353385956,
7.31000448191802));
#111610=CARTESIAN_POINT('Ctrl Pts',(-0.580097388195057,2.36833540694216,
7.26849560360237));
#111611=CARTESIAN_POINT('Ctrl Pts',(-0.576538527924448,2.36147458183712,
7.22703973472027));
#111612=CARTESIAN_POINT('Ctrl Pts',(-0.846114875,2.36069511,7.452119807));
#111613=CARTESIAN_POINT('Ctrl Pts',(-0.440772771,2.42611337,7.49814241400001));
#111614=CARTESIAN_POINT('Ctrl Pts',(-0.032830234,2.491440779,7.499928145));
#111615=CARTESIAN_POINT('Ctrl Pts',(-0.581222202,2.36069511,7.226664566));
#111616=CARTESIAN_POINT('Ctrl Pts',(-0.188143253,2.42611337,7.25827890400001));
#111617=CARTESIAN_POINT('Ctrl Pts',(0.206045687,2.491440779,7.24707148999999));
#111618=CARTESIAN_POINT('Origin',(0.00772170226827618,2.41071388357142,
-0.199513755488948));
#111619=CARTESIAN_POINT('Ctrl Pts',(-1.361241758,3.526465848,7.12106178));
#111620=CARTESIAN_POINT('Ctrl Pts',(-0.971016684,3.460723853,7.195656087));
#111621=CARTESIAN_POINT('Ctrl Pts',(-0.574977339,3.395965514,7.227164109));
#111622=CARTESIAN_POINT('Ctrl Pts',(-1.649014893,3.526465848,7.316471136));
#111623=CARTESIAN_POINT('Ctrl Pts',(-1.248081637,3.460723853,7.406835042));
#111624=CARTESIAN_POINT('Ctrl Pts',(-0.839675095,3.395965514,7.452848163));
#111625=CARTESIAN_POINT('',(-1.35657627656236,3.52567991525468,7.12195203434018));
#111626=CARTESIAN_POINT('Origin',(0.0523978542384437,3.62492142657274,-0.186938114701938));
#111627=CARTESIAN_POINT('Ctrl Pts',(-1.40278481009805,3.4862983188696,7.36764513055359));
#111628=CARTESIAN_POINT('Ctrl Pts',(-1.39511199963782,3.49254601522961,
7.32664918607182));
#111629=CARTESIAN_POINT('Ctrl Pts',(-1.38742201379164,3.49894654287788,
7.2856556149904));
#111630=CARTESIAN_POINT('Ctrl Pts',(-1.37202285368929,3.51206280605285,
7.20377130722841));
#111631=CARTESIAN_POINT('Ctrl Pts',(-1.36430479237325,3.51878610650216,
7.16283330034619));
#111632=CARTESIAN_POINT('Ctrl Pts',(-1.35657627478824,3.52567991511443,
7.12195203641864));
#111633=CARTESIAN_POINT('Ctrl Pts',(-2.14101470880455,3.39148928113836,
6.92670820838241));
#111634=CARTESIAN_POINT('Ctrl Pts',(-2.12808802390228,3.39372739756918,
6.93065105269119));
#111635=CARTESIAN_POINT('Ctrl Pts',(-2.115161339,3.395965514,6.934593897));
#111636=CARTESIAN_POINT('Ctrl Pts',(-1.738674564,3.461150149,7.049428346));
#111637=CARTESIAN_POINT('Ctrl Pts',(-1.35196834,3.526458173,7.122828203));
#111638=CARTESIAN_POINT('Ctrl Pts',(-1.97832240686564,3.39148928113836,
7.23497047159279));
#111639=CARTESIAN_POINT('Ctrl Pts',(-1.96482223297234,3.39372739756918,
7.23860790526758));
#111640=CARTESIAN_POINT('Ctrl Pts',(-1.95132205907898,3.395965514,7.24224533894237));
#111641=CARTESIAN_POINT('Ctrl Pts',(-1.55813254688242,3.461150149,7.34818477228137));
#111642=CARTESIAN_POINT('Ctrl Pts',(-1.15578476260318,3.526458173,7.41093360613679));
#111643=CARTESIAN_POINT('Origin',(0.0444211629504335,3.48214329357323,-0.194615624345732));
#111644=CARTESIAN_POINT('Ctrl Pts',(-2.860234467,3.526465848,6.661948573));
#111645=CARTESIAN_POINT('Ctrl Pts',(-2.495168211,3.460723853,6.818685762));
#111646=CARTESIAN_POINT('Ctrl Pts',(-2.115161339,3.395965514,6.934593897));
#111647=CARTESIAN_POINT('Ctrl Pts',(-3.183286862,3.526465848,6.79092664900001));
#111648=CARTESIAN_POINT('Ctrl Pts',(-2.811152772,3.460723853,6.965366696));
#111649=CARTESIAN_POINT('Ctrl Pts',(-2.422186008,3.395965514,7.098099389));
#111650=CARTESIAN_POINT('',(-2.85586944022338,3.52567991541331,6.66382095494341));
#111651=CARTESIAN_POINT('Origin',(0.0913593601432727,3.62492148818353,-0.171304427496621));
#111652=CARTESIAN_POINT('Ctrl Pts',(-2.95381439782472,3.48629831883926,
6.89383641350067));
#111653=CARTESIAN_POINT('Ctrl Pts',(-2.93750805711256,3.49254601521039,
6.85544835880128));
#111654=CARTESIAN_POINT('Ctrl Pts',(-2.92118545276567,3.4989465428767,6.81706631419639));
#111655=CARTESIAN_POINT('Ctrl Pts',(-2.88854361064173,3.51206280608755,
6.74040678022559));
#111656=CARTESIAN_POINT('Ctrl Pts',(-2.87220553190004,3.51878610654731,
6.70208503630344));
#111657=CARTESIAN_POINT('Ctrl Pts',(-2.85586943938469,3.52567991517898,
6.66382095653845));
#111658=CARTESIAN_POINT('Ctrl Pts',(-3.57999648816175,3.39148928099491,
6.30451074469791));
#111659=CARTESIAN_POINT('Ctrl Pts',(-3.56821961658091,3.39372739749746,
6.31114026284889));
#111660=CARTESIAN_POINT('Ctrl Pts',(-3.556442745,3.395965514,6.317769781));
#111661=CARTESIAN_POINT('Ctrl Pts',(-3.213444034,3.461150149,6.510852992));
#111662=CARTESIAN_POINT('Ctrl Pts',(-2.851557586,3.526458173,6.665667208));
#111663=CARTESIAN_POINT('Ctrl Pts',(-3.48737511649809,3.3914892809949,6.64054004360659));
#111664=CARTESIAN_POINT('Ctrl Pts',(-3.47497250948965,3.39372739749745,
6.64699457464484));
#111665=CARTESIAN_POINT('Ctrl Pts',(-3.4625699024813,3.395965514,6.65344910568322));
#111666=CARTESIAN_POINT('Ctrl Pts',(-3.10134678922173,3.461150149,6.84143585675353));
#111667=CARTESIAN_POINT('Ctrl Pts',(-2.72189481628153,3.526458173,6.98921053722955));
#111668=CARTESIAN_POINT('Origin',(0.0852192425559628,3.48214323855182,-0.180516398354257));
#111669=CARTESIAN_POINT('Ctrl Pts',(-4.225485793,3.526465848,5.891330055));
#111670=CARTESIAN_POINT('Ctrl Pts',(-3.902648444,3.460723853,6.122881269));
#111671=CARTESIAN_POINT('Ctrl Pts',(-3.556442745,3.395965514,6.317769781));
#111672=CARTESIAN_POINT('Ctrl Pts',(-4.56871187600001,3.526465848,5.94784598));
#111673=CARTESIAN_POINT('Ctrl Pts',(-4.242777527,3.460723853,6.198205544));
#111674=CARTESIAN_POINT('Ctrl Pts',(-3.891438196,3.395965514,6.411451378));
#111675=CARTESIAN_POINT('',(-4.22162532483267,3.52567991538939,5.89409701316192));
#111676=CARTESIAN_POINT('Origin',(0.126048906263722,3.62492145840609,-0.147660019288895));
#111677=CARTESIAN_POINT('Ctrl Pts',(-4.36672690769358,3.48629831887157,
6.09767956762302));
#111678=CARTESIAN_POINT('Ctrl Pts',(-4.34254950320055,3.49254601523147,
6.06369438560012));
#111679=CARTESIAN_POINT('Ctrl Pts',(-4.3183575074241,3.49894654285412,6.0297185695337));
#111680=CARTESIAN_POINT('Ctrl Pts',(-4.26999927978729,3.5120628060483,5.96186832409333));
#111681=CARTESIAN_POINT('Ctrl Pts',(-4.24580513409496,3.51878610651955,
5.92795472514906));
#111682=CARTESIAN_POINT('Ctrl Pts',(-4.22162532432222,3.52567991516351,
5.89409701520979));
#111683=CARTESIAN_POINT('Ctrl Pts',(-4.85158160960764,3.39148928105395,
5.38752136628062));
#111684=CARTESIAN_POINT('Ctrl Pts',(-4.84150522530381,3.39372739752697,
5.39652756914034));
#111685=CARTESIAN_POINT('Ctrl Pts',(-4.831428841,3.395965514,5.405533772));
#111686=CARTESIAN_POINT('Ctrl Pts',(-4.537956432,3.461150149,5.667837389));
#111687=CARTESIAN_POINT('Ctrl Pts',(-4.217811169,3.526458173,5.896827024));
#111688=CARTESIAN_POINT('Ctrl Pts',(-4.83336204012894,3.39148928105394,
5.73560534434831));
#111689=CARTESIAN_POINT('Ctrl Pts',(-4.82263693272546,3.39372739752697,
5.74457516578482));
#111690=CARTESIAN_POINT('Ctrl Pts',(-4.811911825322,3.395965514,5.75354498722122));
#111691=CARTESIAN_POINT('Ctrl Pts',(-4.49954550307979,3.461150149,6.01478900351506));
#111692=CARTESIAN_POINT('Ctrl Pts',(-4.16073209479072,3.526458173,6.24067975220765));
#111693=CARTESIAN_POINT('Origin',(0.122032535617754,3.48214323624807,-0.157976378280283));
#111694=CARTESIAN_POINT('Ctrl Pts',(-5.393158098,3.526465848,4.845239491));
#111695=CARTESIAN_POINT('Ctrl Pts',(-5.127645174,3.460723853,5.140777654));
#111696=CARTESIAN_POINT('Ctrl Pts',(-4.83142884100001,3.395965514,5.40553377200001));
#111697=CARTESIAN_POINT('Ctrl Pts',(-5.740508999,3.526465848,4.826650643));
#111698=CARTESIAN_POINT('Ctrl Pts',(-5.476014721,3.460723853,5.14122319));
#111699=CARTESIAN_POINT('Ctrl Pts',(-5.178731058,3.395965514,5.425011025));
#111700=CARTESIAN_POINT('',(-5.38998270028869,3.52567991539829,4.84877164614679));
#111701=CARTESIAN_POINT('Origin',(0.154844449716129,3.62492148424465,-0.11711098248098));
#111702=CARTESIAN_POINT('Ctrl Pts',(-5.57545611982745,3.48629831884877,
5.01640200221238));
#111703=CARTESIAN_POINT('Ctrl Pts',(-5.54453816000373,3.49254601522222,
4.98840880214834));
#111704=CARTESIAN_POINT('Ctrl Pts',(-5.51360796327686,3.49894654288713,
4.96042788561611));
#111705=CARTESIAN_POINT('Ctrl Pts',(-5.45179452686104,3.5120628060797,4.90455953070738));
#111706=CARTESIAN_POINT('Ctrl Pts',(-5.42087560556212,3.51878610652425,
4.87663983909214));
#111707=CARTESIAN_POINT('Ctrl Pts',(-5.3899826994675,3.52567991513125,4.84877164802182));
#111708=CARTESIAN_POINT('Ctrl Pts',(-5.89631216715022,3.39148928109063,
4.21861747589908));
#111709=CARTESIAN_POINT('Ctrl Pts',(-5.88840743057512,3.39372739754531,
4.22957924344953));
#111710=CARTESIAN_POINT('Ctrl Pts',(-5.880502694,3.395965514,4.240541011));
#111711=CARTESIAN_POINT('Ctrl Pts',(-5.650279031,3.461150149,4.559800009));
#111712=CARTESIAN_POINT('Ctrl Pts',(-5.386844588,3.526458173,4.852257761));
#111713=CARTESIAN_POINT('Ctrl Pts',(-5.95334632703453,3.39148928109063,
4.56248011289003));
#111714=CARTESIAN_POINT('Ctrl Pts',(-5.94480021320308,3.39372739754531,
4.57354580586494));
#111715=CARTESIAN_POINT('Ctrl Pts',(-5.93625409937163,3.395965514,4.58461149883985));
#111716=CARTESIAN_POINT('Ctrl Pts',(-5.68735046899794,3.461150149,4.9068973012961));
#111717=CARTESIAN_POINT('Ctrl Pts',(-5.40501816371073,3.526458173,5.20034171740979));
#111718=CARTESIAN_POINT('Origin',(0.153139825867278,3.48214326136743,-0.128049668617121));
#111719=CARTESIAN_POINT('Ctrl Pts',(-6.30865232500001,3.526465848,3.572590914));
#111720=CARTESIAN_POINT('Ctrl Pts',(-6.112878915,3.460723853,3.918296989));
#111721=CARTESIAN_POINT('Ctrl Pts',(-5.880502694,3.395965514,4.240541011));
#111722=CARTESIAN_POINT('Ctrl Pts',(-6.643886303,3.526465848,3.479766486));
#111723=CARTESIAN_POINT('Ctrl Pts',(-6.453199552,3.460723853,3.843842954));
#111724=CARTESIAN_POINT('Ctrl Pts',(-6.223872212,3.395965514,4.184903187));
#111725=CARTESIAN_POINT('',(-6.3063104754868,3.52567991541429,3.57672310566886));
#111726=CARTESIAN_POINT('Origin',(0.176399700344673,3.62492144098057,-0.0810860420705356));
#111727=CARTESIAN_POINT('Ctrl Pts',(-6.52348320097803,3.48629831885008,
3.70056305449003));
#111728=CARTESIAN_POINT('Ctrl Pts',(-6.48727037534097,3.4925460152164,3.6798707673355));
#111729=CARTESIAN_POINT('Ctrl Pts',(-6.45104823951126,3.49894654286907,
3.65919310715012));
#111730=CARTESIAN_POINT('Ctrl Pts',(-6.3786699219615,3.51206280606079,3.6179189850791));
#111731=CARTESIAN_POINT('Ctrl Pts',(-6.34247195938134,3.51878610651248,
3.59729869452434));
#111732=CARTESIAN_POINT('Ctrl Pts',(-6.30631047486904,3.52567991512919,
3.57672310798306));
#111733=CARTESIAN_POINT('Ctrl Pts',(-6.66533772140166,3.39148928113425,
2.85245572182119));
#111734=CARTESIAN_POINT('Ctrl Pts',(-6.65997424920077,3.39372739756712,
2.86486049391057));
#111735=CARTESIAN_POINT('Ctrl Pts',(-6.654610777,3.395965514,2.877265266));
#111736=CARTESIAN_POINT('Ctrl Pts',(-6.49840086199999,3.461150149,3.238551448));
#111737=CARTESIAN_POINT('Ctrl Pts',(-6.303995142,3.526458173,3.580802319));
#111738=CARTESIAN_POINT('Ctrl Pts',(-6.7949587564644,3.39148928113426,3.17601838304456));
#111739=CARTESIAN_POINT('Ctrl Pts',(-6.78899124297181,3.39372739756712,
3.18866252798933));
#111740=CARTESIAN_POINT('Ctrl Pts',(-6.78302372947929,3.395965514,3.20130667293414));
#111741=CARTESIAN_POINT('Ctrl Pts',(-6.60922124844986,3.461150149,3.56956453521738));
#111742=CARTESIAN_POINT('Ctrl Pts',(-6.39657159139355,3.526458173,3.91684148375792));
#111743=CARTESIAN_POINT('Origin',(0.177086448535619,3.48214322481508,-0.0921354177508632));
#111744=CARTESIAN_POINT('Ctrl Pts',(-6.92916098100001,3.526465848,2.132891956));
#111745=CARTESIAN_POINT('Ctrl Pts',(-6.812281231,3.460723853,2.512601111));
#111746=CARTESIAN_POINT('Ctrl Pts',(-6.654610777,3.395965514,2.877265266));
#111747=CARTESIAN_POINT('Ctrl Pts',(-7.236602866,3.526465848,1.970172316));
#111748=CARTESIAN_POINT('Ctrl Pts',(-7.128639944,3.460723853,2.366728893));
#111749=CARTESIAN_POINT('Ctrl Pts',(-6.977992019,3.395965514,2.749113927));
#111750=CARTESIAN_POINT('',(-6.92776218145326,3.52567991543165,2.13743096775294));
#111751=CARTESIAN_POINT('Origin',(0.18970668803777,3.6249214517105,-0.0412695740069899));
#111752=CARTESIAN_POINT('Ctrl Pts',(-7.16647945765255,3.48629831881963,
2.21168989111538));
#111753=CARTESIAN_POINT('Ctrl Pts',(-7.12666503765092,3.49254601519576,
2.19926606514368));
#111754=CARTESIAN_POINT('Ctrl Pts',(-7.08684466969436,3.49894654283194,
2.18685852563207));
#111755=CARTESIAN_POINT('Ctrl Pts',(-7.00728580086712,3.51206280605708,
2.16210856821299));
#111756=CARTESIAN_POINT('Ctrl Pts',(-6.96750137362573,3.51878610653685,
2.14975186042951));
#111757=CARTESIAN_POINT('Ctrl Pts',(-6.92776218168722,3.52567991519186,
2.13743096977317));
#111758=CARTESIAN_POINT('Ctrl Pts',(-7.12269949194841,3.39148928101336,
1.35291630750235));
#111759=CARTESIAN_POINT('Ctrl Pts',(-7.12012807397428,3.39372739750668,
1.36618405125118));
#111760=CARTESIAN_POINT('Ctrl Pts',(-7.11755665599999,3.395965514,1.379451795));
#111761=CARTESIAN_POINT('Ctrl Pts',(-7.042664691,3.461150149,1.765871821));
#111762=CARTESIAN_POINT('Ctrl Pts',(-6.92637789,3.526458173,2.141912539));
#111763=CARTESIAN_POINT('Ctrl Pts',(-7.31884646688559,3.39148928101336,
1.64104956198232));
#111764=CARTESIAN_POINT('Ctrl Pts',(-7.31573658786461,3.39372739750668,
1.65468093325028));
#111765=CARTESIAN_POINT('Ctrl Pts',(-7.31262670884364,3.395965514,1.66831230451831));
#111766=CARTESIAN_POINT('Ctrl Pts',(-7.22205218804404,3.461150149,2.06532289950126));
#111767=CARTESIAN_POINT('Ctrl Pts',(-7.08902844015172,3.526458173,2.45019409568168));
#111768=CARTESIAN_POINT('Origin',(0.192752513181269,3.48214325539603,-0.0519129632307747));
#111769=CARTESIAN_POINT('Ctrl Pts',(-7.22566977100001,3.526465848,0.593461341));
#111770=CARTESIAN_POINT('Ctrl Pts',(-7.193148849,3.460723853,0.989418798));
#111771=CARTESIAN_POINT('Ctrl Pts',(-7.117556656,3.395965514,1.379451795));
#111772=CARTESIAN_POINT('Ctrl Pts',(-7.49094392300001,3.526465848,0.368455079));
#111773=CARTESIAN_POINT('Ctrl Pts',(-7.470753056,3.460723853,0.77894922));
#111774=CARTESIAN_POINT('Ctrl Pts',(-7.405828674,3.395965514,1.184779155));
#111775=CARTESIAN_POINT('',(-7.22527942719966,3.52567991541072,0.598194933891261));
#111776=CARTESIAN_POINT('Origin',(0.194143031089954,3.62492147818242,0.000476651601998418));
#111777=CARTESIAN_POINT('Ctrl Pts',(-7.474379099935,3.48629831882758,0.619400567375752));
#111778=CARTESIAN_POINT('Ctrl Pts',(-7.43282476363648,3.49254601520315,
0.615826126927508));
#111779=CARTESIAN_POINT('Ctrl Pts',(-7.39126811926568,3.49894654288035,
0.612268870771432));
#111780=CARTESIAN_POINT('Ctrl Pts',(-7.3082487833973,3.51206280609374,0.605200358586718));
#111781=CARTESIAN_POINT('Ctrl Pts',(-7.26673816733997,3.5187861065218,0.601685019581434));
#111782=CARTESIAN_POINT('Ctrl Pts',(-7.22527942859502,3.52567991512498,
0.598194936057684));
#111783=CARTESIAN_POINT('Ctrl Pts',(-7.24701174985952,3.3914892810937,-0.209883968754185));
#111784=CARTESIAN_POINT('Ctrl Pts',(-7.2473526229297,3.39372739754685,-0.196373638877095));
#111785=CARTESIAN_POINT('Ctrl Pts',(-7.24769349600001,3.395965514,-0.182863309));
#111786=CARTESIAN_POINT('Ctrl Pts',(-7.257621347,3.461150149,0.21062199));
#111787=CARTESIAN_POINT('Ctrl Pts',(-7.224890905,3.526458173,0.60286931));
#111788=CARTESIAN_POINT('Ctrl Pts',(-7.50051305040811,3.3914892810937,0.0293470895752078));
#111789=CARTESIAN_POINT('Ctrl Pts',(-7.50040622050875,3.39372739754685,
0.0433282987454922));
#111790=CARTESIAN_POINT('Ctrl Pts',(-7.5002993906094,3.395965514,0.0573095079157767));
#111791=CARTESIAN_POINT('Ctrl Pts',(-7.49718799397627,3.461150149,0.464509059725247));
#111792=CARTESIAN_POINT('Ctrl Pts',(-7.45001019763175,3.526458173,0.868978355344271));
#111793=CARTESIAN_POINT('Origin',(0.199405651581279,3.48214325129353,-0.00926317386774702));
#111794=CARTESIAN_POINT('Ctrl Pts',(-7.184314273,3.526465848,-0.973718867));
#111795=CARTESIAN_POINT('Ctrl Pts',(-7.237672821,3.460723853,-0.580027638));
#111796=CARTESIAN_POINT('Ctrl Pts',(-7.247693496,3.395965514,-0.182863309));
#111797=CARTESIAN_POINT('Ctrl Pts',(-7.395016767,3.526465848,-1.250490709));
#111798=CARTESIAN_POINT('Ctrl Pts',(-7.463542058,3.460723853,-0.845253253));
#111799=CARTESIAN_POINT('Ctrl Pts',(-7.487377012,3.395965514,-0.434954574));
#111800=CARTESIAN_POINT('',(-7.18495063795781,3.52567991538893,-0.969012030082798));
#111801=CARTESIAN_POINT('Origin',(0.189501763583084,3.62492144712771,0.0422005216843591));
#111802=CARTESIAN_POINT('Ctrl Pts',(-7.43278508283957,3.48629831884151,
-1.00185123952923));
#111803=CARTESIAN_POINT('Ctrl Pts',(-7.39143386477356,3.49254601521193,
-0.996409157496579));
#111804=CARTESIAN_POINT('Ctrl Pts',(-7.35008408696199,3.49894654284543,
-0.990949796784443));
#111805=CARTESIAN_POINT('Ctrl Pts',(-7.2674861758617,3.5120628060405,-0.980006347682485));
#111806=CARTESIAN_POINT('Ctrl Pts',(-7.22619036093362,3.51878610646488,
-0.974515944472787));
#111807=CARTESIAN_POINT('Ctrl Pts',(-7.18495063964874,3.52567991506207,
-0.969012028304349));
#111808=CARTESIAN_POINT('Ctrl Pts',(-7.03246179338903,3.39148928094506,
-1.76287030428815));
#111809=CARTESIAN_POINT('Ctrl Pts',(-7.03569901869452,3.39372739747253,
-1.74974911564411));
#111810=CARTESIAN_POINT('Ctrl Pts',(-7.03893624400001,3.395965514,-1.736627927));
#111811=CARTESIAN_POINT('Ctrl Pts',(-7.13321969499999,3.461150149,-1.354476291));
#111812=CARTESIAN_POINT('Ctrl Pts',(-7.185576052,3.526458173,-0.964363417));
#111813=CARTESIAN_POINT('Ctrl Pts',(-7.33146397982515,3.39148928094506,
-1.5837276227993));
#111814=CARTESIAN_POINT('Ctrl Pts',(-7.33436519435894,3.39372739747253,
-1.57005032079391));
#111815=CARTESIAN_POINT('Ctrl Pts',(-7.33726640889262,3.395965514,-1.5563730187886));
#111816=CARTESIAN_POINT('Ctrl Pts',(-7.42176362256031,3.461150149,-1.15802470758192));
#111817=CARTESIAN_POINT('Ctrl Pts',(-7.46263775903074,3.526458173,-0.752869847804082));
#111818=CARTESIAN_POINT('Origin',(0.196735211445208,3.482143250559,0.0338197687897776));
#111819=CARTESIAN_POINT('Ctrl Pts',(-6.807028224,3.526465848,-2.495369062));
#111820=CARTESIAN_POINT('Ctrl Pts',(-6.943771255,3.460723853,-2.122352626));
#111821=CARTESIAN_POINT('Ctrl Pts',(-7.038936244,3.395965514,-1.736627927));
#111822=CARTESIAN_POINT('Ctrl Pts',(-6.953306846,3.526465848,-2.810964941));
#111823=CARTESIAN_POINT('Ctrl Pts',(-7.107344128,3.460723853,-2.429932623));
#111824=CARTESIAN_POINT('Ctrl Pts',(-7.218823922,3.395965514,-2.03435031));
#111825=CARTESIAN_POINT('',(-6.8086615418157,3.52567991540629,-2.49090906873649));
#111826=CARTESIAN_POINT('Origin',(0.175999427407891,3.62492148308023,0.0819511757576769));
#111827=CARTESIAN_POINT('Ctrl Pts',(-7.04364229597215,3.48629831884724,
-2.57625759581233));
#111828=CARTESIAN_POINT('Ctrl Pts',(-7.00442773317179,3.49254601521909,
-2.56205345706564));
#111829=CARTESIAN_POINT('Ctrl Pts',(-6.96521829159601,3.49894654281944,
-2.54783275332507));
#111830=CARTESIAN_POINT('Ctrl Pts',(-6.88690399178184,3.51206280604993,
-2.51938904670169));
#111831=CARTESIAN_POINT('Ctrl Pts',(-6.84775392418869,3.51878610654272,
-2.50514962649814));
#111832=CARTESIAN_POINT('Ctrl Pts',(-6.80866154374564,3.52567991521619,
-2.49090906776779));
#111833=CARTESIAN_POINT('Ctrl Pts',(-6.48908173905949,3.39148928095608,
-3.23342678352247));
#111834=CARTESIAN_POINT('Ctrl Pts',(-6.49506394752967,3.39372739747804,
-3.22130826876123));
#111835=CARTESIAN_POINT('Ctrl Pts',(-6.50104615600001,3.395965514,-3.209189754));
#111836=CARTESIAN_POINT('Ctrl Pts',(-6.675276618,3.461150149,-2.856240766));
#111837=CARTESIAN_POINT('Ctrl Pts',(-6.810271649,3.526458173,-2.486503584));
#111838=CARTESIAN_POINT('Ctrl Pts',(-6.81960380219367,3.39148928095609,
-3.12274899055064));
#111839=CARTESIAN_POINT('Ctrl Pts',(-6.8253774035498,3.39372739747804,-3.11001513166759));
#111840=CARTESIAN_POINT('Ctrl Pts',(-6.83115100490594,3.395965514,-3.0972812727845));
#111841=CARTESIAN_POINT('Ctrl Pts',(-6.99930583212015,3.461150149,-2.72641052709717));
#111842=CARTESIAN_POINT('Ctrl Pts',(-7.12632067321713,3.526458173,-2.33951469307182));
#111843=CARTESIAN_POINT('Origin',(0.184865071285664,3.48214320604127,0.0753211970402862));
#111844=CARTESIAN_POINT('Ctrl Pts',(-6.11145310100001,3.526465848,-3.900338574));
#111845=CARTESIAN_POINT('Ctrl Pts',(-6.325186664,3.460723853,-3.565438765));
#111846=CARTESIAN_POINT('Ctrl Pts',(-6.50104615600001,3.395965514,-3.209189754));
#111847=CARTESIAN_POINT('Ctrl Pts',(-6.186468026,3.526465848,-4.240001576));
#111848=CARTESIAN_POINT('Ctrl Pts',(-6.418814686,3.460723853,-3.900991045));
#111849=CARTESIAN_POINT('Ctrl Pts',(-6.612726649,3.395965514,-3.538622086));
#111850=CARTESIAN_POINT('',(-6.11400699950171,3.52567991541422,-3.89633396843858));
#111851=CARTESIAN_POINT('Origin',(0.15426755881971,3.62492150645954,0.117869865155411));
#111852=CARTESIAN_POINT('Ctrl Pts',(-6.32514662409161,3.48629831884354,
-4.03020100952011));
#111853=CARTESIAN_POINT('Ctrl Pts',(-6.28990234594227,3.49254601521795,
-4.00789898382161));
#111854=CARTESIAN_POINT('Ctrl Pts',(-6.25466663006605,3.49894654285478,
-3.9855818812002));
#111855=CARTESIAN_POINT('Ctrl Pts',(-6.18429783112566,3.51206280607743,
-3.94096791317394));
#111856=CARTESIAN_POINT('Ctrl Pts',(-6.14912412478399,3.51878610654907,
-3.9186452955183));
#111857=CARTESIAN_POINT('Ctrl Pts',(-6.11400700156399,3.52567991519606,
-3.89633396700649));
#111858=CARTESIAN_POINT('Ctrl Pts',(-5.64227943465134,3.39148928097793,
-4.55279182018316));
#111859=CARTESIAN_POINT('Ctrl Pts',(-5.65072690482569,3.39372739748896,
-4.54224262759158));
#111860=CARTESIAN_POINT('Ctrl Pts',(-5.659174375,3.395965514,-4.531693435));
#111861=CARTESIAN_POINT('Ctrl Pts',(-5.905205025,3.461150149,-4.224450597));
#111862=CARTESIAN_POINT('Ctrl Pts',(-6.116526512,3.526458173,-3.892377606));
#111863=CARTESIAN_POINT('Ctrl Pts',(-5.98886652980762,3.39148928097793,
-4.51575408564639));
#111864=CARTESIAN_POINT('Ctrl Pts',(-5.99724255079055,3.39372739748897,
-4.50455909097359));
#111865=CARTESIAN_POINT('Ctrl Pts',(-6.00561857177365,3.395965514,-4.49336409630081));
#111866=CARTESIAN_POINT('Ctrl Pts',(-6.24956828030756,3.461150149,-4.16731241937839));
#111867=CARTESIAN_POINT('Ctrl Pts',(-6.45678475223131,3.526458173,-3.81676643166149));
#111868=CARTESIAN_POINT('Origin',(0.164351554709367,3.48214325047369,0.113301003398428));
#111869=CARTESIAN_POINT('Ctrl Pts',(-5.130113223,3.526465848,-5.122932589));
#111870=CARTESIAN_POINT('Ctrl Pts',(-5.410843374,3.460723853,-4.841808949));
#111871=CARTESIAN_POINT('Ctrl Pts',(-5.659174375,3.395965514,-4.531693435));
#111872=CARTESIAN_POINT('Ctrl Pts',(-5.13035683600001,3.526465848,-5.470780451));
#111873=CARTESIAN_POINT('Ctrl Pts',(-5.430148604,3.460723853,-5.189643461));
#111874=CARTESIAN_POINT('Ctrl Pts',(-5.697425627,3.395965514,-4.877431827));
#111875=CARTESIAN_POINT('',(-5.13346828522413,3.52567991540396,-5.119570621364));
#111876=CARTESIAN_POINT('Origin',(0.125322351743835,3.62492145200994,0.148277099372972));
#111877=CARTESIAN_POINT('Ctrl Pts',(-5.31089412599478,3.48629831883356,
-5.29569670360672));
#111878=CARTESIAN_POINT('Ctrl Pts',(-5.2812681157569,3.49254601519222,-5.26633960900819));
#111879=CARTESIAN_POINT('Ctrl Pts',(-5.2516537084966,3.4989465428554,-5.23696963039118));
#111880=CARTESIAN_POINT('Ctrl Pts',(-5.19252077726191,3.51206280604437,
-5.17827150053571));
#111881=CARTESIAN_POINT('Ctrl Pts',(-5.16296811547869,3.51878610651194,
-5.14890946606444));
#111882=CARTESIAN_POINT('Ctrl Pts',(-5.1334682871504,3.52567991514279,-5.11957062045771));
#111883=CARTESIAN_POINT('Ctrl Pts',(-4.53165041690712,3.39148928120598,
-5.65927337102999));
#111884=CARTESIAN_POINT('Ctrl Pts',(-4.54216815395354,3.39372739760299,
-5.65078676951494));
#111885=CARTESIAN_POINT('Ctrl Pts',(-4.552685891,3.395965514,-5.64230016800001));
#111886=CARTESIAN_POINT('Ctrl Pts',(-4.859012609,3.461150149,-5.395129814));
#111887=CARTESIAN_POINT('Ctrl Pts',(-5.136779394,3.526458173,-5.116248377));
#111888=CARTESIAN_POINT('Ctrl Pts',(-4.87809651566209,3.39148928120598,
-5.69760753822724));
#111889=CARTESIAN_POINT('Ctrl Pts',(-4.88868330231097,3.39372739760299,
-5.68847487366667));
#111890=CARTESIAN_POINT('Ctrl Pts',(-4.89927008895973,3.395965514,-5.67934220910622));
#111891=CARTESIAN_POINT('Ctrl Pts',(-5.20760786104525,3.461150149,-5.41335541469938));
#111892=CARTESIAN_POINT('Ctrl Pts',(-5.4853367528461,3.526458173,-5.11555041405223));
#111893=CARTESIAN_POINT('Origin',(0.136152707977599,3.48214322157363,0.145982787016208));
#111894=CARTESIAN_POINT('Ctrl Pts',(-3.908894953,3.526465848,-6.10598397));
#111895=CARTESIAN_POINT('Ctrl Pts',(-4.243495061,3.460723853,-5.89178152900001));
#111896=CARTESIAN_POINT('Ctrl Pts',(-4.552685891,3.395965514,-5.642300168));
#111897=CARTESIAN_POINT('Ctrl Pts',(-3.834355862,3.526465848,-6.445751711));
#111898=CARTESIAN_POINT('Ctrl Pts',(-4.187574808,3.460723853,-6.235633917));
#111899=CARTESIAN_POINT('Ctrl Pts',(-4.51571931500001,3.395965514,-5.988178277));
#111900=CARTESIAN_POINT('',(-3.9128942992225,3.52567991540626,-6.10342184278223));
#111901=CARTESIAN_POINT('Origin',(0.0905172887038647,3.62492145983665,0.171751205630448));
#111902=CARTESIAN_POINT('Ctrl Pts',(-4.04831012087657,3.48629831884072,
-6.31357150580349));
#111903=CARTESIAN_POINT('Ctrl Pts',(-4.02568765781779,3.49254601519901,
-6.27853204729132));
#111904=CARTESIAN_POINT('Ctrl Pts',(-4.00307929618703,3.49894654285463,
-6.24348250033077));
#111905=CARTESIAN_POINT('Ctrl Pts',(-3.95794722285298,3.51206280605495,
-6.17344486789823));
#111906=CARTESIAN_POINT('Ctrl Pts',(-3.93539745539643,3.51878610652987,
-6.13841635280557));
#111907=CARTESIAN_POINT('Ctrl Pts',(-3.91289430129605,3.52567991517878,
-6.10342184208375));
#111908=CARTESIAN_POINT('Ctrl Pts',(-3.20912646051089,3.391489281171,-6.50113358893938));
#111909=CARTESIAN_POINT('Ctrl Pts',(-3.22122266725546,3.3937273975855,-6.49510640196969));
#111910=CARTESIAN_POINT('Ctrl Pts',(-3.233318874,3.395965514,-6.489079215));
#111911=CARTESIAN_POINT('Ctrl Pts',(-3.585618163,3.461150149,-6.313538756));
#111912=CARTESIAN_POINT('Ctrl Pts',(-3.91684218,3.526458173,-6.100889061));
#111913=CARTESIAN_POINT('Ctrl Pts',(-3.53923212929024,3.39148928117102,
-6.61304719478717));
#111914=CARTESIAN_POINT('Ctrl Pts',(-3.5515346557487,3.3937273975855,-6.60640389301607));
#111915=CARTESIAN_POINT('Ctrl Pts',(-3.56383718220717,3.395965514,-6.59976059124494));
#111916=CARTESIAN_POINT('Ctrl Pts',(-3.92214548626916,3.461150149,-6.40627592782903));
#111917=CARTESIAN_POINT('Ctrl Pts',(-4.25740050355601,3.526458173,-6.175136944924));
#111918=CARTESIAN_POINT('Origin',(0.101587567894683,3.48214325638124,0.171838632591572));
#111919=CARTESIAN_POINT('Ctrl Pts',(-2.504901099,3.526465848,-6.803526327));
#111920=CARTESIAN_POINT('Ctrl Pts',(-2.877725636,3.460723853,-6.666260952));
#111921=CARTESIAN_POINT('Ctrl Pts',(-3.233318874,3.395965514,-6.489079215));
#111922=CARTESIAN_POINT('Ctrl Pts',(-2.35906467,3.526465848,-7.119326786));
#111923=CARTESIAN_POINT('Ctrl Pts',(-2.749194668,3.460723853,-6.99005306100001));
#111924=CARTESIAN_POINT('Ctrl Pts',(-3.122862986,3.395965514,-6.81892416500001));
#111925=CARTESIAN_POINT('',(-2.50935772461912,3.5256799154024,-6.80188384143029));
#111926=CARTESIAN_POINT('Origin',(0.0514794809429503,3.62492147913838,0.187194024079387));
#111927=CARTESIAN_POINT('Ctrl Pts',(-2.59643163413031,3.48629831882752,
-7.03623072135717));
#111928=CARTESIAN_POINT('Ctrl Pts',(-2.58187051952427,3.49254601518489,
-6.99714730511123));
#111929=CARTESIAN_POINT('Ctrl Pts',(-2.56732534538742,3.49894654282687,
-6.95805706773302));
#111930=CARTESIAN_POINT('Ctrl Pts',(-2.53830445549345,3.51206280601471,
-6.87995481461204));
#111931=CARTESIAN_POINT('Ctrl Pts',(-2.5238119843407,3.51878610648465,-6.84089771329479));
#111932=CARTESIAN_POINT('Ctrl Pts',(-2.50935772681528,3.52567991512012,
-6.80188384184327));
#111933=CARTESIAN_POINT('Ctrl Pts',(-1.73654731746914,3.39148928114318,
-7.03900802661295));
#111934=CARTESIAN_POINT('Ctrl Pts',(-1.74965638873457,3.39372739757159,
-7.03572207880648));
#111935=CARTESIAN_POINT('Ctrl Pts',(-1.76276546,3.395965514,-7.032436131));
#111936=CARTESIAN_POINT('Ctrl Pts',(-2.144564197,3.461150149,-6.936733644));
#111937=CARTESIAN_POINT('Ctrl Pts',(-2.51375778,3.526458173,-6.800258953));
#111938=CARTESIAN_POINT('Ctrl Pts',(-2.03487718227089,3.39148928114319,
-7.2192681159125));
#111939=CARTESIAN_POINT('Ctrl Pts',(-2.04832019609804,3.39372739757159,
-7.21542481033627));
#111940=CARTESIAN_POINT('Ctrl Pts',(-2.06176320992517,3.395965514,-7.21158150475991));
#111941=CARTESIAN_POINT('Ctrl Pts',(-2.45328794853941,3.461150149,-7.09964609871575));
#111942=CARTESIAN_POINT('Ctrl Pts',(-2.83039293831108,3.526458173,-6.94598093486384));
#111943=CARTESIAN_POINT('Origin',(0.0622722465864306,3.48214326322917,0.189659333558916));
#111944=CARTESIAN_POINT('Ctrl Pts',(-0.983780854,3.526465848,-7.182943354));
#111945=CARTESIAN_POINT('Ctrl Pts',(-1.377396959,3.460723853,-7.129033422));
#111946=CARTESIAN_POINT('Ctrl Pts',(-1.76276546,3.395965514,-7.032436131));
#111947=CARTESIAN_POINT('Ctrl Pts',(-0.773466236,3.526465848,-7.460010052));
#111948=CARTESIAN_POINT('Ctrl Pts',(-1.182265241,3.460723853,-7.417625092));
#111949=CARTESIAN_POINT('Ctrl Pts',(-1.583985056,3.395965514,-7.330824738));
#111950=CARTESIAN_POINT('',(-0.988486371605558,3.5256799154039,-7.18229731209713));
#111951=CARTESIAN_POINT('Origin',(0.0100347628190417,3.62492146056771,0.19388418036362));
#111952=CARTESIAN_POINT('Ctrl Pts',(-1.02314688972635,3.48629831883303,
-7.42988360828838));
#111953=CARTESIAN_POINT('Ctrl Pts',(-1.0173279850979,3.49254601520365,-7.388583731331));
#111954=CARTESIAN_POINT('Ctrl Pts',(-1.01152611461239,3.49894654284631,
-7.34728061954439));
#111955=CARTESIAN_POINT('Ctrl Pts',(-0.999973392745211,3.51206280605282,
-7.26476572022423));
#111956=CARTESIAN_POINT('Ctrl Pts',(-0.994215869778384,3.51878610652593,
-7.22350629936899));
#111957=CARTESIAN_POINT('Ctrl Pts',(-0.988486373856841,3.52567991516553,
-7.18229731247012));
#111958=CARTESIAN_POINT('Ctrl Pts',(-0.182769151460141,3.39148928109655,
-7.24774627167997));
#111959=CARTESIAN_POINT('Ctrl Pts',(-0.196278121730071,3.39372739754827,
-7.24735521034));
#111960=CARTESIAN_POINT('Ctrl Pts',(-0.209787092,3.395965514,-7.24696414899999));
#111961=CARTESIAN_POINT('Ctrl Pts',(-0.603232793,3.461150149,-7.235574576));
#111962=CARTESIAN_POINT('Ctrl Pts',(-0.993132859,3.526458173,-7.181656294));
#111963=CARTESIAN_POINT('Ctrl Pts',(-0.435373639031206,3.39148928109655,
-7.4879240829896));
#111964=CARTESIAN_POINT('Ctrl Pts',(-0.449328559914331,3.39372739754827,
-7.48706048234389));
#111965=CARTESIAN_POINT('Ctrl Pts',(-0.463283480797445,3.395965514,-7.4861968816982));
#111966=CARTESIAN_POINT('Ctrl Pts',(-0.869717392453809,3.461150149,-7.46104470839123));
#111967=CARTESIAN_POINT('Ctrl Pts',(-1.27103934506535,3.526458173,-7.39203857617559));
#111968=CARTESIAN_POINT('Origin',(0.0200451930806927,3.48214323715933,0.198611868377269));
#111969=CARTESIAN_POINT('Ctrl Pts',(0.58333989,3.526465848,-7.226493934));
#111970=CARTESIAN_POINT('Ctrl Pts',(0.18733727,3.460723853,-7.258460213));
#111971=CARTESIAN_POINT('Ctrl Pts',(-0.209787092,3.395965514,-7.246964149));
#111972=CARTESIAN_POINT('Ctrl Pts',(0.84829862,3.526465848,-7.45187154));
#111973=CARTESIAN_POINT('Ctrl Pts',(0.439945595,3.460723853,-7.498357219));
#111974=CARTESIAN_POINT('Ctrl Pts',(0.028958256,3.395965514,-7.499944094));
#111975=CARTESIAN_POINT('',(0.578605504968755,3.52567991539871,-7.2268745428914));
#111976=CARTESIAN_POINT('Origin',(-0.0318792103603806,3.62492147346623,
0.191508480028005));
#111977=CARTESIAN_POINT('Ctrl Pts',(0.5979790664113,3.48629831884111,-7.47612339587756));
#111978=CARTESIAN_POINT('Ctrl Pts',(0.594783675462233,3.49254601521968,
-7.4345381945661));
#111979=CARTESIAN_POINT('Ctrl Pts',(0.591570953208007,3.49894654283551,
-7.39295349612528));
#111980=CARTESIAN_POINT('Ctrl Pts',(0.585115314289095,3.51206280605377,
-7.30988425562773));
#111981=CARTESIAN_POINT('Ctrl Pts',(0.581868673498221,3.51878610651907,
-7.26835175999189));
#111982=CARTESIAN_POINT('Ctrl Pts',(0.578605502673376,3.52567991515746,
-7.2268745441991));
#111983=CARTESIAN_POINT('Ctrl Pts',(1.37955509719461,3.39148928095979,-7.11758795639031));
#111984=CARTESIAN_POINT('Ctrl Pts',(1.36627789209731,3.3937273974799,-7.1201100671952));
#111985=CARTESIAN_POINT('Ctrl Pts',(1.353000687,3.395965514,-7.122632178));
#111986=CARTESIAN_POINT('Ctrl Pts',(0.966305106,3.461150149,-7.196088082));
#111987=CARTESIAN_POINT('Ctrl Pts',(0.57392985,3.526458173,-7.227247369));
#111988=CARTESIAN_POINT('Ctrl Pts',(1.18448749190377,3.39148928095979,-7.40645304119305));
#111989=CARTESIAN_POINT('Ctrl Pts',(1.17067318028301,3.3937273974799,-7.40860952663753));
#111990=CARTESIAN_POINT('Ctrl Pts',(1.15685886866229,3.395965514,-7.41076601208203));
#111991=CARTESIAN_POINT('Ctrl Pts',(0.754520182233867,3.461150149,-7.47357316055637));
#111992=CARTESIAN_POINT('Ctrl Pts',(0.347746635845621,3.526458173,-7.49245271025973));
#111993=CARTESIAN_POINT('Origin',(-0.0231191456030383,3.48214324217312,
0.19827763683482));
#111994=CARTESIAN_POINT('Ctrl Pts',(2.12318431,3.526465848,-6.932141688));
#111995=CARTESIAN_POINT('Ctrl Pts',(1.743311816,3.460723853,-7.048489472));
#111996=CARTESIAN_POINT('Ctrl Pts',(1.353000687,3.395965514,-7.122632178));
#111997=CARTESIAN_POINT('Ctrl Pts',(2.430397975,3.526465848,-7.095291797));
#111998=CARTESIAN_POINT('Ctrl Pts',(2.041585064,3.460723853,-7.228474496));
#111999=CARTESIAN_POINT('Ctrl Pts',(1.640547511,3.395965514,-7.3183744));
#112000=CARTESIAN_POINT('',(2.11864243188285,3.52567991541344,-6.9335311516546));
#112001=CARTESIAN_POINT('Origin',(-0.0723025751553144,3.6249214524772,0.18017811992764));
#112002=CARTESIAN_POINT('Ctrl Pts',(2.19114418540924,3.48629831884211,-7.17278796232453));
#112003=CARTESIAN_POINT('Ctrl Pts',(2.17908391196435,3.49254601521138,-7.13286191455645));
#112004=CARTESIAN_POINT('Ctrl Pts',(2.16700682047426,3.4989465428543,-7.09294008337225));
#112005=CARTESIAN_POINT('Ctrl Pts',(2.14284467989402,3.51206280606465,-7.01320072698359));
#112006=CARTESIAN_POINT('Ctrl Pts',(2.13074568506188,3.5187861065394,-6.97333716963481));
#112007=CARTESIAN_POINT('Ctrl Pts',(2.11864243027881,3.52567991518217,-6.93353115313885));
#112008=CARTESIAN_POINT('Ctrl Pts',(2.87737288140405,3.3914892811314,-6.65461913858258));
#112009=CARTESIAN_POINT('Ctrl Pts',(2.86494826970199,3.3937273975657,-6.65993649029124));
#112010=CARTESIAN_POINT('Ctrl Pts',(2.852523658,3.395965514,-6.665253842));
#112011=CARTESIAN_POINT('Ctrl Pts',(2.490659652,3.461150149,-6.820120508));
#112012=CARTESIAN_POINT('Ctrl Pts',(2.114156238,3.526458173,-6.934900389));
#112013=CARTESIAN_POINT('Ctrl Pts',(2.74896330195076,3.39148928113139,-6.97866448862964));
#112014=CARTESIAN_POINT('Ctrl Pts',(2.73593554238889,3.3937273975657,-6.98374022506011));
#112015=CARTESIAN_POINT('Ctrl Pts',(2.72290778282702,3.395965514,-6.98881596149056));
#112016=CARTESIAN_POINT('Ctrl Pts',(2.34347723180972,3.461150149,-7.13664563715228));
#112017=CARTESIAN_POINT('Ctrl Pts',(1.95027237024044,3.526458173,-7.24252808155912));
#112018=CARTESIAN_POINT('Origin',(-0.065202394651328,3.48214328243972,0.188671929290466));
#112019=CARTESIAN_POINT('Ctrl Pts',(3.563750991,3.526465848,-6.313650202));
#112020=CARTESIAN_POINT('Ctrl Pts',(3.217771039,3.460723853,-6.50893919600001));
#112021=CARTESIAN_POINT('Ctrl Pts',(2.852523658,3.395965514,-6.66525384200001));
#112022=CARTESIAN_POINT('Ctrl Pts',(3.898854622,3.526465848,-6.406944095));
#112023=CARTESIAN_POINT('Ctrl Pts',(3.547762284,3.460723853,-6.620596339));
#112024=CARTESIAN_POINT('Ctrl Pts',(3.175426589,3.395965514,-6.794605653));
#112025=CARTESIAN_POINT('',(3.55961399279691,3.52567991539475,-6.31598355033359));
#112026=CARTESIAN_POINT('Origin',(-0.109345231367666,3.624921467088,0.160422896054845));
#112027=CARTESIAN_POINT('Ctrl Pts',(3.6818538378336,3.4862983188185,-6.53406093560932));
#112028=CARTESIAN_POINT('Ctrl Pts',(3.66149260672344,3.49254601520393,-6.49766093882917));
#112029=CARTESIAN_POINT('Ctrl Pts',(3.64111585723239,3.49894654284766,-6.46126867554383));
#112030=CARTESIAN_POINT('Ctrl Pts',(3.60037700929721,3.51206280607397,-6.38858772696084));
#112031=CARTESIAN_POINT('Ctrl Pts',(3.5799913957474,3.51878610651668,-6.35225708390216));
#112032=CARTESIAN_POINT('Ctrl Pts',(3.55961399137252,3.52567991513177,-6.31598355218538));
#112033=CARTESIAN_POINT('Ctrl Pts',(4.24064790842477,3.39148928092428,-5.8804877258907));
#112034=CARTESIAN_POINT('Ctrl Pts',(4.22965685021238,3.39372739746214,-5.88835168544536));
#112035=CARTESIAN_POINT('Ctrl Pts',(4.218665792,3.395965514,-5.896215645));
#112036=CARTESIAN_POINT('Ctrl Pts',(3.898553722,3.461150149,-6.125251678));
#112037=CARTESIAN_POINT('Ctrl Pts',(3.555527029,3.526458173,-6.318285174));
#112038=CARTESIAN_POINT('Ctrl Pts',(4.18490064530936,3.39148928092428,-6.22456133883201));
#112039=CARTESIAN_POINT('Ctrl Pts',(4.17326860031493,3.39372739746214,-6.23231899095407));
#112040=CARTESIAN_POINT('Ctrl Pts',(4.1616365553205,3.395965514,-6.24007664307597));
#112041=CARTESIAN_POINT('Ctrl Pts',(3.82285589111576,3.461150149,-6.46601649628232));
#112042=CARTESIAN_POINT('Ctrl Pts',(3.4616055353622,3.526458173,-6.6539508899692));
#112043=CARTESIAN_POINT('Origin',(-0.10423690204041,3.4821432418066,0.170244306811728));
#112044=CARTESIAN_POINT('Ctrl Pts',(4.837680637,3.526465848,-5.39993945));
#112045=CARTESIAN_POINT('Ctrl Pts',(4.541770865,3.460723853,-5.66503815800001));
#112046=CARTESIAN_POINT('Ctrl Pts',(4.218665792,3.395965514,-5.896215645));
#112047=CARTESIAN_POINT('Ctrl Pts',(5.18500516,3.526465848,-5.419014808));
#112048=CARTESIAN_POINT('Ctrl Pts',(4.88805008300001,3.460723853,-5.703146456));
#112049=CARTESIAN_POINT('Ctrl Pts',(4.561826248,3.395965514,-5.953128697));
#112050=CARTESIAN_POINT('',(4.83414195952737,3.52567991540482,-5.40310757827952));
#112051=CARTESIAN_POINT('Origin',(-0.1412747507766,3.62492147087993,0.133166016273699));
#112052=CARTESIAN_POINT('Ctrl Pts',(5.00040409687358,3.4862983188267,-5.58980848170412));
#112053=CARTESIAN_POINT('Ctrl Pts',(4.97269397672632,3.49254601519868,-5.55863655952063));
#112054=CARTESIAN_POINT('Ctrl Pts',(4.94497036347985,3.49894654282933,-5.527475526028));
#112055=CARTESIAN_POINT('Ctrl Pts',(4.88955971170044,3.51206280603054,-5.46525146593907));
#112056=CARTESIAN_POINT('Ctrl Pts',(4.86184068816916,3.51878610645722,-5.43415251760096));
#112057=CARTESIAN_POINT('Ctrl Pts',(4.83414195911805,3.5256799150601,-5.40310758066948));
#112058=CARTESIAN_POINT('Ctrl Pts',(5.40563495190804,3.39148928096534,-4.83139124279981));
#112059=CARTESIAN_POINT('Ctrl Pts',(5.39659137745394,3.39372739748267,-4.84143409989997));
#112060=CARTESIAN_POINT('Ctrl Pts',(5.38754780300001,3.395965514,-4.851476957));
#112061=CARTESIAN_POINT('Ctrl Pts',(5.124155752,3.461150149,-5.143972888));
#112062=CARTESIAN_POINT('Ctrl Pts',(4.830645328,3.526458173,-5.406233968));
#112063=CARTESIAN_POINT('Ctrl Pts',(5.42515668503526,3.39148928096534,-5.17940461951063));
#112064=CARTESIAN_POINT('Ctrl Pts',(5.41546425676381,3.39372739748267,-5.18948144778356));
#112065=CARTESIAN_POINT('Ctrl Pts',(5.40577182849223,3.395965514,-5.19955827605655));
#112066=CARTESIAN_POINT('Ctrl Pts',(5.12348205749383,3.461150149,-5.49304360974957));
#112067=CARTESIAN_POINT('Ctrl Pts',(4.8110778735632,3.526458173,-5.7542423504641));
#112068=CARTESIAN_POINT('Origin',(-0.138397360011063,3.48214325877107,0.14385621190067));
#112069=CARTESIAN_POINT('Ctrl Pts',(5.885405712,3.526465848,-4.23373353));
#112070=CARTESIAN_POINT('Ctrl Pts',(5.653402532,3.460723853,-4.556246232));
#112071=CARTESIAN_POINT('Ctrl Pts',(5.387547803,3.395965514,-4.85147695700001));
#112072=CARTESIAN_POINT('Ctrl Pts',(6.22871062,3.526465848,-4.177698412));
#112073=CARTESIAN_POINT('Ctrl Pts',(5.999778092,3.460723853,-4.519023783));
#112074=CARTESIAN_POINT('Ctrl Pts',(5.734919982,3.395965514,-4.83329006));
#112075=CARTESIAN_POINT('',(5.8826308220411,3.52567991540452,-4.23758830006617));
#112076=CARTESIAN_POINT('Origin',(-0.166598778539352,3.62492148010577,0.0996829396709153));
#112077=CARTESIAN_POINT('Ctrl Pts',(6.08514101783682,3.48629831886233,-4.38418279590156));
#112078=CARTESIAN_POINT('Ctrl Pts',(6.0513777031033,3.49254601523024,-4.35969651263282));
#112079=CARTESIAN_POINT('Ctrl Pts',(6.01760355145017,3.49894654286214,-4.33522376406252));
#112080=CARTESIAN_POINT('Ctrl Pts',(5.95011203634992,3.51206280606942,-4.28636611987752));
#112081=CARTESIAN_POINT('Ctrl Pts',(5.91635571338162,3.51878610654161,-4.26195301803481));
#112082=CARTESIAN_POINT('Ctrl Pts',(5.88263082133316,3.52567991518665,-4.2375883020626));
#112083=CARTESIAN_POINT('Ctrl Pts',(6.31786051366746,3.39148928095982,-3.55638427523239));
#112084=CARTESIAN_POINT('Ctrl Pts',(6.31118729033379,3.39372739747991,-3.56813643711619));
#112085=CARTESIAN_POINT('Ctrl Pts',(6.304514067,3.395965514,-3.579888599));
#112086=CARTESIAN_POINT('Ctrl Pts',(6.11015795399999,3.461150149,-3.922167643));
#112087=CARTESIAN_POINT('Ctrl Pts',(5.879888021,3.526458173,-4.241393269));
#112088=CARTESIAN_POINT('Ctrl Pts',(6.41173842758416,3.39148928095982,-3.89206469702066));
#112089=CARTESIAN_POINT('Ctrl Pts',(6.40443882310263,3.39372739747991,-3.90398952023208));
#112090=CARTESIAN_POINT('Ctrl Pts',(6.39713921862109,3.395965514,-3.91591434344356));
#112091=CARTESIAN_POINT('Ctrl Pts',(6.18453989704745,3.461150149,-4.26322210937187));
#112092=CARTESIAN_POINT('Ctrl Pts',(5.93558955777851,3.526458173,-4.58547183331436));
#112093=CARTESIAN_POINT('Origin',(-0.166086502363476,3.48214323145688,0.110741551565392));
#112094=CARTESIAN_POINT('Ctrl Pts',(6.657935758,3.526465848,-2.869562936));
#112095=CARTESIAN_POINT('Ctrl Pts',(6.500687381,3.460723853,-3.234409296));
#112096=CARTESIAN_POINT('Ctrl Pts',(6.30451406700001,3.395965514,-3.579888599));
#112097=CARTESIAN_POINT('Ctrl Pts',(6.981168493,3.526465848,-2.741037481));
#112098=CARTESIAN_POINT('Ctrl Pts',(6.830963147,3.460723853,-3.123596581));
#112099=CARTESIAN_POINT('Ctrl Pts',(6.639855232,3.395965514,-3.487452151));
#112100=CARTESIAN_POINT('',(6.65605440469573,3.52567991541251,-2.87392410309611));
#112101=CARTESIAN_POINT('Origin',(-0.184132620657596,3.62492144599365,0.0615385729235612));
#112102=CARTESIAN_POINT('Ctrl Pts',(6.88534350778262,3.48629831885202,-2.97355759548524));
#112103=CARTESIAN_POINT('Ctrl Pts',(6.84710573362347,3.49254601520656,-2.95690190251033));
#112104=CARTESIAN_POINT('Ctrl Pts',(6.80886028528215,3.49894654285973,-2.94026175731254));
#112105=CARTESIAN_POINT('Ctrl Pts',(6.7324437352632,3.5120628060585,-2.90705505827975));
#112106=CARTESIAN_POINT('Ctrl Pts',(6.69422852120966,3.51878610653489,-2.89046933272017));
#112107=CARTESIAN_POINT('Ctrl Pts',(6.65605440477926,3.52567991518518,-2.8739241051104));
#112108=CARTESIAN_POINT('Ctrl Pts',(6.93466993795907,3.39148928115785,-2.11508473291005));
#112109=CARTESIAN_POINT('Ctrl Pts',(6.93067909847946,3.39372739757893,-2.12799668095506));
#112110=CARTESIAN_POINT('Ctrl Pts',(6.926688259,3.395965514,-2.140908629));
#112111=CARTESIAN_POINT('Ctrl Pts',(6.810455961,3.461150149,-2.516966198));
#112112=CARTESIAN_POINT('Ctrl Pts',(6.654193685,3.526458173,-2.878229735));
#112113=CARTESIAN_POINT('Ctrl Pts',(7.09851440741408,3.39148928115785,-2.42273615647617));
#112114=CARTESIAN_POINT('Ctrl Pts',(7.09394894829047,3.39372739757893,-2.43595138255228));
#112115=CARTESIAN_POINT('Ctrl Pts',(7.08938348916687,3.395965514,-2.44916660862833));
#112116=CARTESIAN_POINT('Ctrl Pts',(6.95641552388255,3.461150149,-2.8340570817505));
#112117=CARTESIAN_POINT('Ctrl Pts',(6.78255967079351,3.526458173,-3.20228974984023));
#112118=CARTESIAN_POINT('Origin',(-0.186009880412594,3.48214322465404,0.0724488708943488));
#112119=CARTESIAN_POINT('Ctrl Pts',(7.119148127,3.526465848,-1.371214768));
#112120=CARTESIAN_POINT('Ctrl Pts',(7.044007313,3.460723853,-1.761334976));
#112121=CARTESIAN_POINT('Ctrl Pts',(6.926688259,3.395965514,-2.140908629));
#112122=CARTESIAN_POINT('Ctrl Pts',(7.407194687,3.526465848,-1.176208683));
#112123=CARTESIAN_POINT('Ctrl Pts',(7.342739956,3.460723853,-1.582113474));
#112124=CARTESIAN_POINT('Ctrl Pts',(7.23431823,3.395965514,-1.978544855));
#112125=CARTESIAN_POINT('',(7.11824828114541,3.52567991539768,-1.37587840931426));
#112126=CARTESIAN_POINT('Origin',(-0.193056728397172,3.62492146203427,0.0205167761913733));
#112127=CARTESIAN_POINT('Ctrl Pts',(7.36359498822141,3.48629831884877,-1.42389214575025));
#112128=CARTESIAN_POINT('Ctrl Pts',(7.32267071009219,3.49254601522387,-1.41584584484627));
#112129=CARTESIAN_POINT('Ctrl Pts',(7.28174227990182,3.49894654283125,-1.40781637803124));
#112130=CARTESIAN_POINT('Ctrl Pts',(7.19997384731184,3.51206280602885,-1.3918133327918));
#112131=CARTESIAN_POINT('Ctrl Pts',(7.15908664291011,3.51878610648578,-1.38383051380354));
#112132=CARTESIAN_POINT('Ctrl Pts',(7.11824828113933,3.52567991511134,-1.37587841117221));
#112133=CARTESIAN_POINT('Ctrl Pts',(7.22722190550165,3.39148928110903,-0.574886177936338));
#112134=CARTESIAN_POINT('Ctrl Pts',(7.22610005675088,3.39372739755452,-0.588354164468173));
#112135=CARTESIAN_POINT('Ctrl Pts',(7.224978208,3.395965514,-0.601822151));
#112136=CARTESIAN_POINT('Ctrl Pts',(7.192304617,3.461150149,-0.994074210999999));
#112137=CARTESIAN_POINT('Ctrl Pts',(7.117356647,3.526458173,-1.380483378));
#112138=CARTESIAN_POINT('Ctrl Pts',(7.45337174375708,3.39148928110902,-0.840123164237828));
#112139=CARTESIAN_POINT('Ctrl Pts',(7.45175390547908,3.39372739755452,-0.854010864550351));
#112140=CARTESIAN_POINT('Ctrl Pts',(7.45013606720119,3.395965514,-0.867898564862873));
#112141=CARTESIAN_POINT('Ctrl Pts',(7.40301689346605,3.461150149,-1.27237469374638));
#112142=CARTESIAN_POINT('Ctrl Pts',(7.31238483253964,3.526458173,-1.66937215709889));
#112143=CARTESIAN_POINT('Origin',(-0.197235680099412,3.48214320229941,0.0307684671072975));
#112144=CARTESIAN_POINT('Ctrl Pts',(7.247477043,3.526465848,0.191249878));
#112145=CARTESIAN_POINT('Ctrl Pts',(7.257957291,3.460723853,-0.20590259));
#112146=CARTESIAN_POINT('Ctrl Pts',(7.224978208,3.395965514,-0.601822151));
#112147=CARTESIAN_POINT('Ctrl Pts',(7.48686869,3.526465848,0.443618325));
#112148=CARTESIAN_POINT('Ctrl Pts',(7.511178407,3.460723853,0.033347501));
#112149=CARTESIAN_POINT('Ctrl Pts',(7.49051254899999,3.395965514,-0.377123002));
#112150=CARTESIAN_POINT('',(7.24760077907798,3.52567991540728,0.186501829924383));
#112151=CARTESIAN_POINT('Origin',(-0.192953488755793,3.62492145760987,-0.0214644009633342));
#112152=CARTESIAN_POINT('Ctrl Pts',(7.49753295086236,3.48629831882052,0.192352917068684));
#112153=CARTESIAN_POINT('Ctrl Pts',(7.45583574284632,3.49254601518459,0.191413589910313));
#112154=CARTESIAN_POINT('Ctrl Pts',(7.41413809829101,3.49894654284407,0.190456929640105));
#112155=CARTESIAN_POINT('Ctrl Pts',(7.33084118470806,3.51206280604116,0.188508036656145));
#112156=CARTESIAN_POINT('Ctrl Pts',(7.28919383066968,3.51878610646118,0.187514681429563));
#112157=CARTESIAN_POINT('Ctrl Pts',(7.24760078045297,3.52567991505855,0.186501827635311));
#112158=CARTESIAN_POINT('Ctrl Pts',(7.18183700810298,3.39148928114563,0.992193416467413));
#112159=CARTESIAN_POINT('Ctrl Pts',(7.18363660655154,3.39372739757282,0.978799139733706));
#112160=CARTESIAN_POINT('Ctrl Pts',(7.185436205,3.395965514,0.965404863000001));
#112161=CARTESIAN_POINT('Ctrl Pts',(7.237849103,3.461150149,0.575299581));
#112162=CARTESIAN_POINT('Ctrl Pts',(7.247719923,3.526458173,0.181812848));
#112163=CARTESIAN_POINT('Ctrl Pts',(7.45971770060393,3.39148928114563,0.781773053476565));
#112164=CARTESIAN_POINT('Ctrl Pts',(7.46112313152643,3.39372739757282,0.76786225255639));
#112165=CARTESIAN_POINT('Ctrl Pts',(7.46252856244906,3.395965514,0.753951451636205));
#112166=CARTESIAN_POINT('Ctrl Pts',(7.5034614203627,3.461150149,0.348802519468901));
#112167=CARTESIAN_POINT('Ctrl Pts',(7.5002910056817,3.526458173,-0.0583965774921274));
#112168=CARTESIAN_POINT('Origin',(-0.19923832847399,3.48214324621981,-0.0123506811089137));
#112169=CARTESIAN_POINT('Ctrl Pts',(7.03692198700001,3.526465848,1.744771892));
#112170=CARTESIAN_POINT('Ctrl Pts',(7.132533254,3.460723853,1.359157572));
#112171=CARTESIAN_POINT('Ctrl Pts',(7.185436205,3.395965514,0.965404863));
#112172=CARTESIAN_POINT('Ctrl Pts',(7.216465034,3.526465848,2.042702233));
#112173=CARTESIAN_POINT('Ctrl Pts',(7.328402503,3.460723853,1.647249183));
#112174=CARTESIAN_POINT('Ctrl Pts',(7.39645882600001,3.395965514,1.241932705));
#112175=CARTESIAN_POINT('',(7.03806351988731,3.52567991539917,1.74016145083006));
#112176=CARTESIAN_POINT('Origin',(-0.18382809921942,3.62492146996118,-0.0624418681181543));
#112177=CARTESIAN_POINT('Ctrl Pts',(7.2808946056302,3.48629831885698,1.79960377156328));
#112178=CARTESIAN_POINT('Ctrl Pts',(7.24037418281053,3.49254601522146,1.78972273822684));
#112179=CARTESIAN_POINT('Ctrl Pts',(7.19985705962658,3.49894654290227,1.77982468312599));
#112180=CARTESIAN_POINT('Ctrl Pts',(7.11892653610697,3.51206280609361,1.76001497998509));
#112181=CARTESIAN_POINT('Ctrl Pts',(7.0784664161188,3.5187861065103,1.75009189878341));
#112182=CARTESIAN_POINT('Ctrl Pts',(7.03806352196428,3.52567991509905,1.74016144855234));
#112183=CARTESIAN_POINT('Ctrl Pts',(6.80063739414523,3.3914892811293,2.51287914801983));
#112184=CARTESIAN_POINT('Ctrl Pts',(6.80527429257269,3.39372739756465,2.50018488250989));
#112185=CARTESIAN_POINT('Ctrl Pts',(6.809911191,3.395965514,2.487490617));
#112186=CARTESIAN_POINT('Ctrl Pts',(6.944959809,3.461150149,2.117773005));
#112187=CARTESIAN_POINT('Ctrl Pts',(7.039187871,3.526458173,1.735607707));
#112188=CARTESIAN_POINT('Ctrl Pts',(7.11725554807386,3.39148928112931,2.36711443152031));
#112189=CARTESIAN_POINT('Ctrl Pts',(7.12161853183056,3.39372739756465,2.35383098346513));
#112190=CARTESIAN_POINT('Ctrl Pts',(7.12598151558714,3.395965514,2.34054753540996));
#112191=CARTESIAN_POINT('Ctrl Pts',(7.2530524307516,3.461150149,1.95367011503013));
#112192=CARTESIAN_POINT('Ctrl Pts',(7.33749190763702,3.526458173,1.55530956171755));
#112193=CARTESIAN_POINT('Origin',(-0.191925213453235,3.48214323319159,-0.0548922832923227));
#112194=CARTESIAN_POINT('Ctrl Pts',(6.497328279,3.526465848,3.216710312));
#112195=CARTESIAN_POINT('Ctrl Pts',(6.673599888,3.460723853,2.860665037));
#112196=CARTESIAN_POINT('Ctrl Pts',(6.809911191,3.395965514,2.487490617));
#112197=CARTESIAN_POINT('Ctrl Pts',(6.608627494,3.526465848,3.546271655));
#112198=CARTESIAN_POINT('Ctrl Pts',(6.802958642,3.460723853,3.184127325));
#112199=CARTESIAN_POINT('Ctrl Pts',(6.956554908,3.395965514,2.802917018));
#112200=CARTESIAN_POINT('',(6.49943423274102,3.52567991543021,3.2124530563957));
#112201=CARTESIAN_POINT('Origin',(-0.166107150037931,3.62492145770722,-0.100499613472969));
#112202=CARTESIAN_POINT('Ctrl Pts',(6.72380972081418,3.4862983188088,3.32270715395699));
#112203=CARTESIAN_POINT('Ctrl Pts',(6.68636077307945,3.49254601517424,3.3043464405831));
#112204=CARTESIAN_POINT('Ctrl Pts',(6.64891870713739,3.49894654282947,3.28596981283343));
#112205=CARTESIAN_POINT('Ctrl Pts',(6.57413879475269,3.51206280603208,3.24922557947771));
#112206=CARTESIAN_POINT('Ctrl Pts',(6.536757778616,3.51878610650794,3.23083676461094));
#112207=CARTESIAN_POINT('Ctrl Pts',(6.49943423450968,3.5256799151533,3.21245305497855));
#112208=CARTESIAN_POINT('Ctrl Pts',(6.10144753459324,3.39148928110132,3.91606544530404));
#112209=CARTESIAN_POINT('Ctrl Pts',(6.10870491679661,3.39372739755066,3.90466476065205));
#112210=CARTESIAN_POINT('Ctrl Pts',(6.115962299,3.395965514,3.893264076));
#112211=CARTESIAN_POINT('Ctrl Pts',(6.327331913,3.461150149,3.561221716));
#112212=CARTESIAN_POINT('Ctrl Pts',(6.501511218,3.526458173,3.208247479));
#112213=CARTESIAN_POINT('Ctrl Pts',(6.44199843683067,3.39148928110133,3.84177217006765));
#112214=CARTESIAN_POINT('Ctrl Pts',(6.44911496517995,3.39372739755066,3.82973719410252));
#112215=CARTESIAN_POINT('Ctrl Pts',(6.45623149352924,3.395965514,3.81770221813733));
#112216=CARTESIAN_POINT('Ctrl Pts',(6.66349877090998,3.461150149,3.4671862672109));
#112217=CARTESIAN_POINT('Ctrl Pts',(6.83159984383319,3.526458173,3.09629115331918));
#112218=CARTESIAN_POINT('Origin',(-0.175638016403085,3.48214322456174,-0.0948672503717629));
#112219=CARTESIAN_POINT('Ctrl Pts',(5.653926723,3.526465848,4.538238933));
#112220=CARTESIAN_POINT('Ctrl Pts',(5.902616409,3.460723853,4.228410983));
#112221=CARTESIAN_POINT('Ctrl Pts',(6.115962299,3.395965514,3.893264076));
#112222=CARTESIAN_POINT('Ctrl Pts',(5.691777876,3.526465848,4.884021356));
#112223=CARTESIAN_POINT('Ctrl Pts',(5.959415997,3.460723853,4.572119212));
#112224=CARTESIAN_POINT('Ctrl Pts',(6.191370215,3.395965514,4.232840047));
#112225=CARTESIAN_POINT('',(5.65689862469282,3.5256799154174,4.53453392705498));
#112226=CARTESIAN_POINT('Origin',(-0.140619338899652,3.62492146217939,-0.133858214481626));
#112227=CARTESIAN_POINT('Ctrl Pts',(5.85232696622104,3.48629831880185,4.69044444304518));
#112228=CARTESIAN_POINT('Ctrl Pts',(5.81970056460953,3.4925460151888,4.66446257602376));
#112229=CARTESIAN_POINT('Ctrl Pts',(5.78708430511003,3.49894654285328,4.63846664610451));
#112230=CARTESIAN_POINT('Ctrl Pts',(5.72195162960035,3.51206280607769,4.58650600149994));
#112231=CARTESIAN_POINT('Ctrl Pts',(5.68939761283673,3.5187861065053,4.56051129344055));
#112232=CARTESIAN_POINT('Ctrl Pts',(5.65689862700699,3.52567991510503,4.53453392596363));
#112233=CARTESIAN_POINT('Ctrl Pts',(5.11696076934136,3.39148928110283,5.13614087364819));
#112234=CARTESIAN_POINT('Ctrl Pts',(5.12649928817063,3.39372739755142,5.12656685332415));
#112235=CARTESIAN_POINT('Ctrl Pts',(5.136037807,3.395965514,5.116992833));
#112236=CARTESIAN_POINT('Ctrl Pts',(5.413845009,3.461150149,4.838151658));
#112237=CARTESIAN_POINT('Ctrl Pts',(5.659831125,3.526458173,4.530873164));
#112238=CARTESIAN_POINT('Ctrl Pts',(5.46552063919645,3.39148928110284,5.136792911313));
#112239=CARTESIAN_POINT('Ctrl Pts',(5.47505795112847,3.39372739755142,5.12656914964218));
#112240=CARTESIAN_POINT('Ctrl Pts',(5.48459526306049,3.395965514,5.11634538797148));
#112241=CARTESIAN_POINT('Ctrl Pts',(5.76236731444876,3.461150149,4.81858064331118));
#112242=CARTESIAN_POINT('Ctrl Pts',(6.00626976343008,3.526458173,4.49249361300634));
#112243=CARTESIAN_POINT('Origin',(-0.151138060335976,3.48214328140649,-0.13040629004142));
#112244=CARTESIAN_POINT('Ctrl Pts',(4.546153837,3.526465848,5.647564545));
#112245=CARTESIAN_POINT('Ctrl Pts',(4.85563314700001,3.460723853,5.398441132));
#112246=CARTESIAN_POINT('Ctrl Pts',(5.136037807,3.395965514,5.11699283300001));
#112247=CARTESIAN_POINT('Ctrl Pts',(4.508787052,3.526465848,5.993399646));
#112248=CARTESIAN_POINT('Ctrl Pts',(4.837217683,3.460723853,5.746323886));
#112249=CARTESIAN_POINT('Ctrl Pts',(5.136683932,3.395965514,5.464840179));
#112250=CARTESIAN_POINT('',(4.54985272407115,3.52567991539807,5.64458503122447));
#112251=CARTESIAN_POINT('Origin',(-0.108556179647278,3.62492147900981,-0.160957689453805));
#112252=CARTESIAN_POINT('Ctrl Pts',(4.70719590746653,3.4862983188276,5.83886176251773));
#112253=CARTESIAN_POINT('Ctrl Pts',(4.68091762642385,3.49254601520108,5.8064736252346));
#112254=CARTESIAN_POINT('Ctrl Pts',(4.65465227342764,3.49894654286217,5.77407393406611));
#112255=CARTESIAN_POINT('Ctrl Pts',(4.60221236624675,3.51206280607866,5.70932650065181));
#112256=CARTESIAN_POINT('Ctrl Pts',(4.57600753795857,3.51878610653334,5.67694138305702));
#112257=CARTESIAN_POINT('Ctrl Pts',(4.54985272626207,3.52567991516297,5.64458503070716));
#112258=CARTESIAN_POINT('Ctrl Pts',(3.89321060505149,3.39148928108099,6.11605606300189));
#112259=CARTESIAN_POINT('Ctrl Pts',(3.90458425002574,3.3937273975405,6.10875637750094));
#112260=CARTESIAN_POINT('Ctrl Pts',(3.915957895,3.395965514,6.101456692));
#112261=CARTESIAN_POINT('Ctrl Pts',(4.247212729,3.461150149,5.88885500499999));
#112262=CARTESIAN_POINT('Ctrl Pts',(4.55350362,3.526458173,5.64164025600001));
#112263=CARTESIAN_POINT('Ctrl Pts',(4.23348117065251,3.39148928108099,6.19162292591446));
#112264=CARTESIAN_POINT('Ctrl Pts',(4.24499331214562,3.3937273975405,6.18368843019944));
#112265=CARTESIAN_POINT('Ctrl Pts',(4.25650545363876,3.395965514,6.17575393448438));
#112266=CARTESIAN_POINT('Ctrl Pts',(4.59179396738459,3.461150149,5.94466354376875));
#112267=CARTESIAN_POINT('Ctrl Pts',(4.90009318391137,3.526458173,5.67863206376881));
#112268=CARTESIAN_POINT('Origin',(-0.119570898867882,3.48214322970563,-0.159847509292387));
#112269=CARTESIAN_POINT('Ctrl Pts',(3.22580785,3.526465848,6.49281631600001));
#112270=CARTESIAN_POINT('Ctrl Pts',(3.581605876,3.460723853,6.316046174));
#112271=CARTESIAN_POINT('Ctrl Pts',(3.915957895,3.395965514,6.101456692));
#112272=CARTESIAN_POINT('Ctrl Pts',(3.114970356,3.526465848,6.822533231));
#112273=CARTESIAN_POINT('Ctrl Pts',(3.488836447,3.460723853,6.651836841));
#112274=CARTESIAN_POINT('Ctrl Pts',(3.841812017,3.395965514,6.441310459));
#112275=CARTESIAN_POINT('',(3.23006076639938,3.52567991540093,6.49070161271788));
#112276=CARTESIAN_POINT('Origin',(-0.0714169527961889,3.62492144218,-0.180530784337261));
#112277=CARTESIAN_POINT('Ctrl Pts',(3.34196159965904,3.48629831886319,6.71426039576971));
#112278=CARTESIAN_POINT('Ctrl Pts',(3.32326018235622,3.49254601522207,6.6769804215401));
#112279=CARTESIAN_POINT('Ctrl Pts',(3.30457387463035,3.49894654285152,6.63969194278602));
#112280=CARTESIAN_POINT('Ctrl Pts',(3.26727876750601,3.51206280604764,6.56518523846719));
#112281=CARTESIAN_POINT('Ctrl Pts',(3.24864843637578,3.51878610652078,6.52792400329999));
#112282=CARTESIAN_POINT('Ctrl Pts',(3.23006076876783,3.52567991516642,6.49070161298076));
#112283=CARTESIAN_POINT('Ctrl Pts',(2.48741823989616,3.39148928091091,6.80999126922818));
#112284=CARTESIAN_POINT('Ctrl Pts',(2.5000951924481,3.39372739745545,6.80530724361409));
#112285=CARTESIAN_POINT('Ctrl Pts',(2.512772145,3.395965514,6.800623218));
#112286=CARTESIAN_POINT('Ctrl Pts',(2.881985503,3.461150149,6.664202038));
#112287=CARTESIAN_POINT('Ctrl Pts',(3.234259347,3.526458173,6.48861052000001));
#112288=CARTESIAN_POINT('Ctrl Pts',(2.80348882619201,3.39148928091091,6.95693953369113));
#112289=CARTESIAN_POINT('Ctrl Pts',(2.81643750275045,3.39372739745545,6.9516653120311));
#112290=CARTESIAN_POINT('Ctrl Pts',(2.82938617930894,3.395965514,6.94639109037117));
#112291=CARTESIAN_POINT('Ctrl Pts',(3.20651343716055,3.461150149,6.79278058485489));
#112292=CARTESIAN_POINT('Ctrl Pts',(3.56479369392163,3.526458173,6.59924399066081));
#112293=CARTESIAN_POINT('Origin',(-0.0824129386034567,3.48214323024491,
-0.181814627493688));
#112294=CARTESIAN_POINT('Ctrl Pts',(1.754626674,3.526465848,7.034471212));
#112295=CARTESIAN_POINT('Ctrl Pts',(2.140106694,3.460723853,6.938319916));
#112296=CARTESIAN_POINT('Ctrl Pts',(2.512772145,3.395965514,6.800623218));
#112297=CARTESIAN_POINT('Ctrl Pts',(1.575501108,3.526465848,7.332652744));
#112298=CARTESIAN_POINT('Ctrl Pts',(1.977321095,3.460723853,7.246317299));
#112299=CARTESIAN_POINT('Ctrl Pts',(2.367301242,3.395965514,7.11659222));
#112300=CARTESIAN_POINT('',(1.7592347577013,3.52567991540696,7.03332020118498));
#112301=CARTESIAN_POINT('Origin',(-0.0309385539742335,3.62492149359909,
-0.191662856884642));
#112302=CARTESIAN_POINT('Ctrl Pts',(1.82046088137077,3.48629831883827,7.27570767517235));
#112303=CARTESIAN_POINT('Ctrl Pts',(1.81021078533887,3.49254601521445,7.23527903401874));
#112304=CARTESIAN_POINT('Ctrl Pts',(1.79997727388744,3.49894654284948,7.19484533535449));
#112305=CARTESIAN_POINT('Ctrl Pts',(1.77957084490071,3.51206280606853,7.11406321064714));
#112306=CARTESIAN_POINT('Ctrl Pts',(1.76938614485983,3.51878610653735,7.07366815198741));
#112307=CARTESIAN_POINT('Ctrl Pts',(1.75923476045434,3.52567991517846,7.03332020138535));
#112308=CARTESIAN_POINT('Ctrl Pts',(0.965316962573027,3.39148928101642,
7.18549885113208));
#112309=CARTESIAN_POINT('Ctrl Pts',(0.978704461786508,3.39372739750821,
7.18364950556611));
#112310=CARTESIAN_POINT('Ctrl Pts',(0.992091961,3.395965514,7.18180016));
#112311=CARTESIAN_POINT('Ctrl Pts',(1.381999838,3.461150149,7.12793839));
#112312=CARTESIAN_POINT('Ctrl Pts',(1.763784701,3.526458173,7.032180567));
#112313=CARTESIAN_POINT('Ctrl Pts',(1.24240846170559,3.3914892810164,7.39695738031954));
#112314=CARTESIAN_POINT('Ctrl Pts',(1.25618820682695,3.39372739750821,7.39459004977929));
#112315=CARTESIAN_POINT('Ctrl Pts',(1.26996795194829,3.395965514,7.39222271923901));
#112316=CARTESIAN_POINT('Ctrl Pts',(1.67129990201468,3.461150149,7.32327475439529));
#112317=CARTESIAN_POINT('Ctrl Pts',(2.06280841283414,3.526458173,7.21128260347993));
#112318=CARTESIAN_POINT('Origin',(-0.0414014279420537,3.48214326373977,
-0.195280406556784));
#112319=CARTESIAN_POINT('Ctrl Pts',(0.201401104,3.526465848,7.247202053));
#112320=CARTESIAN_POINT('Ctrl Pts',(0.598538503,3.460723853,7.23616553));
#112321=CARTESIAN_POINT('Ctrl Pts',(0.992091961000001,3.395965514,7.18180016));
#112322=CARTESIAN_POINT('Ctrl Pts',(-0.037636821,3.526465848,7.499905564));
#112323=CARTESIAN_POINT('Ctrl Pts',(0.373348407,3.460723853,7.501968014));
#112324=CARTESIAN_POINT('Ctrl Pts',(0.782098092,3.395965514,7.459110039));
#112325=CARTESIAN_POINT('',(0.206148887086937,3.52567991542637,7.24706855394498));
#112326=CARTESIAN_POINT('Origin',(0.0109866099485638,3.62492146493991,-0.193832750940208));
#112327=CARTESIAN_POINT('Ctrl Pts',(0.213837435628791,3.48629831884979,
7.49695094993265));
#112328=CARTESIAN_POINT('Ctrl Pts',(0.212517943928668,3.49254601521909,
7.45526404033161));
#112329=CARTESIAN_POINT('Ctrl Pts',(0.211215736273181,3.49894654286066,
7.41357575659991));
#112330=CARTESIAN_POINT('Ctrl Pts',(0.208652167091656,3.51206280608243,
7.33029549416932));
#112331=CARTESIAN_POINT('Ctrl Pts',(0.207389323161436,3.51878610655237,
7.2886554401733));
#112332=CARTESIAN_POINT('Ctrl Pts',(0.206148889088203,3.52567991520143,
7.24706855474586));
#112333=CARTESIAN_POINT('Ctrl Pts',(-0.601921461963398,3.39148928102925,
7.22502049361108));
#112334=CARTESIAN_POINT('Ctrl Pts',(-0.588449400481704,3.39372739751463,
7.22609230130554));
#112335=CARTESIAN_POINT('Ctrl Pts',(-0.574977339,3.395965514,7.227164109));
#112336=CARTESIAN_POINT('Ctrl Pts',(-0.182606604,3.461150149,7.258380265));
#112337=CARTESIAN_POINT('Ctrl Pts',(0.210837442,3.526458173,7.246933667));
#112338=CARTESIAN_POINT('Ctrl Pts',(-0.376765541909082,3.39148928102926,
7.49110172164201));
#112339=CARTESIAN_POINT('Ctrl Pts',(-0.362799053537817,3.39372739751463,
7.49175197583758));
#112340=CARTESIAN_POINT('Ctrl Pts',(-0.348832565166553,3.395965514,7.49240223003305));
#112341=CARTESIAN_POINT('Ctrl Pts',(0.0579382408488792,3.461150149,7.51134073598912));
#112342=CARTESIAN_POINT('Ctrl Pts',(0.46436850244113,3.526458173,7.48612965584789));
#112343=CARTESIAN_POINT('Origin',(0.00154602868513654,3.48214325210162,
-0.199614718843649));
#112344=CARTESIAN_POINT('Ctrl Pts',(0.201310764,2.492226207,7.247204563));
#112345=CARTESIAN_POINT('Ctrl Pts',(0.597708493,2.42647128,7.236193541));
#112346=CARTESIAN_POINT('Ctrl Pts',(0.990540534000001,2.361474582,7.182014303));
#112347=CARTESIAN_POINT('Ctrl Pts',(0.994451674780801,2.36082745750497,
7.1814748800276));
#112348=CARTESIAN_POINT('Ctrl Pts',(0.998362815561602,2.36018033300993,
7.18093545705518));
#112349=CARTESIAN_POINT('Ctrl Pts',(-0.03773031,2.492226207,7.499905094));
#112350=CARTESIAN_POINT('Ctrl Pts',(0.372489288,2.42647128,7.501968815));
#112351=CARTESIAN_POINT('Ctrl Pts',(0.780486766,2.361474582,7.45927881300001));
#112352=CARTESIAN_POINT('Ctrl Pts',(0.78454889792439,2.36082745750497,7.4588537799316));
#112353=CARTESIAN_POINT('Ctrl Pts',(0.788611029848782,2.36018033300993,
7.45842874686319));
#112354=CARTESIAN_POINT('',(0.213277379534241,2.452029426852,7.49696690919716));
#112355=CARTESIAN_POINT('',(0.780486763977484,2.36147458149274,7.45927881126999));
#112356=CARTESIAN_POINT('Origin',(0.0109054895757806,2.55351791639885,-0.188512452785666));
#112357=CARTESIAN_POINT('',(0.885513641295677,2.36147458056994,7.32064655905289));
#112358=CARTESIAN_POINT('Ctrl Pts',(0.21327737739871,2.45202942666989,7.49696690365892));
#112359=CARTESIAN_POINT('Ctrl Pts',(0.212033149998612,2.45828501820065,
7.45527809421543));
#112360=CARTESIAN_POINT('Ctrl Pts',(0.210806624554835,2.46469207979751,
7.41358805137032));
#112361=CARTESIAN_POINT('Ctrl Pts',(0.208395237952903,2.47781843917276,
7.33030329110628));
#112362=CARTESIAN_POINT('Ctrl Pts',(0.207208999418987,2.48454521298205,
7.28866109792748));
#112363=CARTESIAN_POINT('Ctrl Pts',(0.206045687659983,2.49144077620845,
7.2470715019965));
#112364=CARTESIAN_POINT('Ctrl Pts',(0.98273624710617,2.36016764195642,7.18309066712261));
#112365=CARTESIAN_POINT('Ctrl Pts',(0.986638390553085,2.36082111197821,
7.18255248506131));
#112366=CARTESIAN_POINT('Ctrl Pts',(0.990540534,2.361474582,7.18201430300001));
#112367=CARTESIAN_POINT('Ctrl Pts',(1.381189167,2.426894312,7.12813620000001));
#112368=CARTESIAN_POINT('Ctrl Pts',(1.763689251,2.492218586,7.032204507));
#112369=CARTESIAN_POINT('Ctrl Pts',(1.25977250362045,2.36016764195642,7.39344572270517));
#112370=CARTESIAN_POINT('Ctrl Pts',(1.26378877381022,2.36082111197821,7.39275689685258));
#112371=CARTESIAN_POINT('Ctrl Pts',(1.267805044,2.361474582,7.392068071));
#112372=CARTESIAN_POINT('Ctrl Pts',(1.669879053,2.426894312,7.323108823));
#112373=CARTESIAN_POINT('Ctrl Pts',(2.062101341,2.492218586,7.210945712));
#112374=CARTESIAN_POINT('',(1.26780503971333,2.36147458096339,7.39206804979796));
#112375=CARTESIAN_POINT('',(1.81991734971456,2.45202942680341,7.27584365708309));
#112376=CARTESIAN_POINT('Origin',(-0.0403900291321555,2.41071409422485,
-0.188786091166397));
#112377=CARTESIAN_POINT('Ctrl Pts',(1.75913460499445,2.49144077640748,7.03334526460813));
#112378=CARTESIAN_POINT('Ctrl Pts',(1.76921125281641,2.48454521318186,7.07371244111567));
#112379=CARTESIAN_POINT('Ctrl Pts',(1.77932159849006,2.47781843922911,7.11412605749383));
#112380=CARTESIAN_POINT('Ctrl Pts',(1.79958036973389,2.46469207981283,7.19494528958312));
#112381=CARTESIAN_POINT('Ctrl Pts',(1.80974034658981,2.4582850181691,7.2353969759097));
#112382=CARTESIAN_POINT('Ctrl Pts',(1.81991734640429,2.45202942659619,7.27584365226265));
#112383=CARTESIAN_POINT('',(1.12917279935051,2.36147458031212,7.28704118539612));
#112384=CARTESIAN_POINT('Origin',(2.63894808782972E-13,2.45311202899967,
7.8236028766554E-13));
#112385=CARTESIAN_POINT('',(1.82645773667202,2.27159573076564,7.27420457036109));
#112386=CARTESIAN_POINT('Ctrl Pts',(1.8264577281804,2.27159573309127,7.27420457225405));
#112387=CARTESIAN_POINT('Ctrl Pts',(1.7973070705304,2.27631121118619,7.28152392215389));
#112388=CARTESIAN_POINT('Ctrl Pts',(1.76813109415185,2.28101755501093,7.28866334775712));
#112389=CARTESIAN_POINT('Ctrl Pts',(1.73893308895609,2.28571428598668,7.29562277789647));
#112390=CARTESIAN_POINT('Ctrl Pts',(1.59152439382906,2.30942614431015,7.33075807194632));
#112391=CARTESIAN_POINT('Ctrl Pts',(1.4425453427614,2.33338333523652,7.36154196553795));
#112392=CARTESIAN_POINT('Ctrl Pts',(1.29238815216021,2.35752265772375,7.38780974699737));
#112393=CARTESIAN_POINT('Ctrl Pts',(1.28419726093286,2.3588394282627,7.38924262237188));
#112394=CARTESIAN_POINT('Ctrl Pts',(1.27600287000738,2.36015673981136,7.39066207115902));
#112395=CARTESIAN_POINT('Ctrl Pts',(1.26780504503328,2.36147458179854,7.39206807061842));
#112396=CARTESIAN_POINT('',(2.36576386665489,2.36147458149275,7.11710343474374));
#112397=CARTESIAN_POINT('Origin',(-0.0678177627952725,2.41070047484541,
-0.178936091179097));
#112398=CARTESIAN_POINT('Origin',(-0.029874064411306,2.55351790539617,-0.186449428114565));
#112399=CARTESIAN_POINT('Ctrl Pts',(1.754538986,2.492226207,7.034493084));
#112400=CARTESIAN_POINT('Ctrl Pts',(2.139302112,2.42647128,6.938525699));
#112401=CARTESIAN_POINT('Ctrl Pts',(2.511303023,2.361474582,6.801165865));
#112402=CARTESIAN_POINT('Ctrl Pts',(2.5150067634836,2.36082745750497,6.7997982737846));
#112403=CARTESIAN_POINT('Ctrl Pts',(2.5187105039672,2.36018033300993,6.79843068256919));
#112404=CARTESIAN_POINT('Ctrl Pts',(1.575409703,2.492226207,7.332672382));
#112405=CARTESIAN_POINT('Ctrl Pts',(1.976482234,2.42647128,7.246502767));
#112406=CARTESIAN_POINT('Ctrl Pts',(2.365763869,2.361474582,7.117103436));
#112407=CARTESIAN_POINT('Ctrl Pts',(2.36963966098986,2.36082745750497,7.11581510167983));
#112408=CARTESIAN_POINT('Ctrl Pts',(2.37351545297971,2.36018033300993,7.11452676735966));
#112409=CARTESIAN_POINT('',(2.43853343772574,2.36147458056998,6.95913465339936));
#112410=CARTESIAN_POINT('Ctrl Pts',(2.50391258247664,2.36016764195642,6.80389475530675));
#112411=CARTESIAN_POINT('Ctrl Pts',(2.50760780273832,2.36082111197821,6.80253031015338));
#112412=CARTESIAN_POINT('Ctrl Pts',(2.511303023,2.361474582,6.801165865));
#112413=CARTESIAN_POINT('Ctrl Pts',(2.881236308,2.426894312,6.664569494));
#112414=CARTESIAN_POINT('Ctrl Pts',(3.234171275,2.492218586,6.48865441900001));
#112415=CARTESIAN_POINT('Ctrl Pts',(2.81969200434841,2.36016764195642,6.94977722071898));
#112416=CARTESIAN_POINT('Ctrl Pts',(2.82346629917421,2.36082111197821,6.94824111985949));
#112417=CARTESIAN_POINT('Ctrl Pts',(2.827240594,2.361474582,6.946705019));
#112418=CARTESIAN_POINT('Ctrl Pts',(3.205090136,2.426894312,6.79292397300001));
#112419=CARTESIAN_POINT('Ctrl Pts',(3.564030731,2.492218586,6.599066975));
#112420=CARTESIAN_POINT('',(2.82724058529781,2.36147458096342,6.9467049992098));
#112421=CARTESIAN_POINT('',(3.34146000745496,2.45202942687121,6.71451004157885));
#112422=CARTESIAN_POINT('Origin',(-0.0800291984243725,2.4107140862089,-0.175689795986495));
#112423=CARTESIAN_POINT('Ctrl Pts',(3.22996834292614,2.49144077637346,6.49074762063525));
#112424=CARTESIAN_POINT('Ctrl Pts',(3.24848715411197,2.48454521317637,6.52800485345517));
#112425=CARTESIAN_POINT('Ctrl Pts',(3.26704885856273,2.47781843923068,6.56530019645369));
#112426=CARTESIAN_POINT('Ctrl Pts',(3.30420772731042,2.46469208329873,6.63987486303306));
#112427=CARTESIAN_POINT('Ctrl Pts',(3.32282607478242,2.45828502541683,6.67719669328445));
#112428=CARTESIAN_POINT('Ctrl Pts',(3.34146000317469,2.45202942670672,6.7145100372272));
#112429=CARTESIAN_POINT('',(2.66927181826374,2.36147458031212,6.87393543820857));
#112430=CARTESIAN_POINT('Origin',(4.52112305926455E-13,2.45311202899922,
9.03357250114922E-13));
#112431=CARTESIAN_POINT('',(3.34749512840975,2.27159573075016,6.71150328609892));
#112432=CARTESIAN_POINT('Ctrl Pts',(3.34749512062753,2.27159573306644,6.71150328981358));
#112433=CARTESIAN_POINT('Ctrl Pts',(3.32059943308098,2.27631121117738,6.724918047135));
#112434=CARTESIAN_POINT('Ctrl Pts',(3.29364034028498,2.28101755501029,6.73816252941245));
#112435=CARTESIAN_POINT('Ctrl Pts',(3.26662103989866,2.28571428600481,6.75123595998502));
#112436=CARTESIAN_POINT('Ctrl Pts',(3.13021152700453,2.309426179206,6.81723841983366));
#112437=CARTESIAN_POINT('Ctrl Pts',(2.99133294332461,2.33338340554088,6.87932878025919));
#112438=CARTESIAN_POINT('Ctrl Pts',(2.85033292833529,2.35752276396414,6.93726186564666));
#112439=CARTESIAN_POINT('Ctrl Pts',(2.84264176798055,2.35883949911844,6.94042195502391));
#112440=CARTESIAN_POINT('Ctrl Pts',(2.83494430377073,2.36015677525334,6.9435696847162));
#112441=CARTESIAN_POINT('Ctrl Pts',(2.8272405949271,2.36147458179854,6.94670501840523));
#112442=CARTESIAN_POINT('',(3.84042048042676,2.36147458149274,6.44214021129295));
#112443=CARTESIAN_POINT('Origin',(-0.104698240445678,2.41070046968801,-0.160173936573987));
#112444=CARTESIAN_POINT('Origin',(-0.0692568098882768,2.55351788595202,
-0.175668412511882));
#112445=CARTESIAN_POINT('Ctrl Pts',(3.225726914,2.492226207,6.492856527));
#112446=CARTESIAN_POINT('Ctrl Pts',(3.580864341,2.42647128,6.316420107));
#112447=CARTESIAN_POINT('Ctrl Pts',(3.914639774,2.361474582,6.10230247));
#112448=CARTESIAN_POINT('Ctrl Pts',(3.91796293140924,2.36082745750497,6.10017065758514));
#112449=CARTESIAN_POINT('Ctrl Pts',(3.92128608881848,2.36018033300993,6.09803884517028));
#112450=CARTESIAN_POINT('Ctrl Pts',(3.11488531,2.492226207,6.82257206));
#112451=CARTESIAN_POINT('Ctrl Pts',(3.488057068,2.42647128,6.652198303));
#112452=CARTESIAN_POINT('Ctrl Pts',(3.840420483,2.361474582,6.442140212));
#112453=CARTESIAN_POINT('Ctrl Pts',(3.84392870732549,2.36082745750497,6.44004881750999));
#112454=CARTESIAN_POINT('Ctrl Pts',(3.84743693165098,2.36018033300993,6.43795742301998));
#112455=CARTESIAN_POINT('',(3.87753012104247,2.36147458056998,6.2722213456103));
#112456=CARTESIAN_POINT('Ctrl Pts',(3.908008748627,2.36016764195642,6.10655628662292));
#112457=CARTESIAN_POINT('Ctrl Pts',(3.9113242613135,2.36082111197821,6.10442937831146));
#112458=CARTESIAN_POINT('Ctrl Pts',(3.914639774,2.361474582,6.10230247));
#112459=CARTESIAN_POINT('Ctrl Pts',(4.246560042,2.426894312,5.889374925));
#112460=CARTESIAN_POINT('Ctrl Pts',(4.553427044,2.492218586,5.641702062));
#112461=CARTESIAN_POINT('Ctrl Pts',(4.24776584072616,2.36016764195642,6.18114485999082));
#112462=CARTESIAN_POINT('Ctrl Pts',(4.25112167836308,2.36082111197821,6.17883331049541));
#112463=CARTESIAN_POINT('Ctrl Pts',(4.254477516,2.361474582,6.176521761));
#112464=CARTESIAN_POINT('Ctrl Pts',(4.590434767,2.426894312,5.945109548));
#112465=CARTESIAN_POINT('Ctrl Pts',(4.899310006,2.492218586,5.678623201));
#112466=CARTESIAN_POINT('',(4.2544775032456,2.36147458096339,6.17652174354511));
#112467=CARTESIAN_POINT('',(4.70675970893107,2.45202942683396,5.83921339942039));
#112468=CARTESIAN_POINT('Origin',(-0.115926191916461,2.41071410523568,-0.154378239308755));
#112469=CARTESIAN_POINT('Ctrl Pts',(4.54977235062771,2.49144077650933,5.64464983131305));
#112470=CARTESIAN_POINT('Ctrl Pts',(4.5758674060766,2.48454521330205,5.67705501364799));
#112471=CARTESIAN_POINT('Ctrl Pts',(4.60201254479543,2.47781843927961,5.70948819475178));
#112472=CARTESIAN_POINT('Ctrl Pts',(4.65433402260713,2.46469207987452,5.77433130573284));
#112473=CARTESIAN_POINT('Ctrl Pts',(4.68054019026222,2.45828501822244,5.80677819834295));
#112474=CARTESIAN_POINT('Ctrl Pts',(4.70675970388043,2.45202942664259,5.83921339628418));
#112475=CARTESIAN_POINT('',(4.08455865372057,2.3614745803121,6.13941210969819));
#112476=CARTESIAN_POINT('Origin',(1.24856722183431E-12,2.45311202899956,
1.52005144582468E-12));
#112477=CARTESIAN_POINT('',(4.71200736856892,2.27159573077527,5.83497956779286));
#112478=CARTESIAN_POINT('Ctrl Pts',(4.71200736155291,2.27159573310906,5.83497957305765));
#112479=CARTESIAN_POINT('Ctrl Pts',(4.68862425625641,2.27631121119035,5.85386247845562));
#112480=CARTESIAN_POINT('Ctrl Pts',(4.66514262405863,2.28101755500929,5.87259272007343));
#112481=CARTESIAN_POINT('Ctrl Pts',(4.64156542103399,2.28571428599323,5.89116885197322));
#112482=CARTESIAN_POINT('Ctrl Pts',(4.52253390152555,2.30942613223479,5.98495203822414));
#112483=CARTESIAN_POINT('Ctrl Pts',(4.40025006189854,2.33338331075958,6.07544537852409));
#112484=CARTESIAN_POINT('Ctrl Pts',(4.27500070883594,2.35752262072372,6.16233469842595));
#112485=CARTESIAN_POINT('Ctrl Pts',(4.2681684422202,2.35883940358577,6.16707445144753));
#112486=CARTESIAN_POINT('Ctrl Pts',(4.26132736152242,2.36015672746786,6.17180348811389));
#112487=CARTESIAN_POINT('Ctrl Pts',(4.25447751677773,2.36147458179851,6.17652176021973));
#112488=CARTESIAN_POINT('',(5.13550330134351,2.36147458149276,5.46594967184533));
#112489=CARTESIAN_POINT('Origin',(-0.136683026004824,2.41070043159255,-0.133922036617143));
#112490=CARTESIAN_POINT('Origin',(-0.105401060621905,2.55351787062719,-0.156673127077545));
#112491=CARTESIAN_POINT('Ctrl Pts',(4.546083437,2.492226207,5.647621215));
#112492=CARTESIAN_POINT('Ctrl Pts',(4.854989334,2.42647128,5.398965732));
#112493=CARTESIAN_POINT('Ctrl Pts',(5.13493232,2.361474582,5.118102194));
#112494=CARTESIAN_POINT('Ctrl Pts',(5.13771950718071,2.36082745750497,5.11530584155758));
#112495=CARTESIAN_POINT('Ctrl Pts',(5.1405066943614,2.36018033300993,5.11250948911515));
#112496=CARTESIAN_POINT('Ctrl Pts',(4.508712341,2.492226207,5.99345585));
#112497=CARTESIAN_POINT('Ctrl Pts',(4.83653423,2.42647128,5.74684444));
#112498=CARTESIAN_POINT('Ctrl Pts',(5.135503304,2.361474582,5.465949672));
#112499=CARTESIAN_POINT('Ctrl Pts',(5.13847991999737,2.36082745750497,5.46315300862335));
#112500=CARTESIAN_POINT('Ctrl Pts',(5.14145653599474,2.36018033300993,5.46035634524671));
#112501=CARTESIAN_POINT('',(5.13521780570789,2.36147458056998,5.29202593910566));
#112502=CARTESIAN_POINT('Ctrl Pts',(5.1293707691374,2.36016764195642,5.12368203318865));
#112503=CARTESIAN_POINT('Ctrl Pts',(5.13215154456869,2.36082111197821,5.12089211359432));
#112504=CARTESIAN_POINT('Ctrl Pts',(5.13493232,2.361474582,5.118102194));
#112505=CARTESIAN_POINT('Ctrl Pts',(5.413319349,2.426894312,4.838799731));
#112506=CARTESIAN_POINT('Ctrl Pts',(5.659769626,2.492218586,4.530949987));
#112507=CARTESIAN_POINT('Ctrl Pts',(5.47721886760684,2.36016764195642,5.12348903528974));
#112508=CARTESIAN_POINT('Ctrl Pts',(5.47999933280342,2.36082111197821,5.12051012264487));
#112509=CARTESIAN_POINT('Ctrl Pts',(5.48277979800001,2.361474582,5.11753121));
#112510=CARTESIAN_POINT('Ctrl Pts',(5.761135769,2.426894312,4.819308408));
#112511=CARTESIAN_POINT('Ctrl Pts',(6.00550299000001,2.492218586,4.492653318));
#112512=CARTESIAN_POINT('',(5.48277978178718,2.36147458096342,5.11753119569418));
#112513=CARTESIAN_POINT('',(5.85197655738761,2.45202942686292,4.69088162852638));
#112514=CARTESIAN_POINT('Origin',(-0.146402830297621,2.41071406611784,-0.12584841218946));
#112515=CARTESIAN_POINT('Ctrl Pts',(5.65683406098997,2.49144077636711,4.53461449072042));
#112516=CARTESIAN_POINT('Ctrl Pts',(5.68928518494927,2.48454521316727,4.56065239240826));
#112517=CARTESIAN_POINT('Ctrl Pts',(5.72179123964571,2.47781843924977,4.58670687141016));
#112518=CARTESIAN_POINT('Ctrl Pts',(5.78682882247503,2.46469207986781,4.63878641528251));
#112519=CARTESIAN_POINT('Ctrl Pts',(5.81939742714816,2.45828501824452,4.66484116602438));
#112520=CARTESIAN_POINT('Ctrl Pts',(5.85197655176899,2.45202942668633,4.69088162653268));
#112521=CARTESIAN_POINT('',(5.30885606626941,2.36147458031211,5.11781669445923));
#112522=CARTESIAN_POINT('Origin',(5.25187532351978E-13,2.45311202899933,
3.48245737802344E-13));
#112523=CARTESIAN_POINT('',(5.85619138107285,2.27159573078832,4.68561868955803));
#112524=CARTESIAN_POINT('Ctrl Pts',(5.85619137521515,2.27159573313753,4.68561869622839));
#112525=CARTESIAN_POINT('Ctrl Pts',(5.8374142203088,2.27631121119808,4.70908680616086));
#112526=CARTESIAN_POINT('Ctrl Pts',(5.81850802386978,2.28101755500772,4.73242700194082));
#112527=CARTESIAN_POINT('Ctrl Pts',(5.79947536200712,2.28571428599824,4.75563723599132));
#112528=CARTESIAN_POINT('Ctrl Pts',(5.70338729269073,2.30942614547804,4.87281614740652));
#112529=CARTESIAN_POINT('Ctrl Pts',(5.60341571685522,2.33338333746231,4.98748127694228));
#112530=CARTESIAN_POINT('Ctrl Pts',(5.49977319763934,2.35752266107725,5.0992641401815));
#112531=CARTESIAN_POINT('Ctrl Pts',(5.4941196299469,2.3588394304991,5.10536175329394));
#112532=CARTESIAN_POINT('Ctrl Pts',(5.48845515076391,2.3601567409299,5.11145079553456));
#112533=CARTESIAN_POINT('Ctrl Pts',(5.48277979859175,2.36147458179852,5.11753120907084));
#112534=CARTESIAN_POINT('',(6.19045569537311,2.36147458149269,4.23417740041582));
#112535=CARTESIAN_POINT('Origin',(-0.162276638322637,2.4107004468959,-0.101408132842024));
#112536=CARTESIAN_POINT('Origin',(-0.136617111854956,2.55351791166208,-0.130352226288843));
#112537=CARTESIAN_POINT('Ctrl Pts',(5.653870151,2.492226207,4.538309411));
#112538=CARTESIAN_POINT('Ctrl Pts',(5.902100421,2.42647128,4.229061719));
#112539=CARTESIAN_POINT('Ctrl Pts',(6.115121138,2.361474582,3.894585148));
#112540=CARTESIAN_POINT('Ctrl Pts',(6.11724202918621,2.36082745750497,3.89125500987346));
#112541=CARTESIAN_POINT('Ctrl Pts',(6.1193629203724,2.36018033300994,3.88792487174692));
#112542=CARTESIAN_POINT('Ctrl Pts',(5.69171699500001,2.492226207,4.884092306));
#112543=CARTESIAN_POINT('Ctrl Pts',(5.958860426,2.42647128,4.572774518));
#112544=CARTESIAN_POINT('Ctrl Pts',(6.190455698,2.361474582,4.2341774));
#112545=CARTESIAN_POINT('Ctrl Pts',(6.19276152241965,2.36082745750497,4.23080623660635));
#112546=CARTESIAN_POINT('Ctrl Pts',(6.1950673468393,2.36018033300994,4.2274350732127));
#112547=CARTESIAN_POINT('',(6.15278841316685,2.36147458056978,4.06438128131659));
#112548=CARTESIAN_POINT('Ctrl Pts',(6.11088911360345,2.36016764195642,3.90123010271037));
#112549=CARTESIAN_POINT('Ctrl Pts',(6.11300512580173,2.36082111197821,3.89790762535519));
#112550=CARTESIAN_POINT('Ctrl Pts',(6.11512113800001,2.361474582,3.894585148));
#112551=CARTESIAN_POINT('Ctrl Pts',(6.326957859,2.426894312,3.561967638));
#112552=CARTESIAN_POINT('Ctrl Pts',(6.50146767100001,2.492218586,3.208335726));
#112553=CARTESIAN_POINT('Ctrl Pts',(6.45056322737555,2.36016764195642,3.82626455831515));
#112554=CARTESIAN_POINT('Ctrl Pts',(6.45263830868778,2.36082111197821,3.82275757315758));
#112555=CARTESIAN_POINT('Ctrl Pts',(6.45471339,2.361474582,3.819250588));
#112556=CARTESIAN_POINT('Ctrl Pts',(6.662452467,2.426894312,3.468161763));
#112557=CARTESIAN_POINT('Ctrl Pts',(6.830885329,2.492218586,3.096611959));
#112558=CARTESIAN_POINT('',(6.45471337105975,2.36147458096336,3.81925057755459));
#112559=CARTESIAN_POINT('',(6.72356148620511,2.45202942682532,3.32320944645836));
#112560=CARTESIAN_POINT('Origin',(-0.170033501176531,2.41071412305941,-0.0914337445244639));
#112561=CARTESIAN_POINT('Ctrl Pts',(6.49938849766516,2.49144077636212,3.2125456154371));
#112562=CARTESIAN_POINT('Ctrl Pts',(6.53667831149826,2.48454521316004,3.23099873309163));
#112563=CARTESIAN_POINT('Ctrl Pts',(6.57402533555748,2.47781843922486,3.24945623208448));
#112564=CARTESIAN_POINT('Ctrl Pts',(6.64873793827138,2.46469207983345,3.28633702754683));
#112565=CARTESIAN_POINT('Ctrl Pts',(6.68614610834328,2.4582850181975,3.3047813455483));
#112566=CARTESIAN_POINT('Ctrl Pts',(6.72356148043066,2.45202942662919,3.32320944593048));
#112567=CARTESIAN_POINT('',(6.28491726947834,2.36147458031213,3.85691785907295));
#112568=CARTESIAN_POINT('Origin',(7.02563007770607E-14,2.45311202899911,
-5.33427468862868E-14));
#112569=CARTESIAN_POINT('',(6.72654639328456,2.27159573075196,3.31716348945614));
#112570=CARTESIAN_POINT('Ctrl Pts',(6.72654638901667,2.27159573310009,3.31716349722683));
#112571=CARTESIAN_POINT('Ctrl Pts',(6.71325318346979,2.27631121117457,3.34411946911683));
#112572=CARTESIAN_POINT('Ctrl Pts',(6.69980645556126,2.28101755499664,3.3709782575355));
#112573=CARTESIAN_POINT('Ctrl Pts',(6.6862082810288,2.28571428598099,3.3977373088993));
#112574=CARTESIAN_POINT('Ctrl Pts',(6.61755681684858,2.30942610477132,3.53283250499352));
#112575=CARTESIAN_POINT('Ctrl Pts',(6.5445722664743,2.33338325540565,3.66630753594886));
#112576=CARTESIAN_POINT('Ctrl Pts',(6.46738300984023,2.35752253707386,3.79775683820576));
#112577=CARTESIAN_POINT('Ctrl Pts',(6.46317229461663,2.35883934779648,3.80492746793172));
#112578=CARTESIAN_POINT('Ctrl Pts',(6.45894907973879,2.3601566995621,3.81209207243943));
#112579=CARTESIAN_POINT('Ctrl Pts',(6.4547133903781,2.36147458179854,3.81925058696547));
#112580=CARTESIAN_POINT('',(6.95594926052349,2.36147458149275,2.80441969999315));
#112581=CARTESIAN_POINT('Origin',(-0.180282775616545,2.4107004840551,-0.0641527183467833));
#112582=CARTESIAN_POINT('Origin',(-0.161444725146068,2.55351788295849,-0.0979359078788294));
#112583=CARTESIAN_POINT('Ctrl Pts',(6.497288181,2.492226207,3.216791304));
#112584=CARTESIAN_POINT('Ctrl Pts',(6.67323585300001,2.42647128,2.86141148));
#112585=CARTESIAN_POINT('Ctrl Pts',(6.809373687,2.361474582,2.488961628));
#112586=CARTESIAN_POINT('Ctrl Pts',(6.81072911165684,2.36082745750497,2.48525341773983));
#112587=CARTESIAN_POINT('Ctrl Pts',(6.81208453631367,2.36018033300993,2.48154520747966));
#112588=CARTESIAN_POINT('Ctrl Pts',(6.60858328699999,2.492226207,3.546354034));
#112589=CARTESIAN_POINT('Ctrl Pts',(6.802556932,2.42647128,3.184886742));
#112590=CARTESIAN_POINT('Ctrl Pts',(6.955949263,2.361474582,2.804419699));
#112591=CARTESIAN_POINT('Ctrl Pts',(6.95747647804007,2.36082745750497,2.80063166744372));
#112592=CARTESIAN_POINT('Ctrl Pts',(6.95900369308013,2.36018033300993,2.79684363588743));
#112593=CARTESIAN_POINT('',(6.88266147185314,2.36147458056998,2.64669067168334));
#112594=CARTESIAN_POINT('Ctrl Pts',(6.80666907381407,2.36016764195642,2.496360987497));
#112595=CARTESIAN_POINT('Ctrl Pts',(6.80802138040703,2.36082111197821,2.4926613077485));
#112596=CARTESIAN_POINT('Ctrl Pts',(6.809373687,2.361474582,2.488961628));
#112597=CARTESIAN_POINT('Ctrl Pts',(6.944754851,2.426894312,2.118581898));
#112598=CARTESIAN_POINT('Ctrl Pts',(7.039164313,2.492218586,1.735703252));
#112599=CARTESIAN_POINT('Ctrl Pts',(7.12228642016887,2.36016764195642,2.35012820286911));
#112600=CARTESIAN_POINT('Ctrl Pts',(7.12355908908444,2.36082111197821,2.34625712793456));
#112601=CARTESIAN_POINT('Ctrl Pts',(7.124831758,2.361474582,2.342386053));
#112602=CARTESIAN_POINT('Ctrl Pts',(7.252240291,2.426894312,1.954847729));
#112603=CARTESIAN_POINT('Ctrl Pts',(7.336863062,2.492218586,1.555776466));
#112604=CARTESIAN_POINT('',(7.12483173727822,2.3614745809634,2.34238604683087));
#112605=CARTESIAN_POINT('',(7.28076015244391,2.45202942683899,1.80014768399621));
#112606=CARTESIAN_POINT('Origin',(-0.185713957054917,2.41071409415622,-0.0527439563721279));
#112607=CARTESIAN_POINT('Ctrl Pts',(7.03803875139302,2.4914407764281,1.74026167702851));
#112608=CARTESIAN_POINT('Ctrl Pts',(7.07842362486222,2.4845452132121,1.75026716357087));
#112609=CARTESIAN_POINT('Ctrl Pts',(7.11886531295691,2.47781843925694,1.76026463046666));
#112610=CARTESIAN_POINT('Ctrl Pts',(7.19975945731228,2.46469207985518,1.78022217257698));
#112611=CARTESIAN_POINT('Ctrl Pts',(7.24025802831338,2.45828501821586,1.79019362197555));
#112612=CARTESIAN_POINT('Ctrl Pts',(7.28076014663648,2.45202942664997,1.80014768467118));
#112613=CARTESIAN_POINT('',(6.96710272593122,2.36147458031212,2.41567383060393));
#112614=CARTESIAN_POINT('Origin',(-6.62230686954146E-13,2.45311202900033,
-3.47595216498853E-13));
#112615=CARTESIAN_POINT('',(7.28237557187738,2.2715957307624,1.79360141123147));
#112616=CARTESIAN_POINT('Ctrl Pts',(7.28237556955524,2.27159573308897,1.79360141962778));
#112617=CARTESIAN_POINT('Ctrl Pts',(7.27518788909083,2.27631121118345,1.82278482206762));
#112618=CARTESIAN_POINT('Ctrl Pts',(7.26782938382074,2.281017555009,1.85190631585837));
#112619=CARTESIAN_POINT('Ctrl Pts',(7.26030153198921,2.28571428600673,1.88096296104166));
#112620=CARTESIAN_POINT('Ctrl Pts',(7.2222964727339,2.30942616856895,2.02765813658417));
#112621=CARTESIAN_POINT('Ctrl Pts',(7.17971132022375,2.33338338402406,2.17370250603423));
#112622=CARTESIAN_POINT('Ctrl Pts',(7.13258426888173,2.35752273144221,2.31867238862267));
#112623=CARTESIAN_POINT('Ctrl Pts',(7.13001359641854,2.35883947742822,2.32658016291681));
#112624=CARTESIAN_POINT('Ctrl Pts',(7.12742942262058,2.36015676440385,2.33448474022867));
#112625=CARTESIAN_POINT('Ctrl Pts',(7.12483175814687,2.36147458179854,2.34238605190836));
#112626=CARTESIAN_POINT('',(7.39619036979387,2.36147458149275,1.243530451497));
#112627=CARTESIAN_POINT('Origin',(-0.189858677544673,2.41070042531505,-0.023897387776198));
#112628=CARTESIAN_POINT('Origin',(-0.178723583569177,2.55351789973106,-0.0609403871456785));
#112629=CARTESIAN_POINT('Ctrl Pts',(7.036900237,2.492226207,1.74485961));
#112630=CARTESIAN_POINT('Ctrl Pts',(7.132338192,2.42647128,1.359964821));
#112631=CARTESIAN_POINT('Ctrl Pts',(7.18522749100001,2.361474582,0.96695703));
#112632=CARTESIAN_POINT('Ctrl Pts',(7.185754070995,2.36082745750497,0.963044139405232));
#112633=CARTESIAN_POINT('Ctrl Pts',(7.18628065099001,2.36018033300993,0.959131248810464));
#112634=CARTESIAN_POINT('Ctrl Pts',(7.21643957,2.492226207,2.042792189));
#112635=CARTESIAN_POINT('Ctrl Pts',(7.328173436,2.42647128,1.648077202));
#112636=CARTESIAN_POINT('Ctrl Pts',(7.396190372,2.361474582,1.24353045));
#112637=CARTESIAN_POINT('Ctrl Pts',(7.39686756679169,2.36082745750497,1.23950267442584));
#112638=CARTESIAN_POINT('Ctrl Pts',(7.39754476158338,2.36018033300993,1.23547489885168));
#112639=CARTESIAN_POINT('',(7.29070893018589,2.36147458056998,1.1052437486685));
#112640=CARTESIAN_POINT('Ctrl Pts',(7.18417675373603,2.36016764195642,0.974764808487868));
#112641=CARTESIAN_POINT('Ctrl Pts',(7.18470212236801,2.36082111197821,0.970860919243934));
#112642=CARTESIAN_POINT('Ctrl Pts',(7.185227491,2.361474582,0.96695703));
#112643=CARTESIAN_POINT('Ctrl Pts',(7.237822825,2.426894312,0.576133623));
#112644=CARTESIAN_POINT('Ctrl Pts',(7.247717455,2.492218586,0.181911224));
#112645=CARTESIAN_POINT('Ctrl Pts',(7.46097941612226,2.36016764195642,0.764102464106214));
#112646=CARTESIAN_POINT('Ctrl Pts',(7.46139016406113,2.36082111197821,0.760048306553106));
#112647=CARTESIAN_POINT('Ctrl Pts',(7.461800912,2.361474582,0.755994149));
#112648=CARTESIAN_POINT('Ctrl Pts',(7.50292142,2.426894312,0.350127187));
#112649=CARTESIAN_POINT('Ctrl Pts',(7.499777232,2.492218586,-0.057805406));
#112650=CARTESIAN_POINT('Ctrl Pts',(7.24759813527961,2.49144077636324,0.186605038200559));
#112651=CARTESIAN_POINT('Ctrl Pts',(7.28918971677884,2.48454521314802,0.187695047633678));
#112652=CARTESIAN_POINT('Ctrl Pts',(7.3308350603499,2.47781843923321,0.188765011539292));
#112653=CARTESIAN_POINT('Ctrl Pts',(7.41412822619493,2.46469207984091,0.190866107168316));
#112654=CARTESIAN_POINT('Ctrl Pts',(7.45582352990115,2.45828501821583,0.191898433840291));
#112655=CARTESIAN_POINT('Ctrl Pts',(7.49751856038283,2.4520294266588,0.192913017772023));
#112656=CARTESIAN_POINT('',(7.32351420272364,2.36147458031212,0.86147557909768));
#112657=CARTESIAN_POINT('Ctrl Pts',(7.247474658,2.492226207,0.191340221));
#112658=CARTESIAN_POINT('Ctrl Pts',(7.257940325,2.42647128,-0.205072282));
#112659=CARTESIAN_POINT('Ctrl Pts',(7.22510804400001,2.361474582,-0.600261405));
#112660=CARTESIAN_POINT('Ctrl Pts',(7.22478115703626,2.36082745750497,-0.604196013519101));
#112661=CARTESIAN_POINT('Ctrl Pts',(7.2244542700725,2.36018033300993,-0.608130622038201));
#112662=CARTESIAN_POINT('Ctrl Pts',(7.48686316,2.492226207,0.443711652));
#112663=CARTESIAN_POINT('Ctrl Pts',(7.511132695,2.42647128,0.034205403));
#112664=CARTESIAN_POINT('Ctrl Pts',(7.49059384,2.361474582,-0.375504901));
#112665=CARTESIAN_POINT('Ctrl Pts',(7.4903893496708,2.36082745750497,-0.379584086277783));
#112666=CARTESIAN_POINT('Ctrl Pts',(7.49018485934162,2.36018033300993,-0.383663271555566));
#112667=CARTESIAN_POINT('',(7.35785094258008,2.36147458056998,-0.487883144251673));
#112668=CARTESIAN_POINT('Ctrl Pts',(7.2257603139574,2.36016764195642,-0.592410290582772));
#112669=CARTESIAN_POINT('Ctrl Pts',(7.2254341789787,2.36082111197821,-0.596335847791386));
#112670=CARTESIAN_POINT('Ctrl Pts',(7.225108044,2.361474582,-0.600261405));
#112671=CARTESIAN_POINT('Ctrl Pts',(7.192458249,2.426894312,-0.99325402));
#112672=CARTESIAN_POINT('Ctrl Pts',(7.117375384,2.492218586,-1.380386771));
#112673=CARTESIAN_POINT('Ctrl Pts',(7.45080530628486,2.36016764195642,-0.8576518564782));
#112674=CARTESIAN_POINT('Ctrl Pts',(7.45033492714243,2.36082111197821,-0.8616995287391));
#112675=CARTESIAN_POINT('Ctrl Pts',(7.449864548,2.361474582,-0.865747201));
#112676=CARTESIAN_POINT('Ctrl Pts',(7.402774283,2.426894312,-1.270964912));
#112677=CARTESIAN_POINT('Ctrl Pts',(7.312010155,2.492218586,-1.668684361));
#112678=CARTESIAN_POINT('',(7.44986452659274,2.3614745809634,-0.86574719785456));
#112679=CARTESIAN_POINT('',(7.36370134498239,2.45202942682888,-1.42334204951334));
#112680=CARTESIAN_POINT('Origin',(-0.190695837988908,2.41071407000259,0.0301101055091291));
#112681=CARTESIAN_POINT('Ctrl Pts',(7.11826788532725,2.49144077642908,-1.37577704600419));
#112682=CARTESIAN_POINT('Ctrl Pts',(7.15912139879897,2.48454521318342,-1.38365348071112));
#112683=CARTESIAN_POINT('Ctrl Pts',(7.20002310802721,2.47781843927426,-1.39156104960372));
#112684=CARTESIAN_POINT('Ctrl Pts',(7.28182059975392,2.46469207984667,-1.40741464471913));
#112685=CARTESIAN_POINT('Ctrl Pts',(7.32276301032829,2.45828501820481,-1.4153697110069));
#112686=CARTESIAN_POINT('Ctrl Pts',(7.36370133986324,2.45202942663467,-1.42334204651203));
#112687=CARTESIAN_POINT('',(7.33748629495884,2.36147458031212,-0.733004313422165));
#112688=CARTESIAN_POINT('Origin',(1.99926880606327E-12,2.45311202899956,
-3.96167473826203E-13));
#112689=CARTESIAN_POINT('',(7.36241875102517,2.27159573074673,-1.42996158277913));
#112690=CARTESIAN_POINT('Ctrl Pts',(7.36241875243634,2.27159573307529,-1.42996157417025));
#112691=CARTESIAN_POINT('Ctrl Pts',(7.36814918304015,2.27631121117315,-1.40045740682588));
#112692=CARTESIAN_POINT('Ctrl Pts',(7.37369858250963,2.28101755500325,-1.37093769877651));
#112693=CARTESIAN_POINT('Ctrl Pts',(7.37906705789564,2.2857142859868,-1.34140573896273));
#112694=CARTESIAN_POINT('Ctrl Pts',(7.4061702772824,2.30942614453486,-1.19231104347212));
#112695=CARTESIAN_POINT('Ctrl Pts',(7.42884346071946,2.33338333568924,-1.04188387518592));
#112696=CARTESIAN_POINT('Ctrl Pts',(7.44694337228644,2.35752265840788,-0.890524792629102));
#112697=CARTESIAN_POINT('Ctrl Pts',(7.44793070016065,2.35883942871897,-0.882268341172374));
#112698=CARTESIAN_POINT('Ctrl Pts',(7.44890443167442,2.36015674003959,-0.87400912205204));
#112699=CARTESIAN_POINT('Ctrl Pts',(7.44986454767493,2.36147458179854,-0.865747202052421));
#112700=CARTESIAN_POINT('',(7.23474546263687,2.36147458149274,-1.97698205770052));
#112701=CARTESIAN_POINT('Origin',(-0.182345328122927,2.41070047910294,0.0580309238822652));
#112702=CARTESIAN_POINT('Origin',(-0.187793153545018,2.55351788034799,0.019736059035676));
#112703=CARTESIAN_POINT('Ctrl Pts',(7.11916522,2.492226207,-1.371126025));
#112704=CARTESIAN_POINT('Ctrl Pts',(7.044169235,2.42647128,-1.760520432));
#112705=CARTESIAN_POINT('Ctrl Pts',(6.927150574,2.361474582,-2.139412284));
#112706=CARTESIAN_POINT('Ctrl Pts',(6.92598550493897,2.36082745750497,-2.14318463253374));
#112707=CARTESIAN_POINT('Ctrl Pts',(6.92482043587793,2.36018033300993,-2.14695698106747));
#112708=CARTESIAN_POINT('Ctrl Pts',(7.407209349,2.492226207,-1.176116349));
#112709=CARTESIAN_POINT('Ctrl Pts',(7.34287973799999,2.42647128,-1.581265802));
#112710=CARTESIAN_POINT('Ctrl Pts',(7.234745464,2.361474582,-1.97698206));
#112711=CARTESIAN_POINT('Ctrl Pts',(7.23366885027021,2.36082745750497,-1.98092191681603));
#112712=CARTESIAN_POINT('Ctrl Pts',(7.23259223654041,2.36018033300993,-1.98486177363207));
#112713=CARTESIAN_POINT('',(7.08094802144715,2.36147458056998,-2.05819716358091));
#112714=CARTESIAN_POINT('Ctrl Pts',(6.92947535176304,2.36016764195642,-2.1318849430597));
#112715=CARTESIAN_POINT('Ctrl Pts',(6.92831296288152,2.36082111197821,-2.13564861352985));
#112716=CARTESIAN_POINT('Ctrl Pts',(6.92715057400001,2.361474582,-2.139412284));
#112717=CARTESIAN_POINT('Ctrl Pts',(6.810782318,2.426894312,-2.516198208));
#112718=CARTESIAN_POINT('Ctrl Pts',(6.654232751,2.492218586,-2.878139415));
#112719=CARTESIAN_POINT('Ctrl Pts',(7.0922398216647,2.36016764195642,-2.43930332935916));
#112720=CARTESIAN_POINT('Ctrl Pts',(7.09091030983235,2.36082111197821,-2.44315525167958));
#112721=CARTESIAN_POINT('Ctrl Pts',(7.089580798,2.361474582,-2.447007174));
#112722=CARTESIAN_POINT('Ctrl Pts',(6.956481647,2.426894312,-2.832628105));
#112723=CARTESIAN_POINT('Ctrl Pts',(6.782341609,2.492218586,-3.201537489));
#112724=CARTESIAN_POINT('',(7.08958077776817,2.36147458096341,-2.44700716636999));
#112725=CARTESIAN_POINT('',(6.88556563225692,2.45202942686305,-2.97304322297742));
#112726=CARTESIAN_POINT('Origin',(-0.179764760123894,2.41071407563139,0.0704001507666559));
#112727=CARTESIAN_POINT('Ctrl Pts',(6.65609534086865,2.49144077640618,-2.87382932423452));
#112728=CARTESIAN_POINT('Ctrl Pts',(6.69430052125234,2.48454521316161,-2.89030390998572));
#112729=CARTESIAN_POINT('Ctrl Pts',(6.73254607754049,2.47781843927154,-2.90681926266846));
#112730=CARTESIAN_POINT('Ctrl Pts',(6.80902313486423,2.46469207986071,-2.9398862522766));
#112731=CARTESIAN_POINT('Ctrl Pts',(6.84729823036649,2.45828501823745,-2.95645674151964));
#112732=CARTESIAN_POINT('Ctrl Pts',(6.88556562787249,2.45202942668653,-2.97304321894631));
#112733=CARTESIAN_POINT('',(7.00836568274272,2.36147458031212,-2.29320973895468));
#112734=CARTESIAN_POINT('Origin',(-9.76215636105948E-13,2.45311202899922,
4.39969241594618E-13));
#112735=CARTESIAN_POINT('',(6.88289002122442,2.27159573079936,-2.97923227567974));
#112736=CARTESIAN_POINT('Ctrl Pts',(6.88289002437727,2.27159573313914,-2.97923226743001));
#112737=CARTESIAN_POINT('Ctrl Pts',(6.8948290042822,2.27631121120396,-2.95164976425878));
#112738=CARTESIAN_POINT('Ctrl Pts',(6.90659452628485,2.28101755501304,-2.92401316740996));
#112739=CARTESIAN_POINT('Ctrl Pts',(6.91818598809468,2.28571428603837,-2.89632571177384));
#112740=CARTESIAN_POINT('Ctrl Pts',(6.97670677214404,2.30942625373646,-2.75654251561478));
#112741=CARTESIAN_POINT('Ctrl Pts',(7.03118749456151,2.3333835557567,-2.61450565346097));
#112742=CARTESIAN_POINT('Ctrl Pts',(7.08140215982957,2.35752299096738,-2.47057552999628));
#112743=CARTESIAN_POINT('Ctrl Pts',(7.08414106477529,2.35883965051559,-2.46272501610972));
#112744=CARTESIAN_POINT('Ctrl Pts',(7.08686728833517,2.36015685098211,-2.45486887740036));
#112745=CARTESIAN_POINT('Ctrl Pts',(7.08958079745629,2.36147458179854,-2.44700717495794));
#112746=CARTESIAN_POINT('',(6.64060843113895,2.36147458149276,-3.48601773348323));
#112747=CARTESIAN_POINT('Origin',(-0.165607402435284,2.41070043976848,0.0958731050958894));
#112748=CARTESIAN_POINT('Origin',(-0.179160224013873,2.55351789408286,0.0596447154192725));
#112749=CARTESIAN_POINT('Ctrl Pts',(6.657971528,2.492226207,-2.869479942));
#112750=CARTESIAN_POINT('Ctrl Pts',(6.50102062,2.42647128,-3.233648604));
#112751=CARTESIAN_POINT('Ctrl Pts',(6.30528724300001,2.361474582,-3.578526622));
#112752=CARTESIAN_POINT('Ctrl Pts',(6.30333846919071,2.36082745750497,-3.58196031971256));
#112753=CARTESIAN_POINT('Ctrl Pts',(6.30138969538143,2.36018033300993,-3.58539401742512));
#112754=CARTESIAN_POINT('Ctrl Pts',(6.981202661,2.492226207,-2.740950457));
#112755=CARTESIAN_POINT('Ctrl Pts',(6.831281884,2.42647128,-3.122798776));
#112756=CARTESIAN_POINT('Ctrl Pts',(6.640608432,2.361474582,-3.486017736));
#112757=CARTESIAN_POINT('Ctrl Pts',(6.63871003615623,2.36082745750497,-3.48963404103255));
#112758=CARTESIAN_POINT('Ctrl Pts',(6.63681164031246,2.36018033300993,-3.4932503460651));
#112759=CARTESIAN_POINT('',(6.4729478416998,2.36147458056998,-3.5322721713038));
#112760=CARTESIAN_POINT('Ctrl Pts',(6.30917582457058,2.36016764195642,-3.57167502459223));
#112761=CARTESIAN_POINT('Ctrl Pts',(6.30723153378529,2.36082111197821,-3.57510082329612));
#112762=CARTESIAN_POINT('Ctrl Pts',(6.305287243,2.361474582,-3.578526622));
#112763=CARTESIAN_POINT('Ctrl Pts',(6.110641775,2.426894312,-3.921487766));
#112764=CARTESIAN_POINT('Ctrl Pts',(5.87994559000001,2.492218586,-4.241313459));
#112765=CARTESIAN_POINT('Ctrl Pts',(6.40204908504071,2.36016764195642,-3.90689568945038));
#112766=CARTESIAN_POINT('Ctrl Pts',(6.39992260702036,2.36082111197821,-3.91037175022519));
#112767=CARTESIAN_POINT('Ctrl Pts',(6.397796129,2.361474582,-3.913847811));
#112768=CARTESIAN_POINT('Ctrl Pts',(6.184911661,2.426894312,-4.261840756));
#112769=CARTESIAN_POINT('Ctrl Pts',(5.93553830800001,2.492218586,-4.584690283));
#112770=CARTESIAN_POINT('',(6.39779611089142,2.36147458096338,-3.913847799171));
#112771=CARTESIAN_POINT('',(6.08546852367397,2.45202942687596,-4.38372819973879));
#112772=CARTESIAN_POINT('Origin',(-0.160428043470981,2.41071407866953,0.107398362108932));
#112773=CARTESIAN_POINT('Ctrl Pts',(5.88269117573753,2.49144077634923,-4.23750453653325));
#112774=CARTESIAN_POINT('Ctrl Pts',(5.91646159105472,2.48454521315402,-4.26180694017867));
#112775=CARTESIAN_POINT('Ctrl Pts',(5.95026267507658,2.47781843922848,-4.28615783750334));
#112776=CARTESIAN_POINT('Ctrl Pts',(6.01784331582932,2.46469207986924,-4.33489204607862));
#112777=CARTESIAN_POINT('Ctrl Pts',(6.05166139552129,2.45828501825422,-4.35930314069997));
#112778=CARTESIAN_POINT('Ctrl Pts',(6.08546852022469,2.4520294267061,-4.38372819485558));
#112779=CARTESIAN_POINT('',(6.35154168067892,2.36147458031212,-3.74618722552173));
#112780=CARTESIAN_POINT('Origin',(1.95156391047391E-14,2.45311202900011,
-1.23599047663348E-13));
#112781=CARTESIAN_POINT('',(6.08152500337026,2.27159573077931,-4.38919737833573));
#112782=CARTESIAN_POINT('Ctrl Pts',(6.08152500825334,2.27159573310914,-4.38919737108322));
#112783=CARTESIAN_POINT('Ctrl Pts',(6.09911428445537,2.27631121119346,-4.36482625939919));
#112784=CARTESIAN_POINT('Ctrl Pts',(6.11654578662252,2.28101755501234,-4.3403650303756));
#112785=CARTESIAN_POINT('Ctrl Pts',(6.13381823102573,2.28571428600965,-4.31581671390275));
#112786=CARTESIAN_POINT('Ctrl Pts',(6.22101983715752,2.30942618592822,-4.19188216373346));
#112787=CARTESIAN_POINT('Ctrl Pts',(6.30476032883193,2.33338341906849,-4.06487815968526));
#112788=CARTESIAN_POINT('Ctrl Pts',(6.38474151856246,2.35752278440514,-3.93510809695038));
#112789=CARTESIAN_POINT('Ctrl Pts',(6.38910424716817,2.3588395127513,-3.92802953801965));
#112790=CARTESIAN_POINT('Ctrl Pts',(6.39345579887504,2.36015678207248,-3.92094275878753));
#112791=CARTESIAN_POINT('Ctrl Pts',(6.39779612826307,2.36147458179854,-3.91384781181866));
#112792=CARTESIAN_POINT('',(5.73596392970765,2.36147458149275,-4.83205109335265));
#112793=CARTESIAN_POINT('Origin',(-0.141125708619402,2.4107004559566,0.129232339767804));
#112794=CARTESIAN_POINT('Origin',(-0.162149707107304,2.5535178731589,0.0967644146262725));
#112795=CARTESIAN_POINT('Ctrl Pts',(5.885458487,2.492226207,-4.233660165));
#112796=CARTESIAN_POINT('Ctrl Pts',(5.653891507,2.42647128,-4.555574961));
#112797=CARTESIAN_POINT('Ctrl Pts',(5.388595688,2.361474582,-4.850313032));
#112798=CARTESIAN_POINT('Ctrl Pts',(5.38595433192827,2.36082745750497,-4.8532475230008));
#112799=CARTESIAN_POINT('Ctrl Pts',(5.38331297585654,2.36018033300993,-4.85618201400161));
#112800=CARTESIAN_POINT('Ctrl Pts',(6.228762696,2.492226207,-4.177620768));
#112801=CARTESIAN_POINT('Ctrl Pts',(6.000260882,2.42647128,-4.51831315));
#112802=CARTESIAN_POINT('Ctrl Pts',(5.73596393,2.361474582,-4.832051096));
#112803=CARTESIAN_POINT('Ctrl Pts',(5.73333251891506,2.36082745750497,-4.83517475483384));
#112804=CARTESIAN_POINT('Ctrl Pts',(5.73070110783012,2.36018033300993,-4.83829841366768));
#112805=CARTESIAN_POINT('',(5.56227981475606,2.36147458056998,-4.84118205738657));
#112806=CARTESIAN_POINT('Ctrl Pts',(5.39386624760077,2.36016764195642,-4.84445755122613));
#112807=CARTESIAN_POINT('Ctrl Pts',(5.39123096780039,2.36082111197821,-4.84738529161306));
#112808=CARTESIAN_POINT('Ctrl Pts',(5.38859568799999,2.361474582,-4.850313032));
#112809=CARTESIAN_POINT('Ctrl Pts',(5.124774415,2.426894312,-5.143412913));
#112810=CARTESIAN_POINT('Ctrl Pts',(4.830718708,2.492218586,-5.40616839900001));
#112811=CARTESIAN_POINT('Ctrl Pts',(5.41250564892147,2.36016764195642,-5.19180595003168));
#112812=CARTESIAN_POINT('Ctrl Pts',(5.40968163646073,2.36082111197821,-5.19474361251584));
#112813=CARTESIAN_POINT('Ctrl Pts',(5.406857624,2.361474582,-5.197681275));
#112814=CARTESIAN_POINT('Ctrl Pts',(5.12414208000001,2.426894312,-5.49177447));
#112815=CARTESIAN_POINT('Ctrl Pts',(4.811195832,2.492218586,-5.75346805500001));
#112816=CARTESIAN_POINT('',(5.40685760886689,2.36147458096338,-5.19768125953299));
#112817=CARTESIAN_POINT('',(5.00082167051335,2.4520294268514,-5.58943491793815));
#112818=CARTESIAN_POINT('Origin',(-0.133589863414661,2.41071407407032,0.139374754044277));
#112819=CARTESIAN_POINT('Ctrl Pts',(4.83421890979896,2.49144077619964,-5.40303874779536));
#112820=CARTESIAN_POINT('Ctrl Pts',(4.86197549339698,2.48454521296006,-5.43403261592637));
#112821=CARTESIAN_POINT('Ctrl Pts',(4.88975160320432,2.47781843917396,-5.46508043601207));
#112822=CARTESIAN_POINT('Ctrl Pts',(4.94527583200974,2.46469207979229,-5.52720310597014));
#112823=CARTESIAN_POINT('Ctrl Pts',(4.97305559996261,2.45828501819729,-5.5583133701044));
#112824=CARTESIAN_POINT('Ctrl Pts',(5.00082166815137,2.45202942666902,-5.58943491241765));
#112825=CARTESIAN_POINT('',(5.39772664886391,2.36147458031212,-5.02399716116693));
#112826=CARTESIAN_POINT('Origin',(3.0140820395097E-13,2.45311202899956,
-4.33680868994202E-13));
#112827=CARTESIAN_POINT('',(4.99579463605586,2.2715957307672,-5.59392849012071));
#112828=CARTESIAN_POINT('Ctrl Pts',(4.99579464238751,2.27159573309948,-5.5939284840713));
#112829=CARTESIAN_POINT('Ctrl Pts',(5.01821175973075,2.27631121118552,-5.57390832984172));
#112830=CARTESIAN_POINT('Ctrl Pts',(5.04049416430141,2.28101755500763,-5.55376624842468));
#112831=CARTESIAN_POINT('Ctrl Pts',(5.06263995095078,2.28571428598914,-5.53350492287605));
#112832=CARTESIAN_POINT('Ctrl Pts',(5.17444495087571,2.30942615500799,-5.43121379376971));
#112833=CARTESIAN_POINT('Ctrl Pts',(5.28352960527545,2.33338335682526,-5.32518094602194));
#112834=CARTESIAN_POINT('Ctrl Pts',(5.38953747703969,2.35752269035039,-5.21563857865579));
#112835=CARTESIAN_POINT('Ctrl Pts',(5.39532002651813,2.35883945002269,-5.20966322844134));
#112836=CARTESIAN_POINT('Ctrl Pts',(5.40109342709373,2.36015675069572,-5.20367744691155));
#112837=CARTESIAN_POINT('Ctrl Pts',(5.40685762310432,2.36147458179854,-5.1976812756411));
#112838=CARTESIAN_POINT('',(4.56311212928963,2.36147458149275,-5.95214311534979));
#112839=CARTESIAN_POINT('Origin',(-0.110044981492499,2.41070042225928,0.156548632073102));
#112840=CARTESIAN_POINT('Origin',(-0.137556999251891,2.55351788794162,0.129359209222423));
#112841=CARTESIAN_POINT('Ctrl Pts',(4.837747949,2.492226207,-5.399879145));
#112842=CARTESIAN_POINT('Ctrl Pts',(4.542392711,2.42647128,-5.664487697));
#112843=CARTESIAN_POINT('Ctrl Pts',(4.219939387,2.361474582,-5.895304196));
#112844=CARTESIAN_POINT('Ctrl Pts',(4.21672895553369,2.36082745750497,-5.89760226674754));
#112845=CARTESIAN_POINT('Ctrl Pts',(4.21351852406738,2.36018033300993,-5.89990033749508));
#112846=CARTESIAN_POINT('Ctrl Pts',(5.18507271,2.492226207,-5.418950174));
#112847=CARTESIAN_POINT('Ctrl Pts',(4.888674351,2.42647128,-5.702556223));
#112848=CARTESIAN_POINT('Ctrl Pts',(4.563112129,2.361474582,-5.952143118));
#112849=CARTESIAN_POINT('Ctrl Pts',(4.55987074451438,2.36082745750497,-5.95462807182634));
#112850=CARTESIAN_POINT('Ctrl Pts',(4.55662936002876,2.36018033300993,-5.95711302565267));
#112851=CARTESIAN_POINT('',(4.39152576504318,2.36147458056998,-5.92372365177857));
#112852=CARTESIAN_POINT('Ctrl Pts',(4.22634547911204,2.36016764195642,-5.89071862761956));
#112853=CARTESIAN_POINT('Ctrl Pts',(4.22314243305602,2.36082111197821,-5.89301141180978));
#112854=CARTESIAN_POINT('Ctrl Pts',(4.219939387,2.361474582,-5.895304196));
#112855=CARTESIAN_POINT('Ctrl Pts',(3.899278299,2.426894312,-6.12483779));
#112856=CARTESIAN_POINT('Ctrl Pts',(3.555612789,2.492218586,-6.318236914));
#112857=CARTESIAN_POINT('Ctrl Pts',(4.16987946444665,2.36016764195642,-6.23395313325984));
#112858=CARTESIAN_POINT('Ctrl Pts',(4.16648996522332,2.36082111197821,-6.23621503562992));
#112859=CARTESIAN_POINT('Ctrl Pts',(4.163100466,2.361474582,-6.238476938));
#112860=CARTESIAN_POINT('Ctrl Pts',(3.82377331,2.426894312,-6.46491891300001));
#112861=CARTESIAN_POINT('Ctrl Pts',(3.461887187,2.492218586,-6.653220055));
#112862=CARTESIAN_POINT('',(4.16310045450136,2.36147458096341,-6.23847691969746));
#112863=CARTESIAN_POINT('',(3.68234195387786,2.45202942688314,-6.53378587147896));
#112864=CARTESIAN_POINT('Origin',(-0.100505229271112,2.41071409629437,0.164834243166782));
#112865=CARTESIAN_POINT('Ctrl Pts',(3.55970394000875,2.49144077637471,-6.31593287126581));
#112866=CARTESIAN_POINT('Ctrl Pts',(3.58014882443327,2.48454521317143,-6.35216896470848));
#112867=CARTESIAN_POINT('Ctrl Pts',(3.60060118099897,2.47781843924586,-6.38846194721864));
#112868=CARTESIAN_POINT('Ctrl Pts',(3.64147274625851,2.46469207987447,-6.46106829132436));
#112869=CARTESIAN_POINT('Ctrl Pts',(3.66191525146325,2.45828501826216,-6.49742304371203));
#112870=CARTESIAN_POINT('Ctrl Pts',(3.68234195274149,2.4520294267171,-6.5337858655678));
#112871=CARTESIAN_POINT('',(4.19151991788259,2.36147458031212,-6.06689057295364));
#112872=CARTESIAN_POINT('Origin',(-3.29163779566599E-13,2.453112029,5.62917767954474E-13));
#112873=CARTESIAN_POINT('',(3.6764664637425,2.27159573079627,-6.53709372270527));
#112874=CARTESIAN_POINT('Ctrl Pts',(3.67646647129025,2.27159573315182,-6.53709371793003));
#112875=CARTESIAN_POINT('Ctrl Pts',(3.70266323014006,2.27631121120201,-6.52236064107112));
#112876=CARTESIAN_POINT('Ctrl Pts',(3.72875463649749,2.28101755500699,-6.50747952845856));
#112877=CARTESIAN_POINT('Ctrl Pts',(3.75473825304687,2.28571428600847,-6.4924525909729));
#112878=CARTESIAN_POINT('Ctrl Pts',(3.88591898369805,2.30942617320938,-6.41658768496772));
#112879=CARTESIAN_POINT('Ctrl Pts',(4.01524732444754,2.33338339338091,-6.33648373760001));
#112880=CARTESIAN_POINT('Ctrl Pts',(4.14232525569792,2.35752274558242,-6.25229089772399));
#112881=CARTESIAN_POINT('Ctrl Pts',(4.14925703895402,2.35883948685887,-6.24769838892255));
#112882=CARTESIAN_POINT('Ctrl Pts',(4.15618212981563,2.36015676912106,-6.24309372628041));
#112883=CARTESIAN_POINT('Ctrl Pts',(4.16310046498744,2.36147458179854,-6.23847693843357));
#112884=CARTESIAN_POINT('',(3.1768942778333,2.36147458149276,-6.79391954047577));
#112885=CARTESIAN_POINT('Origin',(-0.0738188840871684,2.41070043582995,
0.176545072828828));
#112886=CARTESIAN_POINT('Origin',(-0.106532826126692,2.5535179002561,0.155905997732412));
#112887=CARTESIAN_POINT('Ctrl Pts',(3.563829693,2.492226207,-6.313605778));
#112888=CARTESIAN_POINT('Ctrl Pts',(3.21849668,2.42647128,-6.508535283));
#112889=CARTESIAN_POINT('Ctrl Pts',(2.853963411,2.361474582,-6.664637488));
#112890=CARTESIAN_POINT('Ctrl Pts',(2.85033402035581,2.36082745750497,-6.66619168326981));
#112891=CARTESIAN_POINT('Ctrl Pts',(2.84670462971162,2.36018033300993,-6.6677458785396));
#112892=CARTESIAN_POINT('Ctrl Pts',(3.898934487,2.492226207,-6.406895494));
#112893=CARTESIAN_POINT('Ctrl Pts',(3.548498839,2.42647128,-6.620154104));
#112894=CARTESIAN_POINT('Ctrl Pts',(3.176894277,2.361474582,-6.79391954300001));
#112895=CARTESIAN_POINT('Ctrl Pts',(3.17319448267296,2.36082745750497,-6.79564959814783));
#112896=CARTESIAN_POINT('Ctrl Pts',(3.16949468834593,2.36018033300993,-6.79737965329567));
#112897=CARTESIAN_POINT('',(3.01542885200097,2.36147458056998,-6.72927851191472));
#112898=CARTESIAN_POINT('Ctrl Pts',(2.86120549389769,2.36016764195642,-6.66153624811899));
#112899=CARTESIAN_POINT('Ctrl Pts',(2.85758445244885,2.36082111197821,-6.66308686805949));
#112900=CARTESIAN_POINT('Ctrl Pts',(2.853963411,2.361474582,-6.664637488));
#112901=CARTESIAN_POINT('Ctrl Pts',(2.491456263,2.426894312,-6.819872058));
#112902=CARTESIAN_POINT('Ctrl Pts',(2.114250367,2.492218586,-6.934871692));
#112903=CARTESIAN_POINT('Ctrl Pts',(2.7322743505124,2.36016764195642,-6.98460759756821));
#112904=CARTESIAN_POINT('Ctrl Pts',(2.7284778537562,2.36082111197821,-6.9860879757841));
#112905=CARTESIAN_POINT('Ctrl Pts',(2.724681357,2.361474582,-6.98756835400001));
#112906=CARTESIAN_POINT('Ctrl Pts',(2.344609151,2.426894312,-7.13577093400001));
#112907=CARTESIAN_POINT('Ctrl Pts',(1.950704544,2.492218586,-7.24187488));
#112908=CARTESIAN_POINT('',(2.72468134975038,2.36147458096339,-6.98756833361612));
#112909=CARTESIAN_POINT('',(2.19168002063031,2.45202942684316,-7.1726242596834));
#112910=CARTESIAN_POINT('Origin',(-0.0627208430799763,2.4107140698826,0.182585748484438));
#112911=CARTESIAN_POINT('Ctrl Pts',(2.11874117040428,2.49144077629052,-6.93350099351369));
#112912=CARTESIAN_POINT('Ctrl Pts',(2.13091837590245,2.48454521305579,-6.97328495320926));
#112913=CARTESIAN_POINT('Ctrl Pts',(2.14309064927467,2.47781843918746,-7.01312607778268));
#112914=CARTESIAN_POINT('Ctrl Pts',(2.16739844250754,2.46469207980608,-7.09282110454116));
#112915=CARTESIAN_POINT('Ctrl Pts',(2.17954781629908,2.45828501819535,-7.13272043748061));
#112916=CARTESIAN_POINT('Ctrl Pts',(2.19168002095519,2.45202942665626,-7.17262425381494));
#112917=CARTESIAN_POINT('',(2.78932237430421,2.36147458031212,-6.82610292496196));
#112918=CARTESIAN_POINT('Origin',(-3.60605642568679E-13,2.45311202900022,
9.36750677027476E-13));
#112919=CARTESIAN_POINT('',(2.18523080563448,2.27159573074892,-7.1745917181958));
#112920=CARTESIAN_POINT('Ctrl Pts',(2.1852308139442,2.27159573308574,-7.17459171531735));
#112921=CARTESIAN_POINT('Ctrl Pts',(2.2139822832731,2.27631121117266,-7.16583461865168));
#112922=CARTESIAN_POINT('Ctrl Pts',(2.24266268651128,2.28101755499938,-7.15691029945946));
#112923=CARTESIAN_POINT('Ctrl Pts',(2.2712691678847,2.28571428597161,-7.14782039293411));
#112924=CARTESIAN_POINT('Ctrl Pts',(2.41569123321526,2.30942610013226,-7.10192928621603));
#112925=CARTESIAN_POINT('Ctrl Pts',(2.55921549262729,2.33338324614021,-7.05150006404015));
#112926=CARTESIAN_POINT('Ctrl Pts',(2.70142095576105,2.35752252307876,-6.99659380100814));
#112927=CARTESIAN_POINT('Ctrl Pts',(2.7091783687944,2.35883933846272,-6.99359862381121));
#112928=CARTESIAN_POINT('Ctrl Pts',(2.71693185817446,2.36015669489342,-6.99059013675634));
#112929=CARTESIAN_POINT('Ctrl Pts',(2.72468135591791,2.36147458179854,-6.98756835420575));
#112930=CARTESIAN_POINT('',(1.64212838139087,2.36147458149274,-7.31801983771833));
#112931=CARTESIAN_POINT('Origin',(-0.0341410904291883,2.41070048836924,
0.188286562001653));
#112932=CARTESIAN_POINT('Origin',(-0.0705268457592495,2.55351783676061,
0.175162031699275));
#112933=CARTESIAN_POINT('Ctrl Pts',(2.123270722,2.492226207,-6.932115221));
#112934=CARTESIAN_POINT('Ctrl Pts',(1.744107321,2.42647128,-7.048250993));
#112935=CARTESIAN_POINT('Ctrl Pts',(1.354539278,2.361474582,-7.12233973800001));
#112936=CARTESIAN_POINT('Ctrl Pts',(1.35066063445556,2.36082745750497,-7.12307738534472));
#112937=CARTESIAN_POINT('Ctrl Pts',(1.34678199091112,2.36018033300993,-7.12381503268945));
#112938=CARTESIAN_POINT('Ctrl Pts',(2.430486421,2.492226207,-7.0952615));
#112939=CARTESIAN_POINT('Ctrl Pts',(2.042399466,2.42647128,-7.228200938));
#112940=CARTESIAN_POINT('Ctrl Pts',(1.64212838,2.361474582,-7.31801984));
#112941=CARTESIAN_POINT('Ctrl Pts',(1.63814317409917,2.36082745750497,-7.31891410099156));
#112942=CARTESIAN_POINT('Ctrl Pts',(1.63415796819833,2.36018033300993,-7.31980836198311));
#112943=CARTESIAN_POINT('',(1.49833383758464,2.36147458056998,-7.22017978721851));
#112944=CARTESIAN_POINT('Ctrl Pts',(1.36227871992292,2.36016764195642,-7.12086783712926));
#112945=CARTESIAN_POINT('Ctrl Pts',(1.35840899896146,2.36082111197821,-7.12160378756463));
#112946=CARTESIAN_POINT('Ctrl Pts',(1.354539278,2.361474582,-7.122339738));
#112947=CARTESIAN_POINT('Ctrl Pts',(0.967136502,2.426894312,-7.19601668900001));
#112948=CARTESIAN_POINT('Ctrl Pts',(0.574027948,2.492218586,-7.227239578));
#112949=CARTESIAN_POINT('Ctrl Pts',(1.16691112465914,2.36016764195642,-7.40866957357816));
#112950=CARTESIAN_POINT('Ctrl Pts',(1.16288515032957,2.36082111197821,-7.40929920678909));
#112951=CARTESIAN_POINT('Ctrl Pts',(1.158859176,2.361474582,-7.40992884));
#112952=CARTESIAN_POINT('Ctrl Pts',(0.755813673,2.426894312,-7.472962236));
#112953=CARTESIAN_POINT('Ctrl Pts',(0.348309125,2.492218586,-7.491907685));
#112954=CARTESIAN_POINT('',(1.15885917331566,2.36147458096338,-7.40992881852834));
#112955=CARTESIAN_POINT('',(0.598537565187556,2.45202942683418,-7.47607870941393));
#112956=CARTESIAN_POINT('Origin',(-0.0220039527230042,2.41071407041494,
0.191800369024843));
#112957=CARTESIAN_POINT('Ctrl Pts',(0.578708418762666,2.49144077643974,
-7.226866314466));
#112958=CARTESIAN_POINT('Ctrl Pts',(0.582048552589304,2.48454521326316,
-7.26833788628168));
#112959=CARTESIAN_POINT('Ctrl Pts',(0.58537158092354,2.47781843925376,-7.30986422738255));
#112960=CARTESIAN_POINT('Ctrl Pts',(0.591978996387378,2.4646920798733,-7.39292148573499));
#112961=CARTESIAN_POINT('Ctrl Pts',(0.595267147371582,2.45828501822336,
-7.43449975091216));
#112962=CARTESIAN_POINT('Ctrl Pts',(0.598537566821972,2.45202942664249,
-7.47607870383028));
#112963=CARTESIAN_POINT('',(1.25669921667918,2.36147458031212,-7.26613429078502));
#112964=CARTESIAN_POINT('Origin',(-1.70999011391698E-14,2.45311202899944,
3.44342609981396E-13));
#112965=CARTESIAN_POINT('',(0.591816183403944,2.27159573078526,-7.47661377876439));
#112966=CARTESIAN_POINT('Ctrl Pts',(0.591816192120807,2.27159573311852,
-7.47661377775117));
#112967=CARTESIAN_POINT('Ctrl Pts',(0.621777984919688,2.2763112111963,-7.47424213319847));
#112968=CARTESIAN_POINT('Ctrl Pts',(0.65170632102208,2.28101755501207,-7.47169189856643));
#112969=CARTESIAN_POINT('Ctrl Pts',(0.681598059968947,2.28571428597833,
-7.46896405687537));
#112970=CARTESIAN_POINT('Ctrl Pts',(0.832509017219529,2.30942612645993,
-7.45519231806404));
#112971=CARTESIAN_POINT('Ctrl Pts',(0.983518718670204,2.33338329926306,
-7.43679555110876));
#112972=CARTESIAN_POINT('Ctrl Pts',(1.13420288686114,2.35752260336165,-7.4137429016284));
#112973=CARTESIAN_POINT('Ctrl Pts',(1.1424226433557,2.35883939200654,-7.41248538952506));
#112974=CARTESIAN_POINT('Ctrl Pts',(1.15064142919396,2.36015672167605,-7.41121403583437));
#112975=CARTESIAN_POINT('Ctrl Pts',(1.15885917489897,2.36147458179854,-7.40992883996832));
#112976=CARTESIAN_POINT('',(0.0305783858254816,2.36147458149275,-7.49993766206233));
#112977=CARTESIAN_POINT('Origin',(0.00713314255944587,2.41070046639263,
0.191223796676153));
#112978=CARTESIAN_POINT('Origin',(-0.0312233225700945,2.55351786385627,
0.186228177215475));
#112979=CARTESIAN_POINT('Ctrl Pts',(0.583429972,2.492226207,-7.226486661));
#112980=CARTESIAN_POINT('Ctrl Pts',(0.188165442,2.42647128,-7.25839832));
#112981=CARTESIAN_POINT('Ctrl Pts',(-0.208221606,2.361474582,-7.247009298));
#112982=CARTESIAN_POINT('Ctrl Pts',(-0.212168141380535,2.36082745750497,
-7.24689590585336));
#112983=CARTESIAN_POINT('Ctrl Pts',(-0.216114676761069,2.36018033300993,
-7.24678251370672));
#112984=CARTESIAN_POINT('Ctrl Pts',(0.848391511,2.492226207,-7.451860965));
#112985=CARTESIAN_POINT('Ctrl Pts',(0.440799764,2.42647128,-7.498265129));
#112986=CARTESIAN_POINT('Ctrl Pts',(0.030578384,2.361474582,-7.499937664));
#112987=CARTESIAN_POINT('Ctrl Pts',(0.0264941103129808,2.36082745750497,
-7.49995431620543));
#112988=CARTESIAN_POINT('Ctrl Pts',(0.0224098366259617,2.36018033300993,
-7.49997096841086));
#112989=CARTESIAN_POINT('',(-0.0888216022330978,2.36147458056998,-7.37347348110561));
#112990=CARTESIAN_POINT('Ctrl Pts',(-0.200346692749638,2.36016764195642,
-7.24723556060147));
#112991=CARTESIAN_POINT('Ctrl Pts',(-0.204284149374819,2.36082111197821,
-7.24712242930074));
#112992=CARTESIAN_POINT('Ctrl Pts',(-0.208221606,2.361474582,-7.247009298));
#112993=CARTESIAN_POINT('Ctrl Pts',(-0.602405487,2.426894312,-7.235683577));
#112994=CARTESIAN_POINT('Ctrl Pts',(-0.99303538,2.492218586,-7.181669773));
#112995=CARTESIAN_POINT('Ctrl Pts',(-0.453015568348983,2.36016764195642,
-7.48631039345565));
#112996=CARTESIAN_POINT('Ctrl Pts',(-0.457082770174491,2.36082111197821,
-7.48605984072782));
#112997=CARTESIAN_POINT('Ctrl Pts',(-0.461149972,2.361474582,-7.485809288));
#112998=CARTESIAN_POINT('Ctrl Pts',(-0.868322813,2.426894312,-7.46072613));
#112999=CARTESIAN_POINT('Ctrl Pts',(-1.270372842,2.492218586,-7.391627212));
#113000=CARTESIAN_POINT('',(-0.461149970041696,2.36147458096337,-7.48580926646544));
#113001=CARTESIAN_POINT('',(-1.02259184184624,2.45202942681409,-7.42996002746998));
#113002=CARTESIAN_POINT('Origin',(0.0197418695140492,2.41071412747366,0.192046098608932));
#113003=CARTESIAN_POINT('Ctrl Pts',(-0.988384096490083,2.49144077631088,
-7.18231140053096));
#113004=CARTESIAN_POINT('Ctrl Pts',(-0.994037214993464,2.484545213046,-7.22353142046831));
#113005=CARTESIAN_POINT('Ctrl Pts',(-0.999718812712841,2.47781843921912,
-7.26480125044355));
#113006=CARTESIAN_POINT('Ctrl Pts',(-1.01112073014719,2.4646920797927,-7.34733707540548));
#113007=CARTESIAN_POINT('Ctrl Pts',(-1.01684755219409,2.45828501816591,
-7.38865011890989));
#113008=CARTESIAN_POINT('Ctrl Pts',(-1.02259183909231,2.45202942661235,
-7.42996002228574));
#113009=CARTESIAN_POINT('',(-0.334685799463248,2.36147458031212,-7.36640929252461));
#113010=CARTESIAN_POINT('Origin',(-2.13289672382211E-13,2.45311202900011,
-9.91394466520745E-13));
#113011=CARTESIAN_POINT('',(-1.02927110528062,2.2715957307877,-7.42903768924827));
#113012=CARTESIAN_POINT('Ctrl Pts',(-1.0292710965881,2.27159573311762,-7.42903769016891));
#113013=CARTESIAN_POINT('Ctrl Pts',(-0.99949996036425,2.27631121119929,
-7.43316239308187));
#113014=CARTESIAN_POINT('Ctrl Pts',(-0.969723107050798,2.28101755501532,
-7.43710548900528));
#113015=CARTESIAN_POINT('Ctrl Pts',(-0.939943815032056,2.28571428599494,
-7.44086726299595));
#113016=CARTESIAN_POINT('Ctrl Pts',(-0.78960049165936,2.3094261366726,-7.4598589037277));
#113017=CARTESIAN_POINT('Ctrl Pts',(-0.638166486807453,2.33338331970726,
-7.47435486833261));
#113018=CARTESIAN_POINT('Ctrl Pts',(-0.486049526748782,2.35752263424557,
-7.48423381842671));
#113019=CARTESIAN_POINT('Ctrl Pts',(-0.477751680484724,2.35883941260402,
-7.484772706458));
#113020=CARTESIAN_POINT('Ctrl Pts',(-0.469451806683069,2.3601567319788,
-7.48529786806292));
#113021=CARTESIAN_POINT('Ctrl Pts',(-0.461149973068477,2.36147458179854,
-7.48580928773238));
#113022=CARTESIAN_POINT('',(-1.58240141979816,2.36147458149275,-7.33116673650159));
#113023=CARTESIAN_POINT('Origin',(0.0480737921281871,2.4107004486788,0.185219410287693));
#113024=CARTESIAN_POINT('Origin',(0.00954017434101576,2.55351784356558,
0.188586111362571));
#113025=CARTESIAN_POINT('Ctrl Pts',(-0.983691316,2.492226207,-7.18295561700001));
#113026=CARTESIAN_POINT('Ctrl Pts',(-1.376574843,2.42647128,-7.12915100900001));
#113027=CARTESIAN_POINT('Ctrl Pts',(-1.76124628,2.361474582,-7.032816757));
#113028=CARTESIAN_POINT('Ctrl Pts',(-1.76507617162653,2.36082745750497,
-7.03185762744268));
#113029=CARTESIAN_POINT('Ctrl Pts',(-1.76890606325307,2.36018033300993,
-7.03089849788536));
#113030=CARTESIAN_POINT('Ctrl Pts',(-0.773373243,2.492226207,-7.460019693));
#113031=CARTESIAN_POINT('Ctrl Pts',(-1.181411245,2.42647128,-7.417718777));
#113032=CARTESIAN_POINT('Ctrl Pts',(-1.582401422,2.361474582,-7.33116673800001));
#113033=CARTESIAN_POINT('Ctrl Pts',(-1.586393787363,2.36082745750497,-7.33030500276952));
#113034=CARTESIAN_POINT('Ctrl Pts',(-1.590386152726,2.36018033300993,-7.32944326753903));
#113035=CARTESIAN_POINT('',(-1.67182384246072,2.36147458056997,-7.18199174948777));
#113036=CARTESIAN_POINT('Ctrl Pts',(-1.75360411761002,2.36016764195642,
-7.03473060324848));
#113037=CARTESIAN_POINT('Ctrl Pts',(-1.75742519880501,2.36082111197821,
-7.03377368012423));
#113038=CARTESIAN_POINT('Ctrl Pts',(-1.76124628,2.361474582,-7.032816757));
#113039=CARTESIAN_POINT('Ctrl Pts',(-2.143779666,2.426894312,-6.937017944));
#113040=CARTESIAN_POINT('Ctrl Pts',(-2.513665477,2.492218586,-6.800293072));
#113041=CARTESIAN_POINT('Ctrl Pts',(-2.05175975706096,2.36016764195642,
-7.2138996612507));
#113042=CARTESIAN_POINT('Ctrl Pts',(-2.05567800853048,2.36082111197821,
-7.21278063812536));
#113043=CARTESIAN_POINT('Ctrl Pts',(-2.05959626,2.361474582,-7.211661615));
#113044=CARTESIAN_POINT('Ctrl Pts',(-2.451857488,2.426894312,-7.099634761));
#113045=CARTESIAN_POINT('Ctrl Pts',(-2.829653587,2.492218586,-6.945722466));
#113046=CARTESIAN_POINT('',(-2.05959625342164,2.36147458096337,-7.21166159438652));
#113047=CARTESIAN_POINT('',(-2.59590599068159,2.45202942681774,-7.0364246722059));
#113048=CARTESIAN_POINT('Origin',(0.0605646944270258,2.41071409752193,0.183312664479299));
#113049=CARTESIAN_POINT('Ctrl Pts',(-2.50926086840674,2.49144077630432,
-6.80191958692098));
#113050=CARTESIAN_POINT('Ctrl Pts',(-2.52364290615911,2.48454521307526,
-6.84096065213392));
#113051=CARTESIAN_POINT('Ctrl Pts',(-2.53806346503165,2.47781843922134,
-6.88004424096436));
#113052=CARTESIAN_POINT('Ctrl Pts',(-2.56694157478326,2.46469207980874,
-6.95819934878544));
#113053=CARTESIAN_POINT('Ctrl Pts',(-2.5814155901075,2.45828501817934,-6.9973154187694));
#113054=CARTESIAN_POINT('Ctrl Pts',(-2.59590598689054,2.45202942661805,
-7.03642466765963));
#113055=CARTESIAN_POINT('',(-1.91042128011643,2.36147458031212,-7.12223918328643));
#113056=CARTESIAN_POINT('Origin',(-4.23706209007335E-13,2.45311202900022,
-9.58001039608192E-13));
#113057=CARTESIAN_POINT('',(-2.60223082121476,2.27159573077689,-7.0340880540497));
#113058=CARTESIAN_POINT('Ctrl Pts',(-2.6022308128611,2.27159573311295,-7.03408805678627));
#113059=CARTESIAN_POINT('Ctrl Pts',(-2.57404239845067,2.27631121119102,
-7.04451624071727));
#113060=CARTESIAN_POINT('Ctrl Pts',(-2.54580936050126,2.28101755500866,
-7.05476829257287));
#113061=CARTESIAN_POINT('Ctrl Pts',(-2.51753496199034,2.28571428597445,
-7.06484378586096));
#113062=CARTESIAN_POINT('Ctrl Pts',(-2.37478933436481,2.30942611803928,
-7.11571074207617));
#113063=CARTESIAN_POINT('Ctrl Pts',(-2.23001209113176,2.33338328229228,
-7.16242160133055));
#113064=CARTESIAN_POINT('Ctrl Pts',(-2.0835753404843,2.35752257771581,-7.20477021148193));
#113065=CARTESIAN_POINT('Ctrl Pts',(-2.07558722410083,2.35883937490235,
-7.20708032574677));
#113066=CARTESIAN_POINT('Ctrl Pts',(-2.06759417666474,2.36015671312055,
-7.20937746999141));
#113067=CARTESIAN_POINT('Ctrl Pts',(-2.05959626098597,2.36147458179854,
-7.21166161450894));
#113068=CARTESIAN_POINT('',(-3.1213898945122,2.36147458149274,-6.81959860202504));
#113069=CARTESIAN_POINT('Origin',(0.0867666093167069,2.41070047480533,0.170554746132112));
#113070=CARTESIAN_POINT('Origin',(0.0498576749899327,2.55351787035918,0.182126480656974));
#113071=CARTESIAN_POINT('Ctrl Pts',(-2.50481629,2.492226207,-6.803557551));
#113072=CARTESIAN_POINT('Ctrl Pts',(-2.876948019,2.42647128,-6.66655252));
#113073=CARTESIAN_POINT('Ctrl Pts',(-3.231917035,2.361474582,-6.489777522));
#113074=CARTESIAN_POINT('Ctrl Pts',(-3.23545120138537,2.36082745750497,
-6.48801750287848));
#113075=CARTESIAN_POINT('Ctrl Pts',(-3.23898536777074,2.36018033300993,
-6.48625748375697));
#113076=CARTESIAN_POINT('Ctrl Pts',(-2.358975924,2.492226207,-7.11935619199999));
#113077=CARTESIAN_POINT('Ctrl Pts',(-2.748380777,2.42647128,-6.990328138));
#113078=CARTESIAN_POINT('Ctrl Pts',(-3.121389897,2.361474582,-6.819598603));
#113079=CARTESIAN_POINT('Ctrl Pts',(-3.12510367548184,2.36082745750497,
-6.8178987741237));
#113080=CARTESIAN_POINT('Ctrl Pts',(-3.12881745396368,2.36018033300993,
-6.81619894524741));
#113081=CARTESIAN_POINT('',(-3.17665345808772,2.36147458056998,-6.65468806627697));
#113082=CARTESIAN_POINT('Ctrl Pts',(-3.22486496249061,2.36016764195642,
-6.49328946261241));
#113083=CARTESIAN_POINT('Ctrl Pts',(-3.22839099874531,2.36082111197821,
-6.49153349230621));
#113084=CARTESIAN_POINT('Ctrl Pts',(-3.231917035,2.361474582,-6.489777522));
#113085=CARTESIAN_POINT('Ctrl Pts',(-3.58491309,2.426894312,-6.313985061));
#113086=CARTESIAN_POINT('Ctrl Pts',(-3.916759371,2.492218586,-6.100942225));
#113087=CARTESIAN_POINT('Ctrl Pts',(-3.55456593991965,2.36016764195642,
-6.60417499745423));
#113088=CARTESIAN_POINT('Ctrl Pts',(-3.55815202795983,2.36082111197821,
-6.60223982822711));
#113089=CARTESIAN_POINT('Ctrl Pts',(-3.561738116,2.361474582,-6.600304659));
#113090=CARTESIAN_POINT('Ctrl Pts',(-3.920746033,2.426894312,-6.406572362));
#113091=CARTESIAN_POINT('Ctrl Pts',(-4.256622874,2.492218586,-6.175043458));
#113092=CARTESIAN_POINT('',(-3.56173810521021,2.36147458096338,-6.60030464027285));
#113093=CARTESIAN_POINT('',(-4.04783846069933,2.45202942686021,-6.3138739202179));
#113094=CARTESIAN_POINT('Origin',(0.0985555131148149,2.41071414370196,0.166007272848912));
#113095=CARTESIAN_POINT('Ctrl Pts',(-3.91280739158238,2.4914407763751,-6.10347757308063));
#113096=CARTESIAN_POINT('Ctrl Pts',(-3.93524586013339,2.48454521318475,
-6.13851416683736));
#113097=CARTESIAN_POINT('Ctrl Pts',(-3.95773109099203,2.47781843923352,
-6.17358400978743));
#113098=CARTESIAN_POINT('Ctrl Pts',(-4.00273507261549,2.46469208331324,
-6.2437039360965));
#113099=CARTESIAN_POINT('Ctrl Pts',(-4.02527947815753,2.45828502544634,
-6.27879398664533));
#113100=CARTESIAN_POINT('Ctrl Pts',(-4.04783845597553,2.4520294266905,-6.31387391636804));
#113101=CARTESIAN_POINT('',(-3.39682758479658,2.36147458031212,-6.54504108567515));
#113102=CARTESIAN_POINT('Origin',(-4.72278466334686E-13,2.45311202899944,
-7.53303669442928E-13));
#113103=CARTESIAN_POINT('',(-4.0535131159682,2.27159573076159,-6.3102322787032));
#113104=CARTESIAN_POINT('Ctrl Pts',(-4.05351310848486,2.27159573309017,
-6.31023228319568));
#113105=CARTESIAN_POINT('Ctrl Pts',(-4.02822547480738,2.27631121118252,
-6.32647633788707));
#113106=CARTESIAN_POINT('Ctrl Pts',(-4.00285639763014,2.28101755500765,
-6.34255797109834));
#113107=CARTESIAN_POINT('Ctrl Pts',(-3.97740897208463,2.28571428597299,
-6.35847606489208));
#113108=CARTESIAN_POINT('Ctrl Pts',(-3.84893570007535,2.30942609046359,
-6.43883977728116));
#113109=CARTESIAN_POINT('Ctrl Pts',(-3.71758487779749,2.33338322658657,
-6.51558130515849));
#113110=CARTESIAN_POINT('Ctrl Pts',(-3.58367559790876,2.35752249352444,
-6.58841932518766));
#113111=CARTESIAN_POINT('Ctrl Pts',(-3.57637069016739,2.35883931875173,
-6.59239272431891));
#113112=CARTESIAN_POINT('Ctrl Pts',(-3.56905817816386,2.36015668503395,
-6.59635451619828));
#113113=CARTESIAN_POINT('Ctrl Pts',(-3.56173811685735,2.36147458179854,
-6.60030465830847));
#113114=CARTESIAN_POINT('',(-4.51442564736556,2.36147458149274,-5.98915361657529));
#113115=CARTESIAN_POINT('Origin',(0.121402364642468,2.41070043805478,0.147915157977384));
#113116=CARTESIAN_POINT('Origin',(0.0878437654423592,2.55351790115179,0.167150433932087));
#113117=CARTESIAN_POINT('Ctrl Pts',(-3.908818839,2.492226207,-6.106032696));
#113118=CARTESIAN_POINT('Ctrl Pts',(-4.242798303,2.42647128,-5.892233444));
#113119=CARTESIAN_POINT('Ctrl Pts',(-4.551466941,2.361474582,-5.643283502));
#113120=CARTESIAN_POINT('Ctrl Pts',(-4.55454012844867,2.36082745750497,
-5.64080488984796));
#113121=CARTESIAN_POINT('Ctrl Pts',(-4.55761331589734,2.36018033300993,
-5.63832627769592));
#113122=CARTESIAN_POINT('Ctrl Pts',(-3.834275513,2.492226207,-6.445799508));
#113123=CARTESIAN_POINT('Ctrl Pts',(-4.186839079,2.42647128,-6.236077526));
#113124=CARTESIAN_POINT('Ctrl Pts',(-4.51442565,2.361474582,-5.989153617));
#113125=CARTESIAN_POINT('Ctrl Pts',(-4.51768718944525,2.36082745750497,
-5.98669517657394));
#113126=CARTESIAN_POINT('Ctrl Pts',(-4.52094872889051,2.36018033300993,
-5.98423673614789));
#113127=CARTESIAN_POINT('',(-4.53294628858464,2.36147458056998,-5.81621856488957));
#113128=CARTESIAN_POINT('Ctrl Pts',(-4.54533470543984,2.36016764195642,
-5.64822932251851));
#113129=CARTESIAN_POINT('Ctrl Pts',(-4.54840082321992,2.36082111197821,
-5.64575641225926));
#113130=CARTESIAN_POINT('Ctrl Pts',(-4.551466941,2.361474582,-5.643283502));
#113131=CARTESIAN_POINT('Ctrl Pts',(-4.85841996200001,2.426894312,-5.395717254));
#113132=CARTESIAN_POINT('Ctrl Pts',(-5.136709949,2.492218586,-5.11631810000001));
#113133=CARTESIAN_POINT('Ctrl Pts',(-4.89116456977673,2.36016764195642,
-5.68564645093098));
#113134=CARTESIAN_POINT('Ctrl Pts',(-4.89425081288837,2.36082111197821,
-5.68298562196549));
#113135=CARTESIAN_POINT('Ctrl Pts',(-4.897337056,2.361474582,-5.68032479300001));
#113136=CARTESIAN_POINT('Ctrl Pts',(-5.20630485,2.426894312,-5.41394576));
#113137=CARTESIAN_POINT('Ctrl Pts',(-5.484557207,2.492218586,-5.11562628));
#113138=CARTESIAN_POINT('',(-4.89733704140428,2.36147458096338,-5.68032477704211));
#113139=CARTESIAN_POINT('',(-5.31049850288104,2.45202942688488,-5.2960934406446));
#113140=CARTESIAN_POINT('Origin',(0.131937943596592,2.41071410073285,0.140939548902802));
#113141=CARTESIAN_POINT('Ctrl Pts',(-5.13339538944625,2.49144077639895,
-5.11964373170493));
#113142=CARTESIAN_POINT('Ctrl Pts',(-5.16284109109888,2.48454521322505,
-5.14903758175326));
#113143=CARTESIAN_POINT('Ctrl Pts',(-5.19233960943423,2.47781843926765,
-5.17845385126795));
#113144=CARTESIAN_POINT('Ctrl Pts',(-5.25136513497413,2.46469208324408,
-5.23725988734003));
#113145=CARTESIAN_POINT('Ctrl Pts',(-5.28092578911374,2.45828502525069,
-5.26668317184299));
#113146=CARTESIAN_POINT('Ctrl Pts',(-5.31049849743009,2.45202942672717,
-5.296093437831));
#113147=CARTESIAN_POINT('',(-4.72440200654202,2.36147458031212,-5.66180414078946));
#113148=CARTESIAN_POINT('Origin',(-9.68843061333047E-13,2.45311202899956,
-9.64072571774111E-13));
#113149=CARTESIAN_POINT('',(-5.31525764273741,2.27159573079945,-5.29131705571896));
#113150=CARTESIAN_POINT('Ctrl Pts',(-5.3152576362519,2.2715957331383,-5.29131706170207));
#113151=CARTESIAN_POINT('Ctrl Pts',(-5.29405320487535,2.27631121120431,
-5.31261743299678));
#113152=CARTESIAN_POINT('Ctrl Pts',(-5.27273431832996,2.28101755501361,
-5.3337766881094));
#113153=CARTESIAN_POINT('Ctrl Pts',(-5.25130375898295,2.28571428600374,
-5.35479307001672));
#113154=CARTESIAN_POINT('Ctrl Pts',(-5.1431096261441,2.30942616017083,-5.46089619160282));
#113155=CARTESIAN_POINT('Ctrl Pts',(-5.03132653530554,2.3333833670886,-5.56408038258613));
#113156=CARTESIAN_POINT('Ctrl Pts',(-4.91620564381651,2.35752270584896,
-5.66400230049066));
#113157=CARTESIAN_POINT('Ctrl Pts',(-4.90992602055992,2.35883946035909,
-5.6694528489654));
#113158=CARTESIAN_POINT('Ctrl Pts',(-4.903636476675,2.36015675586587,-5.6748936972916));
#113159=CARTESIAN_POINT('Ctrl Pts',(-4.89733705668865,2.36147458179854,
-5.68032479214033));
#113160=CARTESIAN_POINT('',(-5.69637187435096,2.36147458149277,-4.87866246511143));
#113161=CARTESIAN_POINT('Origin',(0.150361561842405,2.41070048208448,0.118359186090153));
#113162=CARTESIAN_POINT('Origin',(0.1217224472246,2.55351790750067,0.144358771677074));
#113163=CARTESIAN_POINT('Ctrl Pts',(-5.130049363,2.492226207,-5.122996538));
#113164=CARTESIAN_POINT('Ctrl Pts',(-5.410260054,2.42647128,-4.842400082));
#113165=CARTESIAN_POINT('Ctrl Pts',(-5.658195312,2.361474582,-4.532915818));
#113166=CARTESIAN_POINT('Ctrl Pts',(-5.66066382168697,2.36082745750497,
-4.5298345099609));
#113167=CARTESIAN_POINT('Ctrl Pts',(-5.66313233137395,2.36018033300993,
-4.52675320192181));
#113168=CARTESIAN_POINT('Ctrl Pts',(-5.13028864,2.492226207,-5.47084440199999));
#113169=CARTESIAN_POINT('Ctrl Pts',(-5.429525439,2.42647128,-5.190234859));
#113170=CARTESIAN_POINT('Ctrl Pts',(-5.696371877,2.361474582,-4.878662465));
#113171=CARTESIAN_POINT('Ctrl Pts',(-5.69902867144889,2.36082745750497,
-4.8755603669806));
#113172=CARTESIAN_POINT('Ctrl Pts',(-5.70168546589777,2.36018033300993,
-4.87245826896118));
#113173=CARTESIAN_POINT('',(-5.67728358890492,2.36147458056998,-4.70578914825017));
#113174=CARTESIAN_POINT('Ctrl Pts',(-5.65326964992618,2.36016764195642,
-4.53906425736617));
#113175=CARTESIAN_POINT('Ctrl Pts',(-5.6557324809631,2.36082111197821,-4.53599003768308));
#113176=CARTESIAN_POINT('Ctrl Pts',(-5.658195312,2.361474582,-4.532915818));
#113177=CARTESIAN_POINT('Ctrl Pts',(-5.904752516,2.426894312,-4.225151705));
#113178=CARTESIAN_POINT('Ctrl Pts',(-6.116473679,2.492218586,-3.892460627));
#113179=CARTESIAN_POINT('Ctrl Pts',(-5.9990577812363,2.36016764195642,-4.50126339560797));
#113180=CARTESIAN_POINT('Ctrl Pts',(-6.00149987011815,2.36082111197821,
-4.49800132430398));
#113181=CARTESIAN_POINT('Ctrl Pts',(-6.003941959,2.361474582,-4.494739253));
#113182=CARTESIAN_POINT('Ctrl Pts',(-6.248422639,2.426894312,-4.168169071));
#113183=CARTESIAN_POINT('Ctrl Pts',(-6.456039741,2.492218586,-3.817008103));
#113184=CARTESIAN_POINT('',(-6.00394194129903,2.36147458096338,-4.49473924056304));
#113185=CARTESIAN_POINT('',(-6.32484553738381,2.45202942687081,-4.0306735180325));
#113186=CARTESIAN_POINT('Origin',(0.159151262774024,2.41071408942526,0.109281780000698));
#113187=CARTESIAN_POINT('Ctrl Pts',(-6.11395152485902,2.49144077640977,
-3.89642103948569));
#113188=CARTESIAN_POINT('Ctrl Pts',(-6.14902761125584,2.48454521320101,
-3.91879772233175));
#113189=CARTESIAN_POINT('Ctrl Pts',(-6.18416009891479,2.47781843925053,
-3.94118494631363));
#113190=CARTESIAN_POINT('Ctrl Pts',(-6.25444719952214,2.46469208329045,
-3.98592738649413));
#113191=CARTESIAN_POINT('Ctrl Pts',(-6.28964187791987,2.45828502538417,
-4.00830810378044));
#113192=CARTESIAN_POINT('Ctrl Pts',(-6.3248455314697,2.45202942670608,-4.03067351650012));
#113193=CARTESIAN_POINT('',(-5.83106864191144,2.36147458031212,-4.51382752721755));
#113194=CARTESIAN_POINT('Origin',(1.18308141061618E-12,2.45311202899989,
7.16874476447416E-13));
#113195=CARTESIAN_POINT('',(-6.32846662960937,2.27159573078434,-4.02498572816645));
#113196=CARTESIAN_POINT('Ctrl Pts',(-6.32846662458287,2.27159573312165,
-4.02498573540134));
#113197=CARTESIAN_POINT('Ctrl Pts',(-6.31233689126107,2.27631121119474,
-4.05034644181493));
#113198=CARTESIAN_POINT('Ctrl Pts',(-6.29606504286073,2.28101755500958,
-4.0755939357117));
#113199=CARTESIAN_POINT('Ctrl Pts',(-6.27965341894199,2.2857142860166,-4.10072590308884));
#113200=CARTESIAN_POINT('Ctrl Pts',(-6.19679771580215,2.30942619544187,
-4.22760712186647));
#113201=CARTESIAN_POINT('Ctrl Pts',(-6.10980946753997,2.33338343821218,
-4.35240916577372));
#113202=CARTESIAN_POINT('Ctrl Pts',(-6.01886015123036,2.35752281333228,
-4.47474272741705));
#113203=CARTESIAN_POINT('Ctrl Pts',(-6.01389918326844,2.35883953204388,
-4.48141559648969));
#113204=CARTESIAN_POINT('Ctrl Pts',(-6.00892644201457,2.36015679172259,
-4.48808112523777));
#113205=CARTESIAN_POINT('Ctrl Pts',(-6.00394195948775,2.36147458179854,
-4.49473925201239));
#113206=CARTESIAN_POINT('',(-6.6119620824281,2.36147458149273,-3.54005047773608));
#113207=CARTESIAN_POINT('Origin',(0.172289535167827,2.41070046788128,0.0832684843953935));
#113208=CARTESIAN_POINT('Origin',(0.149909449784781,2.55351788003384,0.11481695861501));
#113209=CARTESIAN_POINT('Ctrl Pts',(-6.111404481,2.492226207,-3.900414756));
#113210=CARTESIAN_POINT('Ctrl Pts',(-6.324744057,2.42647128,-3.566141474));
#113211=CARTESIAN_POINT('Ctrl Pts',(-6.50035275900001,2.361474582,-3.210594028));
#113212=CARTESIAN_POINT('Ctrl Pts',(-6.50210116616686,2.36082745750497,
-3.20705410261097));
#113213=CARTESIAN_POINT('Ctrl Pts',(-6.50384957333372,2.36018033300993,
-3.20351417722194));
#113214=CARTESIAN_POINT('Ctrl Pts',(-6.18641517199999,2.492226207,-4.240078693));
#113215=CARTESIAN_POINT('Ctrl Pts',(-6.418333224,2.42647128,-3.901702578));
#113216=CARTESIAN_POINT('Ctrl Pts',(-6.611962085,2.361474582,-3.540050477));
#113217=CARTESIAN_POINT('Ctrl Pts',(-6.61388990568557,2.36082745750497,
-3.53644977203438));
#113218=CARTESIAN_POINT('Ctrl Pts',(-6.61581772637116,2.36018033300993,
-3.53284906706876));
#113219=CARTESIAN_POINT('',(-6.55615741798682,2.36147458056998,-3.37532226029513));
#113220=CARTESIAN_POINT('Ctrl Pts',(-6.49686398890001,2.36016764195642,
-3.21765759201994));
#113221=CARTESIAN_POINT('Ctrl Pts',(-6.49860837395001,2.36082111197821,
-3.21412581000997));
#113222=CARTESIAN_POINT('Ctrl Pts',(-6.50035275900001,2.361474582,-3.210594028));
#113223=CARTESIAN_POINT('Ctrl Pts',(-6.674985405,2.426894312,-2.857022758));
#113224=CARTESIAN_POINT('Ctrl Pts',(-6.81023789800001,2.492218586,-2.486596021));
#113225=CARTESIAN_POINT('Ctrl Pts',(-6.82644171740222,2.36016764195642,
-3.10640626662274));
#113226=CARTESIAN_POINT('Ctrl Pts',(-6.82812546270111,2.36082111197821,
-3.10269548381137));
#113227=CARTESIAN_POINT('Ctrl Pts',(-6.829809208,2.361474582,-3.098984701));
#113228=CARTESIAN_POINT('Ctrl Pts',(-6.99837113000001,2.426894312,-2.727493429));
#113229=CARTESIAN_POINT('Ctrl Pts',(-7.125645032,2.492218586,-2.33991087));
#113230=CARTESIAN_POINT('',(-6.82980918807998,2.36147458096342,-3.09898469261055));
#113231=CARTESIAN_POINT('',(-7.04344982391374,2.45202942682679,-2.5767837820567));
#113232=CARTESIAN_POINT('Origin',(0.178922741658617,2.41071411444908,0.0725140132615187));
#113233=CARTESIAN_POINT('Ctrl Pts',(-6.80862608234284,2.49144077638204,
-2.4910060298125));
#113234=CARTESIAN_POINT('Ctrl Pts',(-6.84769243472193,2.48454521316273,
-2.50531923665124));
#113235=CARTESIAN_POINT('Ctrl Pts',(-6.88681613542936,2.47781843924689,
-2.51963061350475));
#113236=CARTESIAN_POINT('Ctrl Pts',(-6.96507828507022,2.46469207983398,
-2.54821735912881));
#113237=CARTESIAN_POINT('Ctrl Pts',(-7.00426134831749,2.45828501820032,
-2.56250902116586));
#113238=CARTESIAN_POINT('Ctrl Pts',(-7.0434498179514,2.45202942663179,-2.57678378194847));
#113239=CARTESIAN_POINT('',(-6.66508098798106,2.36147458031212,-3.15478935503292));
#113240=CARTESIAN_POINT('Origin',(1.07292646989166E-12,2.45311202900022,
3.62990887348147E-13));
#113241=CARTESIAN_POINT('',(-7.04576355034384,2.27159573077844,-2.57045054130644));
#113242=CARTESIAN_POINT('Ctrl Pts',(-7.04576354714259,2.27159573310333,
-2.57045054939503));
#113243=CARTESIAN_POINT('Ctrl Pts',(-7.03546272052735,2.27631121119429,
-2.59868575241402));
#113244=CARTESIAN_POINT('Ctrl Pts',(-7.02499876399313,2.28101755501505,
-2.62684094026218));
#113245=CARTESIAN_POINT('Ctrl Pts',(-7.01437346494182,2.2857142860237,-2.65491335014355));
#113246=CARTESIAN_POINT('Ctrl Pts',(-6.96073054894625,2.30942621516319,
-2.7966398013827));
#113247=CARTESIAN_POINT('Ctrl Pts',(-6.90260473575005,2.33338347798104,
-2.93722406043176));
#113248=CARTESIAN_POINT('Ctrl Pts',(-6.84007980371666,2.35752287343183,
-3.07624905883119));
#113249=CARTESIAN_POINT('Ctrl Pts',(-6.83666934148838,2.35883957212659,
-3.08383226588809));
#113250=CARTESIAN_POINT('Ctrl Pts',(-6.83324580366523,2.36015681177196,
-3.09141083528376));
#113251=CARTESIAN_POINT('Ctrl Pts',(-6.82980920826404,2.36147458179854,
-3.09898469993063));
#113252=CARTESIAN_POINT('',(-7.2183842936436,2.36147458149276,-2.0359096652279));
#113253=CARTESIAN_POINT('Origin',(0.186162053929598,2.41070043126948,0.04428467012911));
#113254=CARTESIAN_POINT('Origin',(0.171087174909335,2.55351792627012,0.0799066088981509));
#113255=CARTESIAN_POINT('Ctrl Pts',(-6.806997118,2.492226207,-2.495453915));
#113256=CARTESIAN_POINT('Ctrl Pts',(-6.943490059,2.42647128,-2.123134053));
#113257=CARTESIAN_POINT('Ctrl Pts',(-7.038560935,2.361474582,-1.73814843));
#113258=CARTESIAN_POINT('Ctrl Pts',(-7.03950748604824,2.36082745750497,
-1.73431541025369));
#113259=CARTESIAN_POINT('Ctrl Pts',(-7.04045403709647,2.36018033300993,
-1.73048239050737));
#113260=CARTESIAN_POINT('Ctrl Pts',(-6.953271806,2.492226207,-2.811051617));
#113261=CARTESIAN_POINT('Ctrl Pts',(-7.10702688,2.42647128,-2.430731022));
#113262=CARTESIAN_POINT('Ctrl Pts',(-7.218384296,2.361474582,-2.035909664));
#113263=CARTESIAN_POINT('Ctrl Pts',(-7.2194930001929,2.36082745750497,-2.03197871704752));
#113264=CARTESIAN_POINT('Ctrl Pts',(-7.2206017043858,2.36018033300993,-2.02804777009504));
#113265=CARTESIAN_POINT('',(-7.12847261325636,2.36147458056998,-1.8870290554756));
#113266=CARTESIAN_POINT('Ctrl Pts',(-7.03667218785752,2.36016764195642,
-1.7457968342631));
#113267=CARTESIAN_POINT('Ctrl Pts',(-7.03761656142876,2.36082111197821,
-1.74197263213155));
#113268=CARTESIAN_POINT('Ctrl Pts',(-7.038560935,2.361474582,-1.73814843));
#113269=CARTESIAN_POINT('Ctrl Pts',(-7.133103396,2.426894312,-1.355302603));
#113270=CARTESIAN_POINT('Ctrl Pts',(-7.185562962,2.492218586,-0.964460949));
#113271=CARTESIAN_POINT('Ctrl Pts',(-7.3346288266832,2.36016764195642,-1.56629703347739));
#113272=CARTESIAN_POINT('Ctrl Pts',(-7.33547549834161,2.36082111197821,
-1.56231105123869));
#113273=CARTESIAN_POINT('Ctrl Pts',(-7.33632217,2.361474582,-1.558325069));
#113274=CARTESIAN_POINT('Ctrl Pts',(-7.421083566,2.426894312,-1.159283226));
#113275=CARTESIAN_POINT('Ctrl Pts',(-7.462063081,2.492218586,-0.753402005000001));
#113276=CARTESIAN_POINT('',(-7.33632214870979,2.36147458096336,-1.5583250651542));
#113277=CARTESIAN_POINT('',(-7.43271022552165,2.45202942683029,-1.00240649998123));
#113278=CARTESIAN_POINT('Origin',(0.190327760252029,2.41071410057973,0.0323555341147232));
#113279=CARTESIAN_POINT('Ctrl Pts',(-7.18493685111934,2.49144077631594,
-0.969114347424825));
#113280=CARTESIAN_POINT('Ctrl Pts',(-7.22616677029348,2.48454521311534,
-0.97469480841737));
#113281=CARTESIAN_POINT('Ctrl Pts',(-7.26745230369469,2.47781843920833,
-0.980261154015143));
#113282=CARTESIAN_POINT('Ctrl Pts',(-7.35003003316461,2.46469207982352,
-0.991355508541588));
#113283=CARTESIAN_POINT('Ctrl Pts',(-7.39136930313058,2.45828501819801,
-0.996889839059943));
#113284=CARTESIAN_POINT('Ctrl Pts',(-7.43271021980434,2.45202942663669,
-1.00240650126442));
#113285=CARTESIAN_POINT('',(-7.18744155484115,2.36147458031212,-1.64823673929096));
#113286=CARTESIAN_POINT('Origin',(-1.77548947766226E-12,2.45311202899944,
-2.20662247155112E-13));
#113287=CARTESIAN_POINT('',(-7.43360839853097,2.27159573080751,-0.99572394410361));
#113288=CARTESIAN_POINT('Ctrl Pts',(-7.43360839709804,2.27159573313597,
-0.995723952718445));
#113289=CARTESIAN_POINT('Ctrl Pts',(-7.42961813203507,2.27631121121225,
-1.02551340564437));
#113290=CARTESIAN_POINT('Ctrl Pts',(-7.42545135009482,2.28101755502214,
-1.05525978226996));
#113291=CARTESIAN_POINT('Ctrl Pts',(-7.42110920294122,2.28571428598379,
-1.0849599999488));
#113292=CARTESIAN_POINT('Ctrl Pts',(-7.39918750952311,2.30942612443413,
-1.2349040331654));
#113293=CARTESIAN_POINT('Ctrl Pts',(-7.37264222487351,2.33338329510612,
-1.3846962719971));
#113294=CARTESIAN_POINT('Ctrl Pts',(-7.34146551075498,2.35752259707394,
-1.53391139070376));
#113295=CARTESIAN_POINT('Ctrl Pts',(-7.3397648315689,2.35883938781293,-1.54205102484443));
#113296=CARTESIAN_POINT('Ctrl Pts',(-7.33805038360176,2.36015671957836,
-1.55018894037855));
#113297=CARTESIAN_POINT('Ctrl Pts',(-7.33632217002799,2.36147458179854,
-1.55832506789888));
#113298=CARTESIAN_POINT('',(-7.48728287696558,2.36147458149276,-0.436571979715356));
#113299=CARTESIAN_POINT('Origin',(0.191329551311815,2.410700463604,0.00322996651999273));
#113300=CARTESIAN_POINT('Origin',(0.184264765178604,2.55351789729557,0.0412597353890298));
#113301=CARTESIAN_POINT('Ctrl Pts',(-7.184302134,2.492226207,-0.973808422));
#113302=CARTESIAN_POINT('Ctrl Pts',(-7.23756618199999,2.42647128,-0.580851245));
#113303=CARTESIAN_POINT('Ctrl Pts',(-7.247653825,2.361474582,-0.184428943));
#113304=CARTESIAN_POINT('Ctrl Pts',(-7.24775426026954,2.36082745750497,
-0.180482056621221));
#113305=CARTESIAN_POINT('Ctrl Pts',(-7.24785469553907,2.36018033300993,
-0.176535170242441));
#113306=CARTESIAN_POINT('Ctrl Pts',(-7.395001179,2.492226207,-1.250582891));
#113307=CARTESIAN_POINT('Ctrl Pts',(-7.463403859,2.42647128,-0.846101184));
#113308=CARTESIAN_POINT('Ctrl Pts',(-7.487282879,2.361474582,-0.436571978));
#113309=CARTESIAN_POINT('Ctrl Pts',(-7.48752062490456,2.36082745750497,
-0.432494595782302));
#113310=CARTESIAN_POINT('Ctrl Pts',(-7.48775837080912,2.36018033300993,
-0.428417213564603));
#113311=CARTESIAN_POINT('',(-7.36746835163083,2.36147458056998,-0.310500469259762));
#113312=CARTESIAN_POINT('Ctrl Pts',(-7.24745341654421,2.36016764195642,
-0.192304556630875));
#113313=CARTESIAN_POINT('Ctrl Pts',(-7.2475536207721,2.36082111197821,-0.188366749815437));
#113314=CARTESIAN_POINT('Ctrl Pts',(-7.247653825,2.361474582,-0.184428943));
#113315=CARTESIAN_POINT('Ctrl Pts',(-7.25768540000001,2.426894312,0.209789996));
#113316=CARTESIAN_POINT('Ctrl Pts',(-7.224899088,2.492218586,0.602771245));
#113317=CARTESIAN_POINT('Ctrl Pts',(-7.49985684282223,2.36016764195642,
0.0470505078652194));
#113318=CARTESIAN_POINT('Ctrl Pts',(-7.49982685141112,2.36082111197821,
0.0511253094326098));
#113319=CARTESIAN_POINT('Ctrl Pts',(-7.49979686,2.361474582,0.055200111));
#113320=CARTESIAN_POINT('Ctrl Pts',(-7.49679438100001,2.426894312,0.463133772));
#113321=CARTESIAN_POINT('Ctrl Pts',(-7.449563353,2.492218586,0.868335101));
#113322=CARTESIAN_POINT('',(-7.49979683838437,2.3614745809634,0.0552001102070129));
#113323=CARTESIAN_POINT('',(-7.47442535691804,2.45202942686423,0.61884219623295));
#113324=CARTESIAN_POINT('Origin',(0.192833561135066,2.41071405963099,-0.0093157574649749));
#113325=CARTESIAN_POINT('Ctrl Pts',(-7.22528795810139,2.49144077637022,
0.598092045178347));
#113326=CARTESIAN_POINT('Ctrl Pts',(-7.26675357866323,2.48454521316813,
0.601505266194621));
#113327=CARTESIAN_POINT('Ctrl Pts',(-7.30827047909649,2.47781843922539,
0.604944228024006));
#113328=CARTESIAN_POINT('Ctrl Pts',(-7.3913025451355,2.46469207985685,0.611861024276025));
#113329=CARTESIAN_POINT('Ctrl Pts',(-7.43286504331232,2.45828501823807,
0.615342804424006));
#113330=CARTESIAN_POINT('Ctrl Pts',(-7.47442535151781,2.4520294266883,0.618842193790386));
#113331=CARTESIAN_POINT('',(-7.37372534259178,2.36147458031212,-0.0646144055263606));
#113332=CARTESIAN_POINT('Origin',(-3.64291929955129E-14,2.45311202899967,
-8.74747865288461E-14));
#113333=CARTESIAN_POINT('',(-7.47386597965565,2.27159573081918,0.625561598277514));
#113334=CARTESIAN_POINT('Ctrl Pts',(-7.47386598001059,2.27159573315804,
0.625561589457456));
#113335=CARTESIAN_POINT('Ctrl Pts',(-7.47637285672591,2.27631121121701,
0.595610808312338));
#113336=CARTESIAN_POINT('Ctrl Pts',(-7.47869808334634,2.28101755501974,
0.565664150456018));
#113337=CARTESIAN_POINT('Ctrl Pts',(-7.48084212200374,2.28571428600819,
0.53572487394781));
#113338=CARTESIAN_POINT('Ctrl Pts',(-7.49166650280563,2.30942617277422,
0.384573624658953));
#113339=CARTESIAN_POINT('Ctrl Pts',(-7.49794273879163,2.33338339250487,
0.232576683279268));
#113340=CARTESIAN_POINT('Ctrl Pts',(-7.49957174307246,2.35752274425865,
0.0801477478569495));
#113341=CARTESIAN_POINT('Ctrl Pts',(-7.49966060121233,2.358839485976,0.0718331278021478));
#113342=CARTESIAN_POINT('Ctrl Pts',(-7.49973564405799,2.36015676867945,
0.0635172263906127));
#113343=CARTESIAN_POINT('Ctrl Pts',(-7.49979685979061,2.36147458179854,
0.0552001120813991));
#113344=CARTESIAN_POINT('',(-7.40608443439015,2.36147458149275,1.1831793268725));
#113345=CARTESIAN_POINT('Origin',(0.187550563654373,2.41070042117061,-0.0379757253984499));
#113346=CARTESIAN_POINT('Origin',(0.188826312576141,2.55351788305839,0.000683636489218209));
#113347=CARTESIAN_POINT('Ctrl Pts',(-7.225677168,2.492226207,0.59337127));
#113348=CARTESIAN_POINT('Ctrl Pts',(-7.193221754,2.42647128,0.988591523));
#113349=CARTESIAN_POINT('Ctrl Pts',(-7.117854477,2.361474582,1.377914237));
#113350=CARTESIAN_POINT('Ctrl Pts',(-7.117104100249,2.36082745750497,1.38179043798336));
#113351=CARTESIAN_POINT('Ctrl Pts',(-7.11635372349801,2.36018033300993,
1.38566663896671));
#113352=CARTESIAN_POINT('Ctrl Pts',(-7.490948515,2.492226207,0.368361701));
#113353=CARTESIAN_POINT('Ctrl Pts',(-7.470800368,2.42647128,0.778091405));
#113354=CARTESIAN_POINT('Ctrl Pts',(-7.406084436,2.361474582,1.183179329));
#113355=CARTESIAN_POINT('Ctrl Pts',(-7.4054401068863,2.36082745750497,1.18721249262722));
#113356=CARTESIAN_POINT('Ctrl Pts',(-7.40479577777259,2.36018033300993,
1.19124565625443));
#113357=CARTESIAN_POINT('',(-7.26196945802254,2.36147458056998,1.28054677436567));
#113358=CARTESIAN_POINT('Ctrl Pts',(-7.11935177812158,2.36016764195642,
1.37017966895271));
#113359=CARTESIAN_POINT('Ctrl Pts',(-7.1186031275608,2.36082111197821,1.37404695297636));
#113360=CARTESIAN_POINT('Ctrl Pts',(-7.117854477,2.361474582,1.377914237));
#113361=CARTESIAN_POINT('Ctrl Pts',(-7.04290610000001,2.426894312,1.765073048));
#113362=CARTESIAN_POINT('Ctrl Pts',(-6.926406962,2.492218586,2.141818525));
#113363=CARTESIAN_POINT('Ctrl Pts',(-7.31439988922279,2.36016764195642,
1.65819802060071));
#113364=CARTESIAN_POINT('Ctrl Pts',(-7.31349463711139,2.36082111197821,
1.66217110830036));
#113365=CARTESIAN_POINT('Ctrl Pts',(-7.312589385,2.361474582,1.666144196));
#113366=CARTESIAN_POINT('Ctrl Pts',(-7.22196342400001,2.426894312,2.06389515));
#113367=CARTESIAN_POINT('Ctrl Pts',(-7.088730323,2.492218586,2.449469822));
#113368=CARTESIAN_POINT('',(-7.31258936405879,2.36147458096341,1.66614419057183));
#113369=CARTESIAN_POINT('',(-7.16664466774274,2.45202942698552,2.21115451601479));
#113370=CARTESIAN_POINT('Origin',(0.186322575069613,2.41071418679769,-0.050551483569205));
#113371=CARTESIAN_POINT('Ctrl Pts',(-6.92779263031738,2.49144077640028,
2.13733231839907));
#113372=CARTESIAN_POINT('Ctrl Pts',(-6.96755506628153,2.48454521316664,
2.14957962298675));
#113373=CARTESIAN_POINT('Ctrl Pts',(-7.00736204944851,2.47781843924576,
2.16186309014197));
#113374=CARTESIAN_POINT('Ctrl Pts',(-7.08696596546045,2.46469207986141,
2.18646761539597));
#113375=CARTESIAN_POINT('Ctrl Pts',(-7.12680827580072,2.45828501824705,
2.19880270199693));
#113376=CARTESIAN_POINT('Ctrl Pts',(-7.16664466189622,2.45202942670426,
2.21115451533576));
#113377=CARTESIAN_POINT('',(-7.21522192883811,2.36147458031212,1.5220292267485));
#113378=CARTESIAN_POINT('Ctrl Pts',(-6.929187568,2.492226207,2.132805581));
#113379=CARTESIAN_POINT('Ctrl Pts',(-6.812530272,2.42647128,2.511808849));
#113380=CARTESIAN_POINT('Ctrl Pts',(-6.655232165,2.361474582,2.875827678));
#113381=CARTESIAN_POINT('Ctrl Pts',(-6.65366606301029,2.36082745750497,
2.87945194674207));
#113382=CARTESIAN_POINT('Ctrl Pts',(-6.65209996102059,2.36018033300993,
2.88307621548415));
#113383=CARTESIAN_POINT('Ctrl Pts',(-7.236627425,2.492226207,1.970082109));
#113384=CARTESIAN_POINT('Ctrl Pts',(-7.128870556,2.42647128,2.365901304));
#113385=CARTESIAN_POINT('Ctrl Pts',(-6.978585717,2.361474582,2.747606485));
#113386=CARTESIAN_POINT('Ctrl Pts',(-6.97708944098073,2.36082745750497,
2.75140684378909));
#113387=CARTESIAN_POINT('Ctrl Pts',(-6.97559316496146,2.36018033300993,
2.75520720257818));
#113388=CARTESIAN_POINT('',(-6.97858570553615,2.36147458149004,2.74760648257101));
#113389=CARTESIAN_POINT('Origin',(0.184554745902666,2.55351828260427,-0.0399231627928354));
#113390=CARTESIAN_POINT('',(-6.81690894434307,2.36147458056998,2.81171707339485));
#113391=CARTESIAN_POINT('Origin',(9.54097911787244E-14,2.45311202899978,
-1.24683249835833E-13));
#113392=CARTESIAN_POINT('',(-7.16465389442683,2.27159573166205,2.21759657512164));
#113393=CARTESIAN_POINT('Ctrl Pts',(-7.16465389665266,2.27159573308995,
2.21759656681736));
#113394=CARTESIAN_POINT('Ctrl Pts',(-7.17354069681518,2.27631121118133,
2.18888492264391));
#113395=CARTESIAN_POINT('Ctrl Pts',(-7.18224920728836,2.28101755500656,
2.16013825594367));
#113396=CARTESIAN_POINT('Ctrl Pts',(-7.19077917892545,2.28571428597853,
2.13135984807086));
#113397=CARTESIAN_POINT('Ctrl Pts',(-7.23384342168401,2.30942610672504,
1.9860697577258));
#113398=CARTESIAN_POINT('Ctrl Pts',(-7.27264767649734,2.33338325938208,
1.83897603880896));
#113399=CARTESIAN_POINT('Ctrl Pts',(-7.30700624033689,2.35752254308601,
1.69046141520244));
#113400=CARTESIAN_POINT('Ctrl Pts',(-7.30888051535824,2.35883935180626,
1.68235987607438));
#113401=CARTESIAN_POINT('Ctrl Pts',(-7.31074157218808,2.36015670156782,
1.67425411523461));
#113402=CARTESIAN_POINT('Ctrl Pts',(-7.31258938456305,2.36147458179854,
1.6661441970111));
#113403=CARTESIAN_POINT('Origin',(0.17499824870831,2.41070077462701,-0.0774045721351185));
#113404=CARTESIAN_POINT('Ctrl Pts',(-6.65835716353885,2.36016764195642,
2.86859581532773));
#113405=CARTESIAN_POINT('Ctrl Pts',(-6.65679466426943,2.36082111197821,
2.87221174666387));
#113406=CARTESIAN_POINT('Ctrl Pts',(-6.655232165,2.361474582,2.875827678));
#113407=CARTESIAN_POINT('Ctrl Pts',(-6.49880834,2.426894312,3.237823246));
#113408=CARTESIAN_POINT('Ctrl Pts',(-6.304043745,2.492218586,3.580716752));
#113409=CARTESIAN_POINT('Ctrl Pts',(-6.78692972648235,2.36016764195642,
3.19181003665553));
#113410=CARTESIAN_POINT('Ctrl Pts',(-6.78519154224117,2.36082111197821,
3.19549563332777));
#113411=CARTESIAN_POINT('Ctrl Pts',(-6.783453358,2.361474582,3.19918123));
#113412=CARTESIAN_POINT('Ctrl Pts',(-6.609441483,2.426894312,3.568151085));
#113413=CARTESIAN_POINT('Ctrl Pts',(-6.396436141,2.492218586,3.916070057));
#113414=CARTESIAN_POINT('',(-6.78345333872078,2.36147458096338,3.19918122017551));
#113415=CARTESIAN_POINT('',(-6.71934275718553,2.36147458031212,3.03750446354416));
#113416=CARTESIAN_POINT('',(-6.52375963646868,2.45202942685875,3.70007571388178));
#113417=CARTESIAN_POINT('Origin',(0.17109954117571,2.41071407661823,-0.089423536925872));
#113418=CARTESIAN_POINT('Ctrl Pts',(-6.30636141922389,2.49144077637438,
3.57663330860409));
#113419=CARTESIAN_POINT('Ctrl Pts',(-6.34256142319105,2.48454521312223,
3.59714202627954));
#113420=CARTESIAN_POINT('Ctrl Pts',(-6.37879715856625,2.47781843924882,
3.61769563722942));
#113421=CARTESIAN_POINT('Ctrl Pts',(-6.45125073361651,2.46469207983837,
3.65883741112242));
#113422=CARTESIAN_POINT('Ctrl Pts',(-6.48750987377411,2.45828501822364,
3.67944902918302));
#113423=CARTESIAN_POINT('Ctrl Pts',(-6.52375963243751,2.45202942668014,
3.70007570940484));
#113424=CARTESIAN_POINT('Origin',(-1.38821246165044E-12,2.45311202899956,
8.14018991102117E-13));
#113425=CARTESIAN_POINT('',(-6.22477608441886,2.36147458149275,4.18355861340272));
#113426=CARTESIAN_POINT('Origin',(0.171661065249297,2.5535178799818,-0.0786655937107383));
#113427=CARTESIAN_POINT('',(-6.52043055591603,2.27159573079198,3.70593920125996));
#113428=CARTESIAN_POINT('Ctrl Pts',(-6.52043055998516,2.27159573312279,
3.70593919351544));
#113429=CARTESIAN_POINT('Ctrl Pts',(-6.53528174642073,2.2763112112019,3.67980921105351));
#113430=CARTESIAN_POINT('Ctrl Pts',(-6.54996634030221,2.28101755501622,
3.6536066978739));
#113431=CARTESIAN_POINT('Ctrl Pts',(-6.5644833929722,2.28571428599651,3.62733480496704));
#113432=CARTESIAN_POINT('Ctrl Pts',(-6.63777403314015,2.30942615217881,
3.49469880110261));
#113433=CARTESIAN_POINT('Ctrl Pts',(-6.70729199307885,2.33338335102282,
3.35938555588206));
#113434=CARTESIAN_POINT('Ctrl Pts',(-6.77277363651984,2.35752268157398,
3.2217289252915));
#113435=CARTESIAN_POINT('Ctrl Pts',(-6.77634555739711,2.35883944416923,
3.21421997214277));
#113436=CARTESIAN_POINT('Ctrl Pts',(-6.77990547750036,2.36015674776775,
3.20670405495281));
#113437=CARTESIAN_POINT('Ctrl Pts',(-6.78345335735591,2.36147458179854,
3.19918123089353));
#113438=CARTESIAN_POINT('Origin',(0.154270784383641,2.41070044892372,-0.113216334444677));
#113439=CARTESIAN_POINT('Ctrl Pts',(-6.308696859,2.492226207,3.572512274));
#113440=CARTESIAN_POINT('Ctrl Pts',(-6.113292446,2.42647128,3.917576786));
#113441=CARTESIAN_POINT('Ctrl Pts',(-5.881418593,2.361474582,4.239270613));
#113442=CARTESIAN_POINT('Ctrl Pts',(-5.87910999495346,2.36082745750497,
4.24247348271121));
#113443=CARTESIAN_POINT('Ctrl Pts',(-5.87680139690693,2.36018033300993,
4.24567635242242));
#113444=CARTESIAN_POINT('Ctrl Pts',(-6.643929679,2.492226207,3.479683667));
#113445=CARTESIAN_POINT('Ctrl Pts',(-6.453602679,2.42647128,3.843084288));
#113446=CARTESIAN_POINT('Ctrl Pts',(-6.224776085,2.361474582,4.183558616));
#113447=CARTESIAN_POINT('Ctrl Pts',(-6.22249782627842,2.36082745750497,
4.18694846939808));
#113448=CARTESIAN_POINT('Ctrl Pts',(-6.22021956755684,2.36018033300993,
4.19033832279615));
#113449=CARTESIAN_POINT('',(-6.05309734400731,2.36147458056997,4.21141460730296));
#113450=CARTESIAN_POINT('Ctrl Pts',(-5.88602516750172,2.36016764195642,
4.23287960957504));
#113451=CARTESIAN_POINT('Ctrl Pts',(-5.88372188025086,2.36082111197821,
4.23607511128752));
#113452=CARTESIAN_POINT('Ctrl Pts',(-5.881418593,2.361474582,4.239270613));
#113453=CARTESIAN_POINT('Ctrl Pts',(-5.650833524,2.426894312,4.559176427));
#113454=CARTESIAN_POINT('Ctrl Pts',(-5.386910449,2.492218586,4.852184643));
#113455=CARTESIAN_POINT('Ctrl Pts',(-5.9421102725929,2.36016764195642,4.57617656251187));
#113456=CARTESIAN_POINT('Ctrl Pts',(-5.93962043179645,2.36082111197821,
4.57940233375593));
#113457=CARTESIAN_POINT('Ctrl Pts',(-5.93713059100001,2.361474582,4.582628105));
#113458=CARTESIAN_POINT('Ctrl Pts',(-5.68786940500001,2.426894312,4.905564241));
#113459=CARTESIAN_POINT('Ctrl Pts',(-5.405051715,2.492218586,5.199559208));
#113460=CARTESIAN_POINT('',(-5.93713057428633,2.36147458096336,4.58262809126086));
#113461=CARTESIAN_POINT('',(-5.57583085666585,2.45202942684484,5.01598548058866));
#113462=CARTESIAN_POINT('Origin',(0.14787568222294,2.41071408521665,-0.124114020875486));
#113463=CARTESIAN_POINT('Ctrl Pts',(-5.39005175674965,2.4914407764098,4.84869489944713));
#113464=CARTESIAN_POINT('Ctrl Pts',(-5.42099665665192,2.48454521318188,
4.87650606538268));
#113465=CARTESIAN_POINT('Ctrl Pts',(-5.4519668020571,2.47781843928518,4.90436875641983));
#113466=CARTESIAN_POINT('Ctrl Pts',(-5.51388218768978,2.46469207987048,
4.96012403546337));
#113467=CARTESIAN_POINT('Ctrl Pts',(-5.54486272088388,2.4582850182284,4.98804840880374));
#113468=CARTESIAN_POINT('Ctrl Pts',(-5.57583085399527,2.45202942665872,
5.01598547540733));
#113469=CARTESIAN_POINT('',(-5.90927458573466,2.36147458031211,4.41094936739357));
#113470=CARTESIAN_POINT('Origin',(-1.13103970633688E-12,2.45311202899944,
1.05774763947686E-12));
#113471=CARTESIAN_POINT('',(-5.5713191313085,2.27159573083506,5.02099622960137));
#113472=CARTESIAN_POINT('Ctrl Pts',(-5.57131913694017,2.27159573319232,
5.02099622266133));
#113473=CARTESIAN_POINT('Ctrl Pts',(-5.5914402845158,2.27631121122797,4.99866971064512));
#113474=CARTESIAN_POINT('Ctrl Pts',(-5.61141432647901,2.28101755501943,
4.97623655128185));
#113475=CARTESIAN_POINT('Ctrl Pts',(-5.63123965890202,2.28571428598273,
4.95369961782458));
#113476=CARTESIAN_POINT('Ctrl Pts',(-5.731329636829,2.30942615505832,4.83991987603559));
#113477=CARTESIAN_POINT('Ctrl Pts',(-5.82831066571407,2.33338335700141,
4.72271447127471));
#113478=CARTESIAN_POINT('Ctrl Pts',(-5.92185350248422,2.35752269062246,
4.6023527781534));
#113479=CARTESIAN_POINT('Ctrl Pts',(-5.9269561050895,2.35883945020424,4.59578725255997));
#113480=CARTESIAN_POINT('Ctrl Pts',(-5.93204848460138,2.36015675078659,
4.58921234597057));
#113481=CARTESIAN_POINT('Ctrl Pts',(-5.93713059017888,2.36147458179854,
4.58262810573419));
#113482=CARTESIAN_POINT('',(-5.17990284201352,2.36147458149274,5.42389219232862));
#113483=CARTESIAN_POINT('Origin',(0.126325665247499,2.41070046202241,-0.143732892703099));
#113484=CARTESIAN_POINT('Origin',(0.150736867158598,2.55351783920603,-0.113728427993419));
#113485=CARTESIAN_POINT('Ctrl Pts',(-5.393218496,2.492226207,4.845172263));
#113486=CARTESIAN_POINT('Ctrl Pts',(-5.12820386,2.42647128,5.140163186));
#113487=CARTESIAN_POINT('Ctrl Pts',(-4.832596425,2.361474582,5.404489966));
#113488=CARTESIAN_POINT('Ctrl Pts',(-4.82965327837888,2.36082745750497,
5.40712167406049));
#113489=CARTESIAN_POINT('Ctrl Pts',(-4.82671013175777,2.36018033300993,
5.40975338212096));
#113490=CARTESIAN_POINT('Ctrl Pts',(-5.740569165,2.492226207,4.826579084));
#113491=CARTESIAN_POINT('Ctrl Pts',(-5.476571513,2.42647128,5.140568922));
#113492=CARTESIAN_POINT('Ctrl Pts',(-5.179902842,2.361474582,5.423892195));
#113493=CARTESIAN_POINT('Ctrl Pts',(-5.17694912942966,2.36082745750497,
5.42671303722142));
#113494=CARTESIAN_POINT('Ctrl Pts',(-5.17399541685932,2.36018033300993,
5.42953387944285));
#113495=CARTESIAN_POINT('',(-5.00624963993739,2.36147458056997,5.41419107454764));
#113496=CARTESIAN_POINT('Ctrl Pts',(-4.83846917719169,2.36016764195642,
5.39923865803316));
#113497=CARTESIAN_POINT('Ctrl Pts',(-4.83553280109584,2.36082111197821,
5.40186431201658));
#113498=CARTESIAN_POINT('Ctrl Pts',(-4.83259642500001,2.361474582,5.404489966));
#113499=CARTESIAN_POINT('Ctrl Pts',(-4.538632012,2.426894312,5.667347586));
#113500=CARTESIAN_POINT('Ctrl Pts',(-4.217891208,2.492218586,5.896769773));
#113501=CARTESIAN_POINT('Ctrl Pts',(-4.81944434632715,2.36016764195642,
5.74656615832854));
#113502=CARTESIAN_POINT('Ctrl Pts',(-4.81631927116357,2.36082111197821,
5.74918127066428));
#113503=CARTESIAN_POINT('Ctrl Pts',(-4.813194196,2.361474582,5.751796383));
#113504=CARTESIAN_POINT('Ctrl Pts',(-4.500338875,2.426894312,6.01359866500001));
#113505=CARTESIAN_POINT('Ctrl Pts',(-4.160933077,2.492218586,6.23992275));
#113506=CARTESIAN_POINT('',(-4.81319418262263,2.36147458096339,5.75179636599494));
#113507=CARTESIAN_POINT('',(-4.36718242293266,2.45202942683089,6.09735334139361));
#113508=CARTESIAN_POINT('Origin',(0.117737553260419,2.41071407554446,-0.153001151993558));
#113509=CARTESIAN_POINT('Ctrl Pts',(-4.2217092652745,2.49144077645184,5.89403690575462));
#113510=CARTESIAN_POINT('Ctrl Pts',(-4.24595211176852,2.48454521320699,
5.92785010093519));
#113511=CARTESIAN_POINT('Ctrl Pts',(-4.27020853744412,2.47781843925731,
5.96171904380918));
#113512=CARTESIAN_POINT('Ctrl Pts',(-4.31869063871647,2.46469207984206,
6.02948077314091));
#113513=CARTESIAN_POINT('Ctrl Pts',(-4.34294394942702,2.45828501820144,
6.06341218901115));
#113514=CARTESIAN_POINT('Ctrl Pts',(-4.36718242130856,2.45202942663775,
6.09735333570621));
#113515=CARTESIAN_POINT('',(-4.82289530257678,2.36147458031212,5.57814318135047));
#113516=CARTESIAN_POINT('Origin',(-3.28946939132102E-13,2.45311202899922,
5.1911600018606E-13));
#113517=CARTESIAN_POINT('',(-4.36169901639869,2.27159573075345,6.10127705382252));
#113518=CARTESIAN_POINT('Ctrl Pts',(-4.36169902333983,2.27159573307932,
6.10127704857741));
#113519=CARTESIAN_POINT('Ctrl Pts',(-4.38614929003948,2.27631121117809,
6.08379797009143));
#113520=CARTESIAN_POINT('Ctrl Pts',(-4.41047881627064,2.28101755500682,
6.06618311407453));
#113521=CARTESIAN_POINT('Ctrl Pts',(-4.434685417972,2.28571428599309,6.04843494196295));
#113522=CARTESIAN_POINT('Ctrl Pts',(-4.55689457609569,2.30942614485292,
5.95883173353127));
#113523=CARTESIAN_POINT('Ctrl Pts',(-4.67680388863052,2.33338333625891,
5.86521462189015));
#113524=CARTESIAN_POINT('Ctrl Pts',(-4.79403390338584,2.35752265926315,
5.76777590841553));
#113525=CARTESIAN_POINT('Ctrl Pts',(-4.80042865478654,2.35883942928929,
5.76246074786749));
#113526=CARTESIAN_POINT('Ctrl Pts',(-4.80681543861544,2.36015674032481,
5.75713422780452));
#113527=CARTESIAN_POINT('Ctrl Pts',(-4.81319419504025,2.36147458179854,
5.75179638354049));
#113528=CARTESIAN_POINT('',(-3.89282309958484,2.36147458149274,6.4106106013945));
#113529=CARTESIAN_POINT('Origin',(0.0924741257365813,2.41070046819418,-0.1675290846441));
#113530=CARTESIAN_POINT('Origin',(0.122764507635105,2.553517885663,-0.143473533098674));
#113531=CARTESIAN_POINT('Ctrl Pts',(-4.22555923,2.492226207,5.891277382));
#113532=CARTESIAN_POINT('Ctrl Pts',(-3.90332616,2.42647128,6.122401268));
#113533=CARTESIAN_POINT('Ctrl Pts',(-3.557807419,2.361474582,6.317001375));
#113534=CARTESIAN_POINT('Ctrl Pts',(-3.55436734207803,2.36082745750497,
6.31893886567032));
#113535=CARTESIAN_POINT('Ctrl Pts',(-3.55092726515605,2.36018033300993,
6.32087635634062));
#113536=CARTESIAN_POINT('Ctrl Pts',(-4.568786018,2.492226207,5.947789028));
#113537=CARTESIAN_POINT('Ctrl Pts',(-4.243461951,2.42647128,6.197686266));
#113538=CARTESIAN_POINT('Ctrl Pts',(-3.892823099,2.361474582,6.41061060400001));
#113539=CARTESIAN_POINT('Ctrl Pts',(-3.88933204488461,2.36082745750497,
6.41273053561112));
#113540=CARTESIAN_POINT('Ctrl Pts',(-3.88584099076922,2.36018033300993,
6.41485046722225));
#113541=CARTESIAN_POINT('',(-3.72531526656647,2.36147458056997,6.36380598507066));
#113542=CARTESIAN_POINT('Ctrl Pts',(-3.56467174548097,2.36016764195642,
6.31313530783206));
#113543=CARTESIAN_POINT('Ctrl Pts',(-3.56123958224049,2.36082111197821,
6.31506834141603));
#113544=CARTESIAN_POINT('Ctrl Pts',(-3.557807419,2.361474582,6.317001375));
#113545=CARTESIAN_POINT('Ctrl Pts',(-3.214209113,2.426894312,6.51051987));
#113546=CARTESIAN_POINT('Ctrl Pts',(-2.851648061,2.492218586,6.665628503));
#113547=CARTESIAN_POINT('Ctrl Pts',(-3.47142655900055,2.36016764195642,
6.64825270764319));
#113548=CARTESIAN_POINT('Ctrl Pts',(-3.46781237450027,2.36082111197821,
6.6501348813216));
#113549=CARTESIAN_POINT('Ctrl Pts',(-3.46419819,2.361474582,6.652017055));
#113550=CARTESIAN_POINT('Ctrl Pts',(-3.1023775,2.426894312,6.840443899));
#113551=CARTESIAN_POINT('Ctrl Pts',(-2.722253834,2.492218586,6.988514439));
#113552=CARTESIAN_POINT('',(-3.46419818055662,2.36147458096339,6.65201703555471));
#113553=CARTESIAN_POINT('',(-2.95432939283039,2.45202942682624,6.89361573653466));
#113554=CARTESIAN_POINT('Origin',(0.0820942584082386,2.41071412403309,-0.174734328481542));
#113555=CARTESIAN_POINT('Ctrl Pts',(-2.8559643401511,2.49144077638546,6.66378029826372));
#113556=CARTESIAN_POINT('Ctrl Pts',(-2.87237156518068,2.48454521313266,
6.70201445509764));
#113557=CARTESIAN_POINT('Ctrl Pts',(-2.88878006762336,2.47781843920517,
6.7403059752111));
#113558=CARTESIAN_POINT('Ctrl Pts',(-2.92156191563384,2.46469207979522,
6.81690569143143));
#113559=CARTESIAN_POINT('Ctrl Pts',(-2.9379539459407,2.45828501817635,6.85525755431668));
#113560=CARTESIAN_POINT('Ctrl Pts',(-2.95432939247112,2.45202942663078,
6.89361573063811));
#113561=CARTESIAN_POINT('',(-3.51100279528937,2.36147458031211,6.48450921998705));
#113562=CARTESIAN_POINT('Origin',(5.55111512312578E-13,2.45311202900067,
-1.28586377656781E-12));
#113563=CARTESIAN_POINT('',(-2.94813070274797,2.27159573080254,6.89626894453793));
#113564=CARTESIAN_POINT('Ctrl Pts',(-2.94813071078491,2.27159573316313,
6.89626894059832));
#113565=CARTESIAN_POINT('Ctrl Pts',(-2.97576682895059,2.27631121120737,
6.88445459749243));
#113566=CARTESIAN_POINT('Ctrl Pts',(-3.00331421772734,2.28101755500858,
6.87248169581864));
#113567=CARTESIAN_POINT('Ctrl Pts',(-3.03077021493258,2.28571428598784,
6.86035217002096));
#113568=CARTESIAN_POINT('Ctrl Pts',(-3.16938408801206,2.30942612020512,
6.79911525570395));
#113569=CARTESIAN_POINT('Ctrl Pts',(-3.3066147584816,2.33338328651352,6.73346389045273));
#113570=CARTESIAN_POINT('Ctrl Pts',(-3.44205030695843,2.35752258408356,
6.66350430934275));
#113571=CARTESIAN_POINT('Ctrl Pts',(-3.44943829583462,2.35883937914905,
6.65968802467572));
#113572=CARTESIAN_POINT('Ctrl Pts',(-3.45682094517355,2.36015671524464,
6.65585893279283));
#113573=CARTESIAN_POINT('Ctrl Pts',(-3.4641981889465,2.36147458179854,6.65201705532155));
#113574=CARTESIAN_POINT('',(-2.42371927611264,2.36147458149276,7.09757598358083));
#113575=CARTESIAN_POINT('Origin',(0.0542983013924922,2.4107004966354,-0.183491481210859));
#113576=CARTESIAN_POINT('Origin',(0.0890517491531923,2.55351788318359,-0.166509867032308));
#113577=CARTESIAN_POINT('Ctrl Pts',(-2.860317511,2.492226207,6.661912919));
#113578=CARTESIAN_POINT('Ctrl Pts',(-2.495933268,2.42647128,6.818362672));
#113579=CARTESIAN_POINT('Ctrl Pts',(-2.116659292,2.361474582,6.93413682));
#113580=CARTESIAN_POINT('Ctrl Pts',(-2.1128831389376,2.36082745750497,6.93528949835702));
#113581=CARTESIAN_POINT('Ctrl Pts',(-2.1091069858752,2.36018033300993,6.93644217671405));
#113582=CARTESIAN_POINT('Ctrl Pts',(-3.183371514,2.492226207,6.790886967));
#113583=CARTESIAN_POINT('Ctrl Pts',(-2.811932824,2.42647128,6.965006689));
#113584=CARTESIAN_POINT('Ctrl Pts',(-2.423719275,2.361474582,7.097575986));
#113585=CARTESIAN_POINT('Ctrl Pts',(-2.4198541171598,2.36082745750497,7.09889588134881));
#113586=CARTESIAN_POINT('Ctrl Pts',(-2.4159889593196,2.36018033300993,7.10021577669761));
#113587=CARTESIAN_POINT('',(-2.2701892918417,2.36147458056998,7.0158564003008));
#113588=CARTESIAN_POINT('Ctrl Pts',(-2.12419422451128,2.36016764195642,
6.93183676660004));
#113589=CARTESIAN_POINT('Ctrl Pts',(-2.12042675825564,2.36082111197821,
6.93298679330001));
#113590=CARTESIAN_POINT('Ctrl Pts',(-2.116659292,2.361474582,6.93413682));
#113591=CARTESIAN_POINT('Ctrl Pts',(-1.739493367,2.426894312,7.049267482));
#113592=CARTESIAN_POINT('Ctrl Pts',(-1.352065021,2.492218586,7.122809851));
#113593=CARTESIAN_POINT('Ctrl Pts',(-1.96108872313987,2.36016764195642,
7.23907434966039));
#113594=CARTESIAN_POINT('Ctrl Pts',(-1.95715442456993,2.36082111197821,
7.2401355763302));
#113595=CARTESIAN_POINT('Ctrl Pts',(-1.953220126,2.361474582,7.241196803));
#113596=CARTESIAN_POINT('Ctrl Pts',(-1.559352402,2.426894312,7.347437579));
#113597=CARTESIAN_POINT('Ctrl Pts',(-1.156285027,2.492218586,7.41033096));
#113598=CARTESIAN_POINT('',(-1.95322012100067,2.36147458096337,7.24119678195224));
#113599=CARTESIAN_POINT('',(-1.40333520372143,2.45202942685434,7.36754032174613));
#113600=CARTESIAN_POINT('Origin',(0.0426122198937216,2.41071409218959,-0.18829692376378));
#113601=CARTESIAN_POINT('Ctrl Pts',(-1.3566776972798,2.49144077638316,7.121932728778));
#113602=CARTESIAN_POINT('Ctrl Pts',(-1.36448211673127,2.48454521316821,
7.16280006073904));
#113603=CARTESIAN_POINT('Ctrl Pts',(-1.37227545238057,2.47781843928024,
7.20372368937314));
#113604=CARTESIAN_POINT('Ctrl Pts',(-1.38782420408007,2.46469207987779,
7.28557967538297));
#113605=CARTESIAN_POINT('Ctrl Pts',(-1.39558848094723,2.45828501824256,
7.32655869521264));
#113606=CARTESIAN_POINT('Ctrl Pts',(-1.40333520459521,2.45202942667326,
7.36754031585559));
#113607=CARTESIAN_POINT('',(-2.03493969893267,2.36147458031212,7.08766681439043));
#113608=CARTESIAN_POINT('Origin',(-8.35919874986324E-14,2.45311202900044,
5.48606299277665E-13));
#113609=CARTESIAN_POINT('',(-1.39671107471047,2.27159573078887,7.36879896398992));
#113610=CARTESIAN_POINT('Ctrl Pts',(-1.39671108335984,2.27159573313922,
7.36879896191029));
#113611=CARTESIAN_POINT('Ctrl Pts',(-1.42624081901485,2.27631121119733,
7.36320178012557));
#113612=CARTESIAN_POINT('Ctrl Pts',(-1.45571798513491,2.28101755500643,
7.35743067251521));
#113613=CARTESIAN_POINT('Ctrl Pts',(-1.48513956595445,2.28571428599273,
7.3514869560092));
#113614=CARTESIAN_POINT('Ctrl Pts',(-1.6336769181982,2.30942613108789,7.32147959850119));
#113615=CARTESIAN_POINT('Ctrl Pts',(-1.781812381869,2.33338330844784,7.28686364542245));
#113616=CARTESIAN_POINT('Ctrl Pts',(-1.92912083042035,2.35752261723028,
7.24765429772187));
#113617=CARTESIAN_POINT('Ctrl Pts',(-1.9371564131139,2.35883940125587,7.24551545260534));
#113618=CARTESIAN_POINT('Ctrl Pts',(-1.94518953431861,2.36015672630246,
7.24336295208475));
#113619=CARTESIAN_POINT('Ctrl Pts',(-1.953220124902,2.36147458179854,7.24119680308756));
#113620=CARTESIAN_POINT('',(-0.841285032614847,2.36147458149274,7.45266660087847));
#113621=CARTESIAN_POINT('Origin',(0.0135835823357038,2.41070044829264,-0.190873985324191));
#113622=CARTESIAN_POINT('Origin',(0.0511750907285721,2.55351789526579,-0.181760610305085));
#113623=CARTESIAN_POINT('Ctrl Pts',(-1.361330525,2.492226207,7.121044811));
#113624=CARTESIAN_POINT('Ctrl Pts',(-0.971833309999999,2.42647128,7.195505015));
#113625=CARTESIAN_POINT('Ctrl Pts',(-0.576538529,2.361474582,7.22703973500001));
#113626=CARTESIAN_POINT('Ctrl Pts',(-0.572602868521616,2.36082745750497,
7.22735370309967));
#113627=CARTESIAN_POINT('Ctrl Pts',(-0.568667208043231,2.36018033300993,
7.22766767119934));
#113628=CARTESIAN_POINT('Ctrl Pts',(-1.649106096,2.492226207,7.31645058));
#113629=CARTESIAN_POINT('Ctrl Pts',(-1.248920843,2.42647128,7.40665114));
#113630=CARTESIAN_POINT('Ctrl Pts',(-0.841285031000001,2.361474582,7.452666603));
#113631=CARTESIAN_POINT('Ctrl Pts',(-0.837226499918957,2.36082745750497,
7.45312474524682));
#113632=CARTESIAN_POINT('Ctrl Pts',(-0.833167968837915,2.36018033300993,
7.45358288749364));
#113633=CARTESIAN_POINT('',(-0.708911788726928,2.36147458056998,7.33985316815712));
#113634=CARTESIAN_POINT('Origin',(2.954450920023E-15,2.45311202899978,-8.63024929298462E-14));
#113635=CARTESIAN_POINT('',(0.220017211027225,2.27159573079591,7.49677213352331));
#113636=CARTESIAN_POINT('',(-0.350911660640484,2.36147458096338,7.49178621436893));
#113637=CARTESIAN_POINT('Ctrl Pts',(0.220017202257164,2.27159573312873,
7.49677213346454));
#113638=CARTESIAN_POINT('Ctrl Pts',(0.189974626846442,2.27631121120357,
7.49765383118156));
#113639=CARTESIAN_POINT('Ctrl Pts',(0.159946002989426,2.28101755501591,
7.49835436841248));
#113640=CARTESIAN_POINT('Ctrl Pts',(0.129934559153272,2.28571428596736,
7.49887438293933));
#113641=CARTESIAN_POINT('Ctrl Pts',(-0.0215804301581485,2.30942607826874,
7.50149971437863));
#113642=CARTESIAN_POINT('Ctrl Pts',(-0.173693637262223,2.33338320200953,
7.4995378236021));
#113643=CARTESIAN_POINT('Ctrl Pts',(-0.325986608252011,2.35752245638422,
7.49291216606165));
#113644=CARTESIAN_POINT('Ctrl Pts',(-0.334294450196394,2.3588392939815,
7.49255072511486));
#113645=CARTESIAN_POINT('Ctrl Pts',(-0.342602823753382,2.36015667264389,
7.49217541774316));
#113646=CARTESIAN_POINT('Ctrl Pts',(-0.350911659908851,2.36147458179854,
7.49178623584948));
#113647=CARTESIAN_POINT('Origin',(-0.0277662652684496,2.4107004765019,-0.18933166728919));
#113648=CARTESIAN_POINT('Origin',(0.00113769343467042,2.41071408166251,
-0.193055184199305));
#113649=CARTESIAN_POINT('Ctrl Pts',(-0.584391742461101,2.36016764195642,
7.22641324335268));
#113650=CARTESIAN_POINT('Ctrl Pts',(-0.58046513573055,2.36082111197821,
7.22672648917634));
#113651=CARTESIAN_POINT('Ctrl Pts',(-0.576538529,2.361474582,7.227039735));
#113652=CARTESIAN_POINT('Ctrl Pts',(-0.183440845,2.426894312,7.25839918));
#113653=CARTESIAN_POINT('Ctrl Pts',(0.210739078,2.492218586,7.246936528));
#113654=CARTESIAN_POINT('Ctrl Pts',(-0.359052559442651,2.36016764195642,
7.49140492024465));
#113655=CARTESIAN_POINT('Ctrl Pts',(-0.354982110221325,2.36082111197821,
7.49159557812232));
#113656=CARTESIAN_POINT('Ctrl Pts',(-0.350911661,2.361474582,7.491786236));
#113657=CARTESIAN_POINT('Ctrl Pts',(0.056586281,2.426894312,7.510873243));
#113658=CARTESIAN_POINT('Ctrl Pts',(0.463750383,2.492218586,7.485648641));
#113659=CARTESIAN_POINT('',(-0.46372508454669,2.36147458031212,7.35941298615868));
#113660=CARTESIAN_POINT('Ctrl Pts',(-1.16911722834105,3.52699760873882,
7.40832185973167));
#113661=CARTESIAN_POINT('Ctrl Pts',(-1.16504783117053,3.52633876186941,
7.40895947636584));
#113662=CARTESIAN_POINT('Ctrl Pts',(-1.160978434,3.525679915,7.40959709300001));
#113663=CARTESIAN_POINT('Ctrl Pts',(-0.754960220000001,3.459944422,7.47321437));
#113664=CARTESIAN_POINT('Ctrl Pts',(-0.344421845,3.395197164,7.492087399));
#113665=CARTESIAN_POINT('Ctrl Pts',(-1.36439911743497,3.52699760873882,
7.12046195559663));
#113666=CARTESIAN_POINT('Ctrl Pts',(-1.36048769671748,3.52633876186941,
7.12120699579831));
#113667=CARTESIAN_POINT('Ctrl Pts',(-1.356576276,3.525679915,7.121952036));
#113668=CARTESIAN_POINT('Ctrl Pts',(-0.966319934,3.459944422,7.196287344));
#113669=CARTESIAN_POINT('Ctrl Pts',(-0.570277963,3.395197164,7.227536444));
#113670=CARTESIAN_POINT('',(-0.596501776703425,3.43511457442473,7.47624139567237));
#113671=CARTESIAN_POINT('',(-1.16097843672315,3.52567991457199,7.40959709383369));
#113672=CARTESIAN_POINT('Origin',(0.0448629934745826,3.62494886961495,-0.183552747796982));
#113673=CARTESIAN_POINT('',(-1.25877736262446,3.52567991373767,7.26577456317908));
#113674=CARTESIAN_POINT('Ctrl Pts',(-0.596501780179129,3.43511457412329,
7.47624139542084));
#113675=CARTESIAN_POINT('Ctrl Pts',(-0.592954403265114,3.42888807477894,
7.4346863736556));
#113676=CARTESIAN_POINT('Ctrl Pts',(-0.589386786366554,3.42251694825873,
7.39313242858002));
#113677=CARTESIAN_POINT('Ctrl Pts',(-0.582214640223985,3.40947716052633,
7.31011921060845));
#113678=CARTESIAN_POINT('Ctrl Pts',(-0.578606272435709,3.4028015174756,
7.26861546467834));
#113679=CARTESIAN_POINT('Ctrl Pts',(-0.574977340862851,3.39596551404509,
7.22716410908228));
#113680=CARTESIAN_POINT('Ctrl Pts',(-2.426773305,3.395189501,7.096532345));
#113681=CARTESIAN_POINT('Ctrl Pts',(-2.041496927,3.460370723,7.228283796));
#113682=CARTESIAN_POINT('Ctrl Pts',(-1.644221332,3.525679915,7.317549878));
#113683=CARTESIAN_POINT('Ctrl Pts',(-2.119643019,3.395189501,6.93322533));
#113684=CARTESIAN_POINT('Ctrl Pts',(-1.743232708,3.460370723,7.048302433));
#113685=CARTESIAN_POINT('Ctrl Pts',(-1.356576276,3.525679915,7.121952036));
#113686=CARTESIAN_POINT('',(-1.64422134204873,3.52567991637276,7.31754987448137));
#113687=CARTESIAN_POINT('',(-1.50039881645216,3.52567991706905,7.21975095441222));
#113688=CARTESIAN_POINT('',(-2.18972679882163,3.43511457319675,7.17322077734424));
#113689=CARTESIAN_POINT('Origin',(0.0491103654982606,3.48214117966952,-0.186710050349461));
#113690=CARTESIAN_POINT('Ctrl Pts',(-2.11516133959162,3.39596551405412,
6.934593896648));
#113691=CARTESIAN_POINT('Ctrl Pts',(-2.12761629753411,3.40280154624219,
6.97429619650466));
#113692=CARTESIAN_POINT('Ctrl Pts',(-2.14006244103257,3.4094772188388,7.01405410403077));
#113693=CARTESIAN_POINT('Ctrl Pts',(-2.16491218325618,3.42251694822848,
7.09358436376503));
#113694=CARTESIAN_POINT('Ctrl Pts',(-2.17732926107205,3.42888807475033,
7.13339986851063));
#113695=CARTESIAN_POINT('Ctrl Pts',(-2.18972680351047,3.43511457408882,
7.17322077574496));
#113696=CARTESIAN_POINT('Ctrl Pts',(-2.73435412840025,3.52699760873882,
6.98379376576679));
#113697=CARTESIAN_POINT('Ctrl Pts',(-2.73051694020013,3.52633876186941,
6.98529127538339));
#113698=CARTESIAN_POINT('Ctrl Pts',(-2.726679752,3.525679915,6.986788785));
#113699=CARTESIAN_POINT('Ctrl Pts',(-2.343829852,3.459944422,7.13620064));
#113700=CARTESIAN_POINT('Ctrl Pts',(-1.94694678,3.395197164,7.242886043));
#113701=CARTESIAN_POINT('Ctrl Pts',(-2.86318906447492,3.52699760873882,
6.66068403319031));
#113702=CARTESIAN_POINT('Ctrl Pts',(-2.85952925223746,3.52633876186941,
6.66225249459515));
#113703=CARTESIAN_POINT('Ctrl Pts',(-2.85586944,3.525679915,6.663820956));
#113704=CARTESIAN_POINT('Ctrl Pts',(-2.49071697,3.459944422,6.820311923));
#113705=CARTESIAN_POINT('Ctrl Pts',(-2.110651872,3.395197164,6.935967753));
#113706=CARTESIAN_POINT('',(-2.72667975481357,3.52567991457199,6.98678878525083));
#113707=CARTESIAN_POINT('Origin',(0.0832725405001064,3.6249488517541,-0.16961717234676));
#113708=CARTESIAN_POINT('',(-2.7912746031623,3.52567991373766,6.82530486757091));
#113709=CARTESIAN_POINT('Origin',(2.41451823812522E-13,3.61749373599956,
-9.03357250114922E-13));
#113710=CARTESIAN_POINT('',(-2.19122982986197,3.61640598740785,7.17276179905093));
#113711=CARTESIAN_POINT('Origin',(0.0575818226972896,3.62499778718194,-0.183734944048718));
#113712=CARTESIAN_POINT('Origin',(0.0761123372709183,3.48215430157035,-0.17577726192358));
#113713=CARTESIAN_POINT('Ctrl Pts',(-3.895581376,3.395189501,6.408934837));
#113714=CARTESIAN_POINT('Ctrl Pts',(-3.547635213,3.460370723,6.620429044));
#113715=CARTESIAN_POINT('Ctrl Pts',(-3.178837269,3.525679915,6.793010644));
#113716=CARTESIAN_POINT('Ctrl Pts',(-3.560525444,3.395189501,6.315469782));
#113717=CARTESIAN_POINT('Ctrl Pts',(-3.217653573,3.460370723,6.508773536));
#113718=CARTESIAN_POINT('Ctrl Pts',(-2.85586944,3.525679915,6.663820956));
#113719=CARTESIAN_POINT('',(-3.17883727810971,3.52567991637269,6.79301063840168));
#113720=CARTESIAN_POINT('',(-3.01735336610406,3.52567991706893,6.72841579479618));
#113721=CARTESIAN_POINT('',(-3.68056263161433,3.43511457320845,6.53478832800663));
#113722=CARTESIAN_POINT('Origin',(0.0880994187286996,3.4821411487701,-0.171787782088027));
#113723=CARTESIAN_POINT('Ctrl Pts',(-3.55644274523096,3.39596551401258,
6.31776978074831));
#113724=CARTESIAN_POINT('Ctrl Pts',(-3.57714133398142,3.40280154619979,
6.35386641498873));
#113725=CARTESIAN_POINT('Ctrl Pts',(-3.59784326871524,3.40947721887761,
6.39001925214229));
#113726=CARTESIAN_POINT('Ctrl Pts',(-3.63920869283814,3.42251694825907,
6.46234817839716));
#113727=CARTESIAN_POINT('Ctrl Pts',(-3.65989462299297,3.428888074784,6.4985635140514));
#113728=CARTESIAN_POINT('Ctrl Pts',(-3.68056263589092,3.43511457412385,
6.53478832540929));
#113729=CARTESIAN_POINT('Ctrl Pts',(-4.17173566914475,3.52699760873882,
6.23271123756692));
#113730=CARTESIAN_POINT('Ctrl Pts',(-4.16831011257238,3.52633876186941,
6.23499861828346));
#113731=CARTESIAN_POINT('Ctrl Pts',(-4.164884556,3.525679915,6.237285999));
#113732=CARTESIAN_POINT('Ctrl Pts',(-3.823104606,3.459944422,6.4655061));
#113733=CARTESIAN_POINT('Ctrl Pts',(-3.458434647,3.395197164,6.655015386));
#113734=CARTESIAN_POINT('Ctrl Pts',(-4.22809947406292,3.52699760873882,
5.88945992881435));
#113735=CARTESIAN_POINT('Ctrl Pts',(-4.22486239903146,3.52633876186941,
5.89177847190718));
#113736=CARTESIAN_POINT('Ctrl Pts',(-4.221625324,3.525679915,5.894097015));
#113737=CARTESIAN_POINT('Ctrl Pts',(-3.898650847,3.459944422,6.125426297));
#113738=CARTESIAN_POINT('Ctrl Pts',(-3.552334045,3.395197164,6.32008092));
#113739=CARTESIAN_POINT('',(-4.16488455880619,3.52567991457199,6.23728599863403));
#113740=CARTESIAN_POINT('Origin',(0.117788269120822,3.62494884602207,-0.147750345564207));
#113741=CARTESIAN_POINT('',(-4.19325494636514,3.52567991373767,6.06569150259974));
#113742=CARTESIAN_POINT('Origin',(4.6447221069279E-13,3.61749373599978,
-9.05091973590899E-13));
#113743=CARTESIAN_POINT('',(-3.68193185568054,3.61640598737383,6.5340169729667));
#113744=CARTESIAN_POINT('Origin',(0.0957330761232028,3.62499780219289,-0.16706076477176));
#113745=CARTESIAN_POINT('Origin',(0.112119826861367,3.48215433084305,-0.155305859871593));
#113746=CARTESIAN_POINT('Ctrl Pts',(-5.182236391,3.395189501,5.421662659));
#113747=CARTESIAN_POINT('Ctrl Pts',(-4.887890019,3.460370723,5.703010389));
#113748=CARTESIAN_POINT('Ctrl Pts',(-4.564814309,3.525679915,5.950837783));
#113749=CARTESIAN_POINT('Ctrl Pts',(-4.83492165700001,3.395189501,5.402409886));
#113750=CARTESIAN_POINT('Ctrl Pts',(-4.541620533,3.460370723,5.664901623));
#113751=CARTESIAN_POINT('Ctrl Pts',(-4.221625324,3.525679915,5.894097015));
#113752=CARTESIAN_POINT('',(-4.56481431668058,3.52567991637268,5.95083777557618));
#113753=CARTESIAN_POINT('',(-4.39321982671409,3.52567991706893,5.92246739142331));
#113754=CARTESIAN_POINT('',(-4.99929944581776,3.43511457319354,5.59079643925668));
#113755=CARTESIAN_POINT('Origin',(0.122968880900439,3.48214118309511,-0.148832566926366));
#113756=CARTESIAN_POINT('Ctrl Pts',(-4.83142884122636,3.39596551396059,
5.40553377138989));
#113757=CARTESIAN_POINT('Ctrl Pts',(-4.8594032178137,3.40280154614786,5.43633690171973));
#113758=CARTESIAN_POINT('Ctrl Pts',(-4.88739294392432,3.40947721879129,
5.46719420151078));
#113759=CARTESIAN_POINT('Ctrl Pts',(-4.94333984841411,3.42251694818979,
5.5289397744007));
#113760=CARTESIAN_POINT('Ctrl Pts',(-4.97132737958918,3.42888807472649,
5.55986155220594));
#113761=CARTESIAN_POINT('Ctrl Pts',(-4.99929944939275,3.43511457407926,
5.59079643584581));
#113762=CARTESIAN_POINT('Ctrl Pts',(-5.42801715776659,3.53021247069526,
5.17641922555657));
#113763=CARTESIAN_POINT('Ctrl Pts',(-5.41819957354462,3.52794619284766,
5.1866364165488));
#113764=CARTESIAN_POINT('Ctrl Pts',(-5.40838198932263,3.525679915,5.19685360754093));
#113765=CARTESIAN_POINT('Ctrl Pts',(-5.1236138442468,3.459944422,5.49321271798337));
#113766=CARTESIAN_POINT('Ctrl Pts',(-4.80816917351001,3.395197164,5.75668240936443));
#113767=CARTESIAN_POINT('Ctrl Pts',(-5.40830271729218,3.53021247069526,
4.82840678376583));
#113768=CARTESIAN_POINT('Ctrl Pts',(-5.39914270864615,3.52794619284766,
4.83858921588293));
#113769=CARTESIAN_POINT('Ctrl Pts',(-5.3899827,3.525679915,4.848771648));
#113770=CARTESIAN_POINT('Ctrl Pts',(-5.124288145,3.459944422,5.144122545));
#113771=CARTESIAN_POINT('Ctrl Pts',(-4.827913027,3.395197164,5.408674126));
#113772=CARTESIAN_POINT('',(-5.40834399215434,3.52567991457842,5.19613464520341));
#113773=CARTESIAN_POINT('Origin',(0.146796449455316,3.62494884986666,-0.118975073921826));
#113774=CARTESIAN_POINT('',(-5.3991633482704,3.52567991373767,5.02245314433429));
#113775=CARTESIAN_POINT('Origin',(1.20129600711394E-13,3.61749373600033,
-1.42681005899092E-13));
#113776=CARTESIAN_POINT('',(-5.00047084026899,3.61640598737486,5.58974877539373));
#113777=CARTESIAN_POINT('Origin',(0.129407994724612,3.62499781851073,-0.142575166282169));
#113778=CARTESIAN_POINT('Origin',(0.142884588065562,3.48215430997448,-0.127572317519105));
#113779=CARTESIAN_POINT('Ctrl Pts',(-6.226575793,3.395189501,4.180879561));
#113780=CARTESIAN_POINT('Ctrl Pts',(-5.99959252,3.460370723,4.518925306));
#113781=CARTESIAN_POINT('Ctrl Pts',(-5.737345705,3.525679915,4.830410362));
#113782=CARTESIAN_POINT('Ctrl Pts',(-5.88324230700001,3.395189501,4.236739308));
#113783=CARTESIAN_POINT('Ctrl Pts',(-5.653226364,3.460370723,4.556145206));
#113784=CARTESIAN_POINT('Ctrl Pts',(-5.3899827,3.525679915,4.848771648));
#113785=CARTESIAN_POINT('',(-5.73734571087744,3.52567991637269,4.83041035311642));
#113786=CARTESIAN_POINT('',(-5.56366421084652,3.52567991706893,4.83959099540472));
#113787=CARTESIAN_POINT('',(-6.08427457474554,3.43511457319035,4.38538512284339));
#113788=CARTESIAN_POINT('Origin',(0.15208886535066,3.48214117880472,-0.118918515677711));
#113789=CARTESIAN_POINT('Ctrl Pts',(-5.88050269398345,3.39596551395666,
4.24054101087128));
#113790=CARTESIAN_POINT('Ctrl Pts',(-5.91444480768252,3.40280154613216,
4.26461031711559));
#113791=CARTESIAN_POINT('Ctrl Pts',(-5.94841355696679,3.40947721878168,
4.28872922669257));
#113792=CARTESIAN_POINT('Ctrl Pts',(-6.01632592701229,3.42251694817642,
4.33700429172433));
#113793=CARTESIAN_POINT('Ctrl Pts',(-6.05030639351071,3.42888807471328,
4.36118664364647));
#113794=CARTESIAN_POINT('Ctrl Pts',(-6.08427457749733,3.43511457406995,
4.38538511875428));
#113795=CARTESIAN_POINT('Ctrl Pts',(-6.41389025267975,3.53021247057256,
3.88853418349163));
#113796=CARTESIAN_POINT('Ctrl Pts',(-6.40649859234271,3.52794619278631,
3.90062299231468));
#113797=CARTESIAN_POINT('Ctrl Pts',(-6.39910693200571,3.525679915,3.91271180113778));
#113798=CARTESIAN_POINT('Ctrl Pts',(-6.18470495565505,3.459944422,4.26335893388248));
#113799=CARTESIAN_POINT('Ctrl Pts',(-5.93327340240695,3.395197164,4.58848012970719));
#113800=CARTESIAN_POINT('Ctrl Pts',(-6.31982433736954,3.53021247057255,
3.5528961003417));
#113801=CARTESIAN_POINT('Ctrl Pts',(-6.31306740668471,3.52794619278631,
3.56480960367085));
#113802=CARTESIAN_POINT('Ctrl Pts',(-6.306310476,3.525679915,3.576723107));
#113803=CARTESIAN_POINT('Ctrl Pts',(-6.110319423,3.459944422,3.922285341));
#113804=CARTESIAN_POINT('Ctrl Pts',(-5.877744161,3.395197164,4.244363742));
#113805=CARTESIAN_POINT('',(-6.39891526807721,3.52567991503086,3.91201781576554));
#113806=CARTESIAN_POINT('Origin',(0.168940701023456,3.62494882504361,-0.0846367114639096));
#113807=CARTESIAN_POINT('',(-6.35261287342922,3.52567991373767,3.74437045883377));
#113808=CARTESIAN_POINT('Origin',(6.48352899146332E-13,3.61749373600089,
-4.36716635077161E-13));
#113809=CARTESIAN_POINT('',(-6.08519336544766,3.61640598741484,4.38411013764515));
#113810=CARTESIAN_POINT('Origin',(0.157031971607143,3.62499783912985,-0.111422941150182));
#113811=CARTESIAN_POINT('Origin',(0.166968276007746,3.48215435135676,-0.0938737837871401));
#113812=CARTESIAN_POINT('Ctrl Pts',(-6.97976743,3.395189501,2.744603181));
#113813=CARTESIAN_POINT('Ctrl Pts',(-6.830760744,3.460370723,3.123540298));
#113814=CARTESIAN_POINT('Ctrl Pts',(-6.641605193,3.525679915,3.48411832));
#113815=CARTESIAN_POINT('Ctrl Pts',(-6.656469085,3.395189501,2.872963509));
#113816=CARTESIAN_POINT('Ctrl Pts',(-6.50049361399999,3.460370723,3.234348502));
#113817=CARTESIAN_POINT('Ctrl Pts',(-6.306310476,3.525679915,3.576723107));
#113818=CARTESIAN_POINT('',(-6.64160519682503,3.52567991637272,3.48411831007144));
#113819=CARTESIAN_POINT('',(-6.47395784058869,3.52567991706893,3.5304207023348));
#113820=CARTESIAN_POINT('',(-6.8847557866728,3.43511457320295,2.97491807196946));
#113821=CARTESIAN_POINT('Origin',(0.174096893675357,3.48214111904205,-0.0834435547269661));
#113822=CARTESIAN_POINT('Ctrl Pts',(-6.65461077687043,3.3959655139869,2.87726526591025));
#113823=CARTESIAN_POINT('Ctrl Pts',(-6.69293353213603,3.40280154617958,
2.89347529396363));
#113824=CARTESIAN_POINT('Ctrl Pts',(-6.73129296357907,3.40947721884582,
2.90972803983227));
#113825=CARTESIAN_POINT('Ctrl Pts',(-6.80799529206524,3.42251694823562,
2.94227530850979));
#113826=CARTESIAN_POINT('Ctrl Pts',(-6.84637980495893,3.42888807476465,
2.9585874946168));
#113827=CARTESIAN_POINT('Ctrl Pts',(-6.88475578849858,3.43511457410741,
2.97491806733411));
#113828=CARTESIAN_POINT('Ctrl Pts',(-7.09985696847863,3.53021247071098,
2.41882560302897));
#113829=CARTESIAN_POINT('Ctrl Pts',(-7.09523685747579,3.52794619285552,
2.4322207711079));
#113830=CARTESIAN_POINT('Ctrl Pts',(-7.09061674647308,3.525679915,2.44561593918682));
#113831=CARTESIAN_POINT('Ctrl Pts',(-6.95660613795883,3.459944422,2.8341552241401));
#113832=CARTESIAN_POINT('Ctrl Pts',(-6.78094436032421,3.395197164,3.205725619537));
#113833=CARTESIAN_POINT('Ctrl Pts',(-6.93583799490026,3.53021247071098,
2.11125594298556));
#113834=CARTESIAN_POINT('Ctrl Pts',(-6.93180008845007,3.52794619285552,
2.12434345599278));
#113835=CARTESIAN_POINT('Ctrl Pts',(-6.927762182,3.525679915,2.137430969));
#113836=CARTESIAN_POINT('Ctrl Pts',(-6.810638957,3.459944422,2.517046433));
#113837=CARTESIAN_POINT('Ctrl Pts',(-6.652738511,3.395197164,2.881591627));
#113838=CARTESIAN_POINT('',(-7.09028037716511,3.52567991503086,2.44497938085858));
#113839=CARTESIAN_POINT('Origin',(0.183185218093685,3.62494884872823,-0.0463406396412325));
#113840=CARTESIAN_POINT('',(-7.00902128040432,3.52567991373767,2.29120517214497));
#113841=CARTESIAN_POINT('Origin',(-4.28043017697277E-13,3.61749373599989,
1.12540185503995E-13));
#113842=CARTESIAN_POINT('',(-6.88537901244733,3.61640598739985,2.97347538228457));
#113843=CARTESIAN_POINT('Origin',(0.177313480335798,3.6249978219611,-0.0750607932934111));
#113844=CARTESIAN_POINT('Origin',(0.183244805852569,3.48215435875214,-0.0557858511365902));
#113845=CARTESIAN_POINT('Ctrl Pts',(-7.4065929,3.395189501,1.179992206));
#113846=CARTESIAN_POINT('Ctrl Pts',(-7.342530186,3.460370723,1.582102018));
#113847=CARTESIAN_POINT('Ctrl Pts',(-7.235310603,3.525679915,1.974912778));
#113848=CARTESIAN_POINT('Ctrl Pts',(-7.118446767,3.395189501,1.374851129));
#113849=CARTESIAN_POINT('Ctrl Pts',(-7.043805007,3.460370723,1.761317258));
#113850=CARTESIAN_POINT('Ctrl Pts',(-6.927762182,3.525679915,2.137430969));
#113851=CARTESIAN_POINT('',(-7.23531060460634,3.52567991637269,1.97491276746508));
#113852=CARTESIAN_POINT('',(-7.08153639604615,3.52567991706893,2.05617186128694));
#113853=CARTESIAN_POINT('',(-7.36331346968431,3.43511457321339,1.42534715830193));
#113854=CARTESIAN_POINT('Origin',(0.187964634940831,3.48214115787911,-0.0440670445990793));
#113855=CARTESIAN_POINT('Ctrl Pts',(-7.1175566558214,3.39596551405672,1.37945179479932));
#113856=CARTESIAN_POINT('Ctrl Pts',(-7.15846812332044,3.40280154624432,
1.38704458171414));
#113857=CARTESIAN_POINT('Ctrl Pts',(-7.19942459238286,3.40947721888432,
1.39467120346668));
#113858=CARTESIAN_POINT('Ctrl Pts',(-7.2813303637261,3.42251694827523,1.40996880173583));
#113859=CARTESIAN_POINT('Ctrl Pts',(-7.32232410578099,3.42888807479856,
1.41764808237601));
#113860=CARTESIAN_POINT('Ctrl Pts',(-7.36331347047552,3.43511457413836,
1.42534715334153));
#113861=CARTESIAN_POINT('Ctrl Pts',(-7.45384226280907,3.53021247049811,
0.836015428641415));
#113862=CARTESIAN_POINT('Ctrl Pts',(-7.4522097326595,3.52794619274909,0.850090611749254));
#113863=CARTESIAN_POINT('Ctrl Pts',(-7.4505772025098,3.525679915,0.864165794857096));
#113864=CARTESIAN_POINT('Ctrl Pts',(-7.40322414780592,3.459944422,1.27242956615997));
#113865=CARTESIAN_POINT('Ctrl Pts',(-7.31154589717169,3.395197164,1.673074941636));
#113866=CARTESIAN_POINT('Ctrl Pts',(-7.22753957586448,3.53021247049811,
0.570895806820382));
#113867=CARTESIAN_POINT('Ctrl Pts',(-7.22640950193228,3.52794619274909,
0.584545370910196));
#113868=CARTESIAN_POINT('Ctrl Pts',(-7.225279428,3.525679915,0.598194935));
#113869=CARTESIAN_POINT('Ctrl Pts',(-7.192500583,3.459944422,0.994113231));
#113870=CARTESIAN_POINT('Ctrl Pts',(-7.116658202,3.395197164,1.38407949));
#113871=CARTESIAN_POINT('',(-7.45011185602574,3.52567991503086,0.863616428380273));
#113872=CARTESIAN_POINT('Origin',(0.188864586681895,3.6249488631317,-0.00587786011865737));
#113873=CARTESIAN_POINT('',(-7.337695642267,3.52567991373765,0.730905678799971));
#113874=CARTESIAN_POINT('Origin',(-4.90493062832442E-13,3.61749373599933,
2.90566182226115E-14));
#113875=CARTESIAN_POINT('',(-7.36361198950021,3.61640598739899,1.423804222735));
#113876=CARTESIAN_POINT('Origin',(0.189303689547513,3.62499782970624,-0.0351887269185508));
#113877=CARTESIAN_POINT('Origin',(0.190953314121111,3.48215429853827,-0.0150894401907962));
#113878=CARTESIAN_POINT('Ctrl Pts',(-7.487094318,3.395189501,-0.439793892));
#113879=CARTESIAN_POINT('Ctrl Pts',(-7.510971078,3.460370723,-0.033313594));
#113880=CARTESIAN_POINT('Ctrl Pts',(-7.490700931,3.525679915,0.373362509));
#113881=CARTESIAN_POINT('Ctrl Pts',(-7.24757379,3.395189501,-0.187547762));
#113882=CARTESIAN_POINT('Ctrl Pts',(-7.25775590700001,3.460370723,0.205928776));
#113883=CARTESIAN_POINT('Ctrl Pts',(-7.225279428,3.525679915,0.598194935));
#113884=CARTESIAN_POINT('',(-7.49070093030407,3.52567991637267,0.373362498359974));
#113885=CARTESIAN_POINT('',(-7.35799018033778,3.52567991706892,0.485778709310209));
#113886=CARTESIAN_POINT('',(-7.49757079857549,3.43511457319164,-0.190871404225564));
#113887=CARTESIAN_POINT('Origin',(0.193043078825646,3.48214121353905,-0.00262994821670431));
#113888=CARTESIAN_POINT('Ctrl Pts',(-7.24769349603453,3.39596551408267,
-0.182863309194341));
#113889=CARTESIAN_POINT('Ctrl Pts',(-7.28928070096139,3.4028015462638,-0.184242793530343));
#113890=CARTESIAN_POINT('Ctrl Pts',(-7.3309191285908,3.40947721885932,-0.185598908098326));
#113891=CARTESIAN_POINT('Ctrl Pts',(-7.41419852000121,3.42251694823117,
-0.188266278868783));
#113892=CARTESIAN_POINT('Ctrl Pts',(-7.45588466949589,3.42888807474393,
-0.189578978324019));
#113893=CARTESIAN_POINT('Ctrl Pts',(-7.4975707982911,3.43511457407353,-0.190871409149947));
#113894=CARTESIAN_POINT('Ctrl Pts',(-7.46075164741015,3.52699760873882,
-0.766324157850277));
#113895=CARTESIAN_POINT('Ctrl Pts',(-7.46116801620508,3.52633876186941,
-0.762226208925139));
#113896=CARTESIAN_POINT('Ctrl Pts',(-7.461584385,3.525679915,-0.75812826));
#113897=CARTESIAN_POINT('Ctrl Pts',(-7.503126979,3.459944422,-0.349261336));
#113898=CARTESIAN_POINT('Ctrl Pts',(-7.49974623,3.395197164,0.061696714));
#113899=CARTESIAN_POINT('Ctrl Pts',(-7.18388626403411,3.52699760873882,
-0.9769040688728));
#113900=CARTESIAN_POINT('Ctrl Pts',(-7.18441845151706,3.52633876186941,
-0.9729580489364));
#113901=CARTESIAN_POINT('Ctrl Pts',(-7.184950639,3.525679915,-0.969012029));
#113902=CARTESIAN_POINT('Ctrl Pts',(-7.238048875,3.459944422,-0.5753036));
#113903=CARTESIAN_POINT('Ctrl Pts',(-7.247810865,3.395197164,-0.178150666));
#113904=CARTESIAN_POINT('',(-7.46158438599956,3.52567991457199,-0.758128262633195));
#113905=CARTESIAN_POINT('Origin',(0.185712522317807,3.62494885578236,0.0348598660157013));
#113906=CARTESIAN_POINT('',(-7.32326751109379,3.52567991373765,-0.863570152184889));
#113907=CARTESIAN_POINT('Origin',(-1.25507243486922E-12,3.617493736,5.41830035699631E-14));
#113908=CARTESIAN_POINT('',(-7.49753065353308,3.61640598744037,-0.192442439414313));
#113909=CARTESIAN_POINT('Origin',(0.19244229328369,3.62499780846281,0.00632866299894386));
#113910=CARTESIAN_POINT('Origin',(0.189732559278504,3.48215432117043,0.0263126537729071));
#113911=CARTESIAN_POINT('Ctrl Pts',(-7.217507527,3.395189501,-2.039015717));
#113912=CARTESIAN_POINT('Ctrl Pts',(-7.32820731,3.460370723,-1.6471715));
#113913=CARTESIAN_POINT('Ctrl Pts',(-7.39583440900001,3.525679915,-1.245645776));
#113914=CARTESIAN_POINT('Ctrl Pts',(-7.037812317,3.395189501,-1.741177127));
#113915=CARTESIAN_POINT('Ctrl Pts',(-7.132342206,3.460370723,-1.359088706));
#113916=CARTESIAN_POINT('Ctrl Pts',(-7.184950639,3.525679915,-0.969012029));
#113917=CARTESIAN_POINT('',(-7.39583440602979,3.52567991637266,-1.2456457862268));
#113918=CARTESIAN_POINT('',(-7.29039252209027,3.52567991706892,-1.10732891507321));
#113919=CARTESIAN_POINT('',(-7.28125005028088,3.43511457321144,-1.7981650321231));
#113920=CARTESIAN_POINT('Origin',(0.18909539415706,3.4821411876723,0.0389301375708813));
#113921=CARTESIAN_POINT('Ctrl Pts',(-7.03893624352272,3.39596551401659,
-1.73662792835121));
#113922=CARTESIAN_POINT('Ctrl Pts',(-7.07925461423005,3.40280154619732,
-1.74691518075888));
#113923=CARTESIAN_POINT('Ctrl Pts',(-7.11962803441265,3.40947721887202,
-1.75719062129386));
#113924=CARTESIAN_POINT('Ctrl Pts',(-7.20038699401208,3.42251694825527,
-1.77769823777738));
#113925=CARTESIAN_POINT('Ctrl Pts',(-7.24081635299754,3.42888807478671,
-1.78794153696337));
#113926=CARTESIAN_POINT('Ctrl Pts',(-7.28125004891864,3.43511457413287,
-1.7981650369495));
#113927=CARTESIAN_POINT('Ctrl Pts',(-7.121586378581,3.52699760873882,-2.3522489903306));
#113928=CARTESIAN_POINT('Ctrl Pts',(-7.12287395079049,3.52633876186941,
-2.3483363561653));
#113929=CARTESIAN_POINT('Ctrl Pts',(-7.124161523,3.525679915,-2.344423722));
#113930=CARTESIAN_POINT('Ctrl Pts',(-7.252627177,3.459944422,-1.95404631));
#113931=CARTESIAN_POINT('Ctrl Pts',(-7.337669301,3.395197164,-1.551969469));
#113932=CARTESIAN_POINT('Ctrl Pts',(-6.80592549724464,3.52699760873882,
-2.49838778720026));
#113933=CARTESIAN_POINT('Ctrl Pts',(-6.80729352012233,3.52633876186941,
-2.49464842760013));
#113934=CARTESIAN_POINT('Ctrl Pts',(-6.808661543,3.525679915,-2.490909068));
#113935=CARTESIAN_POINT('Ctrl Pts',(-6.945154046,3.459944422,-2.117819875));
#113936=CARTESIAN_POINT('Ctrl Pts',(-7.040063948,3.395197164,-1.732050695));
#113937=CARTESIAN_POINT('',(-7.12416152340778,3.52567991457199,-2.34442372478951));
#113938=CARTESIAN_POINT('Origin',(0.17387673225741,3.62494889075051,0.0739675469353931));
#113939=CARTESIAN_POINT('',(-6.96641153046295,3.52567991373765,-2.41766640231041));
#113940=CARTESIAN_POINT('Origin',(9.87057657830803E-13,3.61749373599967,
1.99384779520084E-13));
#113941=CARTESIAN_POINT('',(-7.28087311717066,3.61640598742399,-1.79969070725064));
#113942=CARTESIAN_POINT('Origin',(0.186582973251562,3.62499781993517,0.0475501875947812));
#113943=CARTESIAN_POINT('Origin',(0.179640094615405,3.48215430651884,0.0664843171575019));
#113944=CARTESIAN_POINT('Ctrl Pts',(-6.61043810600001,3.395189501,-3.542895433));
#113945=CARTESIAN_POINT('Ctrl Pts',(-6.802784713,3.460370723,-3.184009497));
#113946=CARTESIAN_POINT('Ctrl Pts',(-6.955146889,3.525679915,-2.806409048));
#113947=CARTESIAN_POINT('Ctrl Pts',(-6.498970563,3.395189501,-3.213390985));
#113948=CARTESIAN_POINT('Ctrl Pts',(-6.673428112,3.460370723,-2.860556712));
#113949=CARTESIAN_POINT('Ctrl Pts',(-6.808661543,3.525679915,-2.490909068));
#113950=CARTESIAN_POINT('',(-6.95514688390027,3.52567991637267,-2.80640905739783));
#113951=CARTESIAN_POINT('',(-6.88190421143205,3.52567991706892,-2.64865906986872));
#113952=CARTESIAN_POINT('',(-6.72446614188422,3.43511457320662,-3.32137846142375));
#113953=CARTESIAN_POINT('Origin',(0.176305530987173,3.48214118240383,0.0786698416026864));
#113954=CARTESIAN_POINT('Ctrl Pts',(-6.5010461556297,3.39596551395717,-3.20918975482681));
#113955=CARTESIAN_POINT('Ctrl Pts',(-6.5382102399609,3.40280150749901,-3.22790364916677));
#113956=CARTESIAN_POINT('Ctrl Pts',(-6.57543059806044,3.40947714036133,
-3.24661782840647));
#113957=CARTESIAN_POINT('Ctrl Pts',(-6.64989337480597,3.4225169482316,-3.28400700244851));
#113958=CARTESIAN_POINT('Ctrl Pts',(-6.68717551126765,3.42888807476634,
-3.30270193613753));
#113959=CARTESIAN_POINT('Ctrl Pts',(-6.72446613952633,3.4351145741185,-3.32137846582763));
#113960=CARTESIAN_POINT('Ctrl Pts',(-6.44942364563877,3.52699760873882,
-3.82818527497923));
#113961=CARTESIAN_POINT('Ctrl Pts',(-6.45152221581939,3.52633876186941,
-3.82464090598961));
#113962=CARTESIAN_POINT('Ctrl Pts',(-6.45362078600001,3.525679915,-3.821096537));
#113963=CARTESIAN_POINT('Ctrl Pts',(-6.66300258900001,3.459944422,-3.46746225));
#113964=CARTESIAN_POINT('Ctrl Pts',(-6.83249111,3.395197164,-3.093067285));
#113965=CARTESIAN_POINT('Ctrl Pts',(-6.10972721891902,3.52699760873882,
-3.90304966995008));
#113966=CARTESIAN_POINT('Ctrl Pts',(-6.11186710995951,3.52633876186941,
-3.89969181897504));
#113967=CARTESIAN_POINT('Ctrl Pts',(-6.114007001,3.525679915,-3.896333968));
#113968=CARTESIAN_POINT('Ctrl Pts',(-6.327511533,3.459944422,-3.561309246));
#113969=CARTESIAN_POINT('Ctrl Pts',(-6.503131465,3.395197164,-3.204961958));
#113970=CARTESIAN_POINT('',(-6.45362078579712,3.52567991457199,-3.82109653981316));
#113971=CARTESIAN_POINT('Origin',(0.153910590139191,3.62494886094461,0.109616489232645));
#113972=CARTESIAN_POINT('',(-6.28381388945075,3.52567991373765,-3.8587152590941));
#113973=CARTESIAN_POINT('Origin',(-4.33680868994202E-14,3.61749373599989,
-3.81639164714898E-14));
#113974=CARTESIAN_POINT('',(-6.72377004630369,3.61640598738303,-3.3227874378953));
#113975=CARTESIAN_POINT('Origin',(0.171998886139176,3.62499783308384,0.086548303390474));
#113976=CARTESIAN_POINT('Origin',(0.161148226261515,3.48215433566803,0.103547355812011));
#113977=CARTESIAN_POINT('Ctrl Pts',(-5.694271946,3.395189501,-4.881113296));
#113978=CARTESIAN_POINT('Ctrl Pts',(-5.959271464,3.460370723,-4.571966749));
#113979=CARTESIAN_POINT('Ctrl Pts',(-6.189244432,3.525679915,-4.235947753));
#113980=CARTESIAN_POINT('Ctrl Pts',(-5.656244168,3.395189501,-4.535350253));
#113981=CARTESIAN_POINT('Ctrl Pts',(-5.902471935,3.460370723,-4.228268264));
#113982=CARTESIAN_POINT('Ctrl Pts',(-6.114007001,3.525679915,-3.896333968));
#113983=CARTESIAN_POINT('',(-6.18924442501214,3.52567991637268,-4.2359477610336));
#113984=CARTESIAN_POINT('',(-6.15162570948743,3.52567991706892,-4.06614087110926));
#113985=CARTESIAN_POINT('',(-5.85325367059049,3.43511457319961,-4.68928792510928));
#113986=CARTESIAN_POINT('Origin',(0.155271798014792,3.48214117390607,0.114730992146767));
#113987=CARTESIAN_POINT('Ctrl Pts',(-5.65917437478212,3.39596551399065,
-4.53169343554281));
#113988=CARTESIAN_POINT('Ctrl Pts',(-5.6914466679652,3.40280151145959,-4.55795900404419));
#113989=CARTESIAN_POINT('Ctrl Pts',(-5.72377386047523,3.4094771483571,-4.58423694989676));
#113990=CARTESIAN_POINT('Ctrl Pts',(-5.78845813222718,3.42251694823204,
-4.63675924951398));
#113991=CARTESIAN_POINT('Ctrl Pts',(-5.82084977501639,3.42888807475903,
-4.66303166331845));
#113992=CARTESIAN_POINT('Ctrl Pts',(-5.85325366736076,3.43511457409759,
-4.68928792888226));
#113993=CARTESIAN_POINT('Ctrl Pts',(-5.47569303132712,3.52699760873882,
-5.12511987112299));
#113994=CARTESIAN_POINT('Ctrl Pts',(-5.47850447266356,3.52633876186941,
-5.1221094980615));
#113995=CARTESIAN_POINT('Ctrl Pts',(-5.481315914,3.525679915,-5.119099125));
#113996=CARTESIAN_POINT('Ctrl Pts',(-5.761823405,3.459944422,-4.818743509));
#113997=CARTESIAN_POINT('Ctrl Pts',(-6.007833229,3.395197164,-4.489536712));
#113998=CARTESIAN_POINT('Ctrl Pts',(-5.12784488643437,3.52699760873882,
-5.12520928693362));
#113999=CARTESIAN_POINT('Ctrl Pts',(-5.13065658671719,3.52633876186941,
-5.12238995396681));
#114000=CARTESIAN_POINT('Ctrl Pts',(-5.133468287,3.525679915,-5.119570621));
#114001=CARTESIAN_POINT('Ctrl Pts',(-5.41400161399999,3.459944422,-4.83827575400001));
#114002=CARTESIAN_POINT('Ctrl Pts',(-5.66211978200001,3.395197164,-4.528012762));
#114003=CARTESIAN_POINT('',(-5.48131591317618,3.52567991457198,-5.11909912771447));
#114004=CARTESIAN_POINT('Origin',(0.126747988885264,3.62494886090853,0.140139977388261));
#114005=CARTESIAN_POINT('',(-5.30739209512788,3.52567991373765,-5.11933487856947));
#114006=CARTESIAN_POINT('Origin',(-1.0698907038087E-12,3.61749373600011,
-7.5764047813287E-13));
#114007=CARTESIAN_POINT('',(-5.85227096105507,3.61640598736084,-4.69051432075499));
#114008=CARTESIAN_POINT('Origin',(0.149372346596961,3.62499785970808,0.121499565334746));
#114009=CARTESIAN_POINT('Origin',(0.135121027998427,3.48215431755388,0.135768561324429));
#114010=CARTESIAN_POINT('Ctrl Pts',(-4.511847958,3.395189501,-5.991095726));
#114011=CARTESIAN_POINT('Ctrl Pts',(-4.83710930400001,3.460370723,-5.746143917));
#114012=CARTESIAN_POINT('Ctrl Pts',(-5.133939783,3.525679915,-5.467418248));
#114013=CARTESIAN_POINT('Ctrl Pts',(-4.549038082,3.395189501,-5.645241583));
#114014=CARTESIAN_POINT('Ctrl Pts',(-4.855522731,3.460370723,-5.398270692));
#114015=CARTESIAN_POINT('Ctrl Pts',(-5.133468287,3.525679915,-5.119570621));
#114016=CARTESIAN_POINT('',(-5.13393977442977,3.52567991637268,-5.46741825438338));
#114017=CARTESIAN_POINT('',(-5.1337040258707,3.52567991706892,-5.29349444335373));
#114018=CARTESIAN_POINT('',(-4.70834956261549,3.43511457319619,-5.83793149756705));
#114019=CARTESIAN_POINT('Origin',(0.126977794753728,3.48214118365086,0.1454274058658));
#114020=CARTESIAN_POINT('Ctrl Pts',(-4.5526858901545,3.39596551408124,-5.64230016839406));
#114021=CARTESIAN_POINT('Ctrl Pts',(-4.57855748562481,3.40280154627411,
-5.67488941720374));
#114022=CARTESIAN_POINT('Ctrl Pts',(-4.6044800535483,3.40947721887663,-5.70750257674678));
#114023=CARTESIAN_POINT('Ctrl Pts',(-4.65636102058536,3.42251694824849,
-5.7727017880457));
#114024=CARTESIAN_POINT('Ctrl Pts',(-4.6823475723423,3.42888807476058,-5.80532321301078));
#114025=CARTESIAN_POINT('Ctrl Pts',(-4.70834955866205,3.43511457408713,
-5.83793150054941));
#114026=CARTESIAN_POINT('Ctrl Pts',(-4.23007233058158,3.53021247063215,
-6.19396273343257));
#114027=CARTESIAN_POINT('Ctrl Pts',(-4.24174323385752,3.5279461928161,-6.18592743858956));
#114028=CARTESIAN_POINT('Ctrl Pts',(-4.25341413713345,3.525679915,-6.17789214374671));
#114029=CARTESIAN_POINT('Ctrl Pts',(-4.59193952671718,3.459944422,-5.94482095355766));
#114030=CARTESIAN_POINT('Ctrl Pts',(-4.9029716747628,3.395197164,-5.67615643917439));
#114031=CARTESIAN_POINT('Ctrl Pts',(-3.88983386413708,3.53021247063215,
-6.11820585342734));
#114032=CARTESIAN_POINT('Ctrl Pts',(-3.90136408256857,3.5279461928161,-6.1108138482137));
#114033=CARTESIAN_POINT('Ctrl Pts',(-3.912894301,3.525679915,-6.103421843));
#114034=CARTESIAN_POINT('Ctrl Pts',(-4.247338996,3.459944422,-5.889009866));
#114035=CARTESIAN_POINT('Ctrl Pts',(-4.556353671,3.395197164,-5.639338722));
#114036=CARTESIAN_POINT('',(-4.25271079329089,3.52567991457841,-6.17773833197232));
#114037=CARTESIAN_POINT('Origin',(0.0936588060901228,3.6249488395768,0.164110744318613));
#114038=CARTESIAN_POINT('',(-4.0828025445562,3.52567991373765,-6.14058008928441));
#114039=CARTESIAN_POINT('Origin',(5.87637577487143E-13,3.61749373599967,
5.98045918343004E-13));
#114040=CARTESIAN_POINT('',(-4.70712619026899,3.61640598741786,-5.83891796682443));
#114041=CARTESIAN_POINT('Origin',(0.119761026413497,3.62499782828964,0.150769287755076));
#114042=CARTESIAN_POINT('Origin',(0.102775544221599,3.48215432461251,0.161641131742404));
#114043=CARTESIAN_POINT('Ctrl Pts',(-3.118454975,3.395189501,-6.820941179));
#114044=CARTESIAN_POINT('Ctrl Pts',(-3.488769289,3.460370723,-6.651637782));
#114045=CARTESIAN_POINT('Ctrl Pts',(-3.838577816,3.525679915,-6.443238343));
#114046=CARTESIAN_POINT('Ctrl Pts',(-3.229124031,3.395189501,-6.491167691));
#114047=CARTESIAN_POINT('Ctrl Pts',(-3.581534681,3.460370723,-6.315855982));
#114048=CARTESIAN_POINT('Ctrl Pts',(-3.912894301,3.525679915,-6.103421843));
#114049=CARTESIAN_POINT('',(-3.83857780625908,3.52567991637269,-6.44323834739284));
#114050=CARTESIAN_POINT('',(-3.87573604768084,3.52567991706892,-6.2733300996842));
#114051=CARTESIAN_POINT('',(-3.34328826263611,3.43511457320309,-6.71359988169517));
#114052=CARTESIAN_POINT('Origin',(0.092746564593766,3.48214115952456,0.169323927841567));
#114053=CARTESIAN_POINT('Ctrl Pts',(-3.23331887271315,3.39596551408552,
-6.48907921575685));
#114054=CARTESIAN_POINT('Ctrl Pts',(-3.25157987957208,3.40280154624054,
-6.52646817421398));
#114055=CARTESIAN_POINT('Ctrl Pts',(-3.2698855272556,3.40947721889246,-6.56389144238755));
#114056=CARTESIAN_POINT('Ctrl Pts',(-3.30653764307364,3.42251694824908,
-6.63871920666186));
#114057=CARTESIAN_POINT('Ctrl Pts',(-3.32490400166039,3.42888807476787,
-6.67616430135315));
#114058=CARTESIAN_POINT('Ctrl Pts',(-3.3432882581064,3.43511457410804,-6.71359988376915));
#114059=CARTESIAN_POINT('Ctrl Pts',(-2.79965669493376,3.53021247058043,
-6.9584918377492));
#114060=CARTESIAN_POINT('Ctrl Pts',(-2.81278208969923,3.52794619279024,
-6.95315330291087));
#114061=CARTESIAN_POINT('Ctrl Pts',(-2.82590748446468,3.525679915,-6.94781476807245));
#114062=CARTESIAN_POINT('Ctrl Pts',(-3.20662175499411,3.459944422,-6.79296560482672));
#114063=CARTESIAN_POINT('Ctrl Pts',(-3.56813707398946,3.395197164,-6.59744503542102));
#114064=CARTESIAN_POINT('Ctrl Pts',(-2.48365830439741,3.53021247058043,
-6.81136489805072));
#114065=CARTESIAN_POINT('Ctrl Pts',(-2.49650801519868,3.52794619279024,
-6.80662437002537));
#114066=CARTESIAN_POINT('Ctrl Pts',(-2.509357726,3.525679915,-6.801883842));
#114067=CARTESIAN_POINT('Ctrl Pts',(-2.882075527,3.459944422,-6.664380422));
#114068=CARTESIAN_POINT('Ctrl Pts',(-3.237537527,3.395197164,-6.486975471));
#114069=CARTESIAN_POINT('',(-2.82525364939956,3.52567991457841,-6.94751335419762));
#114070=CARTESIAN_POINT('Origin',(0.0561901832822947,3.62494885801425,0.18040787680095));
#114071=CARTESIAN_POINT('',(-2.66730568478583,3.52567991373765,-6.87469859929902));
#114072=CARTESIAN_POINT('Origin',(2.77555756156289E-13,3.61749373600011,
4.81385764583564E-13));
#114073=CARTESIAN_POINT('',(-3.34188142941271,3.61640598742155,-6.71430029892485));
#114074=CARTESIAN_POINT('Origin',(0.084550252916929,3.62499779247149,0.172989665277615));
#114075=CARTESIAN_POINT('Origin',(0.0656247367693708,3.48215435022122,0.179955946192594));
#114076=CARTESIAN_POINT('Ctrl Pts',(-1.579246502,3.395189501,-7.331847004));
#114077=CARTESIAN_POINT('Ctrl Pts',(-1.9772983,3.460370723,-7.24610845700001));
#114078=CARTESIAN_POINT('Ctrl Pts',(-2.363728217,3.525679915,-7.117779774));
#114079=CARTESIAN_POINT('Ctrl Pts',(-1.75821973,3.395189501,-7.033574012));
#114080=CARTESIAN_POINT('Ctrl Pts',(-2.14007805,3.460370723,-6.938118866));
#114081=CARTESIAN_POINT('Ctrl Pts',(-2.509357726,3.525679915,-6.801883842));
#114082=CARTESIAN_POINT('',(-2.36372820654411,3.52567991637267,-7.11777977618988));
#114083=CARTESIAN_POINT('',(-2.43654295949688,3.52567991706892,-6.95983181220213));
#114084=CARTESIAN_POINT('',(-1.82189851888345,3.43511457319319,-7.2753477966558));
#114085=CARTESIAN_POINT('Origin',(0.0541785171027137,3.48214119170741,0.185302837168355));
#114086=CARTESIAN_POINT('Ctrl Pts',(-1.76276545876253,3.39596551404128,
-7.03243613129102));
#114087=CARTESIAN_POINT('Ctrl Pts',(-1.77256201256658,3.40280154620986,
-7.07287653324826));
#114088=CARTESIAN_POINT('Ctrl Pts',(-1.78239478793438,3.40947721887428,
-7.11336003930642));
#114089=CARTESIAN_POINT('Ctrl Pts',(-1.80210424016613,3.42251694823007,
-7.1943174933698));
#114090=CARTESIAN_POINT('Ctrl Pts',(-1.81199161497598,3.42888807474745,
-7.23483536672764));
#114091=CARTESIAN_POINT('Ctrl Pts',(-1.82189851405562,3.43511457407837,
-7.27534779770035));
#114092=CARTESIAN_POINT('Ctrl Pts',(-1.23833222316151,3.53021247064798,
-7.39764959851806));
#114093=CARTESIAN_POINT('Ctrl Pts',(-1.25229838088162,3.52794619282402,
-7.3952574474943));
#114094=CARTESIAN_POINT('Ctrl Pts',(-1.26626453860173,3.525679915,-7.3928652964705));
#114095=CARTESIAN_POINT('Ctrl Pts',(-1.67136591378173,3.459944422,-7.32347873441115));
#114096=CARTESIAN_POINT('Ctrl Pts',(-2.06646034810027,3.395197164,-7.21024443357577));
#114097=CARTESIAN_POINT('Ctrl Pts',(-0.961349642372511,3.53021247064798,
-7.18603209133051));
#114098=CARTESIAN_POINT('Ctrl Pts',(-0.974918007686249,3.52794619282402,
-7.18416470216521));
#114099=CARTESIAN_POINT('Ctrl Pts',(-0.988486373,3.525679915,-7.182297313));
#114100=CARTESIAN_POINT('Ctrl Pts',(-1.38204941,3.459944422,-7.128131956));
#114101=CARTESIAN_POINT('Ctrl Pts',(-1.767337726,3.395197164,-7.031288457));
#114102=CARTESIAN_POINT('',(-1.26569078444363,3.52567991503086,-7.39243037450837));
#114103=CARTESIAN_POINT('Origin',(0.016094124521488,3.62494885332331,0.188269188525618));
#114104=CARTESIAN_POINT('',(-1.12708857585279,3.52567991373765,-7.28736384418274));
#114105=CARTESIAN_POINT('Origin',(-1.69677639993981E-13,3.61749373599967,
-5.16947595841089E-13));
#114106=CARTESIAN_POINT('',(-1.82037400765982,3.61640598742735,-7.27572941129027));
#114107=CARTESIAN_POINT('Origin',(0.0453858973627483,3.62499779203663,0.187121226497711));
#114108=CARTESIAN_POINT('Origin',(0.0254052502516719,3.48215431679144,0.189856002383667));
#114109=CARTESIAN_POINT('Ctrl Pts',(0.033805781,3.395189501,-7.499923811));
#114110=CARTESIAN_POINT('Ctrl Pts',(-0.373371039,3.460370723,-7.501759154));
#114111=CARTESIAN_POINT('Ctrl Pts',(-0.778353314,3.525679915,-7.459501734));
#114112=CARTESIAN_POINT('Ctrl Pts',(-0.205103028,3.395189501,-7.247098229));
#114113=CARTESIAN_POINT('Ctrl Pts',(-0.598553747,3.460370723,-7.23596302300001));
#114114=CARTESIAN_POINT('Ctrl Pts',(-0.988486373,3.525679915,-7.182297313));
#114115=CARTESIAN_POINT('',(-0.883419830874176,3.52567991706892,-7.32089952502357));
#114116=CARTESIAN_POINT('Ctrl Pts',(-0.20978709063981,3.39596551406428,
-7.24696414900821));
#114117=CARTESIAN_POINT('Ctrl Pts',(-0.210661115511315,3.40280154621224,
-7.28856504635459));
#114118=CARTESIAN_POINT('Ctrl Pts',(-0.211561248997317,3.40947721886393,
-7.33021582659437));
#114119=CARTESIAN_POINT('Ctrl Pts',(-0.213406445784567,3.42251694821776,
-7.41351749006351));
#114120=CARTESIAN_POINT('Ctrl Pts',(-0.214352514266222,3.42888807473786,
-7.45521357138656));
#114121=CARTESIAN_POINT('Ctrl Pts',(-0.215318820514567,3.43511457407938,
-7.4969085347325));
#114122=CARTESIAN_POINT('Ctrl Pts',(0.361283325361629,3.52699760873882,
-7.49129776665977));
#114123=CARTESIAN_POINT('Ctrl Pts',(0.357168844680815,3.52633876186941,
-7.49149166632988));
#114124=CARTESIAN_POINT('Ctrl Pts',(0.353054364,3.525679915,-7.491685566));
#114125=CARTESIAN_POINT('Ctrl Pts',(-0.057461992,3.459944422,-7.511031625));
#114126=CARTESIAN_POINT('Ctrl Pts',(-0.467634306,3.395197164,-7.48540701300001));
#114127=CARTESIAN_POINT('Ctrl Pts',(0.586543593611081,3.52699760873882,
-7.22623899646124));
#114128=CARTESIAN_POINT('Ctrl Pts',(0.582574548805541,3.52633876186941,
-7.22655677023062));
#114129=CARTESIAN_POINT('Ctrl Pts',(0.578605504,3.525679915,-7.226874544));
#114130=CARTESIAN_POINT('Ctrl Pts',(0.182599802,3.459944422,-7.258579962));
#114131=CARTESIAN_POINT('Ctrl Pts',(-0.214499177,3.395197164,-7.246826209));
#114132=CARTESIAN_POINT('',(0.46582994172268,3.52567991373765,-7.35928005451117));
#114133=CARTESIAN_POINT('Ctrl Pts',(1.645277344,3.395189501,-7.317312516));
#114134=CARTESIAN_POINT('Ctrl Pts',(1.248014636,3.460370723,-7.40663593));
#114135=CARTESIAN_POINT('Ctrl Pts',(0.843416526,3.525679915,-7.45242568300001));
#114136=CARTESIAN_POINT('Ctrl Pts',(1.357604063,3.395189501,-7.121756188));
#114137=CARTESIAN_POINT('Ctrl Pts',(0.970958263,3.460370723,-7.195461591));
#114138=CARTESIAN_POINT('Ctrl Pts',(0.578605504000001,3.525679915,-7.226874544));
#114139=CARTESIAN_POINT('',(0.843416536403176,3.52567991637269,-7.45242568060099));
#114140=CARTESIAN_POINT('',(0.711011027658161,3.52567991706892,-7.33965011227377));
#114141=CARTESIAN_POINT('',(1.40132893743346,3.43511457320505,-7.36792216210267));
#114142=CARTESIAN_POINT('Origin',(-0.0286356026579147,3.48214115263802,
0.190925565646907));
#114143=CARTESIAN_POINT('Ctrl Pts',(1.35300068819012,3.39596551399878,-7.12263217758401));
#114144=CARTESIAN_POINT('Ctrl Pts',(1.36109001433851,3.40280150691475,-7.16344812417094));
#114145=CARTESIAN_POINT('Ctrl Pts',(1.36916456012132,3.40947713912844,-7.2043183690547));
#114146=CARTESIAN_POINT('Ctrl Pts',(1.38526999695604,3.42251694824015,-7.28606964857968));
#114147=CARTESIAN_POINT('Ctrl Pts',(1.39330947210524,3.42888807476758,-7.32699427545928));
#114148=CARTESIAN_POINT('Ctrl Pts',(1.40132894230255,3.43511457411378,-7.36792216101036));
#114149=CARTESIAN_POINT('Ctrl Pts',(1.96324430040488,3.52699760873882,-7.23849015173953));
#114150=CARTESIAN_POINT('Ctrl Pts',(1.95926769670244,3.52633876186941,-7.23956400986976));
#114151=CARTESIAN_POINT('Ctrl Pts',(1.955291093,3.525679915,-7.240637868));
#114152=CARTESIAN_POINT('Ctrl Pts',(1.558531213,3.459944422,-7.34778050900001));
#114153=CARTESIAN_POINT('Ctrl Pts',(1.152439965,3.395197164,-7.41092991));
#114154=CARTESIAN_POINT('Ctrl Pts',(2.12625830857137,3.52699760873882,-6.93120400959201));
#114155=CARTESIAN_POINT('Ctrl Pts',(2.12245036978568,3.52633876186941,-6.93236758129601));
#114156=CARTESIAN_POINT('Ctrl Pts',(2.118642431,3.525679915,-6.933531153));
#114157=CARTESIAN_POINT('Ctrl Pts',(1.738710849,3.459944422,-7.049624836));
#114158=CARTESIAN_POINT('Ctrl Pts',(1.348369115,3.395197164,-7.123510422));
#114159=CARTESIAN_POINT('',(1.95529109576274,3.52567991457198,-7.24063786855863));
#114160=CARTESIAN_POINT('Origin',(-0.0644455688419812,3.62494888378541,
0.177626244271242));
#114161=CARTESIAN_POINT('',(2.03696676943704,3.52567991373765,-7.08708450836245));
#114162=CARTESIAN_POINT('Origin',(-4.66206934168767E-14,3.61749373599911,
-4.90059381963448E-14));
#114163=CARTESIAN_POINT('',(1.40287278194271,3.61640598739338,-7.36762838021731));
#114164=CARTESIAN_POINT('Origin',(-0.0373790373297064,3.62499777786392,
0.18888364588575));
#114165=CARTESIAN_POINT('Origin',(-0.056661309098946,3.48215429044633,0.182976075754221));
#114166=CARTESIAN_POINT('Ctrl Pts',(3.179817567,3.395189501,-6.792551821));
#114167=CARTESIAN_POINT('Ctrl Pts',(2.811044533,3.460370723,-6.965186642));
#114168=CARTESIAN_POINT('Ctrl Pts',(2.425749146,3.525679915,-7.09688249));
#114169=CARTESIAN_POINT('Ctrl Pts',(2.856831098,3.395189501,-6.663408743));
#114170=CARTESIAN_POINT('Ctrl Pts',(2.495069344,3.460370723,-6.818508373));
#114171=CARTESIAN_POINT('Ctrl Pts',(2.118642431,3.525679915,-6.933531153));
#114172=CARTESIAN_POINT('',(2.4257491556452,3.52567991637267,-7.09688248541667));
#114173=CARTESIAN_POINT('',(2.27219580059861,3.52567991706892,-7.01520681758131));
#114174=CARTESIAN_POINT('',(2.95245211611529,3.43511457319795,-6.89441993772619));
#114175=CARTESIAN_POINT('Origin',(-0.0690095232738826,3.48214119981529,
0.180306178259331));
#114176=CARTESIAN_POINT('Ctrl Pts',(2.85252365852958,3.39596551411236,-6.66525384212721));
#114177=CARTESIAN_POINT('Ctrl Pts',(2.8691981784591,3.40280154625929,-6.70337678750105));
#114178=CARTESIAN_POINT('Ctrl Pts',(2.88586994819414,3.40947721890447,-6.74155596804241));
#114179=CARTESIAN_POINT('Ctrl Pts',(2.9191727537913,3.42251694824652,-6.81793328812538));
#114180=CARTESIAN_POINT('Ctrl Pts',(2.93582185555585,3.42888807475833,-6.8561728703922));
#114181=CARTESIAN_POINT('Ctrl Pts',(2.95245212060851,3.43511457409255,-6.89441993562685));
#114182=CARTESIAN_POINT('Ctrl Pts',(3.47340615432972,3.52699760873882,-6.64721878366841));
#114183=CARTESIAN_POINT('Ctrl Pts',(3.46975336916486,3.52633876186941,-6.6491223878342));
#114184=CARTESIAN_POINT('Ctrl Pts',(3.466100584,3.525679915,-6.651025992));
#114185=CARTESIAN_POINT('Ctrl Pts',(3.10164923,3.459944422,-6.84095534300001));
#114186=CARTESIAN_POINT('Ctrl Pts',(2.718627424,3.395197164,-6.98992596));
#114187=CARTESIAN_POINT('Ctrl Pts',(3.566551547531,3.52699760873882,-6.31207362737036));
#114188=CARTESIAN_POINT('Ctrl Pts',(3.5630827697655,3.52633876186941,-6.31402858968518));
#114189=CARTESIAN_POINT('Ctrl Pts',(3.559613992,3.525679915,-6.315983552));
#114190=CARTESIAN_POINT('Ctrl Pts',(3.21352171,3.459944422,-6.511037088));
#114191=CARTESIAN_POINT('Ctrl Pts',(2.848189165,3.395197164,-6.667107205));
#114192=CARTESIAN_POINT('',(3.46610058684643,3.52567991457198,-6.65102599192097));
#114193=CARTESIAN_POINT('Origin',(-0.101123261420778,3.62494888976623,0.159619578785367));
#114194=CARTESIAN_POINT('',(3.51285729480366,3.52567991373765,-6.48350476831368));
#114195=CARTESIAN_POINT('Origin',(1.26634813746307E-13,3.61749373600033,
-2.15105711021124E-13));
#114196=CARTESIAN_POINT('',(2.95389671194755,3.61640598740987,-6.89380114360488));
#114197=CARTESIAN_POINT('Origin',(-0.0771095214129497,3.62499779838487,
0.176432218884227));
#114198=CARTESIAN_POINT('Origin',(-0.0946710417999042,3.48215430175332,
0.166517704383047));
#114199=CARTESIAN_POINT('Ctrl Pts',(4.565673054,3.395189501,-5.950178952));
#114200=CARTESIAN_POINT('Ctrl Pts',(4.242633113,3.460370723,-6.198052969));
#114201=CARTESIAN_POINT('Ctrl Pts',(3.894656432,3.525679915,-6.40949696));
#114202=CARTESIAN_POINT('Ctrl Pts',(4.222475885,3.395189501,-5.893487711));
#114203=CARTESIAN_POINT('Ctrl Pts',(3.902513756,3.460370723,-6.122729281));
#114204=CARTESIAN_POINT('Ctrl Pts',(3.559613992,3.525679915,-6.315983552));
#114205=CARTESIAN_POINT('',(3.8946564404075,3.52567991637268,-6.40949695345765));
#114206=CARTESIAN_POINT('',(3.72713522297332,3.52567991706892,-6.3627402495721));
#114207=CARTESIAN_POINT('',(4.36552191505787,3.43511457318807,-6.09854229996074));
#114208=CARTESIAN_POINT('Origin',(-0.106156408365024,3.48214118529408,0.161255378447459));
#114209=CARTESIAN_POINT('Ctrl Pts',(4.21866579300694,3.39596551405285,-5.89621564465874));
#114210=CARTESIAN_POINT('Ctrl Pts',(4.24314564013628,3.40280150761502,-5.92986257788553));
#114211=CARTESIAN_POINT('Ctrl Pts',(4.26763487249922,3.40947714050253,-5.96356499748966));
#114212=CARTESIAN_POINT('Ctrl Pts',(4.31657823714961,3.42251694821273,-6.03099794479326));
#114213=CARTESIAN_POINT('Ctrl Pts',(4.34105847192057,3.42888807472854,-6.06476444220809));
#114214=CARTESIAN_POINT('Ctrl Pts',(4.36552191896387,3.43511457406307,-6.09854229697054));
#114215=CARTESIAN_POINT('Ctrl Pts',(4.82115539691061,3.52699760873882,-5.74513085140018));
#114216=CARTESIAN_POINT('Ctrl Pts',(4.8179972304553,3.52633876186941,-5.74777519120009));
#114217=CARTESIAN_POINT('Ctrl Pts',(4.814839064,3.525679915,-5.750419531));
#114218=CARTESIAN_POINT('Ctrl Pts',(4.499737576,3.459944422,-6.01425470800001));
#114219=CARTESIAN_POINT('Ctrl Pts',(4.157694886,3.395197164,-6.242080842));
#114220=CARTESIAN_POINT('Ctrl Pts',(4.84007680111362,3.52699760873882,-5.39779769684762));
#114221=CARTESIAN_POINT('Ctrl Pts',(4.83710938055682,3.52633876186941,-5.40045263792381));
#114222=CARTESIAN_POINT('Ctrl Pts',(4.83414196,3.525679915,-5.403107579));
#114223=CARTESIAN_POINT('Ctrl Pts',(4.538071868,3.459944422,-5.668000483));
#114224=CARTESIAN_POINT('Ctrl Pts',(4.214831056,3.395197164,-5.898957465));
#114225=CARTESIAN_POINT('',(4.81483906674359,3.52567991457198,-5.75041953034411));
#114226=CARTESIAN_POINT('Origin',(-0.133072610412248,3.62494889177638,0.134149317188565));
#114227=CARTESIAN_POINT('',(4.82449051785211,3.52567991373766,-5.57676354993731));
#114228=CARTESIAN_POINT('Origin',(-1.58944038486375E-13,3.61749373599945,
2.90132501357121E-13));
#114229=CARTESIAN_POINT('',(4.36679971533011,3.61640598740656,-6.09762742744872));
#114230=CARTESIAN_POINT('Origin',(-0.113234348334703,3.62499780122883,0.155730897777955));
#114231=CARTESIAN_POINT('Origin',(-0.128254040349813,3.48215433246544,0.14227308511448));
#114232=CARTESIAN_POINT('Ctrl Pts',(5.738042744,3.395189501,-4.829582328));
#114233=CARTESIAN_POINT('Ctrl Pts',(5.475840884,3.460370723,-5.141105227));
#114234=CARTESIAN_POINT('Ctrl Pts',(5.181453912,3.525679915,-5.422410475));
#114235=CARTESIAN_POINT('Ctrl Pts',(5.390682393,3.395189501,-4.847993744));
#114236=CARTESIAN_POINT('Ctrl Pts',(5.127480962,3.460370723,-5.140658173));
#114237=CARTESIAN_POINT('Ctrl Pts',(4.83414196,3.525679915,-5.403107579));
#114238=CARTESIAN_POINT('',(5.18145391881129,3.52567991637267,-5.42241046679963));
#114239=CARTESIAN_POINT('',(5.00779794533496,3.52567991706892,-5.41275901836345));
#114240=CARTESIAN_POINT('',(5.57446476168392,3.4351145731887,-5.01750360199659));
#114241=CARTESIAN_POINT('Origin',(-0.138339562021414,3.48214118888366,0.134664725891545));
#114242=CARTESIAN_POINT('Ctrl Pts',(5.38754780344265,3.39596551400055,-4.85147695703864));
#114243=CARTESIAN_POINT('Ctrl Pts',(5.41868842773454,3.40280150893663,-4.87907480553435));
#114244=CARTESIAN_POINT('Ctrl Pts',(5.44985014661251,3.40947714325031,-4.90672482643989));
#114245=CARTESIAN_POINT('Ctrl Pts',(5.51214531987703,3.42251694820028,-4.96205984035383));
#114246=CARTESIAN_POINT('Ctrl Pts',(5.54331201925207,3.42888807472423,-4.98977436894406));
#114247=CARTESIAN_POINT('Ctrl Pts',(5.57446476485727,3.43511457406497,-5.0175035982347));
#114248=CARTESIAN_POINT('Ctrl Pts',(5.9558672539275,3.53021247061354,-4.5592029476204));
#114249=CARTESIAN_POINT('Ctrl Pts',(5.94721189361869,3.52794619280679,-4.57042171235928));
#114250=CARTESIAN_POINT('Ctrl Pts',(5.93855653331001,3.525679915,-4.58164047709804));
#114251=CARTESIAN_POINT('Ctrl Pts',(5.68749976732975,3.459944422,-4.90705116979723));
#114252=CARTESIAN_POINT('Ctrl Pts',(5.4023903318827,3.395197164,-5.2030819588396));
#114253=CARTESIAN_POINT('Ctrl Pts',(5.89864161721082,3.53021247061353,-4.21536207557745));
#114254=CARTESIAN_POINT('Ctrl Pts',(5.89063621960535,3.5279461928068,-4.22647518878876));
#114255=CARTESIAN_POINT('Ctrl Pts',(5.882630822,3.525679915,-4.237588302));
#114256=CARTESIAN_POINT('Ctrl Pts',(5.650426828,3.459944422,-4.559934474));
#114257=CARTESIAN_POINT('Ctrl Pts',(5.384392131,3.395197164,-4.85497903));
#114258=CARTESIAN_POINT('',(5.93844102538326,3.52567991457841,-4.5809298375767));
#114259=CARTESIAN_POINT('Origin',(-0.158799496831515,3.62494884927284,0.102406236496948));
#114260=CARTESIAN_POINT('',(5.91053592562699,3.52567991373765,-4.40925906729761));
#114261=CARTESIAN_POINT('Origin',(2.00794242344315E-13,3.617493736,-2.71050543121376E-13));
#114262=CARTESIAN_POINT('',(5.57551601667305,3.61640598737761,-5.01633542971883));
#114263=CARTESIAN_POINT('Origin',(-0.144064587206557,3.62499782023102,0.127748007484126));
#114264=CARTESIAN_POINT('Origin',(-0.155839937661904,3.48215431455712,0.111375903320868));
#114265=CARTESIAN_POINT('Ctrl Pts',(6.642107933,3.395189501,-3.483159803));
#114266=CARTESIAN_POINT('Ctrl Pts',(6.45300442,3.460370723,-3.843765118));
#114267=CARTESIAN_POINT('Ctrl Pts',(6.225972366,3.525679915,-4.181778103));
#114268=CARTESIAN_POINT('Ctrl Pts',(6.306826583,3.395189501,-3.575812977));
#114269=CARTESIAN_POINT('Ctrl Pts',(6.112692857,3.460370723,-3.918215602));
#114270=CARTESIAN_POINT('Ctrl Pts',(5.882630822,3.525679915,-4.237588302));
#114271=CARTESIAN_POINT('',(6.22597237087733,3.52567991637267,-4.1817780935345));
#114272=CARTESIAN_POINT('',(6.05430160126011,3.52567991706892,-4.20968319205863));
#114273=CARTESIAN_POINT('',(6.52275183160806,3.43511457319251,-3.7018520124256));
#114274=CARTESIAN_POINT('Origin',(-0.164054713654601,3.48214119996662,0.101777745563075));
#114275=CARTESIAN_POINT('Ctrl Pts',(6.304514067401,3.39596551400235,-3.57988859824468));
#114276=CARTESIAN_POINT('Ctrl Pts',(6.34085934616121,3.40280150582777,-3.60014690173996));
#114277=CARTESIAN_POINT('Ctrl Pts',(6.37723643965595,3.40947713692085,-3.62045162175645));
#114278=CARTESIAN_POINT('Ctrl Pts',(6.44997061389297,3.42251694820707,-3.66110133292935));
#114279=CARTESIAN_POINT('Ctrl Pts',(6.4863664575326,3.42888807473104,-3.68146799218158));
#114280=CARTESIAN_POINT('Ctrl Pts',(6.52275183390539,3.4351145740766,-3.70185200805483));
#114281=CARTESIAN_POINT('Ctrl Pts',(6.79671625250398,3.5302124705803,-3.17227591142549));
#114282=CARTESIAN_POINT('Ctrl Pts',(6.79067495253319,3.52794619279017,-3.18509303418759));
#114283=CARTESIAN_POINT('Ctrl Pts',(6.78463365256231,3.525679915,-3.19791015694976));
#114284=CARTESIAN_POINT('Ctrl Pts',(6.60940013367513,3.459944422,-3.56968271160645));
#114285=CARTESIAN_POINT('Ctrl Pts',(6.39459426724533,3.395197164,-3.9200825665283));
#114286=CARTESIAN_POINT('Ctrl Pts',(6.66691289494691,3.5302124705803,-2.84877566785109));
#114287=CARTESIAN_POINT('Ctrl Pts',(6.66148364997345,3.52794619279017,-2.86134988642553));
#114288=CARTESIAN_POINT('Ctrl Pts',(6.656054405,3.525679915,-2.873924105));
#114289=CARTESIAN_POINT('Ctrl Pts',(6.49857411,3.459944422,-3.238650998));
#114290=CARTESIAN_POINT('Ctrl Pts',(6.302185015,3.395197164,-3.583987171));
#114291=CARTESIAN_POINT('',(6.78436807904918,3.52567991503086,-3.19724096221395));
#114292=CARTESIAN_POINT('Origin',(-0.177101252742581,3.62494886858678,0.065874886723139));
#114293=CARTESIAN_POINT('',(6.72021124318548,3.52567991373765,-3.03558253094795));
#114294=CARTESIAN_POINT('Origin',(1.63410951437015E-12,3.61749373599922,
-9.50411624400793E-13));
#114295=CARTESIAN_POINT('',(6.52352738588612,3.61640598738353,-3.70048516261255));
#114296=CARTESIAN_POINT('Origin',(-0.168158374720755,3.62499780471484,0.0937916323317745));
#114297=CARTESIAN_POINT('Origin',(-0.176139459378517,3.4821543088949,0.0752712603977301));
#114298=CARTESIAN_POINT('Ctrl Pts',(7.235595536,3.395189501,-1.973868596));
#114299=CARTESIAN_POINT('Ctrl Pts',(7.128432643,3.460370723,-2.366694825));
#114300=CARTESIAN_POINT('Ctrl Pts',(6.979371271,3.525679915,-2.745610435));
#114301=CARTESIAN_POINT('Ctrl Pts',(6.928070572,3.395189501,-2.13643117));
#114302=CARTESIAN_POINT('Ctrl Pts',(6.812082027,3.460370723,-2.512561624));
#114303=CARTESIAN_POINT('Ctrl Pts',(6.656054405,3.525679915,-2.873924105));
#114304=CARTESIAN_POINT('',(6.97937127374582,3.52567991637268,-2.74561042469145));
#114305=CARTESIAN_POINT('',(6.81771284284578,3.52567991706892,-2.80976725824203));
#114306=CARTESIAN_POINT('',(7.16604227526424,3.43511457319985,-2.21310593709546));
#114307=CARTESIAN_POINT('Origin',(-0.182097970521191,3.48214116801236,0.0641311704411699));
#114308=CARTESIAN_POINT('Ctrl Pts',(6.9266882594647,3.39596551400351,-2.1409086281669));
#114309=CARTESIAN_POINT('Ctrl Pts',(6.9665387446434,3.40280150624475,-2.15288014373984));
#114310=CARTESIAN_POINT('Ctrl Pts',(7.00643027926497,3.40947713776356,-2.16489015161554));
#114311=CARTESIAN_POINT('Ctrl Pts',(7.0862024503661,3.42251694823578,-2.1889537961222));
#114312=CARTESIAN_POINT('Ctrl Pts',(7.12612560918764,3.4288880747598,-2.20102026370945));
#114313=CARTESIAN_POINT('Ctrl Pts',(7.16604227657517,3.4351145740985,-2.21310593230273));
#114314=CARTESIAN_POINT('Ctrl Pts',(7.31975835219288,3.53021247065002,-1.63701677804991));
#114315=CARTESIAN_POINT('Ctrl Pts',(7.31661359695517,3.52794619282504,-1.65083294474948));
#114316=CARTESIAN_POINT('Ctrl Pts',(7.31346884171736,3.525679915,-1.66464911144911));
#114317=CARTESIAN_POINT('Ctrl Pts',(7.22225229552072,3.459944422,-2.06539985760202));
#114318=CARTESIAN_POINT('Ctrl Pts',(7.08779408178921,3.395197164,-2.45378447035253));
#114319=CARTESIAN_POINT('Ctrl Pts',(7.12344673599801,3.53021247065002,-1.34898367557698));
#114320=CARTESIAN_POINT('Ctrl Pts',(7.12084750899901,3.52794619282504,-1.3624310432885));
#114321=CARTESIAN_POINT('Ctrl Pts',(7.118248282,3.525679915,-1.375878411));
#114322=CARTESIAN_POINT('Ctrl Pts',(7.04285528900001,3.459944422,-1.7659318));
#114323=CARTESIAN_POINT('Ctrl Pts',(6.925294731,3.395197164,-2.145412056));
#114324=CARTESIAN_POINT('',(7.31306561976193,3.52567991457841,-1.66405265299233));
#114325=CARTESIAN_POINT('Origin',(-0.187121738364304,3.62494885490083,0.0262631901970392));
#114326=CARTESIAN_POINT('',(7.21565695159502,3.52567991373765,-1.51996552892804));
#114327=CARTESIAN_POINT('Origin',(8.30065183254902E-13,3.61749373599978,
-2.65737952476197E-13));
#114328=CARTESIAN_POINT('',(7.16650586494504,3.6164059874119,-2.21160432283927));
#114329=CARTESIAN_POINT('Origin',(-0.184389231530323,3.62499784037748,0.0554497127867537));
#114330=CARTESIAN_POINT('Origin',(-0.188202325549108,3.48215429683246,0.035646622946475));
#114331=CARTESIAN_POINT('Ctrl Pts',(7.490754735,3.395189501,-0.372281487));
#114332=CARTESIAN_POINT('Ctrl Pts',(7.470543277,3.460370723,-0.778960512000001));
#114333=CARTESIAN_POINT('Ctrl Pts',(7.406422533,3.525679915,-1.181061074));
#114334=CARTESIAN_POINT('Ctrl Pts',(7.225365682,3.395189501,-0.597152216));
#114335=CARTESIAN_POINT('Ctrl Pts',(7.192945813,3.460370723,-0.989423057));
#114336=CARTESIAN_POINT('Ctrl Pts',(7.118248282,3.525679915,-1.375878411));
#114337=CARTESIAN_POINT('',(7.40642253346363,3.52567991637266,-1.18106106333763));
#114338=CARTESIAN_POINT('',(7.26233540970488,3.52567991706892,-1.27846972997522));
#114339=CARTESIAN_POINT('',(7.47425654613115,3.43511457318359,-0.620877487542569));
#114340=CARTESIAN_POINT('Origin',(-0.191626976407847,3.48214120369069,0.0234861444890657));
#114341=CARTESIAN_POINT('Ctrl Pts',(7.22497820779554,3.3959655139285,-0.601822150021933));
#114342=CARTESIAN_POINT('Ctrl Pts',(7.26647055793215,3.40280151035648,-0.604947103677359));
#114343=CARTESIAN_POINT('Ctrl Pts',(7.30801127578618,3.4094771461764,-0.60810082564552));
#114344=CARTESIAN_POINT('Ctrl Pts',(7.39109133582747,3.42251694818263,-0.614453212584922));
#114345=CARTESIAN_POINT('Ctrl Pts',(7.43267504712686,3.42888807471259,-0.617655273833398));
#114346=CARTESIAN_POINT('Ctrl Pts',(7.47425654638066,3.4351145740495,-0.620877482649554));
#114347=CARTESIAN_POINT('Ctrl Pts',(7.50053668693811,3.53021247056292,-0.0252125605125761));
#114348=CARTESIAN_POINT('Ctrl Pts',(7.50043552175035,3.52794619278149,-0.0393817420581123));
#114349=CARTESIAN_POINT('Ctrl Pts',(7.50033435656256,3.525679915,-0.0535509236036477));
#114350=CARTESIAN_POINT('Ctrl Pts',(7.49739996628298,3.459944422,-0.464541201103576));
#114351=CARTESIAN_POINT('Ctrl Pts',(7.44957652221862,3.395197164,-0.872750138705848));
#114352=CARTESIAN_POINT('Ctrl Pts',(7.24689612386501,3.53021247056292,0.213885293912943));
#114353=CARTESIAN_POINT('Ctrl Pts',(7.24724845193251,3.52794619278149,0.200193561456469));
#114354=CARTESIAN_POINT('Ctrl Pts',(7.24760078,3.525679915,0.186501829));
#114355=CARTESIAN_POINT('Ctrl Pts',(7.257820383,3.459944422,-0.210639594));
#114356=CARTESIAN_POINT('Ctrl Pts',(7.224585363,3.395197164,-0.606519857));
#114357=CARTESIAN_POINT('',(7.49981234078918,3.52567991457841,-0.0530550908287365));
#114358=CARTESIAN_POINT('Origin',(-0.188392868196582,3.62494885611011,-0.0145764597221847));
#114359=CARTESIAN_POINT('',(7.37370656042998,3.52567991373765,0.0667233722378182));
#114360=CARTESIAN_POINT('Origin',(-1.69569219776733E-13,3.61749373600011,
4.07626135536659E-14));
#114361=CARTESIAN_POINT('',(7.47438649539288,3.61640598739424,-0.619311321310272));
#114362=CARTESIAN_POINT('Origin',(-0.191998517910724,3.62499782284084,0.0145151197861249));
#114363=CARTESIAN_POINT('Origin',(-0.191465174249291,3.48215433943968,-0.00564471087924709));
#114364=CARTESIAN_POINT('Ctrl Pts',(7.395654567,3.395189501,1.24671309));
#114365=CARTESIAN_POINT('Ctrl Pts',(7.463339611,3.460370723,0.845197129));
#114366=CARTESIAN_POINT('Ctrl Pts',(7.487157709,3.525679915,0.43871339));
#114367=CARTESIAN_POINT('Ctrl Pts',(7.184810722,3.395189501,0.970048913));
#114368=CARTESIAN_POINT('Ctrl Pts',(7.23747544800001,3.460370723,0.579979832));
#114369=CARTESIAN_POINT('Ctrl Pts',(7.24760078,3.525679915,0.186501829));
#114370=CARTESIAN_POINT('',(7.4871577071628,3.52567991637267,0.438713400513138));
#114371=CARTESIAN_POINT('',(7.36737924396087,3.52567991706892,0.312607622205938));
#114372=CARTESIAN_POINT('',(7.43298288901529,3.43511457321003,1.00038250308341));
#114373=CARTESIAN_POINT('Origin',(-0.192195783444843,3.4821411629602,-0.0182570933746986));
#114374=CARTESIAN_POINT('Ctrl Pts',(7.18543620474245,3.39596551404374,0.965404863421029));
#114375=CARTESIAN_POINT('Ctrl Pts',(7.22663047529356,3.40280154623927,0.971272628899141));
#114376=CARTESIAN_POINT('Ctrl Pts',(7.26787819499172,3.40947721884971,0.977122699753423));
#114377=CARTESIAN_POINT('Ctrl Pts',(7.3503810057172,3.4225169482536,0.988778520276736));
#114378=CARTESIAN_POINT('Ctrl Pts',(7.39168086152302,3.42888807478171,0.994590590171426));
#114379=CARTESIAN_POINT('Ctrl Pts',(7.43298288818389,3.43511457412893,1.00038250802431));
#114380=CARTESIAN_POINT('Ctrl Pts',(7.33416218652337,3.52699760873882,1.56848107737335));
#114381=CARTESIAN_POINT('Ctrl Pts',(7.33501918076169,3.52633876186941,1.56445216818668));
#114382=CARTESIAN_POINT('Ctrl Pts',(7.335876175,3.525679915,1.560423259));
#114383=CARTESIAN_POINT('Ctrl Pts',(7.421381535,3.459944422,1.158444675));
#114384=CARTESIAN_POINT('Ctrl Pts',(7.462452985,3.395197164,0.749530155));
#114385=CARTESIAN_POINT('Ctrl Pts',(7.03615210583643,3.52699760873882,1.74789214721709));
#114386=CARTESIAN_POINT('Ctrl Pts',(7.03710781341822,3.52633876186941,1.74402679860854));
#114387=CARTESIAN_POINT('Ctrl Pts',(7.038063521,3.525679915,1.74016145));
#114388=CARTESIAN_POINT('Ctrl Pts',(7.133417862,3.459944422,1.354501886));
#114389=CARTESIAN_POINT('Ctrl Pts',(7.18606241200001,3.395197164,0.960732536));
#114390=CARTESIAN_POINT('',(7.33587617569046,3.52567991457198,1.56042326175562));
#114391=CARTESIAN_POINT('Origin',(-0.180854831178093,3.62494886848255,-0.0547345692229878));
#114392=CARTESIAN_POINT('',(7.18696984626822,3.52567991373765,1.65029236204186));
#114393=CARTESIAN_POINT('Origin',(4.76615275024628E-13,3.617493735999,8.23993651088983E-14));
#114394=CARTESIAN_POINT('',(7.43277311984018,3.61640598738135,1.00193998853182));
#114395=CARTESIAN_POINT('Origin',(-0.190630119290141,3.62499783977117,-0.0270982572358046));
#114396=CARTESIAN_POINT('Origin',(-0.185775199275259,3.48215434388086,-0.0466720506929474));
#114397=CARTESIAN_POINT('Ctrl Pts',(6.954741811,3.395189501,2.807412748));
#114398=CARTESIAN_POINT('Ctrl Pts',(7.107158479,3.460370723,2.429834291));
#114399=CARTESIAN_POINT('Ctrl Pts',(7.21780171200001,3.525679915,2.037974103));
#114400=CARTESIAN_POINT('Ctrl Pts',(6.808301998,3.395189501,2.491891632));
#114401=CARTESIAN_POINT('Ctrl Pts',(6.943588774,3.460370723,2.122263509));
#114402=CARTESIAN_POINT('Ctrl Pts',(7.038063521,3.525679915,1.74016145));
#114403=CARTESIAN_POINT('',(7.21780170794649,3.52567991637268,2.03797411287136));
#114404=CARTESIAN_POINT('',(7.12793261324207,3.52567991706892,1.88906778879299));
#114405=CARTESIAN_POINT('',(7.04415121226113,3.43511457319547,2.5748657198136));
#114406=CARTESIAN_POINT('Origin',(-0.18377778965417,3.48214119424527,-0.0591467200203382));
#114407=CARTESIAN_POINT('Ctrl Pts',(6.80991119058296,3.39596551402597,2.48749061798307));
#114408=CARTESIAN_POINT('Ctrl Pts',(6.84888096577829,3.40280154620957,2.50207674882005));
#114409=CARTESIAN_POINT('Ctrl Pts',(6.88790674453291,3.40947721884071,2.51665708881238));
#114410=CARTESIAN_POINT('Ctrl Pts',(6.96597502842747,3.422516948223,2.54577606831888));
#114411=CARTESIAN_POINT('Ctrl Pts',(7.00505989332313,3.42888807474518,2.5603305034797));
#114412=CARTESIAN_POINT('Ctrl Pts',(7.04415121041215,3.43511457408519,2.57486572440514));
#114413=CARTESIAN_POINT('Ctrl Pts',(6.82551648286577,3.52699760873882,3.10843893519605));
#114414=CARTESIAN_POINT('Ctrl Pts',(6.82721953743289,3.52633876186941,3.10468844809802));
#114415=CARTESIAN_POINT('Ctrl Pts',(6.828922592,3.525679915,3.100937961));
#114416=CARTESIAN_POINT('Ctrl Pts',(6.998842397,3.459944422,2.726738538));
#114417=CARTESIAN_POINT('Ctrl Pts',(7.126858153,3.395197164,2.33621336));
#114418=CARTESIAN_POINT('Ctrl Pts',(6.49590563527169,3.52699760873882,3.21959211607213));
#114419=CARTESIAN_POINT('Ctrl Pts',(6.49766993463585,3.52633876186941,3.21602258603607));
#114420=CARTESIAN_POINT('Ctrl Pts',(6.49943423400001,3.525679915,3.212453056));
#114421=CARTESIAN_POINT('Ctrl Pts',(6.67546465,3.459944422,2.856308362));
#114422=CARTESIAN_POINT('Ctrl Pts',(6.81152717,3.395197164,2.483062143));
#114423=CARTESIAN_POINT('',(6.8289225920729,3.52567991457198,3.10093796384888));
#114424=CARTESIAN_POINT('Origin',(-0.16486016511682,3.62494886692739,-0.0923333130057202));
#114425=CARTESIAN_POINT('',(6.66417840968742,3.52567991373765,3.15669551549326));
#114426=CARTESIAN_POINT('Origin',(4.53630188967935E-13,3.61749373599956,
2.83410447887711E-13));
#114427=CARTESIAN_POINT('',(7.04361153473072,3.61640598744859,2.5763416980588));
#114428=CARTESIAN_POINT('Origin',(-0.180347906024595,3.62499782659915,-0.0674445278942343));
#114429=CARTESIAN_POINT('Origin',(-0.171399078671139,3.48215430569431,-0.0855171968849683));
#114430=CARTESIAN_POINT('Ctrl Pts',(6.188633058,3.395189501,4.236840907));
#114431=CARTESIAN_POINT('Ctrl Pts',(6.41865451600001,3.460370723,3.900855103));
#114432=CARTESIAN_POINT('Ctrl Pts',(6.610949329,3.525679915,3.541941413));
#114433=CARTESIAN_POINT('Ctrl Pts',(6.11344464,3.395189501,3.897216268));
#114434=CARTESIAN_POINT('Ctrl Pts',(6.325027606,3.460370723,3.565312503));
#114435=CARTESIAN_POINT('Ctrl Pts',(6.499434234,3.525679915,3.212453056));
#114436=CARTESIAN_POINT('',(6.61094932292316,3.5256799163727,3.5419414217492));
#114437=CARTESIAN_POINT('',(6.55519177567553,3.52567991706895,3.37719724580539));
#114438=CARTESIAN_POINT('',(6.3259428542007,3.43511457320914,4.02895107699497));
#114439=CARTESIAN_POINT('Origin',(-0.166766302908787,3.48214114189395,-0.0972706717238127));
#114440=CARTESIAN_POINT('Ctrl Pts',(6.11596229871932,3.39596551408696,3.89326407601825));
#114441=CARTESIAN_POINT('Ctrl Pts',(6.15088539530709,3.40280154630567,3.91588654109528));
#114442=CARTESIAN_POINT('Ctrl Pts',(6.18586443049033,3.4094772188707,3.93851538946913));
#114443=CARTESIAN_POINT('Ctrl Pts',(6.25584780142413,3.42251694827702,3.98373595685815));
#114444=CARTESIAN_POINT('Ctrl Pts',(6.29089011047695,3.42888807479301,4.00635220799284));
#114445=CARTESIAN_POINT('Ctrl Pts',(6.32594285137405,3.43511457412576,4.02895108112679));
#114446=CARTESIAN_POINT('Ctrl Pts',(5.99771721408108,3.52699760873882,4.50304964280461));
#114447=CARTESIAN_POINT('Ctrl Pts',(6.00018669604054,3.52633876186941,4.4997529464023));
#114448=CARTESIAN_POINT('Ctrl Pts',(6.002656178,3.525679915,4.49645625));
#114449=CARTESIAN_POINT('Ctrl Pts',(6.249045167,3.459944422,4.167533137));
#114450=CARTESIAN_POINT('Ctrl Pts',(6.458019356,3.395197164,3.813657824));
#114451=CARTESIAN_POINT('Ctrl Pts',(5.65191783706956,3.52699760873882,4.54074753539395));
#114452=CARTESIAN_POINT('Ctrl Pts',(5.65440823153479,3.52633876186941,4.53764073119698));
#114453=CARTESIAN_POINT('Ctrl Pts',(5.656898626,3.525679915,4.534533927));
#114454=CARTESIAN_POINT('Ctrl Pts',(5.90537413,3.459944422,4.224557034));
#114455=CARTESIAN_POINT('Ctrl Pts',(6.118492488,3.395197164,3.889286524));
#114456=CARTESIAN_POINT('',(6.00265617747834,3.52567991457199,4.49645625278509));
#114457=CARTESIAN_POINT('Origin',(-0.141156974556259,3.62494888824675,-0.125614739924113));
#114458=CARTESIAN_POINT('',(5.82977739726156,3.52567991373766,4.51549509461761));
#114459=CARTESIAN_POINT('Origin',(5.3776427755281E-14,3.61749373599911,
-6.24500451351651E-14));
#114460=CARTESIAN_POINT('',(6.32509850206447,3.6164059874287,4.03027653313337));
#114461=CARTESIAN_POINT('Origin',(-0.161633041163872,3.62499779048983,-0.104637270481759));
#114462=CARTESIAN_POINT('Origin',(-0.149008033408268,3.48215434141335,-0.120363473142919));
#114463=CARTESIAN_POINT('Ctrl Pts',(5.133150701,3.395189501,5.468159094));
#114464=CARTESIAN_POINT('Ctrl Pts',(5.430021402,3.460370723,5.189476265));
#114465=CARTESIAN_POINT('Ctrl Pts',(5.69497630300001,3.525679915,4.880291478));
#114466=CARTESIAN_POINT('Ctrl Pts',(5.132729405,3.395189501,5.120311403));
#114467=CARTESIAN_POINT('Ctrl Pts',(5.410715178,3.460370723,4.841651446));
#114468=CARTESIAN_POINT('Ctrl Pts',(5.656898626,3.525679915,4.534533927));
#114469=CARTESIAN_POINT('',(5.69497629518052,3.52567991637268,4.88029148524294));
#114470=CARTESIAN_POINT('',(5.67593745638144,3.52567991706893,4.70741271228891));
#114471=CARTESIAN_POINT('',(5.31194043917964,3.4351145732143,5.29464716000112));
#114472=CARTESIAN_POINT('Origin',(-0.141957109364025,3.48214116166584,-0.130846379632369));
#114473=CARTESIAN_POINT('Ctrl Pts',(5.13603780670984,3.39596551408558,5.1169928331588));
#114474=CARTESIAN_POINT('Ctrl Pts',(5.16528125939142,3.40280154629497,5.14659383098163));
#114475=CARTESIAN_POINT('Ctrl Pts',(5.19457797078606,3.40947721888794,5.17621308816852));
#114476=CARTESIAN_POINT('Ctrl Pts',(5.2532040840705,3.42251694828979,5.2354207798644));
#114477=CARTESIAN_POINT('Ctrl Pts',(5.28256529793846,3.42888807480765,5.26504133623591));
#114478=CARTESIAN_POINT('Ctrl Pts',(5.31194043551467,3.4351145741414,5.29464716344254));
#114479=CARTESIAN_POINT('Ctrl Pts',(4.87496063697409,3.53021247068103,5.70030219065627));
#114480=CARTESIAN_POINT('Ctrl Pts',(4.88569435681569,3.52794619284054,5.69105215235571));
#114481=CARTESIAN_POINT('Ctrl Pts',(4.89642807665729,3.525679915,5.68180211405501));
#114482=CARTESIAN_POINT('Ctrl Pts',(5.20776958690419,3.459944422,5.41349616449876));
#114483=CARTESIAN_POINT('Ctrl Pts',(5.48793070797208,3.395197164,5.11277808154849));
#114484=CARTESIAN_POINT('Ctrl Pts',(4.52852590289775,3.53021247068103,5.66177564884319));
#114485=CARTESIAN_POINT('Ctrl Pts',(4.53918931444891,3.52794619284054,5.65318033992153));
#114486=CARTESIAN_POINT('Ctrl Pts',(4.549852726,3.525679915,5.644585031));
#114487=CARTESIAN_POINT('Ctrl Pts',(4.859154879,3.459944422,5.395270115));
#114488=CARTESIAN_POINT('Ctrl Pts',(5.139363898,3.395197164,5.11365219));
#114489=CARTESIAN_POINT('',(4.89571222559471,3.52567991503086,5.68172524922569));
#114490=CARTESIAN_POINT('Origin',(-0.110853255847381,3.62494888055425,-0.153022410279826));
#114491=CARTESIAN_POINT('',(4.7227824735572,3.52567991373765,5.66315514195599));
#114492=CARTESIAN_POINT('Origin',(-7.41594285980085E-13,3.61749373599945,
-6.34041430469523E-13));
#114493=CARTESIAN_POINT('',(5.31083089400444,3.61640598738723,5.29576011612747));
#114494=CARTESIAN_POINT('Origin',(-0.135360135003075,3.62499784668088,-0.136937159235024));
#114495=CARTESIAN_POINT('Origin',(-0.119649928874311,3.48215430814406,-0.149581986761579));
#114496=CARTESIAN_POINT('Ctrl Pts',(3.837647923,3.395189501,6.443792239));
#114497=CARTESIAN_POINT('Ctrl Pts',(4.187486522,3.460370723,6.235443285));
#114498=CARTESIAN_POINT('Ctrl Pts',(4.512712514,3.525679915,5.990444538));
#114499=CARTESIAN_POINT('Ctrl Pts',(3.912013447,3.395189501,6.103986467));
#114500=CARTESIAN_POINT('Ctrl Pts',(4.243403721,3.460370723,5.89160015));
#114501=CARTESIAN_POINT('Ctrl Pts',(4.549852726,3.525679915,5.644585031));
#114502=CARTESIAN_POINT('',(4.5127125047959,3.52567991637267,5.99044454340971));
#114503=CARTESIAN_POINT('',(4.53128260996699,3.52567991706892,5.81751479231475));
#114504=CARTESIAN_POINT('',(4.04955759272161,3.43511457319818,6.31277142654194));
#114505=CARTESIAN_POINT('Origin',(-0.110510112930169,3.48214119229473,-0.158303805610382));
#114506=CARTESIAN_POINT('Ctrl Pts',(3.91595789455974,3.39596551410652,6.10145669238762));
#114507=CARTESIAN_POINT('Ctrl Pts',(3.93815431206374,3.40280154626537,6.13665211314041));
#114508=CARTESIAN_POINT('Ctrl Pts',(3.96039881813328,3.40947721889377,6.17187681583231));
#114509=CARTESIAN_POINT('Ctrl Pts',(4.00492638196425,3.42251694824804,6.2423031459704));
#114510=CARTESIAN_POINT('Ctrl Pts',(4.02723360296451,3.42888807475989,6.27754298333113));
#114511=CARTESIAN_POINT('Ctrl Pts',(4.04955758846055,3.43511457409361,6.31277142908387));
#114512=CARTESIAN_POINT('Ctrl Pts',(3.53559029459435,3.53021247059306,6.61500472694062));
#114513=CARTESIAN_POINT('Ctrl Pts',(3.54806155060326,3.52794619279656,6.60827838200748));
#114514=CARTESIAN_POINT('Ctrl Pts',(3.56053280661218,3.525679915,6.60155203707424));
#114515=CARTESIAN_POINT('Ctrl Pts',(3.92227317371199,3.459944422,6.4064481530995));
#114516=CARTESIAN_POINT('Ctrl Pts',(4.26052978288272,3.395197164,6.17298705222511));
#114517=CARTESIAN_POINT('Ctrl Pts',(3.20553707987759,3.53021247059306,6.50290568697574));
#114518=CARTESIAN_POINT('Ctrl Pts',(3.21779892393879,3.52794619279656,6.4968036499879));
#114519=CARTESIAN_POINT('Ctrl Pts',(3.230060768,3.525679915,6.490701613));
#114520=CARTESIAN_POINT('Ctrl Pts',(3.585726947,3.459944422,6.313706361));
#114521=CARTESIAN_POINT('Ctrl Pts',(3.919924364,3.395197164,6.098909163));
#114522=CARTESIAN_POINT('',(3.55985021551222,3.52567991503086,6.60132308264157));
#114523=CARTESIAN_POINT('Origin',(-0.0753663511695235,3.62494888555094,
-0.173275155946407));
#114524=CARTESIAN_POINT('',(3.39495548913079,3.52567991373766,6.54601234906258));
#114525=CARTESIAN_POINT('Origin',(4.4799233767101E-13,3.617493736,7.91467585914418E-13));
#114526=CARTESIAN_POINT('',(4.04823473517133,3.61640598738359,6.313619843195));
#114527=CARTESIAN_POINT('Origin',(-0.10275807953716,3.62499778990581,-0.162834087887939));
#114528=CARTESIAN_POINT('Origin',(-0.0846966427635254,3.48215434346587,
-0.171805656129049));
#114529=CARTESIAN_POINT('Ctrl Pts',(2.362700993,3.395189501,7.118120821));
#114530=CARTESIAN_POINT('Ctrl Pts',(2.749149426,3.460370723,6.989847907));
#114531=CARTESIAN_POINT('Ctrl Pts',(3.119439304,3.525679915,6.82049107000001));
#114532=CARTESIAN_POINT('Ctrl Pts',(2.508376089,3.395189501,6.802245908));
#114533=CARTESIAN_POINT('Ctrl Pts',(2.877675422,3.460370723,6.66606417800001));
#114534=CARTESIAN_POINT('Ctrl Pts',(3.230060768,3.525679915,6.490701613));
#114535=CARTESIAN_POINT('',(3.1194392938772,3.52567991637269,6.82049107327703));
#114536=CARTESIAN_POINT('',(3.17475002452162,3.52567991706892,6.65559634697524));
#114537=CARTESIAN_POINT('',(2.59782193401564,3.43511457318079,7.03571751640869));
#114538=CARTESIAN_POINT('Origin',(-0.0738957832790441,3.48214118551873,
-0.178359144995427));
#114539=CARTESIAN_POINT('Ctrl Pts',(2.51277214422329,3.39596551412194,6.80062321811182));
#114540=CARTESIAN_POINT('Ctrl Pts',(2.52688364670092,3.40280154628805,6.83976736312154));
#114541=CARTESIAN_POINT('Ctrl Pts',(2.54103581861051,3.40947721886961,6.87895044276729));
#114542=CARTESIAN_POINT('Ctrl Pts',(2.56938277353199,3.42251694822021,6.95730235429953));
#114543=CARTESIAN_POINT('Ctrl Pts',(2.58359294074119,3.42888807472082,6.99651369683442));
#114544=CARTESIAN_POINT('Ctrl Pts',(2.59782192937818,3.43511457404109,7.03571751795521));
#114545=CARTESIAN_POINT('Ctrl Pts',(2.03089968052327,3.53021247053072,7.22039699483326));
#114546=CARTESIAN_POINT('Ctrl Pts',(2.04452533064616,3.5279461927654,7.21650885952546));
#114547=CARTESIAN_POINT('Ctrl Pts',(2.05815098076905,3.525679915,7.21262072421754));
#114548=CARTESIAN_POINT('Ctrl Pts',(2.45337562708328,3.459944422,7.09984174574432));
#114549=CARTESIAN_POINT('Ctrl Pts',(2.8339112193165,3.395197164,6.94455400749315));
#114550=CARTESIAN_POINT('Ctrl Pts',(1.73266090633112,3.53021247053073,7.03996708343377));
#114551=CARTESIAN_POINT('Ctrl Pts',(1.74594783266555,3.52794619276539,7.03664364271693));
#114552=CARTESIAN_POINT('Ctrl Pts',(1.759234759,3.525679915,7.033320202));
#114553=CARTESIAN_POINT('Ctrl Pts',(2.144634407,3.459944422,6.936920715));
#114554=CARTESIAN_POINT('Ctrl Pts',(2.517193523,3.395197164,6.798987922));
#114555=CARTESIAN_POINT('',(2.05753356667625,3.52567991503086,7.21225038558017));
#114556=CARTESIAN_POINT('Origin',(-0.0363553141379602,3.62494885502381,
-0.18542562761704));
#114557=CARTESIAN_POINT('',(1.90838416002549,3.52567991373765,7.12278529450262));
#114558=CARTESIAN_POINT('Origin',(3.02709246557953E-13,3.61749373599945,
9.86623976961809E-13));
#114559=CARTESIAN_POINT('',(2.59634761954239,3.61640598744957,7.03626172285194));
#114560=CARTESIAN_POINT('Origin',(-0.0653511308448051,3.62499783906402,
-0.181117100456151));
#114561=CARTESIAN_POINT('Origin',(-0.0457833834977586,3.48215431398279,
-0.185996321826775));
#114562=CARTESIAN_POINT('Ctrl Pts',(0.77727679,3.395189501,7.459613984));
#114563=CARTESIAN_POINT('Ctrl Pts',(1.182265159,3.460370723,7.41741501));
#114564=CARTESIAN_POINT('Ctrl Pts',(1.580304579,3.525679915,7.331619019));
#114565=CARTESIAN_POINT('Ctrl Pts',(0.987449852,3.395189501,7.182439891));
#114566=CARTESIAN_POINT('Ctrl Pts',(1.377390219,3.460370723,7.128830454));
#114567=CARTESIAN_POINT('Ctrl Pts',(1.759234759,3.525679915,7.033320202));
#114568=CARTESIAN_POINT('',(1.58030456839241,3.52567991637267,7.33161902003236));
#114569=CARTESIAN_POINT('',(1.66976965661296,3.52567991706892,7.18246961337972));
#114570=CARTESIAN_POINT('',(1.02461500936863,3.43511457320313,7.42968127573517));
#114571=CARTESIAN_POINT('Origin',(-0.0338261750837945,3.48214117583839,
-0.190074447514669));
#114572=CARTESIAN_POINT('Ctrl Pts',(0.992091959997785,3.39596551403114,
7.18180016033055));
#114573=CARTESIAN_POINT('Ctrl Pts',(0.997458679230474,3.4028015076774,7.22306246019008));
#114574=CARTESIAN_POINT('Ctrl Pts',(1.00285674279637,3.40947714064642,7.26437149719111));
#114575=CARTESIAN_POINT('Ctrl Pts',(1.01369768213607,3.42251694824779,7.34698583753522));
#114576=CARTESIAN_POINT('Ctrl Pts',(1.0191463441452,3.42888807477032,7.38833520666078));
#114577=CARTESIAN_POINT('Ctrl Pts',(1.02461500441485,3.43511457410805,7.42968127625411));
#114578=CARTESIAN_POINT('Ctrl Pts',(0.431246454934853,3.53021247045305,
7.48817152328426));
#114579=CARTESIAN_POINT('Ctrl Pts',(0.445389378855488,3.52794619272655,
7.48730340245222));
#114580=CARTESIAN_POINT('Ctrl Pts',(0.459532302776112,3.525679915,7.48643528162022));
#114581=CARTESIAN_POINT('Ctrl Pts',(0.86976096341033,3.459944422,7.46125462957233));
#114582=CARTESIAN_POINT('Ctrl Pts',(1.27478211834841,3.395197164,7.391401337075));
#114583=CARTESIAN_POINT('Ctrl Pts',(0.178767434650042,3.53021247045304,
7.24784744324904));
#114584=CARTESIAN_POINT('Ctrl Pts',(0.192458161325023,3.52794619272655,
7.2474579991246));
#114585=CARTESIAN_POINT('Ctrl Pts',(0.206148888,3.525679915,7.247068555));
#114586=CARTESIAN_POINT('Ctrl Pts',(0.603261147,3.459944422,7.23577236600001));
#114587=CARTESIAN_POINT('Ctrl Pts',(0.99676151,3.395197164,7.181153563));
#114588=CARTESIAN_POINT('',(0.459008935823992,3.52567991457841,7.48594087527957));
#114589=CARTESIAN_POINT('Origin',(0.00435568230947841,3.62494884631261,
-0.188905893396506));
#114590=CARTESIAN_POINT('',(0.332578908769786,3.52567991373766,7.366504715349));
#114591=CARTESIAN_POINT('Origin',(6.15284732885524E-15,3.617493736,-4.04190569902596E-13));
#114592=CARTESIAN_POINT('',(1.02305817476536,3.61640598740894,7.42989582457253));
#114593=CARTESIAN_POINT('Origin',(-0.024888475145801,3.62499784137454,-0.19093145372851));
#114594=CARTESIAN_POINT('Origin',(-0.00472925965781933,3.4821543278721,
-0.191489718375762));
#114595=CARTESIAN_POINT('Origin',(4.78505852562899E-14,3.61749373599978,
-1.58293517182884E-13));
#114596=CARTESIAN_POINT('',(-0.598068333136022,3.6164059873872,7.47611625540621));
#114597=CARTESIAN_POINT('',(-0.0327234426153162,3.52567991637269,7.499928609745));
#114598=CARTESIAN_POINT('Origin',(0.0167380089118564,3.62499783159569,-0.19181783794649));
#114599=CARTESIAN_POINT('Origin',(0.0365459621040783,3.4821543444113,-0.188029733640196));
#114600=CARTESIAN_POINT('Origin',(0.00782484508443366,3.48214246272938,
-0.19290238903462));
#114601=CARTESIAN_POINT('Ctrl Pts',(-0.844492011,3.395189501,7.452303888));
#114602=CARTESIAN_POINT('Ctrl Pts',(-0.439900514,3.460370723,7.49815203));
#114603=CARTESIAN_POINT('Ctrl Pts',(-0.032723432,3.525679915,7.499928611));
#114604=CARTESIAN_POINT('Ctrl Pts',(-0.579648442,3.395189501,7.226790967));
#114605=CARTESIAN_POINT('Ctrl Pts',(-0.18730022,3.460370723,7.258260542));
#114606=CARTESIAN_POINT('Ctrl Pts',(0.206148888,3.525679915,7.247068555));
#114607=CARTESIAN_POINT('',(0.0867127152835091,3.52567991706892,7.37349858314955));
#114608=CARTESIAN_POINT('Ctrl Pts',(-0.029487061,2.231898283,7.499942034));
#114609=CARTESIAN_POINT('Ctrl Pts',(0.376600717,2.296352134,7.501538624));
#114610=CARTESIAN_POINT('Ctrl Pts',(0.780486766,2.361474582,7.459278813));
#114611=CARTESIAN_POINT('Ctrl Pts',(0.209276124,2.231898283,7.246978923));
#114612=CARTESIAN_POINT('Ctrl Pts',(0.601667098,2.296352134,7.235647572));
#114613=CARTESIAN_POINT('Ctrl Pts',(0.990540534,2.361474582,7.18201430300001));
#114614=CARTESIAN_POINT('',(0.213937949141283,2.23266407427649,7.24684279847903));
#114615=CARTESIAN_POINT('Origin',(-0.0350318282142846,2.4106890065044,-0.193902277117336));
#114616=CARTESIAN_POINT('Ctrl Pts',(0.213937947891224,2.23266407474045,
7.24684279881095));
#114617=CARTESIAN_POINT('Ctrl Pts',(0.215059230318048,2.23947867583925,
7.28843449958464));
#114618=CARTESIAN_POINT('Ctrl Pts',(0.216123655395898,2.24612512499677,
7.33008178274923));
#114619=CARTESIAN_POINT('Ctrl Pts',(0.218146489019095,2.25909150516261,
7.41337727741362));
#114620=CARTESIAN_POINT('Ctrl Pts',(0.219106098113739,2.26541917072379,
7.4550752107625));
#114621=CARTESIAN_POINT('Ctrl Pts',(0.220017220171437,2.27159573038441,
7.49677213338445));
#114622=CARTESIAN_POINT('Ctrl Pts',(1.267805044,2.361474582,7.392068071));
#114623=CARTESIAN_POINT('Ctrl Pts',(1.504915875,2.323357812,7.351401467));
#114624=CARTESIAN_POINT('Ctrl Pts',(1.738933089,2.285714286,7.295622778));
#114625=CARTESIAN_POINT('Ctrl Pts',(1.905464967,2.258926311,7.255929416));
#114626=CARTESIAN_POINT('Ctrl Pts',(2.070012238,2.231887255,7.208678751));
#114627=CARTESIAN_POINT('Ctrl Pts',(0.990540534000001,2.361474582,7.182014303));
#114628=CARTESIAN_POINT('Ctrl Pts',(1.220913599,2.323357812,7.150241342));
#114629=CARTESIAN_POINT('Ctrl Pts',(1.448776863,2.285714286,7.103769816));
#114630=CARTESIAN_POINT('Ctrl Pts',(1.610929454,2.258926311,7.07069964));
#114631=CARTESIAN_POINT('Ctrl Pts',(1.771404205,2.231887255,7.030265083));
#114632=CARTESIAN_POINT('',(1.76679318276177,2.23266407430095,7.03142530562253));
#114633=CARTESIAN_POINT('Ctrl Pts',(1.76679318313451,2.2326640749721,7.03142530665601));
#114634=CARTESIAN_POINT('Ctrl Pts',(1.66111643034258,2.2504649376073,7.05797880923018));
#114635=CARTESIAN_POINT('Ctrl Pts',(1.55505543246003,2.26815682580635,7.08209485553649));
#114636=CARTESIAN_POINT('Ctrl Pts',(1.44877686378956,2.28571428590264,7.10376981601217));
#114637=CARTESIAN_POINT('Ctrl Pts',(1.29741506427075,2.31071959718532,7.13463926700789));
#114638=CARTESIAN_POINT('Ctrl Pts',(1.14451922017561,2.33599777478011,7.16077762395494));
#114639=CARTESIAN_POINT('Ctrl Pts',(0.990540544201328,2.36147458031212,
7.18201430159304));
#114640=CARTESIAN_POINT('Ctrl Pts',(1.82645774549815,2.27159573035706,7.2742045682774));
#114641=CARTESIAN_POINT('Ctrl Pts',(1.81660431901047,2.26541917066066,7.23367836058223));
#114642=CARTESIAN_POINT('Ctrl Pts',(1.80670332189861,2.25909150510592,7.19316158924002));
#114643=CARTESIAN_POINT('Ctrl Pts',(1.78682148080259,2.24612497437885,7.11224740650066));
#114644=CARTESIAN_POINT('Ctrl Pts',(1.77682912854049,2.23947860190669,7.07180313520404));
#114645=CARTESIAN_POINT('Ctrl Pts',(1.76679318370471,2.23266407485744,7.03142530641884));
#114646=CARTESIAN_POINT('Ctrl Pts',(1.583468171,2.231898283,7.330936403));
#114647=CARTESIAN_POINT('Ctrl Pts',(1.980405062,2.296352134,7.245198798));
#114648=CARTESIAN_POINT('Ctrl Pts',(2.365763869,2.361474582,7.117103436));
#114649=CARTESIAN_POINT('Ctrl Pts',(1.762269613,2.231898283,7.032560402));
#114650=CARTESIAN_POINT('Ctrl Pts',(2.1430508,2.296352134,6.937141511));
#114651=CARTESIAN_POINT('Ctrl Pts',(2.511303023,2.361474582,6.801165865));
#114652=CARTESIAN_POINT('Origin',(-0.0758960812681775,2.41068907463865,
-0.181838198609218));
#114653=CARTESIAN_POINT('Ctrl Pts',(2.827240594,2.361474582,6.946705019));
#114654=CARTESIAN_POINT('Ctrl Pts',(3.050065787,2.323357812,6.85601735800001));
#114655=CARTESIAN_POINT('Ctrl Pts',(3.26662104,2.285714286,6.75123596));
#114656=CARTESIAN_POINT('Ctrl Pts',(3.420726596,2.258926311,6.676671176));
#114657=CARTESIAN_POINT('Ctrl Pts',(3.571269346,2.231887255,6.595152406));
#114658=CARTESIAN_POINT('Ctrl Pts',(2.511303023,2.361474582,6.801165865));
#114659=CARTESIAN_POINT('Ctrl Pts',(2.729459846,2.323357812,6.720612339));
#114660=CARTESIAN_POINT('Ctrl Pts',(2.94200579,2.285714286,6.626243425));
#114661=CARTESIAN_POINT('Ctrl Pts',(3.093258233,2.258926311,6.559088397));
#114662=CARTESIAN_POINT('Ctrl Pts',(3.241288939,2.231887255,6.485101851));
#114663=CARTESIAN_POINT('',(3.2370351332511,2.23266407427388,6.487226180923));
#114664=CARTESIAN_POINT('Ctrl Pts',(3.23703513419218,2.23266407494668,6.48722618256281));
#114665=CARTESIAN_POINT('Ctrl Pts',(3.13953726152733,2.25046493790256,6.53587625704972));
#114666=CARTESIAN_POINT('Ctrl Pts',(3.04114014799221,2.26815682610644,6.58222846268839));
#114667=CARTESIAN_POINT('Ctrl Pts',(2.94200578976456,2.28571428604824,6.62624342513513));
#114668=CARTESIAN_POINT('Ctrl Pts',(2.80081876472916,2.31071959711799,6.68892947768875));
#114669=CARTESIAN_POINT('Ctrl Pts',(2.65711651507422,2.3359977746946,6.74732482159475));
#114670=CARTESIAN_POINT('Ctrl Pts',(2.51130303266037,2.36147458031212,6.80116586143295));
#114671=CARTESIAN_POINT('Ctrl Pts',(3.34749513650598,2.27159573034486,6.71150328220306));
#114672=CARTESIAN_POINT('Ctrl Pts',(3.32916014099096,2.26541917064281,6.67404275010762));
#114673=CARTESIAN_POINT('Ctrl Pts',(3.31078071561367,2.25909150509045,6.63660166006047));
#114674=CARTESIAN_POINT('Ctrl Pts',(3.27396951324641,2.24612496366142,6.56185315251622));
#114675=CARTESIAN_POINT('Ctrl Pts',(3.25551646985988,2.23947859656426,6.52450253886267));
#114676=CARTESIAN_POINT('Ctrl Pts',(3.23703513444457,2.23266407473202,6.48722618166756));
#114677=CARTESIAN_POINT('Ctrl Pts',(3.122382191,2.231898283,6.819144334));
#114678=CARTESIAN_POINT('Ctrl Pts',(3.491607867,2.296352134,6.650081528));
#114679=CARTESIAN_POINT('Ctrl Pts',(3.840420483,2.361474582,6.442140212));
#114680=CARTESIAN_POINT('Ctrl Pts',(3.232861335,2.231898283,6.489307173));
#114681=CARTESIAN_POINT('Ctrl Pts',(3.584227827,2.296352134,6.314262424));
#114682=CARTESIAN_POINT('Ctrl Pts',(3.914639774,2.361474582,6.10230247));
#114683=CARTESIAN_POINT('Origin',(-0.113211494847705,2.41068900069649,-0.16127150375959));
#114684=CARTESIAN_POINT('Ctrl Pts',(4.254477516,2.361474582,6.176521761));
#114685=CARTESIAN_POINT('Ctrl Pts',(4.452598014,2.323357812,6.040053497));
#114686=CARTESIAN_POINT('Ctrl Pts',(4.641565421,2.285714286,5.891168852));
#114687=CARTESIAN_POINT('Ctrl Pts',(4.776038851,2.258926311,5.785219212));
#114688=CARTESIAN_POINT('Ctrl Pts',(4.90553787,2.231887255,5.673244064));
#114689=CARTESIAN_POINT('Ctrl Pts',(3.914639774,2.361474582,6.10230247));
#114690=CARTESIAN_POINT('Ctrl Pts',(4.110379585,2.323357812,5.976734973));
#114691=CARTESIAN_POINT('Ctrl Pts',(4.297669796,2.285714286,5.838881257));
#114692=CARTESIAN_POINT('Ctrl Pts',(4.430949694,2.258926311,5.740781472));
#114693=CARTESIAN_POINT('Ctrl Pts',(4.559614604,2.231887255,5.636702463));
#114694=CARTESIAN_POINT('',(4.55591691843822,2.23266407431282,5.63969157044102));
#114695=CARTESIAN_POINT('Ctrl Pts',(4.55591691922223,2.23266407495794,5.63969157124384));
#114696=CARTESIAN_POINT('Ctrl Pts',(4.47115682192384,2.25046493763,5.70816339437997));
#114697=CARTESIAN_POINT('Ctrl Pts',(4.38502453261706,2.26815682582794,5.77458438244212));
#114698=CARTESIAN_POINT('Ctrl Pts',(4.29766979662721,2.28571428587394,5.83888125653835));
#114699=CARTESIAN_POINT('Ctrl Pts',(4.17325929344737,2.31071959707719,5.93045278120617));
#114700=CARTESIAN_POINT('Ctrl Pts',(4.04546999514317,2.33599777466947,6.01837461000912));
#114701=CARTESIAN_POINT('Ctrl Pts',(3.91463978266786,2.36147458031209,6.10230246443955));
#114702=CARTESIAN_POINT('Ctrl Pts',(4.71200737576558,2.27159573036368,5.83497956214766));
#114703=CARTESIAN_POINT('Ctrl Pts',(4.68604813524469,2.26541917068898,5.80233631873936));
#114704=CARTESIAN_POINT('Ctrl Pts',(4.66004968284631,2.25909150510957,5.76972161364608));
#114705=CARTESIAN_POINT('Ctrl Pts',(4.60803103341143,2.24612512498883,5.70463481466443));
#114706=CARTESIAN_POINT('Ctrl Pts',(4.58197979005519,2.23947867584863,5.6721238638597));
#114707=CARTESIAN_POINT('Ctrl Pts',(4.5559169200463,2.23266407478488,5.63969157057813));
#114708=CARTESIAN_POINT('Ctrl Pts',(4.51529709,2.231898283,5.988496655));
#114709=CARTESIAN_POINT('Ctrl Pts',(4.839546969,2.296352134,5.744013838));
#114710=CARTESIAN_POINT('Ctrl Pts',(5.135503304,2.361474582,5.465949672));
#114711=CARTESIAN_POINT('Ctrl Pts',(4.552288053,2.231898283,5.642621154));
#114712=CARTESIAN_POINT('Ctrl Pts',(4.857810345,2.296352134,5.396135444));
#114713=CARTESIAN_POINT('Ctrl Pts',(5.13493232,2.361474582,5.118102194));
#114714=CARTESIAN_POINT('Origin',(-0.145233333309196,2.41068900203097,-0.13316399617367));
#114715=CARTESIAN_POINT('Ctrl Pts',(5.482779798,2.361474582,5.11753121));
#114716=CARTESIAN_POINT('Ctrl Pts',(5.646931706,2.323357812,4.94166344799999));
#114717=CARTESIAN_POINT('Ctrl Pts',(5.799475362,2.285714286,4.755637236));
#114718=CARTESIAN_POINT('Ctrl Pts',(5.908028837,2.258926311,4.623256827));
#114719=CARTESIAN_POINT('Ctrl Pts',(6.010428894,2.231887255,4.486061135));
#114720=CARTESIAN_POINT('Ctrl Pts',(5.13493232,2.361474582,5.118102194));
#114721=CARTESIAN_POINT('Ctrl Pts',(5.299102543,2.323357812,4.953392122));
#114722=CARTESIAN_POINT('Ctrl Pts',(5.452379538,2.285714286,4.77849949));
#114723=CARTESIAN_POINT('Ctrl Pts',(5.561454873,2.258926311,4.654041985));
#114724=CARTESIAN_POINT('Ctrl Pts',(5.664737759,2.231887255,4.52473713300001));
#114725=CARTESIAN_POINT('',(5.66176909176001,2.23266407433869,4.52845125015997));
#114726=CARTESIAN_POINT('Ctrl Pts',(5.66176909332444,2.23266407511861,4.52845125124809));
#114727=CARTESIAN_POINT('Ctrl Pts',(5.59371005768589,2.25046493777582,4.61354315659389));
#114728=CARTESIAN_POINT('Ctrl Pts',(5.52387004230441,2.26815682591767,4.69692715478952));
#114729=CARTESIAN_POINT('Ctrl Pts',(5.45237953861184,2.28571428586119,4.77849948935201));
#114730=CARTESIAN_POINT('Ctrl Pts',(5.35056285566987,2.31071959699885,4.89467470310772));
#114731=CARTESIAN_POINT('Ctrl Pts',(5.24466179475073,2.33599777457497,5.00801189012035));
#114732=CARTESIAN_POINT('Ctrl Pts',(5.13493232726982,2.36147458031211,5.11810218670628));
#114733=CARTESIAN_POINT('Ctrl Pts',(5.85619138690653,2.27159573036205,4.68561868236548));
#114734=CARTESIAN_POINT('Ctrl Pts',(5.82382172662383,2.26541917069934,4.6593190892797));
#114735=CARTESIAN_POINT('Ctrl Pts',(5.79141990591579,2.25909150509652,4.63305579658063));
#114736=CARTESIAN_POINT('Ctrl Pts',(5.72662492635262,2.24612497303148,4.58067254904189));
#114737=CARTESIAN_POINT('Ctrl Pts',(5.69419425737027,2.23947860122615,4.5545222619207));
#114738=CARTESIAN_POINT('Ctrl Pts',(5.66176909363111,2.23266407484144,4.52845125000692));
#114739=CARTESIAN_POINT('Ctrl Pts',(5.697081715,2.231898283,4.87783352800001));
#114740=CARTESIAN_POINT('Ctrl Pts',(5.961194234,2.296352134,4.569362444));
#114741=CARTESIAN_POINT('Ctrl Pts',(6.190455698,2.361474582,4.2341774));
#114742=CARTESIAN_POINT('Ctrl Pts',(5.658854841,2.231898283,4.53209244));
#114743=CARTESIAN_POINT('Ctrl Pts',(5.90424705100001,2.296352134,4.225691167));
#114744=CARTESIAN_POINT('Ctrl Pts',(6.115121138,2.361474582,3.894585148));
#114745=CARTESIAN_POINT('Origin',(-0.170464169393162,2.41068905305429,-0.0988298170244395));
#114746=CARTESIAN_POINT('Ctrl Pts',(6.45471339,2.361474582,3.819250588));
#114747=CARTESIAN_POINT('Ctrl Pts',(6.577221147,2.323357812,3.612206708));
#114748=CARTESIAN_POINT('Ctrl Pts',(6.686208281,2.285714286,3.397737309));
#114749=CARTESIAN_POINT('Ctrl Pts',(6.763765961,2.258926311,3.245116092));
#114750=CARTESIAN_POINT('Ctrl Pts',(6.834278944,2.231887255,3.089114974));
#114751=CARTESIAN_POINT('Ctrl Pts',(6.115121138,2.361474582,3.894585148));
#114752=CARTESIAN_POINT('Ctrl Pts',(6.240045355,2.323357812,3.69843416));
#114753=CARTESIAN_POINT('Ctrl Pts',(6.352142073,2.285714286,3.494680397));
#114754=CARTESIAN_POINT('Ctrl Pts',(6.431912603,2.258926311,3.349684667));
#114755=CARTESIAN_POINT('Ctrl Pts',(6.50498407100001,2.231887255,3.201200124));
#114756=CARTESIAN_POINT('',(6.50288323569477,2.23266407432216,3.20546558258028));
#114757=CARTESIAN_POINT('Ctrl Pts',(6.50288323697012,2.23266407502953,3.2054655830801));
#114758=CARTESIAN_POINT('Ctrl Pts',(6.45470762816993,2.25046493780333,3.30319876787987));
#114759=CARTESIAN_POINT('Ctrl Pts',(6.40442552820004,2.26815682598676,3.39964683318256));
#114760=CARTESIAN_POINT('Ctrl Pts',(6.35214207326452,2.28571428606369,3.49468039721292));
#114761=CARTESIAN_POINT('Ctrl Pts',(6.27768004475488,2.31071959737376,3.63002707721038));
#114762=CARTESIAN_POINT('Ctrl Pts',(6.19861903637983,2.33599777477379,3.76348010121415));
#114763=CARTESIAN_POINT('Ctrl Pts',(6.11512114353184,2.36147458031213,3.89458513931412));
#114764=CARTESIAN_POINT('Ctrl Pts',(6.72654639743712,2.27159573032736,3.31716348119342));
#114765=CARTESIAN_POINT('Ctrl Pts',(6.68927988679343,2.26541917067551,3.29843727796667));
#114766=CARTESIAN_POINT('Ctrl Pts',(6.65198977122115,2.25909150509326,3.2797534400945));
#114767=CARTESIAN_POINT('Ctrl Pts',(6.57744881346161,2.24612497317182,3.24252388941654));
#114768=CARTESIAN_POINT('Ctrl Pts',(6.5401548165271,2.23947860131222,3.22395661652792));
#114769=CARTESIAN_POINT('Ctrl Pts',(6.50288323776577,2.23266407482983,3.205465581897));
#114770=CARTESIAN_POINT('Ctrl Pts',(6.612477132,2.231898283,3.539088327));
#114771=CARTESIAN_POINT('Ctrl Pts',(6.804102681,2.296352134,3.18105274));
#114772=CARTESIAN_POINT('Ctrl Pts',(6.955949263,2.361474582,2.804419699));
#114773=CARTESIAN_POINT('Ctrl Pts',(6.500819867,2.231898283,3.209648121));
#114774=CARTESIAN_POINT('Ctrl Pts',(6.67460772600001,2.296352134,2.857658268));
#114775=CARTESIAN_POINT('Ctrl Pts',(6.809373687,2.361474582,2.488961628));
#114776=CARTESIAN_POINT('Origin',(-0.187724371365596,2.41068903802582,-0.059874491679216));
#114777=CARTESIAN_POINT('Ctrl Pts',(7.124831758,2.361474582,2.342386053));
#114778=CARTESIAN_POINT('Ctrl Pts',(7.199967038,2.323357812,2.113847197));
#114779=CARTESIAN_POINT('Ctrl Pts',(7.260301532,2.285714286,1.880962961));
#114780=CARTESIAN_POINT('Ctrl Pts',(7.303236907,2.258926311,1.715237335));
#114781=CARTESIAN_POINT('Ctrl Pts',(7.338565706,2.231887255,1.547725229));
#114782=CARTESIAN_POINT('Ctrl Pts',(6.809373687,2.361474582,2.488961628));
#114783=CARTESIAN_POINT('Ctrl Pts',(6.889210582,2.323357812,2.270541528));
#114784=CARTESIAN_POINT('Ctrl Pts',(6.954885505,2.285714286,2.047453934));
#114785=CARTESIAN_POINT('Ctrl Pts',(7.001621248,2.258926311,1.888699818));
#114786=CARTESIAN_POINT('Ctrl Pts',(7.04106455800001,2.231887255,1.727978555));
#114787=CARTESIAN_POINT('',(7.03992978615661,2.23266407431315,1.73259590695452));
#114788=CARTESIAN_POINT('Ctrl Pts',(7.03992978791672,2.23266407503294,1.73259590726661));
#114789=CARTESIAN_POINT('Ctrl Pts',(7.01389024407878,2.25046493769433,1.83840047597408));
#114790=CARTESIAN_POINT('Ctrl Pts',(6.98551719494212,2.2681568258671,1.94340280424178));
#114791=CARTESIAN_POINT('Ctrl Pts',(6.95488550524722,2.28571428596627,2.04745393369742));
#114792=CARTESIAN_POINT('Ctrl Pts',(6.91125989250801,2.31071959731997,2.19564341897167));
#114793=CARTESIAN_POINT('Ctrl Pts',(6.86273574210138,2.33599777471104,2.34297216457218));
#114794=CARTESIAN_POINT('Ctrl Pts',(6.80937369053531,2.36147458031212,2.48896161832797));
#114795=CARTESIAN_POINT('Ctrl Pts',(7.28237557417371,2.27159573035333,1.7936014024457));
#114796=CARTESIAN_POINT('Ctrl Pts',(7.24195475347828,2.26541917064691,1.78332420566177));
#114797=CARTESIAN_POINT('Ctrl Pts',(7.20151998735164,2.25909150506858,1.7730934581438));
#114798=CARTESIAN_POINT('Ctrl Pts',(7.12071848928356,2.24612497095763,1.75275841277512));
#114799=CARTESIAN_POINT('Ctrl Pts',(7.08030499745313,2.2394786001742,1.74264234112778));
#114800=CARTESIAN_POINT('Ctrl Pts',(7.03992978796534,2.23266407477575,1.73259590593616));
#114801=CARTESIAN_POINT('Ctrl Pts',(7.218680466,2.231898283,2.034859288));
#114802=CARTESIAN_POINT('Ctrl Pts',(7.328858849,2.296352134,1.644000547));
#114803=CARTESIAN_POINT('Ctrl Pts',(7.39619037200001,2.361474582,1.24353045));
#114804=CARTESIAN_POINT('Ctrl Pts',(7.03881378000001,2.231898283,1.737124223));
#114805=CARTESIAN_POINT('Ctrl Pts',(7.13287116300001,2.296352134,1.356004445));
#114806=CARTESIAN_POINT('Ctrl Pts',(7.185227491,2.361474582,0.96695703));
#114807=CARTESIAN_POINT('Origin',(-0.196206385030984,2.41068903913982,-0.0181194093584404));
#114808=CARTESIAN_POINT('Ctrl Pts',(7.461800912,2.361474582,0.755994149));
#114809=CARTESIAN_POINT('Ctrl Pts',(7.486050472,2.323357812,0.516646541000001));
#114810=CARTESIAN_POINT('Ctrl Pts',(7.494911153,2.285714286,0.276236876));
#114811=CARTESIAN_POINT('Ctrl Pts',(7.501216611,2.258926311,0.105155986));
#114812=CARTESIAN_POINT('Ctrl Pts',(7.499709291,2.231887255,-0.066034427));
#114813=CARTESIAN_POINT('Ctrl Pts',(7.18522749100001,2.361474582,0.96695703));
#114814=CARTESIAN_POINT('Ctrl Pts',(7.216243979,2.323357812,0.736480897));
#114815=CARTESIAN_POINT('Ctrl Pts',(7.23242622,2.285714286,0.5044908));
#114816=CARTESIAN_POINT('Ctrl Pts',(7.243941865,2.258926311,0.339401464));
#114817=CARTESIAN_POINT('Ctrl Pts',(7.247912692,2.231887255,0.173958629));
#114818=CARTESIAN_POINT('',(7.2477970451692,2.23266407429643,0.178711971874644));
#114819=CARTESIAN_POINT('Ctrl Pts',(7.24779704645978,2.23266407497284,0.178711971795929));
#114820=CARTESIAN_POINT('Ctrl Pts',(7.24511114718299,2.25046493769331,0.287640621109034));
#114821=CARTESIAN_POINT('Ctrl Pts',(7.23997384111706,2.26815682588451,0.396287419958082));
#114822=CARTESIAN_POINT('Ctrl Pts',(7.23242622039952,2.2857142860497,0.504490799940314));
#114823=CARTESIAN_POINT('Ctrl Pts',(7.2216769093882,2.31071959743364,0.658593914725088));
#114824=CARTESIAN_POINT('Ctrl Pts',(7.20595855182678,2.33599777477318,0.812909454265743));
#114825=CARTESIAN_POINT('Ctrl Pts',(7.18522749238694,2.36147458029557,0.966957019694019));
#114826=CARTESIAN_POINT('Ctrl Pts',(7.49768896349729,2.27159573034331,0.186172514983504));
#114827=CARTESIAN_POINT('Ctrl Pts',(7.45600386576791,2.26541917068799,0.184824874870608));
#114828=CARTESIAN_POINT('Ctrl Pts',(7.41431513363566,2.25909150511074,0.183525596002686));
#114829=CARTESIAN_POINT('Ctrl Pts',(7.33103228497458,2.24612512496663,0.181035935895053));
#114830=CARTESIAN_POINT('Ctrl Pts',(7.28938845439867,2.23947867582963,0.179844061553129));
#114831=CARTESIAN_POINT('Ctrl Pts',(7.24779704649391,2.23266407474667,0.178711970411905));
#114832=CARTESIAN_POINT('Ctrl Pts',(7.487346326,2.231898283,0.435482491));
#114833=CARTESIAN_POINT('Ctrl Pts',(7.51092572300001,2.296352134,0.030076714));
#114834=CARTESIAN_POINT('Ctrl Pts',(7.49059384,2.361474582,-0.375504901));
#114835=CARTESIAN_POINT('Ctrl Pts',(7.247680585,2.231898283,0.183374327));
#114836=CARTESIAN_POINT('Ctrl Pts',(7.257609471,2.296352134,-0.209054639));
#114837=CARTESIAN_POINT('Ctrl Pts',(7.225108044,2.361474582,-0.600261405));
#114838=CARTESIAN_POINT('Origin',(-0.195514704584165,2.41068902671274,0.024482796679206));
#114839=CARTESIAN_POINT('Ctrl Pts',(7.449864548,2.361474582,-0.865747201));
#114840=CARTESIAN_POINT('Ctrl Pts',(7.422094506,2.323357812,-1.104711934));
#114841=CARTESIAN_POINT('Ctrl Pts',(7.379067058,2.285714286,-1.341405739));
#114842=CARTESIAN_POINT('Ctrl Pts',(7.348447764,2.258926311,-1.509842339));
#114843=CARTESIAN_POINT('Ctrl Pts',(7.310174806,2.231887255,-1.676706386));
#114844=CARTESIAN_POINT('Ctrl Pts',(7.22510804400001,2.361474582,-0.600261405));
#114845=CARTESIAN_POINT('Ctrl Pts',(7.205853827,2.323357812,-0.832016762));
#114846=CARTESIAN_POINT('Ctrl Pts',(7.171786724,2.285714286,-1.062061763));
#114847=CARTESIAN_POINT('Ctrl Pts',(7.147543812,2.258926311,-1.225766926));
#114848=CARTESIAN_POINT('Ctrl Pts',(7.115856484,2.231887255,-1.38819541));
#114849=CARTESIAN_POINT('',(7.11676536944114,2.23266407431948,-1.38352833649661));
#114850=CARTESIAN_POINT('Ctrl Pts',(7.11676537048806,2.23266407505902,-1.38352833682321));
#114851=CARTESIAN_POINT('Ctrl Pts',(7.13755870587416,2.25046493778714,-1.27656898971806));
#114852=CARTESIAN_POINT('Ctrl Pts',(7.15589735726919,2.26815682595888,-1.16935792323182));
#114853=CARTESIAN_POINT('Ctrl Pts',(7.17178672398835,2.28571428598712,-1.06206176307869));
#114854=CARTESIAN_POINT('Ctrl Pts',(7.19441633923325,2.31071959711604,-0.909250710690481));
#114855=CARTESIAN_POINT('Ctrl Pts',(7.21223874829608,2.33599777471621,-0.755163999525554));
#114856=CARTESIAN_POINT('Ctrl Pts',(7.22510804314739,2.36147458031212,-0.600261415262548));
#114857=CARTESIAN_POINT('Ctrl Pts',(7.36241874941791,2.27159573033712,-1.42996159172988));
#114858=CARTESIAN_POINT('Ctrl Pts',(7.32141852321828,2.26541917064899,-1.42231666083323));
#114859=CARTESIAN_POINT('Ctrl Pts',(7.28042514401651,2.25909150509139,-1.4146237181863));
#114860=CARTESIAN_POINT('Ctrl Pts',(7.19855320613131,2.2461249677874,-1.39915163326171));
#114861=CARTESIAN_POINT('Ctrl Pts',(7.15762729706395,2.23947859868821,-1.39136354853802));
#114862=CARTESIAN_POINT('Ctrl Pts',(7.11676537024756,2.23266407490757,-1.38352833763891));
#114863=CARTESIAN_POINT('Ctrl Pts',(7.405912192,2.231898283,-1.184256983));
#114864=CARTESIAN_POINT('Ctrl Pts',(7.341790058,2.296352134,-1.585253472));
#114865=CARTESIAN_POINT('Ctrl Pts',(7.234745464,2.361474582,-1.97698206));
#114866=CARTESIAN_POINT('Ctrl Pts',(7.1176539,2.231898283,-1.378949948));
#114867=CARTESIAN_POINT('Ctrl Pts',(7.042990027,2.296352134,-1.764338561));
#114868=CARTESIAN_POINT('Ctrl Pts',(6.92715057400001,2.361474582,-2.139412284));
#114869=CARTESIAN_POINT('Origin',(-0.185680398792335,2.41068904855154,0.0659402369516504));
#114870=CARTESIAN_POINT('Ctrl Pts',(7.089580798,2.361474582,-2.447007174));
#114871=CARTESIAN_POINT('Ctrl Pts',(7.011089651,2.323357812,-2.674415306));
#114872=CARTESIAN_POINT('Ctrl Pts',(6.918185988,2.285714286,-2.896325712));
#114873=CARTESIAN_POINT('Ctrl Pts',(6.852073667,2.258926311,-3.054242115));
#114874=CARTESIAN_POINT('Ctrl Pts',(6.778824671,2.231887255,-3.208977419));
#114875=CARTESIAN_POINT('Ctrl Pts',(6.927150574,2.361474582,-2.139412284));
#114876=CARTESIAN_POINT('Ctrl Pts',(6.85852596,2.323357812,-2.361610241));
#114877=CARTESIAN_POINT('Ctrl Pts',(6.775802451,2.285714286,-2.578953498));
#114878=CARTESIAN_POINT('Ctrl Pts',(6.716934554,2.258926311,-2.733619816));
#114879=CARTESIAN_POINT('Ctrl Pts',(6.651070736,2.231887255,-2.885438973));
#114880=CARTESIAN_POINT('',(6.65296165417311,2.23266407429542,-2.88107639695278));
#114881=CARTESIAN_POINT('Ctrl Pts',(6.65296165572569,2.2326640749522,-2.88107639774204));
#114882=CARTESIAN_POINT('Ctrl Pts',(6.69626195237868,2.25046493781858,-2.78108765271941));
#114883=CARTESIAN_POINT('Ctrl Pts',(6.7372190663883,2.26815682601796,-2.68032538955622));
#114884=CARTESIAN_POINT('Ctrl Pts',(6.77580245113989,2.28571428600938,-2.5789534982117));
#114885=CARTESIAN_POINT('Ctrl Pts',(6.83075285835864,2.31071959717538,-2.43457978113306));
#114886=CARTESIAN_POINT('Ctrl Pts',(6.88128267700351,2.33599777462944,-2.28792682359601));
#114887=CARTESIAN_POINT('Ctrl Pts',(6.92715057096117,2.36147458031212,-2.13941229383932));
#114888=CARTESIAN_POINT('Ctrl Pts',(6.88289001768539,2.2715957303853,-2.97923228418401));
#114889=CARTESIAN_POINT('Ctrl Pts',(6.84449178839268,2.26541917071604,-2.96295225085749));
#114890=CARTESIAN_POINT('Ctrl Pts',(6.80611056655863,2.25909150509519,-2.94662680000792));
#114891=CARTESIAN_POINT('Ctrl Pts',(6.72947874958299,2.24612496091193,-2.91391637996682));
#114892=CARTESIAN_POINT('Ctrl Pts',(6.69118389512109,2.23947859526083,-2.89751252473308));
#114893=CARTESIAN_POINT('Ctrl Pts',(6.65296165534006,2.23266407482084,-2.88107639831275));
#114894=CARTESIAN_POINT('Ctrl Pts',(6.978185836,2.231898283,-2.748621917));
#114895=CARTESIAN_POINT('Ctrl Pts',(6.82936045,2.296352134,-3.126458967));
#114896=CARTESIAN_POINT('Ctrl Pts',(6.640608432,2.361474582,-3.486017736));
#114897=CARTESIAN_POINT('Ctrl Pts',(6.65481363,2.231898283,-2.876796057));
#114898=CARTESIAN_POINT('Ctrl Pts',(6.499048197,2.296352134,-3.237123972));
#114899=CARTESIAN_POINT('Ctrl Pts',(6.305287243,2.361474582,-3.578526622));
#114900=CARTESIAN_POINT('Origin',(-0.167164222466163,2.41068902856424,0.104314448275361));
#114901=CARTESIAN_POINT('Ctrl Pts',(6.397796129,2.361474582,-3.913847811));
#114902=CARTESIAN_POINT('Ctrl Pts',(6.272254035,2.323357812,-4.119065991));
#114903=CARTESIAN_POINT('Ctrl Pts',(6.133818231,2.285714286,-4.315816714));
#114904=CARTESIAN_POINT('Ctrl Pts',(6.03530422,2.258926311,-4.455828924));
#114905=CARTESIAN_POINT('Ctrl Pts',(5.93050422900001,2.231887255,-4.59120023400001));
#114906=CARTESIAN_POINT('Ctrl Pts',(6.30528724300001,2.361474582,-3.578526622));
#114907=CARTESIAN_POINT('Ctrl Pts',(6.190501041,2.323357812,-3.780777451));
#114908=CARTESIAN_POINT('Ctrl Pts',(6.062989186,2.285714286,-3.975256234));
#114909=CARTESIAN_POINT('Ctrl Pts',(5.972248902,2.258926311,-4.113651681));
#114910=CARTESIAN_POINT('Ctrl Pts',(5.875288312,2.231887255,-4.247762617));
#114911=CARTESIAN_POINT('',(5.87807284653492,2.23266407431278,-4.24390852719617));
#114912=CARTESIAN_POINT('Ctrl Pts',(5.87807284777009,2.23266407494115,-4.24390852821457));
#114913=CARTESIAN_POINT('Ctrl Pts',(5.94185543176464,2.25046493763868,-4.1555657488572));
#114914=CARTESIAN_POINT('Ctrl Pts',(6.00351589915871,2.26815682584352,-4.06596382001813));
#114915=CARTESIAN_POINT('Ctrl Pts',(6.06298918606306,2.28571428599601,-3.97525623438882));
#114916=CARTESIAN_POINT('Ctrl Pts',(6.14769096577208,2.31071959740257,-3.84607060732515));
#114917=CARTESIAN_POINT('Ctrl Pts',(6.22856547567653,2.33599777468241,-3.71370873206035));
#114918=CARTESIAN_POINT('Ctrl Pts',(6.30528723791706,2.36147458031212,-3.57852663095604));
#114919=CARTESIAN_POINT('Ctrl Pts',(6.08152499814079,2.27159573036892,-4.38919738580205));
#114920=CARTESIAN_POINT('Ctrl Pts',(6.0475242237988,2.26541917066132,-4.36504348623608));
#114921=CARTESIAN_POINT('Ctrl Pts',(6.01354982319035,2.25909150506665,-4.34084888729227));
#114922=CARTESIAN_POINT('Ctrl Pts',(5.94574154086183,2.24612498991411,-4.29242975155489));
#114923=CARTESIAN_POINT('Ctrl Pts',(5.91186826160298,2.23947860946582,-4.26817708978734));
#114924=CARTESIAN_POINT('Ctrl Pts',(5.87807284692885,2.23266407475115,-4.24390852816372));
#114925=CARTESIAN_POINT('Ctrl Pts',(6.224167265,2.231898283,-4.184464345));
#114926=CARTESIAN_POINT('Ctrl Pts',(5.997597537,2.296352134,-4.521474716));
#114927=CARTESIAN_POINT('Ctrl Pts',(5.73596393,2.361474582,-4.832051096));
#114928=CARTESIAN_POINT('Ctrl Pts',(5.88080167,2.231898283,-4.240126379));
#114929=CARTESIAN_POINT('Ctrl Pts',(5.651218096,2.296352134,-4.558545065));
#114930=CARTESIAN_POINT('Ctrl Pts',(5.38859568799999,2.361474582,-4.850313032));
#114931=CARTESIAN_POINT('Origin',(-0.140831315020765,2.41068907822503,0.137810861324849));
#114932=CARTESIAN_POINT('Ctrl Pts',(5.406857624,2.361474582,-5.197681275));
#114933=CARTESIAN_POINT('Ctrl Pts',(5.240134792,2.323357812,-5.371113728));
#114934=CARTESIAN_POINT('Ctrl Pts',(5.062639951,2.285714286,-5.533504923));
#114935=CARTESIAN_POINT('Ctrl Pts',(4.936330656,2.258926311,-5.649066125));
#114936=CARTESIAN_POINT('Ctrl Pts',(4.804880001,2.231887255,-5.75874362900001));
#114937=CARTESIAN_POINT('Ctrl Pts',(5.388595688,2.361474582,-4.850313032));
#114938=CARTESIAN_POINT('Ctrl Pts',(5.233015174,2.323357812,-5.023159709));
#114939=CARTESIAN_POINT('Ctrl Pts',(5.066677286,2.285714286,-5.185680407));
#114940=CARTESIAN_POINT('Ctrl Pts',(4.948307528,2.258926311,-5.301333767));
#114941=CARTESIAN_POINT('Ctrl Pts',(4.824783936,2.231887255,-5.411465603));
#114942=CARTESIAN_POINT('',(4.82833188580182,2.23266407432321,-5.40830021117995));
#114943=CARTESIAN_POINT('Ctrl Pts',(4.82833188697985,2.23266407514971,-5.40830021270223));
#114944=CARTESIAN_POINT('Ctrl Pts',(4.90961435553651,2.25046493782872,-5.33573420872998));
#114945=CARTESIAN_POINT('Ctrl Pts',(4.98909500158218,2.26815682596581,-5.26148230116632));
#114946=CARTESIAN_POINT('Ctrl Pts',(5.06667728571463,2.28571428593542,-5.18568040727882));
#114947=CARTESIAN_POINT('Ctrl Pts',(5.17716987488111,2.31071959712958,-5.07772344732761));
#114948=CARTESIAN_POINT('Ctrl Pts',(5.28460747541412,2.33599777470134,-4.9658417475096));
#114949=CARTESIAN_POINT('Ctrl Pts',(5.38859568103647,2.36147458029396,-4.85031303973633));
#114950=CARTESIAN_POINT('Ctrl Pts',(4.99579462933249,2.27159573035622,-5.5939284962985));
#114951=CARTESIAN_POINT('Ctrl Pts',(4.96778114863446,2.26541917067387,-5.5630301401288));
#114952=CARTESIAN_POINT('Ctrl Pts',(4.93980217415092,2.25909150509699,-5.53209770567045));
#114953=CARTESIAN_POINT('Ctrl Pts',(4.88398774231265,2.24612495461544,-5.47023363762829));
#114954=CARTESIAN_POINT('Ctrl Pts',(4.85612008818721,2.23947859218347,-5.43926632584869));
#114955=CARTESIAN_POINT('Ctrl Pts',(4.82833188556729,2.23266407483626,-5.40830021364951));
#114956=CARTESIAN_POINT('Ctrl Pts',(5.179113551,2.231898283,-5.424645871));
#114957=CARTESIAN_POINT('Ctrl Pts',(4.88539363,2.296352134,-5.70507133300001));
#114958=CARTESIAN_POINT('Ctrl Pts',(4.563112129,2.361474582,-5.952143118));
#114959=CARTESIAN_POINT('Ctrl Pts',(4.831809961,2.231898283,-5.405193105));
#114960=CARTESIAN_POINT('Ctrl Pts',(4.539143318,2.296352134,-5.666813656));
#114961=CARTESIAN_POINT('Ctrl Pts',(4.219939387,2.361474582,-5.895304196));
#114962=CARTESIAN_POINT('Origin',(-0.107913617262737,2.41068904470201,0.164863647007863));
#114963=CARTESIAN_POINT('Ctrl Pts',(4.163100466,2.361474582,-6.238476938));
#114964=CARTESIAN_POINT('Ctrl Pts',(3.96299267,2.323357812,-6.372014157));
#114965=CARTESIAN_POINT('Ctrl Pts',(3.754738253,2.285714286,-6.492452591));
#114966=CARTESIAN_POINT('Ctrl Pts',(3.606539757,2.258926311,-6.578159272));
#114967=CARTESIAN_POINT('Ctrl Pts',(3.454584923,2.231887255,-6.657014572));
#114968=CARTESIAN_POINT('Ctrl Pts',(4.219939387,2.361474582,-5.895304196));
#114969=CARTESIAN_POINT('Ctrl Pts',(4.030839333,2.323357812,-6.030664602));
#114970=CARTESIAN_POINT('Ctrl Pts',(3.833453187,2.285714286,-6.153627927));
#114971=CARTESIAN_POINT('Ctrl Pts',(3.692988795,2.258926311,-6.241131377));
#114972=CARTESIAN_POINT('Ctrl Pts',(3.548678026,2.231887255,-6.322134471));
#114973=CARTESIAN_POINT('',(3.55282349234905,2.23266407432664,-6.31980578879384));
#114974=CARTESIAN_POINT('Ctrl Pts',(3.55282349310941,2.23266407512854,-6.3198057904137));
#114975=CARTESIAN_POINT('Ctrl Pts',(3.64780516867989,2.25046493775314,-6.26640966745086));
#114976=CARTESIAN_POINT('Ctrl Pts',(3.7413895667195,2.26815682589727,-6.21097971756903));
#114977=CARTESIAN_POINT('Ctrl Pts',(3.83345318643646,2.28571428589253,-6.15362792735106));
#114978=CARTESIAN_POINT('Ctrl Pts',(3.96457007518036,2.31071959710664,-6.07194758186058));
#114979=CARTESIAN_POINT('Ctrl Pts',(4.09354710207664,2.33599777463646,-5.98577752262925));
#114980=CARTESIAN_POINT('Ctrl Pts',(4.21993937862631,2.36147458031212,-5.89530420199401));
#114981=CARTESIAN_POINT('Ctrl Pts',(3.67646645566478,2.27159573037149,-6.53709372734915));
#114982=CARTESIAN_POINT('Ctrl Pts',(3.65575014805859,2.26541917073199,-6.50089568752884));
#114983=CARTESIAN_POINT('Ctrl Pts',(3.63507486542068,2.25909150510569,-6.46467178342126));
#114984=CARTESIAN_POINT('Ctrl Pts',(3.5938643406885,2.24612497056415,-6.39225569889695));
#114985=CARTESIAN_POINT('Ctrl Pts',(3.57330524632176,2.23947860000625,-6.35602161625964));
#114986=CARTESIAN_POINT('Ctrl Pts',(3.55282349163871,2.2326640748214,-6.31980579073514));
#114987=CARTESIAN_POINT('Ctrl Pts',(3.891890244,2.231898283,-6.41117698500001));
#114988=CARTESIAN_POINT('Ctrl Pts',(3.544754146,2.296352134,-6.621905155));
#114989=CARTESIAN_POINT('Ctrl Pts',(3.176894277,2.361474582,-6.793919543));
#114990=CARTESIAN_POINT('Ctrl Pts',(3.556888188,2.231898283,-6.317519008));
#114991=CARTESIAN_POINT('Ctrl Pts',(3.214823244,2.296352134,-6.510108339));
#114992=CARTESIAN_POINT('Ctrl Pts',(2.853963411,2.361474582,-6.664637488));
#114993=CARTESIAN_POINT('Origin',(-0.0699498367566476,2.41068901350358,
0.184207422519518));
#114994=CARTESIAN_POINT('Ctrl Pts',(2.724681357,2.361474582,-6.98756835400001));
#114995=CARTESIAN_POINT('Ctrl Pts',(2.500545415,2.323357812,-7.074966286));
#114996=CARTESIAN_POINT('Ctrl Pts',(2.271269168,2.285714286,-7.147820393));
#114997=CARTESIAN_POINT('Ctrl Pts',(2.108111067,2.258926311,-7.199665003));
#114998=CARTESIAN_POINT('Ctrl Pts',(1.942757295,2.231887255,-7.244010912));
#114999=CARTESIAN_POINT('Ctrl Pts',(2.853963411,2.361474582,-6.664637488));
#115000=CARTESIAN_POINT('Ctrl Pts',(2.640185925,2.323357812,-6.75618232100001));
#115001=CARTESIAN_POINT('Ctrl Pts',(2.420981077,2.285714286,-6.833838645));
#115002=CARTESIAN_POINT('Ctrl Pts',(2.264990009,2.258926311,-6.88910062));
#115003=CARTESIAN_POINT('Ctrl Pts',(2.106639876,2.231887255,-6.937187358));
#115004=CARTESIAN_POINT('',(2.11118902096935,2.23266407433893,-6.93580427183575));
#115005=CARTESIAN_POINT('Ctrl Pts',(2.11118902140619,2.23266407505294,-6.93580427367143));
#115006=CARTESIAN_POINT('Ctrl Pts',(2.2154286670018,2.25046493793859,-6.90407477398938));
#115007=CARTESIAN_POINT('Ctrl Pts',(2.31874091402043,2.26815682610242,-6.87005862536604));
#115008=CARTESIAN_POINT('Ctrl Pts',(2.42098107672611,2.28571428598661,-6.8338386454385));
#115009=CARTESIAN_POINT('Ctrl Pts',(2.5665913847569,2.31071959703924,-6.78225419630704));
#115010=CARTESIAN_POINT('Ctrl Pts',(2.71107701654516,2.33599777463872,-6.72582499334375));
#115011=CARTESIAN_POINT('Ctrl Pts',(2.85396340153355,2.36147458031212,-6.66463749205377));
#115012=CARTESIAN_POINT('Ctrl Pts',(2.18523079690101,2.27159573033634,-7.17459172099152));
#115013=CARTESIAN_POINT('Ctrl Pts',(2.17278033336348,2.2654191706762,-7.13478657730633));
#115014=CARTESIAN_POINT('Ctrl Pts',(2.16037549591216,2.25909150508723,-7.09496499356541));
#115015=CARTESIAN_POINT('Ctrl Pts',(2.13569578957734,2.24612498190645,-7.01538298196319));
#115016=CARTESIAN_POINT('Ctrl Pts',(2.12340660065055,2.23947860556987,-6.9755763973687));
#115017=CARTESIAN_POINT('Ctrl Pts',(2.11118902034456,2.23266407481316,-6.93580427345659));
#115018=CARTESIAN_POINT('Ctrl Pts',(2.422686474,2.231898283,-7.097928589));
#115019=CARTESIAN_POINT('Ctrl Pts',(2.038365897,2.296352134,-7.229106051));
#115020=CARTESIAN_POINT('Ctrl Pts',(1.64212838,2.361474582,-7.31801984));
#115021=CARTESIAN_POINT('Ctrl Pts',(2.115650277,2.231898283,-6.934444744));
#115022=CARTESIAN_POINT('Ctrl Pts',(1.740181607,2.296352134,-7.04899759200001));
#115023=CARTESIAN_POINT('Ctrl Pts',(1.354539278,2.361474582,-7.122339738));
#115024=CARTESIAN_POINT('Origin',(-0.0287152926699252,2.41068906715292,
0.194937925583135));
#115025=CARTESIAN_POINT('Ctrl Pts',(1.158859176,2.361474582,-7.40992884));
#115026=CARTESIAN_POINT('Ctrl Pts',(0.921175436,2.323357812,-7.447100854));
#115027=CARTESIAN_POINT('Ctrl Pts',(0.68159806,2.285714286,-7.468964057));
#115028=CARTESIAN_POINT('Ctrl Pts',(0.511109446,2.258926311,-7.48452240000001));
#115029=CARTESIAN_POINT('Ctrl Pts',(0.340088494,2.231887255,-7.492285353));
#115030=CARTESIAN_POINT('Ctrl Pts',(1.354539278,2.361474582,-7.12233973800001));
#115031=CARTESIAN_POINT('Ctrl Pts',(1.126080358,2.323357812,-7.165788463));
#115032=CARTESIAN_POINT('Ctrl Pts',(0.895306583,2.285714286,-7.194506663));
#115033=CARTESIAN_POINT('Ctrl Pts',(0.731082809,2.258926311,-7.214943176));
#115034=CARTESIAN_POINT('Ctrl Pts',(0.566097586,2.231887255,-7.227865074));
#115035=CARTESIAN_POINT('',(0.570837697299746,2.23266407433622,-7.22749225539564));
#115036=CARTESIAN_POINT('Ctrl Pts',(0.570837697322891,2.2326640750753,-7.22749225722226));
#115037=CARTESIAN_POINT('Ctrl Pts',(0.67946118151483,2.25046493771607,-7.21891301886173));
#115038=CARTESIAN_POINT('Ctrl Pts',(0.787670512609784,2.26815682588018,
-7.20790122760538));
#115039=CARTESIAN_POINT('Ctrl Pts',(0.895306582512715,2.28571428592052,
-7.19450666306064));
#115040=CARTESIAN_POINT('Ctrl Pts',(1.04860173579021,2.31071959723866,-7.17543014161265));
#115041=CARTESIAN_POINT('Ctrl Pts',(1.20183998314738,2.33599777462408,-7.15138036210171));
#115042=CARTESIAN_POINT('Ctrl Pts',(1.35453926788343,2.36147458031212,-7.12233973992399));
#115043=CARTESIAN_POINT('Ctrl Pts',(0.591816174293166,2.27159573037352,
-7.4766137796155));
#115044=CARTESIAN_POINT('Ctrl Pts',(0.588213725050591,2.26541917069486,
-7.43506277642082));
#115045=CARTESIAN_POINT('Ctrl Pts',(0.584659369354717,2.25909150512078,
-7.39350552607491));
#115046=CARTESIAN_POINT('Ctrl Pts',(0.577664433621786,2.24612496820187,
-7.31047860262288));
#115047=CARTESIAN_POINT('Ctrl Pts',(0.574219802158501,2.23947859887087,
-7.26896090857373));
#115048=CARTESIAN_POINT('Ctrl Pts',(0.570837696147924,2.23266407485203,
-7.22749225711022));
#115049=CARTESIAN_POINT('Ctrl Pts',(0.840200577,2.231898283,-7.45278894));
#115050=CARTESIAN_POINT('Ctrl Pts',(0.436665925,2.296352134,-7.498281983));
#115051=CARTESIAN_POINT('Ctrl Pts',(0.030578384,2.361474582,-7.49993766400001));
#115052=CARTESIAN_POINT('Ctrl Pts',(0.57548691,2.231898283,-7.22712355100001));
#115053=CARTESIAN_POINT('Ctrl Pts',(0.184171013,2.296352134,-7.258283552));
#115054=CARTESIAN_POINT('Ctrl Pts',(-0.208221606,2.361474582,-7.247009298));
#115055=CARTESIAN_POINT('Origin',(0.0138619466249593,2.41068905855906,0.196553253636468));
#115056=CARTESIAN_POINT('Ctrl Pts',(-0.461149972000001,2.361474582,-7.485809288));
#115057=CARTESIAN_POINT('Ctrl Pts',(-0.701267683,2.323357812,-7.47101726400001));
#115058=CARTESIAN_POINT('Ctrl Pts',(-0.939943815,2.285714286,-7.440867263));
#115059=CARTESIAN_POINT('Ctrl Pts',(-1.109791084,2.258926311,-7.419411849));
#115060=CARTESIAN_POINT('Ctrl Pts',(-1.278482467,2.231887255,-7.390228859));
#115061=CARTESIAN_POINT('Ctrl Pts',(-0.208221606,2.361474582,-7.247009298));
#115062=CARTESIAN_POINT('Ctrl Pts',(-0.440679476,2.323357812,-7.240330301));
#115063=CARTESIAN_POINT('Ctrl Pts',(-0.672231452,2.285714286,-7.218767545));
#115064=CARTESIAN_POINT('Ctrl Pts',(-0.837009012,2.258926311,-7.203423007));
#115065=CARTESIAN_POINT('Ctrl Pts',(-1.000914798,2.231887255,-7.180575852));
#115066=CARTESIAN_POINT('',(-0.996205363460386,2.23266407429648,-7.18123073377563));
#115067=CARTESIAN_POINT('Ctrl Pts',(-0.996205363775867,2.2326640749913,
-7.18123073522375));
#115068=CARTESIAN_POINT('Ctrl Pts',(-0.888277152906397,2.25046493778098,
-7.19620291315496));
#115069=CARTESIAN_POINT('Ctrl Pts',(-0.780230486021345,2.26815682597183,
-7.20871037895824));
#115070=CARTESIAN_POINT('Ctrl Pts',(-0.672231451769396,2.28571428607959,
-7.21876754526045));
#115071=CARTESIAN_POINT('Ctrl Pts',(-0.51841936674453,2.31071959735153,
-7.23309094942261));
#115072=CARTESIAN_POINT('Ctrl Pts',(-0.363593751971703,2.33599777473477,
-7.24254513359495));
#115073=CARTESIAN_POINT('Ctrl Pts',(-0.208221616445147,2.36147458028728,
-7.24700929769989));
#115074=CARTESIAN_POINT('Ctrl Pts',(-1.02927111432502,2.27159573037741,
-7.42903768812546));
#115075=CARTESIAN_POINT('Ctrl Pts',(-1.02385710290779,2.26541917069792,
-7.38768370412906));
#115076=CARTESIAN_POINT('Ctrl Pts',(-1.01839477945185,2.25909150513843,
-7.34633395778414));
#115077=CARTESIAN_POINT('Ctrl Pts',(-1.00737797669102,2.2461251250009,-7.2637454516772));
#115078=CARTESIAN_POINT('Ctrl Pts',(-1.00181692800756,2.2394786758839,-7.2224573914154));
#115079=CARTESIAN_POINT('Ctrl Pts',(-0.996205364803582,2.2326640748218,
-7.18123073508118));
#115080=CARTESIAN_POINT('Ctrl Pts',(-0.781572165,2.231898283,-7.459165164));
#115081=CARTESIAN_POINT('Ctrl Pts',(-1.18545206,2.296352134,-7.416846584));
#115082=CARTESIAN_POINT('Ctrl Pts',(-1.582401422,2.361474582,-7.331166738));
#115083=CARTESIAN_POINT('Ctrl Pts',(-0.991585586000001,2.231898283,-7.181870093));
#115084=CARTESIAN_POINT('Ctrl Pts',(-1.380451213,2.296352134,-7.128180239));
#115085=CARTESIAN_POINT('Ctrl Pts',(-1.76124628,2.361474582,-7.032816757));
#115086=CARTESIAN_POINT('Origin',(0.0557910479257062,2.41068902562531,0.188978279005378));
#115087=CARTESIAN_POINT('Ctrl Pts',(-2.05959626,2.361474582,-7.211661615));
#115088=CARTESIAN_POINT('Ctrl Pts',(-2.290920304,2.323357812,-7.14559720900001));
#115089=CARTESIAN_POINT('Ctrl Pts',(-2.517534962,2.285714286,-7.064843786));
#115090=CARTESIAN_POINT('Ctrl Pts',(-2.678799016,2.258926311,-7.007377845));
#115091=CARTESIAN_POINT('Ctrl Pts',(-2.837273008,2.231887255,-6.942613476));
#115092=CARTESIAN_POINT('Ctrl Pts',(-1.76124628,2.361474582,-7.032816757));
#115093=CARTESIAN_POINT('Ctrl Pts',(-1.986833627,2.323357812,-6.976322341));
#115094=CARTESIAN_POINT('Ctrl Pts',(-2.208336691,2.285714286,-6.905486881));
#115095=CARTESIAN_POINT('Ctrl Pts',(-2.365963221,2.258926311,-6.855078784));
#115096=CARTESIAN_POINT('Ctrl Pts',(-2.521125518,2.231887255,-6.79753088400001));
#115097=CARTESIAN_POINT('',(-2.5166669678886,2.23266407430148,-6.79918284460187));
#115098=CARTESIAN_POINT('Ctrl Pts',(-2.51666696834917,2.23266407497599,
-6.79918284552874));
#115099=CARTESIAN_POINT('Ctrl Pts',(-2.41448063483361,2.25046493773397,
-6.83700635708861));
#115100=CARTESIAN_POINT('Ctrl Pts',(-2.31164877451872,2.2681568259284,-6.87244824524909));
#115101=CARTESIAN_POINT('Ctrl Pts',(-2.20833669139914,2.28571428594652,
-6.90548688094287));
#115102=CARTESIAN_POINT('Ctrl Pts',(-2.06119975667221,2.3107195970458,-6.95254046229072));
#115103=CARTESIAN_POINT('Ctrl Pts',(-1.91202624773585,2.33599777477677,
-6.99505654399887));
#115104=CARTESIAN_POINT('Ctrl Pts',(-1.76124628998941,2.36147458031212,
-7.03281675449832));
#115105=CARTESIAN_POINT('Ctrl Pts',(-2.60223082985633,2.27159573036453,
-7.03408805099112));
#115106=CARTESIAN_POINT('Ctrl Pts',(-2.58805351088558,2.26541917068779,
-6.99486475257262));
#115107=CARTESIAN_POINT('Ctrl Pts',(-2.57382992027057,2.25909150510029,
-6.95565597813173));
#115108=CARTESIAN_POINT('Ctrl Pts',(-2.54531627113145,2.24612497696501,
-6.87736573852533));
#115109=CARTESIAN_POINT('Ctrl Pts',(-2.53100969657328,2.23947860318275,
-6.83823890827247));
#115110=CARTESIAN_POINT('Ctrl Pts',(-2.51666696900843,2.23266407487449,
-6.79918284534824));
#115111=CARTESIAN_POINT('Ctrl Pts',(-2.366799461,2.231898283,-7.116759116));
#115112=CARTESIAN_POINT('Ctrl Pts',(-2.752139625,2.296352134,-6.988607681));
#115113=CARTESIAN_POINT('Ctrl Pts',(-3.121389897,2.361474582,-6.819598603));
#115114=CARTESIAN_POINT('Ctrl Pts',(-2.512292641,2.231898283,-6.800800371));
#115115=CARTESIAN_POINT('Ctrl Pts',(-2.880525075,2.296352134,-6.66477114200001));
#115116=CARTESIAN_POINT('Ctrl Pts',(-3.231917035,2.361474582,-6.489777522));
#115117=CARTESIAN_POINT('Origin',(0.0951113206744036,2.41068903468273,0.172566421100852));
#115118=CARTESIAN_POINT('Ctrl Pts',(-3.561738116,2.361474582,-6.600304659));
#115119=CARTESIAN_POINT('Ctrl Pts',(-3.773452038,2.323357812,-6.48605697100001));
#115120=CARTESIAN_POINT('Ctrl Pts',(-3.977408972,2.285714286,-6.358476065));
#115121=CARTESIAN_POINT('Ctrl Pts',(-4.122549284,2.258926311,-6.267686641));
#115122=CARTESIAN_POINT('Ctrl Pts',(-4.263395817,2.231887255,-6.170369204));
#115123=CARTESIAN_POINT('Ctrl Pts',(-3.231917035,2.361474582,-6.489777522));
#115124=CARTESIAN_POINT('Ctrl Pts',(-3.440085645,2.323357812,-6.386109302));
#115125=CARTESIAN_POINT('Ctrl Pts',(-3.641182561,2.285714286,-6.269313324));
#115126=CARTESIAN_POINT('Ctrl Pts',(-3.78428762,2.258926311,-6.18619869600001));
#115127=CARTESIAN_POINT('Ctrl Pts',(-3.923451211,2.231887255,-6.096640927));
#115128=CARTESIAN_POINT('',(-3.91945202178794,2.23266407430098,-6.09921272207512));
#115129=CARTESIAN_POINT('Ctrl Pts',(-3.91945202254244,2.23266407500049,
-6.09921272303784));
#115130=CARTESIAN_POINT('Ctrl Pts',(-3.82778568593043,2.25046493774357,
-6.15811898272353));
#115131=CARTESIAN_POINT('Ctrl Pts',(-3.73497693549523,2.26815682593041,
-6.214838069248));
#115132=CARTESIAN_POINT('Ctrl Pts',(-3.64118256128412,2.28571428597374,
-6.26931332395667));
#115133=CARTESIAN_POINT('Ctrl Pts',(-3.50760073483172,2.31071959716862,
-6.34689691106505));
#115134=CARTESIAN_POINT('Ctrl Pts',(-3.37105452079006,2.33599777477738,
-6.42048688524898));
#115135=CARTESIAN_POINT('Ctrl Pts',(-3.23191704421808,2.36147458031212,
-6.48977751740939));
#115136=CARTESIAN_POINT('Ctrl Pts',(-4.05351312369268,2.2715957303518,-6.31023227389436));
#115137=CARTESIAN_POINT('Ctrl Pts',(-4.03123541291977,2.26541917067448,
-6.27497369889219));
#115138=CARTESIAN_POINT('Ctrl Pts',(-4.00891563465973,2.25909150511891,
-6.23973925558646));
#115139=CARTESIAN_POINT('Ctrl Pts',(-3.96423904170362,2.24612512499576,
-6.1694097929572));
#115140=CARTESIAN_POINT('Ctrl Pts',(-3.94185556402805,2.23947867587992,
-6.13427278807419));
#115141=CARTESIAN_POINT('Ctrl Pts',(-3.9194520233861,2.23266407483665,-6.09921272249569));
#115142=CARTESIAN_POINT('Ctrl Pts',(-3.841357845,2.231898283,-6.44158132));
#115143=CARTESIAN_POINT('Ctrl Pts',(-4.190140199,2.296352134,-6.23358925));
#115144=CARTESIAN_POINT('Ctrl Pts',(-4.51442565,2.361474582,-5.989153617));
#115145=CARTESIAN_POINT('Ctrl Pts',(-3.915527685,2.231898283,-6.101732783));
#115146=CARTESIAN_POINT('Ctrl Pts',(-4.245908786,2.296352134,-5.88972475300001));
#115147=CARTESIAN_POINT('Ctrl Pts',(-4.551466941,2.361474582,-5.643283502));
#115148=CARTESIAN_POINT('Origin',(0.129984324614556,2.41068904740896,0.148085736443294));
#115149=CARTESIAN_POINT('Ctrl Pts',(-4.897337056,2.361474582,-5.680324793));
#115150=CARTESIAN_POINT('Ctrl Pts',(-5.079541349,2.323357812,-5.523235918));
#115151=CARTESIAN_POINT('Ctrl Pts',(-5.251303759,2.285714286,-5.35479307));
#115152=CARTESIAN_POINT('Ctrl Pts',(-5.373533729,2.258926311,-5.234925376));
#115153=CARTESIAN_POINT('Ctrl Pts',(-5.490166976,2.231887255,-5.109605325));
#115154=CARTESIAN_POINT('Ctrl Pts',(-4.551466941,2.361474582,-5.643283502));
#115155=CARTESIAN_POINT('Ctrl Pts',(-4.732483083,2.323357812,-5.49728889));
#115156=CARTESIAN_POINT('Ctrl Pts',(-4.903770781,2.285714286,-5.339993645));
#115157=CARTESIAN_POINT('Ctrl Pts',(-5.025662935,2.258926311,-5.228058833));
#115158=CARTESIAN_POINT('Ctrl Pts',(-5.142320686,2.231887255,-5.110678816));
#115159=CARTESIAN_POINT('',(-5.13896785483513,2.23266407435047,-5.11405019176887));
#115160=CARTESIAN_POINT('Ctrl Pts',(-5.13896785595135,2.23266407511824,
-5.11405019270273));
#115161=CARTESIAN_POINT('Ctrl Pts',(-5.0621077315837,2.25046493787097,-5.19128480983772));
#115162=CARTESIAN_POINT('Ctrl Pts',(-4.98366172519896,2.2681568260187,-5.26662897364023));
#115163=CARTESIAN_POINT('Ctrl Pts',(-4.90377078122153,2.28571428595199,
-5.3399936447995));
#115164=CARTESIAN_POINT('Ctrl Pts',(-4.78999020241981,2.31071959705392,
-5.44447951406395));
#115165=CARTESIAN_POINT('Ctrl Pts',(-4.67245603173986,2.3359977748075,-5.54570239561369));
#115166=CARTESIAN_POINT('Ctrl Pts',(-4.55146694901571,2.36147458031212,
-5.6432834955351));
#115167=CARTESIAN_POINT('Ctrl Pts',(-5.31525764932166,2.27159573038573,
-5.2913170492895));
#115168=CARTESIAN_POINT('Ctrl Pts',(-5.28592122760232,2.26541917071696,
-5.26167184967998));
#115169=CARTESIAN_POINT('Ctrl Pts',(-5.25654890930045,2.25909150511919,
-5.23205926051504));
#115170=CARTESIAN_POINT('Ctrl Pts',(-5.19779733318026,2.24612496134411,
-5.17297746284238));
#115171=CARTESIAN_POINT('Ctrl Pts',(-5.16838414603642,2.23947859552117,
-5.14347412631359));
#115172=CARTESIAN_POINT('Ctrl Pts',(-5.13896785724193,2.23266407489063,
-5.11405019171443));
#115173=CARTESIAN_POINT('Ctrl Pts',(-5.136298605,2.231898283,-5.465202342));
#115174=CARTESIAN_POINT('Ctrl Pts',(-5.432214475,2.296352134,-5.187095114));
#115175=CARTESIAN_POINT('Ctrl Pts',(-5.696371877,2.361474582,-4.878662465));
#115176=CARTESIAN_POINT('Ctrl Pts',(-5.135677006,2.231898283,-5.117354951));
#115177=CARTESIAN_POINT('Ctrl Pts',(-5.41275852000001,2.296352134,-4.83928138000001));
#115178=CARTESIAN_POINT('Ctrl Pts',(-5.658195312,2.361474582,-4.532915818));
#115179=CARTESIAN_POINT('Origin',(0.15877967775259,2.41068903813253,0.116681024699704));
#115180=CARTESIAN_POINT('Ctrl Pts',(-6.003941959,2.361474582,-4.494739253));
#115181=CARTESIAN_POINT('Ctrl Pts',(-6.14811695100001,2.323357812,-4.302154492));
#115182=CARTESIAN_POINT('Ctrl Pts',(-6.279653419,2.285714286,-4.100725903));
#115183=CARTESIAN_POINT('Ctrl Pts',(-6.373257709,2.258926311,-3.957384819));
#115184=CARTESIAN_POINT('Ctrl Pts',(-6.460224029,2.231887255,-3.80992198));
#115185=CARTESIAN_POINT('Ctrl Pts',(-5.658195312,2.361474582,-4.532915818));
#115186=CARTESIAN_POINT('Ctrl Pts',(-5.803594871,2.323357812,-4.351421359));
#115187=CARTESIAN_POINT('Ctrl Pts',(-5.93706413,2.285714286,-4.160981797));
#115188=CARTESIAN_POINT('Ctrl Pts',(-6.032043837,2.258926311,-4.025460749));
#115189=CARTESIAN_POINT('Ctrl Pts',(-6.120740961,2.231887255,-3.885747044));
#115190=CARTESIAN_POINT('',(-6.11819126292683,2.23266407432955,-3.88976035831329));
#115191=CARTESIAN_POINT('Ctrl Pts',(-6.11819126454179,2.23266407512976,
-3.8897603591851));
#115192=CARTESIAN_POINT('Ctrl Pts',(-6.05973124664646,2.25046493787191,
-3.98171192826723));
#115193=CARTESIAN_POINT('Ctrl Pts',(-5.99931603244148,2.26815682601324,
-4.07215815960735));
#115194=CARTESIAN_POINT('Ctrl Pts',(-5.93706413017151,2.28571428595903,
-4.16098179678812));
#115195=CARTESIAN_POINT('Ctrl Pts',(-5.84840505098194,2.31071959712034,
-4.2874843062922));
#115196=CARTESIAN_POINT('Ctrl Pts',(-5.75537869179094,2.33599777473392,
-4.41160702508984));
#115197=CARTESIAN_POINT('Ctrl Pts',(-5.65819531864777,2.36147458025728,
-4.53291580970195));
#115198=CARTESIAN_POINT('Ctrl Pts',(-6.32846663464899,2.27159573037118,
-4.02498572048494));
#115199=CARTESIAN_POINT('Ctrl Pts',(-6.2934432405714,2.26541917070497,-4.00234007259233));
#115200=CARTESIAN_POINT('Ctrl Pts',(-6.25839179936662,2.2590915051017,-3.97973398939621));
#115201=CARTESIAN_POINT('Ctrl Pts',(-6.18831295557712,2.24612496007342,
-3.93466333912423));
#115202=CARTESIAN_POINT('Ctrl Pts',(-6.15324509058793,2.23947859485753,
-3.9121727422877));
#115203=CARTESIAN_POINT('Ctrl Pts',(-6.11819126522844,2.23266407483229,
-3.88976035771312));
#115204=CARTESIAN_POINT('Ctrl Pts',(-6.191071751,2.231898283,-4.233276576));
#115205=CARTESIAN_POINT('Ctrl Pts',(-6.42028444,2.296352134,-3.898058176));
#115206=CARTESIAN_POINT('Ctrl Pts',(-6.61196208500001,2.361474582,-3.540050477));
#115207=CARTESIAN_POINT('Ctrl Pts',(-6.115687778,2.231898283,-3.893695289));
#115208=CARTESIAN_POINT('Ctrl Pts',(-6.326513683,2.296352134,-3.562558589));
#115209=CARTESIAN_POINT('Ctrl Pts',(-6.50035275900001,2.361474582,-3.210594028));
#115210=CARTESIAN_POINT('Origin',(0.180150236420007,2.4106890271346,0.0798200253204628));
#115211=CARTESIAN_POINT('Ctrl Pts',(-6.829809208,2.361474582,-3.098984701));
#115212=CARTESIAN_POINT('Ctrl Pts',(-6.929213439,2.323357812,-2.879909103));
#115213=CARTESIAN_POINT('Ctrl Pts',(-7.014373465,2.285714286,-2.65491335));
#115214=CARTESIAN_POINT('Ctrl Pts',(-7.074975242,2.258926311,-2.494801346));
#115215=CARTESIAN_POINT('Ctrl Pts',(-7.128208186,2.231887255,-2.332090918));
#115216=CARTESIAN_POINT('Ctrl Pts',(-6.50035275900001,2.361474582,-3.210594028));
#115217=CARTESIAN_POINT('Ctrl Pts',(-6.60333701300001,2.323357812,-3.002086202));
#115218=CARTESIAN_POINT('Ctrl Pts',(-6.692746959,2.285714286,-2.787407065));
#115219=CARTESIAN_POINT('Ctrl Pts',(-6.756373074,2.258926311,-2.634636595));
#115220=CARTESIAN_POINT('Ctrl Pts',(-6.812962191,2.231887255,-2.479122059));
#115221=CARTESIAN_POINT('',(-6.81133484766748,2.23266407431936,-2.48358965366023));
#115222=CARTESIAN_POINT('Ctrl Pts',(-6.8113348493112,2.23266407506945,-2.48358965412914));
#115223=CARTESIAN_POINT('Ctrl Pts',(-6.7740084640474,2.25046493778705,-2.58595862225407));
#115224=CARTESIAN_POINT('Ctrl Pts',(-6.73444899030339,2.26815682595422,
-2.68727775611435));
#115225=CARTESIAN_POINT('Ctrl Pts',(-6.69274695897743,2.2857142860095,-2.78740706505419));
#115226=CARTESIAN_POINT('Ctrl Pts',(-6.63335497939657,2.31071959724752,
-2.93001109840022));
#115227=CARTESIAN_POINT('Ctrl Pts',(-6.56918624068048,2.33599777467704,
-3.07122981342259));
#115228=CARTESIAN_POINT('Ctrl Pts',(-6.50035276356033,2.36147458031212,
-3.2105940187669));
#115229=CARTESIAN_POINT('Ctrl Pts',(-7.04576355357195,2.27159573036992,
-2.57045053283274));
#115230=CARTESIAN_POINT('Ctrl Pts',(-7.00669084185951,2.26541917066254,
-2.55586332198084));
#115231=CARTESIAN_POINT('Ctrl Pts',(-6.96759924437638,2.25909150507993,
-2.54132078029164));
#115232=CARTESIAN_POINT('Ctrl Pts',(-6.88947012216532,2.24612498904905,
-2.5123688015418));
#115233=CARTESIAN_POINT('Ctrl Pts',(-6.8503872175269,2.23947860905116,-2.49794254199318));
#115234=CARTESIAN_POINT('Ctrl Pts',(-6.81133484909264,2.23266407477659,
-2.48358965283265));
#115235=CARTESIAN_POINT('Ctrl Pts',(-6.956357263,2.231898283,-2.803407502));
#115236=CARTESIAN_POINT('Ctrl Pts',(-7.108149039,2.296352134,-2.42675237));
#115237=CARTESIAN_POINT('Ctrl Pts',(-7.218384296,2.361474582,-2.035909664));
#115238=CARTESIAN_POINT('Ctrl Pts',(-6.809735786,2.231898283,-2.487970763));
#115239=CARTESIAN_POINT('Ctrl Pts',(-6.944448097,2.296352134,-2.119254517));
#115240=CARTESIAN_POINT('Ctrl Pts',(-7.038560935,2.361474582,-1.73814843));
#115241=CARTESIAN_POINT('Origin',(0.193097256276927,2.41068906716603,0.0392268638322035));
#115242=CARTESIAN_POINT('Ctrl Pts',(-7.33632217,2.361474582,-1.558325069));
#115243=CARTESIAN_POINT('Ctrl Pts',(-7.386307607,2.323357812,-1.323002365));
#115244=CARTESIAN_POINT('Ctrl Pts',(-7.421109203,2.285714286,-1.08496));
#115245=CARTESIAN_POINT('Ctrl Pts',(-7.445874796,2.258926311,-0.915563734));
#115246=CARTESIAN_POINT('Ctrl Pts',(-7.462885252,2.231887255,-0.745213877));
#115247=CARTESIAN_POINT('Ctrl Pts',(-7.038560935,2.361474582,-1.73814843));
#115248=CARTESIAN_POINT('Ctrl Pts',(-7.094314455,2.323357812,-1.51237683));
#115249=CARTESIAN_POINT('Ctrl Pts',(-7.135484378,2.285714286,-1.283496277));
#115250=CARTESIAN_POINT('Ctrl Pts',(-7.164781814,2.258926311,-1.120619762));
#115251=CARTESIAN_POINT('Ctrl Pts',(-7.18661688100001,2.231887255,-0.956576082));
#115252=CARTESIAN_POINT('',(-7.18598798505211,2.23266407432236,-0.96128905722973));
#115253=CARTESIAN_POINT('Ctrl Pts',(-7.18598798657416,2.23266407502328,
-0.961289057317811));
#115254=CARTESIAN_POINT('Ctrl Pts',(-7.17154057331441,2.25046493780431,
-1.06928876573398));
#115255=CARTESIAN_POINT('Ctrl Pts',(-7.1546865971327,2.26815682598154,-1.17674323189176));
#115256=CARTESIAN_POINT('Ctrl Pts',(-7.13548437813034,2.28571428597987,
-1.28349627680228));
#115257=CARTESIAN_POINT('Ctrl Pts',(-7.10813660149529,2.31071959718438,
-1.43553382661598));
#115258=CARTESIAN_POINT('Ctrl Pts',(-7.07582594134178,2.33599777472798,
-1.58724530929748));
#115259=CARTESIAN_POINT('Ctrl Pts',(-7.03856093751762,2.36147458027879,
-1.73814841980497));
#115260=CARTESIAN_POINT('Ctrl Pts',(-7.43360839986752,2.2715957303976,-0.995723935096617));
#115261=CARTESIAN_POINT('Ctrl Pts',(-7.39231336732167,2.26541917070341,
-0.98987724314556));
#115262=CARTESIAN_POINT('Ctrl Pts',(-7.35100949311984,2.25909150512737,
-0.984078235985104));
#115263=CARTESIAN_POINT('Ctrl Pts',(-7.26848306530838,2.24612497315279,
-0.972598576198767));
#115264=CARTESIAN_POINT('Ctrl Pts',(-7.22721273214972,2.23947860128824,
-0.966911271517868));
#115265=CARTESIAN_POINT('Ctrl Pts',(-7.18598798672256,2.23266407482623,
-0.961289056131126));
#115266=CARTESIAN_POINT('Ctrl Pts',(-7.396371241,2.231898283,-1.24245421));
#115267=CARTESIAN_POINT('Ctrl Pts',(-7.46364449,2.296352134,-0.84197432));
#115268=CARTESIAN_POINT('Ctrl Pts',(-7.487282879,2.361474582,-0.436571978));
#115269=CARTESIAN_POINT('Ctrl Pts',(-7.185368118,2.231898283,-0.96591149));
#115270=CARTESIAN_POINT('Ctrl Pts',(-7.237667836,2.296352134,-0.57685646));
#115271=CARTESIAN_POINT('Ctrl Pts',(-7.247653825,2.361474582,-0.184428943));
#115272=CARTESIAN_POINT('Origin',(0.197015451126664,2.41068906325541,-0.00320043539546667));
#115273=CARTESIAN_POINT('Ctrl Pts',(-7.49979686,2.361474582,0.055200111));
#115274=CARTESIAN_POINT('Ctrl Pts',(-7.49802624,2.323357812,0.295766492));
#115275=CARTESIAN_POINT('Ctrl Pts',(-7.480842122,2.285714286,0.535724874));
#115276=CARTESIAN_POINT('Ctrl Pts',(-7.46861352000001,2.258926311,0.706484620000001));
#115277=CARTESIAN_POINT('Ctrl Pts',(-7.448606097,2.231887255,0.876508537));
#115278=CARTESIAN_POINT('Ctrl Pts',(-7.247653825,2.361474582,-0.184428943));
#115279=CARTESIAN_POINT('Ctrl Pts',(-7.253569639,2.323357812,0.048049601));
#115280=CARTESIAN_POINT('Ctrl Pts',(-7.244574478,2.285714286,0.28042937));
#115281=CARTESIAN_POINT('Ctrl Pts',(-7.238173321,2.258926311,0.445796006));
#115282=CARTESIAN_POINT('Ctrl Pts',(-7.224233354,2.231887255,0.61069833));
#115283=CARTESIAN_POINT('',(-7.2246323116338,2.23266407427139,0.605960348384108));
#115284=CARTESIAN_POINT('Ctrl Pts',(-7.22463231308464,2.23266407487673,
0.605960348605037));
#115285=CARTESIAN_POINT('Ctrl Pts',(-7.23373941730284,2.25046493768212,
0.497379846342098));
#115286=CARTESIAN_POINT('Ctrl Pts',(-7.24037901137527,2.26815682590636,
0.388814498640126));
#115287=CARTESIAN_POINT('Ctrl Pts',(-7.24457447820918,2.28571428599811,
0.280429370238197));
#115288=CARTESIAN_POINT('Ctrl Pts',(-7.25054965718974,2.31071959731194,
0.126067410023992));
#115289=CARTESIAN_POINT('Ctrl Pts',(-7.25160788627812,2.3359977747573,-0.0290429788908016));
#115290=CARTESIAN_POINT('Ctrl Pts',(-7.24765382527071,2.36147458025578,
-0.18442893236182));
#115291=CARTESIAN_POINT('Ctrl Pts',(-7.47386597901761,2.27159573040534,
0.625561607462204));
#115292=CARTESIAN_POINT('Ctrl Pts',(-7.43227953564301,2.26541917071843,
0.62239439562222));
#115293=CARTESIAN_POINT('Ctrl Pts',(-7.39069470784731,2.25909150510652,
0.619178713156272));
#115294=CARTESIAN_POINT('Ctrl Pts',(-7.30762990237436,2.24612497119073,
0.612649241444927));
#115295=CARTESIAN_POINT('Ctrl Pts',(-7.26610185095944,2.23947860030007,
0.60933167900063));
#115296=CARTESIAN_POINT('Ctrl Pts',(-7.22463231290839,2.23266407477602,
0.605960349071764));
#115297=CARTESIAN_POINT('Ctrl Pts',(-7.49053912,2.231898283,0.376594861));
#115298=CARTESIAN_POINT('Ctrl Pts',(-7.47014822,2.296352134,0.782173513));
#115299=CARTESIAN_POINT('Ctrl Pts',(-7.406084436,2.361474582,1.183179329));
#115300=CARTESIAN_POINT('Ctrl Pts',(-7.225020623,2.231898283,0.601312732));
#115301=CARTESIAN_POINT('Ctrl Pts',(-7.192462271,2.296352134,0.992514764));
#115302=CARTESIAN_POINT('Ctrl Pts',(-7.117854477,2.361474582,1.377914237));
#115303=CARTESIAN_POINT('Origin',(0.191721477608199,2.41068901772705,-0.045478126261897));
#115304=CARTESIAN_POINT('Ctrl Pts',(-7.312589385,2.361474582,1.666144196));
#115305=CARTESIAN_POINT('Ctrl Pts',(-7.2591455,2.323357812,1.900705638));
#115306=CARTESIAN_POINT('Ctrl Pts',(-7.190779179,2.285714286,2.131359848));
#115307=CARTESIAN_POINT('Ctrl Pts',(-7.142128177,2.258926311,2.295498538));
#115308=CARTESIAN_POINT('Ctrl Pts',(-7.086038399,2.231887255,2.457246386));
#115309=CARTESIAN_POINT('Ctrl Pts',(-7.117854477,2.361474582,1.377914237));
#115310=CARTESIAN_POINT('Ctrl Pts',(-7.073655968,2.323357812,1.606229286));
#115311=CARTESIAN_POINT('Ctrl Pts',(-7.014916327,2.285714286,1.831242452));
#115312=CARTESIAN_POINT('Ctrl Pts',(-6.973115887,2.258926311,1.991366848));
#115313=CARTESIAN_POINT('Ctrl Pts',(-6.92405270400001,2.231887255,2.149417167));
#115314=CARTESIAN_POINT('',(-6.92546085993488,2.232664074283,2.14487572022464));
#115315=CARTESIAN_POINT('Ctrl Pts',(-6.92546086172287,2.23266407495847,
2.14487572089392));
#115316=CARTESIAN_POINT('Ctrl Pts',(-6.95769664487577,2.25046493772654,
2.04079152850569));
#115317=CARTESIAN_POINT('Ctrl Pts',(-6.98751934933272,2.26815682591951,
1.93619169499266));
#115318=CARTESIAN_POINT('Ctrl Pts',(-7.0149163272947,2.28571428602102,1.8312424523213));
#115319=CARTESIAN_POINT('Ctrl Pts',(-7.05393506896648,2.31071959734436,
1.68177387550864));
#115320=CARTESIAN_POINT('Ctrl Pts',(-7.08831270552657,2.33599777462343,
1.53051737006403));
#115321=CARTESIAN_POINT('Ctrl Pts',(-7.11785447504281,2.36147458031212,
1.37791424711019));
#115322=CARTESIAN_POINT('Ctrl Pts',(-7.16465389193971,2.27159573037728,
2.21759658403499));
#115323=CARTESIAN_POINT('Ctrl Pts',(-7.12472057326613,2.26541917070527,
2.20556356386122));
#115324=CARTESIAN_POINT('Ctrl Pts',(-7.08479925216011,2.25909150510694,
2.19348355357122));
#115325=CARTESIAN_POINT('Ctrl Pts',(-7.0050800612742,2.24612496508977,2.16925024806764));
#115326=CARTESIAN_POINT('Ctrl Pts',(-6.96523611042108,2.23947859730079,
2.1570829508967));
#115327=CARTESIAN_POINT('Ctrl Pts',(-6.92546086106448,2.23266407478612,
2.14487572124463));
#115328=CARTESIAN_POINT('Ctrl Pts',(-7.234457715,2.231898283,1.978034774));
#115329=CARTESIAN_POINT('Ctrl Pts',(-7.127356121,2.296352134,2.369747783));
#115330=CARTESIAN_POINT('Ctrl Pts',(-6.978585717,2.361474582,2.747606485));
#115331=CARTESIAN_POINT('Ctrl Pts',(-6.926839193,2.231898283,2.140420238));
#115332=CARTESIAN_POINT('Ctrl Pts',(-6.810945164,2.296352134,2.515477101));
#115333=CARTESIAN_POINT('Ctrl Pts',(-6.655232165,2.361474582,2.875827678));
#115334=CARTESIAN_POINT('Origin',(0.177462767707922,2.41068904305774,-0.0856293542727959));
#115335=CARTESIAN_POINT('Ctrl Pts',(-6.783453358,2.361474582,3.19918123));
#115336=CARTESIAN_POINT('Ctrl Pts',(-6.680835185,2.323357812,3.4167699));
#115337=CARTESIAN_POINT('Ctrl Pts',(-6.564483393,2.285714286,3.627334805));
#115338=CARTESIAN_POINT('Ctrl Pts',(-6.481684858,2.258926311,3.777177496));
#115339=CARTESIAN_POINT('Ctrl Pts',(-6.392135422,2.231887255,3.923086125));
#115340=CARTESIAN_POINT('Ctrl Pts',(-6.655232165,2.361474582,2.875827678));
#115341=CARTESIAN_POINT('Ctrl Pts',(-6.562986005,2.323357812,3.089303476));
#115342=CARTESIAN_POINT('Ctrl Pts',(-6.457248486,2.285714286,3.296428672));
#115343=CARTESIAN_POINT('Ctrl Pts',(-6.382003305,2.258926311,3.44382359));
#115344=CARTESIAN_POINT('Ctrl Pts',(-6.30011104500001,2.231887255,3.587631646));
#115345=CARTESIAN_POINT('',(-6.30246255593898,2.23266407428407,3.58349908789824));
#115346=CARTESIAN_POINT('Ctrl Pts',(-6.30246255736635,2.23266407492913,
3.58349908883104));
#115347=CARTESIAN_POINT('Ctrl Pts',(-6.3563197106885,2.25046493770011,3.48877806770818));
#115348=CARTESIAN_POINT('Ctrl Pts',(-6.4079310492588,2.2681568259098,3.39303471968367));
#115349=CARTESIAN_POINT('Ctrl Pts',(-6.45724848585561,2.2857142859486,3.29642867228284));
#115350=CARTESIAN_POINT('Ctrl Pts',(-6.52748631567317,2.31071959719169,
3.15884246443922));
#115351=CARTESIAN_POINT('Ctrl Pts',(-6.5935759005777,2.33599777471149,3.01851242710723));
#115352=CARTESIAN_POINT('Ctrl Pts',(-6.65523216073996,2.36147458023972,
2.87582768785858));
#115353=CARTESIAN_POINT('Ctrl Pts',(-6.52043055152139,2.27159573038141,
3.7059392092535));
#115354=CARTESIAN_POINT('Ctrl Pts',(-6.48401759527572,2.26541917068676,
3.68560303129541));
#115355=CARTESIAN_POINT('Ctrl Pts',(-6.44762645771656,2.2590915050952,3.6652235410452));
#115356=CARTESIAN_POINT('Ctrl Pts',(-6.37498057901858,2.2461249788959,3.62441957076062));
#115357=CARTESIAN_POINT('Ctrl Pts',(-6.33868372537222,2.23947860406256,
3.6039714434621));
#115358=CARTESIAN_POINT('Ctrl Pts',(-6.30246255660136,2.23266407476234,
3.58349908877191));
#115359=CARTESIAN_POINT('Ctrl Pts',(-6.640101108,2.231898283,3.48698398));
#115360=CARTESIAN_POINT('Ctrl Pts',(-6.45129677200001,2.296352134,3.846515279));
#115361=CARTESIAN_POINT('Ctrl Pts',(-6.224776085,2.361474582,4.183558616));
#115362=CARTESIAN_POINT('Ctrl Pts',(-6.304766461,2.231898283,3.579444073));
#115363=CARTESIAN_POINT('Ctrl Pts',(-6.110955831,2.296352134,3.920818525));
#115364=CARTESIAN_POINT('Ctrl Pts',(-5.881418593,2.361474582,4.239270613));
#115365=CARTESIAN_POINT('Origin',(0.154905876767801,2.4106890658271,-0.121776562416487));
#115366=CARTESIAN_POINT('Ctrl Pts',(-5.937130591,2.361474582,4.582628105));
#115367=CARTESIAN_POINT('Ctrl Pts',(-5.790136441,2.323357812,4.773069799));
#115368=CARTESIAN_POINT('Ctrl Pts',(-5.631239659,2.285714286,4.953699618));
#115369=CARTESIAN_POINT('Ctrl Pts',(-5.518165158,2.258926311,5.082239832));
#115370=CARTESIAN_POINT('Ctrl Pts',(-5.399343297,2.231887255,5.20548671700001));
#115371=CARTESIAN_POINT('Ctrl Pts',(-5.881418593,2.361474582,4.239270613));
#115372=CARTESIAN_POINT('Ctrl Pts',(-5.745438112,2.323357812,4.427925268));
#115373=CARTESIAN_POINT('Ctrl Pts',(-5.597646882,2.285714286,4.607477551));
#115374=CARTESIAN_POINT('Ctrl Pts',(-5.492475341,2.258926311,4.73525096800001));
#115375=CARTESIAN_POINT('Ctrl Pts',(-5.381583195,2.231887255,4.858092456));
#115376=CARTESIAN_POINT('',(-5.38476810755608,2.23266407431186,4.85456202018608));
#115377=CARTESIAN_POINT('Ctrl Pts',(-5.38476810829647,2.23266407501123,
4.85456202100741));
#115378=CARTESIAN_POINT('Ctrl Pts',(-5.45772833098115,2.25046493773274,
4.77363322114774));
#115379=CARTESIAN_POINT('Ctrl Pts',(-5.52871501487491,2.26815682591559,
4.69122321183394));
#115380=CARTESIAN_POINT('Ctrl Pts',(-5.59764688191103,2.28571428597216,
4.6074775513424));
#115381=CARTESIAN_POINT('Ctrl Pts',(-5.69581955863213,2.3107195972295,4.48820709001268));
#115382=CARTESIAN_POINT('Ctrl Pts',(-5.79053081512901,2.33599777465455,
4.36536519804431));
#115383=CARTESIAN_POINT('Ctrl Pts',(-5.88141858688418,2.36147458028567,
4.23927062148488));
#115384=CARTESIAN_POINT('Ctrl Pts',(-5.57131912513177,2.27159573041001,
5.02099623658654));
#115385=CARTESIAN_POINT('Ctrl Pts',(-5.54012916098098,2.26541917075981,
4.99330779807958));
#115386=CARTESIAN_POINT('Ctrl Pts',(-5.50896981593093,2.25909150513737,
4.96558174989394));
#115387=CARTESIAN_POINT('Ctrl Pts',(-5.44679396116879,2.24612496979083,
4.91011499786757));
#115388=CARTESIAN_POINT('Ctrl Pts',(-5.4157414743458,2.23947859965913,4.8823422066781));
#115389=CARTESIAN_POINT('Ctrl Pts',(-5.3847681076767,2.23266407485813,4.85456202185309));
#115390=CARTESIAN_POINT('Ctrl Pts',(-5.735260753,2.231898283,4.832885691));
#115391=CARTESIAN_POINT('Ctrl Pts',(-5.473581956,2.296352134,5.143423997));
#115392=CARTESIAN_POINT('Ctrl Pts',(-5.179902842,2.361474582,5.423892195));
#115393=CARTESIAN_POINT('Ctrl Pts',(-5.387889857,2.231898283,4.851097081));
#115394=CARTESIAN_POINT('Ctrl Pts',(-5.125224996,2.296352134,5.142826832));
#115395=CARTESIAN_POINT('Ctrl Pts',(-4.83259642500001,2.361474582,5.404489966));
#115396=CARTESIAN_POINT('Origin',(0.125105786846226,2.41068905209741,-0.152229557512465));
#115397=CARTESIAN_POINT('Ctrl Pts',(-4.813194196,2.361474582,5.751796383));
#115398=CARTESIAN_POINT('Ctrl Pts',(-4.628697353,2.323357812,5.906186259));
#115399=CARTESIAN_POINT('Ctrl Pts',(-4.434685418,2.285714286,6.048434942));
#115400=CARTESIAN_POINT('Ctrl Pts',(-4.29662219,2.258926311,6.149662283));
#115401=CARTESIAN_POINT('Ctrl Pts',(-4.15408388,2.231887255,6.244484536));
#115402=CARTESIAN_POINT('Ctrl Pts',(-4.832596425,2.361474582,5.404489966));
#115403=CARTESIAN_POINT('Ctrl Pts',(-4.659239917,2.323357812,5.559502196));
#115404=CARTESIAN_POINT('Ctrl Pts',(-4.476305531,2.285714286,5.703085901));
#115405=CARTESIAN_POINT('Ctrl Pts',(-4.346125334,2.258926311,5.805263274));
#115406=CARTESIAN_POINT('Ctrl Pts',(-4.211418497,2.231887255,5.901394263));
#115407=CARTESIAN_POINT('',(-4.21528788729399,2.23266407432337,5.89863102775519));
#115408=CARTESIAN_POINT('Ctrl Pts',(-4.21528788838403,2.23266407510249,
5.89863102949945));
#115409=CARTESIAN_POINT('Ctrl Pts',(-4.30393964099989,2.25046493788637,
5.83527859085858));
#115410=CARTESIAN_POINT('Ctrl Pts',(-4.39098241129342,2.26815682603576,
5.77005532067875));
#115411=CARTESIAN_POINT('Ctrl Pts',(-4.4763055306873,2.28571428593814,5.70308590133612));
#115412=CARTESIAN_POINT('Ctrl Pts',(-4.59782260737445,2.31071959704973,
5.6077081405588));
#115413=CARTESIAN_POINT('Ctrl Pts',(-4.71672694388695,2.3359977746627,5.50809834397294));
#115414=CARTESIAN_POINT('Ctrl Pts',(-4.83259641732343,2.36147458031211,
5.40448997286425));
#115415=CARTESIAN_POINT('Ctrl Pts',(-4.36169900909674,2.27159573034486,
6.10127705920046));
#115416=CARTESIAN_POINT('Ctrl Pts',(-4.33719044449114,2.26541917064638,
6.0675310404069));
#115417=CARTESIAN_POINT('Ctrl Pts',(-4.3127198683797,2.25909150506767,6.03375487391214));
#115418=CARTESIAN_POINT('Ctrl Pts',(-4.26392139898229,2.24612497942368,
5.96621898333419));
#115419=CARTESIAN_POINT('Ctrl Pts',(-4.23956521153354,2.23947860431857,
5.93242011068925));
#115420=CARTESIAN_POINT('Ctrl Pts',(-4.21528788699178,2.2326640747801,5.89863102936508));
#115421=CARTESIAN_POINT('Ctrl Pts',(-4.56224597900001,2.231898283,5.952807038));
#115422=CARTESIAN_POINT('Ctrl Pts',(-4.23992853,2.296352134,6.19983192400001));
#115423=CARTESIAN_POINT('Ctrl Pts',(-3.892823099,2.361474582,6.410610604));
#115424=CARTESIAN_POINT('Ctrl Pts',(-4.219081511,2.231898283,5.89591818099999));
#115425=CARTESIAN_POINT('Ctrl Pts',(-3.899844336,2.296352134,6.124362272));
#115426=CARTESIAN_POINT('Ctrl Pts',(-3.557807419,2.361474582,6.317001375));
#115427=CARTESIAN_POINT('Origin',(0.089456009380211,2.41068903096621,-0.17556451321962));
#115428=CARTESIAN_POINT('Ctrl Pts',(-3.46419819,2.361474582,6.652017055));
#115429=CARTESIAN_POINT('Ctrl Pts',(-3.250825521,2.323357812,6.763136014));
#115430=CARTESIAN_POINT('Ctrl Pts',(-3.030770215,2.285714286,6.86035217));
#115431=CARTESIAN_POINT('Ctrl Pts',(-2.874173942,2.258926311,6.929533359));
#115432=CARTESIAN_POINT('Ctrl Pts',(-2.714584117,2.231887255,6.991497198));
#115433=CARTESIAN_POINT('Ctrl Pts',(-3.557807419,2.361474582,6.31700137500001));
#115434=CARTESIAN_POINT('Ctrl Pts',(-3.355180843,2.323357812,6.43112298));
#115435=CARTESIAN_POINT('Ctrl Pts',(-3.145657109,2.285714286,6.532024292));
#115436=CARTESIAN_POINT('Ctrl Pts',(-2.996555338,2.258926311,6.603827921));
#115437=CARTESIAN_POINT('Ctrl Pts',(-2.84433255,2.231887255,6.668753433));
#115438=CARTESIAN_POINT('',(-2.84870549026514,2.23266407433,6.66688660531187));
#115439=CARTESIAN_POINT('Ctrl Pts',(-2.84870549087027,2.23266407513038,
6.66688660706084));
#115440=CARTESIAN_POINT('Ctrl Pts',(-2.94890351649421,2.25046493782023,
6.62407281963628));
#115441=CARTESIAN_POINT('Ctrl Pts',(-3.04793235054105,2.26815682595923,
6.57908605560133));
#115442=CARTESIAN_POINT('Ctrl Pts',(-3.14565710867187,2.28571428595922,
6.53202429239836));
#115443=CARTESIAN_POINT('Ctrl Pts',(-3.28483658331461,2.31071959718301,
6.46499899052546));
#115444=CARTESIAN_POINT('Ctrl Pts',(-3.42237416391989,2.33599777470832,
6.3932789329289));
#115445=CARTESIAN_POINT('Ctrl Pts',(-3.5578074100273,2.36147458031211,6.31700138005354));
#115446=CARTESIAN_POINT('Ctrl Pts',(-2.9481306941972,2.27159573037685,6.89626894828925));
#115447=CARTESIAN_POINT('Ctrl Pts',(-2.93144952302019,2.26541917074977,
6.85804327622383));
#115448=CARTESIAN_POINT('Ctrl Pts',(-2.9148119327911,2.25909150512727,6.81979632704012));
#115449=CARTESIAN_POINT('Ctrl Pts',(-2.88167293465899,2.24612512420583,
6.74335001312441));
#115450=CARTESIAN_POINT('Ctrl Pts',(-2.86515174144512,2.2394786754138,6.7051050243239));
#115451=CARTESIAN_POINT('Ctrl Pts',(-2.84870548936965,2.23266407486858,
6.66688660775785));
#115452=CARTESIAN_POINT('Ctrl Pts',(-3.175905654,2.231898283,6.79438174400001));
#115453=CARTESIAN_POINT('Ctrl Pts',(-2.808020759,2.296352134,6.966342602));
#115454=CARTESIAN_POINT('Ctrl Pts',(-2.423719275,2.361474582,7.097575986));
#115455=CARTESIAN_POINT('Ctrl Pts',(-2.852993603,2.231898283,6.665052701));
#115456=CARTESIAN_POINT('Ctrl Pts',(-2.492111289,2.296352134,6.819529339));
#115457=CARTESIAN_POINT('Ctrl Pts',(-2.116659292,2.361474582,6.93413682));
#115458=CARTESIAN_POINT('Origin',(0.0496234282576166,2.4106890156939,-0.190690422859716));
#115459=CARTESIAN_POINT('Ctrl Pts',(-1.953220126,2.361474582,7.241196803));
#115460=CARTESIAN_POINT('Ctrl Pts',(-1.720948701,2.323357812,7.303849046));
#115461=CARTESIAN_POINT('Ctrl Pts',(-1.485139566,2.285714286,7.351486956));
#115462=CARTESIAN_POINT('Ctrl Pts',(-1.317332516,2.258926311,7.385387158));
#115463=CARTESIAN_POINT('Ctrl Pts',(-1.148153419,2.231887255,7.411595221));
#115464=CARTESIAN_POINT('Ctrl Pts',(-2.116659292,2.361474582,6.93413682));
#115465=CARTESIAN_POINT('Ctrl Pts',(-1.894237241,2.323357812,7.002031601));
#115466=CARTESIAN_POINT('Ctrl Pts',(-1.667921256,2.285714286,7.055532488));
#115467=CARTESIAN_POINT('Ctrl Pts',(-1.506869744,2.258926311,7.093604914));
#115468=CARTESIAN_POINT('Ctrl Pts',(-1.344248775,2.231887255,7.124289104));
#115469=CARTESIAN_POINT('',(-1.34892079077827,2.23266407431317,7.12340597438253));
#115470=CARTESIAN_POINT('Ctrl Pts',(-1.34892079104794,2.2326640750857,7.12340597648489));
#115471=CARTESIAN_POINT('Ctrl Pts',(-1.45597994114529,2.25046493783544,
7.10313276514847));
#115472=CARTESIAN_POINT('Ctrl Pts',(-1.56236436026021,2.26815682598767,
7.08048603900714));
#115473=CARTESIAN_POINT('Ctrl Pts',(-1.66792125556938,2.28571428593661,
7.05553248817024));
#115474=CARTESIAN_POINT('Ctrl Pts',(-1.81825525022986,2.3107195971373,7.01999367250149));
#115475=CARTESIAN_POINT('Ctrl Pts',(-1.96799497131678,2.33599777477943,
6.97951690438721));
#115476=CARTESIAN_POINT('Ctrl Pts',(-2.11665928215075,2.36147458031212,
6.9341368230065));
#115477=CARTESIAN_POINT('Ctrl Pts',(-1.3967110656066,2.27159573036363,7.36879896579079));
#115478=CARTESIAN_POINT('Ctrl Pts',(-1.38863728042462,2.26541917071644,
7.32788102979332));
#115479=CARTESIAN_POINT('Ctrl Pts',(-1.38061063127253,2.25909150509517,
7.28695168286009));
#115480=CARTESIAN_POINT('Ctrl Pts',(-1.3646799069082,2.24612496514739,7.20516773311084));
#115481=CARTESIAN_POINT('Ctrl Pts',(-1.3567666176599,2.23947859731389,7.16426585760438));
#115482=CARTESIAN_POINT('Ctrl Pts',(-1.34892078967418,2.23266407477031,
7.12340597607662));
#115483=CARTESIAN_POINT('Ctrl Pts',(-1.64106351,2.231898283,7.31825871100001));
#115484=CARTESIAN_POINT('Ctrl Pts',(-1.244813059,2.296352134,7.407114842));
#115485=CARTESIAN_POINT('Ctrl Pts',(-0.841285031,2.361474582,7.452666603));
#115486=CARTESIAN_POINT('Ctrl Pts',(-1.353502885,2.231898283,7.122536763));
#115487=CARTESIAN_POINT('Ctrl Pts',(-0.967849888,2.296352134,7.195822793));
#115488=CARTESIAN_POINT('Ctrl Pts',(-0.576538529,2.361474582,7.227039735));
#115489=CARTESIAN_POINT('Origin',(0.00747050078381883,2.41068901051413,
-0.196900006855639));
#115490=CARTESIAN_POINT('Ctrl Pts',(-0.350911661,2.361474582,7.491786236));
#115491=CARTESIAN_POINT('Ctrl Pts',(-0.110602232,2.323357812,7.503042214));
#115492=CARTESIAN_POINT('Ctrl Pts',(0.129934559,2.285714286,7.498874383));
#115493=CARTESIAN_POINT('Ctrl Pts',(0.301105915,2.258926311,7.495908461));
#115494=CARTESIAN_POINT('Ctrl Pts',(0.471963657,2.231887255,7.48513529));
#115495=CARTESIAN_POINT('Ctrl Pts',(-0.576538529,2.361474582,7.22703973500001));
#115496=CARTESIAN_POINT('Ctrl Pts',(-0.344721211,2.323357812,7.245533007));
#115497=CARTESIAN_POINT('Ctrl Pts',(-0.112195259,2.285714286,7.249131826));
#115498=CARTESIAN_POINT('Ctrl Pts',(0.053275404,2.258926311,7.251692825));
#115499=CARTESIAN_POINT('Ctrl Pts',(0.218690579,2.231887255,7.246700934));
#115500=CARTESIAN_POINT('Ctrl Pts',(0.213937951383149,2.23266407437781,
7.24684279994555));
#115501=CARTESIAN_POINT('Ctrl Pts',(0.105023643191308,2.25046493706875,
7.25005811733432));
#115502=CARTESIAN_POINT('Ctrl Pts',(-0.00374194605548129,2.26815682549406,
7.25081036438579));
#115503=CARTESIAN_POINT('Ctrl Pts',(-0.112195259309469,2.28571428606866,
7.24913182611169));
#115504=CARTESIAN_POINT('Ctrl Pts',(-0.266654322558138,2.31071959712748,
7.24674125320845));
#115505=CARTESIAN_POINT('Ctrl Pts',(-0.4215945208895,2.3359977747927,7.23940042340816));
#115506=CARTESIAN_POINT('Ctrl Pts',(-0.576538518734711,2.36147458031212,
7.22703973581892));
#115507=CARTESIAN_POINT('Ctrl Pts',(-1.36436745820684,3.52436392548355,
7.12046798599309));
#115508=CARTESIAN_POINT('Ctrl Pts',(-1.36047186710342,3.52502192024177,
7.12121001099655));
#115509=CARTESIAN_POINT('Ctrl Pts',(-1.356576276,3.525679915,7.121952036));
#115510=CARTESIAN_POINT('Ctrl Pts',(-0.967402251,3.591414347,7.196081186));
#115511=CARTESIAN_POINT('Ctrl Pts',(-0.572468102,3.656498153,7.2273633));
#115512=CARTESIAN_POINT('Ctrl Pts',(-1.16908429046732,3.52436392548355,
7.40832702063338));
#115513=CARTESIAN_POINT('Ctrl Pts',(-1.16503136223366,3.52502192024177,
7.40896205681669));
#115514=CARTESIAN_POINT('Ctrl Pts',(-1.160978434,3.525679915,7.409597093));
#115515=CARTESIAN_POINT('Ctrl Pts',(-0.756086249,3.591414347,7.473037937));
#115516=CARTESIAN_POINT('Ctrl Pts',(-0.346692162,3.656498153,7.491982685));
#115517=CARTESIAN_POINT('',(-0.577160368164006,3.65572482702379,7.22699010131578));
#115518=CARTESIAN_POINT('Ctrl Pts',(-0.577160369470976,3.6557248264673,
7.22699010111248));
#115519=CARTESIAN_POINT('Ctrl Pts',(-0.58068380245636,3.64885401015902,
7.26844871272591));
#115520=CARTESIAN_POINT('Ctrl Pts',(-0.584188197121918,3.64214700170532,
7.30996068621342));
#115521=CARTESIAN_POINT('Ctrl Pts',(-0.591154981583553,3.62905099610467,
7.39298959490074));
#115522=CARTESIAN_POINT('Ctrl Pts',(-0.594621219303742,3.622654765003,7.43455243089213));
#115523=CARTESIAN_POINT('Ctrl Pts',(-0.598068334408679,3.6164059873883,
7.47611625530082));
#115524=CARTESIAN_POINT('Origin',(0.0440243728265652,3.48216462733526,-0.192296609468819));
#115525=CARTESIAN_POINT('Ctrl Pts',(-2.121755383,3.656505752,6.93257918100001));
#115526=CARTESIAN_POINT('Ctrl Pts',(-1.744320898,3.590992329,7.048095157));
#115527=CARTESIAN_POINT('Ctrl Pts',(-1.356576276,3.525679915,7.121952036));
#115528=CARTESIAN_POINT('Ctrl Pts',(-2.428935412,3.656505752,7.09579261));
#115529=CARTESIAN_POINT('Ctrl Pts',(-2.042615002,3.590992329,7.228032569));
#115530=CARTESIAN_POINT('Ctrl Pts',(-1.644221332,3.525679915,7.31754987800001));
#115531=CARTESIAN_POINT('',(-2.11725592263229,3.65572482705533,6.93395466884954));
#115532=CARTESIAN_POINT('Origin',(0.053364361895534,3.62499993732917,-0.192199315869914));
#115533=CARTESIAN_POINT('Ctrl Pts',(-2.1912298310443,3.61640598740892,7.17276179868612));
#115534=CARTESIAN_POINT('Ctrl Pts',(-2.17892831394179,3.62265476504301,
7.13291074101982));
#115535=CARTESIAN_POINT('Ctrl Pts',(-2.16660833371638,3.62905099621088,
7.09306475921216));
#115536=CARTESIAN_POINT('Ctrl Pts',(-2.14195551550789,3.64214708279692,
7.01347418081946));
#115537=CARTESIAN_POINT('Ctrl Pts',(-2.12960928518368,3.648854050219,6.97368633665899));
#115538=CARTESIAN_POINT('Ctrl Pts',(-2.11725592405794,3.65572482662799,
6.93395466915322));
#115539=CARTESIAN_POINT('Ctrl Pts',(-2.86315944180208,3.52436392548355,
6.6606967283916));
#115540=CARTESIAN_POINT('Ctrl Pts',(-2.85951444090104,3.52502192024177,
6.66225884219581));
#115541=CARTESIAN_POINT('Ctrl Pts',(-2.85586944,3.525679915,6.663820956));
#115542=CARTESIAN_POINT('Ctrl Pts',(-2.491729664,3.591414347,6.819877919));
#115543=CARTESIAN_POINT('Ctrl Pts',(-2.112753586,3.656498153,6.935327843));
#115544=CARTESIAN_POINT('Ctrl Pts',(-2.73432307002075,3.52436392548355,
6.98380588667783));
#115545=CARTESIAN_POINT('Ctrl Pts',(-2.73050141101038,3.52502192024177,
6.98529733583892));
#115546=CARTESIAN_POINT('Ctrl Pts',(-2.726679752,3.525679915,6.986788785));
#115547=CARTESIAN_POINT('Ctrl Pts',(-2.344891628,3.591414347,7.135786269));
#115548=CARTESIAN_POINT('Ctrl Pts',(-1.949141507,3.656498153,7.242295726));
#115549=CARTESIAN_POINT('Origin',(0.0843333478850994,3.48216454650792,-0.178337430489187));
#115550=CARTESIAN_POINT('Ctrl Pts',(-3.562449519,3.656505752,6.314384643));
#115551=CARTESIAN_POINT('Ctrl Pts',(-3.218671763,3.590992329,6.508337177));
#115552=CARTESIAN_POINT('Ctrl Pts',(-2.85586944,3.525679915,6.663820956));
#115553=CARTESIAN_POINT('Ctrl Pts',(-3.897533913,3.656505752,6.407747607));
#115554=CARTESIAN_POINT('Ctrl Pts',(-3.548673142,3.590992329,6.619943338));
#115555=CARTESIAN_POINT('Ctrl Pts',(-3.178837269,3.525679915,6.793010644));
#115556=CARTESIAN_POINT('',(-3.55835094254514,3.6557248270686,6.31669522457157));
#115557=CARTESIAN_POINT('Origin',(0.0934339420682495,3.62499996819879,-0.176234096549057));
#115558=CARTESIAN_POINT('Ctrl Pts',(-3.68193185676624,3.61640598737491,
6.53401697235091));
#115559=CARTESIAN_POINT('Ctrl Pts',(-3.66135114289402,3.62265476502698,
6.49774207271943));
#115560=CARTESIAN_POINT('Ctrl Pts',(-3.6407534887579,3.62905099620307,6.46147609934633));
#115561=CARTESIAN_POINT('Ctrl Pts',(-3.59956739575239,3.64214708992088,
6.38904589216658));
#115562=CARTESIAN_POINT('Ctrl Pts',(-3.57895661493682,3.64885405374133,
6.35284236110603));
#115563=CARTESIAN_POINT('Ctrl Pts',(-3.55835094491586,3.65572482666612,
6.31669522370334));
#115564=CARTESIAN_POINT('Ctrl Pts',(-4.22807327301959,3.52436392548355,
5.88947869519783));
#115565=CARTESIAN_POINT('Ctrl Pts',(-4.22484929850979,3.52502192024177,
5.89178785509892));
#115566=CARTESIAN_POINT('Ctrl Pts',(-4.221625324,3.525679915,5.894097015));
#115567=CARTESIAN_POINT('Ctrl Pts',(-3.899546568,3.591414347,6.124784741));
#115568=CARTESIAN_POINT('Ctrl Pts',(-3.554249061,3.656498153,6.319004163));
#115569=CARTESIAN_POINT('Ctrl Pts',(-4.17170794254552,3.52436392548355,
6.23272975173752));
#115570=CARTESIAN_POINT('Ctrl Pts',(-4.16829624927276,3.52502192024177,
6.23500787536876));
#115571=CARTESIAN_POINT('Ctrl Pts',(-4.164884556,3.525679915,6.23728599900001));
#115572=CARTESIAN_POINT('Ctrl Pts',(-3.82405248,3.591414347,6.464873166));
#115573=CARTESIAN_POINT('Ctrl Pts',(-3.460451162,3.656498153,6.653967069));
#115574=CARTESIAN_POINT('Origin',(0.120698810537666,3.48216456265301,-0.156038612835599));
#115575=CARTESIAN_POINT('Ctrl Pts',(-4.836567476,3.656505752,5.400936498));
#115576=CARTESIAN_POINT('Ctrl Pts',(-4.542521114,3.590992329,5.66425658500001));
#115577=CARTESIAN_POINT('Ctrl Pts',(-4.221625324,3.525679915,5.894097015));
#115578=CARTESIAN_POINT('Ctrl Pts',(-5.18388806,3.656505752,5.420083448));
#115579=CARTESIAN_POINT('Ctrl Pts',(-4.88879927000001,3.590992329,5.702312914));
#115580=CARTESIAN_POINT('Ctrl Pts',(-4.564814309,3.525679915,5.950837783));
#115581=CARTESIAN_POINT('',(-4.83306142853521,3.65572482707056,5.40407413172743));
#115582=CARTESIAN_POINT('Origin',(0.129134690010613,3.62499996686943,-0.152028384945294));
#115583=CARTESIAN_POINT('Ctrl Pts',(-5.00047084119201,3.61640598737593,
5.58974877456337));
#115584=CARTESIAN_POINT('Ctrl Pts',(-4.9725732618041,3.62265476502778,5.55874620709649));
#115585=CARTESIAN_POINT('Ctrl Pts',(-4.94466105705915,3.62905099620991,
5.52775599881448));
#115586=CARTESIAN_POINT('Ctrl Pts',(-4.88886753538952,3.64214708596028,
5.46587298098712));
#115587=CARTESIAN_POINT('Ctrl Pts',(-4.86095592515247,3.64885405180903,
5.43494656698116));
#115588=CARTESIAN_POINT('Ctrl Pts',(-4.83306143032981,3.65572482669157,
5.40407413074731));
#115589=CARTESIAN_POINT('Ctrl Pts',(-5.4082532696763,3.52114709502067,4.82846175061348));
#115590=CARTESIAN_POINT('Ctrl Pts',(-5.39911798483816,3.52341350501031,
4.8386166993068));
#115591=CARTESIAN_POINT('Ctrl Pts',(-5.3899827,3.525679915,4.848771648));
#115592=CARTESIAN_POINT('Ctrl Pts',(-5.125025008,3.591414347,5.143303435));
#115593=CARTESIAN_POINT('Ctrl Pts',(-4.8295518,3.656498153,5.407210872));
#115594=CARTESIAN_POINT('Ctrl Pts',(-5.42796399453673,3.52114709502066,
5.17647145195521));
#115595=CARTESIAN_POINT('Ctrl Pts',(-5.4181729145251,3.52341350501031,5.18666106539168));
#115596=CARTESIAN_POINT('Ctrl Pts',(-5.40838183451358,3.525679915,5.19685067882805));
#115597=CARTESIAN_POINT('Ctrl Pts',(-5.12440361073537,3.591414347,5.49238787403437));
#115598=CARTESIAN_POINT('Ctrl Pts',(-4.80991356956551,3.656498153,5.75522219454662));
#115599=CARTESIAN_POINT('Origin',(0.151420717534398,3.48216457228584,-0.126443930581133));
#115600=CARTESIAN_POINT('Ctrl Pts',(-5.884532912,3.656505752,4.234946565));
#115601=CARTESIAN_POINT('Ctrl Pts',(-5.653967226,3.590992329,4.55532165));
#115602=CARTESIAN_POINT('Ctrl Pts',(-5.3899827,3.525679915,4.848771648));
#115603=CARTESIAN_POINT('Ctrl Pts',(-6.22784936200001,3.656505752,4.178982211));
#115604=CARTESIAN_POINT('Ctrl Pts',(-6.000330577,3.590992329,4.518048676));
#115605=CARTESIAN_POINT('Ctrl Pts',(-5.737345705,3.525679915,4.830410362));
#115606=CARTESIAN_POINT('',(-5.88178333324202,3.65572482709196,4.23876453860927));
#115607=CARTESIAN_POINT('Origin',(0.158797259040004,3.62499998761159,-0.120713940849514));
#115608=CARTESIAN_POINT('Ctrl Pts',(-6.08519336616646,3.6164059874159,4.38411013664156));
#115609=CARTESIAN_POINT('Ctrl Pts',(-6.05128338114145,3.62265476506354,
4.35982954685296));
#115610=CARTESIAN_POINT('Ctrl Pts',(-6.01736176949393,3.62905099625138,
4.33556417130597));
#115611=CARTESIAN_POINT('Ctrl Pts',(-5.94956971260826,3.64214707386253,
4.28712194686511));
#115612=CARTESIAN_POINT('Ctrl Pts',(-5.91566236205225,3.6488540458823,4.26291872248395));
#115613=CARTESIAN_POINT('Ctrl Pts',(-5.88178333430147,3.65572482674346,
4.23876453754314));
#115614=CARTESIAN_POINT('Ctrl Pts',(-6.31978786236768,3.52114709501928,
3.55296041125809));
#115615=CARTESIAN_POINT('Ctrl Pts',(-6.31304916918384,3.52341350500961,
3.56484175912901));
#115616=CARTESIAN_POINT('Ctrl Pts',(-6.306310476,3.525679915,3.576723107));
#115617=CARTESIAN_POINT('Ctrl Pts',(-6.110862975,3.591414347,3.921326977));
#115618=CARTESIAN_POINT('Ctrl Pts',(-5.879030064,3.656498153,4.24258241));
#115619=CARTESIAN_POINT('Ctrl Pts',(-6.41384955991653,3.52114709501927,
3.88859661673224));
#115620=CARTESIAN_POINT('Ctrl Pts',(-6.40647785557602,3.52341350500961,
3.90065279546533));
#115621=CARTESIAN_POINT('Ctrl Pts',(-6.39910615123553,3.525679915,3.91270897419841));
#115622=CARTESIAN_POINT('Ctrl Pts',(-6.18529894082314,3.591414347,4.26238359815085));
#115623=CARTESIAN_POINT('Ctrl Pts',(-5.93466311169445,3.656498153,4.58667905973639));
#115624=CARTESIAN_POINT('Origin',(0.175062231256731,3.48216460447819,-0.0909367358897484));
#115625=CARTESIAN_POINT('Ctrl Pts',(-6.65734413,3.656505752,2.870935237));
#115626=CARTESIAN_POINT('Ctrl Pts',(-6.501040115,3.590992329,3.233384938));
#115627=CARTESIAN_POINT('Ctrl Pts',(-6.306310476,3.525679915,3.576723107));
#115628=CARTESIAN_POINT('Ctrl Pts',(-6.98060335100001,3.656505752,2.74247641));
#115629=CARTESIAN_POINT('Ctrl Pts',(-6.831293095,3.590992329,3.122525503));
#115630=CARTESIAN_POINT('Ctrl Pts',(-6.64160519300001,3.525679915,3.48411832));
#115631=CARTESIAN_POINT('',(-6.65547958607909,3.65572482707743,2.87525502706408));
#115632=CARTESIAN_POINT('Origin',(0.181034478709273,3.62499995426716,-0.0837549443061048));
#115633=CARTESIAN_POINT('Ctrl Pts',(-6.8853790129272,3.61640598740089,2.9734753811648));
#115634=CARTESIAN_POINT('Ctrl Pts',(-6.84704221537427,3.62265476505728,
2.95705210249716));
#115635=CARTESIAN_POINT('Ctrl Pts',(-6.8086973335704,3.629050996263,2.94064618172772));
#115636=CARTESIAN_POINT('Ctrl Pts',(-6.73207659066832,3.6421470704921,2.90790980639303));
#115637=CARTESIAN_POINT('Ctrl Pts',(-6.69375898669547,3.64885404423382,
2.89156151352313));
#115638=CARTESIAN_POINT('Ctrl Pts',(-6.65547958665254,3.6557248267469,2.87525502557864));
#115639=CARTESIAN_POINT('Ctrl Pts',(-6.93581619739237,3.52114709500757,
2.11132659215546));
#115640=CARTESIAN_POINT('Ctrl Pts',(-6.93178918969624,3.52341350500376,
2.12437878057777));
#115641=CARTESIAN_POINT('Ctrl Pts',(-6.927762182,3.525679915,2.137430969));
#115642=CARTESIAN_POINT('Ctrl Pts',(-6.810963781,3.591414347,2.515993627));
#115643=CARTESIAN_POINT('Ctrl Pts',(-6.653611416,3.656498153,2.87957551));
#115644=CARTESIAN_POINT('Ctrl Pts',(-7.09983064816225,3.52114709500757,
2.41889532507528));
#115645=CARTESIAN_POINT('Ctrl Pts',(-7.09522301220064,3.52341350500376,
2.43225433561989));
#115646=CARTESIAN_POINT('Ctrl Pts',(-7.09061537623906,3.525679915,2.44561334616444));
#115647=CARTESIAN_POINT('Ctrl Pts',(-6.95697656715272,3.591414347,2.83307500212556));
#115648=CARTESIAN_POINT('Ctrl Pts',(-6.78191440265768,3.656498153,3.20366791037357));
#115649=CARTESIAN_POINT('Origin',(0.19051800560537,3.48216457483211,-0.051177446463225));
#115650=CARTESIAN_POINT('Ctrl Pts',(-7.118865336,3.656505752,1.372682168));
#115651=CARTESIAN_POINT('Ctrl Pts',(-7.044131593,3.590992329,1.760258739));
#115652=CARTESIAN_POINT('Ctrl Pts',(-6.927762182,3.525679915,2.137430969));
#115653=CARTESIAN_POINT('Ctrl Pts',(-7.40695208500001,3.656505752,1.17773546));
#115654=CARTESIAN_POINT('Ctrl Pts',(-7.34283194100001,3.590992329,1.580996508));
#115655=CARTESIAN_POINT('Ctrl Pts',(-7.235310603,3.525679915,1.974912778));
#115656=CARTESIAN_POINT('',(-7.11797301064352,3.65572482706536,1.37730178611899));
#115657=CARTESIAN_POINT('Origin',(0.194806978521487,3.62499997097553,-0.0428797811535073));
#115658=CARTESIAN_POINT('Ctrl Pts',(-7.36361198972982,3.61640598740004,
1.42380422152945));
#115659=CARTESIAN_POINT('Ctrl Pts',(-7.32264096578964,3.62265476504334,
1.41600618821163));
#115660=CARTESIAN_POINT('Ctrl Pts',(-7.28166577807003,3.62905099623261,
1.40822684487029));
#115661=CARTESIAN_POINT('Ctrl Pts',(-7.1997989301185,3.64214708684124,1.39272700326385));
#115662=CARTESIAN_POINT('Ctrl Pts',(-7.15886282522454,3.64885405225192,
1.38499808700501));
#115663=CARTESIAN_POINT('Ctrl Pts',(-7.11797301143247,3.65572482669986,
1.37730178429856));
#115664=CARTESIAN_POINT('Ctrl Pts',(-7.22753347549519,3.52114709522439,
0.570969490054872));
#115665=CARTESIAN_POINT('Ctrl Pts',(-7.22640645174754,3.52341350511217,
0.584582212527431));
#115666=CARTESIAN_POINT('Ctrl Pts',(-7.225279428,3.525679915,0.598194935));
#115667=CARTESIAN_POINT('Ctrl Pts',(-7.19259149,3.591414347,0.993015212));
#115668=CARTESIAN_POINT('Ctrl Pts',(-7.117077294,3.656498153,1.38192286));
#115669=CARTESIAN_POINT('Ctrl Pts',(-7.4538315460106,3.52114709522438,0.836089178790157));
#115670=CARTESIAN_POINT('Ctrl Pts',(-7.45220342644917,3.52341350511217,
0.850126367903856));
#115671=CARTESIAN_POINT('Ctrl Pts',(-7.45057530688761,3.525679915,0.864163557017569));
#115672=CARTESIAN_POINT('Ctrl Pts',(-7.40335370095443,3.591414347,1.27129496701621));
#115673=CARTESIAN_POINT('Ctrl Pts',(-7.31205091454397,3.656498153,1.67085681056018));
#115674=CARTESIAN_POINT('Origin',(0.197065557393947,3.48216456643412,-0.00902521413211094));
#115675=CARTESIAN_POINT('Ctrl Pts',(-7.24751631,3.656505752,-0.189755993));
#115676=CARTESIAN_POINT('Ctrl Pts',(-7.25784730700001,3.590992329,0.204824799));
#115677=CARTESIAN_POINT('Ctrl Pts',(-7.225279428,3.525679915,0.598194935));
#115678=CARTESIAN_POINT('Ctrl Pts',(-7.486959971,3.656505752,-0.44207509));
#115679=CARTESIAN_POINT('Ctrl Pts',(-7.511028126,3.590992329,-0.034458126));
#115680=CARTESIAN_POINT('Ctrl Pts',(-7.490700931,3.525679915,0.373362509));
#115681=CARTESIAN_POINT('',(-7.24763792833492,3.65572482708963,-0.18505255615449));
#115682=CARTESIAN_POINT('Origin',(0.199470203544115,3.62499995356544,4.69240348278943E-7));
#115683=CARTESIAN_POINT('Ctrl Pts',(-7.49753065349767,3.61640598744145,
-0.192442440658621));
#115684=CARTESIAN_POINT('Ctrl Pts',(-7.45584116260823,3.62265476509222,
-0.191250601216073));
#115685=CARTESIAN_POINT('Ctrl Pts',(-7.41415162318376,3.62905099626916,
-0.190039613672391));
#115686=CARTESIAN_POINT('Ctrl Pts',(-7.33086684937623,3.64214707419444,
-0.187578127585177));
#115687=CARTESIAN_POINT('Ctrl Pts',(-7.28922627644256,3.64885404603143,
-0.186326292333282));
#115688=CARTESIAN_POINT('Ctrl Pts',(-7.24763792841524,3.65572482669476,
-0.185052557297352));
#115689=CARTESIAN_POINT('Ctrl Pts',(-7.18389057158659,3.52436392548355,
-0.976872129593754));
#115690=CARTESIAN_POINT('Ctrl Pts',(-7.1844206052933,3.52502192024177,-0.972942079296878));
#115691=CARTESIAN_POINT('Ctrl Pts',(-7.184950639,3.525679915,-0.969012029));
#115692=CARTESIAN_POINT('Ctrl Pts',(-7.23790161500001,3.591414347,-0.576395491));
#115693=CARTESIAN_POINT('Ctrl Pts',(-7.24775654700001,3.656498153,-0.180346967));
#115694=CARTESIAN_POINT('Ctrl Pts',(-7.46075501751712,3.52436392548355,
-0.766290988866588));
#115695=CARTESIAN_POINT('Ctrl Pts',(-7.46116970125857,3.52502192024177,
-0.762209624433295));
#115696=CARTESIAN_POINT('Ctrl Pts',(-7.461584385,3.525679915,-0.75812826));
#115697=CARTESIAN_POINT('Ctrl Pts',(-7.503011767,3.591414347,-0.350395266));
#115698=CARTESIAN_POINT('Ctrl Pts',(-7.499764582,3.656498153,0.0594240580000001));
#115699=CARTESIAN_POINT('Origin',(0.194398464463127,3.4821645223859,0.0335490630156204));
#115700=CARTESIAN_POINT('Ctrl Pts',(-7.037281477,3.656505752,-1.743321375));
#115701=CARTESIAN_POINT('Ctrl Pts',(-7.132194147,3.590992329,-1.360186522));
#115702=CARTESIAN_POINT('Ctrl Pts',(-7.184950639,3.525679915,-0.969012029));
#115703=CARTESIAN_POINT('Ctrl Pts',(-7.216885931,3.656505752,-2.041214701));
#115704=CARTESIAN_POINT('Ctrl Pts',(-7.328016983,3.590992329,-1.648301537));
#115705=CARTESIAN_POINT('Ctrl Pts',(-7.395834409,3.525679915,-1.245645776));
#115706=CARTESIAN_POINT('',(-7.03841135162036,3.65572482709059,-1.73875404613841));
#115707=CARTESIAN_POINT('Origin',(0.194806796920498,3.62499999752868,0.0428807018726299));
#115708=CARTESIAN_POINT('Ctrl Pts',(-7.28087311686949,3.61640598742508,
-1.79969070845467));
#115709=CARTESIAN_POINT('Ctrl Pts',(-7.24041451346179,3.62265476507037,
-1.78956472535037));
#115710=CARTESIAN_POINT('Ctrl Pts',(-7.19995997890244,3.6290509962478,-1.77942003139437));
#115711=CARTESIAN_POINT('Ctrl Pts',(-7.11915142346629,3.64214708718919,
-1.75911230892189));
#115712=CARTESIAN_POINT('Ctrl Pts',(-7.07875353435021,3.64885405242303,
-1.74893825936027));
#115713=CARTESIAN_POINT('Ctrl Pts',(-7.0384113518051,3.65572482670577,-1.73875404767568));
#115714=CARTESIAN_POINT('Ctrl Pts',(-6.80593657008117,3.52436392548355,
-2.49835752065326));
#115715=CARTESIAN_POINT('Ctrl Pts',(-6.80729905654059,3.52502192024177,
-2.49463329432663));
#115716=CARTESIAN_POINT('Ctrl Pts',(-6.808661543,3.525679915,-2.490909068));
#115717=CARTESIAN_POINT('Ctrl Pts',(-6.944775505,3.591414347,-2.118854581));
#115718=CARTESIAN_POINT('Ctrl Pts',(-7.03953876,3.656498153,-1.734183971));
#115719=CARTESIAN_POINT('Ctrl Pts',(-7.121596800251,3.52436392548355,-2.35221732129617));
#115720=CARTESIAN_POINT('Ctrl Pts',(-7.12287916162549,3.52502192024177,
-2.34832052164809));
#115721=CARTESIAN_POINT('Ctrl Pts',(-7.124161523,3.525679915,-2.344423722));
#115722=CARTESIAN_POINT('Ctrl Pts',(-7.25227089700001,3.591414347,-1.955128962));
#115723=CARTESIAN_POINT('Ctrl Pts',(-7.33719866900001,3.656498153,-1.554192937));
#115724=CARTESIAN_POINT('Origin',(0.182641489301882,3.48216454051536,0.0745546352115367));
#115725=CARTESIAN_POINT('Ctrl Pts',(-6.497991183,3.656505752,-3.215370987));
#115726=CARTESIAN_POINT('Ctrl Pts',(-6.673047516,3.590992329,-2.861597032));
#115727=CARTESIAN_POINT('Ctrl Pts',(-6.808661543,3.525679915,-2.490909068));
#115728=CARTESIAN_POINT('Ctrl Pts',(-6.609358326,3.656505752,-3.544909382));
#115729=CARTESIAN_POINT('Ctrl Pts',(-6.80235591100001,3.590992329,-3.1850722));
#115730=CARTESIAN_POINT('Ctrl Pts',(-6.955146889,3.525679915,-2.806409048));
#115731=CARTESIAN_POINT('',(-6.50007648309978,3.65572482710153,-3.21115332982368));
#115732=CARTESIAN_POINT('Origin',(0.181034151573773,3.6249999647383,0.0837558341557831));
#115733=CARTESIAN_POINT('Ctrl Pts',(-6.7237700457547,3.61640598738409,-3.32278743899844));
#115734=CARTESIAN_POINT('Ctrl Pts',(-6.6864341290363,3.62265476504407,-3.30420079200989));
#115735=CARTESIAN_POINT('Ctrl Pts',(-6.64910620829098,3.62905099623725,
-3.28559674629475));
#115736=CARTESIAN_POINT('Ctrl Pts',(-6.57455251052107,3.64214708041289,
-3.24839237571768));
#115737=CARTESIAN_POINT('Ctrl Pts',(-6.53728620099037,3.64885404908062,
-3.22977182764316));
#115738=CARTESIAN_POINT('Ctrl Pts',(-6.50007648257382,3.6557248266913,-3.21115333145444));
#115739=CARTESIAN_POINT('Ctrl Pts',(-6.10974453928919,3.52436392548355,
-3.90302249135112));
#115740=CARTESIAN_POINT('Ctrl Pts',(-6.11187577014459,3.52502192024177,
-3.89967822967556));
#115741=CARTESIAN_POINT('Ctrl Pts',(-6.114007001,3.525679915,-3.896333968));
#115742=CARTESIAN_POINT('Ctrl Pts',(-6.326919411,3.591414347,-3.562238386));
#115743=CARTESIAN_POINT('Ctrl Pts',(-6.502159964,3.656498153,-3.20693246));
#115744=CARTESIAN_POINT('Ctrl Pts',(-6.44944063157123,3.52436392548355,
-3.8281565867108));
#115745=CARTESIAN_POINT('Ctrl Pts',(-6.45153070878562,3.52502192024177,
-3.8246265618554));
#115746=CARTESIAN_POINT('Ctrl Pts',(-6.453620786,3.525679915,-3.821096537));
#115747=CARTESIAN_POINT('Ctrl Pts',(-6.6624219,3.591414347,-3.468443));
#115748=CARTESIAN_POINT('Ctrl Pts',(-6.831553502,3.656498153,-3.095137598));
#115749=CARTESIAN_POINT('Origin',(0.162344440831546,3.48216455730966,0.112074132583539));
#115750=CARTESIAN_POINT('Ctrl Pts',(-5.65486204400001,3.656505752,-4.537073425));
#115751=CARTESIAN_POINT('Ctrl Pts',(-5.9018766,3.590992329,-4.229202446));
#115752=CARTESIAN_POINT('Ctrl Pts',(-6.114007001,3.525679915,-3.896333968));
#115753=CARTESIAN_POINT('Ctrl Pts',(-5.692784471,3.656505752,-4.882848039));
#115754=CARTESIAN_POINT('Ctrl Pts',(-5.958624237,3.590992329,-4.572912427));
#115755=CARTESIAN_POINT('Ctrl Pts',(-6.189244432,3.525679915,-4.235947753));
#115756=CARTESIAN_POINT('',(-5.65780526222359,3.65572482709928,-4.53340265263039));
#115757=CARTESIAN_POINT('Origin',(0.158796591899044,3.6249999668739,0.120714626165824));
#115758=CARTESIAN_POINT('Ctrl Pts',(-5.85227096027948,3.6164059873619,-4.69051432171717));
#115759=CARTESIAN_POINT('Ctrl Pts',(-5.81980351626557,3.62265476501948,
-4.66433610172348));
#115760=CARTESIAN_POINT('Ctrl Pts',(-5.78734762151533,3.62905099620998,
-4.63814260870191));
#115761=CARTESIAN_POINT('Ctrl Pts',(-5.72253480594774,3.64214707671741,
-4.58578122911816));
#115762=CARTESIAN_POINT('Ctrl Pts',(-5.69014261976763,3.6488540472637,-4.5595848563537));
#115763=CARTESIAN_POINT('Ctrl Pts',(-5.65780526166865,3.65572482670257,
-4.53340265385012));
#115764=CARTESIAN_POINT('Ctrl Pts',(-5.12786764447628,3.52436392548355,
-5.1251864671127));
#115765=CARTESIAN_POINT('Ctrl Pts',(-5.13066796573815,3.52502192024177,
-5.12237854405635));
#115766=CARTESIAN_POINT('Ctrl Pts',(-5.133468287,3.525679915,-5.119570621));
#115767=CARTESIAN_POINT('Ctrl Pts',(-5.413223597,3.591414347,-4.839055883));
#115768=CARTESIAN_POINT('Ctrl Pts',(-5.660747395,3.656498153,-4.529728351));
#115769=CARTESIAN_POINT('Ctrl Pts',(-5.47571578726615,3.52436392548355,
-5.12509550503651));
#115770=CARTESIAN_POINT('Ctrl Pts',(-5.47851585063307,3.52502192024177,
-5.12209731501825));
#115771=CARTESIAN_POINT('Ctrl Pts',(-5.481315914,3.525679915,-5.119099125));
#115772=CARTESIAN_POINT('Ctrl Pts',(-5.76104546,3.591414347,-4.819576499));
#115773=CARTESIAN_POINT('Ctrl Pts',(-6.006472486,3.656498153,-4.491357064));
#115774=CARTESIAN_POINT('Origin',(0.134456337787808,3.48216453075468,0.144353208218625));
#115775=CARTESIAN_POINT('Ctrl Pts',(-4.54731784,3.656505752,-5.646627353));
#115776=CARTESIAN_POINT('Ctrl Pts',(-4.854740493,3.590992329,-5.399055054));
#115777=CARTESIAN_POINT('Ctrl Pts',(-5.133468287,3.525679915,-5.119570621));
#115778=CARTESIAN_POINT('Ctrl Pts',(-4.510022341,3.656505752,-5.992470149));
#115779=CARTESIAN_POINT('Ctrl Pts',(-4.836273917,3.590992329,-5.746928351));
#115780=CARTESIAN_POINT('Ctrl Pts',(-5.133939783,3.525679915,-5.467418248));
#115781=CARTESIAN_POINT('',(-4.55098135572124,3.65572482706278,-5.64367510519807));
#115782=CARTESIAN_POINT('Origin',(0.129133949453862,3.62499998608658,0.152028971897459));
#115783=CARTESIAN_POINT('Ctrl Pts',(-4.70712618881638,3.6164059874195,-5.83891796798881));
#115784=CARTESIAN_POINT('Ctrl Pts',(-4.681045359071,3.62265476505457,-5.8063722394639));
#115785=CARTESIAN_POINT('Ctrl Pts',(-4.65497909171544,3.62905099624552,
-5.77381407758711));
#115786=CARTESIAN_POINT('Ctrl Pts',(-4.60293773645466,3.64214707069617,
-5.70874406817838));
#115787=CARTESIAN_POINT('Ctrl Pts',(-4.5769342946032,3.64885404428948,-5.67619677349355));
#115788=CARTESIAN_POINT('Ctrl Pts',(-4.5509813544537,3.65572482666267,-5.64367510615619));
#115789=CARTESIAN_POINT('Ctrl Pts',(-3.8898961054492,3.52114709484942,-6.11816595059717));
#115790=CARTESIAN_POINT('Ctrl Pts',(-3.90139520322457,3.52341350492468,
-6.11079389679852));
#115791=CARTESIAN_POINT('Ctrl Pts',(-3.912894301,3.525679915,-6.103421843));
#115792=CARTESIAN_POINT('Ctrl Pts',(-4.246411465,3.591414347,-5.889604505));
#115793=CARTESIAN_POINT('Ctrl Pts',(-4.55464456900001,3.656498153,-5.640719178));
#115794=CARTESIAN_POINT('Ctrl Pts',(-4.23013246864957,3.52114709484942,
-6.1939187206583));
#115795=CARTESIAN_POINT('Ctrl Pts',(-4.24177187036649,3.52341350492468,
-6.18590511891521));
#115796=CARTESIAN_POINT('Ctrl Pts',(-4.25341127208348,3.525679915,-6.17789151717195));
#115797=CARTESIAN_POINT('Ctrl Pts',(-4.59099777905268,3.591414347,-5.9454668714277));
#115798=CARTESIAN_POINT('Ctrl Pts',(-4.90124848342061,3.656498153,-5.67764161846073));
#115799=CARTESIAN_POINT('Origin',(0.100281084784133,3.48216457830553,0.169882325752175));
#115800=CARTESIAN_POINT('Ctrl Pts',(-3.227146108,3.656505752,-6.492151261));
#115801=CARTESIAN_POINT('Ctrl Pts',(-3.580602117,3.590992329,-6.316453848));
#115802=CARTESIAN_POINT('Ctrl Pts',(-3.912894301,3.525679915,-6.103421843));
#115803=CARTESIAN_POINT('Ctrl Pts',(-3.116376579,3.656505752,-6.821891015));
#115804=CARTESIAN_POINT('Ctrl Pts',(-3.487784803,3.590992329,-6.652224292));
#115805=CARTESIAN_POINT('Ctrl Pts',(-3.838577816,3.525679915,-6.443238343));
#115806=CARTESIAN_POINT('',(-3.23135861876458,3.65572482706242,-6.49005558269118));
#115807=CARTESIAN_POINT('Origin',(0.0934331116377524,3.62499994453812,0.176234561179893));
#115808=CARTESIAN_POINT('Ctrl Pts',(-3.34188142830791,3.61640598742262,
-6.7143002994709));
#115809=CARTESIAN_POINT('Ctrl Pts',(-3.32340672345575,3.62265476506398,
-6.67690886461093));
#115810=CARTESIAN_POINT('Ctrl Pts',(-3.30494891336774,3.62905099624106,
-6.63950841770322));
#115811=CARTESIAN_POINT('Ctrl Pts',(-3.26811231382241,3.64214709583241,
-6.56477221270267));
#115812=CARTESIAN_POINT('Ctrl Pts',(-3.24971356186776,3.64885405664215,
-6.52739596079861));
#115813=CARTESIAN_POINT('Ctrl Pts',(-3.23135861705088,3.65572482665306,
-6.49005558433552));
#115814=CARTESIAN_POINT('Ctrl Pts',(-2.48372766966525,3.52114709510818,
-6.81133930780071));
#115815=CARTESIAN_POINT('Ctrl Pts',(-2.49654269783263,3.52341350505406,
-6.80661157490037));
#115816=CARTESIAN_POINT('Ctrl Pts',(-2.509357726,3.525679915,-6.801883842));
#115817=CARTESIAN_POINT('Ctrl Pts',(-2.881041851,3.591414347,-6.66476176600001));
#115818=CARTESIAN_POINT('Ctrl Pts',(-3.235571625,3.656498153,-6.487956247));
#115819=CARTESIAN_POINT('Ctrl Pts',(-2.79972488961055,3.52114709510818,
-6.95846178142387));
#115820=CARTESIAN_POINT('Ctrl Pts',(-2.81281485533693,3.52341350505406,
-6.95313766082784));
#115821=CARTESIAN_POINT('Ctrl Pts',(-2.82590482106331,3.525679915,-6.94781354023191));
#115822=CARTESIAN_POINT('Ctrl Pts',(-3.20556317169257,3.591414347,-6.79339397288846));
#115823=CARTESIAN_POINT('Ctrl Pts',(-3.56613489948184,3.656498153,-6.5985250570152));
#115824=CARTESIAN_POINT('Origin',(0.0614169840414003,3.48216457005707,0.187468286320412));
#115825=CARTESIAN_POINT('Ctrl Pts',(-1.756076611,3.656505752,-7.034109392));
#115826=CARTESIAN_POINT('Ctrl Pts',(-2.139038765,3.590992329,-6.93850228));
#115827=CARTESIAN_POINT('Ctrl Pts',(-2.509357726,3.525679915,-6.801883842));
#115828=CARTESIAN_POINT('Ctrl Pts',(-1.577012512,3.656505752,-7.332327839));
#115829=CARTESIAN_POINT('Ctrl Pts',(-1.976210748,3.590992329,-7.246469619));
#115830=CARTESIAN_POINT('Ctrl Pts',(-2.363728217,3.525679915,-7.117779774));
#115831=CARTESIAN_POINT('',(-1.76064114414197,3.65572482706168,-7.03296827468653));
#115832=CARTESIAN_POINT('Origin',(0.053363518657509,3.62499993664306,0.192199759904212));
#115833=CARTESIAN_POINT('Ctrl Pts',(-1.82037400642531,3.61640598742844,
-7.27572941159549));
#115834=CARTESIAN_POINT('Ctrl Pts',(-1.81036928315251,3.62265476507407,
-7.23524065217722));
#115835=CARTESIAN_POINT('Ctrl Pts',(-1.80038299703673,3.62905099622303,
-7.19474672351256));
#115836=CARTESIAN_POINT('Ctrl Pts',(-1.78047370801797,3.64214708508883,
-7.11383909568418));
#115837=CARTESIAN_POINT('Ctrl Pts',(-1.77053988931242,3.64885405136343,
-7.07338145667437));
#115838=CARTESIAN_POINT('Ctrl Pts',(-1.7606411424949,3.65572482666902,-7.03296827582325));
#115839=CARTESIAN_POINT('Ctrl Pts',(-0.96142288802051,3.5211470951993,-7.18602201069066));
#115840=CARTESIAN_POINT('Ctrl Pts',(-0.974954630510261,3.52341350509963,
-7.18415966184533));
#115841=CARTESIAN_POINT('Ctrl Pts',(-0.988486373,3.525679915,-7.182297313));
#115842=CARTESIAN_POINT('Ctrl Pts',(-1.380957923,3.591414347,-7.128282175));
#115843=CARTESIAN_POINT('Ctrl Pts',(-1.765206948,3.656498153,-7.031823692));
#115844=CARTESIAN_POINT('Ctrl Pts',(-1.23840528569355,3.5211470951993,-7.39763490453268));
#115845=CARTESIAN_POINT('Ctrl Pts',(-1.25233374354749,3.52341350509963,
-7.39524921465165));
#115846=CARTESIAN_POINT('Ctrl Pts',(-1.26626220140147,3.525679915,-7.3928635247706));
#115847=CARTESIAN_POINT('Ctrl Pts',(-1.6702399926727,3.591414347,-7.32366952361838));
#115848=CARTESIAN_POINT('Ctrl Pts',(-2.06427281173036,3.656498153,-7.21086879729882));
#115849=CARTESIAN_POINT('Origin',(0.019680936437359,3.48216458086525,0.196288130968899));
#115850=CARTESIAN_POINT('Ctrl Pts',(-0.202894923,3.656505752,-7.247160385));
#115851=CARTESIAN_POINT('Ctrl Pts',(-0.597456338000001,3.590992329,-7.23611405800001));
#115852=CARTESIAN_POINT('Ctrl Pts',(-0.988486373,3.525679915,-7.182297313));
#115853=CARTESIAN_POINT('Ctrl Pts',(0.036090908,3.656505752,-7.499913163));
#115854=CARTESIAN_POINT('Ctrl Pts',(-0.372231275,3.590992329,-7.501878081));
#115855=CARTESIAN_POINT('Ctrl Pts',(-0.778353314,3.525679915,-7.459501734));
#115856=CARTESIAN_POINT('',(-0.207598047069502,3.65572482706502,-7.24702718637008));
#115857=CARTESIAN_POINT('Origin',(0.010798619422784,3.62499991866262,0.199177593573561));
#115858=CARTESIAN_POINT('Ctrl Pts',(-0.213747918968888,3.6164059912397,
-7.49695347696992));
#115859=CARTESIAN_POINT('Ctrl Pts',(-0.212680986910659,3.62265476894078,
-7.45526060255481));
#115860=CARTESIAN_POINT('Ctrl Pts',(-0.211633172836877,3.62905099623971,
-7.41356666842584));
#115861=CARTESIAN_POINT('Ctrl Pts',(-0.209582099320455,3.64214709043449,
-7.33027067337734));
#115862=CARTESIAN_POINT('Ctrl Pts',(-0.208577724648146,3.64885405398644,
-7.28862345213346));
#115863=CARTESIAN_POINT('Ctrl Pts',(-0.207598044645775,3.65572482664597,
-7.24702718686974));
#115864=CARTESIAN_POINT('Ctrl Pts',(0.586511467990447,3.52436392548355,
-7.22624156853374));
#115865=CARTESIAN_POINT('Ctrl Pts',(0.582558485995224,3.52502192024177,
-7.22655805626688));
#115866=CARTESIAN_POINT('Ctrl Pts',(0.578605504000001,3.525679915,-7.226874544));
#115867=CARTESIAN_POINT('Ctrl Pts',(0.183698063,3.591414347,-7.258492032));
#115868=CARTESIAN_POINT('Ctrl Pts',(-0.212303156,3.656498153,-7.246890876));
#115869=CARTESIAN_POINT('Ctrl Pts',(0.361250022558109,3.52436392548355,
-7.49129933610564));
#115870=CARTESIAN_POINT('Ctrl Pts',(0.357152193279055,3.52502192024177,
-7.49149245105282));
#115871=CARTESIAN_POINT('Ctrl Pts',(0.353054364,3.525679915,-7.491685566));
#115872=CARTESIAN_POINT('Ctrl Pts',(-0.056323487,3.591414347,-7.510977971));
#115873=CARTESIAN_POINT('Ctrl Pts',(-0.465365977,3.656498153,-7.485548377));
#115874=CARTESIAN_POINT('Origin',(-0.0229753300832009,3.48216457544246,
0.195929666396335));
#115875=CARTESIAN_POINT('Ctrl Pts',(1.359773906,3.656505752,-7.121342214));
#115876=CARTESIAN_POINT('Ctrl Pts',(0.972062484,3.590992329,-7.19537318400001));
#115877=CARTESIAN_POINT('Ctrl Pts',(0.578605504,3.525679915,-7.226874544));
#115878=CARTESIAN_POINT('Ctrl Pts',(1.647506757,3.656505752,-7.316810882));
#115879=CARTESIAN_POINT('Ctrl Pts',(1.249153319,3.590992329,-7.406507061));
#115880=CARTESIAN_POINT('Ctrl Pts',(0.843416526,3.525679915,-7.452425683));
#115881=CARTESIAN_POINT('',(1.35515210503228,3.65572482705034,-7.12222316170083));
#115882=CARTESIAN_POINT('Origin',(-0.032271179737238,3.62499994809109,0.196842596556915));
#115883=CARTESIAN_POINT('Ctrl Pts',(1.40287278318669,3.61640598739448,-7.36762837997685));
#115884=CARTESIAN_POINT('Ctrl Pts',(1.39495203533521,3.62265476504023,-7.32668090293707));
#115885=CARTESIAN_POINT('Ctrl Pts',(1.38701238381459,3.62905099619008,-7.28573647595259));
#115886=CARTESIAN_POINT('Ctrl Pts',(1.37110933111604,3.6421470873043,-7.2039469941694));
#115887=CARTESIAN_POINT('Ctrl Pts',(1.36313730042969,3.64885405241763,-7.1630575408346));
#115888=CARTESIAN_POINT('Ctrl Pts',(1.35515210661499,3.65572482658934,-7.12222316207102));
#115889=CARTESIAN_POINT('Ctrl Pts',(2.12622748692775,3.52436392548355,-6.93121342759178));
#115890=CARTESIAN_POINT('Ctrl Pts',(2.12243495896388,3.52502192024177,-6.93237229029589));
#115891=CARTESIAN_POINT('Ctrl Pts',(2.118642431,3.525679915,-6.933531153));
#115892=CARTESIAN_POINT('Ctrl Pts',(1.739764532,3.591414347,-7.049302868));
#115893=CARTESIAN_POINT('Ctrl Pts',(1.350527695,3.656498153,-7.123101498));
#115894=CARTESIAN_POINT('Ctrl Pts',(1.96321211359414,3.52436392548355,-7.23849884360055));
#115895=CARTESIAN_POINT('Ctrl Pts',(1.95925160329707,3.52502192024177,-7.23956835580028));
#115896=CARTESIAN_POINT('Ctrl Pts',(1.955291093,3.525679915,-7.240637868));
#115897=CARTESIAN_POINT('Ctrl Pts',(1.559631566,3.591414347,-7.347483365));
#115898=CARTESIAN_POINT('Ctrl Pts',(1.154685651,3.656498153,-7.410580345));
#115899=CARTESIAN_POINT('Origin',(-0.0645573202639896,3.48216453713675,
0.186410085550968));
#115900=CARTESIAN_POINT('Ctrl Pts',(2.858861218,3.656505752,-6.662537995));
#115901=CARTESIAN_POINT('Ctrl Pts',(2.496128744,3.590992329,-6.818184657));
#115902=CARTESIAN_POINT('Ctrl Pts',(2.118642431,3.525679915,-6.933531153));
#115903=CARTESIAN_POINT('Ctrl Pts',(3.18188702,3.656505752,-6.791582657));
#115904=CARTESIAN_POINT('Ctrl Pts',(2.812128892,3.590992329,-6.96481600299999));
#115905=CARTESIAN_POINT('Ctrl Pts',(2.425749146,3.525679915,-7.09688249));
#115906=CARTESIAN_POINT('',(2.85453685021956,3.65572482706825,-6.66439189739295));
#115907=CARTESIAN_POINT('Origin',(-0.0738320489144723,3.62499994952612,
0.185303204393322));
#115908=CARTESIAN_POINT('Ctrl Pts',(2.95389671312415,3.61640598741098,-6.89380114309683));
#115909=CARTESIAN_POINT('Ctrl Pts',(2.93735865075867,3.62265476505422,-6.85551372191689));
#115910=CARTESIAN_POINT('Ctrl Pts',(2.92080278241446,3.62905099619161,-6.81723334327981));
#115911=CARTESIAN_POINT('Ctrl Pts',(2.88768921050766,3.64214708846666,-6.74077473349498));
#115912=CARTESIAN_POINT('Ctrl Pts',(2.87111353932749,3.64885405299546,-6.70255500733749));
#115913=CARTESIAN_POINT('Ctrl Pts',(2.85453685203003,3.65572482661415,-6.66439189733454));
#115914=CARTESIAN_POINT('Ctrl Pts',(3.56652347108936,3.52436392548355,-6.31208945091949));
#115915=CARTESIAN_POINT('Ctrl Pts',(3.56306873154468,3.52502192024177,-6.31403650145974));
#115916=CARTESIAN_POINT('Ctrl Pts',(3.559613992,3.525679915,-6.315983552));
#115917=CARTESIAN_POINT('Ctrl Pts',(3.214481544,3.591414347,-6.510496137));
#115918=CARTESIAN_POINT('Ctrl Pts',(2.850209373,3.656498153,-6.66624381));
#115919=CARTESIAN_POINT('Ctrl Pts',(3.47337658852555,3.52436392548355,-6.64723419152526));
#115920=CARTESIAN_POINT('Ctrl Pts',(3.46973858626278,3.52502192024177,-6.64913009176263));
#115921=CARTESIAN_POINT('Ctrl Pts',(3.466100584,3.525679915,-6.651025992));
#115922=CARTESIAN_POINT('Ctrl Pts',(3.10265998,3.591414347,-6.840428603));
#115923=CARTESIAN_POINT('Ctrl Pts',(2.720745461,3.656498153,-6.989101812));
#115924=CARTESIAN_POINT('Origin',(-0.103120705606788,3.48216456522747,0.168174104007248));
#115925=CARTESIAN_POINT('Ctrl Pts',(4.224271357,3.656505752,-5.892200905));
#115926=CARTESIAN_POINT('Ctrl Pts',(3.903478799,3.590992329,-6.122185394));
#115927=CARTESIAN_POINT('Ctrl Pts',(3.559613992,3.525679915,-6.315983552));
#115928=CARTESIAN_POINT('Ctrl Pts',(4.567485784,3.656505752,-5.948787575));
#115929=CARTESIAN_POINT('Ctrl Pts',(4.243612444,3.590992329,-6.19745789));
#115930=CARTESIAN_POINT('Ctrl Pts',(3.894656432,3.525679915,-6.40949695999999));
#115931=CARTESIAN_POINT('',(4.22044662440661,3.65572482707631,-5.89494107545148));
#115932=CARTESIAN_POINT('Origin',(-0.111940529212393,3.62500000250486,0.165099073719102));
#115933=CARTESIAN_POINT('Ctrl Pts',(4.36679971634736,3.61640598740763,-6.09762742671591));
#115934=CARTESIAN_POINT('Ctrl Pts',(4.34241764086447,3.62265476506328,-6.06379033863146));
#115935=CARTESIAN_POINT('Ctrl Pts',(4.31801968949399,3.62905099623956,-6.02996395608197));
#115936=CARTESIAN_POINT('Ctrl Pts',(4.26924399912361,3.64214707620876,-5.9624114087969));
#115937=CARTESIAN_POINT('Ctrl Pts',(4.24483972189627,3.64885404703329,-5.92864848400591));
#115938=CARTESIAN_POINT('Ctrl Pts',(4.22044662594176,3.65572482672606,-5.89494107440452));
#115939=CARTESIAN_POINT('Ctrl Pts',(4.84005278268171,3.52436392548355,-5.39781918605993));
#115940=CARTESIAN_POINT('Ctrl Pts',(4.83709737134085,3.52502192024177,-5.40046338252997));
#115941=CARTESIAN_POINT('Ctrl Pts',(4.83414196,3.525679915,-5.403107579));
#115942=CARTESIAN_POINT('Ctrl Pts',(4.538892973,3.591414347,-5.667265843));
#115943=CARTESIAN_POINT('Ctrl Pts',(4.216618428,3.656498153,-5.89767997));
#115944=CARTESIAN_POINT('Ctrl Pts',(4.82112983456621,3.52436392548355,-5.74515225479416));
#115945=CARTESIAN_POINT('Ctrl Pts',(4.8179844492831,3.52502192024177,-5.74778589289708));
#115946=CARTESIAN_POINT('Ctrl Pts',(4.814839064,3.525679915,-5.750419531));
#115947=CARTESIAN_POINT('Ctrl Pts',(4.500611462,3.591414347,-6.013523002));
#115948=CARTESIAN_POINT('Ctrl Pts',(4.159586238,3.656498153,-6.240820646));
#115949=CARTESIAN_POINT('Origin',(-0.136862052139013,3.48216458582086,0.142074134038869));
#115950=CARTESIAN_POINT('Ctrl Pts',(5.392159262,3.656505752,-4.846351049));
#115951=CARTESIAN_POINT('Ctrl Pts',(5.128306523,3.590992329,-5.13991954600001));
#115952=CARTESIAN_POINT('Ctrl Pts',(4.83414196,3.525679915,-5.403107579));
#115953=CARTESIAN_POINT('Ctrl Pts',(5.739513988,3.656505752,-4.82783379800001));
#115954=CARTESIAN_POINT('Ctrl Pts',(5.476669394,3.590992329,-5.140313533));
#115955=CARTESIAN_POINT('Ctrl Pts',(5.181453912,3.525679915,-5.422410475));
#115956=CARTESIAN_POINT('',(5.38901300557768,3.65572482710028,-4.84984935993923));
#115957=CARTESIAN_POINT('Origin',(-0.144814768043657,3.62499998182717,0.137175170862209));
#115958=CARTESIAN_POINT('Ctrl Pts',(5.57551601750765,3.61640598737869,-5.01633542878598));
#115959=CARTESIAN_POINT('Ctrl Pts',(5.54443000772658,3.62265476503998,-4.98853085853212));
#115960=CARTESIAN_POINT('Ctrl Pts',(5.51333079461945,3.62905099622165,-4.96074015636159));
#115961=CARTESIAN_POINT('Ctrl Pts',(5.4511736065851,3.64214708579882,-4.90525224101104));
#115962=CARTESIAN_POINT('Ctrl Pts',(5.42008188133836,3.64885405174569,-4.87752489447732));
#115963=CARTESIAN_POINT('Ctrl Pts',(5.38901300719692,3.65572482672889,-4.8498493588364));
#115964=CARTESIAN_POINT('Ctrl Pts',(5.89859840263569,3.52114709502404,-4.21542206610258));
#115965=CARTESIAN_POINT('Ctrl Pts',(5.8906146123179,3.52341350501199,-4.22650518405128));
#115966=CARTESIAN_POINT('Ctrl Pts',(5.882630822,3.525679915,-4.237588302));
#115967=CARTESIAN_POINT('Ctrl Pts',(5.651070811,3.591414347,-4.559040496));
#115968=CARTESIAN_POINT('Ctrl Pts',(5.385863092,3.656498153,-4.85334717));
#115969=CARTESIAN_POINT('Ctrl Pts',(5.95582004930385,3.52114709502404,-4.55926061542002));
#115970=CARTESIAN_POINT('Ctrl Pts',(5.94718805603239,3.52341350501199,-4.5704490988617));
#115971=CARTESIAN_POINT('Ctrl Pts',(5.93855606276091,3.525679915,-4.58163758230349));
#115972=CARTESIAN_POINT('Ctrl Pts',(5.68819572295812,3.591414347,-4.90614577273627));
#115973=CARTESIAN_POINT('Ctrl Pts',(5.40396662443608,3.656498153,-5.20144170171409));
#115974=CARTESIAN_POINT('Origin',(-0.164204111051689,3.48216453571289,0.109331279387648));
#115975=CARTESIAN_POINT('Ctrl Pts',(6.307915794,3.656505752,-3.573891204));
#115976=CARTESIAN_POINT('Ctrl Pts',(6.113340333,3.590992329,-3.917316773));
#115977=CARTESIAN_POINT('Ctrl Pts',(5.882630822,3.525679915,-4.237588302));
#115978=CARTESIAN_POINT('Ctrl Pts',(6.64316889699999,3.656505752,-3.481135878));
#115979=CARTESIAN_POINT('Ctrl Pts',(6.45364337,3.590992329,-3.842813829));
#115980=CARTESIAN_POINT('Ctrl Pts',(6.225972366,3.525679915,-4.181778103));
#115981=CARTESIAN_POINT('',(6.30559512823114,3.65572482705793,-3.57798407890505));
#115982=CARTESIAN_POINT('Origin',(-0.170917924835829,3.62499994017976,0.102837358193317));
#115983=CARTESIAN_POINT('Ctrl Pts',(6.52352738649046,3.6164059873846,-3.70048516154021));
#115984=CARTESIAN_POINT('Ctrl Pts',(6.48719098968864,3.62265476503472,-3.68001321990407));
#115985=CARTESIAN_POINT('Ctrl Pts',(6.45084467935911,3.629050996223,-3.65955766037544));
#115986=CARTESIAN_POINT('Ctrl Pts',(6.37821247405543,3.64214707787778,-3.61872900434467));
#115987=CARTESIAN_POINT('Ctrl Pts',(6.34188707287837,3.64885404782154,-3.59833369652542));
#115988=CARTESIAN_POINT('Ctrl Pts',(6.30559512916798,3.65572482665186,-3.57798407767736));
#115989=CARTESIAN_POINT('Ctrl Pts',(6.66688358641299,3.5211470952643,-2.84884354685972));
#115990=CARTESIAN_POINT('Ctrl Pts',(6.66146899570655,3.52341350513212,-2.86138382592987));
#115991=CARTESIAN_POINT('Ctrl Pts',(6.656054405,3.525679915,-2.873924105));
#115992=CARTESIAN_POINT('Ctrl Pts',(6.499010858,3.591414347,-3.237639483));
#115993=CARTESIAN_POINT('Ctrl Pts',(6.303270783,3.656498153,-3.582077251));
#115994=CARTESIAN_POINT('Ctrl Pts',(6.79668254788956,3.52114709526431,-3.17234237973408));
#115995=CARTESIAN_POINT('Ctrl Pts',(6.79065755929905,3.52341350513212,-3.18512490534756));
#115996=CARTESIAN_POINT('Ctrl Pts',(6.78463257070837,3.525679915,-3.19790743096098));
#115997=CARTESIAN_POINT('Ctrl Pts',(6.60988518347408,3.591414347,-3.56864887214242));
#115998=CARTESIAN_POINT('Ctrl Pts',(6.39578110022067,3.656498153,-3.91814180101807));
#115999=CARTESIAN_POINT('Origin',(-0.183868084565093,3.4821645266703,0.0714761343232284));
#116000=CARTESIAN_POINT('Ctrl Pts',(6.928721193,3.656505752,-2.134320179));
#116001=CARTESIAN_POINT('Ctrl Pts',(6.812521145,3.590992329,-2.511544621));
#116002=CARTESIAN_POINT('Ctrl Pts',(6.656054405,3.525679915,-2.873924105));
#116003=CARTESIAN_POINT('Ctrl Pts',(7.236196612,3.656505752,-1.971663914));
#116004=CARTESIAN_POINT('Ctrl Pts',(7.128852155,3.590992329,-2.365628421));
#116005=CARTESIAN_POINT('Ctrl Pts',(6.979371271,3.525679915,-2.745610435));
#116006=CARTESIAN_POINT('',(6.92733463065445,3.65572482707099,-2.13881623882443));
#116007=CARTESIAN_POINT('Origin',(-0.189028709533438,3.62499997568123,0.0636906784467089));
#116008=CARTESIAN_POINT('Ctrl Pts',(7.1665058654886,3.61640598741355,-2.21160432106036));
#116009=CARTESIAN_POINT('Ctrl Pts',(7.1266181312516,3.62265476504783,-2.1994222532773));
#116010=CARTESIAN_POINT('Ctrl Pts',(7.08672423682204,3.62905099624073,-2.1872583156536));
#116011=CARTESIAN_POINT('Ctrl Pts',(7.00701313044391,3.64214708572923,-2.16299797339197));
#116012=CARTESIAN_POINT('Ctrl Pts',(6.96715263420202,3.64885405168379,-2.15088839165116));
#116013=CARTESIAN_POINT('Ctrl Pts',(6.92733463189405,3.65572482668139,-2.13881623722737));
#116014=CARTESIAN_POINT('Ctrl Pts',(7.12343270488168,3.52114709501716,-1.34905626701452));
#116015=CARTESIAN_POINT('Ctrl Pts',(7.12084049344087,3.52341350500855,-1.36246733900726));
#116016=CARTESIAN_POINT('Ctrl Pts',(7.118248282,3.525679915,-1.375878411));
#116017=CARTESIAN_POINT('Ctrl Pts',(7.04306438,3.591414347,-1.764850046));
#116018=CARTESIAN_POINT('Ctrl Pts',(6.925944539,3.656498153,-2.14331338));
#116019=CARTESIAN_POINT('Ctrl Pts',(7.3197397245431,3.52114709501716,-1.63708893683821));
#116020=CARTESIAN_POINT('Ctrl Pts',(7.31660346185319,3.52341350500854,-1.65086780930878));
#116021=CARTESIAN_POINT('Ctrl Pts',(7.31346719916323,3.525679915,-1.66464668177927));
#116022=CARTESIAN_POINT('Ctrl Pts',(7.22250376037485,3.591414347,-2.06428591689887));
#116023=CARTESIAN_POINT('Ctrl Pts',(7.08853595975396,3.656498153,-2.45163394443485));
#116024=CARTESIAN_POINT('Origin',(-0.194934900058013,3.48216454405651,0.0302789327722805));
#116025=CARTESIAN_POINT('Ctrl Pts',(7.225547291,3.656505752,-0.594950714));
#116026=CARTESIAN_POINT('Ctrl Pts',(7.193156039,3.590992329,-0.988335434000001));
#116027=CARTESIAN_POINT('Ctrl Pts',(7.118248282,3.525679915,-1.375878411));
#116028=CARTESIAN_POINT('Ctrl Pts',(7.490867816,3.656505752,-0.369999136));
#116029=CARTESIAN_POINT('Ctrl Pts',(7.470723736,3.590992329,-0.777828857000001));
#116030=CARTESIAN_POINT('Ctrl Pts',(7.406422533,3.525679915,-1.181061074));
#116031=CARTESIAN_POINT('',(7.22515966529974,3.65572482707165,-0.599639729012796));
#116032=CARTESIAN_POINT('Origin',(-0.198301150914787,3.62499996314961,0.0215660772445236));
#116033=CARTESIAN_POINT('Ctrl Pts',(7.47438649549291,3.61640598739533,-0.619311320060682));
#116034=CARTESIAN_POINT('Ctrl Pts',(7.43281252968464,3.62265476505147,-0.615988746101276));
#116035=CARTESIAN_POINT('Ctrl Pts',(7.39123644540361,3.62905099622712,-0.612685202723241));
#116036=CARTESIAN_POINT('Ctrl Pts',(7.30817373059722,3.64214707835014,-0.60612758932348));
#116037=CARTESIAN_POINT('Ctrl Pts',(7.26664192340405,3.64885404807934,-0.60286994943576));
#116038=CARTESIAN_POINT('Ctrl Pts',(7.22515966554175,3.65572482670755,-0.599639727228977));
#116039=CARTESIAN_POINT('Ctrl Pts',(7.24689802585418,3.52114709524965,0.213811382512832));
#116040=CARTESIAN_POINT('Ctrl Pts',(7.2472494029271,3.5234135051248,0.200156605756419));
#116041=CARTESIAN_POINT('Ctrl Pts',(7.24760078,3.525679915,0.186501829));
#116042=CARTESIAN_POINT('Ctrl Pts',(7.25779204,3.591414347,-0.209538183));
#116043=CARTESIAN_POINT('Ctrl Pts',(7.224768825,3.656498153,-0.604330558));
#116044=CARTESIAN_POINT('Ctrl Pts',(7.50053400671784,3.52114709524965,-0.0252870375102526));
#116045=CARTESIAN_POINT('Ctrl Pts',(7.50043311840226,3.5234135051248,-0.0394179706665876));
#116046=CARTESIAN_POINT('Ctrl Pts',(7.50033223008661,3.525679915,-0.0535489038229223));
#116047=CARTESIAN_POINT('Ctrl Pts',(7.49740608852792,3.591414347,-0.463399246793597));
#116048=CARTESIAN_POINT('Ctrl Pts',(7.44983875710106,3.656498153,-0.870490409396995));
#116049=CARTESIAN_POINT('Origin',(-0.196886367454507,3.48216458971207,-0.0123342117782992));
#116050=CARTESIAN_POINT('Ctrl Pts',(7.184514827,3.656505752,0.972237985));
#116051=CARTESIAN_POINT('Ctrl Pts',(7.23744695100001,3.590992329,0.58108722));
#116052=CARTESIAN_POINT('Ctrl Pts',(7.24760078,3.525679915,0.186501829));
#116053=CARTESIAN_POINT('Ctrl Pts',(7.395274366,3.656505752,1.24896639));
#116054=CARTESIAN_POINT('Ctrl Pts',(7.463272578,3.590992329,0.84634112));
#116055=CARTESIAN_POINT('Ctrl Pts',(7.487157709,3.525679915,0.43871339));
#116056=CARTESIAN_POINT('',(7.18514426360252,3.65572482705992,0.967575269034057));
#116057=CARTESIAN_POINT('Origin',(-0.198300997752782,3.62499997613515,-0.0215670094842793));
#116058=CARTESIAN_POINT('Ctrl Pts',(7.43277311966718,3.61640598738244,1.00193998978875));
#116059=CARTESIAN_POINT('Ctrl Pts',(7.39145687490788,3.62265476503386,0.996247710126081));
#116060=CARTESIAN_POINT('Ctrl Pts',(7.35014265232034,3.62905099618932,0.990536389400853));
#116061=CARTESIAN_POINT('Ctrl Pts',(7.26761217221783,3.64214708344315,0.979084656609767));
#116062=CARTESIAN_POINT('Ctrl Pts',(7.22635107668164,3.64885405053422,0.973338026201712));
#116063=CARTESIAN_POINT('Ctrl Pts',(7.18514426386498,3.65572482661952,0.967575270475477));
#116064=CARTESIAN_POINT('Ctrl Pts',(7.03615984138259,3.52436392548355,1.74786086090946));
#116065=CARTESIAN_POINT('Ctrl Pts',(7.0371116811913,3.52502192024177,1.74401115545473));
#116066=CARTESIAN_POINT('Ctrl Pts',(7.038063521,3.525679915,1.74016145));
#116067=CARTESIAN_POINT('Ctrl Pts',(7.133153411,3.591414347,1.355571454));
#116068=CARTESIAN_POINT('Ctrl Pts',(7.185770951,3.656498153,0.962910089));
#116069=CARTESIAN_POINT('Ctrl Pts',(7.33416912307217,3.52436392548355,1.56844846720524));
#116070=CARTESIAN_POINT('Ctrl Pts',(7.33502264903608,3.52502192024177,1.56443586310262));
#116071=CARTESIAN_POINT('Ctrl Pts',(7.335876175,3.525679915,1.560423259));
#116072=CARTESIAN_POINT('Ctrl Pts',(7.421144399,3.591414347,1.159559501));
#116073=CARTESIAN_POINT('Ctrl Pts',(7.462225511,3.656498153,0.751791473));
#116074=CARTESIAN_POINT('Origin',(-0.189631658845381,3.48216453482775,-0.0543705811770401));
#116075=CARTESIAN_POINT('Ctrl Pts',(6.807542435,3.656505752,2.493965916));
#116076=CARTESIAN_POINT('Ctrl Pts',(6.943322888,3.590992329,2.12333888));
#116077=CARTESIAN_POINT('Ctrl Pts',(7.038063521,3.525679915,1.74016145));
#116078=CARTESIAN_POINT('Ctrl Pts',(6.953886107,3.656505752,2.809531636));
#116079=CARTESIAN_POINT('Ctrl Pts',(7.10684709,3.590992329,2.430937126));
#116080=CARTESIAN_POINT('Ctrl Pts',(7.217801712,3.525679915,2.037974103));
#116081=CARTESIAN_POINT('',(6.80915950247847,3.65572482704387,2.48954752166462));
#116082=CARTESIAN_POINT('Origin',(-0.189028489598825,3.62499993456761,-0.0636916109347949));
#116083=CARTESIAN_POINT('Ctrl Pts',(7.04361153430038,3.61640598744965,2.57634169922523));
#116084=CARTESIAN_POINT('Ctrl Pts',(7.00448491229197,3.62265476508227,2.56190073060411));
#116085=CARTESIAN_POINT('Ctrl Pts',(6.96536435829456,3.62905099623963,2.5474416007531));
#116086=CARTESIAN_POINT('Ctrl Pts',(6.88722514371671,3.6421470893655,2.51851597651896));
#116087=CARTESIAN_POINT('Ctrl Pts',(6.84816408409976,3.64885405342756,2.50403379027225));
#116088=CARTESIAN_POINT('Ctrl Pts',(6.8091595022488,3.65572482658445,2.48954752411671));
#116089=CARTESIAN_POINT('Ctrl Pts',(6.49591991560068,3.52436392548355,3.21956322413365));
#116090=CARTESIAN_POINT('Ctrl Pts',(6.49767707480033,3.52502192024177,3.21600814006683));
#116091=CARTESIAN_POINT('Ctrl Pts',(6.499434234,3.525679915,3.212453056));
#116092=CARTESIAN_POINT('Ctrl Pts',(6.674976456,3.591414347,2.857296075));
#116093=CARTESIAN_POINT('Ctrl Pts',(6.810774414,3.656498153,2.485126131));
#116094=CARTESIAN_POINT('Ctrl Pts',(6.82553026747355,3.52436392548355,3.10840857858364));
#116095=CARTESIAN_POINT('Ctrl Pts',(6.82722642973678,3.52502192024177,3.10467326979182));
#116096=CARTESIAN_POINT('Ctrl Pts',(6.828922592,3.525679915,3.100937961));
#116097=CARTESIAN_POINT('Ctrl Pts',(6.99837115,3.591414347,2.727776323));
#116098=CARTESIAN_POINT('Ctrl Pts',(7.126149882,3.656498153,2.33837291));
#116099=CARTESIAN_POINT('Origin',(-0.173510263844352,3.48216456917264,-0.0938646918006852));
#116100=CARTESIAN_POINT('Ctrl Pts',(6.112256925,3.656505752,3.899078773));
#116101=CARTESIAN_POINT('Ctrl Pts',(6.324536764,3.590992329,3.566305575));
#116102=CARTESIAN_POINT('Ctrl Pts',(6.499434234,3.525679915,3.212453056));
#116103=CARTESIAN_POINT('Ctrl Pts',(6.187341861,3.656505752,4.238726305));
#116104=CARTESIAN_POINT('Ctrl Pts',(6.41811333,3.590992329,3.901865214));
#116105=CARTESIAN_POINT('Ctrl Pts',(6.610949329,3.525679915,3.541941413));
#116106=CARTESIAN_POINT('',(6.11478601009459,3.65572482707945,3.89511130062054));
#116107=CARTESIAN_POINT('Origin',(-0.170917169114783,3.62499992226006,-0.102838001281196));
#116108=CARTESIAN_POINT('Ctrl Pts',(6.32509850137208,3.6164059874298,4.03027653421334));
#116109=CARTESIAN_POINT('Ctrl Pts',(6.28999101930424,3.62265476509319,4.00776212019126));
#116110=CARTESIAN_POINT('Ctrl Pts',(6.25489336773236,3.62905099624141,3.98523127410475));
#116111=CARTESIAN_POINT('Ctrl Pts',(6.18479924655914,3.64214707297698,3.94018434989972));
#116112=CARTESIAN_POINT('Ctrl Pts',(6.14976460795097,3.64885404539754,3.91764374585424));
#116113=CARTESIAN_POINT('Ctrl Pts',(6.11478600941526,3.6557248266398,3.89511130181848));
#116114=CARTESIAN_POINT('Ctrl Pts',(5.65193799443724,3.52436392548355,4.54072238877234));
#116115=CARTESIAN_POINT('Ctrl Pts',(5.65441831021862,3.52502192024177,4.53762815788617));
#116116=CARTESIAN_POINT('Ctrl Pts',(5.656898626,3.525679915,4.534533927));
#116117=CARTESIAN_POINT('Ctrl Pts',(5.904685021,3.591414347,4.225416708));
#116118=CARTESIAN_POINT('Ctrl Pts',(6.117313634,3.656498153,3.891140437));
#116119=CARTESIAN_POINT('Ctrl Pts',(5.9977372021746,3.52436392548355,4.5030229591959));
#116120=CARTESIAN_POINT('Ctrl Pts',(6.00019669008729,3.52502192024177,4.49973960459795));
#116121=CARTESIAN_POINT('Ctrl Pts',(6.002656178,3.525679915,4.49645625));
#116122=CARTESIAN_POINT('Ctrl Pts',(6.248361845,3.591414347,4.168445355));
#116123=CARTESIAN_POINT('Ctrl Pts',(6.45686340400001,3.656498153,3.815614628));
#116124=CARTESIAN_POINT('Origin',(-0.149275386552372,3.48216457406842,-0.128969635675024));
#116125=CARTESIAN_POINT('Ctrl Pts',(5.131169075,3.656505752,5.12187504));
#116126=CARTESIAN_POINT('Ctrl Pts',(5.410022329,3.590992329,4.842515785));
#116127=CARTESIAN_POINT('Ctrl Pts',(5.656898626,3.525679915,4.534533927));
#116128=CARTESIAN_POINT('Ctrl Pts',(5.131484387,3.656505752,5.469722844));
#116129=CARTESIAN_POINT('Ctrl Pts',(5.429275724,3.590992329,5.19034642200001));
#116130=CARTESIAN_POINT('Ctrl Pts',(5.694976303,3.525679915,4.880291478));
#116131=CARTESIAN_POINT('',(5.1344919203829,3.65572482709323,5.11854400289229));
#116132=CARTESIAN_POINT('Origin',(-0.144814243661942,3.62499997372534,-0.137175988992));
#116133=CARTESIAN_POINT('Ctrl Pts',(5.31083089269157,3.61640598739114,5.29576011741492));
#116134=CARTESIAN_POINT('Ctrl Pts',(5.28138452430637,3.62265468298331,5.26622539498499));
#116135=CARTESIAN_POINT('Ctrl Pts',(5.25195069654516,3.62905095586431,5.23667614406137));
#116136=CARTESIAN_POINT('Ctrl Pts',(5.19317884859688,3.64214708734628,5.1776139811862));
#116137=CARTESIAN_POINT('Ctrl Pts',(5.16380889825466,3.64885405250065,5.14806898668562));
#116138=CARTESIAN_POINT('Ctrl Pts',(5.13449191955353,3.65572482670683,5.11854400434703));
#116139=CARTESIAN_POINT('Ctrl Pts',(4.52858346663779,3.52114709512928,5.66172924920744));
#116140=CARTESIAN_POINT('Ctrl Pts',(4.53921809631889,3.52341350506461,5.65315714010372));
#116141=CARTESIAN_POINT('Ctrl Pts',(4.549852726,3.525679915,5.644585031));
#116142=CARTESIAN_POINT('Ctrl Pts',(4.858297077,3.591414347,5.395961552));
#116143=CARTESIAN_POINT('Ctrl Pts',(5.137814068,3.656498153,5.115209341));
#116144=CARTESIAN_POINT('Ctrl Pts',(4.87501566544565,3.52114709512928,5.70025193256472));
#116145=CARTESIAN_POINT('Ctrl Pts',(4.88572041302767,3.52341350506461,5.69102686673961));
#116146=CARTESIAN_POINT('Ctrl Pts',(4.89642516060955,3.525679915,5.68180180091448));
#116147=CARTESIAN_POINT('Ctrl Pts',(5.20690319506136,3.591414347,5.41424011548773));
#116148=CARTESIAN_POINT('Ctrl Pts',(5.48637819367963,3.656498153,5.11444086518291));
#116149=CARTESIAN_POINT('Origin',(-0.118060676874366,3.4821645603223,-0.158044115061321));
#116150=CARTESIAN_POINT('Ctrl Pts',(3.910153461,3.656505752,6.105178123));
#116151=CARTESIAN_POINT('Ctrl Pts',(4.242541264,3.590992329,5.89229533900001));
#116152=CARTESIAN_POINT('Ctrl Pts',(4.549852726,3.525679915,5.644585031));
#116153=CARTESIAN_POINT('Ctrl Pts',(3.835684406,3.656505752,6.44496122100001));
#116154=CARTESIAN_POINT('Ctrl Pts',(4.18657122,3.590992329,6.236132799));
#116155=CARTESIAN_POINT('Ctrl Pts',(4.512712514,3.525679915,5.990444538));
#116156=CARTESIAN_POINT('',(3.91411469504543,3.65572482704546,6.1026392772109));
#116157=CARTESIAN_POINT('Origin',(-0.111939653749157,3.6249999645308,-0.165099488252253));
#116158=CARTESIAN_POINT('Ctrl Pts',(4.04823473411853,3.61640598738466,6.31361984386591));
#116159=CARTESIAN_POINT('Ctrl Pts',(4.02582560354184,3.62265476502366,6.27844506607371));
#116160=CARTESIAN_POINT('Ctrl Pts',(4.00343229437542,3.62905099618508,6.24325950250079));
#116161=CARTESIAN_POINT('Ctrl Pts',(3.95873127978742,3.64214708044663,6.17294422349425));
#116162=CARTESIAN_POINT('Ctrl Pts',(3.93639927058861,3.64885404904875,6.13777628396584));
#116163=CARTESIAN_POINT('Ctrl Pts',(3.91411469397674,3.65572482660295,6.10263927839537));
#116164=CARTESIAN_POINT('Ctrl Pts',(3.20560327165695,3.52114709508196,6.50287274703964));
#116165=CARTESIAN_POINT('Ctrl Pts',(3.21783201982848,3.52341350504095,6.49678718001982));
#116166=CARTESIAN_POINT('Ctrl Pts',(3.230060768,3.525679915,6.490701613));
#116167=CARTESIAN_POINT('Ctrl Pts',(3.584740561,3.591414347,6.31419723));
#116168=CARTESIAN_POINT('Ctrl Pts',(3.918076027,3.656498153,6.100096741));
#116169=CARTESIAN_POINT('Ctrl Pts',(3.53565483972605,3.52114709508197,6.6149674737033));
#116170=CARTESIAN_POINT('Ctrl Pts',(3.54809243290119,3.52341350504095,6.60825928905035));
#116171=CARTESIAN_POINT('Ctrl Pts',(3.56053002607633,3.525679915,6.60155110439752));
#116172=CARTESIAN_POINT('Ctrl Pts',(3.92126711141813,3.591414347,6.40698846309505));
#116173=CARTESIAN_POINT('Ctrl Pts',(4.25865611687768,3.656498153,6.17427721525413));
#116174=CARTESIAN_POINT('Origin',(-0.0813257725780459,3.48216458113227,
-0.179728872209758));
#116175=CARTESIAN_POINT('Ctrl Pts',(2.506303418,3.656505752,6.803009862));
#116176=CARTESIAN_POINT('Ctrl Pts',(2.876683684,3.590992329,6.666557711));
#116177=CARTESIAN_POINT('Ctrl Pts',(3.230060768,3.525679915,6.490701613));
#116178=CARTESIAN_POINT('Ctrl Pts',(2.360532086,3.656505752,7.118840374));
#116179=CARTESIAN_POINT('Ctrl Pts',(2.748107298,3.590992329,6.99032453800001));
#116180=CARTESIAN_POINT('Ctrl Pts',(3.119439304,3.525679915,6.82049107000001));
#116181=CARTESIAN_POINT('',(2.51071781714977,3.65572482706423,6.8013819211087));
#116182=CARTESIAN_POINT('Origin',(-0.0738311105697187,3.62499995453911,
-0.185303373843084));
#116183=CARTESIAN_POINT('Ctrl Pts',(2.59634761838851,3.61640598745063,7.03626172327406));
#116184=CARTESIAN_POINT('Ctrl Pts',(2.58202393835233,3.6226547650867,6.99709201155439));
#116185=CARTESIAN_POINT('Ctrl Pts',(2.56771802844582,3.62905099626518,6.95791516722619));
#116186=CARTESIAN_POINT('Ctrl Pts',(2.53917783475695,3.64214706707844,6.87963450385756));
#116187=CARTESIAN_POINT('Ctrl Pts',(2.52492798746055,3.64885404252505,6.84048800649528));
#116188=CARTESIAN_POINT('Ctrl Pts',(2.51071781591352,3.65572482669336,6.80138192161454));
#116189=CARTESIAN_POINT('Ctrl Pts',(1.73273263100486,3.52114709502825,7.03994914305568));
#116190=CARTESIAN_POINT('Ctrl Pts',(1.74598369500246,3.5234135050141,7.03663467252785));
#116191=CARTESIAN_POINT('Ctrl Pts',(1.759234759,3.525679915,7.033320202));
#116192=CARTESIAN_POINT('Ctrl Pts',(2.14356556,3.591414347,6.937188064));
#116193=CARTESIAN_POINT('Ctrl Pts',(2.515133105,3.656498153,6.79975039700001));
#116194=CARTESIAN_POINT('Ctrl Pts',(2.03097072435524,3.52114709502825,7.22037448802775));
#116195=CARTESIAN_POINT('Ctrl Pts',(2.04455959505472,3.5234135050141,7.21649685182525));
#116196=CARTESIAN_POINT('Ctrl Pts',(2.05814846575428,3.525679915,7.21261921562272));
#116197=CARTESIAN_POINT('Ctrl Pts',(2.45227693435169,3.591414347,7.1001531504088));
#116198=CARTESIAN_POINT('Ctrl Pts',(2.83180401175584,3.656498153,6.94541122514516));
#116199=CARTESIAN_POINT('Origin',(-0.0407880620217441,3.48216455172988,
-0.193009651875642));
#116200=CARTESIAN_POINT('Ctrl Pts',(0.985261412,3.656505752,7.182740421));
#116201=CARTESIAN_POINT('Ctrl Pts',(1.376315572,3.590992329,7.129099254));
#116202=CARTESIAN_POINT('Ctrl Pts',(1.759234759,3.525679915,7.033320202));
#116203=CARTESIAN_POINT('Ctrl Pts',(0.775003908,3.656505752,7.459850464));
#116204=CARTESIAN_POINT('Ctrl Pts',(1.181144933,3.590992329,7.41765647));
#116205=CARTESIAN_POINT('Ctrl Pts',(1.580304579,3.525679915,7.331619019));
#116206=CARTESIAN_POINT('',(0.989922564157426,3.65572482707808,7.18209950545577));
#116207=CARTESIAN_POINT('Origin',(-0.032270264785814,3.62499995560225,-0.196842784054748));
#116208=CARTESIAN_POINT('Ctrl Pts',(1.02305817352954,3.61640598741002,7.42989582473919));
#116209=CARTESIAN_POINT('Ctrl Pts',(1.01748970331473,3.62265476506886,7.3885627112426));
#116210=CARTESIAN_POINT('Ctrl Pts',(1.01194012110595,3.62905099625209,7.34722645205932));
#116211=CARTESIAN_POINT('Ctrl Pts',(1.00089520291465,3.64214707546473,7.26464059626709));
#116212=CARTESIAN_POINT('Ctrl Pts',(0.995393852702379,3.64885404668247,
7.22334605429106));
#116213=CARTESIAN_POINT('Ctrl Pts',(0.989922562679225,3.65572482674932,
7.18209950578354));
#116214=CARTESIAN_POINT('Ctrl Pts',(0.178841338619978,3.52114709502879,
7.24784534093733));
#116215=CARTESIAN_POINT('Ctrl Pts',(0.192495113309986,3.52341350501437,
7.24745694796873));
#116216=CARTESIAN_POINT('Ctrl Pts',(0.206148888,3.525679915,7.247068555));
#116217=CARTESIAN_POINT('Ctrl Pts',(0.602159817,3.591414347,7.235803695));
#116218=CARTESIAN_POINT('Ctrl Pts',(0.994585354,3.656498153,7.181455282));
#116219=CARTESIAN_POINT('Ctrl Pts',(0.431320675651514,3.52114709502879,
7.4881648150128));
#116220=CARTESIAN_POINT('Ctrl Pts',(0.445425423261039,3.52341350501437,
7.48729904133021));
#116221=CARTESIAN_POINT('Ctrl Pts',(0.459530170870565,3.525679915,7.48643326764763));
#116222=CARTESIAN_POINT('Ctrl Pts',(0.868621014316521,3.591414347,7.46132256763059));
#116223=CARTESIAN_POINT('Ctrl Pts',(1.27253989906597,3.656498153,7.39178552538709));
#116224=CARTESIAN_POINT('Origin',(0.00165692198660666,3.48216459974148,
-0.197265124310521));
#116225=CARTESIAN_POINT('Ctrl Pts',(-0.581850323,3.656505752,7.226614021));
#116226=CARTESIAN_POINT('Ctrl Pts',(-0.188407526,3.590992329,7.25829204));
#116227=CARTESIAN_POINT('Ctrl Pts',(0.206148888,3.525679915,7.247068555));
#116228=CARTESIAN_POINT('Ctrl Pts',(-0.846762591,3.656505752,7.452046237));
#116229=CARTESIAN_POINT('Ctrl Pts',(-0.441046456,3.590992329,7.49814703));
#116230=CARTESIAN_POINT('Ctrl Pts',(-0.032723432,3.525679915,7.499928611));
#116231=CARTESIAN_POINT('Origin',(0.0107995551809671,3.62499992801169,-0.199177769006146));
#116232=CARTESIAN_POINT('Ctrl Pts',(0.206121509127986,2.23138000478158,
7.24707355226295));
#116233=CARTESIAN_POINT('Ctrl Pts',(0.210029728063993,2.23202203989079,
7.24695817563148));
#116234=CARTESIAN_POINT('Ctrl Pts',(0.213937947,2.232664075,7.24684279900001));
#116235=CARTESIAN_POINT('Ctrl Pts',(0.606333568,2.297126115,7.23525867700001));
#116236=CARTESIAN_POINT('Ctrl Pts',(0.995184151,2.362252267,7.181372327));
#116237=CARTESIAN_POINT('Ctrl Pts',(0.458980806959231,2.23138000478158,
7.48594697166454));
#116238=CARTESIAN_POINT('Ctrl Pts',(0.463017702979616,2.23202203989079,
7.48569508933227));
#116239=CARTESIAN_POINT('Ctrl Pts',(0.467054599,2.232664075,7.48544320700001));
#116240=CARTESIAN_POINT('Ctrl Pts',(0.872369743,2.297126115,7.460153548));
#116241=CARTESIAN_POINT('Ctrl Pts',(1.272584422,2.362252267,7.391246775));
#116242=CARTESIAN_POINT('',(0.467054605055031,2.23266407419427,7.48544320450419));
#116243=CARTESIAN_POINT('',(1.02641184425845,2.32233405367783,7.42943327080472));
#116244=CARTESIAN_POINT('Origin',(-0.0399076795548507,2.41067415053388,
-0.185339256409806));
#116245=CARTESIAN_POINT('Ctrl Pts',(0.990540536095505,2.36147458198366,
7.18201430225601));
#116246=CARTESIAN_POINT('Ctrl Pts',(0.996473310122438,2.35461430679531,
7.22319414246324));
#116247=CARTESIAN_POINT('Ctrl Pts',(1.00243339649902,2.34792815753381,7.26442562949533));
#116248=CARTESIAN_POINT('Ctrl Pts',(1.01438950164634,2.33489257429051,7.34688486757673));
#116249=CARTESIAN_POINT('Ctrl Pts',(1.02039254146659,2.32853549393583,7.38816102848141));
#116250=CARTESIAN_POINT('Ctrl Pts',(1.02641184256769,2.32233405371974,7.42943327094841));
#116251=CARTESIAN_POINT('',(0.340496287632723,2.23266407264717,7.36614300232361));
#116252=CARTESIAN_POINT('Origin',(-9.86623976961809E-15,2.32340998499933,
-2.43728648374741E-13));
#116253=CARTESIAN_POINT('',(1.02848533178705,2.14301213123783,7.42914651337806));
#116254=CARTESIAN_POINT('Origin',(-0.0453595884940869,2.01794103942791,
-0.181798662226462));
#116255=CARTESIAN_POINT('',(1.58818371752705,2.23266407449123,7.3299162650956));
#116256=CARTESIAN_POINT('Origin',(-0.0659827140321631,2.41052396785092,
-0.170978110656799));
#116257=CARTESIAN_POINT('Ctrl Pts',(1.02641184540738,2.3223340532383,7.42943327079627));
#116258=CARTESIAN_POINT('Ctrl Pts',(1.1035495486996,2.31006874162245,7.41877632682905));
#116259=CARTESIAN_POINT('Ctrl Pts',(1.18040467460891,2.29785936479557,7.40693385917979));
#116260=CARTESIAN_POINT('Ctrl Pts',(1.25692390206011,2.28571428601282,7.39392604080063));
#116261=CARTESIAN_POINT('Ctrl Pts',(1.36754346318794,2.26815682559423,7.37512136685907));
#116262=CARTESIAN_POINT('Ctrl Pts',(1.47802088647235,2.25046493734972,7.35378540900434));
#116263=CARTESIAN_POINT('Ctrl Pts',(1.58818372237067,2.23266407446841,7.32991626615202));
#116264=CARTESIAN_POINT('Ctrl Pts',(0.985822492000001,2.36225522,7.182663435));
#116265=CARTESIAN_POINT('Ctrl Pts',(1.218577958,2.323743665,7.15071768400001));
#116266=CARTESIAN_POINT('Ctrl Pts',(1.448776863,2.285714286,7.103769816));
#116267=CARTESIAN_POINT('Ctrl Pts',(1.608598834,2.259311335,7.071174957));
#116268=CARTESIAN_POINT('Ctrl Pts',(1.766793184,2.232664075,7.031425307));
#116269=CARTESIAN_POINT('Ctrl Pts',(1.77065896195487,2.23201289883432,7.03045394916905));
#116270=CARTESIAN_POINT('Ctrl Pts',(1.77452473990974,2.23136172266864,7.02948259133811));
#116271=CARTESIAN_POINT('Ctrl Pts',(0.775586635,2.36225522,7.459789901));
#116272=CARTESIAN_POINT('Ctrl Pts',(1.017322434,2.323743665,7.43465688100001));
#116273=CARTESIAN_POINT('Ctrl Pts',(1.256923902,2.285714286,7.393926041));
#116274=CARTESIAN_POINT('Ctrl Pts',(1.423273863,2.259311335,7.365647527));
#116275=CARTESIAN_POINT('Ctrl Pts',(1.588183719,2.232664075,7.329916267));
#116276=CARTESIAN_POINT('Ctrl Pts',(1.59221360303736,2.23201289883432,7.3290431061241));
#116277=CARTESIAN_POINT('Ctrl Pts',(1.59624348707472,2.23136172266864,7.32816994524821));
#116278=CARTESIAN_POINT('',(1.6774884429112,2.23266407357604,7.18067078900645));
#116279=CARTESIAN_POINT('Ctrl Pts',(1.7592090952449,2.23138000478158,7.03333096846917));
#116280=CARTESIAN_POINT('Ctrl Pts',(1.76300113962245,2.23202203989079,7.03237813773459));
#116281=CARTESIAN_POINT('Ctrl Pts',(1.766793184,2.232664075,7.031425307));
#116282=CARTESIAN_POINT('Ctrl Pts',(2.147524569,2.297126115,6.935758556));
#116283=CARTESIAN_POINT('Ctrl Pts',(2.51570007,2.362252267,6.799540658));
#116284=CARTESIAN_POINT('Ctrl Pts',(2.05750740624301,2.23138000478158,7.21226238556066));
#116285=CARTESIAN_POINT('Ctrl Pts',(2.06139577462151,2.23202203989079,7.21114857878033));
#116286=CARTESIAN_POINT('Ctrl Pts',(2.065284143,2.232664075,7.210034772));
#116287=CARTESIAN_POINT('Ctrl Pts',(2.455686715,2.297126115,7.098205596));
#116288=CARTESIAN_POINT('Ctrl Pts',(2.831731678,2.362252267,6.944875499));
#116289=CARTESIAN_POINT('',(2.06528414837267,2.23266407419428,7.21003476826059));
#116290=CARTESIAN_POINT('',(2.59952344630951,2.32233405371967,7.03508904333622));
#116291=CARTESIAN_POINT('Origin',(-0.0788171249275074,2.41067414467123,
-0.172427152005246));
#116292=CARTESIAN_POINT('Ctrl Pts',(2.51130302491251,2.36147458180911,6.8011658645237));
#116293=CARTESIAN_POINT('Ctrl Pts',(2.52594953276537,2.3546143112292,6.84010754589003));
#116294=CARTESIAN_POINT('Ctrl Pts',(2.54063381526986,2.34792816677927,6.8790937912037));
#116295=CARTESIAN_POINT('Ctrl Pts',(2.57003670947,2.33489257586038,6.95705501495986));
#116296=CARTESIAN_POINT('Ctrl Pts',(2.58477255187177,2.32853549717823,6.99607567507759));
#116297=CARTESIAN_POINT('Ctrl Pts',(2.59952344478407,2.32233405377372,7.03508904374644));
#116298=CARTESIAN_POINT('',(1.91603867764522,2.23266407264717,7.12073003569382));
#116299=CARTESIAN_POINT('Origin',(2.3115190317391E-13,2.32340998499989,
6.26668855696622E-13));
#116300=CARTESIAN_POINT('',(2.60148681280772,2.14301213126887,7.0343632519323));
#116301=CARTESIAN_POINT('Origin',(-0.0833804322487564,2.01794103357697,
-0.167797302228523));
#116302=CARTESIAN_POINT('',(3.12676819112557,2.23266407449122,6.8171343424829));
#116303=CARTESIAN_POINT('Origin',(-0.101195453099118,2.41052401725478,-0.152796690784625));
#116304=CARTESIAN_POINT('Ctrl Pts',(2.59952344744715,2.32233405329015,7.03508904319684));
#116305=CARTESIAN_POINT('Ctrl Pts',(2.67256678623818,2.31006874164898,7.00809892682557));
#116306=CARTESIAN_POINT('Ctrl Pts',(2.74507930171928,2.29785936480543,6.980011749429));
#116307=CARTESIAN_POINT('Ctrl Pts',(2.81701325564113,2.28571428610092,6.95085867462188));
#116308=CARTESIAN_POINT('Ctrl Pts',(2.92100414282236,2.26815682581014,6.90871370711777));
#116309=CARTESIAN_POINT('Ctrl Pts',(3.02431206591993,2.25046493734972,6.86412719177494));
#116310=CARTESIAN_POINT('Ctrl Pts',(3.12676819610958,2.23266407446841,6.81713434244728));
#116311=CARTESIAN_POINT('Ctrl Pts',(2.50683483,2.36225522,6.80281406));
#116312=CARTESIAN_POINT('Ctrl Pts',(2.727281211,2.323743665,6.721579638));
#116313=CARTESIAN_POINT('Ctrl Pts',(2.94200579,2.285714286,6.626243425));
#116314=CARTESIAN_POINT('Ctrl Pts',(3.09108428,2.259311335,6.560053617));
#116315=CARTESIAN_POINT('Ctrl Pts',(3.237035134,2.232664075,6.487226182));
#116316=CARTESIAN_POINT('Ctrl Pts',(3.24060171898795,2.23201289883432,6.48544650597028));
#116317=CARTESIAN_POINT('Ctrl Pts',(3.24416830397589,2.23136172266864,6.48366682994055));
#116318=CARTESIAN_POINT('Ctrl Pts',(2.36108817,2.36225522,7.118655958));
#116319=CARTESIAN_POINT('Ctrl Pts',(2.591769463,2.323743665,7.042144483));
#116320=CARTESIAN_POINT('Ctrl Pts',(2.817013256,2.285714286,6.950858675));
#116321=CARTESIAN_POINT('Ctrl Pts',(2.973395002,2.259311335,6.887480972));
#116322=CARTESIAN_POINT('Ctrl Pts',(3.126768193,2.232664075,6.817134344));
#116323=CARTESIAN_POINT('Ctrl Pts',(3.13051615682195,2.23201289883432,6.81541529117844));
#116324=CARTESIAN_POINT('Ctrl Pts',(3.13426412064389,2.23136172266864,6.81369623835689));
#116325=CARTESIAN_POINT('',(3.18190165554338,2.23266407357605,6.65218026680585));
#116326=CARTESIAN_POINT('Ctrl Pts',(3.2300380178948,2.23138000478159,6.49071764506209));
#116327=CARTESIAN_POINT('Ctrl Pts',(3.2335365759474,2.23202203989079,6.48897191353105));
#116328=CARTESIAN_POINT('Ctrl Pts',(3.237035134,2.232664075,6.48722618199999));
#116329=CARTESIAN_POINT('Ctrl Pts',(3.588299708,2.297126115,6.31195007300001));
#116330=CARTESIAN_POINT('Ctrl Pts',(3.918584648,2.362252267,6.099770025));
#116331=CARTESIAN_POINT('Ctrl Pts',(3.55982724710697,2.23138000478159,6.60134042570219));
#116332=CARTESIAN_POINT('Ctrl Pts',(3.56338527205348,2.23202203989079,6.5994167748511));
#116333=CARTESIAN_POINT('Ctrl Pts',(3.566943297,2.232664075,6.597493124));
#116334=CARTESIAN_POINT('Ctrl Pts',(3.924178506,2.297126115,6.40435344));
#116335=CARTESIAN_POINT('Ctrl Pts',(4.258470309,2.362252267,6.173769564));
#116336=CARTESIAN_POINT('',(3.5669433014604,2.23266407419313,6.59749311918321));
#116337=CARTESIAN_POINT('',(4.0510842215557,2.32233405368084,6.31179187167886));
#116338=CARTESIAN_POINT('Origin',(-0.114041131822303,2.41067409909671,-0.151452518478992));
#116339=CARTESIAN_POINT('Ctrl Pts',(3.91463977526644,2.36147458191302,6.10230246946548));
#116340=CARTESIAN_POINT('Ctrl Pts',(3.93731515696421,2.35461431419793,6.13718513497579));
#116341=CARTESIAN_POINT('Ctrl Pts',(3.96003700857577,2.3479281727242,6.17210320002542));
#116342=CARTESIAN_POINT('Ctrl Pts',(4.00551186472225,2.33489257415327,6.24192102140471));
#116343=CARTESIAN_POINT('Ctrl Pts',(4.02829148668957,2.32853549366127,6.27686164025753));
#116344=CARTESIAN_POINT('Ctrl Pts',(4.05108422007071,2.32233405372159,6.31179187253635));
#116345=CARTESIAN_POINT('',(3.40198922851562,2.23266407264367,6.54235964623195));
#116346=CARTESIAN_POINT('Origin',(-3.07046055247895E-13,2.32340998499933,
-6.88251539093798E-13));
#116347=CARTESIAN_POINT('',(4.05284566193626,2.14301213127652,6.31066098286521));
#116348=CARTESIAN_POINT('Origin',(-0.117502649176756,2.01794102805717,-0.145950205159407));
#116349=CARTESIAN_POINT('',(4.51914845885334,2.23266407449122,5.98559079590574));
#116350=CARTESIAN_POINT('Origin',(-0.131676465731563,2.41052406519318,-0.127470530570108));
#116351=CARTESIAN_POINT('Ctrl Pts',(4.05108422259417,2.32233405323947,6.3117918711683));
#116352=CARTESIAN_POINT('Ctrl Pts',(4.11661777123175,2.3100687416239,6.26973060984927));
#116353=CARTESIAN_POINT('Ctrl Pts',(4.18139707119067,2.29785936479657,6.2267120475812));
#116354=CARTESIAN_POINT('Ctrl Pts',(4.24538220001676,2.28571428600411,6.18277688176229));
#116355=CARTESIAN_POINT('Ctrl Pts',(4.33788191716383,2.26815682557287,6.11926227365498));
#116356=CARTESIAN_POINT('Ctrl Pts',(4.42918977469998,2.25046493734972,6.05351001663829));
#116357=CARTESIAN_POINT('Ctrl Pts',(4.51914846370308,2.23266407446841,5.98559079481506));
#116358=CARTESIAN_POINT('Ctrl Pts',(3.910630358,2.36225522,6.104872661));
#116359=CARTESIAN_POINT('Ctrl Pts',(4.108459826,2.323743665,5.978147999));
#116360=CARTESIAN_POINT('Ctrl Pts',(4.297669796,2.285714286,5.838881257));
#116361=CARTESIAN_POINT('Ctrl Pts',(4.429034062,2.259311335,5.74219146));
#116362=CARTESIAN_POINT('Ctrl Pts',(4.55591692,2.232664075,5.639691571));
#116363=CARTESIAN_POINT('Ctrl Pts',(4.55901754246412,2.23201289883432,5.6371867924711));
#116364=CARTESIAN_POINT('Ctrl Pts',(4.56211816492825,2.23136172266864,5.63468201394221));
#116365=CARTESIAN_POINT('Ctrl Pts',(3.836187846,2.36225522,6.444661575));
#116366=CARTESIAN_POINT('Ctrl Pts',(4.045028233,2.323743665,6.320349236));
#116367=CARTESIAN_POINT('Ctrl Pts',(4.2453822,2.285714286,6.182776882));
#116368=CARTESIAN_POINT('Ctrl Pts',(4.384483496,2.259311335,6.087263462));
#116369=CARTESIAN_POINT('Ctrl Pts',(4.519148461,2.232664075,5.985590797));
#116370=CARTESIAN_POINT('Ctrl Pts',(4.52243925395809,2.23201289883432,5.98310623325313));
#116371=CARTESIAN_POINT('Ctrl Pts',(4.52573004691619,2.23136172266864,5.98062166950626));
#116372=CARTESIAN_POINT('',(4.5375326835475,2.23266407357604,5.81264118942734));
#116373=CARTESIAN_POINT('Ctrl Pts',(4.54983395395533,2.23138000478158,5.64460557872374));
#116374=CARTESIAN_POINT('Ctrl Pts',(4.55287543697766,2.23202203989079,5.64214857486187));
#116375=CARTESIAN_POINT('Ctrl Pts',(4.55591692,2.232664075,5.639691571));
#116376=CARTESIAN_POINT('Ctrl Pts',(4.86128994,2.297126115,5.39300182));
#116377=CARTESIAN_POINT('Ctrl Pts',(5.138240564,2.362252267,5.114780924));
#116378=CARTESIAN_POINT('Ctrl Pts',(4.89569352152841,2.23138000478158,5.68174712431132));
#116379=CARTESIAN_POINT('Ctrl Pts',(4.89875483376421,2.23202203989079,5.67910357715566));
#116380=CARTESIAN_POINT('Ctrl Pts',(4.901816146,2.232664075,5.67646003));
#116381=CARTESIAN_POINT('Ctrl Pts',(5.209180072,2.297126115,5.411040834));
#116382=CARTESIAN_POINT('Ctrl Pts',(5.4860876,2.362252267,5.113985026));
#116383=CARTESIAN_POINT('',(4.90181614931828,2.23266407419428,5.67646002434556));
#116384=CARTESIAN_POINT('',(5.31322080074589,2.32233405367292,5.29336232676854));
#116385=CARTESIAN_POINT('Origin',(-0.143932727089013,2.41067416005679,-0.12339615861267));
#116386=CARTESIAN_POINT('Ctrl Pts',(5.13493232101444,2.36147458193287,5.1181021922724));
#116387=CARTESIAN_POINT('Ctrl Pts',(5.16457633450321,2.35461430775493,5.14729481144356));
#116388=CARTESIAN_POINT('Ctrl Pts',(5.19427334574813,2.34792815954324,5.1765120169118));
#116389=CARTESIAN_POINT('Ctrl Pts',(5.25369373417348,2.33489257381224,5.23492172925327));
#116390=CARTESIAN_POINT('Ctrl Pts',(5.28345198322634,2.32853549297563,5.26414851222337));
#116391=CARTESIAN_POINT('Ctrl Pts',(5.31322079946837,2.32233405371025,5.2933623279704));
#116392=CARTESIAN_POINT('',(4.72886654423971,2.23266407264716,5.65807579110616));
#116393=CARTESIAN_POINT('Origin',(-3.31765864780564E-13,2.32340998499933,
-3.35235311732518E-13));
#116394=CARTESIAN_POINT('',(5.31469795198158,2.14301213129531,5.29187922010486));
#116395=CARTESIAN_POINT('Origin',(-0.146130295056051,2.01794105968598,-0.117278192493951));
#116396=CARTESIAN_POINT('',(5.70021836766514,2.23266407449122,4.87416767540015));
#116397=CARTESIAN_POINT('Origin',(-0.156000037177539,2.41052396677109,-0.0961835375339043));
#116398=CARTESIAN_POINT('Ctrl Pts',(5.31322080163106,2.32233405322908,5.29336232599744));
#116399=CARTESIAN_POINT('Ctrl Pts',(5.36818028465233,2.31006874161876,5.23819665780963));
#116400=CARTESIAN_POINT('Ctrl Pts',(5.42219736154694,2.29785936479515,5.1822582110242));
#116401=CARTESIAN_POINT('Ctrl Pts',(5.47524179152955,2.28571428609777,5.12559531379656));
#116402=CARTESIAN_POINT('Ctrl Pts',(5.55192515209581,2.26815682580241,5.04368093717354));
#116403=CARTESIAN_POINT('Ctrl Pts',(5.62696349193861,2.25046493734972,4.95983744082139));
#116404=CARTESIAN_POINT('Ctrl Pts',(5.7002183721701,2.23266407446841,4.87416767328428));
#116405=CARTESIAN_POINT('Ctrl Pts',(5.131569157,2.36225522,5.121474201));
#116406=CARTESIAN_POINT('Ctrl Pts',(5.297531425,2.323743665,4.95518480299999));
#116407=CARTESIAN_POINT('Ctrl Pts',(5.452379538,2.285714286,4.77849949));
#116408=CARTESIAN_POINT('Ctrl Pts',(5.559887133,2.259311335,4.655830813));
#116409=CARTESIAN_POINT('Ctrl Pts',(5.661769094,2.232664075,4.52845125000001));
#116410=CARTESIAN_POINT('Ctrl Pts',(5.66425877229023,2.23201289883432,4.52533848961035));
#116411=CARTESIAN_POINT('Ctrl Pts',(5.66674845058047,2.23136172266864,4.5222257292207));
#116412=CARTESIAN_POINT('Ctrl Pts',(5.131911641,2.36225522,5.469321979));
#116413=CARTESIAN_POINT('Ctrl Pts',(5.30914597800001,2.323743665,5.303021483));
#116414=CARTESIAN_POINT('Ctrl Pts',(5.475241792,2.285714286,5.125595314));
#116415=CARTESIAN_POINT('Ctrl Pts',(5.59055841400001,2.259311335,5.002412278));
#116416=CARTESIAN_POINT('Ctrl Pts',(5.70021837,2.232664075,4.874167676));
#116417=CARTESIAN_POINT('Ctrl Pts',(5.70289811829972,2.23201289883432,4.87103377674732));
#116418=CARTESIAN_POINT('Ctrl Pts',(5.70557786659942,2.23136172266864,4.86789987749465));
#116419=CARTESIAN_POINT('',(5.68099372637676,2.23266407357604,4.70130946979503));
#116420=CARTESIAN_POINT('Ctrl Pts',(5.65688471072712,2.23138000478158,4.5345580288374));
#116421=CARTESIAN_POINT('Ctrl Pts',(5.65932690236356,2.23202203989079,4.5315046394187));
#116422=CARTESIAN_POINT('Ctrl Pts',(5.661769094,2.232664075,4.52845125));
#116423=CARTESIAN_POINT('Ctrl Pts',(5.906971658,2.297126115,4.221882796));
#116424=CARTESIAN_POINT('Ctrl Pts',(6.117638062,2.362252267,3.890630353));
#116425=CARTESIAN_POINT('Ctrl Pts',(6.00264260807393,2.23138000478158,4.49648164327883));
#116426=CARTESIAN_POINT('Ctrl Pts',(6.00506406403696,2.23202203989079,4.49324180913942));
#116427=CARTESIAN_POINT('Ctrl Pts',(6.00748552,2.232664075,4.490001975));
#116428=CARTESIAN_POINT('Ctrl Pts',(6.25060616700001,2.297126115,4.164713973));
#116429=CARTESIAN_POINT('Ctrl Pts',(6.457181533,2.362252267,3.815076231));
#116430=CARTESIAN_POINT('',(6.00748552200209,2.23266407419427,4.49000196877962));
#116431=CARTESIAN_POINT('',(6.32691708062088,2.32233405363403,4.0274210425946));
#116432=CARTESIAN_POINT('Origin',(-0.167094205500953,2.41067417005038,-0.0895699468138367));
#116433=CARTESIAN_POINT('Ctrl Pts',(6.11512113831182,2.36147458190962,3.89458514642993));
#116434=CARTESIAN_POINT('Ctrl Pts',(6.15034763234554,2.35461430951217,3.91672266572962));
#116435=CARTESIAN_POINT('Ctrl Pts',(6.18563116880774,2.34792816317999,3.9388728027073));
#116436=CARTESIAN_POINT('Ctrl Pts',(6.25621872661867,2.3348925730979,3.98314331589693));
#116437=CARTESIAN_POINT('Ctrl Pts',(6.29156414285186,2.32853549156021,4.00528965158357));
#116438=CARTESIAN_POINT('Ctrl Pts',(6.32691707962809,2.32233405366459,4.027421044131));
#116439=CARTESIAN_POINT('',(5.8346273159575,2.23266407264717,4.50922660090961));
#116440=CARTESIAN_POINT('Origin',(3.48679418671338E-13,2.32340998499922,
1.50270421106491E-13));
#116441=CARTESIAN_POINT('',(6.32804087298349,2.14301213123153,4.02565506642255));
#116442=CARTESIAN_POINT('Origin',(-0.167925446394461,2.01794106053296,-0.0831227669844309));
#116443=CARTESIAN_POINT('',(6.61475240058951,2.23266407449122,3.53483389192556));
#116444=CARTESIAN_POINT('Origin',(-0.173029777855993,2.41052396444191,-0.060399601320052));
#116445=CARTESIAN_POINT('Ctrl Pts',(6.32691708126275,2.32233405318557,4.02742104157157));
#116446=CARTESIAN_POINT('Ctrl Pts',(6.36873265401809,2.31006874159296,3.96173045210923));
#116447=CARTESIAN_POINT('Ctrl Pts',(6.40946172897266,2.29785936478348,3.89548774047974));
#116448=CARTESIAN_POINT('Ctrl Pts',(6.44908516184669,2.28571428602514,3.82874660589252));
#116449=CARTESIAN_POINT('Ctrl Pts',(6.5063665396354,2.26815682562442,3.73226268612071));
#116450=CARTESIAN_POINT('Ctrl Pts',(6.56162665075071,2.25046493734972,3.63424837905487));
#116451=CARTESIAN_POINT('Ctrl Pts',(6.61475240453563,2.23266407446841,3.53483388888147));
#116452=CARTESIAN_POINT('Ctrl Pts',(6.112561485,2.36225522,3.898601299));
#116453=CARTESIAN_POINT('Ctrl Pts',(6.23889634300001,2.323743665,3.700522674));
#116454=CARTESIAN_POINT('Ctrl Pts',(6.352142073,2.285714286,3.494680397));
#116455=CARTESIAN_POINT('Ctrl Pts',(6.43076606,2.259311335,3.351768692));
#116456=CARTESIAN_POINT('Ctrl Pts',(6.502883238,2.232664075,3.205465582));
#116457=CARTESIAN_POINT('Ctrl Pts',(6.50464555755743,2.23201289883432,3.20189038897088));
#116458=CARTESIAN_POINT('Ctrl Pts',(6.50640787711486,2.23136172266864,3.19831519594175));
#116459=CARTESIAN_POINT('Ctrl Pts',(6.187672952,2.36225522,4.238242965));
#116460=CARTESIAN_POINT('Ctrl Pts',(6.325013958,2.323743665,4.03773034));
#116461=CARTESIAN_POINT('Ctrl Pts',(6.449085162,2.285714286,3.828746606));
#116462=CARTESIAN_POINT('Ctrl Pts',(6.53522503500001,2.259311335,3.683653856));
#116463=CARTESIAN_POINT('Ctrl Pts',(6.614752403,2.232664075,3.534833892));
#116464=CARTESIAN_POINT('Ctrl Pts',(6.61669580455652,2.23201289883432,3.53119719488613));
#116465=CARTESIAN_POINT('Ctrl Pts',(6.61863920611304,2.23136172266864,3.52756049777226));
#116466=CARTESIAN_POINT('',(6.55881781646897,2.23266407357604,3.370149744845));
#116467=CARTESIAN_POINT('Ctrl Pts',(6.49942582582478,2.23138000478158,3.21247958576346));
#116468=CARTESIAN_POINT('Ctrl Pts',(6.5011545319124,2.23202203989079,3.20897258388173));
#116469=CARTESIAN_POINT('Ctrl Pts',(6.502883238,2.232664075,3.205465582));
#116470=CARTESIAN_POINT('Ctrl Pts',(6.676449947,2.297126115,2.853353225));
#116471=CARTESIAN_POINT('Ctrl Pts',(6.810981603,2.362252267,2.48455823));
#116472=CARTESIAN_POINT('Ctrl Pts',(6.82891479781365,2.23138000478158,3.10096567712822));
#116473=CARTESIAN_POINT('Ctrl Pts',(6.83058317290683,2.23202203989079,3.09728104706411));
#116474=CARTESIAN_POINT('Ctrl Pts',(6.832251548,2.232664075,3.093596417));
#116475=CARTESIAN_POINT('Ctrl Pts',(6.999760864,2.297126115,2.723649716));
#116476=CARTESIAN_POINT('Ctrl Pts',(7.126344834,2.362252267,2.337778712));
#116477=CARTESIAN_POINT('',(6.83225154862371,2.23266407419428,3.09359641048888));
#116478=CARTESIAN_POINT('',(7.04477374955499,2.32233405367244,2.57316202661038));
#116479=CARTESIAN_POINT('Origin',(-0.182442567298916,2.41067412336642,-0.05155556175439));
#116480=CARTESIAN_POINT('Ctrl Pts',(6.80937368739757,2.36147458196701,2.48896162643404));
#116481=CARTESIAN_POINT('Ctrl Pts',(6.84853550980437,2.35461431097957,2.50300892515723));
#116482=CARTESIAN_POINT('Ctrl Pts',(6.88775575231982,2.3479281660991,2.5170562837039));
#116483=CARTESIAN_POINT('Ctrl Pts',(6.96620988394452,2.33489257270089,2.54511754579731));
#116484=CARTESIAN_POINT('Ctrl Pts',(7.00548975460885,2.32853549069996,2.5591478939061));
#116485=CARTESIAN_POINT('Ctrl Pts',(7.04477374892139,2.3223340536994,2.57316202839838));
#116486=CARTESIAN_POINT('',(6.66756739925649,2.23266407264717,3.14953098625499));
#116487=CARTESIAN_POINT('Origin',(1.2641797331181E-12,2.32340998499933,
5.06756095419725E-13));
#116488=CARTESIAN_POINT('',(7.04549163556671,2.14301213123943,2.5711957558057));
#116489=CARTESIAN_POINT('Origin',(-0.181868274181169,2.01794103510997,-0.0450803477170658));
#116490=CARTESIAN_POINT('',(7.21998796362812,2.23266407449122,2.03021520441984));
#116491=CARTESIAN_POINT('Origin',(-0.181968764875902,2.4105239964154,-0.0217912721690444));
#116492=CARTESIAN_POINT('Ctrl Pts',(7.0447737499108,2.32233405321779,2.57316202540825));
#116493=CARTESIAN_POINT('Ctrl Pts',(7.07149016287349,2.3100687416172,2.50001813309078));
#116494=CARTESIAN_POINT('Ctrl Pts',(7.09702678981718,2.29785936479699,2.42656859183786));
#116495=CARTESIAN_POINT('Ctrl Pts',(7.1213764777493,2.28571428606199,2.35286996114428));
#116496=CARTESIAN_POINT('Ctrl Pts',(7.1565774577418,2.26815682571472,2.24632797948178));
#116497=CARTESIAN_POINT('Ctrl Pts',(7.18947543979843,2.25046493734972,2.13872590177396));
#116498=CARTESIAN_POINT('Ctrl Pts',(7.21998796682949,2.23266407446841,2.0302152006245));
#116499=CARTESIAN_POINT('Ctrl Pts',(6.807737232,2.36225522,2.493434134));
#116500=CARTESIAN_POINT('Ctrl Pts',(6.888537402,2.323743665,2.272828217));
#116501=CARTESIAN_POINT('Ctrl Pts',(6.954885505,2.285714286,2.047453934));
#116502=CARTESIAN_POINT('Ctrl Pts',(7.000949515,2.259311335,1.890981591));
#116503=CARTESIAN_POINT('Ctrl Pts',(7.039929788,2.232664075,1.732595906));
#116504=CARTESIAN_POINT('Ctrl Pts',(7.0408823446497,2.23201289883432,1.72872545241275));
#116505=CARTESIAN_POINT('Ctrl Pts',(7.04183490129941,2.23136172266864,1.7248549988255));
#116506=CARTESIAN_POINT('Ctrl Pts',(6.954105553,2.36225522,2.808988422));
#116507=CARTESIAN_POINT('Ctrl Pts',(7.045131315,2.323743665,2.583639413));
#116508=CARTESIAN_POINT('Ctrl Pts',(7.121376478,2.285714286,2.352869961));
#116509=CARTESIAN_POINT('Ctrl Pts',(7.174311796,2.259311335,2.192651873));
#116510=CARTESIAN_POINT('Ctrl Pts',(7.219987966,2.232664075,2.030215204));
#116511=CARTESIAN_POINT('Ctrl Pts',(7.22110414954922,2.23201289883432,2.0262457569617));
#116512=CARTESIAN_POINT('Ctrl Pts',(7.22222033309843,2.23136172266864,2.02227630992341));
#116513=CARTESIAN_POINT('',(7.12995887474965,2.23266407357604,1.88140556352814));
#116514=CARTESIAN_POINT('Ctrl Pts',(7.03806101166501,2.23138000478158,1.74018916767838));
#116515=CARTESIAN_POINT('Ctrl Pts',(7.0389953998325,2.23202203989079,1.73639253683919));
#116516=CARTESIAN_POINT('Ctrl Pts',(7.039929788,2.232664075,1.732595906));
#116517=CARTESIAN_POINT('Ctrl Pts',(7.133744856,2.297126115,1.351404028));
#116518=CARTESIAN_POINT('Ctrl Pts',(7.185851215,2.362252267,0.962310925));
#116519=CARTESIAN_POINT('Ctrl Pts',(7.3358745212548,2.23138000478158,1.56045200257577));
#116520=CARTESIAN_POINT('Ctrl Pts',(7.3367118041274,2.23202203989079,1.55649486578788));
#116521=CARTESIAN_POINT('Ctrl Pts',(7.337549087,2.232664075,1.552537729));
#116522=CARTESIAN_POINT('Ctrl Pts',(7.421614524,2.297126115,1.155230625));
#116523=CARTESIAN_POINT('Ctrl Pts',(7.462288171,2.362252267,0.751169259));
#116524=CARTESIAN_POINT('',(7.33754908621416,2.23266407419427,1.5525377224994));
#116525=CARTESIAN_POINT('',(7.43322462809307,2.32233405369076,0.998584814253996));
#116526=CARTESIAN_POINT('Origin',(-0.189259838612895,2.41067412263089,-0.0111304280783903));
#116527=CARTESIAN_POINT('Ctrl Pts',(7.18522749154915,2.3614745818536,0.966957027476653));
#116528=CARTESIAN_POINT('Ctrl Pts',(7.22649349810488,2.35461430893834,0.972257275442808));
#116529=CARTESIAN_POINT('Ctrl Pts',(7.26781657349002,2.34792816205629,0.977545023481249));
#116530=CARTESIAN_POINT('Ctrl Pts',(7.35046881019824,2.33489257229042,0.988084906829652));
#116531=CARTESIAN_POINT('Ctrl Pts',(7.39184645224129,2.32853548990041,0.99334322253187));
#116532=CARTESIAN_POINT('Ctrl Pts',(7.43322462785181,2.32233405371819,0.998584816191025));
#116533=CARTESIAN_POINT('',(7.18873944076293,2.23266407264717,1.64256680321968));
#116534=CARTESIAN_POINT('Origin',(-9.44556932669371E-13,2.32340998499944,
-1.57263525119022E-13));
#116535=CARTESIAN_POINT('',(7.43350303971341,2.14301213123584,0.996510189563523));
#116536=CARTESIAN_POINT('Origin',(-0.187307222202631,2.0179410143598,-0.00493008707019446));
#116537=CARTESIAN_POINT('',(7.48762491278476,2.23266407449122,0.430665910956783));
#116538=CARTESIAN_POINT('Origin',(-0.182398313896053,2.41052395036109,0.017836156865229));
#116539=CARTESIAN_POINT('Ctrl Pts',(7.43322462815202,2.32233405322792,0.998584812966175));
#116540=CARTESIAN_POINT('Ctrl Pts',(7.4435926514556,2.31006874162622,0.921407745357249));
#116541=CARTESIAN_POINT('Ctrl Pts',(7.45274276603645,2.29785936480243,0.844185793800922));
#116542=CARTESIAN_POINT('Ctrl Pts',(7.4606801448002,2.28571428603199,0.766975732997686));
#116543=CARTESIAN_POINT('Ctrl Pts',(7.47215476891025,2.2681568256412,0.655357473043764));
#116544=CARTESIAN_POINT('Ctrl Pts',(7.48115234803254,2.25046493734972,0.543198978937179));
#116545=CARTESIAN_POINT('Ctrl Pts',(7.48762491508439,2.23266407446841,0.430665906525027));
#116546=CARTESIAN_POINT('Ctrl Pts',(7.184590752,2.36225522,0.971676760000001));
#116547=CARTESIAN_POINT('Ctrl Pts',(7.21607810799999,2.323743665,0.738858839));
#116548=CARTESIAN_POINT('Ctrl Pts',(7.23242622,2.285714286,0.5044908));
#116549=CARTESIAN_POINT('Ctrl Pts',(7.243776351,2.259311335,0.341774293));
#116550=CARTESIAN_POINT('Ctrl Pts',(7.247797047,2.232664075,0.178711971));
#116551=CARTESIAN_POINT('Ctrl Pts',(7.24789530030652,2.23201289883432,0.174727234948065));
#116552=CARTESIAN_POINT('Ctrl Pts',(7.24799355361303,2.23136172266864,0.170742498896129));
#116553=CARTESIAN_POINT('Ctrl Pts',(7.39537190800001,2.36225522,1.248388701));
#116554=CARTESIAN_POINT('Ctrl Pts',(7.435826162,2.323743665,1.008740379));
#116555=CARTESIAN_POINT('Ctrl Pts',(7.460680145,2.285714286,0.766975733));
#116556=CARTESIAN_POINT('Ctrl Pts',(7.477935712,2.259311335,0.599123926));
#116557=CARTESIAN_POINT('Ctrl Pts',(7.487624915,2.232664075,0.43066591));
#116558=CARTESIAN_POINT('Ctrl Pts',(7.48786168898945,2.23201289883432,0.42654931996645));
#116559=CARTESIAN_POINT('Ctrl Pts',(7.4880984629789,2.23136172266864,0.4224327299329));
#116560=CARTESIAN_POINT('',(7.36771098063556,2.23266407357604,0.304688949312516));
#116561=CARTESIAN_POINT('Ctrl Pts',(7.24760428844329,2.23138000478158,0.186529438107579));
#116562=CARTESIAN_POINT('Ctrl Pts',(7.24770066772165,2.23202203989079,0.182620704553789));
#116563=CARTESIAN_POINT('Ctrl Pts',(7.247797047,2.232664075,0.178711971));
#116564=CARTESIAN_POINT('Ctrl Pts',(7.257473784,2.297126115,-0.213735319));
#116565=CARTESIAN_POINT('Ctrl Pts',(7.22471841,2.362252267,-0.604932968));
#116566=CARTESIAN_POINT('Ctrl Pts',(7.49981690556088,2.23138000478158,-0.0530266736009007));
#116567=CARTESIAN_POINT('Ctrl Pts',(7.49978394578045,2.23202203989079,-0.0570712858004503));
#116568=CARTESIAN_POINT('Ctrl Pts',(7.49975098600001,2.232664075,-0.061115898));
#116569=CARTESIAN_POINT('Ctrl Pts',(7.496441736,2.297126115,-0.467205767));
#116570=CARTESIAN_POINT('Ctrl Pts',(7.449303207,2.362252267,-0.870564034));
#116571=CARTESIAN_POINT('',(7.49975098383396,2.23266407419428,-0.0611159041764366));
#116572=CARTESIAN_POINT('',(7.47410618406036,2.32233405362781,-0.622685114197929));
#116573=CARTESIAN_POINT('Origin',(-0.187228056671962,2.41067415935372,0.0298150878062447));
#116574=CARTESIAN_POINT('Ctrl Pts',(7.22510804352427,2.36147458190683,-0.60026140704127));
#116575=CARTESIAN_POINT('Ctrl Pts',(7.26654867589849,2.35461430806005,-0.603956047999222));
#116576=CARTESIAN_POINT('Ctrl Pts',(7.30804235665987,2.34792816019782,-0.607675164886424));
#116577=CARTESIAN_POINT('Ctrl Pts',(7.39102797852344,2.33489257272257,-0.615149484637324));
#116578=CARTESIAN_POINT('Ctrl Pts',(7.43256861342513,2.32853549078482,-0.618909075139608));
#116579=CARTESIAN_POINT('Ctrl Pts',(7.47410618422981,2.32233405365464,-0.622685112329022));
#116580=CARTESIAN_POINT('',(7.3737740166168,2.23266407264717,0.0587980218521181));
#116581=CARTESIAN_POINT('Origin',(-1.03779831950312E-12,2.32340998499944,
3.63919235458338E-14));
#116582=CARTESIAN_POINT('',(7.47393210382702,2.14301213124514,-0.624771085990036));
#116583=CARTESIAN_POINT('Origin',(-0.18398813477026,2.01794104937221,0.0354506976473318));
#116584=CARTESIAN_POINT('',(7.40514884403309,2.23266407449122,-1.18902084260639));
#116585=CARTESIAN_POINT('Origin',(-0.17430000017074,2.41052401608581,0.0566294523303079));
#116586=CARTESIAN_POINT('Ctrl Pts',(7.47410618389678,2.32233405317591,-0.622685115421782));
#116587=CARTESIAN_POINT('Ctrl Pts',(7.46764102034714,2.31006874158847,-0.700286644744279));
#116588=CARTESIAN_POINT('Ctrl Pts',(7.45997677338716,2.29785936478234,-0.777670194344572));
#116589=CARTESIAN_POINT('Ctrl Pts',(7.45113069970861,2.28571428608203,-0.854781428739722));
#116590=CARTESIAN_POINT('Ctrl Pts',(7.43834242647713,2.26815682576385,-0.966256820570834));
#116591=CARTESIAN_POINT('Ctrl Pts',(7.42301888672561,2.25046493734972,-1.0777273253983));
#116592=CARTESIAN_POINT('Ctrl Pts',(7.40514884533586,2.23266407446841,-1.18902084741156));
#116593=CARTESIAN_POINT('Ctrl Pts',(7.225500794,2.36225522,-0.595515139));
#116594=CARTESIAN_POINT('Ctrl Pts',(7.206203021,2.323743665,-0.829658758));
#116595=CARTESIAN_POINT('Ctrl Pts',(7.171786724,2.285714286,-1.062061763));
#116596=CARTESIAN_POINT('Ctrl Pts',(7.147892255,2.259311335,-1.22341399));
#116597=CARTESIAN_POINT('Ctrl Pts',(7.11676537100001,2.232664075,-1.383528337));
#116598=CARTESIAN_POINT('Ctrl Pts',(7.11600472675467,2.23201289883432,-1.38744103371067));
#116599=CARTESIAN_POINT('Ctrl Pts',(7.11524408250935,2.23136172266864,-1.39135373042133));
#116600=CARTESIAN_POINT('Ctrl Pts',(7.490838891,2.36225522,-0.370584287));
#116601=CARTESIAN_POINT('Ctrl Pts',(7.47883004200001,2.323743665,-0.613326232999999));
#116602=CARTESIAN_POINT('Ctrl Pts',(7.4511307,2.285714286,-0.854781429));
#116603=CARTESIAN_POINT('Ctrl Pts',(7.43189966400001,2.259311335,-1.022418391));
#116604=CARTESIAN_POINT('Ctrl Pts',(7.405148846,2.232664075,-1.189020844));
#116605=CARTESIAN_POINT('Ctrl Pts',(7.40449513919885,2.23201289883432,-1.19309208984433));
#116606=CARTESIAN_POINT('Ctrl Pts',(7.40384143239769,2.23136172266864,-1.19716333568867));
#116607=CARTESIAN_POINT('',(7.26095711003851,2.23266407357604,-1.28627458181517));
#116608=CARTESIAN_POINT('Ctrl Pts',(7.11825764338815,2.23138000478158,-1.37585220051464));
#116609=CARTESIAN_POINT('Ctrl Pts',(7.11751150719407,2.23202203989079,-1.37969026875732));
#116610=CARTESIAN_POINT('Ctrl Pts',(7.116765371,2.232664075,-1.383528337));
#116611=CARTESIAN_POINT('Ctrl Pts',(7.041851304,2.297126115,-1.768880641));
#116612=CARTESIAN_POINT('Ctrl Pts',(6.925765802,2.362252267,-2.143890869));
#116613=CARTESIAN_POINT('Ctrl Pts',(7.3130761865187,2.23138000478158,-1.6640258809411));
#116614=CARTESIAN_POINT('Ctrl Pts',(7.31217452525935,2.23202203989079,-1.66796884697055));
#116615=CARTESIAN_POINT('Ctrl Pts',(7.31127286400001,2.232664075,-1.671911813));
#116616=CARTESIAN_POINT('Ctrl Pts',(7.220743665,2.297126115,-2.067796135));
#116617=CARTESIAN_POINT('Ctrl Pts',(7.087997104,2.362252267,-2.45159072));
#116618=CARTESIAN_POINT('',(7.31127286055811,2.23266407419428,-1.6719118185767));
#116619=CARTESIAN_POINT('',(7.1655068417734,2.32233405367377,-2.21483897860599));
#116620=CARTESIAN_POINT('Origin',(-0.176441304273448,2.41067412198656,0.0693664900664823));
#116621=CARTESIAN_POINT('Ctrl Pts',(6.92715057363297,2.36147458189601,-2.13941228615809));
#116622=CARTESIAN_POINT('Ctrl Pts',(6.96682809443332,2.35461431046545,-2.15192905488734));
#116623=CARTESIAN_POINT('Ctrl Pts',(7.00655215963655,2.34792816513596,-2.16448113041335));
#116624=CARTESIAN_POINT('Ctrl Pts',(7.08599089882905,2.33489257228985,-2.18962017048139));
#116625=CARTESIAN_POINT('Ctrl Pts',(7.12575213894984,2.32853548992283,-2.2022218732359));
#116626=CARTESIAN_POINT('Ctrl Pts',(7.16550684236562,2.32233405370095,-2.21483897675337));
#116627=CARTESIAN_POINT('',(7.21401911446521,2.23266407264717,-1.52772008933053));
#116628=CARTESIAN_POINT('Origin',(-1.05167610731094E-12,2.32340998500022,
2.90457762008867E-13));
#116629=CARTESIAN_POINT('',(7.16488840930825,2.14301213126003,-2.21683875915713));
#116630=CARTESIAN_POINT('Origin',(-0.172065475689857,2.01794104906444,0.0741738152460494));
#116631=CARTESIAN_POINT('',(6.97641624536834,2.23266407449123,-2.75311030322781));
#116632=CARTESIAN_POINT('Origin',(-0.158051170809693,2.41052394479208,0.0927747698878856));
#116633=CARTESIAN_POINT('Ctrl Pts',(7.1655068412746,2.32233405321481,-2.21483897978952));
#116634=CARTESIAN_POINT('Ctrl Pts',(7.14251079480109,2.3100687416172,-2.28923640953947));
#116635=CARTESIAN_POINT('Ctrl Pts',(7.1183905580205,2.29785936479817,-2.36316318834194));
#116636=CARTESIAN_POINT('Ctrl Pts',(7.09317466455831,2.28571428613813,-2.43656996049194));
#116637=CARTESIAN_POINT('Ctrl Pts',(7.05672145941097,2.26815682590133,-2.54269001813063));
#116638=CARTESIAN_POINT('Ctrl Pts',(7.0177933125215,2.25046493734972,-2.64826029694318));
#116639=CARTESIAN_POINT('Ctrl Pts',(6.97641624561796,2.23266407446841,-2.75311030818904));
#116640=CARTESIAN_POINT('Ctrl Pts',(6.92855444900001,2.36225522,-2.134861413));
#116641=CARTESIAN_POINT('Ctrl Pts',(6.859373891,2.323743665,-2.359382433));
#116642=CARTESIAN_POINT('Ctrl Pts',(6.775802451,2.285714286,-2.578953498));
#116643=CARTESIAN_POINT('Ctrl Pts',(6.717780663,2.259311335,-2.731396796));
#116644=CARTESIAN_POINT('Ctrl Pts',(6.65296165500001,2.232664075,-2.881076398));
#116645=CARTESIAN_POINT('Ctrl Pts',(6.65137768002123,2.23201289883432,-2.88473410199325));
#116646=CARTESIAN_POINT('Ctrl Pts',(6.64979370504246,2.23136172266864,-2.88839180598651));
#116647=CARTESIAN_POINT('Ctrl Pts',(7.236042573,2.36225522,-1.972229166));
#116648=CARTESIAN_POINT('Ctrl Pts',(7.172132141,2.323743665,-2.206714393));
#116649=CARTESIAN_POINT('Ctrl Pts',(7.093174665,2.285714286,-2.436569961));
#116650=CARTESIAN_POINT('Ctrl Pts',(7.038356248,2.259311335,-2.596153559));
#116651=CARTESIAN_POINT('Ctrl Pts',(6.976416247,2.232664075,-2.753110305));
#116652=CARTESIAN_POINT('Ctrl Pts',(6.97490262599906,2.23201289883432,-2.75694583976186));
#116653=CARTESIAN_POINT('Ctrl Pts',(6.97338900499812,2.23136172266864,-2.76078137452372));
#116654=CARTESIAN_POINT('',(6.81468895436952,2.23266407357604,-2.81709334334895));
#116655=CARTESIAN_POINT('Ctrl Pts',(6.65606918130503,2.23138000478158,-2.87390051977844));
#116656=CARTESIAN_POINT('Ctrl Pts',(6.65451541815251,2.23202203989079,-2.87748845888922));
#116657=CARTESIAN_POINT('Ctrl Pts',(6.652961655,2.232664075,-2.881076398));
#116658=CARTESIAN_POINT('Ctrl Pts',(6.496959684,2.297126115,-3.241315069));
#116659=CARTESIAN_POINT('Ctrl Pts',(6.302972082,2.362252267,-3.582602815));
#116660=CARTESIAN_POINT('Ctrl Pts',(6.78438415313431,2.23138000478158,-3.1972170876818));
#116661=CARTESIAN_POINT('Ctrl Pts',(6.78265595106716,2.23202203989079,-3.2008740388409));
#116662=CARTESIAN_POINT('Ctrl Pts',(6.780927749,2.232664075,-3.20453099));
#116663=CARTESIAN_POINT('Ctrl Pts',(6.607411645,2.297126115,-3.571698655));
#116664=CARTESIAN_POINT('Ctrl Pts',(6.395264134,2.362252267,-3.917983749));
#116665=CARTESIAN_POINT('',(6.78092774444002,2.23266407419428,-3.20453099470365));
#116666=CARTESIAN_POINT('',(6.52185636336245,2.32233405368499,-3.70342943434098));
#116667=CARTESIAN_POINT('Origin',(-0.157404492658647,2.41067413902249,0.105674428825331));
#116668=CARTESIAN_POINT('Ctrl Pts',(6.30528724150653,2.36147458185392,-3.57852662370195));
#116669=CARTESIAN_POINT('Ctrl Pts',(6.34134640862966,2.3546143066515,-3.5992802631257));
#116670=CARTESIAN_POINT('Ctrl Pts',(6.37744344503381,2.34792815738207,-3.62007839131622));
#116671=CARTESIAN_POINT('Ctrl Pts',(6.44962074858874,2.33489257385853,-3.66170664582743));
#116672=CARTESIAN_POINT('Ctrl Pts',(6.48574338974461,2.32853549307499,-3.68256121353421));
#116673=CARTESIAN_POINT('Ctrl Pts',(6.52185636417603,2.32233405372278,-3.70342943278937));
#116674=CARTESIAN_POINT('',(6.71694469595552,2.23266407264717,-3.0428037073431));
#116675=CARTESIAN_POINT('Origin',(-1.48535697630514E-12,2.32340998499956,
9.15933995315754E-13));
#116676=CARTESIAN_POINT('',(6.52082249544694,2.14301213121499,-3.70524951652264));
#116677=CARTESIAN_POINT('Origin',(-0.152097410899558,2.01794104260894,0.109428621450758));
#116678=CARTESIAN_POINT('',(6.22147417679742,2.23266407449122,-4.18846738491079));
#116679=CARTESIAN_POINT('Origin',(-0.134411997813026,2.41052396482033,0.124581958717048));
#116680=CARTESIAN_POINT('Ctrl Pts',(6.52185636285941,2.32233405324098,-3.70342943540267));
#116681=CARTESIAN_POINT('Ctrl Pts',(6.483404702948,2.3100687416266,-3.77114402426926));
#116682=CARTESIAN_POINT('Ctrl Pts',(6.44395631178173,2.29785936479879,-3.83815729788785));
#116683=CARTESIAN_POINT('Ctrl Pts',(6.40354966577465,2.28571428603063,-3.90442718890095));
#116684=CARTESIAN_POINT('Ctrl Pts',(6.34513604105734,2.26815682563787,-4.00022985843361));
#116685=CARTESIAN_POINT('Ctrl Pts',(6.28442352312462,2.25046493734972,-4.0949635606698));
#116686=CARTESIAN_POINT('Ctrl Pts',(6.22147417596399,2.23266407446841,-4.18846738981751));
#116687=CARTESIAN_POINT('Ctrl Pts',(6.307636598,2.36225522,-3.574383939));
#116688=CARTESIAN_POINT('Ctrl Pts',(6.191808061,2.323743665,-3.778784008));
#116689=CARTESIAN_POINT('Ctrl Pts',(6.062989186,2.285714286,-3.975256234));
#116690=CARTESIAN_POINT('Ctrl Pts',(5.973553112,2.259311335,-4.111662523));
#116691=CARTESIAN_POINT('Ctrl Pts',(5.878072847,2.232664075,-4.243908529));
#116692=CARTESIAN_POINT('Ctrl Pts',(5.87573960625175,2.23201289883432,-4.24714021012271));
#116693=CARTESIAN_POINT('Ctrl Pts',(5.87340636550352,2.23136172266864,-4.25037189124542));
#116694=CARTESIAN_POINT('Ctrl Pts',(6.642896946,2.36225522,-3.481654802));
#116695=CARTESIAN_POINT('Ctrl Pts',(6.530073313,2.323743665,-3.696919041));
#116696=CARTESIAN_POINT('Ctrl Pts',(6.403549666,2.285714286,-3.904427189));
#116697=CARTESIAN_POINT('Ctrl Pts',(6.315707117,2.259311335,-4.048495473));
#116698=CARTESIAN_POINT('Ctrl Pts',(6.221474178,2.232664075,-4.188467387));
#116699=CARTESIAN_POINT('Ctrl Pts',(6.21917141802021,2.23201289883432,-4.19188786528789));
#116700=CARTESIAN_POINT('Ctrl Pts',(6.21686865804042,2.23136172266864,-4.19530834357579));
#116701=CARTESIAN_POINT('',(6.04977351754298,2.23266407357604,-4.21618795076387));
#116702=CARTESIAN_POINT('Ctrl Pts',(5.88265032276119,2.23138000478158,-4.23756844513487));
#116703=CARTESIAN_POINT('Ctrl Pts',(5.8803615848806,2.23202203989079,-4.24073848706743));
#116704=CARTESIAN_POINT('Ctrl Pts',(5.878072847,2.232664075,-4.243908529));
#116705=CARTESIAN_POINT('Ctrl Pts',(5.64827745,2.297126115,-4.562189207));
#116706=CARTESIAN_POINT('Ctrl Pts',(5.385458394,2.362252267,-4.853796235));
#116707=CARTESIAN_POINT('Ctrl Pts',(5.93846185711766,2.23138000478158,-4.58090997634739));
#116708=CARTESIAN_POINT('Ctrl Pts',(5.93598792305883,2.23202203989079,-4.5841099176737));
#116709=CARTESIAN_POINT('Ctrl Pts',(5.933513989,2.232664075,-4.587309859));
#116710=CARTESIAN_POINT('Ctrl Pts',(5.685124401,2.297126115,-4.908592516));
#116711=CARTESIAN_POINT('Ctrl Pts',(5.403495721,2.362252267,-5.201176212));
#116712=CARTESIAN_POINT('',(5.93351398353206,2.23266407419428,-4.58730986262407));
#116713=CARTESIAN_POINT('',(5.57325113022134,2.3223340536832,-5.01885164571133));
#116714=CARTESIAN_POINT('Origin',(-0.131007258613514,2.41067415088804,0.137040855787069));
#116715=CARTESIAN_POINT('Ctrl Pts',(5.3885956869058,2.36147458187527,-4.85031303370965));
#116716=CARTESIAN_POINT('Ctrl Pts',(5.41935036612432,2.35461431232922,-4.87833309640803));
#116717=CARTESIAN_POINT('Ctrl Pts',(5.45013246168415,2.34792816896932,-4.90640474497083));
#116718=CARTESIAN_POINT('Ctrl Pts',(5.51167351162437,2.3348925735735,-4.9625757919582));
#116719=CARTESIAN_POINT('Ctrl Pts',(5.54246851123432,2.32853549252457,-4.99070809286661));
#116720=CARTESIAN_POINT('Ctrl Pts',(5.57325113138551,2.32233405371842,-5.01885164435842));
#116721=CARTESIAN_POINT('',(5.90579340922846,2.23266407264717,-4.41560920573176));
#116722=CARTESIAN_POINT('Origin',(-4.95697233260373E-13,2.32340998500067,
4.70110061989715E-13));
#116723=CARTESIAN_POINT('',(5.57185016995924,2.14301213124523,-5.02040692436461));
#116724=CARTESIAN_POINT('Origin',(-0.125017759930015,2.0179410069928,0.139566873922891));
#116725=CARTESIAN_POINT('',(5.1756228902727,2.23266407449123,-5.42797638770235));
#116726=CARTESIAN_POINT('Origin',(-0.104488342135182,2.41052403993646,0.150564189044248));
#116727=CARTESIAN_POINT('Ctrl Pts',(5.57325112946139,2.32233405323673,-5.01885164662856));
#116728=CARTESIAN_POINT('Ctrl Pts',(5.5211418130037,2.31006874162515,-5.0767171358636));
#116729=CARTESIAN_POINT('Ctrl Pts',(5.46820983040542,2.29785936479876,-5.13368343845998));
#116730=CARTESIAN_POINT('Ctrl Pts',(5.41450180158365,2.28571428604938,-5.18971774176479));
#116731=CARTESIAN_POINT('Ctrl Pts',(5.33685911222919,2.26815682568383,-5.27072339526756));
#116732=CARTESIAN_POINT('Ctrl Pts',(5.25720107397725,2.25046493734972,-5.35019087963778));
#116733=CARTESIAN_POINT('Ctrl Pts',(5.17562288840667,2.23266407446841,-5.42797639231399));
#116734=CARTESIAN_POINT('Ctrl Pts',(5.391780671,2.36225522,-4.846772245));
#116735=CARTESIAN_POINT('Ctrl Pts',(5.234720168,2.323743665,-5.021493842));
#116736=CARTESIAN_POINT('Ctrl Pts',(5.066677286,2.285714286,-5.185680407));
#116737=CARTESIAN_POINT('Ctrl Pts',(4.950008857,2.259311335,-5.29967148));
#116738=CARTESIAN_POINT('Ctrl Pts',(4.828331886,2.232664075,-5.408300213));
#116739=CARTESIAN_POINT('Ctrl Pts',(4.82535847922468,2.23201289883432,-5.41095476141654));
#116740=CARTESIAN_POINT('Ctrl Pts',(4.82238507244937,2.23136172266864,-5.41360930983306));
#116741=CARTESIAN_POINT('Ctrl Pts',(5.739136842,2.36225522,-4.828282128));
#116742=CARTESIAN_POINT('Ctrl Pts',(5.58267551400001,2.323743665,-5.014259863));
#116743=CARTESIAN_POINT('Ctrl Pts',(5.414501802,2.285714286,-5.189717742));
#116744=CARTESIAN_POINT('Ctrl Pts',(5.29774254,2.259311335,-5.311534238));
#116745=CARTESIAN_POINT('Ctrl Pts',(5.175622891,2.232664075,-5.42797639000001));
#116746=CARTESIAN_POINT('Ctrl Pts',(5.17263866655102,2.23201289883432,-5.43082187407841));
#116747=CARTESIAN_POINT('Ctrl Pts',(5.16965444210204,2.23136172266864,-5.43366735815682));
#116748=CARTESIAN_POINT('',(5.00197739498063,2.23266407357604,-5.41813829551714));
#116749=CARTESIAN_POINT('Ctrl Pts',(4.83416527354552,2.23138000478158,-5.40309237873128));
#116750=CARTESIAN_POINT('Ctrl Pts',(4.83124857977277,2.23202203989079,-5.40569629586564));
#116751=CARTESIAN_POINT('Ctrl Pts',(4.828331886,2.232664075,-5.40830021300001));
#116752=CARTESIAN_POINT('Ctrl Pts',(4.53548804,2.297126115,-5.669740449));
#116753=CARTESIAN_POINT('Ctrl Pts',(4.216126656,2.362252267,-5.898031538));
#116754=CARTESIAN_POINT('Ctrl Pts',(4.81486368430831,2.23138000478158,-5.75040460645348));
#116755=CARTESIAN_POINT('Ctrl Pts',(4.81175969665416,2.23202203989079,-5.75299791222674));
#116756=CARTESIAN_POINT('Ctrl Pts',(4.808655709,2.232664075,-5.755591218));
#116757=CARTESIAN_POINT('Ctrl Pts',(4.497007057,2.297126115,-6.015966045));
#116758=CARTESIAN_POINT('Ctrl Pts',(4.159065854,2.362252267,-6.241167457));
#116759=CARTESIAN_POINT('',(4.80865570287358,2.23266407419429,-5.75559122037632));
#116760=CARTESIAN_POINT('',(4.36404686809461,2.3223340536569,-6.09959793199742));
#116761=CARTESIAN_POINT('Origin',(-0.0984849361830059,2.41067415219992,
0.161999976496024));
#116762=CARTESIAN_POINT('Ctrl Pts',(4.21993938588018,2.36147458191207,-5.89530419738615));
#116763=CARTESIAN_POINT('Ctrl Pts',(4.24395154837877,2.35461431359499,-5.92928050741024));
#116764=CARTESIAN_POINT('Ctrl Pts',(4.26797939614879,2.34792817149799,-5.96331309003516));
#116765=CARTESIAN_POINT('Ctrl Pts',(4.31600654425107,2.33489257380625,-6.03140040752346));
#116766=CARTESIAN_POINT('Ctrl Pts',(4.34003395981166,2.32853549297441,-6.06549500410895));
#116767=CARTESIAN_POINT('Ctrl Pts',(4.36404686948249,2.3223340536942,-6.09959793093269));
#116768=CARTESIAN_POINT('',(4.81849378641155,2.23266407264717,-5.58194572507186));
#116769=CARTESIAN_POINT('Origin',(2.45246531416221E-13,2.32340998499944,
-3.56919355182228E-13));
#116770=CARTESIAN_POINT('',(4.36234432276977,2.14301213124795,-6.10081568386786));
#116771=CARTESIAN_POINT('Origin',(-0.0920919309245477,2.01794106337157,
0.163178683584191));
#116772=CARTESIAN_POINT('',(3.88776522976379,2.23266407449123,-6.4136792476037));
#116773=CARTESIAN_POINT('Origin',(-0.0696785071243489,2.41052398726883,
0.169505791714497));
#116774=CARTESIAN_POINT('Ctrl Pts',(4.36404686719633,2.32233405321387,-6.09959793274587));
#116775=CARTESIAN_POINT('Ctrl Pts',(4.30071646795032,2.31006874160842,-6.14490859616822));
#116776=CARTESIAN_POINT('Ctrl Pts',(4.23677593453902,2.29785936478988,-6.18916424668093));
#116777=CARTESIAN_POINT('Ctrl Pts',(4.17227785102704,2.28571428609381,-6.23234286055701));
#116778=CARTESIAN_POINT('Ctrl Pts',(4.07903658490318,2.26815682579272,-6.29476376356859));
#116779=CARTESIAN_POINT('Ctrl Pts',(3.98415774636946,2.25046493734972,-6.35524921920965));
#116780=CARTESIAN_POINT('Ctrl Pts',(3.88776522696987,2.23266407446841,-6.41367925170241));
#116781=CARTESIAN_POINT('Ctrl Pts',(4.223811072,2.36225522,-5.89253086800001));
#116782=CARTESIAN_POINT('Ctrl Pts',(4.032862577,2.323743665,-6.029404205));
#116783=CARTESIAN_POINT('Ctrl Pts',(3.833453187,2.285714286,-6.153627927));
#116784=CARTESIAN_POINT('Ctrl Pts',(3.69500769,2.259311335,-6.239873689));
#116785=CARTESIAN_POINT('Ctrl Pts',(3.552823492,2.232664075,-6.319805791));
#116786=CARTESIAN_POINT('Ctrl Pts',(3.549348952371,2.23201289883432,-6.32175908299683));
#116787=CARTESIAN_POINT('Ctrl Pts',(3.54587441274199,2.23136172266864,-6.32371237499365));
#116788=CARTESIAN_POINT('Ctrl Pts',(4.567021077,2.36225522,-5.949144349));
#116789=CARTESIAN_POINT('Ctrl Pts',(4.374238013,2.323743665,-6.097139466));
#116790=CARTESIAN_POINT('Ctrl Pts',(4.172277851,2.285714286,-6.232342861));
#116791=CARTESIAN_POINT('Ctrl Pts',(4.032061411,2.259311335,-6.326211565));
#116792=CARTESIAN_POINT('Ctrl Pts',(3.88776523,2.232664075,-6.41367925));
#116793=CARTESIAN_POINT('Ctrl Pts',(3.88423908007441,2.23201289883432,-6.41581668821089));
#116794=CARTESIAN_POINT('Ctrl Pts',(3.88071293014881,2.23136172266864,-6.41795412642177));
#116795=CARTESIAN_POINT('',(3.72029436861526,2.23266407357604,-6.36674251605016));
#116796=CARTESIAN_POINT('Ctrl Pts',(3.55964002860692,2.23138000478158,-6.31597371891253));
#116797=CARTESIAN_POINT('Ctrl Pts',(3.55623176030346,2.23202203989079,-6.31788975495627));
#116798=CARTESIAN_POINT('Ctrl Pts',(3.552823492,2.232664075,-6.319805791));
#116799=CARTESIAN_POINT('Ctrl Pts',(3.21062425,2.297126115,-6.512180928));
#116800=CARTESIAN_POINT('Ctrl Pts',(2.849653521,2.362252267,-6.666481441));
#116801=CARTESIAN_POINT('Ctrl Pts',(3.46612783746513,2.23138000478158,-6.65101670874053));
#116802=CARTESIAN_POINT('Ctrl Pts',(3.46253893523256,2.23202203989079,-6.65288211887026));
#116803=CARTESIAN_POINT('Ctrl Pts',(3.458950033,2.232664075,-6.654747529));
#116804=CARTESIAN_POINT('Ctrl Pts',(3.098614662,2.297126115,-6.842039689));
#116805=CARTESIAN_POINT('Ctrl Pts',(2.72016269,2.362252267,-6.989328647));
#116806=CARTESIAN_POINT('',(3.45895002652983,2.23266407419428,-6.65474752997787));
#116807=CARTESIAN_POINT('',(2.95078462496021,2.3223340536514,-6.89513379816407));
#116808=CARTESIAN_POINT('Origin',(-0.0613571587393019,2.41067416161038,
0.179383781189104));
#116809=CARTESIAN_POINT('Ctrl Pts',(2.853963409154,2.36147458188161,-6.66463748826855));
#116810=CARTESIAN_POINT('Ctrl Pts',(2.87011029019925,2.35461430857168,-6.7029813842314));
#116811=CARTESIAN_POINT('Ctrl Pts',(2.88626039459709,2.34792816125834,-6.74138361339339));
#116812=CARTESIAN_POINT('Ctrl Pts',(2.91852790927514,2.33489257365021,-6.81820344517192));
#116813=CARTESIAN_POINT('Ctrl Pts',(2.9346642473191,2.32853549264739,-6.85666611430339));
#116814=CARTESIAN_POINT('Ctrl Pts',(2.95078462656646,2.3223340536871,-6.89513379742501));
#116815=CARTESIAN_POINT('',(3.50588674961313,2.23266407264717,-6.48727666696439));
#116816=CARTESIAN_POINT('Origin',(2.83193607453214E-13,2.32340998499989,
-6.30138302648575E-13));
#116817=CARTESIAN_POINT('',(2.94886010308049,2.14301213124642,-6.89595708322331));
#116818=CARTESIAN_POINT('Origin',(-0.0548604496304522,2.0179410552179,0.1791610850029));
#116819=CARTESIAN_POINT('',(2.4181199873082,2.23266407449122,-7.09948559360941));
#116820=CARTESIAN_POINT('Origin',(-0.0316109121132391,2.41052400205891,
0.180522180259263));
#116821=CARTESIAN_POINT('Ctrl Pts',(2.95078462390421,2.32233405320707,-6.89513379868537));
#116822=CARTESIAN_POINT('Ctrl Pts',(2.87919440088891,2.31006874160469,-6.92577096014036));
#116823=CARTESIAN_POINT('Ctrl Pts',(2.80723510491418,2.29785936478813,-6.95524661337074));
#116824=CARTESIAN_POINT('Ctrl Pts',(2.73496282489214,2.28571428602063,-6.98355055384198));
#116825=CARTESIAN_POINT('Ctrl Pts',(2.63048283853519,2.26815682561336,-7.02446797583331));
#116826=CARTESIAN_POINT('Ctrl Pts',(2.52481962986214,2.25046493734972,-7.06314316892451));
#116827=CARTESIAN_POINT('Ctrl Pts',(2.41811998367477,2.23266407446841,-7.09948559701123));
#116828=CARTESIAN_POINT('Ctrl Pts',(2.858340762,2.36225522,-6.662761296));
#116829=CARTESIAN_POINT('Ctrl Pts',(2.642432815,2.323743665,-6.755386329));
#116830=CARTESIAN_POINT('Ctrl Pts',(2.420981077,2.285714286,-6.833838645));
#116831=CARTESIAN_POINT('Ctrl Pts',(2.26723207,2.259311335,-6.88830634));
#116832=CARTESIAN_POINT('Ctrl Pts',(2.11118902,2.232664075,-6.935804274));
#116833=CARTESIAN_POINT('Ctrl Pts',(2.10737581312693,2.23201289883432,-6.93696497579598));
#116834=CARTESIAN_POINT('Ctrl Pts',(2.10356260625386,2.23136172266864,-6.93812567759196));
#116835=CARTESIAN_POINT('Ctrl Pts',(3.181356483,2.36225522,-6.791831191));
#116836=CARTESIAN_POINT('Ctrl Pts',(2.961266004,2.323743665,-6.894923605));
#116837=CARTESIAN_POINT('Ctrl Pts',(2.734962825,2.285714286,-6.983550554));
#116838=CARTESIAN_POINT('Ctrl Pts',(2.577845571,2.259311335,-7.04508227100001));
#116839=CARTESIAN_POINT('Ctrl Pts',(2.418119987,2.232664075,-7.099485596));
#116840=CARTESIAN_POINT('Ctrl Pts',(2.41421679044806,2.23201289883432,-7.10081504407736));
#116841=CARTESIAN_POINT('Ctrl Pts',(2.41031359389613,2.23136172266864,-7.10214449215472));
#116842=CARTESIAN_POINT('',(2.2646545118938,2.23266407357604,-7.01764493229125));
#116843=CARTESIAN_POINT('Ctrl Pts',(2.11866997199718,2.23138000478158,-6.93352714751366));
#116844=CARTESIAN_POINT('Ctrl Pts',(2.11492949599859,2.23202203989079,-6.93466571075683));
#116845=CARTESIAN_POINT('Ctrl Pts',(2.11118902,2.232664075,-6.93580427400001));
#116846=CARTESIAN_POINT('Ctrl Pts',(1.735635238,2.297126115,-7.050119065));
#116847=CARTESIAN_POINT('Ctrl Pts',(1.349933756,2.362252267,-7.123214082));
#116848=CARTESIAN_POINT('Ctrl Pts',(1.95531970545204,2.23138000478158,-7.24063466103159));
#116849=CARTESIAN_POINT('Ctrl Pts',(1.95141370172602,2.23202203989079,-7.2416849510158));
#116850=CARTESIAN_POINT('Ctrl Pts',(1.947507698,2.232664075,-7.242735241));
#116851=CARTESIAN_POINT('Ctrl Pts',(1.55533449,2.297126115,-7.348187161));
#116852=CARTESIAN_POINT('Ctrl Pts',(1.154067742,2.362252267,-7.410676599));
#116853=CARTESIAN_POINT('',(1.94750769146921,2.23266407419429,-7.24273524056529));
#116854=CARTESIAN_POINT('',(1.39954697245937,2.32233405367958,-7.36826087172726));
#116855=CARTESIAN_POINT('Origin',(-0.0213604939950876,2.41067413430914,
0.188380002614758));
#116856=CARTESIAN_POINT('Ctrl Pts',(1.35453927669525,2.361474581882,-7.12233973837894));
#116857=CARTESIAN_POINT('Ctrl Pts',(1.36206584259948,2.35461431368943,-7.16325824691342));
#116858=CARTESIAN_POINT('Ctrl Pts',(1.36958301587436,2.34792817173249,-7.20423441295965));
#116859=CARTESIAN_POINT('Ctrl Pts',(1.3845821538606,2.33489257278914,-7.28619487280359));
#116860=CARTESIAN_POINT('Ctrl Pts',(1.39207289747177,2.32853549090866,-7.32722714788656));
#116861=CARTESIAN_POINT('Ctrl Pts',(1.39954697431476,2.32233405370702,-7.36826087139055));
#116862=CARTESIAN_POINT('',(2.02934834491728,2.23266407264717,-7.08926976153127));
#116863=CARTESIAN_POINT('Origin',(8.84166871661929E-14,2.32340998499967,
-5.66387214906428E-13));
#116864=CARTESIAN_POINT('',(1.3974904628466,2.14301213120873,-7.36865119339408));
#116865=CARTESIAN_POINT('Origin',(-0.0150634728038704,2.01794104739631,
0.186765608589459));
#116866=CARTESIAN_POINT('',(0.83540614281881,2.23266407449122,-7.45332788373253));
#116867=CARTESIAN_POINT('Origin',(0.00793508467594406,2.41052395448723,
0.183096902090448));
#116868=CARTESIAN_POINT('Ctrl Pts',(1.39954697122311,2.32233405322557,-7.36826087189618));
#116869=CARTESIAN_POINT('Ctrl Pts',(1.32304440380988,2.31006874162192,-7.38279197187679));
#116870=CARTESIAN_POINT('Ctrl Pts',(1.24643108191867,2.29785936479934,-7.3961093793232));
#116871=CARTESIAN_POINT('Ctrl Pts',(1.1697639772822,2.28571428612184,-7.40821518549939));
#116872=CARTESIAN_POINT('Ctrl Pts',(1.05893063938031,2.26815682586141,-7.42571587085398));
#116873=CARTESIAN_POINT('Ctrl Pts',(0.947423753831489,2.25046493734972,
-7.44077239346166));
#116874=CARTESIAN_POINT('Ctrl Pts',(0.835406138535195,2.23266407446841,
-7.45332788627282));
#116875=CARTESIAN_POINT('Ctrl Pts',(1.359217614,2.36225522,-7.121448411));
#116876=CARTESIAN_POINT('Ctrl Pts',(1.128445831,2.323743665,-7.16549409600001));
#116877=CARTESIAN_POINT('Ctrl Pts',(0.895306583,2.285714286,-7.194506663));
#116878=CARTESIAN_POINT('Ctrl Pts',(0.733443198,2.259311335,-7.214649441));
#116879=CARTESIAN_POINT('Ctrl Pts',(0.570837696,2.232664075,-7.227492257));
#116880=CARTESIAN_POINT('Ctrl Pts',(0.566864123208228,2.23201289883432,
-7.22780609548393));
#116881=CARTESIAN_POINT('Ctrl Pts',(0.562890550416455,2.23136172266864,
-7.22811993396787));
#116882=CARTESIAN_POINT('Ctrl Pts',(1.646935195,2.36225522,-7.316939556));
#116883=CARTESIAN_POINT('Ctrl Pts',(1.409828488,2.323743665,-7.370308779));
#116884=CARTESIAN_POINT('Ctrl Pts',(1.169763977,2.285714286,-7.408215186));
#116885=CARTESIAN_POINT('Ctrl Pts',(1.003092537,2.259311335,-7.434532759));
#116886=CARTESIAN_POINT('Ctrl Pts',(0.835406142,2.232664075,-7.453327886));
#116887=CARTESIAN_POINT('Ctrl Pts',(0.831308407984072,2.23201289883432,
-7.45378718045404));
#116888=CARTESIAN_POINT('Ctrl Pts',(0.827210673968144,2.23136172266864,
-7.45424647490808));
#116889=CARTESIAN_POINT('',(0.703121927779861,2.23266407357604,-7.340410070659));
#116890=CARTESIAN_POINT('Ctrl Pts',(0.57863326237553,2.23138000478158,-7.22687655198706));
#116891=CARTESIAN_POINT('Ctrl Pts',(0.574735479187765,2.23202203989079,
-7.22718440449353));
#116892=CARTESIAN_POINT('Ctrl Pts',(0.570837696,2.232664075,-7.227492257));
#116893=CARTESIAN_POINT('Ctrl Pts',(0.179489852,2.297126115,-7.258401471));
#116894=CARTESIAN_POINT('Ctrl Pts',(-0.212907412,2.362252267,-7.246873149));
#116895=CARTESIAN_POINT('Ctrl Pts',(0.35308299665963,2.23138000478158,-7.49168858409584));
#116896=CARTESIAN_POINT('Ctrl Pts',(0.349042531829815,2.23202203989079,
-7.49187464354792));
#116897=CARTESIAN_POINT('Ctrl Pts',(0.345002067,2.232664075,-7.492060703));
#116898=CARTESIAN_POINT('Ctrl Pts',(-0.060671395,2.297126115,-7.510741569));
#116899=CARTESIAN_POINT('Ctrl Pts',(-0.465990131,2.362252267,-7.485509548));
#116900=CARTESIAN_POINT('Ctrl Pts',(-0.208221607850005,2.36147458189157,
-7.24700929787493));
#116901=CARTESIAN_POINT('Ctrl Pts',(-0.209667279061951,2.35461431131095,
-7.2885891579842));
#116902=CARTESIAN_POINT('Ctrl Pts',(-0.211134518176119,2.34792816686656,
-7.33022331072456));
#116903=CARTESIAN_POINT('Ctrl Pts',(-0.214105126604883,2.33489257361319,
-7.41349191549236));
#116904=CARTESIAN_POINT('Ctrl Pts',(-0.21561023850716,2.32853549257574,
-7.4551751613142));
#116905=CARTESIAN_POINT('Ctrl Pts',(-0.217131939497084,2.32233405373809,
-7.49685625574536));
#116906=CARTESIAN_POINT('',(0.457919866879924,2.23266407264717,-7.35977648090965));
#116907=CARTESIAN_POINT('Ctrl Pts',(-0.203461038,2.36225522,-7.24714451400001));
#116908=CARTESIAN_POINT('Ctrl Pts',(-0.438306025,2.323743665,-7.240551323));
#116909=CARTESIAN_POINT('Ctrl Pts',(-0.672231452,2.285714286,-7.218767545));
#116910=CARTESIAN_POINT('Ctrl Pts',(-0.834640663,2.259311335,-7.203643554));
#116911=CARTESIAN_POINT('Ctrl Pts',(-0.996205363999999,2.232664075,-7.181230735));
#116912=CARTESIAN_POINT('Ctrl Pts',(-1.00015350285206,2.23201289883432,
-7.18068303540392));
#116913=CARTESIAN_POINT('Ctrl Pts',(-1.00410164170411,2.23136172266864,
-7.18013533580784));
#116914=CARTESIAN_POINT('Ctrl Pts',(0.035505048,2.36225522,-7.49991595900001));
#116915=CARTESIAN_POINT('Ctrl Pts',(-0.207531042,2.323743665,-7.501066506));
#116916=CARTESIAN_POINT('Ctrl Pts',(-0.450131734,2.285714286,-7.486479909));
#116917=CARTESIAN_POINT('Ctrl Pts',(-0.618563989,2.259311335,-7.476352759));
#116918=CARTESIAN_POINT('Ctrl Pts',(-0.786370366,2.232664075,-7.458660848));
#116919=CARTESIAN_POINT('Ctrl Pts',(-0.790471032002883,2.23201289883432,
-7.45822851271418));
#116920=CARTESIAN_POINT('Ctrl Pts',(-0.794571698005766,2.23136172266864,
-7.45779617742834));
#116921=CARTESIAN_POINT('',(-0.891287856244616,2.23266407357604,-7.31994579256607));
#116922=CARTESIAN_POINT('Ctrl Pts',(-0.988459695241115,2.23138000478158,
-7.18230524117258));
#116923=CARTESIAN_POINT('Ctrl Pts',(-0.992332529620557,2.23202203989079,
-7.18176798808629));
#116924=CARTESIAN_POINT('Ctrl Pts',(-0.996205364,2.232664075,-7.181230735));
#116925=CARTESIAN_POINT('Ctrl Pts',(-1.385048281,2.297126115,-7.12728909));
#116926=CARTESIAN_POINT('Ctrl Pts',(-1.765793266,2.362252267,-7.031676482));
#116927=CARTESIAN_POINT('Ctrl Pts',(-1.26566348041818,2.23138000478158,
-7.39243947503579));
#116928=CARTESIAN_POINT('Ctrl Pts',(-1.26964947870909,2.23202203989079,
-7.3917526040179));
#116929=CARTESIAN_POINT('Ctrl Pts',(-1.273635477,2.232664075,-7.391065733));
#116930=CARTESIAN_POINT('Ctrl Pts',(-1.673840353,2.297126115,-7.322102048));
#116931=CARTESIAN_POINT('Ctrl Pts',(-2.064258824,2.362252267,-7.210328391));
#116932=CARTESIAN_POINT('',(-1.27363548277204,2.23266407419429,-7.39106572986814));
#116933=CARTESIAN_POINT('',(-1.82365800664062,2.32233405365439,-7.27490697348646));
#116934=CARTESIAN_POINT('Origin',(0.0597124100100879,2.41067413317871,0.179937914551258));
#116935=CARTESIAN_POINT('Ctrl Pts',(-1.76124628115219,2.36147458186449,
-7.03281675718452));
#116936=CARTESIAN_POINT('Ctrl Pts',(-1.77159658621436,2.35461431668314,
-7.07311369487819));
#116937=CARTESIAN_POINT('Ctrl Pts',(-1.78197962485504,2.34792817786205,
-7.11345901463161));
#116938=CARTESIAN_POINT('Ctrl Pts',(-1.80278108757618,2.33489257408083,
-7.19414231772472));
#116939=CARTESIAN_POINT('Ctrl Pts',(-1.81321167554102,2.32853549357603,
-7.23452747417755));
#116940=CARTESIAN_POINT('Ctrl Pts',(-1.82365800496382,2.32233405369464,
-7.27490697382443));
#116941=CARTESIAN_POINT('',(-1.13492043497381,2.23266407264717,-7.28614823174549));
#116942=CARTESIAN_POINT('Origin',(2.73544208118093E-13,2.32340998500055,
1.10978934375616E-12));
#116943=CARTESIAN_POINT('',(-1.82568833581608,2.1430121312241,-7.27439771363291));
#116944=CARTESIAN_POINT('Origin',(0.06474963453826,2.01794105213501,0.175829002095066));
#116945=CARTESIAN_POINT('',(-2.37137706833043,2.23266407449123,-7.11523511726562));
#116946=CARTESIAN_POINT('Origin',(0.084081980906319,2.41052391280545,0.162842126679255));
#116947=CARTESIAN_POINT('Ctrl Pts',(-1.82365800778149,2.32233405321442,
-7.27490697333454));
#116948=CARTESIAN_POINT('Ctrl Pts',(-1.89919130811697,2.31006874160714,
-7.25597244811295));
#116949=CARTESIAN_POINT('Ctrl Pts',(-1.97431551001625,2.29785936478844,
-7.23588990102137));
#116950=CARTESIAN_POINT('Ctrl Pts',(-2.04897978584046,2.28571428607925,
-7.2146851515026));
#116951=CARTESIAN_POINT('Ctrl Pts',(-2.15691774703239,2.26815682575704,
-7.18403063233674));
#116952=CARTESIAN_POINT('Ctrl Pts',(-2.26444072465366,2.25046493734972,
-7.15087503667013));
#116953=CARTESIAN_POINT('Ctrl Pts',(-2.37137707325913,2.23266407446841,
-7.11523511779276));
#116954=CARTESIAN_POINT('Ctrl Pts',(-1.756626078,2.36225522,-7.033972194));
#116955=CARTESIAN_POINT('Ctrl Pts',(-1.984563179,2.323743665,-6.977048418));
#116956=CARTESIAN_POINT('Ctrl Pts',(-2.208336691,2.285714286,-6.905486881));
#116957=CARTESIAN_POINT('Ctrl Pts',(-2.363697654,2.259311335,-6.8558033));
#116958=CARTESIAN_POINT('Ctrl Pts',(-2.516666969,2.232664075,-6.79918284600001));
#116959=CARTESIAN_POINT('Ctrl Pts',(-2.52040506334849,2.23201289883432,
-6.7977992181848));
#116960=CARTESIAN_POINT('Ctrl Pts',(-2.52414315769698,2.23136172266864,
-6.79641559036959));
#116961=CARTESIAN_POINT('Ctrl Pts',(-1.577585275,2.36225522,-7.332204628));
#116962=CARTESIAN_POINT('Ctrl Pts',(-1.81518665,2.323743665,-7.2810827));
#116963=CARTESIAN_POINT('Ctrl Pts',(-2.048979786,2.285714286,-7.214685152));
#116964=CARTESIAN_POINT('Ctrl Pts',(-2.211297151,2.259311335,-7.16858681300001));
#116965=CARTESIAN_POINT('Ctrl Pts',(-2.37137707,2.232664075,-7.115235119));
#116966=CARTESIAN_POINT('Ctrl Pts',(-2.37528892539741,2.23201289883432,
-7.11393136951387));
#116967=CARTESIAN_POINT('Ctrl Pts',(-2.37920078079482,2.23136172266864,
-7.11262762002775));
#116968=CARTESIAN_POINT('',(-2.44402201117849,2.23266407357604,-6.9572089854233));
#116969=CARTESIAN_POINT('Ctrl Pts',(-2.5093333767475,2.23138000478158,-6.80189732065103));
#116970=CARTESIAN_POINT('Ctrl Pts',(-2.51300017287375,2.23202203989079,
-6.80054008332552));
#116971=CARTESIAN_POINT('Ctrl Pts',(-2.516666969,2.232664075,-6.799182846));
#116972=CARTESIAN_POINT('Ctrl Pts',(-2.884823095,2.297126115,-6.662912593));
#116973=CARTESIAN_POINT('Ctrl Pts',(-3.23611259,2.362252267,-6.487686437));
#116974=CARTESIAN_POINT('Ctrl Pts',(-2.82522894021175,2.23138000478158,
-6.94752811231027));
#116975=CARTESIAN_POINT('Ctrl Pts',(-2.82897409110587,2.23202203989079,
-6.94600042815513));
#116976=CARTESIAN_POINT('Ctrl Pts',(-2.832719242,2.232664075,-6.944472744));
#116977=CARTESIAN_POINT('Ctrl Pts',(-3.208742396,2.297126115,-6.791089174));
#116978=CARTESIAN_POINT('Ctrl Pts',(-3.566005068,2.362252267,-6.598000292));
#116979=CARTESIAN_POINT('',(-2.83271924697018,2.23266407419429,-6.94447273970029));
#116980=CARTESIAN_POINT('',(-3.34491185041081,2.32233405366361,-6.71279112679404));
#116981=CARTESIAN_POINT('Origin',(0.0969976335030265,2.4106740959476,0.162894538142772));
#116982=CARTESIAN_POINT('Ctrl Pts',(-3.23191703662375,2.36147458186189,
-6.48977752055159));
#116983=CARTESIAN_POINT('Ctrl Pts',(-3.25068803512464,2.354614306655,-6.52690738309182));
#116984=CARTESIAN_POINT('Ctrl Pts',(-3.26950140686306,2.34792815738699,
-6.56407746796472));
#116985=CARTESIAN_POINT('Ctrl Pts',(-3.30716101048175,2.33489257347995,
-6.63840262764445));
#116986=CARTESIAN_POINT('Ctrl Pts',(-3.32602935391116,2.32853549231932,
-6.67560133771195));
#116987=CARTESIAN_POINT('Ctrl Pts',(-3.34491184879149,2.32233405369777,
-6.71279112756188));
#116988=CARTESIAN_POINT('',(-2.67469311915078,2.23266407264717,-6.87182778968677));
#116989=CARTESIAN_POINT('Origin',(-1.81929124543068E-13,2.32340998499989,
-3.81205483845903E-13));
#116990=CARTESIAN_POINT('',(-3.34678523568675,2.14301213127624,-6.71185731238674));
#116991=CARTESIAN_POINT('Origin',(0.101033801869133,2.01794101580762,0.157798815744163));
#116992=CARTESIAN_POINT('',(-3.84550081497575,2.23266407449122,-6.43910890169064));
#116993=CARTESIAN_POINT('Origin',(0.117122493431832,2.4105239843923,0.140959894913686));
#116994=CARTESIAN_POINT('Ctrl Pts',(-3.34491185149413,2.32233405321711,
-6.71279112629689));
#116995=CARTESIAN_POINT('Ctrl Pts',(-3.41460886186971,2.31006874161239,
-6.67806185287211));
#116996=CARTESIAN_POINT('Ctrl Pts',(-3.48365954759103,2.29785936479251,
-6.64229934151317));
#116997=CARTESIAN_POINT('Ctrl Pts',(-3.55201981983207,2.28571428604147,
-6.60553973487858));
#116998=CARTESIAN_POINT('Ctrl Pts',(-3.65084443614975,2.26815682566445,
-6.5523984313499));
#116999=CARTESIAN_POINT('Ctrl Pts',(-3.74872611297771,2.25046493734972,
-6.49690373263539));
#117000=CARTESIAN_POINT('Ctrl Pts',(-3.84550081992341,2.23266407446841,
-6.43910890112039));
#117001=CARTESIAN_POINT('Ctrl Pts',(-3.227653236,2.36225522,-6.491899151));
#117002=CARTESIAN_POINT('Ctrl Pts',(-3.438024365,2.323743665,-6.387306483));
#117003=CARTESIAN_POINT('Ctrl Pts',(-3.641182561,2.285714286,-6.269313324));
#117004=CARTESIAN_POINT('Ctrl Pts',(-3.78223077,2.259311335,-6.187393303));
#117005=CARTESIAN_POINT('Ctrl Pts',(-3.919452023,2.232664075,-6.09921272300001));
#117006=CARTESIAN_POINT('Ctrl Pts',(-3.92280528368717,2.23201289883432,
-6.09705786385231));
#117007=CARTESIAN_POINT('Ctrl Pts',(-3.92615854437433,2.23136172266864,
-6.09490300470461));
#117008=CARTESIAN_POINT('Ctrl Pts',(-3.116909465,2.36225522,-6.821647557));
#117009=CARTESIAN_POINT('Ctrl Pts',(-3.337966148,2.323743665,-6.72064355999999));
#117010=CARTESIAN_POINT('Ctrl Pts',(-3.55201982,2.285714286,-6.605539735));
#117011=CARTESIAN_POINT('Ctrl Pts',(-3.700632515,2.259311335,-6.525625715));
#117012=CARTESIAN_POINT('Ctrl Pts',(-3.845500817,2.232664075,-6.439108903));
#117013=CARTESIAN_POINT('Ctrl Pts',(-3.84904094778363,2.23201289883432,
-6.43699470116816));
#117014=CARTESIAN_POINT('Ctrl Pts',(-3.85258107856726,2.23136172266864,
-6.43488049933635));
#117015=CARTESIAN_POINT('',(-3.88247641250146,2.23266407357604,-6.26916081764383));
#117016=CARTESIAN_POINT('Ctrl Pts',(-3.91287341787142,2.23138000478158,
-6.10344024028336));
#117017=CARTESIAN_POINT('Ctrl Pts',(-3.91616272043571,2.23202203989079,
-6.10132648164168));
#117018=CARTESIAN_POINT('Ctrl Pts',(-3.919452023,2.232664075,-6.09921272300001));
#117019=CARTESIAN_POINT('Ctrl Pts',(-4.249706787,2.297126115,-5.886985709));
#117020=CARTESIAN_POINT('Ctrl Pts',(-4.555114885,2.362252267,-5.640339386));
#117021=CARTESIAN_POINT('Ctrl Pts',(-4.25268983415697,2.23138000478158,
-6.17775805698345));
#117022=CARTESIAN_POINT('Ctrl Pts',(-4.25601901857848,2.23202203989079,
-6.17546099249173));
#117023=CARTESIAN_POINT('Ctrl Pts',(-4.259348203,2.232664075,-6.173163928));
#117024=CARTESIAN_POINT('Ctrl Pts',(-4.593607212,2.297126115,-5.942532517));
#117025=CARTESIAN_POINT('Ctrl Pts',(-4.901008879,2.362252267,-5.677157033));
#117026=CARTESIAN_POINT('',(-4.2593482069289,2.23266407419428,-6.17316392273257));
#117027=CARTESIAN_POINT('',(-4.70976133415161,2.32233405363239,-5.83679262770778));
#117028=CARTESIAN_POINT('Origin',(0.129747478483248,2.41067415754769,0.138234636497682));
#117029=CARTESIAN_POINT('Ctrl Pts',(-4.55146694246914,2.3614745818666,-5.64328350111219));
#117030=CARTESIAN_POINT('Ctrl Pts',(-4.57778088593664,2.3546143125077,-5.67551005075196));
#117031=CARTESIAN_POINT('Ctrl Pts',(-4.60414485515913,2.34792816933081,
-5.70776676917776));
#117032=CARTESIAN_POINT('Ctrl Pts',(-4.65690176272403,2.33489257255299,
-5.7722586097785));
#117033=CARTESIAN_POINT('Ctrl Pts',(-4.68332560212223,2.32853549046343,
-5.80453150350009));
#117034=CARTESIAN_POINT('Ctrl Pts',(-4.70976133268649,2.3223340536587,-5.83679262891339));
#117035=CARTESIAN_POINT('',(-4.08940012518944,2.23266407264717,-6.13618831737648));
#117036=CARTESIAN_POINT('Origin',(5.29090660172926E-14,2.32340998499989,
7.84962372879505E-14));
#117037=CARTESIAN_POINT('',(-4.71139017771449,2.14301213125108,-5.83547792273423));
#117038=CARTESIAN_POINT('Origin',(0.132593752782683,2.01794102669776,0.132390265305984));
#117039=CARTESIAN_POINT('',(-5.13981321874104,2.23266407449122,-5.46189711015753));
#117040=CARTESIAN_POINT('Origin',(0.144686138640672,2.41052395745531,0.112486115523932));
#117041=CARTESIAN_POINT('Ctrl Pts',(-4.70976133507838,2.32233405317635,
-5.83679262687341));
#117042=CARTESIAN_POINT('Ctrl Pts',(-4.77036310094747,2.31006874158962,
-5.78789250779538));
#117043=CARTESIAN_POINT('Ctrl Pts',(-4.83011153734743,2.29785936478343,
-5.73812224794854));
#117044=CARTESIAN_POINT('Ctrl Pts',(-4.88897135546675,2.28571428611673,
-5.68752662272347));
#117045=CARTESIAN_POINT('Ctrl Pts',(-4.97406169678273,2.2681568258489,-5.61438336118433));
#117046=CARTESIAN_POINT('Ctrl Pts',(-5.05772523537544,2.25046493734972,
-5.53914443058292));
#117047=CARTESIAN_POINT('Ctrl Pts',(-5.139813223451,2.23266407446841,-5.46189710853589));
#117048=CARTESIAN_POINT('Ctrl Pts',(-4.547758915,2.36225522,-5.64627212));
#117049=CARTESIAN_POINT('Ctrl Pts',(-4.730727352,2.323743665,-5.498901196));
#117050=CARTESIAN_POINT('Ctrl Pts',(-4.903770781,2.285714286,-5.339993645));
#117051=CARTESIAN_POINT('Ctrl Pts',(-5.023910978,2.259311335,-5.229667673));
#117052=CARTESIAN_POINT('Ctrl Pts',(-5.138967857,2.232664075,-5.114050192));
#117053=CARTESIAN_POINT('Ctrl Pts',(-5.14177948931427,2.23201289883432,
-5.11122486031624));
#117054=CARTESIAN_POINT('Ctrl Pts',(-5.14459112162854,2.23136172266864,
-5.10839952863248));
#117055=CARTESIAN_POINT('Ctrl Pts',(-4.510490432,2.36225522,-5.992117828));
#117056=CARTESIAN_POINT('Ctrl Pts',(-4.704666059,2.323743665,-5.845954596));
#117057=CARTESIAN_POINT('Ctrl Pts',(-4.888971356,2.285714286,-5.687526623));
#117058=CARTESIAN_POINT('Ctrl Pts',(-5.016930416,2.259311335,-5.577533611));
#117059=CARTESIAN_POINT('Ctrl Pts',(-5.139813221,2.232664075,-5.461897111));
#117060=CARTESIAN_POINT('Ctrl Pts',(-5.14281609460832,2.23201289883432,
-5.45907131455102));
#117061=CARTESIAN_POINT('Ctrl Pts',(-5.14581896821665,2.23136172266864,
-5.45624551810205));
#117062=CARTESIAN_POINT('',(-5.13939053267506,2.23266407357604,-5.28797365764722));
#117063=CARTESIAN_POINT('Ctrl Pts',(-5.13345184724536,2.23138000478158,
-5.11959307791208));
#117064=CARTESIAN_POINT('Ctrl Pts',(-5.13620985212268,2.23202203989079,
-5.11682163495604));
#117065=CARTESIAN_POINT('Ctrl Pts',(-5.138967857,2.232664075,-5.114050192));
#117066=CARTESIAN_POINT('Ctrl Pts',(-5.415878914,2.297126115,-4.835789916));
#117067=CARTESIAN_POINT('Ctrl Pts',(-5.66112507100001,2.362252267,-4.529256333));
#117068=CARTESIAN_POINT('Ctrl Pts',(-5.48129967805377,2.23138000478158,
-5.11912290128042));
#117069=CARTESIAN_POINT('Ctrl Pts',(-5.48405722702689,2.23202203989079,
-5.11616386464021));
#117070=CARTESIAN_POINT('Ctrl Pts',(-5.48681477600001,2.232664075,-5.113204828));
#117071=CARTESIAN_POINT('Ctrl Pts',(-5.763680059,2.297126115,-4.816109645));
#117072=CARTESIAN_POINT('Ctrl Pts',(-6.006846961,2.362252267,-4.49085622));
#117073=CARTESIAN_POINT('',(-5.48681477869489,2.23266407419428,-5.11320482201616));
#117074=CARTESIAN_POINT('',(-5.85438761178372,2.32233405365653,-4.68787219229255));
#117075=CARTESIAN_POINT('Origin',(0.156430345808302,2.41067413916276,0.107110851889194));
#117076=CARTESIAN_POINT('Ctrl Pts',(-5.65819531310717,2.36147458187234,
-4.5329158161281));
#117077=CARTESIAN_POINT('Ctrl Pts',(-5.6908218202369,2.35461430965226,-4.55873221783808));
#117078=CARTESIAN_POINT('Ctrl Pts',(-5.72350367110793,2.34792816349843,
-4.58456733051178));
#117079=CARTESIAN_POINT('Ctrl Pts',(-5.78889096359627,2.33489257215201,
-4.63621019074896));
#117080=CARTESIAN_POINT('Ctrl Pts',(-5.8216347488704,2.32853548963579,-4.66204821970733));
#117081=CARTESIAN_POINT('Ctrl Pts',(-5.85438761057469,2.3223340536835,-4.68787219383246));
#117082=CARTESIAN_POINT('',(-5.31289132665814,2.23266407264717,-5.11362749944603));
#117083=CARTESIAN_POINT('Origin',(-9.39786443110435E-13,2.32340998499933,
-5.47738937539677E-13));
#117084=CARTESIAN_POINT('',(-5.85569575168534,2.14301213125127,-4.68623807130231));
#117085=CARTESIAN_POINT('Origin',(0.157953816337484,2.01794102736107,0.100791350753756));
#117086=CARTESIAN_POINT('',(-6.19379366761472,2.23266407449123,-4.22929308165503));
#117087=CARTESIAN_POINT('Origin',(0.16548488433682,2.41052395892396,0.0787531823237286));
#117088=CARTESIAN_POINT('Ctrl Pts',(-5.85438761247407,2.32233405319692,
-4.68787219120225));
#117089=CARTESIAN_POINT('Ctrl Pts',(-5.90306046264052,2.31006874160582,
-4.62708774125359));
#117090=CARTESIAN_POINT('Ctrl Pts',(-5.95071287908218,2.29785936479246,
-4.56563693457481));
#117091=CARTESIAN_POINT('Ctrl Pts',(-5.99732002373333,2.28571428605796,
-4.50357108604458));
#117092=CARTESIAN_POINT('Ctrl Pts',(-6.06469736209479,2.26815682570485,
-4.41384596610625));
#117093=CARTESIAN_POINT('Ctrl Pts',(-6.130230746824,2.25046493734972,-4.32238089219941));
#117094=CARTESIAN_POINT('Ctrl Pts',(-6.19379367186398,2.23266407446841,
-4.22929307906654));
#117095=CARTESIAN_POINT('Ctrl Pts',(-5.655216442,2.36225522,-4.536631679));
#117096=CARTESIAN_POINT('Ctrl Pts',(-5.802226786,2.323743665,-4.3533734));
#117097=CARTESIAN_POINT('Ctrl Pts',(-5.93706413,2.285714286,-4.160981797));
#117098=CARTESIAN_POINT('Ctrl Pts',(-6.030678693,2.259311335,-4.027408594));
#117099=CARTESIAN_POINT('Ctrl Pts',(-6.118191265,2.232664075,-3.889760358));
#117100=CARTESIAN_POINT('Ctrl Pts',(-6.12032980010958,2.23201289883432,
-3.88639666317616));
#117101=CARTESIAN_POINT('Ctrl Pts',(-6.12246833521915,2.23136172266864,
-3.88303296835232));
#117102=CARTESIAN_POINT('Ctrl Pts',(-5.69316587900001,2.36225522,-4.88240333000001));
#117103=CARTESIAN_POINT('Ctrl Pts',(-5.851381014,2.323743665,-4.697915292));
#117104=CARTESIAN_POINT('Ctrl Pts',(-5.997320024,2.285714286,-4.503571086));
#117105=CARTESIAN_POINT('Ctrl Pts',(-6.09864222700001,2.259311335,-4.368642235));
#117106=CARTESIAN_POINT('Ctrl Pts',(-6.19379367,2.232664075,-4.229293082));
#117107=CARTESIAN_POINT('Ctrl Pts',(-6.19611887536115,2.23201289883432,
-4.22588782205426));
#117108=CARTESIAN_POINT('Ctrl Pts',(-6.1984440807223,2.23136172266864,-4.22248256210852));
#117109=CARTESIAN_POINT('',(-6.15599246264441,2.23266407357604,-4.05952672736318));
#117110=CARTESIAN_POINT('Ctrl Pts',(-6.11399577311955,2.23138000478158,
-3.89635943336084));
#117111=CARTESIAN_POINT('Ctrl Pts',(-6.11609351905978,2.23202203989079,
-3.89305989568042));
#117112=CARTESIAN_POINT('Ctrl Pts',(-6.118191265,2.232664075,-3.889760358));
#117113=CARTESIAN_POINT('Ctrl Pts',(-6.328810561,2.297126115,-3.558477961));
#117114=CARTESIAN_POINT('Ctrl Pts',(-6.50242734,2.362252267,-3.206390288));
#117115=CARTESIAN_POINT('Ctrl Pts',(-6.45361004080255,2.23138000478158,
-3.82112324805941));
#117116=CARTESIAN_POINT('Ctrl Pts',(-6.45566701440128,2.23202203989079,
-3.8176406005297));
#117117=CARTESIAN_POINT('Ctrl Pts',(-6.457723988,2.232664075,-3.814157953));
#117118=CARTESIAN_POINT('Ctrl Pts',(-6.664249632,2.297126115,-3.464490838));
#117119=CARTESIAN_POINT('Ctrl Pts',(-6.831811556,2.362252267,-3.094567962));
#117120=CARTESIAN_POINT('',(-6.45772398935623,2.23266407419428,-3.8141579465679));
#117121=CARTESIAN_POINT('',(-6.72526923157056,2.3223340536739,-3.31975206353202));
#117122=CARTESIAN_POINT('Origin',(0.175799019391143,2.41067416086851,0.0709788985909582));
#117123=CARTESIAN_POINT('Ctrl Pts',(-6.50035275888918,2.36147458185405,
-3.21059402588741));
#117124=CARTESIAN_POINT('Ctrl Pts',(-6.53776626144959,2.35461430567979,
-3.22879313047535));
#117125=CARTESIAN_POINT('Ctrl Pts',(-6.57523783952024,2.34792815538496,
-3.24699861286064));
#117126=CARTESIAN_POINT('Ctrl Pts',(-6.65019804501835,2.33489257396561,
-3.28337772900175));
#117127=CARTESIAN_POINT('Ctrl Pts',(-6.68773069966166,2.32853549328887,
-3.30157272760519));
#117128=CARTESIAN_POINT('Ctrl Pts',(-6.72526923074275,2.32233405371269,
-3.3197520650575));
#117129=CARTESIAN_POINT('',(-6.28795763415186,2.23266407264717,-3.85195914300908));
#117130=CARTESIAN_POINT('Origin',(-8.95550994473027E-13,2.32340998499911,
-4.43872369415566E-13));
#117131=CARTESIAN_POINT('',(-6.72619550060074,2.14301213124985,-3.31787493578972));
#117132=CARTESIAN_POINT('Origin',(0.175927995196032,2.01794103833251,0.064479450497496));
#117133=CARTESIAN_POINT('',(-6.95815920959667,2.23266407449123,-2.798932008156));
#117134=CARTESIAN_POINT('Origin',(0.178546055849216,2.41052401352776,0.0413378320593671));
#117135=CARTESIAN_POINT('Ctrl Pts',(-6.72526923217753,2.32233405323146,
-3.31975206253709));
#117136=CARTESIAN_POINT('Ctrl Pts',(-6.7597372782509,2.31006874161956,-3.24992549503813));
#117137=CARTESIAN_POINT('Ctrl Pts',(-6.79306550086175,2.29785936479525,
-3.1796675130989));
#117138=CARTESIAN_POINT('Ctrl Pts',(-6.82524067351545,2.28571428611621,
-3.10903357124698));
#117139=CARTESIAN_POINT('Ctrl Pts',(-6.87175451781382,2.26815682584759,
-3.00692203889695));
#117140=CARTESIAN_POINT('Ctrl Pts',(-6.91609348176508,2.25046493734972,
-2.90350762661701));
#117141=CARTESIAN_POINT('Ctrl Pts',(-6.95815921318946,2.23266407446841,
-2.79893200473371));
#117142=CARTESIAN_POINT('Ctrl Pts',(-6.498242333,2.36225522,-3.214863384));
#117143=CARTESIAN_POINT('Ctrl Pts',(-6.602420544,2.323743665,-3.004286703));
#117144=CARTESIAN_POINT('Ctrl Pts',(-6.692746959,2.285714286,-2.787407065));
#117145=CARTESIAN_POINT('Ctrl Pts',(-6.755458575,2.259311335,-2.636832366));
#117146=CARTESIAN_POINT('Ctrl Pts',(-6.81133485,2.232664075,-2.483589653));
#117147=CARTESIAN_POINT('Ctrl Pts',(-6.81270029239472,2.23201289883432,
-2.47984487765461));
#117148=CARTESIAN_POINT('Ctrl Pts',(-6.81406573478944,2.23136172266864,
-2.47610010230922));
#117149=CARTESIAN_POINT('Ctrl Pts',(-6.609635218,2.36225522,-3.544393078));
#117150=CARTESIAN_POINT('Ctrl Pts',(-6.724491896,2.323743665,-3.330206691));
#117151=CARTESIAN_POINT('Ctrl Pts',(-6.825240674,2.285714286,-3.109033571));
#117152=CARTESIAN_POINT('Ctrl Pts',(-6.895188305,2.259311335,-2.955478003));
#117153=CARTESIAN_POINT('Ctrl Pts',(-6.958159212,2.232664075,-2.798932008));
#117154=CARTESIAN_POINT('Ctrl Pts',(-6.95969802513763,2.23201289883432,
-2.79510651071521));
#117155=CARTESIAN_POINT('Ctrl Pts',(-6.96123683827525,2.23136172266864,
-2.79128101343042));
#117156=CARTESIAN_POINT('',(-6.88474702784079,2.23266407357604,-2.64126083873485));
#117157=CARTESIAN_POINT('Ctrl Pts',(-6.80865605252724,2.23138000478158,
-2.49093635239381));
#117158=CARTESIAN_POINT('Ctrl Pts',(-6.80999545126362,2.23202203989079,
-2.4872630026969));
#117159=CARTESIAN_POINT('Ctrl Pts',(-6.81133485,2.232664075,-2.483589653));
#117160=CARTESIAN_POINT('Ctrl Pts',(-6.945814061,2.297126115,-2.114775531));
#117161=CARTESIAN_POINT('Ctrl Pts',(-7.039683335,2.362252267,-1.733596997));
#117162=CARTESIAN_POINT('Ctrl Pts',(-7.12415677113848,2.23138000478158,
-2.3444521183563));
#117163=CARTESIAN_POINT('Ctrl Pts',(-7.12541698756924,2.23202203989079,
-2.34060870467815));
#117164=CARTESIAN_POINT('Ctrl Pts',(-7.126677204,2.232664075,-2.336765291));
#117165=CARTESIAN_POINT('Ctrl Pts',(-7.2532063,2.297126115,-1.950876291));
#117166=CARTESIAN_POINT('Ctrl Pts',(-7.337328235,2.362252267,-1.553581145));
#117167=CARTESIAN_POINT('',(-7.12667720394274,2.23266407419429,-2.33676528442554));
#117168=CARTESIAN_POINT('',(-7.28168473677128,2.32233405368831,-1.79640401797926));
#117169=CARTESIAN_POINT('Origin',(0.186947018560235,2.41067412192715,0.0315277854019649));
#117170=CARTESIAN_POINT('Ctrl Pts',(-7.03856093580355,2.36147458185582,
-1.73814842744207));
#117171=CARTESIAN_POINT('Ctrl Pts',(-7.07901198255375,2.35461430875897,
-1.74787924556015));
#117172=CARTESIAN_POINT('Ctrl Pts',(-7.11952111529154,2.34792816168966,
-1.75760380725075));
#117173=CARTESIAN_POINT('Ctrl Pts',(-7.2005492650654,2.3348925741771,-1.777018180687));
#117174=CARTESIAN_POINT('Ctrl Pts',(-7.24111581222357,2.32853549374325,
-1.78671937873909));
#117175=CARTESIAN_POINT('Ctrl Pts',(-7.28168473628263,2.32233405372934,
-1.79640401961946));
#117176=CARTESIAN_POINT('',(-6.96900603178777,2.23266407264717,-2.41017745815618));
#117177=CARTESIAN_POINT('Origin',(1.56515425620007E-12,2.32340998500011,
3.71989765379777E-13));
#117178=CARTESIAN_POINT('',(-7.28218582274825,2.14301213123374,-1.79437165622682));
#117179=CARTESIAN_POINT('Origin',(0.185675943570865,2.01794100957163,0.0251525977595751));
#117180=CARTESIAN_POINT('',(-7.39716895968944,2.23266407449122,-1.23769598468383));
#117181=CARTESIAN_POINT('Origin',(0.183257870512463,2.41052394691905,0.00198920916004167));
#117182=CARTESIAN_POINT('Ctrl Pts',(-7.28168473717622,2.32233405324734,
-1.79640401689558));
#117183=CARTESIAN_POINT('Ctrl Pts',(-7.30033629147207,2.3100687416291,-1.72080034473311));
#117184=CARTESIAN_POINT('Ctrl Pts',(-7.31778192934196,2.29785936479937,
-1.6450203727789));
#117185=CARTESIAN_POINT('Ctrl Pts',(-7.33402065462615,2.28571428606948,
-1.56912110203));
#117186=CARTESIAN_POINT('Ctrl Pts',(-7.35749606995706,2.26815682573308,
-1.45939777797517));
#117187=CARTESIAN_POINT('Ctrl Pts',(-7.3785673717505,2.25046493734972,-1.34886957116084));
#117188=CARTESIAN_POINT('Ctrl Pts',(-7.39716896245992,2.23266407446841,
-1.23769598055493));
#117189=CARTESIAN_POINT('Ctrl Pts',(-7.037417636,2.36225522,-1.742771649));
#117190=CARTESIAN_POINT('Ctrl Pts',(-7.09389245600001,2.323743665,-1.514722898));
#117191=CARTESIAN_POINT('Ctrl Pts',(-7.135484378,2.285714286,-1.283496277));
#117192=CARTESIAN_POINT('Ctrl Pts',(-7.164360722,2.259311335,-1.122960787));
#117193=CARTESIAN_POINT('Ctrl Pts',(-7.185987987,2.232664075,-0.961289056000001));
#117194=CARTESIAN_POINT('Ctrl Pts',(-7.18651649009927,2.23201289883432,
-0.957338301667589));
#117195=CARTESIAN_POINT('Ctrl Pts',(-7.18704499319853,2.23136172266864,
-0.953387547335178));
#117196=CARTESIAN_POINT('Ctrl Pts',(-7.21704536000001,2.36225522,-2.040650945));
#117197=CARTESIAN_POINT('Ctrl Pts',(-7.283173011,2.323743665,-1.806781326));
#117198=CARTESIAN_POINT('Ctrl Pts',(-7.334020655,2.285714286,-1.569121102));
#117199=CARTESIAN_POINT('Ctrl Pts',(-7.36932304100001,2.259311335,-1.404118904));
#117200=CARTESIAN_POINT('Ctrl Pts',(-7.397168962,2.232664075,-1.237695984));
#117201=CARTESIAN_POINT('Ctrl Pts',(-7.39784942971288,2.23201289883432,
-1.23362912538387));
#117202=CARTESIAN_POINT('Ctrl Pts',(-7.39852989742575,2.23136172266864,
-1.22956226676773));
#117203=CARTESIAN_POINT('',(-7.2915784731849,2.23266407357604,-1.09949252872145));
#117204=CARTESIAN_POINT('Ctrl Pts',(-7.18495114151865,2.23138000478158,
-0.969039855917186));
#117205=CARTESIAN_POINT('Ctrl Pts',(-7.18546956425932,2.23202203989079,
-0.965164455958594));
#117206=CARTESIAN_POINT('Ctrl Pts',(-7.18598798700001,2.232664075,-0.961289056));
#117207=CARTESIAN_POINT('Ctrl Pts',(-7.238039015,2.297126115,-0.572188548));
#117208=CARTESIAN_POINT('Ctrl Pts',(-7.24777156,2.362252267,-0.179742638));
#117209=CARTESIAN_POINT('Ctrl Pts',(-7.46158584913562,2.23138000478158,
-0.758157013164344));
#117210=CARTESIAN_POINT('Ctrl Pts',(-7.46199038206781,2.23202203989079,
-0.754132547082172));
#117211=CARTESIAN_POINT('Ctrl Pts',(-7.462394915,2.232664075,-0.750108081));
#117212=CARTESIAN_POINT('Ctrl Pts',(-7.503011102,2.297126115,-0.346040936));
#117213=CARTESIAN_POINT('Ctrl Pts',(-7.499759601,2.362252267,0.0600494));
#117214=CARTESIAN_POINT('',(-7.46239491352179,2.23266407419428,-0.750108074610252));
#117215=CARTESIAN_POINT('',(-7.4976167565496,2.32233405366971,-0.189058116750282));
#117216=CARTESIAN_POINT('Origin',(0.189354078892694,2.41067411514136,-0.00939739047842211));
#117217=CARTESIAN_POINT('Ctrl Pts',(-7.24765382489752,2.36147458195797,
-0.184428940551477));
#117218=CARTESIAN_POINT('Ctrl Pts',(-7.2892509864714,2.35461430889961,-0.185236478159344));
#117219=CARTESIAN_POINT('Ctrl Pts',(-7.33090353101137,2.34792816187836,
-0.18602541882174));
#117220=CARTESIAN_POINT('Ctrl Pts',(-7.41421080436065,2.3348925742867,-0.187567237801838));
#117221=CARTESIAN_POINT('Ctrl Pts',(-7.45591439820413,2.32853549395716,
-0.188321018621582));
#117222=CARTESIAN_POINT('Ctrl Pts',(-7.49761675641736,2.32233405371167,
-0.189058118439435));
#117223=CARTESIAN_POINT('',(-7.32419145269983,2.23266407264717,-0.855698553950613));
#117224=CARTESIAN_POINT('Origin',(1.34441069388203E-14,2.32340998499944,
7.28312809367138E-14));
#117225=CARTESIAN_POINT('',(-7.49766922989768,2.14301213117642,-0.186965551736699));
#117226=CARTESIAN_POINT('Origin',(0.186742279180522,2.01794106467577,-0.0153502760989665));
#117227=CARTESIAN_POINT('',(-7.49029531088826,2.23266407449123,0.381413326840851));
#117228=CARTESIAN_POINT('Origin',(0.179400584072913,2.41052393661623,-0.037452316932809));
#117229=CARTESIAN_POINT('Ctrl Pts',(-7.49761675672826,2.32233405323064,
-0.189058115616846));
#117230=CARTESIAN_POINT('Ctrl Pts',(-7.49957969341663,2.31006874161717,
-0.111212482487324));
#117231=CARTESIAN_POINT('Ctrl Pts',(-7.50032700817362,2.29785936479299,
-0.0334539078254175));
#117232=CARTESIAN_POINT('Ctrl Pts',(-7.49986998160248,2.28571428605214,
0.044161726036502));
#117233=CARTESIAN_POINT('Ctrl Pts',(-7.49920928364054,2.26815682569059,
0.156366300485565));
#117234=CARTESIAN_POINT('Ctrl Pts',(-7.49602765287769,2.25046493734972,
0.268840125821957));
#117235=CARTESIAN_POINT('Ctrl Pts',(-7.49029531270869,2.23266407446841,
0.381413331463295));
#117236=CARTESIAN_POINT('Ctrl Pts',(-7.247531111,2.36225522,-0.189189849));
#117237=CARTESIAN_POINT('Ctrl Pts',(-7.253661841,2.323743665,0.045667665));
#117238=CARTESIAN_POINT('Ctrl Pts',(-7.244574478,2.285714286,0.28042937));
#117239=CARTESIAN_POINT('Ctrl Pts',(-7.238265325,2.259311335,0.443419191));
#117240=CARTESIAN_POINT('Ctrl Pts',(-7.224632313,2.232664075,0.605960349000001));
#117241=CARTESIAN_POINT('Ctrl Pts',(-7.22429916458321,2.23201289883432,
0.609932349424512));
#117242=CARTESIAN_POINT('Ctrl Pts',(-7.22396601616642,2.23136172266864,
0.613904349849024));
#117243=CARTESIAN_POINT('Ctrl Pts',(-7.48699448200001,2.36225522,-0.441490242));
#117244=CARTESIAN_POINT('Ctrl Pts',(-7.50130105,2.323743665,-0.198872874));
#117245=CARTESIAN_POINT('Ctrl Pts',(-7.499869982,2.285714286,0.044161726));
#117246=CARTESIAN_POINT('Ctrl Pts',(-7.498876423,2.259311335,0.212895234));
#117247=CARTESIAN_POINT('Ctrl Pts',(-7.490295313,2.232664075,0.381413328));
#117248=CARTESIAN_POINT('Ctrl Pts',(-7.49008561735748,2.23201289883432,
0.385531386153037));
#117249=CARTESIAN_POINT('Ctrl Pts',(-7.48987592171496,2.23136172266864,
0.389649444306074));
#117250=CARTESIAN_POINT('',(-7.3574638135905,2.23266407357604,0.493686829699741));
#117251=CARTESIAN_POINT('Ctrl Pts',(-7.22528590126796,2.23138000478158,
0.598167867343195));
#117252=CARTESIAN_POINT('Ctrl Pts',(-7.22495910713398,2.23202203989079,
0.602064108171597));
#117253=CARTESIAN_POINT('Ctrl Pts',(-7.224632313,2.232664075,0.605960349000001));
#117254=CARTESIAN_POINT('Ctrl Pts',(-7.191821309,2.297126115,0.997153336));
#117255=CARTESIAN_POINT('Ctrl Pts',(-7.116962042,2.362252267,1.382516288));
#117256=CARTESIAN_POINT('Ctrl Pts',(-7.45011946511826,2.23138000478158,
0.86358867113768));
#117257=CARTESIAN_POINT('Ctrl Pts',(-7.44964939905913,2.23202203989079,
0.867606010068841));
#117258=CARTESIAN_POINT('Ctrl Pts',(-7.449179333,2.232664075,0.871623349000001));
#117259=CARTESIAN_POINT('Ctrl Pts',(-7.401983445,2.297126115,1.274974909));
#117260=CARTESIAN_POINT('Ctrl Pts',(-7.311510543,2.362252267,1.670872101));
#117261=CARTESIAN_POINT('',(-7.4491793301853,2.23266407419428,0.871623354933439));
#117262=CARTESIAN_POINT('',(-7.36296854853005,2.32233405328145,1.42712793824915));
#117263=CARTESIAN_POINT('Origin',(0.182906554548377,2.41067414117802,-0.0498831559296685));
#117264=CARTESIAN_POINT('Ctrl Pts',(-7.11785447610388,2.36147458187397,
1.37791423853736));
#117265=CARTESIAN_POINT('Ctrl Pts',(-7.15865271725039,2.35461430863267,
1.3860677412664));
#117266=CARTESIAN_POINT('Ctrl Pts',(-7.1995010489045,2.34792816140926,1.39425131177284));
#117267=CARTESIAN_POINT('Ctrl Pts',(-7.28119202925304,2.33489258355776,
1.41065412866113));
#117268=CARTESIAN_POINT('Ctrl Pts',(-7.32208259018484,2.32853551289289,
1.41888299719396));
#117269=CARTESIAN_POINT('Ctrl Pts',(-7.36296855028178,2.32233405367328,
1.42712792985716));
#117270=CARTESIAN_POINT('',(-7.3369058215324,2.23266407264717,0.738791863574644));
#117271=CARTESIAN_POINT('Ctrl Pts',(-7.118758086,2.36225522,1.373238257));
#117272=CARTESIAN_POINT('Ctrl Pts',(-7.07425806000001,2.323743665,1.60392286));
#117273=CARTESIAN_POINT('Ctrl Pts',(-7.014916327,2.285714286,1.831242452));
#117274=CARTESIAN_POINT('Ctrl Pts',(-6.973716685,2.259311335,1.98906538));
#117275=CARTESIAN_POINT('Ctrl Pts',(-6.925460861,2.232664075,2.144875721));
#117276=CARTESIAN_POINT('Ctrl Pts',(-6.92428163872934,2.23201289883432,
2.1486832411888));
#117277=CARTESIAN_POINT('Ctrl Pts',(-6.92310241645868,2.23136172266864,
2.15249076137759));
#117278=CARTESIAN_POINT('Ctrl Pts',(-7.406860063,2.36225522,1.178314054));
#117279=CARTESIAN_POINT('Ctrl Pts',(-7.368676589,2.323743665,1.418334652));
#117280=CARTESIAN_POINT('Ctrl Pts',(-7.315033724,2.285714286,1.655379601));
#117281=CARTESIAN_POINT('Ctrl Pts',(-7.277790677,2.259311335,1.819954627));
#117282=CARTESIAN_POINT('Ctrl Pts',(-7.23318378,2.232664075,1.982688177));
#117283=CARTESIAN_POINT('Ctrl Pts',(-7.23209372615764,2.23201289883432,
1.98666487888668));
#117284=CARTESIAN_POINT('Ctrl Pts',(-7.23100367231527,2.23136172266864,
1.99064158077337));
#117285=CARTESIAN_POINT('',(-7.23318377818739,2.23266407449123,1.98268817541319));
#117286=CARTESIAN_POINT('Ctrl Pts',(-7.36296854667059,2.3223340510831,1.42712794630432));
#117287=CARTESIAN_POINT('Ctrl Pts',(-7.34815108198387,2.31006874017642,
1.5035755606298));
#117288=CARTESIAN_POINT('Ctrl Pts',(-7.33216513098452,2.29785936406956,
1.57967682912431));
#117289=CARTESIAN_POINT('Ctrl Pts',(-7.31503372343977,2.28571428610238,
1.65537960077473));
#117290=CARTESIAN_POINT('Ctrl Pts',(-7.29026780498927,2.26815682581373,
1.76481886348275));
#117291=CARTESIAN_POINT('Ctrl Pts',(-7.26298201160635,2.25046493734972,
1.87397915710076));
#117292=CARTESIAN_POINT('Ctrl Pts',(-7.23318377897099,2.23266407446841,
1.9826881803197));
#117293=CARTESIAN_POINT('',(-7.07932232296849,2.23266407357604,2.06378194053243));
#117294=CARTESIAN_POINT('Origin',(-9.98333360424652E-13,2.323409985,1.0993810029003E-13));
#117295=CARTESIAN_POINT('',(-7.36256995669525,2.14301213123928,1.4291828538933));
#117296=CARTESIAN_POINT('Origin',(0.179076531732111,2.01794103526846,-0.0551354734157353));
#117297=CARTESIAN_POINT('Origin',(0.167155057818781,2.41052400122714,-0.075142510148061));
#117298=CARTESIAN_POINT('Ctrl Pts',(-6.92777432193795,2.23138000478158,
2.13740592539923));
#117299=CARTESIAN_POINT('Ctrl Pts',(-6.92661759146898,2.23202203989079,
2.14114082319961));
#117300=CARTESIAN_POINT('Ctrl Pts',(-6.925460861,2.232664075,2.144875721));
#117301=CARTESIAN_POINT('Ctrl Pts',(-6.809322032,2.297126115,2.519869437));
#117302=CARTESIAN_POINT('Ctrl Pts',(-6.65337129,2.362252267,2.880130289));
#117303=CARTESIAN_POINT('Ctrl Pts',(-7.0902937755932,2.23138000478158,2.44495390907349));
#117304=CARTESIAN_POINT('Ctrl Pts',(-7.0889710902966,2.23202203989079,2.44877627453674));
#117305=CARTESIAN_POINT('Ctrl Pts',(-7.08764840500001,2.232664075,2.45259864));
#117306=CARTESIAN_POINT('Ctrl Pts',(-6.95484726800001,2.297126115,2.836374343));
#117307=CARTESIAN_POINT('Ctrl Pts',(-6.781383379,2.362252267,3.20356668));
#117308=CARTESIAN_POINT('',(-7.08764840097537,2.23266407419428,2.45259864517374));
#117309=CARTESIAN_POINT('',(-7.0065546284336,2.23266407264717,2.29873719441841));
#117310=CARTESIAN_POINT('',(-6.88403611738364,2.32233405365637,2.97658306401144));
#117311=CARTESIAN_POINT('Origin',(0.167907100873431,2.41067411058327,-0.0880364936196407));
#117312=CARTESIAN_POINT('Ctrl Pts',(-6.65523216405864,2.36147458188244,
2.87582767986542));
#117313=CARTESIAN_POINT('Ctrl Pts',(-6.69332378753527,2.35461431140157,
2.89256096716532));
#117314=CARTESIAN_POINT('Ctrl Pts',(-6.73145786438581,2.34792816706396,
2.90933438625966));
#117315=CARTESIAN_POINT('Ctrl Pts',(-6.8077129334402,2.33489257223886,2.94291490396888));
#117316=CARTESIAN_POINT('Ctrl Pts',(-6.84587860805331,2.32853548981077,
2.95974168147538));
#117317=CARTESIAN_POINT('Ctrl Pts',(-6.88403611817317,2.32233405368326,
2.9765830622325));
#117318=CARTESIAN_POINT('Origin',(3.17454396103756E-13,2.323409985,-1.94289029309402E-13));
#117319=CARTESIAN_POINT('',(-6.63785661058304,2.23266407449122,3.4912547290495));
#117320=CARTESIAN_POINT('Ctrl Pts',(-6.88403611677099,2.32233405319557,
2.97658306513664));
#117321=CARTESIAN_POINT('Ctrl Pts',(-6.85313109707468,2.31006874160445,
3.0480580637289));
#117322=CARTESIAN_POINT('Ctrl Pts',(-6.82115936347794,2.29785936479146,
3.11894362395074));
#117323=CARTESIAN_POINT('Ctrl Pts',(-6.78815461857248,2.28571428603294,
3.189193764977));
#117324=CARTESIAN_POINT('Ctrl Pts',(-6.74044150717939,2.26815682564355,
3.29075045918057));
#117325=CARTESIAN_POINT('Ctrl Pts',(-6.69032740376249,2.25046493734972,
3.39149300637366));
#117326=CARTESIAN_POINT('Ctrl Pts',(-6.63785661028138,2.23266407446841,
3.4912547340209));
#117327=CARTESIAN_POINT('',(-6.88320509555524,2.14301213128533,2.97850425752067));
#117328=CARTESIAN_POINT('Origin',(0.163037348640993,2.01794103639389,-0.0923426108204922));
#117329=CARTESIAN_POINT('Origin',(0.147094092923629,2.41052394262412,-0.109319328977406));
#117330=CARTESIAN_POINT('Ctrl Pts',(-6.657119845,2.36225522,2.87145527));
#117331=CARTESIAN_POINT('Ctrl Pts',(-6.564069834,2.323743665,3.087180404));
#117332=CARTESIAN_POINT('Ctrl Pts',(-6.457248486,2.285714286,3.296428672));
#117333=CARTESIAN_POINT('Ctrl Pts',(-6.383084804,2.259311335,3.441705082));
#117334=CARTESIAN_POINT('Ctrl Pts',(-6.30246255700001,2.232664075,3.583499089));
#117335=CARTESIAN_POINT('Ctrl Pts',(-6.30049240000562,2.23201289883432,
3.58696409357439));
#117336=CARTESIAN_POINT('Ctrl Pts',(-6.29852224301123,2.23136172266863,
3.59042909814879));
#117337=CARTESIAN_POINT('Ctrl Pts',(-6.9803891,2.36225522,2.743021695));
#117338=CARTESIAN_POINT('Ctrl Pts',(-6.891501001,2.323743665,2.969222426));
#117339=CARTESIAN_POINT('Ctrl Pts',(-6.788154619,2.285714286,3.189193765));
#117340=CARTESIAN_POINT('Ctrl Pts',(-6.716403528,2.259311335,3.341914965));
#117341=CARTESIAN_POINT('Ctrl Pts',(-6.637856612,2.232664075,3.491254731));
#117342=CARTESIAN_POINT('Ctrl Pts',(-6.63593716964131,2.23201289883432,
3.49490413045825));
#117343=CARTESIAN_POINT('Ctrl Pts',(-6.63401772728261,2.23136172266864,
3.4985535299165));
#117344=CARTESIAN_POINT('',(-6.47015958873108,2.23266407357604,3.53737690226101));
#117345=CARTESIAN_POINT('Ctrl Pts',(-6.30632771577688,2.23138000478159,
3.5767012587878));
#117346=CARTESIAN_POINT('Ctrl Pts',(-6.30439513638845,2.23202203989079,
3.5801001738939));
#117347=CARTESIAN_POINT('Ctrl Pts',(-6.302462557,2.232664075,3.583499089));
#117348=CARTESIAN_POINT('Ctrl Pts',(-6.108426424,2.297126115,3.924759245));
#117349=CARTESIAN_POINT('Ctrl Pts',(-5.87867629,2.362252267,4.243072598));
#117350=CARTESIAN_POINT('Ctrl Pts',(-6.39893382949064,2.23138000478159,
3.91199581910429));
#117351=CARTESIAN_POINT('Ctrl Pts',(-6.39682037224532,2.23202203989079,
3.91544448155215));
#117352=CARTESIAN_POINT('Ctrl Pts',(-6.394706915,2.232664075,3.918893144));
#117353=CARTESIAN_POINT('Ctrl Pts',(-6.182510162,2.297126115,4.265148066));
#117354=CARTESIAN_POINT('Ctrl Pts',(-5.934166264,2.362252267,4.586466041));
#117355=CARTESIAN_POINT('',(-6.39470690994674,2.23266407419309,3.91889314820226));
#117356=CARTESIAN_POINT('',(-6.08321380637901,2.32233405369499,4.38685648066802));
#117357=CARTESIAN_POINT('Origin',(0.145056308722421,2.41067415180002,-0.12207334860511));
#117358=CARTESIAN_POINT('Ctrl Pts',(-5.88141859146556,2.361474581931,4.23927061465615));
#117359=CARTESIAN_POINT('Ctrl Pts',(-5.91502250640472,2.35461430846379,
4.26380127089592));
#117360=CARTESIAN_POINT('Ctrl Pts',(-5.94865925730689,2.34792816100449,
4.28838024850817));
#117361=CARTESIAN_POINT('Ctrl Pts',(-6.01591266561634,2.3348925741105,4.33756822829429));
#117362=CARTESIAN_POINT('Ctrl Pts',(-6.04956877750614,2.32853549356583,
4.36220608912047));
#117363=CARTESIAN_POINT('Ctrl Pts',(-6.08321380732606,2.32233405373527,
4.38685647922582));
#117364=CARTESIAN_POINT('',(-6.3485847285369,2.23266407264357,3.75119612913068));
#117365=CARTESIAN_POINT('Origin',(5.3256010712488E-13,2.32340998499967,
-3.86843335142828E-13));
#117366=CARTESIAN_POINT('',(-6.0819892141391,2.143012131239,4.38855411225098));
#117367=CARTESIAN_POINT('Origin',(0.139374592124883,2.01794105755577,-0.125231830788222));
#117368=CARTESIAN_POINT('',(-5.73215064603916,2.23266407449122,4.83657409078815));
#117369=CARTESIAN_POINT('Origin',(0.120154476291418,2.41052397133765,-0.138384219056065));
#117370=CARTESIAN_POINT('Ctrl Pts',(-6.08321380579988,2.32233405325243,
4.38685648167792));
#117371=CARTESIAN_POINT('Ctrl Pts',(-6.0376663161811,2.31006874163299,4.45001676899957));
#117372=CARTESIAN_POINT('Ctrl Pts',(-5.99120376380507,2.29785936480149,
4.51237208663772));
#117373=CARTESIAN_POINT('Ctrl Pts',(-5.94386894792437,2.28571428605536,
4.57388477374788));
#117374=CARTESIAN_POINT('Ctrl Pts',(-5.87543965642865,2.26815682569848,
4.66281021972723));
#117375=CARTESIAN_POINT('Ctrl Pts',(-5.8048405226744,2.25046493734972,4.75042441136098));
#117376=CARTESIAN_POINT('Ctrl Pts',(-5.73215064467174,2.23266407446841,
4.83657409558084));
#117377=CARTESIAN_POINT('Ctrl Pts',(-5.884202079,2.36225522,4.235406225));
#117378=CARTESIAN_POINT('Ctrl Pts',(-5.746952999,2.323743665,4.426084824));
#117379=CARTESIAN_POINT('Ctrl Pts',(-5.597646882,2.285714286,4.607477551));
#117380=CARTESIAN_POINT('Ctrl Pts',(-5.493986972,2.259311335,4.73341448));
#117381=CARTESIAN_POINT('Ctrl Pts',(-5.384768108,2.232664075,4.854562022));
#117382=CARTESIAN_POINT('Ctrl Pts',(-5.38209913861705,2.23201289883432,
4.857522491177));
#117383=CARTESIAN_POINT('Ctrl Pts',(-5.37943016923408,2.23136172266864,
4.860482960354));
#117384=CARTESIAN_POINT('Ctrl Pts',(-6.2275229,2.36225522,4.17946869));
#117385=CARTESIAN_POINT('Ctrl Pts',(-6.092086485,2.323743665,4.38127266));
#117386=CARTESIAN_POINT('Ctrl Pts',(-5.943868948,2.285714286,4.573884774));
#117387=CARTESIAN_POINT('Ctrl Pts',(-5.840964815,2.259311335,4.707611073));
#117388=CARTESIAN_POINT('Ctrl Pts',(-5.732150647,2.232664075,4.836574093));
#117389=CARTESIAN_POINT('Ctrl Pts',(-5.72949156712874,2.23201289883432,
4.83972554815443));
#117390=CARTESIAN_POINT('Ctrl Pts',(-5.72683248725748,2.23136172266864,
4.84287700330887));
#117391=CARTESIAN_POINT('',(-5.55845938329581,2.23266407357604,4.84556805085149));
#117392=CARTESIAN_POINT('Ctrl Pts',(-5.39000423404587,2.23138000478158,
4.8487540161696));
#117393=CARTESIAN_POINT('Ctrl Pts',(-5.38738617102294,2.23202203989079,
4.85165801908481));
#117394=CARTESIAN_POINT('Ctrl Pts',(-5.384768108,2.232664075,4.854562022));
#117395=CARTESIAN_POINT('Ctrl Pts',(-5.121907587,2.297126115,5.146131672));
#117396=CARTESIAN_POINT('Ctrl Pts',(-4.829100921,2.362252267,5.407613549));
#117397=CARTESIAN_POINT('Ctrl Pts',(-5.40836684853112,2.23138000478158,
5.19611715339498));
#117398=CARTESIAN_POINT('Ctrl Pts',(-5.40556144226556,2.23202203989079,
5.19903085719749));
#117399=CARTESIAN_POINT('Ctrl Pts',(-5.402756036,2.232664075,5.201944561));
#117400=CARTESIAN_POINT('Ctrl Pts',(-5.121085753,2.297126115,5.49448820600001));
#117401=CARTESIAN_POINT('Ctrl Pts',(-4.809474131,2.362252267,5.754907348));
#117402=CARTESIAN_POINT('',(-5.40275603017245,2.23266407419428,5.20194456401123));
#117403=CARTESIAN_POINT('',(-4.99794717941593,2.32233405365546,5.59200536389098));
#117404=CARTESIAN_POINT('Origin',(0.115422726916476,2.41067414184866,-0.150402059332356));
#117405=CARTESIAN_POINT('Ctrl Pts',(-4.83259642346235,2.3614745818336,5.40448996725973));
#117406=CARTESIAN_POINT('Ctrl Pts',(-4.86014132679959,2.35461430959202,
5.43567095312031));
#117407=CARTESIAN_POINT('Ctrl Pts',(-4.88770790993196,2.34792816341103,
5.46690618859985));
#117408=CARTESIAN_POINT('Ctrl Pts',(-4.94281497963354,2.3348925835358,5.52940164191918));
#117409=CARTESIAN_POINT('Ctrl Pts',(-4.97038777243001,2.32853551289827,
5.56069850005182));
#117410=CARTESIAN_POINT('Ctrl Pts',(-4.99794718101468,2.32233405368386,
5.59200536248922));
#117411=CARTESIAN_POINT('',(-5.39376206201143,2.23266407264716,5.02825330221466));
#117412=CARTESIAN_POINT('Origin',(8.38738800634786E-13,2.32340998500067,
-8.78637440582253E-13));
#117413=CARTESIAN_POINT('',(-4.99638627678617,2.14301213126216,5.59340005498915));
#117414=CARTESIAN_POINT('Origin',(0.109194973362047,2.01794105197273,-0.152265416766924));
#117415=CARTESIAN_POINT('',(-4.55841568752372,2.23266407449122,5.95574062463771));
#117416=CARTESIAN_POINT('Origin',(0.0875969833547863,2.41052397966279,-0.160978744647284));
#117417=CARTESIAN_POINT('Ctrl Pts',(-4.99794717819094,2.32233405317691,
5.59200536459627));
#117418=CARTESIAN_POINT('Ctrl Pts',(-4.93988696921939,2.31006874159968,
5.6438976355639));
#117419=CARTESIAN_POINT('Ctrl Pts',(-4.88110613546204,2.29785936479266,
5.69480704519649));
#117420=CARTESIAN_POINT('Ctrl Pts',(-4.82165457190422,2.28571428604934,
5.74470601375661));
#117421=CARTESIAN_POINT('Ctrl Pts',(-4.73570877678458,2.26815682568374,
5.81684215755424));
#117422=CARTESIAN_POINT('Ctrl Pts',(-4.64792575016144,2.25046493734972,
5.88723125139048));
#117423=CARTESIAN_POINT('Ctrl Pts',(-4.55841568517172,2.23266407446841,
5.95574062902004));
#117424=CARTESIAN_POINT('Ctrl Pts',(-4.836145564,2.36225522,5.40131429200001));
#117425=CARTESIAN_POINT('Ctrl Pts',(-4.661115028,2.323743665,5.558030436));
#117426=CARTESIAN_POINT('Ctrl Pts',(-4.476305531,2.285714286,5.703085901));
#117427=CARTESIAN_POINT('Ctrl Pts',(-4.347996415,2.259311335,5.803794678));
#117428=CARTESIAN_POINT('Ctrl Pts',(-4.215287887,2.232664075,5.89863103));
#117429=CARTESIAN_POINT('Ctrl Pts',(-4.21204490327798,2.23201289883432,
5.90094853551699));
#117430=CARTESIAN_POINT('Ctrl Pts',(-4.20880191955596,2.23136172266864,
5.90326604103399));
#117431=CARTESIAN_POINT('Ctrl Pts',(-5.183464651,2.36225522,5.420488373));
#117432=CARTESIAN_POINT('Ctrl Pts',(-5.007812776,2.323743665,5.588459453));
#117433=CARTESIAN_POINT('Ctrl Pts',(-4.821654572,2.285714286,5.744706014));
#117434=CARTESIAN_POINT('Ctrl Pts',(-4.692409079,2.259311335,5.85318452000001));
#117435=CARTESIAN_POINT('Ctrl Pts',(-4.558415688,2.232664075,5.955740627));
#117436=CARTESIAN_POINT('Ctrl Pts',(-4.55514130622198,2.23201289883432,
5.95824677932199));
#117437=CARTESIAN_POINT('Ctrl Pts',(-4.55186692444396,2.23136172266864,
5.96075293164397));
#117438=CARTESIAN_POINT('',(-4.38685179458954,2.23266407357604,5.92718582325286));
#117439=CARTESIAN_POINT('Ctrl Pts',(-4.2216501449166,2.23138000478158,5.89408442443341));
#117440=CARTESIAN_POINT('Ctrl Pts',(-4.2184690159583,2.23202203989079,5.8963577272167));
#117441=CARTESIAN_POINT('Ctrl Pts',(-4.215287887,2.232664075,5.89863103));
#117442=CARTESIAN_POINT('Ctrl Pts',(-3.895894042,2.297126115,6.126876702));
#117443=CARTESIAN_POINT('Ctrl Pts',(-3.55372216,2.362252267,6.3193005));
#117444=CARTESIAN_POINT('Ctrl Pts',(-4.16491064522116,2.23138000478158,
6.23727382379452));
#117445=CARTESIAN_POINT('Ctrl Pts',(-4.16154446761058,2.23202203989079,
6.23951632739726));
#117446=CARTESIAN_POINT('Ctrl Pts',(-4.15817829,2.232664075,6.241758831));
#117447=CARTESIAN_POINT('Ctrl Pts',(-3.820205066,2.297126115,6.466912183));
#117448=CARTESIAN_POINT('Ctrl Pts',(-3.459896332,2.362252267,6.654255583));
#117449=CARTESIAN_POINT('',(-4.15817828364985,2.2326640741942,6.24175883270281));
#117450=CARTESIAN_POINT('',(-3.67898209720619,2.32233405367819,6.53567829105955));
#117451=CARTESIAN_POINT('Origin',(0.0803922093623644,2.41067409671174,-0.171698205551547));
#117452=CARTESIAN_POINT('Ctrl Pts',(-3.55780741732799,2.36147458182567,
6.31700137554612));
#117453=CARTESIAN_POINT('Ctrl Pts',(-3.57800534560663,2.35461430959786,
6.35337470724872));
#117454=CARTESIAN_POINT('Ctrl Pts',(-3.59821278482228,2.34792816344734,
6.38980568064731));
#117455=CARTESIAN_POINT('Ctrl Pts',(-3.63859683118454,2.3348925756605,6.46268646034612));
#117456=CARTESIAN_POINT('Ctrl Pts',(-3.65879711607804,2.32853549679951,
6.49917900151715));
#117457=CARTESIAN_POINT('Ctrl Pts',(-3.67898209851557,2.32233405373059,
6.53567829016408));
#117458=CARTESIAN_POINT('',(-4.18673307644033,2.23266407264691,6.07019493881779));
#117459=CARTESIAN_POINT('Origin',(-2.31802424477401E-13,2.32340998500022,
4.01588484688631E-13));
#117460=CARTESIAN_POINT('',(-3.67715786974614,2.14301213125802,6.53670482748408));
#117461=CARTESIAN_POINT('Origin',(0.0739095778989851,2.01794107123741,-0.172179361219065));
#117462=CARTESIAN_POINT('',(-3.1715342780386,2.23266407449122,6.7964233455909));
#117463=CARTESIAN_POINT('Origin',(0.0509434473407411,2.41052397934557,-0.176046121056599));
#117464=CARTESIAN_POINT('Ctrl Pts',(-3.67898209636072,2.32233405324916,
6.53567829182381));
#117465=CARTESIAN_POINT('Ctrl Pts',(-3.61112399808775,2.3100687416221,6.57387612183453));
#117466=CARTESIAN_POINT('Ctrl Pts',(-3.54277340934683,2.29785936479204,
6.61095915618321));
#117467=CARTESIAN_POINT('Ctrl Pts',(-3.47398498685931,2.28571428605154,
6.64691118569604));
#117468=CARTESIAN_POINT('Ctrl Pts',(-3.37454141752927,2.26815682568914,
6.69888502086905));
#117469=CARTESIAN_POINT('Ctrl Pts',(-3.27367913498384,2.25046493734972,
6.7487577009611));
#117470=CARTESIAN_POINT('Ctrl Pts',(-3.17153427480362,2.23266407446842,
6.7964233493648));
#117471=CARTESIAN_POINT('Ctrl Pts',(-3.561956257,2.36225522,6.314662906));
#117472=CARTESIAN_POINT('Ctrl Pts',(-3.3573285,2.323743665,6.43008872300001));
#117473=CARTESIAN_POINT('Ctrl Pts',(-3.145657109,2.285714286,6.532024292));
#117474=CARTESIAN_POINT('Ctrl Pts',(-2.998698378,2.259311335,6.602795887));
#117475=CARTESIAN_POINT('Ctrl Pts',(-2.84870549,2.232664075,6.666886607));
#117476=CARTESIAN_POINT('Ctrl Pts',(-2.84504013027118,2.23201289883432,
6.66845278488491));
#117477=CARTESIAN_POINT('Ctrl Pts',(-2.84137477054235,2.23136172266864,
6.67001896276982));
#117478=CARTESIAN_POINT('Ctrl Pts',(-3.897033357,2.36225522,6.408052045));
#117479=CARTESIAN_POINT('Ctrl Pts',(-3.689379308,2.323743665,6.534336094));
#117480=CARTESIAN_POINT('Ctrl Pts',(-3.473984987,2.285714286,6.646911186));
#117481=CARTESIAN_POINT('Ctrl Pts',(-3.324441509,2.259311335,6.725069564));
#117482=CARTESIAN_POINT('Ctrl Pts',(-3.171534278,2.232664075,6.796423348));
#117483=CARTESIAN_POINT('Ctrl Pts',(-3.1677977007914,2.23201289883432,6.79816701258211));
#117484=CARTESIAN_POINT('Ctrl Pts',(-3.16406112358279,2.23136172266864,
6.7999106771642));
#117485=CARTESIAN_POINT('',(-3.01011989205181,2.23266407357603,6.73165497389956));
#117486=CARTESIAN_POINT('Ctrl Pts',(-2.85589638766259,2.23138000478158,
6.66381399592141));
#117487=CARTESIAN_POINT('Ctrl Pts',(-2.85230093883129,2.23202203989079,
6.6653503014607));
#117488=CARTESIAN_POINT('Ctrl Pts',(-2.84870549,2.232664075,6.666886607));
#117489=CARTESIAN_POINT('Ctrl Pts',(-2.487712823,2.297126115,6.821135787));
#117490=CARTESIAN_POINT('Ctrl Pts',(-2.112175301,2.362252267,6.935503983));
#117491=CARTESIAN_POINT('Ctrl Pts',(-2.72670784948992,2.23138000478158,
6.98678250313632));
#117492=CARTESIAN_POINT('Ctrl Pts',(-2.72293829924496,2.23202203989079,
6.98824894956816));
#117493=CARTESIAN_POINT('Ctrl Pts',(-2.719168749,2.232664075,6.989715396));
#117494=CARTESIAN_POINT('Ctrl Pts',(-2.340695835,2.297126115,7.136950535));
#117495=CARTESIAN_POINT('Ctrl Pts',(-1.948537627,2.362252267,7.242458223));
#117496=CARTESIAN_POINT('',(-2.71916874245356,2.23266407419428,6.98971539627998));
#117497=CARTESIAN_POINT('',(-2.18799190079208,2.32233405367884,7.17375016572119));
#117498=CARTESIAN_POINT('Origin',(0.0416026617872733,2.41067415701389,-0.18496603163382));
#117499=CARTESIAN_POINT('Ctrl Pts',(-2.11665929066327,2.36147458189896,
6.93413682048104));
#117500=CARTESIAN_POINT('Ctrl Pts',(-2.12856580561413,2.35461431306305,
6.97400170170876));
#117501=CARTESIAN_POINT('Ctrl Pts',(-2.14046921697517,2.34792817043707,
7.01392491861478));
#117502=CARTESIAN_POINT('Ctrl Pts',(-2.16424190922401,2.33489257395381,
7.0937832155994));
#117503=CARTESIAN_POINT('Ctrl Pts',(-2.17612510861286,2.32853549326735,
7.13376505783009));
#117504=CARTESIAN_POINT('Ctrl Pts',(-2.18799190243431,2.32233405371755,
7.17375016515142));
#117505=CARTESIAN_POINT('',(-2.78393710593565,2.23266407264716,6.82830100703027));
#117506=CARTESIAN_POINT('Origin',(1.87350135405495E-13,2.32340998500022,
-3.6125616387217E-13));
#117507=CARTESIAN_POINT('',(-2.18598964825113,2.14301213127997,7.17436054675462));
#117508=CARTESIAN_POINT('Origin',(0.0351680361798976,2.01794102414299,-0.184042014620551));
#117509=CARTESIAN_POINT('',(-1.63635545054791,2.23266407449123,7.31931286465458));
#117510=CARTESIAN_POINT('Origin',(0.0119076089986403,2.41052401647693,-0.182881204939523));
#117511=CARTESIAN_POINT('Ctrl Pts',(-2.18799189970922,2.32233405323606,
7.1737501661576));
#117512=CARTESIAN_POINT('Ctrl Pts',(-2.11350888185077,2.31006874162273,
7.1964674666809));
#117513=CARTESIAN_POINT('Ctrl Pts',(-2.03878453578529,2.29785936479673,
7.21799016405599));
#117514=CARTESIAN_POINT('Ctrl Pts',(-1.96387572496019,2.2857142860707,7.23831417758776));
#117515=CARTESIAN_POINT('Ctrl Pts',(-1.85558425318112,2.26815682573609,
7.26769546520652));
#117516=CARTESIAN_POINT('Ctrl Pts',(-1.74635892260611,2.25046493734973,
7.29471974078601));
#117517=CARTESIAN_POINT('Ctrl Pts',(-1.63635544658503,2.23266407446843,
7.31931286764579));
#117518=CARTESIAN_POINT('Ctrl Pts',(-2.121213834,2.36225522,6.932744901));
#117519=CARTESIAN_POINT('Ctrl Pts',(-1.896557022,2.323743665,7.001483207));
#117520=CARTESIAN_POINT('Ctrl Pts',(-1.667921256,2.285714286,7.055532488));
#117521=CARTESIAN_POINT('Ctrl Pts',(-1.509184538,2.259311335,7.093057699));
#117522=CARTESIAN_POINT('Ctrl Pts',(-1.34892079,2.232664075,7.123405976));
#117523=CARTESIAN_POINT('Ctrl Pts',(-1.34500444239351,2.23201289883432,
7.12414759351159));
#117524=CARTESIAN_POINT('Ctrl Pts',(-1.34108809478702,2.23136172266863,
7.12488921102318));
#117525=CARTESIAN_POINT('Ctrl Pts',(-2.428381113,2.36225522,7.095982326));
#117526=CARTESIAN_POINT('Ctrl Pts',(-2.198434563,2.323743665,7.174674441));
#117527=CARTESIAN_POINT('Ctrl Pts',(-1.963875725,2.285714286,7.238314178));
#117528=CARTESIAN_POINT('Ctrl Pts',(-1.80102675,2.259311335,7.282497829));
#117529=CARTESIAN_POINT('Ctrl Pts',(-1.63635545,2.232664075,7.319312867));
#117530=CARTESIAN_POINT('Ctrl Pts',(-1.63233139552941,2.23201289883432,
7.32021251203984));
#117531=CARTESIAN_POINT('Ctrl Pts',(-1.62830734105882,2.23136172266863,
7.32111215707968));
#117532=CARTESIAN_POINT('',(-1.49263812863751,2.23266407357604,7.22135941971465));
#117533=CARTESIAN_POINT('Ctrl Pts',(-1.35660408902388,2.23138000478158,
7.12195103128405));
#117534=CARTESIAN_POINT('Ctrl Pts',(-1.35276243951194,2.23202203989079,
7.12267850364202));
#117535=CARTESIAN_POINT('Ctrl Pts',(-1.34892079,2.232664075,7.123405976));
#117536=CARTESIAN_POINT('Ctrl Pts',(-0.963208917,2.297126115,7.196446144));
#117537=CARTESIAN_POINT('Ctrl Pts',(-0.571865472,2.362252267,7.227411008));
#117538=CARTESIAN_POINT('Ctrl Pts',(-1.16100722477529,2.23138000478158,
7.40959699727959));
#117539=CARTESIAN_POINT('Ctrl Pts',(-1.15701056188764,2.23202203989079,
7.4102188171398));
#117540=CARTESIAN_POINT('Ctrl Pts',(-1.153013899,2.232664075,7.410840637));
#117541=CARTESIAN_POINT('Ctrl Pts',(-0.751738269,2.297126115,7.473273012));
#117542=CARTESIAN_POINT('Ctrl Pts',(-0.346067467,2.362252267,7.492011566));
#117543=CARTESIAN_POINT('',(-1.15301389253179,2.23266407419428,7.41084063587417));
#117544=CARTESIAN_POINT('',(-0.594693634848295,2.32233405365367,7.47638545564975));
#117545=CARTESIAN_POINT('Origin',(0.000867775816465743,2.41067412545509,
-0.189584793094087));
#117546=CARTESIAN_POINT('Ctrl Pts',(-0.57653852750269,2.36147458197995,
7.22703973428062));
#117547=CARTESIAN_POINT('Ctrl Pts',(-0.579596905800721,2.35461430851645,
7.26853217341958));
#117548=CARTESIAN_POINT('Ctrl Pts',(-0.58263971288678,2.34792816106259,
7.31008092149065));
#117549=CARTESIAN_POINT('Ctrl Pts',(-0.588689435203046,2.33489257412025,
7.3931825410563));
#117550=CARTESIAN_POINT('Ctrl Pts',(-0.591699897721052,2.32853549358989,
7.43478416549529));
#117551=CARTESIAN_POINT('Ctrl Pts',(-0.594693636545425,2.32233405369389,
7.47638545543475));
#117552=CARTESIAN_POINT('',(-1.25096733006398,2.23266407264717,7.26712330898502));
#117553=CARTESIAN_POINT('Origin',(1.12435153418536E-14,2.32340998499911,
6.68735899989059E-13));
#117554=CARTESIAN_POINT('',(-0.592606979590432,2.14301213124966,7.47655114136116));
#117555=CARTESIAN_POINT('Origin',(-0.00521771807271636,2.01794103025283,
-0.18729966987722));
#117556=CARTESIAN_POINT('',(-0.0246624610398414,2.23266407449122,7.4999594488273));
#117557=CARTESIAN_POINT('Origin',(-0.0276848262311025,2.4105240391559,-0.181165925910276));
#117558=CARTESIAN_POINT('Ctrl Pts',(-0.594693633718621,2.32233405321371,
7.47638545586976));
#117559=CARTESIAN_POINT('Ctrl Pts',(-0.517068439203315,2.31006874160668,
7.4825599914261));
#117560=CARTESIAN_POINT('Ctrl Pts',(-0.439464362910036,2.29785936478825,
7.48751597444643));
#117561=CARTESIAN_POINT('Ctrl Pts',(-0.361937816336615,2.28571428609189,
7.49126164372934));
#117562=CARTESIAN_POINT('Ctrl Pts',(-0.2498620313125,2.268156825788,7.49667654805276));
#117563=CARTESIAN_POINT('Ctrl Pts',(-0.137380907420494,2.25046493734972,
7.4995887933537));
#117564=CARTESIAN_POINT('Ctrl Pts',(-0.0246624565258185,2.23266407446841,
7.49995945089641));
#117565=CARTESIAN_POINT('Ctrl Pts',(-0.58128581,2.36225522,7.22665945000001));
#117566=CARTESIAN_POINT('Ctrl Pts',(-0.347104645,2.323743665,7.245496119));
#117567=CARTESIAN_POINT('Ctrl Pts',(-0.112195259,2.285714286,7.249131826));
#117568=CARTESIAN_POINT('Ctrl Pts',(0.050897094,2.259311335,7.251656016));
#117569=CARTESIAN_POINT('Ctrl Pts',(0.213937947,2.232664075,7.246842799));
#117570=CARTESIAN_POINT('Ctrl Pts',(0.21792215841634,2.23201289883432,7.24672517894485));
#117571=CARTESIAN_POINT('Ctrl Pts',(0.221906369832681,2.23136172266864,
7.24660755888971));
#117572=CARTESIAN_POINT('Ctrl Pts',(-0.846180468000001,2.36225522,7.452112359));
#117573=CARTESIAN_POINT('Ctrl Pts',(-0.604693462,2.323743665,7.479532986));
#117574=CARTESIAN_POINT('Ctrl Pts',(-0.361937816,2.285714286,7.491261644));
#117575=CARTESIAN_POINT('Ctrl Pts',(-0.193397981,2.259311335,7.49940459));
#117576=CARTESIAN_POINT('Ctrl Pts',(-0.02466246,2.232664075,7.499959451));
#117577=CARTESIAN_POINT('Ctrl Pts',(-0.0205390886072463,2.23201289883432,
7.49997301007732));
#117578=CARTESIAN_POINT('Ctrl Pts',(-0.0164157172144926,2.23136172266864,
7.49998656915463));
#117579=CARTESIAN_POINT('',(0.0946377346806782,2.23266407357604,7.3734011251132));
#117580=CARTESIAN_POINT('Ctrl Pts',(-1.648995459,3.524895017,7.31647551600001));
#117581=CARTESIAN_POINT('Ctrl Pts',(-1.249180034,3.590632927,7.406586365));
#117582=CARTESIAN_POINT('Ctrl Pts',(-0.841926282,3.655724827,7.452594188));
#117583=CARTESIAN_POINT('Ctrl Pts',(-0.837869811072231,3.65637317805554,
7.45305245117261));
#117584=CARTESIAN_POINT('Ctrl Pts',(-0.833813340144462,3.65702152911109,
7.45351071434522));
#117585=CARTESIAN_POINT('Ctrl Pts',(-1.361222842,3.524895017,7.121065396));
#117586=CARTESIAN_POINT('Ctrl Pts',(-0.972085781,3.590632927,7.19545065));
#117587=CARTESIAN_POINT('Ctrl Pts',(-0.577160368,3.655724827,7.2269901));
#117588=CARTESIAN_POINT('Ctrl Pts',(-0.573226694096189,3.65637317805554,
7.22730425023526));
#117589=CARTESIAN_POINT('Ctrl Pts',(-0.569293020192376,3.65702152911109,
7.22761840047053));
#117590=CARTESIAN_POINT('',(-0.841926282128663,3.65572482719224,7.45259418698503));
#117591=CARTESIAN_POINT('',(-0.709543328283387,3.65572482753831,7.33979214368259));
#117592=CARTESIAN_POINT('',(-1.40345265024402,3.56509183363777,7.36751787445755));
#117593=CARTESIAN_POINT('Origin',(0.0485051084111301,3.48217865508547,-0.183541900715324));
#117594=CARTESIAN_POINT('Ctrl Pts',(-1.35657627490457,3.5256799153084,7.12195203649257));
#117595=CARTESIAN_POINT('Ctrl Pts',(-1.36441779022401,3.53257385732365,
7.16281259654519));
#117596=CARTESIAN_POINT('Ctrl Pts',(-1.37224786814811,3.53929993066044,
7.20372923721993));
#117597=CARTESIAN_POINT('Ctrl Pts',(-1.38786954498679,3.55242657232483,
7.28557141202438));
#117598=CARTESIAN_POINT('Ctrl Pts',(-1.3956699808557,3.55883456252376,7.32654325840034));
#117599=CARTESIAN_POINT('Ctrl Pts',(-1.40345265295455,3.5650918265975,7.36751787501784));
#117600=CARTESIAN_POINT('Ctrl Pts',(-1.98065117357706,3.66023518238734,
7.23433615161429));
#117601=CARTESIAN_POINT('Ctrl Pts',(-1.96707967046083,3.65798000469366,
7.23799719735335));
#117602=CARTESIAN_POINT('Ctrl Pts',(-1.95350816734467,3.655724827,7.24165824309244));
#117603=CARTESIAN_POINT('Ctrl Pts',(-1.55924996584151,3.590210912,7.34801325007673));
#117604=CARTESIAN_POINT('Ctrl Pts',(-1.15577569402086,3.524902621,7.41093724298845));
#117605=CARTESIAN_POINT('Ctrl Pts',(-2.14324560227677,3.66023518238734,
6.92601882209799));
#117606=CARTESIAN_POINT('Ctrl Pts',(-2.13025076263838,3.65798000469366,
6.92998674554904));
#117607=CARTESIAN_POINT('Ctrl Pts',(-2.117255923,3.655724827,6.933954669));
#117608=CARTESIAN_POINT('Ctrl Pts',(-1.739750052,3.590210912,7.04922461000001));
#117609=CARTESIAN_POINT('Ctrl Pts',(-1.351961251,3.524902621,7.122829548));
#117610=CARTESIAN_POINT('',(-1.9538431656242,3.65572482796969,7.24102876003761));
#117611=CARTESIAN_POINT('Origin',(0.0455076985269759,3.62500080274065,-0.187575497393542));
#117612=CARTESIAN_POINT('',(-2.03554954552453,3.65572482783621,7.08749169292897));
#117613=CARTESIAN_POINT('Origin',(1.77700736070374E-13,3.74685310400044,
-5.76795555762288E-13));
#117614=CARTESIAN_POINT('',(-1.3977596385386,3.74576903896356,7.36860013775438));
#117615=CARTESIAN_POINT('Origin',(0.0166322859562379,3.6250069064723,-0.191260385052409));
#117616=CARTESIAN_POINT('Origin',(0.0739319513853717,3.48232180518702,-0.168097046009336));
#117617=CARTESIAN_POINT('Ctrl Pts',(-3.183268824,3.524895017,6.79093510500001));
#117618=CARTESIAN_POINT('Ctrl Pts',(-2.812172031,3.590632927,6.96488771));
#117619=CARTESIAN_POINT('Ctrl Pts',(-2.424329967,3.655724827,7.097367414));
#117620=CARTESIAN_POINT('Ctrl Pts',(-2.42046684714056,3.65637317805554,
7.09868698457524));
#117621=CARTESIAN_POINT('Ctrl Pts',(-2.41660372728112,3.65702152911109,
7.10000655515048));
#117622=CARTESIAN_POINT('Ctrl Pts',(-2.860216771,3.524895017,6.661956171));
#117623=CARTESIAN_POINT('Ctrl Pts',(-2.496168149,3.590632927,6.818255304));
#117624=CARTESIAN_POINT('Ctrl Pts',(-2.117255923,3.655724827,6.933954669));
#117625=CARTESIAN_POINT('Ctrl Pts',(-2.11348174922899,3.65637317805554,
6.9351070981874));
#117626=CARTESIAN_POINT('Ctrl Pts',(-2.10970757545797,3.65702152911109,
6.93625952737481));
#117627=CARTESIAN_POINT('',(-2.42432996689638,3.65572482719223,7.0973674129809));
#117628=CARTESIAN_POINT('',(-2.27079294813839,3.65572482753831,7.01566104048418));
#117629=CARTESIAN_POINT('',(-2.95443926801662,3.56509183364827,6.89356856695547));
#117630=CARTESIAN_POINT('Origin',(0.0868271680473698,3.48217862574191,-0.168823614740856));
#117631=CARTESIAN_POINT('Ctrl Pts',(-2.8558694398306,3.52567991525912,6.66382095678268));
#117632=CARTESIAN_POINT('Ctrl Pts',(-2.87231143739544,3.53257385729302,
6.70204052566982));
#117633=CARTESIAN_POINT('Ctrl Pts',(-2.88875432070427,3.5392999306393,6.74031732272066));
#117634=CARTESIAN_POINT('Ctrl Pts',(-2.9216044198429,3.5524265723222,6.81688787423154));
#117635=CARTESIAN_POINT('Ctrl Pts',(-2.93803022178784,3.55883456252969,
6.85522495849874));
#117636=CARTESIAN_POINT('Ctrl Pts',(-2.9544392707911,3.56509182660857,6.89356856691695));
#117637=CARTESIAN_POINT('Ctrl Pts',(-3.4895130783971,3.66023518275518,6.63941993631662));
#117638=CARTESIAN_POINT('Ctrl Pts',(-3.47704588511778,3.65798000487759,
6.64591286140526));
#117639=CARTESIAN_POINT('Ctrl Pts',(-3.46457869183844,3.655724827,6.65240578649394));
#117640=CARTESIAN_POINT('Ctrl Pts',(-3.10240121177959,3.590210912,6.84102813268988));
#117641=CARTESIAN_POINT('Ctrl Pts',(-2.72188674166561,3.524902621,6.98921603906657));
#117642=CARTESIAN_POINT('Ctrl Pts',(-3.58202702740848,3.66023518275517,
6.30335789998202));
#117643=CARTESIAN_POINT('Ctrl Pts',(-3.57018898520421,3.65798000487759,
6.310026562491));
#117644=CARTESIAN_POINT('Ctrl Pts',(-3.558350943,3.655724827,6.316695225));
#117645=CARTESIAN_POINT('Ctrl Pts',(-3.21445058,3.590210912,6.510422821));
#117646=CARTESIAN_POINT('Ctrl Pts',(-2.851550952,3.524902621,6.665670046));
#117647=CARTESIAN_POINT('',(-3.46477053722386,3.65572482796921,6.65171900613451));
#117648=CARTESIAN_POINT('Origin',(0.0847667939926843,3.62500083493656,-0.173406924032474));
#117649=CARTESIAN_POINT('',(-3.51156073694809,3.6557248278362,6.48420709396512));
#117650=CARTESIAN_POINT('Origin',(3.52365706057789E-13,3.74685310400033,
-7.35522753814166E-13));
#117651=CARTESIAN_POINT('',(-2.94911201028439,3.74576903892179,6.89584935664121));
#117652=CARTESIAN_POINT('Origin',(0.0573589000497271,3.62500690824354,-0.183213729323725));
#117653=CARTESIAN_POINT('Origin',(0.108339344283563,3.48232178954017,-0.148273784597132));
#117654=CARTESIAN_POINT('Ctrl Pts',(-4.568696076,3.524895017,5.947858115));
#117655=CARTESIAN_POINT('Ctrl Pts',(-4.243669988,3.590632927,6.197518646));
#117656=CARTESIAN_POINT('Ctrl Pts',(-3.893374677,3.655724827,6.410275628));
#117657=CARTESIAN_POINT('Ctrl Pts',(-3.88988554341135,3.65637317805554,
6.41239480433152));
#117658=CARTESIAN_POINT('Ctrl Pts',(-3.88639640982271,3.65702152911109,
6.41451398066305));
#117659=CARTESIAN_POINT('Ctrl Pts',(-4.225470143,3.524895017,5.891341279));
#117660=CARTESIAN_POINT('Ctrl Pts',(-3.903532469,3.590632927,6.122245918));
#117661=CARTESIAN_POINT('Ctrl Pts',(-3.558350943,3.655724827,6.316695225));
#117662=CARTESIAN_POINT('Ctrl Pts',(-3.55491274551712,3.65637317805554,
6.31863204683871));
#117663=CARTESIAN_POINT('Ctrl Pts',(-3.55147454803423,3.65702152911109,
6.32056886867742));
#117664=CARTESIAN_POINT('',(-3.89337467666367,3.65572482719222,6.41027562703023));
#117665=CARTESIAN_POINT('',(-3.72586281284665,3.65572482753831,6.36348542483327));
#117666=CARTESIAN_POINT('',(-4.36727958874213,3.56509183365971,6.09728365434218));
#117667=CARTESIAN_POINT('Origin',(0.121089349492222,3.48217863436218,-0.146211419860039));
#117668=CARTESIAN_POINT('Ctrl Pts',(-4.22162532422951,3.52567991517959,
5.89409701454771));
#117669=CARTESIAN_POINT('Ctrl Pts',(-4.24589899453622,3.53257385725303,
5.92788848789027));
#117670=CARTESIAN_POINT('Ctrl Pts',(-4.27018583224941,3.53929993064236,
5.9617356610522));
#117671=CARTESIAN_POINT('Ctrl Pts',(-4.31872831917925,3.5524265723403,6.02945423542216));
#117672=CARTESIAN_POINT('Ctrl Pts',(-4.34301143468863,3.55883456254377,
6.06336395806092));
#117673=CARTESIAN_POINT('Ctrl Pts',(-4.36727959145042,3.56509182661936,
6.09728365370327));
#117674=CARTESIAN_POINT('Ctrl Pts',(-4.83520922754559,3.66023518254056,
5.734051826069));
#117675=CARTESIAN_POINT('Ctrl Pts',(-4.82442929775634,3.65798000477028,
5.74307302777226));
#117676=CARTESIAN_POINT('Ctrl Pts',(-4.81364936796707,3.655724827,5.75209422947556));
#117677=CARTESIAN_POINT('Ctrl Pts',(-4.50048762381256,3.590210912,6.01416414226722));
#117678=CARTESIAN_POINT('Ctrl Pts',(-4.16072539051528,3.524902621,6.24068686043289));
#117679=CARTESIAN_POINT('Ctrl Pts',(-4.85331684811587,3.66023518254055,
5.38595896879557));
#117680=CARTESIAN_POINT('Ctrl Pts',(-4.8431891385579,3.65798000477028,5.39501655039777));
#117681=CARTESIAN_POINT('Ctrl Pts',(-4.83306142900001,3.655724827,5.404074132));
#117682=CARTESIAN_POINT('Ctrl Pts',(-4.538846972,3.590210912,5.667200897));
#117683=CARTESIAN_POINT('Ctrl Pts',(-4.2178053,3.524902621,5.896831221));
#117684=CARTESIAN_POINT('',(-4.81368909063475,3.65572482796923,5.75138226461583));
#117685=CARTESIAN_POINT('Origin',(0.120062423877048,3.62500079669572,-0.151130525073971));
#117686=CARTESIAN_POINT('',(-4.8233752520844,3.65572482783621,5.57772817788604));
#117687=CARTESIAN_POINT('Origin',(-1.32272665043232E-14,3.74685310399945,
-1.3834419720915E-13));
#117688=CARTESIAN_POINT('',(-4.36256718226609,3.74576903900012,6.10065632338557));
#117689=CARTESIAN_POINT('Origin',(0.0954033633209156,3.62500690501871,-0.166599734340824));
#117690=CARTESIAN_POINT('Origin',(0.137680597554032,3.48232182391876,-0.12151708137942));
#117691=CARTESIAN_POINT('Ctrl Pts',(-5.740496178,3.524895017,4.826665891));
#117692=CARTESIAN_POINT('Ctrl Pts',(-5.476738654,3.590632927,5.140360499));
#117693=CARTESIAN_POINT('Ctrl Pts',(-5.180369514,3.655724827,5.423446478));
#117694=CARTESIAN_POINT('Ctrl Pts',(-5.17741751467674,3.65637317805554,
5.42626616974804));
#117695=CARTESIAN_POINT('Ctrl Pts',(-5.17446551535348,3.65702152911109,
5.42908586149607));
#117696=CARTESIAN_POINT('Ctrl Pts',(-5.393145228,3.524895017,4.845253817));
#117697=CARTESIAN_POINT('Ctrl Pts',(-5.128371949,3.590632927,5.139967117));
#117698=CARTESIAN_POINT('Ctrl Pts',(-4.833061429,3.655724827,5.404074132));
#117699=CARTESIAN_POINT('Ctrl Pts',(-4.83011997411306,3.65637317805554,
5.40670478284829));
#117700=CARTESIAN_POINT('Ctrl Pts',(-4.82717851922612,3.65702152911109,
5.40933543369657));
#117701=CARTESIAN_POINT('',(-5.18036951346671,3.65572482719222,5.42344647712341));
#117702=CARTESIAN_POINT('',(-5.0067154739218,3.65572482753831,5.41376030276029));
#117703=CARTESIAN_POINT('',(-5.57591077020258,3.56509183361144,5.01589653507367));
#117704=CARTESIAN_POINT('Origin',(0.149689339756273,3.48217862564796,-0.11676230994226));
#117705=CARTESIAN_POINT('Ctrl Pts',(-5.38998270015482,3.52567991529733,
4.84877164788896));
#117706=CARTESIAN_POINT('Ctrl Pts',(-5.4209530333726,3.53257385731543,4.87655497351864));
#117707=CARTESIAN_POINT('Ctrl Pts',(-5.45194819991669,3.53929993065206,
4.9043898661806));
#117708=CARTESIAN_POINT('Ctrl Pts',(-5.51391328222832,3.55242657230943,
4.96009001803131));
#117709=CARTESIAN_POINT('Ctrl Pts',(-5.54491826003029,3.5588345625054,4.98798679819863));
#117710=CARTESIAN_POINT('Ctrl Pts',(-5.57591077268672,3.56509182657088,
5.01589653389362));
#117711=CARTESIAN_POINT('Ctrl Pts',(-5.95481636838717,3.66023518243299,
4.56056582557203));
#117712=CARTESIAN_POINT('Ctrl Pts',(-5.9462277592515,3.6579800047165,4.57169348256676));
#117713=CARTESIAN_POINT('Ctrl Pts',(-5.93763915011584,3.655724827,4.58282113956136));
#117714=CARTESIAN_POINT('Ctrl Pts',(-5.68813623743456,3.590210912,4.90608452105027));
#117715=CARTESIAN_POINT('Ctrl Pts',(-5.405013144833,3.524902621,5.20035010028962));
#117716=CARTESIAN_POINT('Ctrl Pts',(-5.89767096768627,3.66023518243299,
4.21671858239213));
#117717=CARTESIAN_POINT('Ctrl Pts',(-5.88972715084314,3.6579800047165,4.22774156069603));
#117718=CARTESIAN_POINT('Ctrl Pts',(-5.881783334,3.655724827,4.238764539));
#117719=CARTESIAN_POINT('Ctrl Pts',(-5.651011924,3.590210912,4.558986958));
#117720=CARTESIAN_POINT('Ctrl Pts',(-5.386839759,3.524902621,4.852263122));
#117721=CARTESIAN_POINT('',(-5.93752489301315,3.65572482796969,4.58211728013338));
#117722=CARTESIAN_POINT('Origin',(0.149744069363979,3.62500078453731,-0.121787357599193));
#117723=CARTESIAN_POINT('',(-5.90965410140387,3.6557248278362,4.41044089164858));
#117724=CARTESIAN_POINT('Origin',(-5.31692745386891E-13,3.74685310399945,
5.28656979303932E-13));
#117725=CARTESIAN_POINT('',(-5.57203356115642,3.74576903893306,5.0202033813573));
#117726=CARTESIAN_POINT('Origin',(0.128986941211358,3.62500691642831,-0.1421958581512));
#117727=CARTESIAN_POINT('Origin',(0.160584885775001,3.48232175534712,-0.0890793231381287));
#117728=CARTESIAN_POINT('Ctrl Pts',(-6.643877059,3.524895017,3.479784134));
#117729=CARTESIAN_POINT('Ctrl Pts',(-6.45372110700001,3.590632927,3.842844807));
#117730=CARTESIAN_POINT('Ctrl Pts',(-6.225136031,3.655724827,4.183022998));
#117731=CARTESIAN_POINT('Ctrl Pts',(-6.22285919816356,3.65637317805554,
4.18641135951976));
#117732=CARTESIAN_POINT('Ctrl Pts',(-6.22058236532713,3.65702152911109,
4.18979972103951));
#117733=CARTESIAN_POINT('Ctrl Pts',(-6.308642835,3.524895017,3.572607672));
#117734=CARTESIAN_POINT('Ctrl Pts',(-6.113414457,3.590632927,3.917349167));
#117735=CARTESIAN_POINT('Ctrl Pts',(-5.881783334,3.655724827,4.238764539));
#117736=CARTESIAN_POINT('Ctrl Pts',(-5.87947616086335,3.65637317805554,
4.24196601254285));
#117737=CARTESIAN_POINT('Ctrl Pts',(-5.87716898772669,3.65702152911109,
4.24516748608571));
#117738=CARTESIAN_POINT('',(-6.2251360300065,3.65572482719341,4.18302299766136));
#117739=CARTESIAN_POINT('',(-6.05345968438371,3.65572482753831,4.21089376579204));
#117740=CARTESIAN_POINT('',(-6.52381856146396,3.56509183365653,3.69997166835753));
#117741=CARTESIAN_POINT('Origin',(0.171290316374076,3.48217861527856,-0.0818537976551986));
#117742=CARTESIAN_POINT('Ctrl Pts',(-6.30631047561056,3.52567991521273,
3.57672310740658));
#117743=CARTESIAN_POINT('Ctrl Pts',(-6.3425293335264,3.53257385729465,3.59719916832424));
#117744=CARTESIAN_POINT('Ctrl Pts',(-6.37878352962734,3.53929993068875,
3.61772025216271));
#117745=CARTESIAN_POINT('Ctrl Pts',(-6.45127378889825,3.55242657236831,
3.65879750424727));
#117746=CARTESIAN_POINT('Ctrl Pts',(-6.48755087059545,3.55883456255701,
3.67937691930957));
#117747=CARTESIAN_POINT('Ctrl Pts',(-6.52381856365252,3.56509182661619,
3.69997166664249));
#117748=CARTESIAN_POINT('Ctrl Pts',(-6.79598291391073,3.66023518252636,
3.17383283411095));
#117749=CARTESIAN_POINT('Ctrl Pts',(-6.78998721890074,3.65798000476318,
3.18654663001993));
#117750=CARTESIAN_POINT('Ctrl Pts',(-6.78399152389072,3.655724827,3.19926042592882));
#117751=CARTESIAN_POINT('Ctrl Pts',(-6.60981392261041,3.590210912,3.56860184020761));
#117752=CARTESIAN_POINT('Ctrl Pts',(-6.39656849161497,3.524902621,3.91685074986811));
#117753=CARTESIAN_POINT('Ctrl Pts',(-6.66625654791415,3.66023518252636,
2.85030912050949));
#117754=CARTESIAN_POINT('Ctrl Pts',(-6.66086806745706,3.65798000476318,
2.86278207375473));
#117755=CARTESIAN_POINT('Ctrl Pts',(-6.655479587,3.655724827,2.875255027));
#117756=CARTESIAN_POINT('Ctrl Pts',(-6.49894183800001,3.590210912,3.237599855));
#117757=CARTESIAN_POINT('Ctrl Pts',(-6.303991579,3.524902621,3.580808593));
#117758=CARTESIAN_POINT('',(-6.78372862907646,3.65572482796968,3.19859758423855));
#117759=CARTESIAN_POINT('Origin',(0.172423757110239,3.62500079678153,-0.0867494472170341));
#117760=CARTESIAN_POINT('',(-6.71960409236808,3.6557248278362,3.03692629071717));
#117761=CARTESIAN_POINT('Origin',(-4.58400678526871E-13,3.74685310399922,
2.42210765333262E-13));
#117762=CARTESIAN_POINT('',(-6.52095784402233,3.74576903896765,3.70501130866201));
#117763=CARTESIAN_POINT('Origin',(0.1565391361659,3.62500690036652,-0.111142978870203));
#117764=CARTESIAN_POINT('Origin',(0.175979677428308,3.48232175808432,-0.0524755584305797));
#117765=CARTESIAN_POINT('Ctrl Pts',(-7.236597633,3.524895017,1.970191539));
#117766=CARTESIAN_POINT('Ctrl Pts',(-7.128934734,3.590632927,2.365641964));
#117767=CARTESIAN_POINT('Ctrl Pts',(-6.978822105,3.655724827,2.747006012));
#117768=CARTESIAN_POINT('Ctrl Pts',(-6.97732690081234,3.65637317805554,
2.75080460726404));
#117769=CARTESIAN_POINT('Ctrl Pts',(-6.97583169662468,3.65702152911109,
2.75460320252807));
#117770=CARTESIAN_POINT('Ctrl Pts',(-6.929155316,3.524895017,2.132910362));
#117771=CARTESIAN_POINT('Ctrl Pts',(-6.812600499,3.590632927,2.511560324));
#117772=CARTESIAN_POINT('Ctrl Pts',(-6.655479587,3.655724827,2.875255027));
#117773=CARTESIAN_POINT('Ctrl Pts',(-6.65391457646654,3.65637317805554,
2.87887762588843));
#117774=CARTESIAN_POINT('Ctrl Pts',(-6.65234956593308,3.65702152911109,
2.88250022477685));
#117775=CARTESIAN_POINT('',(-6.97882210397194,3.65572482719341,2.74700601187689));
#117776=CARTESIAN_POINT('',(-6.81715084725753,3.65572482753831,2.81113051645041));
#117777=CARTESIAN_POINT('',(-7.16667984697849,3.56509183358835,2.21104023908412));
#117778=CARTESIAN_POINT('Origin',(0.184881715215719,3.48217862292307,-0.0431177229222868));
#117779=CARTESIAN_POINT('Ctrl Pts',(-6.92776218226152,3.52567991532782,
2.13743097000641));
#117780=CARTESIAN_POINT('Ctrl Pts',(-6.96753601101609,3.53257385732146,
2.14964232807016));
#117781=CARTESIAN_POINT('Ctrl Pts',(-7.00735403030485,3.53929993063986,
2.16189005980139));
#117782=CARTESIAN_POINT('Ctrl Pts',(-7.0869799025562,3.5524265722855,2.18642368566547));
#117783=CARTESIAN_POINT('Ctrl Pts',(-7.12683281221999,3.55883456247887,
2.19872346528053));
#117784=CARTESIAN_POINT('Ctrl Pts',(-7.16667984873252,3.56509182654799,
2.21104023698621));
#117785=CARTESIAN_POINT('Ctrl Pts',(-7.31937685100235,3.66023518245291,
1.63869494790891));
#117786=CARTESIAN_POINT('Ctrl Pts',(-7.31625442236225,3.65798000472645,
1.65240039930247));
#117787=CARTESIAN_POINT('Ctrl Pts',(-7.31313199372215,3.655724827,1.66610585069603));
#117788=CARTESIAN_POINT('Ctrl Pts',(-7.22242405433387,3.590210912,2.06425530344297));
#117789=CARTESIAN_POINT('Ctrl Pts',(-7.08902740513761,3.524902621,2.4502038113659));
#117790=CARTESIAN_POINT('Ctrl Pts',(-7.12313537988812,3.6602351824529,1.35062237334953));
#117791=CARTESIAN_POINT('Ctrl Pts',(-7.12055419544399,3.65798000472645,
1.36396207967477));
#117792=CARTESIAN_POINT('Ctrl Pts',(-7.117973011,3.655724827,1.377301786));
#117793=CARTESIAN_POINT('Ctrl Pts',(-7.042988456,3.590210912,1.764826182));
#117794=CARTESIAN_POINT('Ctrl Pts',(-6.926375758,3.524902621,2.141919433));
#117795=CARTESIAN_POINT('',(-7.31273275387848,3.65572482796968,1.66551502051135));
#117796=CARTESIAN_POINT('Origin',(0.187041280494084,3.62500079681395,-0.0476553129920807));
#117797=CARTESIAN_POINT('',(-7.21535286393197,3.6557248278362,1.52140839206518));
#117798=CARTESIAN_POINT('Origin',(3.19622800448727E-13,3.74685310400067,
-1.90602741922952E-13));
#117799=CARTESIAN_POINT('',(-7.16496938536899,3.74576903896349,2.21657702469344));
#117800=CARTESIAN_POINT('Origin',(0.176771704888491,3.62500695122242,-0.0748931927977434));
#117801=CARTESIAN_POINT('Origin',(0.183145646297144,3.48232178901916,-0.0134181692116192));
#117802=CARTESIAN_POINT('Ctrl Pts',(-7.490942944,3.524895017,0.368474977));
#117803=CARTESIAN_POINT('Ctrl Pts',(-7.470807296,3.590632927,0.777824331000001));
#117804=CARTESIAN_POINT('Ctrl Pts',(-7.406186214,3.655724827,1.182542078));
#117805=CARTESIAN_POINT('Ctrl Pts',(-7.40554255255019,3.65637317805554,
1.18657328892585));
#117806=CARTESIAN_POINT('Ctrl Pts',(-7.40489889110037,3.65702152911109,
1.19060449985171));
#117807=CARTESIAN_POINT('Ctrl Pts',(-7.225668194,3.524895017,0.593480535));
#117808=CARTESIAN_POINT('Ctrl Pts',(-7.19323691400001,3.590632927,0.988333711));
#117809=CARTESIAN_POINT('Ctrl Pts',(-7.117973011,3.655724827,1.377301786));
#117810=CARTESIAN_POINT('Ctrl Pts',(-7.11722334121076,3.65637317805554,
1.38117612154711));
#117811=CARTESIAN_POINT('Ctrl Pts',(-7.11647367142152,3.65702152911109,
1.38505045709422));
#117812=CARTESIAN_POINT('',(-7.40618621304264,3.65572482719222,1.18254207762938));
#117813=CARTESIAN_POINT('',(-7.26207961307256,3.65572482753831,1.27992192875138));
#117814=CARTESIAN_POINT('',(-7.47443514863315,3.56509183364457,0.618723025311942));
#117815=CARTESIAN_POINT('Origin',(0.189828274593485,3.48217859273075,-0.002365545620195));
#117816=CARTESIAN_POINT('Ctrl Pts',(-7.22527942811084,3.5256799152277,0.59819493566734));
#117817=CARTESIAN_POINT('Ctrl Pts',(-7.26674844813655,3.53257385726692,
0.601570601551338));
#117818=CARTESIAN_POINT('Ctrl Pts',(-7.30826844481787,3.53929993062775,
0.604972290989346));
#117819=CARTESIAN_POINT('Ctrl Pts',(-7.39130671308658,3.55242657231642,
0.611815125443492));
#117820=CARTESIAN_POINT('Ctrl Pts',(-7.43287197300667,3.55883456252145,
0.615260145453034));
#117821=CARTESIAN_POINT('Ctrl Pts',(-7.4744351498985,3.56509182660472,0.61872302284527));
#117822=CARTESIAN_POINT('Ctrl Pts',(-7.50052486205555,3.66023518270933,
0.0269335060383855));
#117823=CARTESIAN_POINT('Ctrl Pts',(-7.5004217009998,3.65798000485466,0.0409897622297917));
#117824=CARTESIAN_POINT('Ctrl Pts',(-7.5003185399441,3.655724827,0.0550460184211978));
#117825=CARTESIAN_POINT('Ctrl Pts',(-7.49732166560829,3.590210912,0.463386483204042));
#117826=CARTESIAN_POINT('Ctrl Pts',(-7.4500112758201,3.524902621,0.868988066263494));
#117827=CARTESIAN_POINT('Ctrl Pts',(-7.24694431946642,3.66023518270933,
-0.212217977081353));
#117828=CARTESIAN_POINT('Ctrl Pts',(-7.24729112423315,3.65798000485466,
-0.198635266540677));
#117829=CARTESIAN_POINT('Ctrl Pts',(-7.24763792900001,3.655724827,-0.185052556));
#117830=CARTESIAN_POINT('Ctrl Pts',(-7.257712761,3.590210912,0.209531198));
#117831=CARTESIAN_POINT('Ctrl Pts',(-7.224890305,3.524902621,0.602876501));
#117832=CARTESIAN_POINT('',(-7.49980162322622,3.65572482796921,0.0545548269909637));
#117833=CARTESIAN_POINT('Origin',(0.192912584456805,3.62500082539466,-0.00633279149226233));
#117834=CARTESIAN_POINT('',(-7.3737197555458,3.65572482783619,-0.0652488718236939));
#117835=CARTESIAN_POINT('Origin',(1.24249568966839E-12,3.746853104,-1.76270944455409E-13));
#117836=CARTESIAN_POINT('',(-7.47395492125183,3.7457690389483,0.62449806318162));
#117837=CARTESIAN_POINT('Origin',(0.188738899842835,3.62500689805883,-0.0351415693773142));
#117838=CARTESIAN_POINT('Origin',(0.181748235893762,3.4823217650145,0.0262664429100363));
#117839=CARTESIAN_POINT('Ctrl Pts',(-7.39502008900001,3.524895017,-1.250471066));
#117840=CARTESIAN_POINT('Ctrl Pts',(-7.463353212,3.590632927,-0.846363502));
#117841=CARTESIAN_POINT('Ctrl Pts',(-7.487245287,3.655724827,-0.437216209));
#117842=CARTESIAN_POINT('Ctrl Pts',(-7.48748326518231,3.65637317805554,
-0.433140877364431));
#117843=CARTESIAN_POINT('Ctrl Pts',(-7.48772124336463,3.65702152911109,
-0.429065545728861));
#117844=CARTESIAN_POINT('Ctrl Pts',(-7.184316859,3.524895017,-0.973699783));
#117845=CARTESIAN_POINT('Ctrl Pts',(-7.237525565,3.590632927,-0.581106288000001));
#117846=CARTESIAN_POINT('Ctrl Pts',(-7.24763792900001,3.655724827,-0.185052556));
#117847=CARTESIAN_POINT('Ctrl Pts',(-7.24773865369652,3.65637317805554,
-0.181107643419569));
#117848=CARTESIAN_POINT('Ctrl Pts',(-7.24783937839304,3.65702152911109,
-0.177162730839138));
#117849=CARTESIAN_POINT('',(-7.48724528598708,3.65572482719222,-0.437216209161948));
#117850=CARTESIAN_POINT('',(-7.36744160786082,3.6557248275383,-0.311134385795709));
#117851=CARTESIAN_POINT('',(-7.43269416944146,3.56509183362407,-1.00252498910139));
#117852=CARTESIAN_POINT('Origin',(0.185898731912409,3.48217863734023,0.0384972227116154));
#117853=CARTESIAN_POINT('Ctrl Pts',(-7.18495063902355,3.52567991522723,
-0.969012029225632));
#117854=CARTESIAN_POINT('Ctrl Pts',(-7.22617580481923,3.53257385729222,
-0.974629897902441));
#117855=CARTESIAN_POINT('Ctrl Pts',(-7.26745634979461,3.53929993067353,
-0.980233309912086));
#117856=CARTESIAN_POINT('Ctrl Pts',(-7.35002423646398,3.55242657234091,
-0.991401229939742));
#117857=CARTESIAN_POINT('Ctrl Pts',(-7.39135830107595,3.55883456252679,
-0.996972054680568));
#117858=CARTESIAN_POINT('Ctrl Pts',(-7.43269417014898,3.56509182658403,
-1.00252499176763));
#117859=CARTESIAN_POINT('Ctrl Pts',(-7.33095666743836,3.66023518241854,
-1.58608731454857));
#117860=CARTESIAN_POINT('Ctrl Pts',(-7.3338775975828,3.65798000470928,-1.57233751009812));
#117861=CARTESIAN_POINT('Ctrl Pts',(-7.33679852772727,3.655724827,-1.55858770564767));
#117862=CARTESIAN_POINT('Ctrl Pts',(-7.42165284693166,3.590210912,-1.15914977384803));
#117863=CARTESIAN_POINT('Ctrl Pts',(-7.46264089952596,3.524902621,-0.752860595137903));
#117864=CARTESIAN_POINT('Ctrl Pts',(-7.03189419658587,3.66023518241855,
-1.76513524738259));
#117865=CARTESIAN_POINT('Ctrl Pts',(-7.03515277429293,3.65798000470927,
-1.75194464669127));
#117866=CARTESIAN_POINT('Ctrl Pts',(-7.038411352,3.655724827,-1.738754046));
#117867=CARTESIAN_POINT('Ctrl Pts',(-7.13307448300001,3.590210912,-1.355561232));
#117868=CARTESIAN_POINT('Ctrl Pts',(-7.185577012,3.524902621,-0.964356266));
#117869=CARTESIAN_POINT('',(-7.33618810462917,3.65572482796923,-1.55895629147011));
#117870=CARTESIAN_POINT('Origin',(0.18976414911995,3.62500081621431,0.0352858245829443));
#117871=CARTESIAN_POINT('',(-7.18729970665748,3.65572482783619,-1.64885517145456));
#117872=CARTESIAN_POINT('Origin',(1.38647773817446E-12,3.74685310399989,
1.68756068147369E-13));
#117873=CARTESIAN_POINT('',(-7.43346663204992,3.74576903894809,-0.99678173471832));
#117874=CARTESIAN_POINT('Origin',(0.191880327280147,3.62500693360438,0.00625327433957518));
#117875=CARTESIAN_POINT('Origin',(0.171852892384567,3.48232180857018,0.064722890966695));
#117876=CARTESIAN_POINT('Ctrl Pts',(-6.953314313,3.524895017,-2.810946471));
#117877=CARTESIAN_POINT('Ctrl Pts',(-7.106921026,3.590632927,-2.430976319));
#117878=CARTESIAN_POINT('Ctrl Pts',(-7.21820909200001,3.655724827,-2.036530753));
#117879=CARTESIAN_POINT('Ctrl Pts',(-7.21931758222782,3.65637317805554,
-2.03260185863572));
#117880=CARTESIAN_POINT('Ctrl Pts',(-7.22042607245565,3.65702152911109,
-2.02867296427143));
#117881=CARTESIAN_POINT('Ctrl Pts',(-6.807034852,3.524895017,-2.495350981));
#117882=CARTESIAN_POINT('Ctrl Pts',(-6.943395564,3.590632927,-2.123374403));
#117883=CARTESIAN_POINT('Ctrl Pts',(-7.038411352,3.655724827,-1.738754046));
#117884=CARTESIAN_POINT('Ctrl Pts',(-7.03935776140644,3.65637317805554,
-1.7349230161108));
#117885=CARTESIAN_POINT('Ctrl Pts',(-7.04030417081289,3.65702152911109,
-1.73109198622161));
#117886=CARTESIAN_POINT('',(-7.21820909110468,3.65572482719347,-2.03653075247278));
#117887=CARTESIAN_POINT('',(-7.12831022115529,3.65572482753849,-1.88764240268987));
#117888=CARTESIAN_POINT('',(-7.04340867175693,3.5650918336432,-2.5768960497187));
#117889=CARTESIAN_POINT('Origin',(0.173276962231453,3.48217863691368,0.0775599817067715));
#117890=CARTESIAN_POINT('Ctrl Pts',(-6.80866154308647,3.52567991522762,
-2.49090906827572));
#117891=CARTESIAN_POINT('Ctrl Pts',(-6.84771521166626,3.53257385728763,
-2.50525778638665));
#117892=CARTESIAN_POINT('Ctrl Pts',(-6.88682607244739,3.5392999306626,-2.51960429069231));
#117893=CARTESIAN_POINT('Ctrl Pts',(-6.96506279516603,3.55242657233973,
-2.54826076596736));
#117894=CARTESIAN_POINT('Ctrl Pts',(-7.00423292972117,3.55883456253521,
-2.56258695001126));
#117895=CARTESIAN_POINT('Ctrl Pts',(-7.04340867186995,3.56509182660347,
-2.57689605248768));
#117896=CARTESIAN_POINT('Ctrl Pts',(-6.81860108506758,3.66023518271245,
-3.12494445771658));
#117897=CARTESIAN_POINT('Ctrl Pts',(-6.82440952740602,3.65798000485622,
-3.1121440288865));
#117898=CARTESIAN_POINT('Ctrl Pts',(-6.83021796974439,3.655724827,-3.09934360005647));
#117899=CARTESIAN_POINT('Ctrl Pts',(-6.99895579083881,3.590210912,-2.72748547630777));
#117900=CARTESIAN_POINT('Ctrl Pts',(-7.12632572833151,3.524902621,-2.33950633195554));
#117901=CARTESIAN_POINT('Ctrl Pts',(-6.48804051683436,3.66023518271245,
-3.23551675937307));
#117902=CARTESIAN_POINT('Ctrl Pts',(-6.49405850041722,3.65798000485622,
-3.22333504468654));
#117903=CARTESIAN_POINT('Ctrl Pts',(-6.500076484,3.655724827,-3.21115333));
#117904=CARTESIAN_POINT('Ctrl Pts',(-6.674901571,3.590210912,-2.857269126));
#117905=CARTESIAN_POINT('Ctrl Pts',(-6.810274123,3.524902621,-2.486496806));
#117906=CARTESIAN_POINT('',(-6.8295425829065,3.65572482796921,-3.0995723456306));
#117907=CARTESIAN_POINT('Origin',(0.177741842606053,3.62500083374336,0.0752544236285414));
#117908=CARTESIAN_POINT('',(-6.66480951171505,3.65572482783619,-3.15536283582134));
#117909=CARTESIAN_POINT('Origin',(-1.01915004213637E-12,3.74685310399945,
-3.9942008034366E-13));
#117910=CARTESIAN_POINT('',(-7.04539770494289,3.74576903893068,-2.57145312554884));
#117911=CARTESIAN_POINT('Origin',(0.186050156975672,3.62500693608475,0.0473557262033941));
#117912=CARTESIAN_POINT('Origin',(0.153921800927286,3.48232180130307,0.10015310657206));
#117913=CARTESIAN_POINT('Ctrl Pts',(-6.186479288,3.524895017,-4.239985143));
#117914=CARTESIAN_POINT('Ctrl Pts',(-6.418177113,3.590632927,-3.901919385));
#117915=CARTESIAN_POINT('Ctrl Pts',(-6.611657462,3.655724827,-3.540619381));
#117916=CARTESIAN_POINT('Ctrl Pts',(-6.61358463248514,3.65637317805554,
-3.53702063462816));
#117917=CARTESIAN_POINT('Ctrl Pts',(-6.61551180297026,3.65702152911109,
-3.53342188825632));
#117918=CARTESIAN_POINT('Ctrl Pts',(-6.111463461,3.524895017,-3.90032234));
#117919=CARTESIAN_POINT('Ctrl Pts',(-6.324600105,3.590632927,-3.56635589));
#117920=CARTESIAN_POINT('Ctrl Pts',(-6.500076484,3.655724827,-3.21115333));
#117921=CARTESIAN_POINT('Ctrl Pts',(-6.50182432506083,3.65637317805554,
-3.20761531751753));
#117922=CARTESIAN_POINT('Ctrl Pts',(-6.50357216612167,3.65702152911109,
-3.20407730503506));
#117923=CARTESIAN_POINT('',(-6.61165746100982,3.65572482719223,-3.54061938074149));
#117924=CARTESIAN_POINT('',(-6.55586697148985,3.6557248275383,-3.37588635843267));
#117925=CARTESIAN_POINT('',(-6.32478121320232,3.56509183364413,-4.03077431486429));
#117926=CARTESIAN_POINT('Origin',(0.152552477801926,3.48217864579776,0.112995930087421));
#117927=CARTESIAN_POINT('Ctrl Pts',(-6.11400700101208,3.52567991521301,
-3.89633396802979));
#117928=CARTESIAN_POINT('Ctrl Pts',(-6.14906306633873,3.53257385726894,
-3.91874260539261));
#117929=CARTESIAN_POINT('Ctrl Pts',(-6.18417546266473,3.53929993065058,
-3.94116137533083));
#117930=CARTESIAN_POINT('Ctrl Pts',(-6.25442275923254,3.55242657233169,
-3.98596646072884));
#117931=CARTESIAN_POINT('Ctrl Pts',(-6.28959741171118,3.5588345625289,-4.00837812752732));
#117932=CARTESIAN_POINT('Ctrl Pts',(-6.32478121271705,3.56509182660387,
-4.03077431759362));
#117933=CARTESIAN_POINT('Ctrl Pts',(-5.98741529591276,3.6602351824927,-4.51768266859114));
#117934=CARTESIAN_POINT('Ctrl Pts',(-5.99583965351217,3.65798000474635,
-4.50643015061259));
#117935=CARTESIAN_POINT('Ctrl Pts',(-6.00426401111169,3.655724827,-4.49517763263396));
#117936=CARTESIAN_POINT('Ctrl Pts',(-6.24899534042545,3.590210912,-4.16828698839096));
#117937=CARTESIAN_POINT('Ctrl Pts',(-6.45679148737917,3.524902621,-3.81675935347235));
#117938=CARTESIAN_POINT('Ctrl Pts',(-5.64081327373058,3.6602351824927,-4.55460910073637));
#117939=CARTESIAN_POINT('Ctrl Pts',(-5.64930926836524,3.65798000474635,
-4.5440058768682));
#117940=CARTESIAN_POINT('Ctrl Pts',(-5.657805263,3.655724827,-4.533402653));
#117941=CARTESIAN_POINT('Ctrl Pts',(-5.90461768,3.590210912,-4.225374291));
#117942=CARTESIAN_POINT('Ctrl Pts',(-6.11653038600001,3.524902621,-3.892371519));
#117943=CARTESIAN_POINT('',(-6.00355524095616,3.65572482796921,-4.49525584204769));
#117944=CARTESIAN_POINT('Origin',(0.157409015298306,3.62500080212542,0.111704365062237));
#117945=CARTESIAN_POINT('',(-5.83068023116903,3.65572482783619,-4.5143292409069));
#117946=CARTESIAN_POINT('Origin',(8.11416905888152E-13,3.746853104,4.95046711956881E-13));
#117947=CARTESIAN_POINT('',(-6.32789381133044,3.74576903895181,-4.02588622646399));
#117948=CARTESIAN_POINT('Origin',(0.171520220307716,3.62500688869145,0.0862437827618023));
#117949=CARTESIAN_POINT('Origin',(0.128792829381679,3.48232179096176,0.130899938843843));
#117950=CARTESIAN_POINT('Ctrl Pts',(-5.130371368,3.524895017,-5.470766823));
#117951=CARTESIAN_POINT('Ctrl Pts',(-5.42932637000001,3.590632927,-5.190413038));
#117952=CARTESIAN_POINT('Ctrl Pts',(-5.695952078,3.655724827,-4.87915258300001));
#117953=CARTESIAN_POINT('Ctrl Pts',(-5.69860781641318,3.65637317805554,
-4.87605225800491));
#117954=CARTESIAN_POINT('Ctrl Pts',(-5.70126355482636,3.65702152911109,
-4.87295193300981));
#117955=CARTESIAN_POINT('Ctrl Pts',(-5.130126831,3.524895017,-5.122918962));
#117956=CARTESIAN_POINT('Ctrl Pts',(-5.410073373,3.590632927,-4.84257854));
#117957=CARTESIAN_POINT('Ctrl Pts',(-5.657805263,3.655724827,-4.533402653));
#117958=CARTESIAN_POINT('Ctrl Pts',(-5.66027280861432,3.65637317805554,
-4.53032309144649));
#117959=CARTESIAN_POINT('Ctrl Pts',(-5.66274035422865,3.65702152911109,
-4.52724352989298));
#117960=CARTESIAN_POINT('',(-5.69595207709824,3.65572482719222,-4.87915258250859));
#117961=CARTESIAN_POINT('',(-5.67687866839472,3.6557248275383,-4.70627762053947));
#117962=CARTESIAN_POINT('',(-5.31041401431081,3.56509183366011,-5.29617805336075));
#117963=CARTESIAN_POINT('Origin',(0.124695323616197,3.48217858686857,0.143148643923253));
#117964=CARTESIAN_POINT('Ctrl Pts',(-5.13346828674902,3.52567991526401,
-5.11957062121533));
#117965=CARTESIAN_POINT('Ctrl Pts',(-5.16288756611796,3.53257385730878,
-5.14899137500095));
#117966=CARTESIAN_POINT('Ctrl Pts',(-5.19235968126349,3.53929993068155,
-5.17843413396552));
#117967=CARTESIAN_POINT('Ctrl Pts',(-5.25133286608943,3.55242657235264,
-5.23729279388202));
#117968=CARTESIAN_POINT('Ctrl Pts',(-5.28086730881873,3.55883456254548,
-5.26674199901425));
#117969=CARTESIAN_POINT('Ctrl Pts',(-5.31041401324188,3.56509182661964,
-5.2961780559303));
#117970=CARTESIAN_POINT('Ctrl Pts',(-4.87626462183353,3.6602351825012,-5.69917906100448));
#117971=CARTESIAN_POINT('Ctrl Pts',(-4.88691098140035,3.65798000475061,
-5.69000060847828));
#117972=CARTESIAN_POINT('Ctrl Pts',(-4.89755734096719,3.655724827,-5.68082215595224));
#117973=CARTESIAN_POINT('Ctrl Pts',(-5.20683881358382,3.590210912,-5.4141840346501));
#117974=CARTESIAN_POINT('Ctrl Pts',(-5.4853448518014,3.524902621,-5.11554494931966));
#117975=CARTESIAN_POINT('Ctrl Pts',(-4.52982787051219,3.66023518250122,
-5.6607329833822));
#117976=CARTESIAN_POINT('Ctrl Pts',(-4.54040461325608,3.65798000475061,
-5.65220404469116));
#117977=CARTESIAN_POINT('Ctrl Pts',(-4.550981356,3.655724827,-5.643675106));
#117978=CARTESIAN_POINT('Ctrl Pts',(-4.858240429,3.590210912,-5.39590565));
#117979=CARTESIAN_POINT('Ctrl Pts',(-5.136784486,3.524902621,-5.116243265));
#117980=CARTESIAN_POINT('',(-4.89684832804113,3.65572482796969,-5.68074617259837));
#117981=CARTESIAN_POINT('Origin',(0.129715678256187,3.62500078845805,0.14293098103293));
#117982=CARTESIAN_POINT('',(-4.72391482347484,3.65572482783619,-5.66221062818384));
#117983=CARTESIAN_POINT('Origin',(1.27415439310496E-12,3.74685310400078,
1.28065960613988E-12));
#117984=CARTESIAN_POINT('',(-5.31450463647661,3.74576903894741,-5.29207336199999));
#117985=CARTESIAN_POINT('Origin',(0.148970427180682,3.62500693028495,0.121099350128863));
#117986=CARTESIAN_POINT('Origin',(0.0976423688931122,3.48232175760876,0.155526501769297));
#117987=CARTESIAN_POINT('Ctrl Pts',(-3.834372984,3.524895017,-6.445741526));
#117988=CARTESIAN_POINT('Ctrl Pts',(-4.186606361,3.590632927,-6.236208745));
#117989=CARTESIAN_POINT('Ctrl Pts',(-4.513910305,3.655724827,-5.989542033));
#117990=CARTESIAN_POINT('Ctrl Pts',(-4.51717043195245,3.65637317805554,
-5.98708509714327));
#117991=CARTESIAN_POINT('Ctrl Pts',(-4.52043055890489,3.65702152911109,
-5.98462816128654));
#117992=CARTESIAN_POINT('Ctrl Pts',(-3.908911172,3.524895017,-6.105973587));
#117993=CARTESIAN_POINT('Ctrl Pts',(-4.242577624,3.590632927,-5.892367599));
#117994=CARTESIAN_POINT('Ctrl Pts',(-4.550981356,3.655724827,-5.643675106));
#117995=CARTESIAN_POINT('Ctrl Pts',(-4.55405322646585,3.65637317805554,
-5.64119799225248));
#117996=CARTESIAN_POINT('Ctrl Pts',(-4.5571250969317,3.65702152911109,-5.63872087850496));
#117997=CARTESIAN_POINT('',(-4.51391030460831,3.65572482719341,-5.98954203202406));
#117998=CARTESIAN_POINT('',(-4.53244582789803,3.6557248275383,-5.81660857152752));
#117999=CARTESIAN_POINT('',(-4.04773775792123,3.5650918336188,-6.31393839137917));
#118000=CARTESIAN_POINT('Origin',(0.0910073196940303,3.48217860516275,0.16660777581755));
#118001=CARTESIAN_POINT('Ctrl Pts',(-3.91289430058519,3.52567991523439,
-6.10342184256814));
#118002=CARTESIAN_POINT('Ctrl Pts',(-3.93530118122091,3.53257385728072,
-6.13847903075732));
#118003=CARTESIAN_POINT('Ctrl Pts',(-3.95775493185482,3.53929993065187,
-6.17356906780972));
#118004=CARTESIAN_POINT('Ctrl Pts',(-4.00269648435988,3.55242657232069,
-6.24372913625754));
#118005=CARTESIAN_POINT('Ctrl Pts',(-4.02520971961444,3.5588345625106,-6.27883886740677));
#118006=CARTESIAN_POINT('Ctrl Pts',(-4.04773775635048,3.56509182657902,
-6.31393839364233));
#118007=CARTESIAN_POINT('Ctrl Pts',(-3.53710523200821,3.66023518267594,
-6.61418817373702));
#118008=CARTESIAN_POINT('Ctrl Pts',(-3.54947578204589,3.65798000483796,
-6.60751296069411));
#118009=CARTESIAN_POINT('Ctrl Pts',(-3.56184633208361,3.655724827,-6.60083774765122));
#118010=CARTESIAN_POINT('Ctrl Pts',(-3.92121628953467,3.590210912,-6.40691985233655));
#118011=CARTESIAN_POINT('Ctrl Pts',(-4.25740958765534,3.524902621,-6.17513334797329));
#118012=CARTESIAN_POINT('Ctrl Pts',(-3.20703274994005,3.66023518267593,
-6.50216728302699));
#118013=CARTESIAN_POINT('Ctrl Pts',(-3.21919568447,3.65798000483796,-6.49611143301358));
#118014=CARTESIAN_POINT('Ctrl Pts',(-3.231358619,3.655724827,-6.490055583));
#118015=CARTESIAN_POINT('Ctrl Pts',(-3.584697254,3.590210912,-6.314130458));
#118016=CARTESIAN_POINT('Ctrl Pts',(-3.916848252,3.524902621,-6.10088516300001));
#118017=CARTESIAN_POINT('',(-3.56117022965222,3.65572482796966,-6.60061112390672));
#118018=CARTESIAN_POINT('Origin',(0.095957020842885,3.62500083064261,0.167474319064722));
#118019=CARTESIAN_POINT('',(-3.39626440859483,3.6557248278362,-6.54533333861582));
#118020=CARTESIAN_POINT('Origin',(7.66530935947252E-13,3.74685310400089,
1.24769986009632E-12));
#118021=CARTESIAN_POINT('',(-4.05261513061144,3.74576903895328,-6.31080902873435));
#118022=CARTESIAN_POINT('Origin',(0.119454723690957,3.62500693046372,0.150292257934594));
#118023=CARTESIAN_POINT('Origin',(0.0619259432285724,3.48232178816845,0.17288060055575));
#118024=CARTESIAN_POINT('Ctrl Pts',(-2.359083581,3.524895017,-7.11932051900001));
#118025=CARTESIAN_POINT('Ctrl Pts',(-2.748125292,3.590632927,-6.99040626299999));
#118026=CARTESIAN_POINT('Ctrl Pts',(-3.120803103,3.655724827,-6.81986715399999));
#118027=CARTESIAN_POINT('Ctrl Pts',(-3.12451517857529,3.65637317805554,
-6.81816849085863));
#118028=CARTESIAN_POINT('Ctrl Pts',(-3.12822725415059,3.65702152911109,
-6.81646982771726));
#118029=CARTESIAN_POINT('Ctrl Pts',(-2.504919172,3.524895017,-6.803519673));
#118030=CARTESIAN_POINT('Ctrl Pts',(-2.87670366,3.590632927,-6.66663609900001));
#118031=CARTESIAN_POINT('Ctrl Pts',(-3.231358619,3.655724827,-6.490055583));
#118032=CARTESIAN_POINT('Ctrl Pts',(-3.23489117707591,3.65637317805554,
-6.48829674412854));
#118033=CARTESIAN_POINT('Ctrl Pts',(-3.23842373515182,3.65702152911109,
-6.48653790525709));
#118034=CARTESIAN_POINT('',(-3.12080310282607,3.65572482719341,-6.81986715296628));
#118035=CARTESIAN_POINT('',(-3.17608085802301,3.6557248275383,-6.65496136992077));
#118036=CARTESIAN_POINT('',(-2.59579378301225,3.56509183361683,-7.03646598849934));
#118037=CARTESIAN_POINT('Origin',(0.0530637683764096,3.48217861931808,0.182276192629589));
#118038=CARTESIAN_POINT('Ctrl Pts',(-2.50935772659468,3.52567991518581,
-6.80188384193689));
#118039=CARTESIAN_POINT('Ctrl Pts',(-2.52370448737854,3.53257385723308,
-6.84093822952236));
#118040=CARTESIAN_POINT('Ctrl Pts',(-2.53808996089894,3.53929993059772,
-6.88003477361846));
#118041=CARTESIAN_POINT('Ctrl Pts',(-2.56689846389596,3.55242657228965,
-6.9582156441211));
#118042=CARTESIAN_POINT('Ctrl Pts',(-2.5813377978392,3.55883456249658,-6.99734420948112));
#118043=CARTESIAN_POINT('Ctrl Pts',(-2.59579378099291,3.56509182657663,
-7.03646599037154));
#118044=CARTESIAN_POINT('Ctrl Pts',(-2.0325547345735,3.66023518250409,-7.21992519859157));
#118045=CARTESIAN_POINT('Ctrl Pts',(-2.04607104101206,3.65798000475204,
-7.21606535104289));
#118046=CARTESIAN_POINT('Ctrl Pts',(-2.05958734745061,3.655724827,-7.21220550349425));
#118047=CARTESIAN_POINT('Ctrl Pts',(-2.45224205075605,3.590210912,-7.10007521842663));
#118048=CARTESIAN_POINT('Ctrl Pts',(-2.83040258307706,3.524902621,-6.94597937575816));
#118049=CARTESIAN_POINT('Ctrl Pts',(-1.73428034373308,3.66023518250408,
-7.03956746721845));
#118050=CARTESIAN_POINT('Ctrl Pts',(-1.74746074386651,3.65798000475204,
-7.03626787110924));
#118051=CARTESIAN_POINT('Ctrl Pts',(-1.760641144,3.655724827,-7.032968275));
#118052=CARTESIAN_POINT('Ctrl Pts',(-2.14353762,3.590210912,-6.937113543));
#118053=CARTESIAN_POINT('Ctrl Pts',(-2.513764547,3.524902621,-6.800256451));
#118054=CARTESIAN_POINT('',(-2.05897576934496,3.65572482796967,-7.21183883606633));
#118055=CARTESIAN_POINT('Origin',(0.0577116199150312,3.62500080581228,0.184186927122787));
#118056=CARTESIAN_POINT('',(-1.90980844449988,3.65572482783619,-7.12240353765932));
#118057=CARTESIAN_POINT('Origin',(1.07986536379556E-13,3.74685310400033,
2.95336671785051E-13));
#118058=CARTESIAN_POINT('',(-2.60122984621702,3.74576903893663,-7.03445827951591));
#118059=CARTESIAN_POINT('Origin',(0.0843535976532561,3.62500687597838,0.172457830982561));
#118060=CARTESIAN_POINT('Origin',(0.0233139335965546,3.48232177458421,0.182151020955458));
#118061=CARTESIAN_POINT('Ctrl Pts',(-0.773486052000001,3.524895017,-7.460007998));
#118062=CARTESIAN_POINT('Ctrl Pts',(-1.181144938,3.590632927,-7.417740153));
#118063=CARTESIAN_POINT('Ctrl Pts',(-1.581770616,3.655724827,-7.33130286600001));
#118064=CARTESIAN_POINT('Ctrl Pts',(-1.58576106767231,3.65637317805554,
-7.3304419031726));
#118065=CARTESIAN_POINT('Ctrl Pts',(-1.58975151934463,3.65702152911109,
-7.3295809403452));
#118066=CARTESIAN_POINT('Ctrl Pts',(-0.983799934,3.524895017,-7.182940741));
#118067=CARTESIAN_POINT('Ctrl Pts',(-1.37631823,3.590632927,-7.129180104));
#118068=CARTESIAN_POINT('Ctrl Pts',(-1.760641144,3.655724827,-7.032968275));
#118069=CARTESIAN_POINT('Ctrl Pts',(-1.76446921119364,3.65637317805554,
-7.03200995236865));
#118070=CARTESIAN_POINT('Ctrl Pts',(-1.76829727838728,3.65702152911109,
-7.03105162973729));
#118071=CARTESIAN_POINT('',(-1.58177061555191,3.65572482719222,-7.33130286508043));
#118072=CARTESIAN_POINT('',(-1.67120587678719,3.6557248275383,-7.18213557124759));
#118073=CARTESIAN_POINT('',(-1.02247337587459,3.56509183364358,-7.42997625638912));
#118074=CARTESIAN_POINT('Origin',(0.0126391814059199,3.48217861389325,0.189421790792401));
#118075=CARTESIAN_POINT('Ctrl Pts',(-0.988486372994223,3.52567991519632,
-7.18229731285625));
#118076=CARTESIAN_POINT('Ctrl Pts',(-0.994102175902777,3.53257385726828,
-7.22352276015149));
#118077=CARTESIAN_POINT('Ctrl Pts',(-0.999746723952424,3.53929993065635,
-7.26479770048792));
#118078=CARTESIAN_POINT('Ctrl Pts',(-1.0110751242192,3.55242657234039,-7.3473437222239));
#118079=CARTESIAN_POINT('Ctrl Pts',(-1.01676538966102,3.55883456253443,
-7.38866151338171));
#118080=CARTESIAN_POINT('Ctrl Pts',(-1.02247337348076,3.56509182660379,
-7.42997625778604));
#118081=CARTESIAN_POINT('Ctrl Pts',(-0.432964236225081,3.66023518261545,
-7.48806654611535));
#118082=CARTESIAN_POINT('Ctrl Pts',(-0.446994292381468,3.65798000480772,
-7.48720254598314));
#118083=CARTESIAN_POINT('Ctrl Pts',(-0.461024348537847,3.655724827,-7.48633854585082));
#118084=CARTESIAN_POINT('Ctrl Pts',(-0.868603699188754,3.590210912,-7.4612389590092));
#118085=CARTESIAN_POINT('Ctrl Pts',(-1.27104909975372,3.524902621,-7.39203912715354));
#118086=CARTESIAN_POINT('Ctrl Pts',(-0.180434915674636,3.66023518261545,
-7.24780530097854));
#118087=CARTESIAN_POINT('Ctrl Pts',(-0.194016481337319,3.65798000480772,
-7.24741624398922));
#118088=CARTESIAN_POINT('Ctrl Pts',(-0.207598047,3.655724827,-7.247027187));
#118089=CARTESIAN_POINT('Ctrl Pts',(-0.60214855,3.590210912,-7.23572490900001));
#118090=CARTESIAN_POINT('Ctrl Pts',(-0.993140006000001,3.524902621,-7.181655306));
#118091=CARTESIAN_POINT('',(-0.460505891419481,3.65572482796966,-7.48584897967103));
#118092=CARTESIAN_POINT('Origin',(0.0167675994576022,3.62500082997759,0.192286946163568));
#118093=CARTESIAN_POINT('',(-0.334051961171194,3.65572482783619,-7.3664380632655));
#118094=CARTESIAN_POINT('Origin',(1.43006266550838E-13,3.74685310400067,
5.2952434104192E-13));
#118095=CARTESIAN_POINT('',(-1.02821394480032,3.74576903896483,-7.42918407892651));
#118096=CARTESIAN_POINT('Origin',(0.0453081133289925,3.62500687504689,0.186559308707741));
#118097=CARTESIAN_POINT('Origin',(-0.0163882141384704,3.48232176110686,
0.182904204562684));
#118098=CARTESIAN_POINT('Ctrl Pts',(0.848278826,3.524895017,-7.451873793));
#118099=CARTESIAN_POINT('Ctrl Pts',(0.44106444,3.590632927,-7.49822875700001));
#118100=CARTESIAN_POINT('Ctrl Pts',(0.031223706,3.655724827,-7.499935005));
#118101=CARTESIAN_POINT('Ctrl Pts',(0.027141467311413,3.65637317805554,
-7.49995200016671));
#118102=CARTESIAN_POINT('Ctrl Pts',(0.0230592286228261,3.65702152911109,
-7.49996899533341));
#118103=CARTESIAN_POINT('Ctrl Pts',(0.583320695,3.524895017,-7.226495483));
#118104=CARTESIAN_POINT('Ctrl Pts',(0.188422311,3.590632927,-7.25837157));
#118105=CARTESIAN_POINT('Ctrl Pts',(-0.207598047,3.655724827,-7.247027187));
#118106=CARTESIAN_POINT('Ctrl Pts',(-0.21154262715707,3.65637317805554,
-7.24691419071793));
#118107=CARTESIAN_POINT('Ctrl Pts',(-0.215487207314141,3.65702152911109,
-7.24680119443587));
#118108=CARTESIAN_POINT('',(0.0312237062235909,3.65572482719222,-7.49993500399947));
#118109=CARTESIAN_POINT('',(-0.0881871672015895,3.6557248275383,-7.37348109603945));
#118110=CARTESIAN_POINT('',(0.59865674998268,3.56509183372456,-7.47606909195671));
#118111=CARTESIAN_POINT('Origin',(-0.0283764114982865,3.48217863417679,
0.187710425900819));
#118112=CARTESIAN_POINT('Ctrl Pts',(0.578605504166122,3.52567991521001,
-7.22687454364312));
#118113=CARTESIAN_POINT('Ctrl Pts',(0.581983248302078,3.53257385729805,
-7.26834339445086));
#118114=CARTESIAN_POINT('Ctrl Pts',(0.585343558783091,3.53929993070054,
-7.30986676056336));
#118115=CARTESIAN_POINT('Ctrl Pts',(0.592024964821285,3.55242657240916,
-7.3929181733487));
#118116=CARTESIAN_POINT('Ctrl Pts',(0.595349838307345,3.55883456261099,
-7.43449321637042));
#118117=CARTESIAN_POINT('Ctrl Pts',(0.598656752679924,3.56509182668411,
-7.47606909280178));
#118118=CARTESIAN_POINT('Ctrl Pts',(1.18687118926983,3.66023518255067,-7.4060742236875));
#118119=CARTESIAN_POINT('Ctrl Pts',(1.17298341369048,3.65798000477534,-7.40824647072547));
#118120=CARTESIAN_POINT('Ctrl Pts',(1.15909563811114,3.655724827,-7.41041871776356));
#118121=CARTESIAN_POINT('Ctrl Pts',(0.755649595500152,3.590210912,-7.47352345804971));
#118122=CARTESIAN_POINT('Ctrl Pts',(0.3477372264216,3.524902621,-7.49245534442631));
#118123=CARTESIAN_POINT('Ctrl Pts',(1.38184744851904,3.66023518255067,-7.11714381383192));
#118124=CARTESIAN_POINT('Ctrl Pts',(1.36849977675952,3.65798000477534,-7.11968348791595));
#118125=CARTESIAN_POINT('Ctrl Pts',(1.355152105,3.655724827,-7.122223162));
#118126=CARTESIAN_POINT('Ctrl Pts',(0.967396318,3.590210912,-7.196001821));
#118127=CARTESIAN_POINT('Ctrl Pts',(0.573922658000001,3.524902621,-7.22724794000001));
#118128=CARTESIAN_POINT('',(1.15949673172118,3.65572482796968,-7.40982914442963));
#118129=CARTESIAN_POINT('Origin',(-0.0249604152249596,3.62500078965105,
0.191395883719061));
#118130=CARTESIAN_POINT('',(1.25732442189929,3.65572482783619,-7.26602613188263));
#118131=CARTESIAN_POINT('Origin',(-3.67934171628323E-14,3.74685310399933,
-1.82145964977565E-13));
#118132=CARTESIAN_POINT('',(0.59288009775944,3.74576903896458,-7.47652948820546));
#118133=CARTESIAN_POINT('Origin',(0.0041440898913598,3.62500689541319,0.191937658093946));
#118134=CARTESIAN_POINT('Origin',(-0.0553240300614782,3.48232179305368,
0.175104735946446));
#118135=CARTESIAN_POINT('Ctrl Pts',(2.430379128,3.524895017,-7.095298253));
#118136=CARTESIAN_POINT('Ctrl Pts',(2.042650135,3.590632927,-7.228108519));
#118137=CARTESIAN_POINT('Ctrl Pts',(1.642758043,3.655724827,-7.31787851900001));
#118138=CARTESIAN_POINT('Ctrl Pts',(1.63877489824694,3.65637317805554,-7.31877267747834));
#118139=CARTESIAN_POINT('Ctrl Pts',(1.63479175349388,3.65702152911109,-7.31966683595668));
#118140=CARTESIAN_POINT('Ctrl Pts',(2.123165896,3.524895017,-6.932147328));
#118141=CARTESIAN_POINT('Ctrl Pts',(1.744352434,3.590632927,-7.048169649));
#118142=CARTESIAN_POINT('Ctrl Pts',(1.355152105,3.655724827,-7.122223162));
#118143=CARTESIAN_POINT('Ctrl Pts',(1.35127545607555,3.65637317805554,-7.12296077564041));
#118144=CARTESIAN_POINT('Ctrl Pts',(1.34739880715111,3.65702152911109,-7.12369838928082));
#118145=CARTESIAN_POINT('',(1.64275804250961,3.65572482719341,-7.31787851806958));
#118146=CARTESIAN_POINT('',(1.49895507722978,3.6557248275383,-7.22005083982947));
#118147=CARTESIAN_POINT('',(2.19179435121699,3.56509183362882,-7.17258924590931));
#118148=CARTESIAN_POINT('Origin',(-0.0680652196647022,3.48217863853533,
0.177221885982551));
#118149=CARTESIAN_POINT('Ctrl Pts',(2.11864243056491,3.52567991520743,-6.93353115305763));
#118150=CARTESIAN_POINT('Ctrl Pts',(2.13085578201956,3.53257385728076,-6.97330436997477));
#118151=CARTESIAN_POINT('Ctrl Pts',(2.14306382660055,3.5392999306645,-7.0131345753751));
#118152=CARTESIAN_POINT('Ctrl Pts',(2.16744262385646,3.55242657234158,-7.09280798740711));
#118153=CARTESIAN_POINT('Ctrl Pts',(2.17962716896065,3.55883456253058,-7.13269627949745));
#118154=CARTESIAN_POINT('Ctrl Pts',(2.19179435396591,3.56509182658866,-7.17258924617516));
#118155=CARTESIAN_POINT('Ctrl Pts',(2.7512098358553,3.66023518259726,-6.97778210206156));
#118156=CARTESIAN_POINT('Ctrl Pts',(2.73811371755116,3.65798000479863,-6.98288902444044));
#118157=CARTESIAN_POINT('Ctrl Pts',(2.725017599247,3.655724827,-6.98799594681922));
#118158=CARTESIAN_POINT('Ctrl Pts',(2.34456955567036,3.590210912,-7.13635430634087));
#118159=CARTESIAN_POINT('Ctrl Pts',(1.95026374733726,3.524902621,-7.24253267697325));
#118160=CARTESIAN_POINT('Ctrl Pts',(2.87951616181174,3.66023518259726,-6.65369259232325));
#118161=CARTESIAN_POINT('Ctrl Pts',(2.86702650590587,3.65798000479863,-6.65904224516163));
#118162=CARTESIAN_POINT('Ctrl Pts',(2.85453685,3.655724827,-6.664391898));
#118163=CARTESIAN_POINT('Ctrl Pts',(2.491706808,3.590210912,-6.819801685));
#118164=CARTESIAN_POINT('Ctrl Pts',(2.114149336,3.524902621,-6.934902493));
#118165=CARTESIAN_POINT('',(2.7252825740502,3.65572482796922,-6.9873339345461));
#118166=CARTESIAN_POINT('Origin',(-0.065521295201377,3.62500080738625,0.181555350276441));
#118167=CARTESIAN_POINT('',(2.78990971120828,3.65572482783619,-6.8258628944585));
#118168=CARTESIAN_POINT('Origin',(-3.50630982581812E-13,3.746853104,9.64506252643105E-13));
#118169=CARTESIAN_POINT('',(2.18625172566659,3.74576903899511,-7.17428068773578));
#118170=CARTESIAN_POINT('Origin',(-0.0372137556890989,3.62500689313507,
0.188341216217426));
#118171=CARTESIAN_POINT('Origin',(-0.0916730539911931,3.48232175921621,
0.159118208518176));
#118172=CARTESIAN_POINT('Ctrl Pts',(3.898837603,3.524895017,-6.40695445200001));
#118173=CARTESIAN_POINT('Ctrl Pts',(3.54872378,3.590632927,-6.62000996));
#118174=CARTESIAN_POINT('Ctrl Pts',(3.177478839,3.655724827,-6.793646166));
#118175=CARTESIAN_POINT('Ctrl Pts',(3.17378103559647,3.65637317805554,-6.7953756779276));
#118176=CARTESIAN_POINT('Ctrl Pts',(3.17008323219293,3.65702152911109,-6.79710518985521));
#118177=CARTESIAN_POINT('Ctrl Pts',(3.56373422,3.524895017,-6.313659668));
#118178=CARTESIAN_POINT('Ctrl Pts',(3.218718575,3.590632927,-6.508403149));
#118179=CARTESIAN_POINT('Ctrl Pts',(2.85453685,3.655724827,-6.664391898));
#118180=CARTESIAN_POINT('Ctrl Pts',(2.85090940010511,3.65637317805554,-6.66594563156849));
#118181=CARTESIAN_POINT('Ctrl Pts',(2.84728195021021,3.65702152911109,-6.66749936513699));
#118182=CARTESIAN_POINT('',(3.17747883877563,3.65572482719221,-6.7936461649991));
#118183=CARTESIAN_POINT('',(3.01600784751012,3.6557248275383,-6.72901903065084));
#118184=CARTESIAN_POINT('',(3.68244608528429,3.5650918335834,-6.53372709883351));
#118185=CARTESIAN_POINT('Origin',(-0.104571314098206,3.4821786308546,0.158446455861564));
#118186=CARTESIAN_POINT('Ctrl Pts',(3.55961399212263,3.52567991522661,-6.31598355143909));
#118187=CARTESIAN_POINT('Ctrl Pts',(3.58009186818585,3.53257385728007,-6.35220138326043));
#118188=CARTESIAN_POINT('Ctrl Pts',(3.60057681230707,3.53929993065276,-6.38847601200459));
#118189=CARTESIAN_POINT('Ctrl Pts',(3.64151307537039,3.55242657230514,-6.46104598330199));
#118190=CARTESIAN_POINT('Ctrl Pts',(3.66198755634127,3.55883456248648,-6.49738239230802));
#118191=CARTESIAN_POINT('Ctrl Pts',(3.68244608799738,3.56509182654294,-6.53372709851843));
#118192=CARTESIAN_POINT('Ctrl Pts',(4.18690496959621,3.66023518258216,-6.22321664433177));
#118193=CARTESIAN_POINT('Ctrl Pts',(4.17521286864247,3.65798000479108,-6.23101944800773));
#118194=CARTESIAN_POINT('Ctrl Pts',(4.16352076768874,3.655724827,-6.2388222516838));
#118195=CARTESIAN_POINT('Ctrl Pts',(3.82386004954764,3.590210912,-6.46549715900866));
#118196=CARTESIAN_POINT('Ctrl Pts',(3.46159810317059,3.524902621,-6.65395723145168));
#118197=CARTESIAN_POINT('Ctrl Pts',(4.24254189986292,3.66023518258215,-5.87912210056792));
#118198=CARTESIAN_POINT('Ctrl Pts',(4.23149426243145,3.65798000479108,-5.887031588284));
#118199=CARTESIAN_POINT('Ctrl Pts',(4.220446625,3.655724827,-5.894941076));
#118200=CARTESIAN_POINT('Ctrl Pts',(3.899507858,3.590210912,-6.124715202));
#118201=CARTESIAN_POINT('Ctrl Pts',(3.555520741,3.524902621,-6.318288713));
#118202=CARTESIAN_POINT('',(4.1636372344602,3.65572482796924,-6.23811875514344));
#118203=CARTESIAN_POINT('Origin',(-0.103018465060341,3.62500078945646,0.16322552726801));
#118204=CARTESIAN_POINT('',(4.19204192424133,3.65572482783619,-6.06652989444278));
#118205=CARTESIAN_POINT('Origin',(1.70219741080224E-13,3.74685310400067,
-4.30645102911242E-13));
#118206=CARTESIAN_POINT('',(3.67739665309663,3.74576903894327,-6.53657049634743));
#118207=CARTESIAN_POINT('Origin',(-0.0768314298786682,3.62500687472217,
0.175937908449575));
#118208=CARTESIAN_POINT('Origin',(-0.123735352695494,3.48232183506359,0.135690896681645));
#118209=CARTESIAN_POINT('Ctrl Pts',(5.184990765,3.524895017,-5.419028581));
#118210=CARTESIAN_POINT('Ctrl Pts',(4.888863046,3.590632927,-5.702367093));
#118211=CARTESIAN_POINT('Ctrl Pts',(4.56362425700001,3.655724827,-5.951750469));
#118212=CARTESIAN_POINT('Ctrl Pts',(4.56038470012501,3.65637317805554,-5.95423446432146));
#118213=CARTESIAN_POINT('Ctrl Pts',(4.55714514325,3.65702152911109,-5.95671845964291));
#118214=CARTESIAN_POINT('Ctrl Pts',(4.837666293,3.524895017,-5.3999523));
#118215=CARTESIAN_POINT('Ctrl Pts',(4.542581014,3.590632927,-5.664310951));
#118216=CARTESIAN_POINT('Ctrl Pts',(4.220446625,3.655724827,-5.894941076));
#118217=CARTESIAN_POINT('Ctrl Pts',(4.21723798965313,3.65637317805554,-5.89723827864709));
#118218=CARTESIAN_POINT('Ctrl Pts',(4.21402935430626,3.65702152911109,-5.89953548129418));
#118219=CARTESIAN_POINT('',(4.56362425617658,3.65572482719341,-5.95175046836352));
#118220=CARTESIAN_POINT('',(4.39203544364972,3.6557248275383,-5.92334577053529));
#118221=CARTESIAN_POINT('',(5.00091073256986,3.56509183364167,-5.5893551342245));
#118222=CARTESIAN_POINT('Origin',(-0.136187625454915,3.48217863687975,0.13226210935372));
#118223=CARTESIAN_POINT('Ctrl Pts',(4.83414195973404,3.52567991526989,-5.40310757969719));
#118224=CARTESIAN_POINT('Ctrl Pts',(4.86192683761031,3.53257385730368,-5.43407652037869));
#118225=CARTESIAN_POINT('Ctrl Pts',(4.88973082787118,3.53929993065564,-5.46509941075241));
#118226=CARTESIAN_POINT('Ctrl Pts',(4.94531042240983,3.55242657232849,-5.52717264983697));
#118227=CARTESIAN_POINT('Ctrl Pts',(4.97311747519163,3.55883456253002,-5.5582581256464));
#118228=CARTESIAN_POINT('Ctrl Pts',(5.00091073518349,3.56509182660111,-5.58935513330523));
#118229=CARTESIAN_POINT('Ctrl Pts',(5.42682507887805,3.66023518234146,-5.17766049455861));
#118230=CARTESIAN_POINT('Ctrl Pts',(5.41708370537352,3.65798000467073,-5.18779432855361));
#118231=CARTESIAN_POINT('Ctrl Pts',(5.40734233186913,3.655724827,-5.19792816254849));
#118232=CARTESIAN_POINT('Ctrl Pts',(5.1243510961745,3.590210912,-5.49232055015615));
#118233=CARTESIAN_POINT('Ctrl Pts',(4.8110719779955,3.524902621,-5.75425014158161));
#118234=CARTESIAN_POINT('Ctrl Pts',(5.40719109246663,3.66023518234146,-4.82965039351245));
#118235=CARTESIAN_POINT('Ctrl Pts',(5.3981020492333,3.65798000467073,-4.83974987675623));
#118236=CARTESIAN_POINT('Ctrl Pts',(5.389013006,3.655724827,-4.84984936));
#118237=CARTESIAN_POINT('Ctrl Pts',(5.124972255,3.590210912,-5.143243843));
#118238=CARTESIAN_POINT('Ctrl Pts',(4.830639948,3.524902621,-5.406238775));
#118239=CARTESIAN_POINT('',(5.40730484475352,3.65572482796924,-5.1972160764868));
#118240=CARTESIAN_POINT('Origin',(-0.135698834732586,3.62500078415649,0.137263720372715));
#118241=CARTESIAN_POINT('',(5.39815891547351,3.65572482783619,-5.02353269878948));
#118242=CARTESIAN_POINT('Origin',(-6.48352899146332E-13,3.74685310400033,
7.49834222490975E-13));
#118243=CARTESIAN_POINT('',(4.99659059976157,3.7457690389762,-5.59321753308891));
#118244=CARTESIAN_POINT('Origin',(-0.112856569653407,3.62500690610598,0.155308033448146));
#118245=CARTESIAN_POINT('Origin',(-0.150011969543891,3.48232183530511,0.105919035512763));
#118246=CARTESIAN_POINT('Ctrl Pts',(6.228699522,3.524895017,-4.177714957));
#118247=CARTESIAN_POINT('Ctrl Pts',(6.000404509,3.590632927,-4.518087878));
#118248=CARTESIAN_POINT('Ctrl Pts',(5.736379676,3.655724827,-4.831557535));
#118249=CARTESIAN_POINT('Ctrl Pts',(5.73374984372955,3.65637317805554,-4.83467986485974));
#118250=CARTESIAN_POINT('Ctrl Pts',(5.73112001145909,3.65702152911109,-4.83780219471947));
#118251=CARTESIAN_POINT('Ctrl Pts',(5.885394466,3.524895017,-4.233749163));
#118252=CARTESIAN_POINT('Ctrl Pts',(5.654037413,3.590632927,-4.555361869));
#118253=CARTESIAN_POINT('Ctrl Pts',(5.389013006,3.655724827,-4.84984936));
#118254=CARTESIAN_POINT('Ctrl Pts',(5.3863732174238,3.65637317805554,-4.8527826170663));
#118255=CARTESIAN_POINT('Ctrl Pts',(5.38373342884759,3.65702152911109,-4.85571587413261));
#118256=CARTESIAN_POINT('',(5.73637967537562,3.65572482719222,-4.83155753418609));
#118257=CARTESIAN_POINT('',(5.56269634316541,3.6557248275383,-4.84070344501162));
#118258=CARTESIAN_POINT('',(6.08553835246286,3.56509183360283,-4.38363113539836));
#118259=CARTESIAN_POINT('Origin',(-0.161436092508902,3.48217862844388,0.099893592570503));
#118260=CARTESIAN_POINT('Ctrl Pts',(5.88263082197757,3.52567991525343,-4.23758830135811));
#118261=CARTESIAN_POINT('Ctrl Pts',(5.91642351169788,3.53257385731059,-4.26186027829801));
#118262=CARTESIAN_POINT('Ctrl Pts',(5.95024646463923,3.5392999306834,-4.28618083490518));
#118263=CARTESIAN_POINT('Ctrl Pts',(6.0178705506578,3.55242657233255,-4.33485486628895));
#118264=CARTESIAN_POINT('Ctrl Pts',(6.05170994837978,3.5588345625107,-4.35923588648579));
#118265=CARTESIAN_POINT('Ctrl Pts',(6.08553835480099,3.56509182656289,-4.38363113396183));
#118266=CARTESIAN_POINT('Ctrl Pts',(6.41299288018051,3.66023518264005,-3.89000269152138));
#118267=CARTESIAN_POINT('Ctrl Pts',(6.40565772889045,3.65798000482003,-3.90199371024413));
#118268=CARTESIAN_POINT('Ctrl Pts',(6.39832257760057,3.655724827,-3.91398472896682));
#118269=CARTESIAN_POINT('Ctrl Pts',(6.18523318223122,3.590210912,-4.26232913639525));
#118270=CARTESIAN_POINT('Ctrl Pts',(5.93558547476414,3.524902621,-4.58548070971702));
#118271=CARTESIAN_POINT('Ctrl Pts',(6.31900604215917,3.66023518264005,-3.55434960027559));
#118272=CARTESIAN_POINT('Ctrl Pts',(6.31230058557958,3.65798000482002,-3.56616683963779));
#118273=CARTESIAN_POINT('Ctrl Pts',(6.305595129,3.655724827,-3.577984079));
#118274=CARTESIAN_POINT('Ctrl Pts',(6.11079864400001,3.590210912,-3.921280119));
#118275=CARTESIAN_POINT('Ctrl Pts',(5.8798838,3.524902621,-4.241399121));
#118276=CARTESIAN_POINT('',(6.39813288944175,3.65572482796921,-3.91329734966681));
#118277=CARTESIAN_POINT('Origin',(-0.162033723642388,3.625000821317,0.104883187102724));
#118278=CARTESIAN_POINT('',(6.35186399537058,3.65572482783619,-3.74564069745897));
#118279=CARTESIAN_POINT('Origin',(-1.09504419421036E-12,3.74685310400022,
8.21391565875018E-13));
#118280=CARTESIAN_POINT('',(6.08214952370044,3.74576903895158,-4.38833193457553));
#118281=CARTESIAN_POINT('Origin',(-0.143604888526815,3.62500691428628,0.127416356990091));
#118282=CARTESIAN_POINT('Origin',(-0.169274007653364,3.48232181604004,0.0711943981419716));
#118283=CARTESIAN_POINT('Ctrl Pts',(6.981161212,3.524895017,-2.741056025));
#118284=CARTESIAN_POINT('Ctrl Pts',(6.831373726,3.590632927,-3.122547895));
#118285=CARTESIAN_POINT('Ctrl Pts',(6.640908357,3.655724827,-3.485446341));
#118286=CARTESIAN_POINT('Ctrl Pts',(6.63901121737071,3.65637317805554,-3.48906100873161));
#118287=CARTESIAN_POINT('Ctrl Pts',(6.63711407774142,3.65702152911109,-3.49267567646322));
#118288=CARTESIAN_POINT('Ctrl Pts',(6.657928135,3.524895017,-2.869580621));
#118289=CARTESIAN_POINT('Ctrl Pts',(6.501117306,3.590632927,-3.233409128));
#118290=CARTESIAN_POINT('Ctrl Pts',(6.305595129,3.655724827,-3.577984079));
#118291=CARTESIAN_POINT('Ctrl Pts',(6.30364762078715,3.65637317805554,-3.58141623466291));
#118292=CARTESIAN_POINT('Ctrl Pts',(6.3017001125743,3.65702152911109,-3.58484839032582));
#118293=CARTESIAN_POINT('',(6.64090835621227,3.65572482719221,-3.48544634034164));
#118294=CARTESIAN_POINT('',(6.47325174457986,3.6557248275383,-3.5317152071043));
#118295=CARTESIAN_POINT('',(6.88561296283959,3.56509183365582,-2.9729334170755));
#118296=CARTESIAN_POINT('Origin',(-0.179136108976734,3.48217859046664,0.0628542098480828));
#118297=CARTESIAN_POINT('Ctrl Pts',(6.65605440467583,3.52567991529962,-2.8739241044273));
#118298=CARTESIAN_POINT('Ctrl Pts',(6.6942747977918,3.532573857343,-2.89036418659647));
#118299=CARTESIAN_POINT('Ctrl Pts',(6.73253518976221,3.53929993071124,-2.90684520700562));
#118300=CARTESIAN_POINT('Ctrl Pts',(6.80904174042197,3.55242657236825,-2.93984408706979));
#118301=CARTESIAN_POINT('Ctrl Pts',(6.84733119056229,3.55883456255224,-2.95638062236419));
#118302=CARTESIAN_POINT('Ctrl Pts',(6.88561296482973,3.56509182661546,-2.97293341513429));
#118303=CARTESIAN_POINT('Ctrl Pts',(7.09929626144607,3.66023518257403,-2.42045268846277));
#118304=CARTESIAN_POINT('Ctrl Pts',(7.09471031655864,3.65798000478701,-2.43374020435282));
#118305=CARTESIAN_POINT('Ctrl Pts',(7.09012437167135,3.655724827,-2.44702772024295));
#118306=CARTESIAN_POINT('Ctrl Pts',(6.95690063859252,3.590210912,-2.83303595054817));
#118307=CARTESIAN_POINT('Ctrl Pts',(6.7825575919012,3.524902621,-3.20229929665602));
#118308=CARTESIAN_POINT('Ctrl Pts',(6.93535129000859,3.66023518257402,-2.11285137176261));
#118309=CARTESIAN_POINT('Ctrl Pts',(6.93134296050429,3.65798000478701,-2.12583380538133));
#118310=CARTESIAN_POINT('Ctrl Pts',(6.927334631,3.655724827,-2.138816239));
#118311=CARTESIAN_POINT('Ctrl Pts',(6.810890881,3.590210912,-2.515961694));
#118312=CARTESIAN_POINT('Ctrl Pts',(6.65419082,3.524902621,-2.878236358));
#118313=CARTESIAN_POINT('',(7.0897913521598,3.65572482796968,-2.44639718807978));
#118314=CARTESIAN_POINT('Origin',(-0.180792207890397,3.62500079491804,0.067598601871706));
#118315=CARTESIAN_POINT('',(7.0085629743906,3.65572482783619,-2.29260670041997));
#118316=CARTESIAN_POINT('Origin',(-1.05904868208384E-12,3.74685310399967,
4.43005007677577E-13));
#118317=CARTESIAN_POINT('',(6.88331389544986,3.74576903895486,-2.97825281201177));
#118318=CARTESIAN_POINT('Origin',(-0.167638058101914,3.62500693769422,0.0935665359519333));
#118319=CARTESIAN_POINT('Origin',(-0.180621310204258,3.48232174501777,0.03314105327856));
#118320=CARTESIAN_POINT('Ctrl Pts',(7.407191563,3.524895017,-1.176228359));
#118321=CARTESIAN_POINT('Ctrl Pts',(7.3429155,3.590632927,-1.581001044));
#118322=CARTESIAN_POINT('Ctrl Pts',(7.23491554400001,3.655724827,-1.976359549));
#118323=CARTESIAN_POINT('Ctrl Pts',(7.23383980515275,3.65637317805554,-1.98029753673787));
#118324=CARTESIAN_POINT('Ctrl Pts',(7.2327640663055,3.65702152911109,-1.98423552447575));
#118325=CARTESIAN_POINT('Ctrl Pts',(7.119144485,3.524895017,-1.371233679));
#118326=CARTESIAN_POINT('Ctrl Pts',(7.04421218,3.590632927,-1.76026577));
#118327=CARTESIAN_POINT('Ctrl Pts',(6.927334631,3.655724827,-2.138816239));
#118328=CARTESIAN_POINT('Ctrl Pts',(6.9261704664532,3.65637317805554,-2.14258680947271));
#118329=CARTESIAN_POINT('Ctrl Pts',(6.92500630190641,3.65702152911109,-2.14635737994542));
#118330=CARTESIAN_POINT('',(7.23491554310333,3.65572482719222,-1.97635954850634));
#118331=CARTESIAN_POINT('',(7.08112508842043,3.6557248275383,-2.05758789083237));
#118332=CARTESIAN_POINT('',(7.36372396347785,3.5650918336313,-1.42322463610039));
#118333=CARTESIAN_POINT('Origin',(-0.18845974150441,3.48217865323327,0.0228757456814541));
#118334=CARTESIAN_POINT('Ctrl Pts',(7.11824828163573,3.52567991527641,-1.37587841094358));
#118335=CARTESIAN_POINT('Ctrl Pts',(7.15910923468992,3.53257385730954,-1.38371787822706));
#118336=CARTESIAN_POINT('Ctrl Pts',(7.20001805195165,3.53929993065615,-1.39158872810488));
#118337=CARTESIAN_POINT('Ctrl Pts',(7.28182970571336,3.55242657232356,-1.40736946568701));
#118338=CARTESIAN_POINT('Ctrl Pts',(7.32277883614221,3.5588345625215,-1.41528828600276));
#118339=CARTESIAN_POINT('Ctrl Pts',(7.36372396500073,3.56509182659103,-1.42322463379433));
#118340=CARTESIAN_POINT('Ctrl Pts',(7.45364443950742,3.6602351826602,-0.837725005818015));
#118341=CARTESIAN_POINT('Ctrl Pts',(7.45202213458921,3.6579800048301,-0.851687709842381));
#118342=CARTESIAN_POINT('Ctrl Pts',(7.45039982967101,3.655724827,-0.865650413866756));
#118343=CARTESIAN_POINT('Ctrl Pts',(7.40327115312175,3.590210912,-1.27127315120231));
#118344=CARTESIAN_POINT('Ctrl Pts',(7.31238485399817,3.524902621,-1.66938192753812));
#118345=CARTESIAN_POINT('Ctrl Pts',(7.22740722112359,3.6602351826602,-0.572558560699135));
#118346=CARTESIAN_POINT('Ctrl Pts',(7.22628344356181,3.6579800048301,-0.586099144849566));
#118347=CARTESIAN_POINT('Ctrl Pts',(7.225159666,3.655724827,-0.599639729));
#118348=CARTESIAN_POINT('Ctrl Pts',(7.19251343,3.590210912,-0.992999697));
#118349=CARTESIAN_POINT('Ctrl Pts',(7.11735527300001,3.524902621,-1.380490461));
#118350=CARTESIAN_POINT('',(7.44993905018901,3.65572482796966,-0.865106212554298));
#118351=CARTESIAN_POINT('Origin',(-0.1910970176312,3.62500080004091,0.0271531853036942));
#118352=CARTESIAN_POINT('',(7.33754933848588,3.65572482783619,-0.732372961650914));
#118353=CARTESIAN_POINT('Origin',(5.8113236445223E-14,3.74685310400044,
-2.49908600757909E-14));
#118354=CARTESIAN_POINT('',(7.36262215976636,3.74576903890217,-1.42891389836548));
#118355=CARTESIAN_POINT('Origin',(-0.18383269441779,3.62500689138061,0.0553417618585858));
#118356=CARTESIAN_POINT('Origin',(-0.18352264207554,3.48232177509209,-0.00646204176435239));
#118357=CARTESIAN_POINT('Ctrl Pts',(7.486869868,3.524895017,0.443598437));
#118358=CARTESIAN_POINT('Ctrl Pts',(7.511110706,3.590632927,0.03447166));
#118359=CARTESIAN_POINT('Ctrl Pts',(7.490626122,3.655724827,-0.374860382));
#118360=CARTESIAN_POINT('Ctrl Pts',(7.49042208429856,3.65637317805554,-0.378937553837026));
#118361=CARTESIAN_POINT('Ctrl Pts',(7.49021804659711,3.65702152911109,-0.383014725674051));
#118362=CARTESIAN_POINT('Ctrl Pts',(7.24747755100001,3.524895017,0.191230626));
#118363=CARTESIAN_POINT('Ctrl Pts',(7.257927521,3.590632927,-0.204814342));
#118364=CARTESIAN_POINT('Ctrl Pts',(7.225159666,3.655724827,-0.599639729));
#118365=CARTESIAN_POINT('Ctrl Pts',(7.22483328017661,3.65637317805554,-0.603572406589943));
#118366=CARTESIAN_POINT('Ctrl Pts',(7.22450689435324,3.65702152911109,-0.607505084179886));
#118367=CARTESIAN_POINT('',(7.35789289421796,3.6557248275383,-0.487250052208563));
#118368=CARTESIAN_POINT('Ctrl Pts',(7.24760078043643,3.52567991527447,0.186501828081928));
#118369=CARTESIAN_POINT('Ctrl Pts',(7.28919168065719,3.53257385729426,0.187629540275512));
#118370=CARTESIAN_POINT('Ctrl Pts',(7.33083607233944,3.53929993063177,0.188736892956231));
#118371=CARTESIAN_POINT('Ctrl Pts',(7.41412740695866,3.55242657232097,0.190912187476825));
#118372=CARTESIAN_POINT('Ctrl Pts',(7.45582148165056,3.55883456253418,0.19198135736837));
#118373=CARTESIAN_POINT('Ctrl Pts',(7.49751541623966,3.56509182662043,0.193032549343876));
#118374=CARTESIAN_POINT('Ctrl Pts',(7.45946848896609,3.66023518245835,0.784173763584061));
#118375=CARTESIAN_POINT('Ctrl Pts',(7.46088568114384,3.65798000472918,0.770188752851863));
#118376=CARTESIAN_POINT('Ctrl Pts',(7.46230287332171,3.655724827,0.756203742119653));
#118377=CARTESIAN_POINT('Ctrl Pts',(7.50347293574159,3.590210912,0.349932966859502));
#118378=CARTESIAN_POINT('Ctrl Pts',(7.50029312680127,3.524902621,-0.0584061149389999));
#118379=CARTESIAN_POINT('Ctrl Pts',(7.18151762197959,3.66023518245835,0.99450645132611));
#118380=CARTESIAN_POINT('Ctrl Pts',(7.18333094298972,3.65798000472918,0.981040860163056));
#118381=CARTESIAN_POINT('Ctrl Pts',(7.18514426400001,3.655724827,0.967575269));
#118382=CARTESIAN_POINT('Ctrl Pts',(7.237822045,3.590210912,0.576393863));
#118383=CARTESIAN_POINT('Ctrl Pts',(7.247720104,3.524902621,0.181805635));
#118384=CARTESIAN_POINT('',(7.32344005060519,3.65572482783619,0.862105722358991));
#118385=CARTESIAN_POINT('Ctrl Pts',(7.21647046,3.524895017,2.042683064));
#118386=CARTESIAN_POINT('Ctrl Pts',(7.328094724,3.590632927,1.648332506));
#118387=CARTESIAN_POINT('Ctrl Pts',(7.396083347,3.655724827,1.24416684));
#118388=CARTESIAN_POINT('Ctrl Pts',(7.39676055100675,3.65637317805554,1.24014112810397));
#118389=CARTESIAN_POINT('Ctrl Pts',(7.39743775501351,3.65702152911109,1.23611541620793));
#118390=CARTESIAN_POINT('Ctrl Pts',(7.036926621,3.524895017,1.7447532));
#118391=CARTESIAN_POINT('Ctrl Pts',(7.132270238,3.590632927,1.360213978));
#118392=CARTESIAN_POINT('Ctrl Pts',(7.18514426400001,3.655724827,0.967575269));
#118393=CARTESIAN_POINT('Ctrl Pts',(7.18567091832362,3.65637317805554,0.963664371923291));
#118394=CARTESIAN_POINT('Ctrl Pts',(7.18619757264725,3.65702152911109,0.959753474846583));
#118395=CARTESIAN_POINT('',(7.39608334597518,3.65572482719222,1.24416684004987));
#118396=CARTESIAN_POINT('',(7.29061380500531,3.6557248275383,1.10587105776134));
#118397=CARTESIAN_POINT('',(7.28073138003579,3.56509183364385,1.80026374265344));
#118398=CARTESIAN_POINT('Origin',(-0.180646895504575,3.48217863662677,-0.0583707780274595));
#118399=CARTESIAN_POINT('Ctrl Pts',(7.03806352124642,3.52567991521218,1.7401614500682));
#118400=CARTESIAN_POINT('Ctrl Pts',(7.07843962488291,3.53257385728293,1.7502036110421));
#118401=CARTESIAN_POINT('Ctrl Pts',(7.11887234611513,3.53929993067132,1.76023738760649));
#118402=CARTESIAN_POINT('Ctrl Pts',(7.19974875170204,3.55242657234967,1.78026699959728));
#118403=CARTESIAN_POINT('Ctrl Pts',(7.24023820213086,3.55883456254047,1.79027416635503));
#118404=CARTESIAN_POINT('Ctrl Pts',(7.28073138044745,3.56509182660367,1.80026374539461));
#118405=CARTESIAN_POINT('Ctrl Pts',(7.11649608109494,3.66023518243807,2.36940544160283));
#118406=CARTESIAN_POINT('Ctrl Pts',(7.12088650402253,3.65798000471904,2.35605204714253));
#118407=CARTESIAN_POINT('Ctrl Pts',(7.12527692695003,3.655724827,2.34269865268223));
#118408=CARTESIAN_POINT('Ctrl Pts',(7.25282066421712,3.590210912,1.95477660900104));
#118409=CARTESIAN_POINT('Ctrl Pts',(7.33749603053574,3.524902621,1.55530070319499));
#118410=CARTESIAN_POINT('Ctrl Pts',(6.79982824183194,3.66023518243808,2.51506944727944));
#118411=CARTESIAN_POINT('Ctrl Pts',(6.8044938724159,3.65798000471904,2.50230848463969));
#118412=CARTESIAN_POINT('Ctrl Pts',(6.809159503,3.655724827,2.489547522));
#118413=CARTESIAN_POINT('Ctrl Pts',(6.944698145,3.590210912,2.118835886));
#118414=CARTESIAN_POINT('Ctrl Pts',(7.039189599,3.524902621,1.735600702));
#118415=CARTESIAN_POINT('',(7.1246302310521,3.65572482796922,2.34299907947824));
#118416=CARTESIAN_POINT('Origin',(-0.184836620676564,3.62500080738618,-0.0555960842180652));
#118417=CARTESIAN_POINT('',(6.96689484519621,3.65572482783619,2.41627330110929));
#118418=CARTESIAN_POINT('Origin',(5.73759789679329E-13,3.74685310399911,
1.59052458703624E-13));
#118419=CARTESIAN_POINT('',(7.2821202696205,3.74576903894091,1.79463767308797));
#118420=CARTESIAN_POINT('Origin',(-0.190079571027402,3.6250068814924,-0.0269625511958518));
#118421=CARTESIAN_POINT('Origin',(-0.163847624695173,3.48232176305973,-0.0829240434496378));
#118422=CARTESIAN_POINT('Ctrl Pts',(6.608636913,3.524895017,3.546254101));
#118423=CARTESIAN_POINT('Ctrl Pts',(6.802425177,3.590632927,3.185119157));
#118424=CARTESIAN_POINT('Ctrl Pts',(6.955707935,3.655724827,2.805018204));
#118425=CARTESIAN_POINT('Ctrl Pts',(6.95723471541271,3.65637317805554,2.80123218985553));
#118426=CARTESIAN_POINT('Ctrl Pts',(6.95876149582542,3.65702152911109,2.79744617571105));
#118427=CARTESIAN_POINT('Ctrl Pts',(6.497336824,3.524895017,3.216693053));
#118428=CARTESIAN_POINT('Ctrl Pts',(6.673115926,3.590632927,2.861640204));
#118429=CARTESIAN_POINT('Ctrl Pts',(6.809159503,3.655724827,2.489547522));
#118430=CARTESIAN_POINT('Ctrl Pts',(6.81051457170667,3.65637317805554,2.48584127463075));
#118431=CARTESIAN_POINT('Ctrl Pts',(6.81186964041335,3.65702152911109,2.48213502726149));
#118432=CARTESIAN_POINT('',(6.95570793398814,3.65572482719221,2.8050182038267));
#118433=CARTESIAN_POINT('',(6.88243371781578,3.6557248275383,2.64728286607875));
#118434=CARTESIAN_POINT('',(6.72350843674559,3.56509183364709,3.32331660677712));
#118435=CARTESIAN_POINT('Origin',(-0.163875473105116,3.48217864288177,-0.0958398440449543));
#118436=CARTESIAN_POINT('Ctrl Pts',(6.49943423469484,3.52567991526485,3.21245305500109));
#118437=CARTESIAN_POINT('Ctrl Pts',(6.53670759947093,3.53257385731295,3.23094010477315));
#118438=CARTESIAN_POINT('Ctrl Pts',(6.5740380605636,3.53929993067782,3.24943113723722));
#118439=CARTESIAN_POINT('Ctrl Pts',(6.64871784602487,3.55242657234897,3.28637850488452));
#118440=CARTESIAN_POINT('Ctrl Pts',(6.68610943050522,3.55883456254205,3.30485574479466));
#118441=CARTESIAN_POINT('Ctrl Pts',(6.72350843655732,3.56509182660701,3.32331660954475));
#118442=CARTESIAN_POINT('Ctrl Pts',(6.44076422642631,3.660235182589,3.84384635591007));
#118443=CARTESIAN_POINT('Ctrl Pts',(6.44792258902591,3.6579800047945,3.83174896713056));
#118444=CARTESIAN_POINT('Ctrl Pts',(6.45508095162562,3.655724827,3.81965157835112));
#118445=CARTESIAN_POINT('Ctrl Pts',(6.663034559558,3.590210912,3.46821706966159));
#118446=CARTESIAN_POINT('Ctrl Pts',(6.83160577317824,3.524902621,3.09628338849629));
#118447=CARTESIAN_POINT('Ctrl Pts',(6.1001864494939,3.660235182589,3.91803059333484));
#118448=CARTESIAN_POINT('Ctrl Pts',(6.10748623024694,3.6579800047945,3.90657094716742));
#118449=CARTESIAN_POINT('Ctrl Pts',(6.114786011,3.655724827,3.895111301));
#118450=CARTESIAN_POINT('Ctrl Pts',(6.326847879,3.590210912,3.562203498));
#118451=CARTESIAN_POINT('Ctrl Pts',(6.501514411,3.524902621,3.208241008));
#118452=CARTESIAN_POINT('',(6.45438479219936,3.65572482796923,3.81980596085165));
#118453=CARTESIAN_POINT('Origin',(-0.168563572421865,3.62500081258431,-0.0940305921459722));
#118454=CARTESIAN_POINT('',(6.28458538020791,3.65572482783619,3.85745862658826));
#118455=CARTESIAN_POINT('Origin',(-1.34441069388203E-12,3.74685310400044,
-6.36426675248991E-13));
#118456=CARTESIAN_POINT('',(6.72607429379896,3.74576903896969,3.31812064153517));
#118457=CARTESIAN_POINT('Origin',(-0.179839597766256,3.62500689088592,-0.0671937332775935));
#118458=CARTESIAN_POINT('Origin',(-0.142191017882454,3.48232181496895,-0.116207852334306));
#118459=CARTESIAN_POINT('Ctrl Pts',(5.69179085,3.524895017,4.884006237));
#118460=CARTESIAN_POINT('Ctrl Pts',(5.958681789,3.590632927,4.572973176));
#118461=CARTESIAN_POINT('Ctrl Pts',(6.190091351,3.655724827,4.234710034));
#118462=CARTESIAN_POINT('Ctrl Pts',(6.19239631726747,3.65637317805554,4.23134074741953));
#118463=CARTESIAN_POINT('Ctrl Pts',(6.19470128353494,3.65702152911109,4.22797146083906));
#118464=CARTESIAN_POINT('Ctrl Pts',(5.653938778,3.524895017,4.538223914));
#118465=CARTESIAN_POINT('Ctrl Pts',(5.90193413,3.590632927,4.229259314));
#118466=CARTESIAN_POINT('Ctrl Pts',(6.114786011,3.655724827,3.895111301));
#118467=CARTESIAN_POINT('Ctrl Pts',(6.11690613257765,3.65637317805554,3.89178300336333));
#118468=CARTESIAN_POINT('Ctrl Pts',(6.11902625415531,3.65702152911109,3.88845470572666));
#118469=CARTESIAN_POINT('',(6.19009135031808,3.65572482719341,4.23471003320417));
#118470=CARTESIAN_POINT('',(6.15243867918163,3.6557248275383,4.06491067025219));
#118471=CARTESIAN_POINT('',(5.85190171216796,3.56509183364086,4.69097487982885));
#118472=CARTESIAN_POINT('Origin',(-0.139441555156309,3.48217860768295,-0.128827649737256));
#118473=CARTESIAN_POINT('Ctrl Pts',(5.65689862657596,3.52567991524778,4.53453392617591));
#118474=CARTESIAN_POINT('Ctrl Pts',(5.68932639171087,3.53257385728754,4.56060143058841));
#118475=CARTESIAN_POINT('Ctrl Pts',(5.72180906204669,3.53929993064708,4.58668509863778));
#118476=CARTESIAN_POINT('Ctrl Pts',(5.78680028387411,3.5524265723281,4.63882260382768));
#118477=CARTESIAN_POINT('Ctrl Pts',(5.81934561351409,3.55883456252675,4.66490594159134));
#118478=CARTESIAN_POINT('Ctrl Pts',(5.85190171139198,3.56509182660114,4.69097488248765));
#118479=CARTESIAN_POINT('Ctrl Pts',(5.46386939543312,3.66023518256184,5.13855328504425));
#118480=CARTESIAN_POINT('Ctrl Pts',(5.47346098040717,3.65798000478092,5.12827756291872));
#118481=CARTESIAN_POINT('Ctrl Pts',(5.48305256538124,3.655724827,5.11800184079321));
#118482=CARTESIAN_POINT('Ctrl Pts',(5.76169236399178,3.590210912,4.81948755442943));
#118483=CARTESIAN_POINT('Ctrl Pts',(6.00627722401707,3.524902621,4.4924873040965));
#118484=CARTESIAN_POINT('Ctrl Pts',(5.11530671890459,3.66023518256184,5.13778898070581));
#118485=CARTESIAN_POINT('Ctrl Pts',(5.12489931995231,3.65798000478092,5.1281664918529));
#118486=CARTESIAN_POINT('Ctrl Pts',(5.134491921,3.655724827,5.118544003));
#118487=CARTESIAN_POINT('Ctrl Pts',(5.413161237,3.590210912,4.839006433));
#118488=CARTESIAN_POINT('Ctrl Pts',(5.659835635,3.524902621,4.530867531));
#118489=CARTESIAN_POINT('',(5.48233949409281,3.65572482796922,5.11800296022109));
#118490=CARTESIAN_POINT('Origin',(-0.144408942952712,3.6250008350005,-0.128068477123946));
#118491=CARTESIAN_POINT('',(5.308415687593,3.65572482783619,5.11827347277353));
#118492=CARTESIAN_POINT('Origin',(2.91867224833098E-13,3.74685310399922,
2.51968584885631E-13));
#118493=CARTESIAN_POINT('',(5.85552455969037,3.74576903894377,4.68645197666851));
#118494=CARTESIAN_POINT('Origin',(-0.16119026828776,3.62500687370807,-0.104282894806315));
#118495=CARTESIAN_POINT('Origin',(-0.113885433031731,3.48232172951026,-0.144057869348729));
#118496=CARTESIAN_POINT('Ctrl Pts',(4.508802972,3.524895017,5.99338767));
#118497=CARTESIAN_POINT('Ctrl Pts',(4.836317064,3.590632927,5.747000052));
#118498=CARTESIAN_POINT('Ctrl Pts',(5.135032975,3.655724827,5.466391529));
#118499=CARTESIAN_POINT('Ctrl Pts',(5.13800834945065,3.65637317805554,5.46359651407369));
#118500=CARTESIAN_POINT('Ctrl Pts',(5.14098372390131,3.65702152911109,5.46080149914739));
#118501=CARTESIAN_POINT('Ctrl Pts',(4.546168838,3.524895017,5.647552469));
#118502=CARTESIAN_POINT('Ctrl Pts',(4.854784453,3.590632927,5.39912296));
#118503=CARTESIAN_POINT('Ctrl Pts',(5.134491921,3.655724827,5.118544003));
#118504=CARTESIAN_POINT('Ctrl Pts',(5.13727796092388,3.65637317805554,5.11574928256728));
#118505=CARTESIAN_POINT('Ctrl Pts',(5.14006400084776,3.65702152911109,5.11295456213456));
#118506=CARTESIAN_POINT('',(5.13503297415595,3.65572482719221,5.46639152841513));
#118507=CARTESIAN_POINT('',(5.1347624456325,3.6557248275383,5.29246776829695));
#118508=CARTESIAN_POINT('',(4.70666656738194,3.56509183363972,5.83928838101205));
#118509=CARTESIAN_POINT('Origin',(-0.108487181196059,3.48217862674873,-0.155791336103154));
#118510=CARTESIAN_POINT('Ctrl Pts',(4.54985272534518,3.5256799152631,5.64458503093839));
#118511=CARTESIAN_POINT('Ctrl Pts',(4.57591860460814,3.53257385730365,5.67701410253778));
#118512=CARTESIAN_POINT('Ctrl Pts',(4.60203463073502,3.5392999306659,5.70947076287906));
#118513=CARTESIAN_POINT('Ctrl Pts',(4.6542983717518,3.55242657233496,5.77436051365568));
#118514=CARTESIAN_POINT('Ctrl Pts',(4.68047566321139,3.5588345625283,5.80683032126513));
#118515=CARTESIAN_POINT('Ctrl Pts',(4.70666656605314,3.56509182659974,5.83928838344145));
#118516=CARTESIAN_POINT('Ctrl Pts',(4.23149010313324,3.66023518260803,6.1929871736484));
#118517=CARTESIAN_POINT('Ctrl Pts',(4.24306641882883,3.65798000480402,6.18501359937273));
#118518=CARTESIAN_POINT('Ctrl Pts',(4.25464273452441,3.655724827,6.17704002509703));
#118519=CARTESIAN_POINT('Ctrl Pts',(4.59093983763609,3.590210912,5.94540415744501));
#118520=CARTESIAN_POINT('Ctrl Pts',(4.90010182696033,3.524902621,5.67862750629276));
#118521=CARTESIAN_POINT('Ctrl Pts',(3.89124093061716,3.66023518260803,6.11731006767163));
#118522=CARTESIAN_POINT('Ctrl Pts',(3.90267781280862,3.65798000480402,6.10997467283589));
#118523=CARTESIAN_POINT('Ctrl Pts',(3.914114695,3.655724827,6.102639278));
#118524=CARTESIAN_POINT('Ctrl Pts',(4.246361193,3.590210912,5.889542806));
#118525=CARTESIAN_POINT('Ctrl Pts',(4.553509235,3.524902621,5.641635724));
#118526=CARTESIAN_POINT('',(4.25394609309613,3.65572482796967,6.17688782937028));
#118527=CARTESIAN_POINT('Origin',(-0.113501710319515,3.62500081890866,-0.156117841935746));
#118528=CARTESIAN_POINT('',(4.08403037681007,3.65572482783619,6.13976354063303));
#118529=CARTESIAN_POINT('Origin',(2.14238349283136E-13,3.74685310400067,
3.43908929112402E-13));
#118530=CARTESIAN_POINT('',(4.71117700472489,3.74576903895635,5.83565002592714));
#118531=CARTESIAN_POINT('Origin',(-0.135004131882551,3.62500692857403,-0.136496139368398));
#118532=CARTESIAN_POINT('Origin',(-0.0802545157818219,3.48232179160699,
-0.165171658052808));
#118533=CARTESIAN_POINT('Ctrl Pts',(3.114988478,3.524895017,6.822524956));
#118534=CARTESIAN_POINT('Ctrl Pts',(3.487811527,3.590632927,6.652303593));
#118535=CARTESIAN_POINT('Ctrl Pts',(3.839866164,3.655724827,6.442470632));
#118536=CARTESIAN_POINT('Ctrl Pts',(3.84337282144137,3.65637317805554,6.44038058052275));
#118537=CARTESIAN_POINT('Ctrl Pts',(3.84687947888274,3.65702152911109,6.4382905290455));
#118538=CARTESIAN_POINT('Ctrl Pts',(3.225825097,3.524895017,6.492807747));
#118539=CARTESIAN_POINT('Ctrl Pts',(3.580630451,3.590632927,6.316529616));
#118540=CARTESIAN_POINT('Ctrl Pts',(3.914114695,3.655724827,6.102639278));
#118541=CARTESIAN_POINT('Ctrl Pts',(3.91743638113306,3.65637317805554,6.10050881282057));
#118542=CARTESIAN_POINT('Ctrl Pts',(3.92075806726612,3.65702152911109,6.09837834764114));
#118543=CARTESIAN_POINT('',(3.83986616329884,3.65572482719222,6.44247063125054));
#118544=CARTESIAN_POINT('',(3.87699042669408,3.6557248275383,6.27255495673431));
#118545=CARTESIAN_POINT('',(3.34135292461231,3.56509183369146,6.71456324749908));
#118546=CARTESIAN_POINT('Origin',(-0.0724602166674065,3.48217860567644,
-0.175470452308175));
#118547=CARTESIAN_POINT('Ctrl Pts',(3.230060768144,3.5256799151844,6.49070161308116));
#118548=CARTESIAN_POINT('Ctrl Pts',(3.24854594976219,3.53257385725448,6.52797590452752));
#118549=CARTESIAN_POINT('Ctrl Pts',(3.26707417510236,3.53929993064325,6.56528791979451));
#118550=CARTESIAN_POINT('Ctrl Pts',(3.30416664053201,3.55242657235513,6.63989574360624));
#118551=CARTESIAN_POINT('Ctrl Pts',(3.32275187260552,3.55883456256649,6.67723376899636));
#118552=CARTESIAN_POINT('Ctrl Pts',(3.3413529227585,3.56509182665127,6.71456324960291));
#118553=CARTESIAN_POINT('Ctrl Pts',(2.80125103830434,3.66023518240983,6.95784386525036));
#118554=CARTESIAN_POINT('Ctrl Pts',(2.81427078837048,3.65798000470493,6.95254527459315));
#118555=CARTESIAN_POINT('Ctrl Pts',(2.82729053843668,3.655724827,6.94724668393587));
#118556=CARTESIAN_POINT('Ctrl Pts',(3.20552006655533,3.590210912,6.79332026954184));
#118557=CARTESIAN_POINT('Ctrl Pts',(3.56480311451474,3.524902621,6.59924139770641));
#118558=CARTESIAN_POINT('Ctrl Pts',(2.48522504358556,3.66023518240984,6.81079253315187));
#118559=CARTESIAN_POINT('Ctrl Pts',(2.49797143029281,3.65798000470493,6.80608722757588));
#118560=CARTESIAN_POINT('Ctrl Pts',(2.510717817,3.655724827,6.801381922));
#118561=CARTESIAN_POINT('Ctrl Pts',(2.881006018,3.590210912,6.664690703));
#118562=CARTESIAN_POINT('Ctrl Pts',(3.234265804,3.524902621,6.488607301));
#118563=CARTESIAN_POINT('',(2.82664290169905,3.65572482796968,6.94694828916187));
#118564=CARTESIAN_POINT('Origin',(-0.0772874867209844,3.6250008063393,-0.176867614939211));
#118565=CARTESIAN_POINT('',(2.66868034532562,3.65572482783619,6.87416508912661));
#118566=CARTESIAN_POINT('Origin',(4.88758339356465E-13,3.74685310399989,
9.87925019568792E-13));
#118567=CARTESIAN_POINT('',(3.34654004947767,3.74576903895837,6.71197956588787));
#118568=CARTESIAN_POINT('Origin',(-0.102505000056622,3.62500693001679,-0.162326509812541));
#118569=CARTESIAN_POINT('Origin',(-0.0428713111393131,3.48232180333034,
-0.178562645459894));
#118570=CARTESIAN_POINT('Ctrl Pts',(1.575520586,3.524895017,7.332648559));
#118571=CARTESIAN_POINT('Ctrl Pts',(1.9762198,3.590632927,7.246552811));
#118572=CARTESIAN_POINT('Ctrl Pts',(2.365151479,3.655724827,7.11730696800001));
#118573=CARTESIAN_POINT('Ctrl Pts',(2.36902545202297,3.65637317805554,7.11601960845552));
#118574=CARTESIAN_POINT('Ctrl Pts',(2.37289942504594,3.65702152911109,7.11473224891103));
#118575=CARTESIAN_POINT('Ctrl Pts',(1.754645359,3.524895017,7.03446655100001));
#118576=CARTESIAN_POINT('Ctrl Pts',(2.139050148,3.590632927,6.938582368));
#118577=CARTESIAN_POINT('Ctrl Pts',(2.510717817,3.655724827,6.801381922));
#118578=CARTESIAN_POINT('Ctrl Pts',(2.51441983100647,3.65637317805554,6.80001533024304));
#118579=CARTESIAN_POINT('Ctrl Pts',(2.51812184501293,3.65702152911109,6.79864873848607));
#118580=CARTESIAN_POINT('',(2.36515147845739,3.65572482719223,7.11730696713216));
#118581=CARTESIAN_POINT('',(2.43793464488681,3.65572482753831,6.95934444609059));
#118582=CARTESIAN_POINT('',(1.81980133343817,3.5650918336497,7.27587259882722));
#118583=CARTESIAN_POINT('Origin',(-0.0330452042788285,3.48217859242297,
-0.186944949984029));
#118584=CARTESIAN_POINT('Ctrl Pts',(1.75923475895739,3.52567991519402,7.03332020162641));
#118585=CARTESIAN_POINT('Ctrl Pts',(1.76927489669448,3.53257385725999,7.07369680843662));
#118586=CARTESIAN_POINT('Ctrl Pts',(1.77934896227731,3.53929993064844,7.11411951025837));
#118587=CARTESIAN_POINT('Ctrl Pts',(1.79953575004537,3.55242657233731,7.1949568280426));
#118588=CARTESIAN_POINT('Ctrl Pts',(1.80965989807368,3.55883456253557,7.2354171865551));
#118589=CARTESIAN_POINT('Ctrl Pts',(1.81980133120497,3.56509182660936,7.27587260047597));
#118590=CARTESIAN_POINT('Ctrl Pts',(1.24002858623345,3.66023518253582,7.39735951019233));
#118591=CARTESIAN_POINT('Ctrl Pts',(1.25388298254613,3.65798000476791,7.39498365900624));
#118592=CARTESIAN_POINT('Ctrl Pts',(1.26773737885882,3.655724827,7.39260780782015));
#118593=CARTESIAN_POINT('Ctrl Pts',(1.67021374028811,3.590210912,7.32358827646765));
#118594=CARTESIAN_POINT('Ctrl Pts',(2.06281817067519,3.524902621,7.21128209545936));
#118595=CARTESIAN_POINT('Ctrl Pts',(0.963002793498291,3.66023518253582,
7.1858099096259));
#118596=CARTESIAN_POINT('Ctrl Pts',(0.976462678749152,3.65798000476791,
7.18395470781295));
#118597=CARTESIAN_POINT('Ctrl Pts',(0.989922564,3.655724827,7.182099506));
#118598=CARTESIAN_POINT('Ctrl Pts',(1.380938204,3.590210912,7.12820507));
#118599=CARTESIAN_POINT('Ctrl Pts',(1.763791699,3.524902621,7.032178812));
#118600=CARTESIAN_POINT('',(1.26716903033796,3.65572482796929,7.39217716664284));
#118601=CARTESIAN_POINT('Origin',(-0.037459188035332,3.62500079716236,-0.189346868690627));
#118602=CARTESIAN_POINT('',(1.12854578661594,3.65572482783626,7.28713831720771));
#118603=CARTESIAN_POINT('Origin',(3.20490162186715E-13,3.74685310399967,
1.17700987845026E-12));
#118604=CARTESIAN_POINT('',(1.82542260129696,3.7457690389737,7.274464401048));
#118605=CARTESIAN_POINT('Origin',(-0.0652131106448975,3.62500690827945,
-0.180566992370154));
#118606=CARTESIAN_POINT('Origin',(-0.00348321090670733,3.48232174858048,
-0.183603634743864));
#118607=CARTESIAN_POINT('Ctrl Pts',(-0.037616899,3.524895017,7.49990566400001));
#118608=CARTESIAN_POINT('Ctrl Pts',(0.372222232,3.590632927,7.501961273));
#118609=CARTESIAN_POINT('Ctrl Pts',(0.77984494,3.655724827,7.459345941));
#118610=CARTESIAN_POINT('Ctrl Pts',(0.783905085932064,3.65637317805554,
7.45892146890003));
#118611=CARTESIAN_POINT('Ctrl Pts',(0.787965231864128,3.65702152911109,
7.45849699680004));
#118612=CARTESIAN_POINT('Ctrl Pts',(0.201420355,3.524895017,7.247201518));
#118613=CARTESIAN_POINT('Ctrl Pts',(0.597450238,3.590632927,7.23619472));
#118614=CARTESIAN_POINT('Ctrl Pts',(0.989922563999999,3.655724827,7.182099506));
#118615=CARTESIAN_POINT('Ctrl Pts',(0.993831803810694,3.65637317805554,
7.18156068797354));
#118616=CARTESIAN_POINT('Ctrl Pts',(0.997741043621388,3.65702152911109,
7.18102186994708));
#118617=CARTESIAN_POINT('',(0.779844939665669,3.65572482719222,7.45934594003148));
#118618=CARTESIAN_POINT('',(0.88488374872519,3.6557248275383,7.32072272389584));
#118619=CARTESIAN_POINT('',(0.213157853479665,3.56509183362931,7.49697023446842));
#118620=CARTESIAN_POINT('Origin',(0.00791499949564178,3.48217862741154,
-0.189678175733404));
#118621=CARTESIAN_POINT('Ctrl Pts',(0.206148889001752,3.52567991523746,
7.24706855475945));
#118622=CARTESIAN_POINT('Ctrl Pts',(0.207274516531135,3.5325738572827,7.28865951157601));
#118623=CARTESIAN_POINT('Ctrl Pts',(0.208423369727975,3.5392999306431,7.33030277919583));
#118624=CARTESIAN_POINT('Ctrl Pts',(0.210760567333695,3.55242657232236,
7.4135897279966));
#118625=CARTESIAN_POINT('Ctrl Pts',(0.211950237156683,3.55883456252139,
7.45528053840675));
#118626=CARTESIAN_POINT('Ctrl Pts',(0.213157850959172,3.56509182658913,
7.4969702355981));
#118627=CARTESIAN_POINT('Ctrl Pts',(-0.379176222983314,3.66023518244822,
7.49098284762322));
#118628=CARTESIAN_POINT('Ctrl Pts',(-0.365134997269743,3.65798000472411,
7.49164082814761));
#118629=CARTESIAN_POINT('Ctrl Pts',(-0.351093771556175,3.655724827,7.49229880867192));
#118630=CARTESIAN_POINT('Ctrl Pts',(0.0568100748054015,3.590210912,7.51141343528446));
#118631=CARTESIAN_POINT('Ctrl Pts',(0.464378140806264,3.524902621,7.48613125750417));
#118632=CARTESIAN_POINT('Ctrl Pts',(-0.60424839578379,3.66023518244822,
7.22482680159335));
#118633=CARTESIAN_POINT('Ctrl Pts',(-0.590704381891892,3.65798000472411,
7.22590845079669));
#118634=CARTESIAN_POINT('Ctrl Pts',(-0.577160368,3.655724827,7.2269901));
#118635=CARTESIAN_POINT('Ctrl Pts',(-0.183700746,3.590210912,7.25841249));
#118636=CARTESIAN_POINT('Ctrl Pts',(0.210844655,3.524902621,7.24693345700001));
#118637=CARTESIAN_POINT('',(-0.351556258027216,3.65572482796968,7.4917560572968));
#118638=CARTESIAN_POINT('Origin',(0.00412055726725919,3.62500080754839,
-0.192972789225312));
#118639=CARTESIAN_POINT('',(-0.464358318833719,3.6557248278362,7.35937305782598));
#118640=CARTESIAN_POINT('Origin',(4.42896587460329E-14,3.74685310400067,
5.41233724504764E-13));
#118641=CARTESIAN_POINT('',(0.218950420586282,3.74576903894199,7.49680336605748));
#118642=CARTESIAN_POINT('Origin',(-0.0248718918509416,3.62500691765216,
-0.190364284633733));
#118643=CARTESIAN_POINT('Origin',(0.0360675772053069,3.48232171708846,-0.180060425093342));
#118644=CARTESIAN_POINT('Ctrl Pts',(0.467054599,2.232664075,7.485443207));
#118645=CARTESIAN_POINT('Ctrl Pts',(0.87318754,2.168401865,7.460102522));
#118646=CARTESIAN_POINT('Ctrl Pts',(1.274194673,2.103255924,7.39096935));
#118647=CARTESIAN_POINT('Ctrl Pts',(0.213937947,2.232664075,7.246842799));
#118648=CARTESIAN_POINT('Ctrl Pts',(0.607125298,2.168401865,7.235235304));
#118649=CARTESIAN_POINT('Ctrl Pts',(0.996748685,2.103255924,7.181155343));
#118650=CARTESIAN_POINT('',(0.992091960527736,2.10403448620838,7.18180016027124));
#118651=CARTESIAN_POINT('Origin',(-0.0408077731901307,2.01791740531367,
-0.190716934482191));
#118652=CARTESIAN_POINT('Ctrl Pts',(1.02848533315001,2.14301213123373,7.42914651317701));
#118653=CARTESIAN_POINT('Ctrl Pts',(1.02259958178598,2.1370611205462,7.38936730565107));
#118654=CARTESIAN_POINT('Ctrl Pts',(1.01650022449132,2.13073653553286,7.34805528870324));
#118655=CARTESIAN_POINT('Ctrl Pts',(1.00415932290291,2.11752971609119,7.26418729613499));
#118656=CARTESIAN_POINT('Ctrl Pts',(0.998112042998285,2.11086974920619,
7.22296771414384));
#118657=CARTESIAN_POINT('Ctrl Pts',(0.992091959548518,2.10403448636993,
7.18180016038761));
#118658=CARTESIAN_POINT('Ctrl Pts',(0.777222552,2.103262031,7.459619635));
#118659=CARTESIAN_POINT('Ctrl Pts',(0.902618358,2.123129682,7.446554566));
#118660=CARTESIAN_POINT('Ctrl Pts',(1.027504195,2.142857143,7.429282275));
#118661=CARTESIAN_POINT('Ctrl Pts',(1.309731339,2.187438859,7.390248953));
#118662=CARTESIAN_POINT('Ctrl Pts',(1.588183719,2.232664075,7.329916267));
#118663=CARTESIAN_POINT('Ctrl Pts',(0.98739763,2.103262031,7.182447071));
#118664=CARTESIAN_POINT('Ctrl Pts',(1.10813418,2.123129682,7.165848969));
#118665=CARTESIAN_POINT('Ctrl Pts',(1.228244647,2.142857143,7.145202243));
#118666=CARTESIAN_POINT('Ctrl Pts',(1.499680022,2.187438859,7.098543095));
#118667=CARTESIAN_POINT('Ctrl Pts',(1.766793184,2.232664075,7.031425307));
#118668=CARTESIAN_POINT('Ctrl Pts',(1.76679317507296,2.23266407348855,7.03142530924311));
#118669=CARTESIAN_POINT('Ctrl Pts',(1.62253262275256,2.20823916463419,7.06767380049264));
#118670=CARTESIAN_POINT('Ctrl Pts',(1.47748684829027,2.183982876726,7.09939539754149));
#118671=CARTESIAN_POINT('Ctrl Pts',(1.33207819674674,2.15996092288709,7.126574751153));
#118672=CARTESIAN_POINT('Ctrl Pts',(1.29748568338354,2.15424613390885,7.13304068108929));
#118673=CARTESIAN_POINT('Ctrl Pts',(1.2628726178915,2.14854459021232,7.13924977054086));
#118674=CARTESIAN_POINT('Ctrl Pts',(1.22824464580779,2.14285714281195,7.14520224326374));
#118675=CARTESIAN_POINT('Ctrl Pts',(1.14987371677628,2.12998516349532,7.15867403410597));
#118676=CARTESIAN_POINT('Ctrl Pts',(1.07113569834775,2.11704095619703,7.1708810795655));
#118677=CARTESIAN_POINT('Ctrl Pts',(0.992091965201322,2.1040344873685,7.18180016009835));
#118678=CARTESIAN_POINT('Ctrl Pts',(2.065284143,2.232664075,7.210034772));
#118679=CARTESIAN_POINT('Ctrl Pts',(2.456474424,2.168401865,7.097979961));
#118680=CARTESIAN_POINT('Ctrl Pts',(2.833244645,2.103255924,6.944258404));
#118681=CARTESIAN_POINT('Ctrl Pts',(1.766793184,2.232664075,7.031425307));
#118682=CARTESIAN_POINT('Ctrl Pts',(2.148292764,2.168401865,6.93556553));
#118683=CARTESIAN_POINT('Ctrl Pts',(2.51718138,2.103255924,6.798992418));
#118684=CARTESIAN_POINT('',(2.51277214473806,2.10403448615021,6.80062321801409));
#118685=CARTESIAN_POINT('Origin',(-0.0808521565263137,2.01791771072404,
-0.177485649792515));
#118686=CARTESIAN_POINT('Ctrl Pts',(2.6014868140917,2.14301213126478,7.03436325144443));
#118687=CARTESIAN_POINT('Ctrl Pts',(2.58718731604052,2.13706112120453,6.99677932611909));
#118688=CARTESIAN_POINT('Ctrl Pts',(2.57234969575751,2.13073653613662,6.9577443421695));
#118689=CARTESIAN_POINT('Ctrl Pts',(2.54226833099551,2.11752978378426,6.8784904682225));
#118690=CARTESIAN_POINT('Ctrl Pts',(2.52750135875876,2.11086978246806,6.83953434665737));
#118691=CARTESIAN_POINT('Ctrl Pts',(2.51277214242083,2.10403448654085,6.80062321882262));
#118692=CARTESIAN_POINT('Ctrl Pts',(2.362649238,2.103262031,7.118138));
#118693=CARTESIAN_POINT('Ctrl Pts',(2.482304756,2.123129682,7.078421992));
#118694=CARTESIAN_POINT('Ctrl Pts',(2.600557799,2.142857143,7.034706755));
#118695=CARTESIAN_POINT('Ctrl Pts',(2.867795619,2.187438859,6.935915516));
#118696=CARTESIAN_POINT('Ctrl Pts',(3.126768193,2.232664075,6.817134344));
#118697=CARTESIAN_POINT('Ctrl Pts',(2.50832663,2.103262031,6.802264146));
#118698=CARTESIAN_POINT('Ctrl Pts',(2.622672326,2.123129682,6.76009931));
#118699=CARTESIAN_POINT('Ctrl Pts',(2.735536241,2.142857143,6.714115092));
#118700=CARTESIAN_POINT('Ctrl Pts',(2.99059527,2.187438859,6.610196228));
#118701=CARTESIAN_POINT('Ctrl Pts',(3.237035134,2.232664075,6.487226182));
#118702=CARTESIAN_POINT('Ctrl Pts',(3.23703512624068,2.23266407357605,6.48722618587179));
#118703=CARTESIAN_POINT('Ctrl Pts',(3.10393962719884,2.20823915874926,6.55363897853008));
#118704=CARTESIAN_POINT('Ctrl Pts',(2.969104115023,2.18398286498676,6.61579951009992));
#118705=CARTESIAN_POINT('Ctrl Pts',(2.83293776111239,2.1599609054766,6.67360199905533));
#118706=CARTESIAN_POINT('Ctrl Pts',(2.80054401808973,2.15424612233873,6.68735311245094));
#118707=CARTESIAN_POINT('Ctrl Pts',(2.76807499048703,2.14854458445958,6.70085780874828));
#118708=CARTESIAN_POINT('Ctrl Pts',(2.7355362399328,2.14285714285121,6.71411509285976));
#118709=CARTESIAN_POINT('Ctrl Pts',(2.6618936167638,2.12998516357859,6.74411935469137));
#118710=CARTESIAN_POINT('Ctrl Pts',(2.58762060356933,2.11704095629822,6.77296735215525));
#118711=CARTESIAN_POINT('Ctrl Pts',(2.51277214949572,2.10403448774872,6.80062321598498));
#118712=CARTESIAN_POINT('Ctrl Pts',(3.566943297,2.232664075,6.597493124));
#118713=CARTESIAN_POINT('Ctrl Pts',(3.924899294,2.168401865,6.403963745));
#118714=CARTESIAN_POINT('Ctrl Pts',(4.259815245,2.103255924,6.172841653));
#118715=CARTESIAN_POINT('Ctrl Pts',(3.237035134,2.232664075,6.487226182));
#118716=CARTESIAN_POINT('Ctrl Pts',(3.589008448,2.168401865,6.311596421));
#118717=CARTESIAN_POINT('Ctrl Pts',(3.919913471,2.103255924,6.098916164));
#118718=CARTESIAN_POINT('',(3.91595789500394,2.10403448615343,6.10145669215797));
#118719=CARTESIAN_POINT('Origin',(-0.117115990262643,2.01791771245111,-0.155955219364138));
#118720=CARTESIAN_POINT('Ctrl Pts',(4.05284566323258,2.14301213126278,6.31066098193969));
#118721=CARTESIAN_POINT('Ctrl Pts',(4.03080108980658,2.13706113288446,6.27702978339675));
#118722=CARTESIAN_POINT('Ctrl Pts',(4.00791888512396,2.1307365166235,6.24209689464461));
#118723=CARTESIAN_POINT('Ctrl Pts',(3.96150363406452,2.1175297837628,6.1711626411393));
#118724=CARTESIAN_POINT('Ctrl Pts',(3.9387074907344,2.11086978244736,6.13629175453385));
#118725=CARTESIAN_POINT('Ctrl Pts',(3.91595789307703,2.10403448653057,6.10145669334236));
#118726=CARTESIAN_POINT('Ctrl Pts',(3.837601071,2.103262031,6.443820142));
#118727=CARTESIAN_POINT('Ctrl Pts',(3.945921342,2.123129682,6.379310274));
#118728=CARTESIAN_POINT('Ctrl Pts',(4.052012211,2.142857143,6.311196166));
#118729=CARTESIAN_POINT('Ctrl Pts',(4.291764963,2.187438859,6.157266379));
#118730=CARTESIAN_POINT('Ctrl Pts',(4.519148461,2.232664075,5.985590797));
#118731=CARTESIAN_POINT('Ctrl Pts',(3.911969065,2.103262031,6.104014911));
#118732=CARTESIAN_POINT('Ctrl Pts',(4.014577229,2.123129682,6.03825492));
#118733=CARTESIAN_POINT('Ctrl Pts',(4.114917201,2.142857143,5.969083383));
#118734=CARTESIAN_POINT('Ctrl Pts',(4.341673608,2.187438859,5.812763932));
#118735=CARTESIAN_POINT('Ctrl Pts',(4.55591692,2.232664075,5.639691571));
#118736=CARTESIAN_POINT('Ctrl Pts',(4.55591691329171,2.23266407358393,5.63969157641916));
#118737=CARTESIAN_POINT('Ctrl Pts',(4.44020990789959,2.20823916035437,5.73316326695541));
#118738=CARTESIAN_POINT('Ctrl Pts',(4.32188945961225,2.18398286813883,5.82285616395298));
#118739=CARTESIAN_POINT('Ctrl Pts',(4.20133243362317,2.15996091009865,5.90857899901553));
#118740=CARTESIAN_POINT('Ctrl Pts',(4.17265211345323,2.15424612539781,5.92897232188741));
#118741=CARTESIAN_POINT('Ctrl Pts',(4.14384529634021,2.14854458596021,5.94914117258918));
#118742=CARTESIAN_POINT('Ctrl Pts',(4.11491719997479,2.14285714279844,5.96908338370675));
#118743=CARTESIAN_POINT('Ctrl Pts',(4.04944632956831,2.12998516349913,6.01421714887343));
#118744=CARTESIAN_POINT('Ctrl Pts',(3.98311124483373,2.11704095625173,6.05835719870953));
#118745=CARTESIAN_POINT('Ctrl Pts',(3.91595789925707,2.10403448771939,6.10145668921002));
#118746=CARTESIAN_POINT('Ctrl Pts',(4.901816146,2.232664075,5.67646003));
#118747=CARTESIAN_POINT('Ctrl Pts',(5.209800235,2.168401865,5.410505303));
#118748=CARTESIAN_POINT('Ctrl Pts',(5.48720162,2.103255924,5.112789687));
#118749=CARTESIAN_POINT('Ctrl Pts',(4.55591692,2.232664075,5.639691571));
#118750=CARTESIAN_POINT('Ctrl Pts',(4.861906086,2.168401865,5.392504079));
#118751=CARTESIAN_POINT('Ctrl Pts',(5.139354765,2.103255924,5.113661369));
#118752=CARTESIAN_POINT('',(5.13603780693689,2.10403448615971,5.11699283304007));
#118753=CARTESIAN_POINT('Origin',(-0.147903519018688,2.01791776476396,-0.127132470961947));
#118754=CARTESIAN_POINT('Ctrl Pts',(5.3146979529777,2.14301213129116,5.29187921908646));
#118755=CARTESIAN_POINT('Ctrl Pts',(5.28593899785615,2.13706112090324,5.26377317422809));
#118756=CARTESIAN_POINT('Ctrl Pts',(5.25608237635443,2.13073653635175,5.23457613979777));
#118757=CARTESIAN_POINT('Ctrl Pts',(5.19550343018011,2.11752978375768,5.17527810805184));
#118758=CARTESIAN_POINT('Ctrl Pts',(5.16574403856045,2.1108697824829,5.14612298051484));
#118759=CARTESIAN_POINT('Ctrl Pts',(5.13603780536316,2.10403448654035,5.11699283455561));
#118760=CARTESIAN_POINT('Ctrl Pts',(5.133110943,2.103262031,5.468196417));
#118761=CARTESIAN_POINT('Ctrl Pts',(5.22503103100001,2.123129682,5.381909097));
#118762=CARTESIAN_POINT('Ctrl Pts',(5.313999035,2.142857143,5.292581058));
#118763=CARTESIAN_POINT('Ctrl Pts',(5.51505614700001,2.187438859,5.09071031));
#118764=CARTESIAN_POINT('Ctrl Pts',(5.70021837,2.232664075,4.874167676));
#118765=CARTESIAN_POINT('Ctrl Pts',(5.132692175,2.103262031,5.120348722));
#118766=CARTESIAN_POINT('Ctrl Pts',(5.218764963,2.123129682,5.03406844200001));
#118767=CARTESIAN_POINT('Ctrl Pts',(5.301889206,2.142857143,4.944943968));
#118768=CARTESIAN_POINT('Ctrl Pts',(5.489740113,2.187438859,4.743533254));
#118769=CARTESIAN_POINT('Ctrl Pts',(5.661769094,2.232664075,4.52845125));
#118770=CARTESIAN_POINT('Ctrl Pts',(5.66176908835685,2.23266407351645,4.52845125705543));
#118771=CARTESIAN_POINT('Ctrl Pts',(5.56886090028387,2.20823916067901,4.64461121517142));
#118772=CARTESIAN_POINT('Ctrl Pts',(5.47258804156651,2.18398286888765,4.75764253910149));
#118773=CARTESIAN_POINT('Ctrl Pts',(5.3732774492891,2.15996091126762,4.86727741707001));
#118774=CARTESIAN_POINT('Ctrl Pts',(5.3496516190285,2.15424612616522,4.89335937830019));
#118775=CARTESIAN_POINT('Ctrl Pts',(5.32585399435101,2.14854458632816,4.91924930846668));
#118776=CARTESIAN_POINT('Ctrl Pts',(5.30188920503029,2.14285714276879,4.94494396917447));
#118777=CARTESIAN_POINT('Ctrl Pts',(5.24765143282067,2.12998516346269,5.0030968345205));
#118778=CARTESIAN_POINT('Ctrl Pts',(5.19235603125489,2.11704095613966,5.06046499702258));
#118779=CARTESIAN_POINT('Ctrl Pts',(5.13603781027864,2.10403448767572,5.11699282926966));
#118780=CARTESIAN_POINT('Ctrl Pts',(6.00748552,2.232664075,4.490001975));
#118781=CARTESIAN_POINT('Ctrl Pts',(6.251096707,2.168401865,4.164057646));
#118782=CARTESIAN_POINT('Ctrl Pts',(6.458012545,2.103255924,3.813669358));
#118783=CARTESIAN_POINT('Ctrl Pts',(5.661769094,2.232664075,4.52845125000001));
#118784=CARTESIAN_POINT('Ctrl Pts',(5.907466399,2.168401865,4.221264238));
#118785=CARTESIAN_POINT('Ctrl Pts',(6.11848554200001,2.103255924,3.889297452));
#118786=CARTESIAN_POINT('',(6.11596229886022,2.10403448614595,3.89326407593993));
#118787=CARTESIAN_POINT('Origin',(-0.171775416579336,2.01791771392519,-0.0923653430460797));
#118788=CARTESIAN_POINT('Ctrl Pts',(6.32804087377597,2.14301213122732,4.02565506515197));
#118789=CARTESIAN_POINT('Ctrl Pts',(6.2939123810826,2.13706113181295,4.00438848838436));
#118790=CARTESIAN_POINT('Ctrl Pts',(6.2584771297729,2.13073651823195,3.98229225490456));
#118791=CARTESIAN_POINT('Ctrl Pts',(6.18656726015707,2.11752978376512,3.93740332255265));
#118792=CARTESIAN_POINT('Ctrl Pts',(6.15123613580716,2.11086978246197,3.91532721515228));
#118793=CARTESIAN_POINT('Ctrl Pts',(6.11596229761108,2.10403448649821,3.89326407782788));
#118794=CARTESIAN_POINT('Ctrl Pts',(6.188602252,2.103262031,4.236885904));
#118795=CARTESIAN_POINT('Ctrl Pts',(6.259824077,2.123129682,4.132855832));
#118796=CARTESIAN_POINT('Ctrl Pts',(6.327509171,2.142857143,4.026490742));
#118797=CARTESIAN_POINT('Ctrl Pts',(6.480469435,2.187438859,3.786118284));
#118798=CARTESIAN_POINT('Ctrl Pts',(6.614752403,2.232664075,3.534833892));
#118799=CARTESIAN_POINT('Ctrl Pts',(6.113416303,2.103262031,3.897260718));
#118800=CARTESIAN_POINT('Ctrl Pts',(6.178929047,2.123129682,3.794494518));
#118801=CARTESIAN_POINT('Ctrl Pts',(6.240950764,2.142857143,3.68958447));
#118802=CARTESIAN_POINT('Ctrl Pts',(6.381112471,2.187438859,3.452500234));
#118803=CARTESIAN_POINT('Ctrl Pts',(6.502883238,2.232664075,3.205465582));
#118804=CARTESIAN_POINT('Ctrl Pts',(6.50288323411111,2.23266407355568,3.20546558988933));
#118805=CARTESIAN_POINT('Ctrl Pts',(6.43711819122571,2.20823917803144,3.33888221223235));
#118806=CARTESIAN_POINT('Ctrl Pts',(6.36739458367594,2.18398290322023,3.46996665495728));
#118807=CARTESIAN_POINT('Ctrl Pts',(6.29397413275033,2.159960962177,3.59838708563228));
#118808=CARTESIAN_POINT('Ctrl Pts',(6.2765074614521,2.15424616006317,3.62893821167822));
#118809=CARTESIAN_POINT('Ctrl Pts',(6.25883172995105,2.14854460328905,3.65933872608122));
#118810=CARTESIAN_POINT('Ctrl Pts',(6.24095076365543,2.14285714287543,3.68958447084559));
#118811=CARTESIAN_POINT('Ctrl Pts',(6.20048218741084,2.12998516355731,3.75803727196376));
#118812=CARTESIAN_POINT('Ctrl Pts',(6.15881202082062,2.1170409562234,3.8259510754514));
#118813=CARTESIAN_POINT('Ctrl Pts',(6.11596230129555,2.10403448764277,3.89326407151601));
#118814=CARTESIAN_POINT('Ctrl Pts',(6.832251548,2.232664075,3.093596417));
#118815=CARTESIAN_POINT('Ctrl Pts',(7.000098845,2.168401865,2.722903281));
#118816=CARTESIAN_POINT('Ctrl Pts',(7.126853981,2.103255924,2.336226088));
#118817=CARTESIAN_POINT('Ctrl Pts',(6.502883238,2.232664075,3.205465582));
#118818=CARTESIAN_POINT('Ctrl Pts',(6.676800149,2.168401865,2.852642774));
#118819=CARTESIAN_POINT('Ctrl Pts',(6.811522736,2.103255924,2.483074308));
#118820=CARTESIAN_POINT('',(6.80991119082281,2.10403448614523,2.48749061760122));
#118821=CARTESIAN_POINT('Origin',(-0.18761523090055,2.01791774112694,-0.0532792561436141));
#118822=CARTESIAN_POINT('Ctrl Pts',(7.04549163606581,2.14301213123522,2.57119575439931));
#118823=CARTESIAN_POINT('Ctrl Pts',(7.0075893623576,2.13706113168265,2.55776299520579));
#118824=CARTESIAN_POINT('Ctrl Pts',(6.96823253200764,2.13073651834497,2.54380089153319));
#118825=CARTESIAN_POINT('Ctrl Pts',(6.88835362328561,2.11752970809174,2.51541977092132));
#118826=CARTESIAN_POINT('Ctrl Pts',(6.84910305541128,2.11086974536017,2.50145502478111));
#118827=CARTESIAN_POINT('Ctrl Pts',(6.80991119013385,2.10403448647952,2.48749061958345));
#118828=CARTESIAN_POINT('Ctrl Pts',(6.954721399,2.103262031,2.807463316));
#118829=CARTESIAN_POINT('Ctrl Pts',(7.001914706,2.123129682,2.690554822));
#118830=CARTESIAN_POINT('Ctrl Pts',(7.04515201,2.142857143,2.572126194));
#118831=CARTESIAN_POINT('Ctrl Pts',(7.142863175,2.187438859,2.304491575));
#118832=CARTESIAN_POINT('Ctrl Pts',(7.219987966,2.232664075,2.030215204));
#118833=CARTESIAN_POINT('Ctrl Pts',(6.808283879,2.103262031,2.491941134));
#118834=CARTESIAN_POINT('Ctrl Pts',(6.850173276,2.123129682,2.377494247));
#118835=CARTESIAN_POINT('Ctrl Pts',(6.888192401,2.142857143,2.261704102));
#118836=CARTESIAN_POINT('Ctrl Pts',(6.974111103,2.187438859,2.00003214));
#118837=CARTESIAN_POINT('Ctrl Pts',(7.039929788,2.232664075,1.732595906));
#118838=CARTESIAN_POINT('Ctrl Pts',(7.03992978592764,2.23266407357604,1.73259591442046));
#118839=CARTESIAN_POINT('Ctrl Pts',(7.0043828991772,2.2082391610559,1.87703097072648));
#118840=CARTESIAN_POINT('Ctrl Pts',(6.96446864068666,2.18398286961989,2.02003934379038));
#118841=CARTESIAN_POINT('Ctrl Pts',(6.92037127959601,2.15996091242376,2.16124069710796));
#118842=CARTESIAN_POINT('Ctrl Pts',(6.90988058740402,2.15424612694543,2.19483227488293));
#118843=CARTESIAN_POINT('Ctrl Pts',(6.89915334705155,2.14854458673851,2.2283217045661));
#118844=CARTESIAN_POINT('Ctrl Pts',(6.88819240064526,2.14285714281593,2.26170410308038));
#118845=CARTESIAN_POINT('Ctrl Pts',(6.86338528583572,2.12998516352363,2.33725606329273));
#118846=CARTESIAN_POINT('Ctrl Pts',(6.83728880486597,2.11704095620497,2.41253993402923));
#118847=CARTESIAN_POINT('Ctrl Pts',(6.80991119222406,2.10403448758666,2.48749061268677));
#118848=CARTESIAN_POINT('Ctrl Pts',(7.337549087,2.232664075,1.552537729));
#118849=CARTESIAN_POINT('Ctrl Pts',(7.421784141,2.168401865,1.154428985));
#118850=CARTESIAN_POINT('Ctrl Pts',(7.462451646,2.103255924,0.749543483));
#118851=CARTESIAN_POINT('Ctrl Pts',(7.039929788,2.232664075,1.732595906));
#118852=CARTESIAN_POINT('Ctrl Pts',(7.133934145,2.168401865,1.350634904));
#118853=CARTESIAN_POINT('Ctrl Pts',(7.186060697,2.103255924,0.960745369));
#118854=CARTESIAN_POINT('',(7.18543620485501,2.10403448618026,0.965404863172399));
#118855=CARTESIAN_POINT('Origin',(-0.194682222779703,2.01791775279427,-0.0117018739600151));
#118856=CARTESIAN_POINT('Ctrl Pts',(7.43350303989041,2.14301213123168,0.9965101881476));
#118857=CARTESIAN_POINT('Ctrl Pts',(7.39359918050729,2.13706112069452,0.991539338668986));
#118858=CARTESIAN_POINT('Ctrl Pts',(7.35216123765767,2.13073653596577,0.986364239354941));
#118859=CARTESIAN_POINT('Ctrl Pts',(7.26804866643051,2.11752971237787,0.97581824705879));
#118860=CARTESIAN_POINT('Ctrl Pts',(7.22671373277042,2.11086974748737,0.970617699025719));
#118861=CARTESIAN_POINT('Ctrl Pts',(7.18543620457699,2.10403448656051,0.965404864875282));
#118862=CARTESIAN_POINT('Ctrl Pts',(7.395645502,2.103262031,1.246766863));
#118863=CARTESIAN_POINT('Ctrl Pts',(7.416603586,2.123129682,1.122446458));
#118864=CARTESIAN_POINT('Ctrl Pts',(7.433371371,2.142857143,0.997491884));
#118865=CARTESIAN_POINT('Ctrl Pts',(7.471264572,2.187438859,0.715109402));
#118866=CARTESIAN_POINT('Ctrl Pts',(7.487624915,2.232664075,0.43066591));
#118867=CARTESIAN_POINT('Ctrl Pts',(7.184803668,2.103262031,0.970101153));
#118868=CARTESIAN_POINT('Ctrl Pts',(7.201111017,2.123129682,0.849324988));
#118869=CARTESIAN_POINT('Ctrl Pts',(7.213349817,2.142857143,0.728068964));
#118870=CARTESIAN_POINT('Ctrl Pts',(7.241008051,2.187438859,0.454044767));
#118871=CARTESIAN_POINT('Ctrl Pts',(7.247797047,2.232664075,0.178711971));
#118872=CARTESIAN_POINT('Ctrl Pts',(7.24779704678624,2.23266407357604,0.178711979669084));
#118873=CARTESIAN_POINT('Ctrl Pts',(7.2441304941737,2.20823916217468,0.327411748160941));
#118874=CARTESIAN_POINT('Ctrl Pts',(7.23589198219421,2.18398287173784,0.475657044536055));
#118875=CARTESIAN_POINT('Ctrl Pts',(7.22317971082102,2.15996091544561,0.623036812005189));
#118876=CARTESIAN_POINT('Ctrl Pts',(7.22015548100198,2.15424612896897,0.658098232141686));
#118877=CARTESIAN_POINT('Ctrl Pts',(7.21687827448317,2.14854458776399,0.693110743211409));
#118878=CARTESIAN_POINT('Ctrl Pts',(7.21334981720885,2.14285714284448,0.728068965329833));
#118879=CARTESIAN_POINT('Ctrl Pts',(7.20536411757946,2.12998516353824,0.80718735947546));
#118880=CARTESIAN_POINT('Ctrl Pts',(7.19606156435664,2.11704095622061,0.886321106970012));
#118881=CARTESIAN_POINT('Ctrl Pts',(7.18543620520422,2.10403448763058,0.965404858045334));
#118882=CARTESIAN_POINT('Ctrl Pts',(7.499750986,2.232664075,-0.061115898));
#118883=CARTESIAN_POINT('Ctrl Pts',(7.496435059,2.168401865,-0.468025127));
#118884=CARTESIAN_POINT('Ctrl Pts',(7.449113366,2.103255924,-0.872186943));
#118885=CARTESIAN_POINT('Ctrl Pts',(7.247797047,2.232664075,0.178711971));
#118886=CARTESIAN_POINT('Ctrl Pts',(7.257493309,2.168401865,-0.214527153));
#118887=CARTESIAN_POINT('Ctrl Pts',(7.224586446,2.103255924,-0.606506955));
#118888=CARTESIAN_POINT('',(7.22497820779803,2.10403448615812,-0.60182215072398));
#118889=CARTESIAN_POINT('Origin',(-0.19264630124107,2.01791774916566,0.0304226431543164));
#118890=CARTESIAN_POINT('Ctrl Pts',(7.47393210366752,2.14301213123845,-0.624771087536083));
#118891=CARTESIAN_POINT('Ctrl Pts',(7.43389266566128,2.1370611321497,-0.621047578195944));
#118892=CARTESIAN_POINT('Ctrl Pts',(7.39231082795438,2.13073651714187,-0.617193735242821));
#118893=CARTESIAN_POINT('Ctrl Pts',(7.30789826191783,2.11752978375747,-0.609411504752216));
#118894=CARTESIAN_POINT('Ctrl Pts',(7.26641150752387,2.11086978240992,-0.605604655337827));
#118895=CARTESIAN_POINT('Ctrl Pts',(7.22497820791532,2.10403448648335,-0.601822148851471));
#118896=CARTESIAN_POINT('Ctrl Pts',(7.49075744100001,2.103262031,-0.372227023));
#118897=CARTESIAN_POINT('Ctrl Pts',(7.484500325,2.123129682,-0.498146254));
#118898=CARTESIAN_POINT('Ctrl Pts',(7.474014549,2.142857143,-0.623784038));
#118899=CARTESIAN_POINT('Ctrl Pts',(7.45031794100001,2.187438859,-0.907710493));
#118900=CARTESIAN_POINT('Ctrl Pts',(7.405148846,2.232664075,-1.189020844));
#118901=CARTESIAN_POINT('Ctrl Pts',(7.225370023,2.103262031,-0.597099681));
#118902=CARTESIAN_POINT('Ctrl Pts',(7.21533281000001,2.123129682,-0.718557763));
#118903=CARTESIAN_POINT('Ctrl Pts',(7.201219013,2.142857143,-0.839609869));
#118904=CARTESIAN_POINT('Ctrl Pts',(7.16932351,2.187438859,-1.113173236));
#118905=CARTESIAN_POINT('Ctrl Pts',(7.116765371,2.232664075,-1.383528337));
#118906=CARTESIAN_POINT('Ctrl Pts',(7.11676537265484,2.23266407357604,-1.38352832848763));
#118907=CARTESIAN_POINT('Ctrl Pts',(7.14515060543227,2.20823915451187,-1.23751683208644));
#118908=CARTESIAN_POINT('Ctrl Pts',(7.16897306784405,2.18398285663643,-1.09096634643821));
#118909=CARTESIAN_POINT('Ctrl Pts',(7.18824029892274,2.15996089312086,-0.944299428321259));
#118910=CARTESIAN_POINT('Ctrl Pts',(7.1928239362316,2.15424611408736,-0.909407649886073));
#118911=CARTESIAN_POINT('Ctrl Pts',(7.19714999795818,2.14854458029521,-0.874509254573029));
#118912=CARTESIAN_POINT('Ctrl Pts',(7.201219013176,2.14285714275399,-0.839609867490446));
#118913=CARTESIAN_POINT('Ctrl Pts',(7.21042813048085,2.12998516345522,-0.760624528096376));
#118914=CARTESIAN_POINT('Ctrl Pts',(7.21835448240667,2.11704095613337,-0.681341109868308));
#118915=CARTESIAN_POINT('Ctrl Pts',(7.2249782070012,2.10403448753746,-0.601822155615398));
#118916=CARTESIAN_POINT('Ctrl Pts',(7.311272864,2.232664075,-1.671911813));
#118917=CARTESIAN_POINT('Ctrl Pts',(7.22056100600001,2.168401865,-2.068594904));
#118918=CARTESIAN_POINT('Ctrl Pts',(7.087462824,2.103255924,-2.453134876));
#118919=CARTESIAN_POINT('Ctrl Pts',(7.11676537100001,2.232664075,-1.383528337));
#118920=CARTESIAN_POINT('Ctrl Pts',(7.041700152,2.168401865,-1.769658159));
#118921=CARTESIAN_POINT('Ctrl Pts',(6.925298563,2.103255924,-2.145399688));
#118922=CARTESIAN_POINT('',(6.9266882593708,2.10403448615338,-2.14090862880051));
#118923=CARTESIAN_POINT('Origin',(-0.181602426183516,2.01791772037682,0.0711246562100257));
#118924=CARTESIAN_POINT('Ctrl Pts',(7.16488840885302,2.1430121312558,-2.21683876058331));
#118925=CARTESIAN_POINT('Ctrl Pts',(7.12658551329033,2.13706113188681,-2.20459500866285));
#118926=CARTESIAN_POINT('Ctrl Pts',(7.0868043014371,2.13073651737911,-2.19189240173367));
#118927=CARTESIAN_POINT('Ctrl Pts',(7.00603766334665,2.11752969561696,-2.16614573670162));
#118928=CARTESIAN_POINT('Ctrl Pts',(6.96633949502101,2.11086973926319,-2.15350955562722));
#118929=CARTESIAN_POINT('Ctrl Pts',(6.92668826047007,2.10403448652366,-2.14090862668333));
#118930=CARTESIAN_POINT('Ctrl Pts',(7.235609888,2.103262031,-1.973815986));
#118931=CARTESIAN_POINT('Ctrl Pts',(7.202430147,2.123129682,-2.095446201));
#118932=CARTESIAN_POINT('Ctrl Pts',(7.165181113,2.142857143,-2.215892511));
#118933=CARTESIAN_POINT('Ctrl Pts',(7.081002724,2.187438859,-2.488086853));
#118934=CARTESIAN_POINT('Ctrl Pts',(6.976416247,2.232664075,-2.753110305));
#118935=CARTESIAN_POINT('Ctrl Pts',(6.928086106,2.103262031,-2.136380796));
#118936=CARTESIAN_POINT('Ctrl Pts',(6.892173659,2.123129682,-2.252841553));
#118937=CARTESIAN_POINT('Ctrl Pts',(6.852367211,2.142857143,-2.368029478));
#118938=CARTESIAN_POINT('Ctrl Pts',(6.76240936900001,2.187438859,-2.628340495));
#118939=CARTESIAN_POINT('Ctrl Pts',(6.652961655,2.232664075,-2.881076398));
#118940=CARTESIAN_POINT('Ctrl Pts',(6.65296165844605,2.23266407357604,-2.88107639004239));
#118941=CARTESIAN_POINT('Ctrl Pts',(6.71207139004059,2.20823916520409,-2.74458060686293));
#118942=CARTESIAN_POINT('Ctrl Pts',(6.7668408976219,2.18398287772463,-2.60657757543584));
#118943=CARTESIAN_POINT('Ctrl Pts',(6.81718670611509,2.15996092424679,-2.46748159380732));
#118944=CARTESIAN_POINT('Ctrl Pts',(6.82916390418536,2.15424613480453,-2.43439085253997));
#118945=CARTESIAN_POINT('Ctrl Pts',(6.84089097018248,2.14854459064272,-2.40123827769394));
#118946=CARTESIAN_POINT('Ctrl Pts',(6.85236721156548,2.14285714277589,-2.36802947663634));
#118947=CARTESIAN_POINT('Ctrl Pts',(6.87834053749264,2.12998516342169,-2.29287045888821));
#118948=CARTESIAN_POINT('Ctrl Pts',(6.90312516711685,2.11704095609726,-2.21714457406265));
#118949=CARTESIAN_POINT('Ctrl Pts',(6.92668825783225,2.10403448760368,-2.14090863337329));
#118950=CARTESIAN_POINT('Ctrl Pts',(6.780927749,2.232664075,-3.20453099));
#118951=CARTESIAN_POINT('Ctrl Pts',(6.60706154500001,2.168401865,-3.572439483));
#118952=CARTESIAN_POINT('Ctrl Pts',(6.39441039699999,2.103255924,-3.919376949));
#118953=CARTESIAN_POINT('Ctrl Pts',(6.65296165500001,2.232664075,-2.881076398));
#118954=CARTESIAN_POINT('Ctrl Pts',(6.496644922,2.168401865,-3.242041916));
#118955=CARTESIAN_POINT('Ctrl Pts',(6.302191415,2.103255924,-3.583975916));
#118956=CARTESIAN_POINT('',(6.30451406692602,2.10403448613635,-3.57988859897104));
#118957=CARTESIAN_POINT('Origin',(-0.162066820169903,2.01791775098821,0.108500875694056));
#118958=CARTESIAN_POINT('Ctrl Pts',(6.52082249472584,2.1430121312108,-3.70524951776582));
#118959=CARTESIAN_POINT('Ctrl Pts',(6.48604707792739,2.13706112048613,-3.68505798914409));
#118960=CARTESIAN_POINT('Ctrl Pts',(6.44992678160988,2.13073653562651,-3.6641006748843));
#118961=CARTESIAN_POINT('Ctrl Pts',(6.37658358245868,2.11752978372462,-3.62159373779538));
#118962=CARTESIAN_POINT('Ctrl Pts',(6.34052967847826,2.11086978237466,-3.60071889880975));
#118963=CARTESIAN_POINT('Ctrl Pts',(6.3045140674439,2.1040344864438,-3.57988859797476));
#118964=CARTESIAN_POINT('Ctrl Pts',(6.642133258,2.103262031,-3.483111508));
#118965=CARTESIAN_POINT('Ctrl Pts',(6.58358234,2.123129682,-3.594765413));
#118966=CARTESIAN_POINT('Ctrl Pts',(6.521311771,2.142857143,-3.704388314));
#118967=CARTESIAN_POINT('Ctrl Pts',(6.380587689,2.187438859,-3.952123038));
#118968=CARTESIAN_POINT('Ctrl Pts',(6.221474178,2.232664075,-4.188467387));
#118969=CARTESIAN_POINT('Ctrl Pts',(6.306852583,2.103262031,-3.575767121));
#118970=CARTESIAN_POINT('Ctrl Pts',(6.246744129,2.123129682,-3.681784975));
#118971=CARTESIAN_POINT('Ctrl Pts',(6.183106334,2.142857143,-3.785722661));
#118972=CARTESIAN_POINT('Ctrl Pts',(6.039292483,2.187438859,-4.020609474));
#118973=CARTESIAN_POINT('Ctrl Pts',(5.878072847,2.232664075,-4.243908529));
#118974=CARTESIAN_POINT('Ctrl Pts',(5.87807285211789,2.23266407356433,-4.24390852191141));
#118975=CARTESIAN_POINT('Ctrl Pts',(5.96514322424147,2.20823915554531,-4.12331073155852));
#118976=CARTESIAN_POINT('Ctrl Pts',(6.04829885431209,2.18398285863974,-4.00030791039458));
#118977=CARTESIAN_POINT('Ctrl Pts',(6.12736915752677,2.15996089602006,-3.87528672607273));
#118978=CARTESIAN_POINT('Ctrl Pts',(6.14617983486012,2.15424611601566,-3.84554442001723));
#118979=CARTESIAN_POINT('Ctrl Pts',(6.16475952120855,2.14854458125394,-3.81568795542351));
#118980=CARTESIAN_POINT('Ctrl Pts',(6.18310633482256,2.14285714274501,-3.78572265965654));
#118981=CARTESIAN_POINT('Ctrl Pts',(6.22462938632703,2.1299851634521,-3.71790431536696));
#118982=CARTESIAN_POINT('Ctrl Pts',(6.26511339219194,2.11704095609181,-3.64927682231));
#118983=CARTESIAN_POINT('Ctrl Pts',(6.30451406510162,2.1040344874241,-3.57988860303163));
#118984=CARTESIAN_POINT('Ctrl Pts',(5.933513989,2.232664075,-4.587309859));
#118985=CARTESIAN_POINT('Ctrl Pts',(5.684623229,2.168401865,-4.909240762));
#118986=CARTESIAN_POINT('Ctrl Pts',(5.402362448,2.103255924,-5.202353312));
#118987=CARTESIAN_POINT('Ctrl Pts',(5.878072847,2.232664075,-4.243908529));
#118988=CARTESIAN_POINT('Ctrl Pts',(5.647813796,2.168401865,-4.562831397));
#118989=CARTESIAN_POINT('Ctrl Pts',(5.384400802,2.103255924,-4.854969413));
#118990=CARTESIAN_POINT('',(5.38754780319582,2.10403448614009,-4.85147695721227));
#118991=CARTESIAN_POINT('Origin',(-0.134953223403402,2.01791771288928,0.140803705752561));
#118992=CARTESIAN_POINT('Ctrl Pts',(5.57185016888731,2.14301213123745,-5.02040692549819));
#118993=CARTESIAN_POINT('Ctrl Pts',(5.54222842210557,2.13706113221689,-4.99321183034187));
#118994=CARTESIAN_POINT('Ctrl Pts',(5.51145765309236,2.13073651663086,-4.96497955430377));
#118995=CARTESIAN_POINT('Ctrl Pts',(5.44896662714916,2.11752970447619,-4.90769952435097));
#118996=CARTESIAN_POINT('Ctrl Pts',(5.41824331752903,2.11086974357807,-4.8795623880085));
#118997=CARTESIAN_POINT('Ctrl Pts',(5.38754780472493,2.10403448646141,-4.85147695546285));
#118998=CARTESIAN_POINT('Ctrl Pts',(5.73807786,2.103262031,-4.829540607));
#118999=CARTESIAN_POINT('Ctrl Pts',(5.656893541,2.123129682,-4.92599738900001));
#119000=CARTESIAN_POINT('Ctrl Pts',(5.57251314,2.142857143,-5.019671036));
#119001=CARTESIAN_POINT('Ctrl Pts',(5.38182346500001,2.187438859,-5.231362342));
#119002=CARTESIAN_POINT('Ctrl Pts',(5.17562289100001,2.232664075,-5.42797639));
#119003=CARTESIAN_POINT('Ctrl Pts',(5.39071764200001,2.103262031,-4.847954548));
#119004=CARTESIAN_POINT('Ctrl Pts',(5.309223786,2.123129682,-4.93857222300001));
#119005=CARTESIAN_POINT('Ctrl Pts',(5.224730277,2.142857143,-5.026399659));
#119006=CARTESIAN_POINT('Ctrl Pts',(5.033784992,2.187438859,-5.224879222));
#119007=CARTESIAN_POINT('Ctrl Pts',(4.828331886,2.232664075,-5.40830021300001));
#119008=CARTESIAN_POINT('Ctrl Pts',(4.82833189246886,2.23266407357604,-5.40830020722484));
#119009=CARTESIAN_POINT('Ctrl Pts',(4.93929153811201,2.20823916200544,-5.30923950860549));
#119010=CARTESIAN_POINT('Ctrl Pts',(5.04694497896374,2.18398287142066,-5.20698845514794));
#119011=CARTESIAN_POINT('Ctrl Pts',(5.15104249613844,2.15996091496511,-5.10188800353165));
#119012=CARTESIAN_POINT('Ctrl Pts',(5.17580713464865,2.1542461286371,-5.07688476846726));
#119013=CARTESIAN_POINT('Ctrl Pts',(5.20037072289607,2.14854458757901,-5.05172038722873));
#119014=CARTESIAN_POINT('Ctrl Pts',(5.22473027788515,2.14285714280411,-5.026399658127));
#119015=CARTESIAN_POINT('Ctrl Pts',(5.2798614829953,2.12998516349225,-4.96909309752418));
#119016=CARTESIAN_POINT('Ctrl Pts',(5.33415187731937,2.11704095622504,-4.91077294193982));
#119017=CARTESIAN_POINT('Ctrl Pts',(5.3875477996425,2.10403448764827,-4.85147696088472));
#119018=CARTESIAN_POINT('Ctrl Pts',(4.808655709,2.232664075,-5.755591218));
#119019=CARTESIAN_POINT('Ctrl Pts',(4.49637825,2.168401865,-6.016491399));
#119020=CARTESIAN_POINT('Ctrl Pts',(4.157706034,2.103255924,-6.242073416));
#119021=CARTESIAN_POINT('Ctrl Pts',(4.828331886,2.232664075,-5.408300213));
#119022=CARTESIAN_POINT('Ctrl Pts',(4.534897174,2.168401865,-5.670267952));
#119023=CARTESIAN_POINT('Ctrl Pts',(4.214841591,2.103255924,-5.89894993700001));
#119024=CARTESIAN_POINT('',(4.21866579235029,2.10403448613268,-5.89621564507842));
#119025=CARTESIAN_POINT('Origin',(-0.10152958199823,2.0179177372351,0.16652289096133));
#119026=CARTESIAN_POINT('Ctrl Pts',(4.36234432157512,2.14301213124375,-6.10081568470611));
#119027=CARTESIAN_POINT('Ctrl Pts',(4.33926125518818,2.13706113194744,-6.06788859432327));
#119028=CARTESIAN_POINT('Ctrl Pts',(4.31527899933983,2.13073651770443,-6.03370157478219));
#119029=CARTESIAN_POINT('Ctrl Pts',(4.26656278041319,2.11752978376772,-5.96432740782818));
#119030=CARTESIAN_POINT('Ctrl Pts',(4.24260626070986,2.11086978241002,-5.93024327565625));
#119031=CARTESIAN_POINT('Ctrl Pts',(4.21866579364788,2.10403448646565,-5.8962156440986));
#119032=CARTESIAN_POINT('Ctrl Pts',(4.56571631700001,2.103262031,-5.950145755));
#119033=CARTESIAN_POINT('Ctrl Pts',(4.465694686,2.123129682,-6.026895202));
#119034=CARTESIAN_POINT('Ctrl Pts',(4.363149987,2.142857143,-6.100239519));
#119035=CARTESIAN_POINT('Ctrl Pts',(4.131411158,2.187438859,-6.265988957));
#119036=CARTESIAN_POINT('Ctrl Pts',(3.88776523,2.232664075,-6.41367925));
#119037=CARTESIAN_POINT('Ctrl Pts',(4.222518736,2.103262031,-5.89345701));
#119038=CARTESIAN_POINT('Ctrl Pts',(4.123450039,2.123129682,-5.964437323));
#119039=CARTESIAN_POINT('Ctrl Pts',(4.022051639,2.142857143,-6.032047796));
#119040=CARTESIAN_POINT('Ctrl Pts',(3.79290331,2.187438859,-6.184839426));
#119041=CARTESIAN_POINT('Ctrl Pts',(3.552823492,2.232664075,-6.319805791));
#119042=CARTESIAN_POINT('Ctrl Pts',(3.55282349975592,2.23266407353897,-6.31980578663983));
#119043=CARTESIAN_POINT('Ctrl Pts',(3.68248410597432,2.20823915946357,-6.24691410877597));
#119044=CARTESIAN_POINT('Ctrl Pts',(3.80960163581233,2.18398286641657,-6.17019592741199));
#119045=CARTESIAN_POINT('Ctrl Pts',(3.93385891325753,2.15996090757301,-6.08993054588538));
#119046=CARTESIAN_POINT('Ctrl Pts',(3.96341951185059,2.15424612371975,-6.07083554579355));
#119047=CARTESIAN_POINT('Ctrl Pts',(3.99281840242606,2.14854458512651,-6.05153994733617));
#119048=CARTESIAN_POINT('Ctrl Pts',(4.02205164024343,2.14285714280556,-6.03204779538241));
#119049=CARTESIAN_POINT('Ctrl Pts',(4.08821312487487,2.12998516350552,-5.98793260951333));
#119050=CARTESIAN_POINT('Ctrl Pts',(4.15377134973306,2.11704095621315,-5.94264677680663));
#119051=CARTESIAN_POINT('Ctrl Pts',(4.21866578869385,2.10403448753419,-5.89621564797567));
#119052=CARTESIAN_POINT('Ctrl Pts',(3.458950033,2.232664075,-6.65474752900001));
#119053=CARTESIAN_POINT('Ctrl Pts',(3.09788762,2.168401865,-6.842417585));
#119054=CARTESIAN_POINT('Ctrl Pts',(2.718639907,2.103255924,-6.989921105));
#119055=CARTESIAN_POINT('Ctrl Pts',(3.552823492,2.232664075,-6.319805791));
#119056=CARTESIAN_POINT('Ctrl Pts',(3.2099338,2.168401865,-6.51256908));
#119057=CARTESIAN_POINT('Ctrl Pts',(2.848201072,2.103255924,-6.667102118));
#119058=CARTESIAN_POINT('',(2.85252365806424,2.10403448616781,-6.66525384222965));
#119059=CARTESIAN_POINT('Origin',(-0.0633584653971375,2.01791772718142,
0.184455723869529));
#119060=CARTESIAN_POINT('Ctrl Pts',(2.94886010157405,2.14301213123103,-6.89595708377018));
#119061=CARTESIAN_POINT('Ctrl Pts',(2.93339505702871,2.13706113248801,-6.85883763699611));
#119062=CARTESIAN_POINT('Ctrl Pts',(2.91732268763611,2.13073651658488,-6.82029440453739));
#119063=CARTESIAN_POINT('Ctrl Pts',(2.88465882512707,2.11752978380204,-6.74206962658952));
#119064=CARTESIAN_POINT('Ctrl Pts',(2.86858947662357,2.11086978246595,-6.70363241887223));
#119065=CARTESIAN_POINT('Ctrl Pts',(2.85252365959982,2.10403448655234,-6.66525384151835));
#119066=CARTESIAN_POINT('Ctrl Pts',(3.179866955,2.103262031,-6.792528701));
#119067=CARTESIAN_POINT('Ctrl Pts',(3.065684911,2.123129682,-6.845982094));
#119068=CARTESIAN_POINT('Ctrl Pts',(2.94977079,2.142857143,-6.895567583));
#119069=CARTESIAN_POINT('Ctrl Pts',(2.687818656,2.187438859,-7.007624892));
#119070=CARTESIAN_POINT('Ctrl Pts',(2.418119987,2.232664075,-7.099485596));
#119071=CARTESIAN_POINT('Ctrl Pts',(2.856879547,2.103262031,-6.663387971));
#119072=CARTESIAN_POINT('Ctrl Pts',(2.744868352,2.123129682,-6.711411963));
#119073=CARTESIAN_POINT('Ctrl Pts',(2.631306337,2.142857143,-6.755644082));
#119074=CARTESIAN_POINT('Ctrl Pts',(2.374669684,2.187438859,-6.855603411));
#119075=CARTESIAN_POINT('Ctrl Pts',(2.11118902,2.232664075,-6.93580427400001));
#119076=CARTESIAN_POINT('Ctrl Pts',(2.11118902852914,2.23266407353601,-6.93580427140382));
#119077=CARTESIAN_POINT('Ctrl Pts',(2.25348776161027,2.20823916567505,-6.89248996866132));
#119078=CARTESIAN_POINT('Ctrl Pts',(2.3941254605974,2.18398287874681,-6.84489194029667));
#119079=CARTESIAN_POINT('Ctrl Pts',(2.53273232253612,2.15996092583572,-6.79321477552511));
#119080=CARTESIAN_POINT('Ctrl Pts',(2.56570670678256,2.15424613585664,-6.78092084819633));
#119081=CARTESIAN_POINT('Ctrl Pts',(2.59856628612993,2.148544591162,-6.76839624943633));
#119082=CARTESIAN_POINT('Ctrl Pts',(2.63130633851113,2.1428571427663,-6.75564408154887));
#119083=CARTESIAN_POINT('Ctrl Pts',(2.70540446514762,2.12998516346204,-6.7267830475775));
#119084=CARTESIAN_POINT('Ctrl Pts',(2.77916509043874,2.11704095622701,-6.69664905294933));
#119085=CARTESIAN_POINT('Ctrl Pts',(2.85252365304596,2.10403448768073,-6.66525384416611));
#119086=CARTESIAN_POINT('Ctrl Pts',(1.947507698,2.232664075,-7.242735241));
#119087=CARTESIAN_POINT('Ctrl Pts',(1.554543209,2.168401865,-7.34839993));
#119088=CARTESIAN_POINT('Ctrl Pts',(1.1524532,2.103255924,-7.410927852));
#119089=CARTESIAN_POINT('Ctrl Pts',(2.11118902,2.232664075,-6.935804274));
#119090=CARTESIAN_POINT('Ctrl Pts',(1.73487749,2.168401865,-7.050349716));
#119091=CARTESIAN_POINT('Ctrl Pts',(1.348381837,2.103255924,-7.123508014));
#119092=CARTESIAN_POINT('',(1.35300068745991,2.10403448615076,-7.12263217777289));
#119093=CARTESIAN_POINT('Origin',(-0.0222246460937434,2.01791773180016,
0.193763435003071));
#119094=CARTESIAN_POINT('Ctrl Pts',(1.39749046141378,2.14301213120456,-7.36865119365262));
#119095=CARTESIAN_POINT('Ctrl Pts',(1.3903665633665,2.13706113123047,-7.32907504328819));
#119096=CARTESIAN_POINT('Ctrl Pts',(1.38295561590674,2.13073651802702,-7.28797786324355));
#119097=CARTESIAN_POINT('Ctrl Pts',(1.36787133931593,2.11752970466789,-7.20455966330647));
#119098=CARTESIAN_POINT('Ctrl Pts',(1.36044059487456,2.11086974367532,-7.16356692879696));
#119099=CARTESIAN_POINT('Ctrl Pts',(1.35300068947363,2.10403448647302,-7.12263217749919));
#119100=CARTESIAN_POINT('Ctrl Pts',(1.645330548,2.103262031,-7.317300553));
#119101=CARTESIAN_POINT('Ctrl Pts',(1.522327117,2.123129682,-7.344958472));
#119102=CARTESIAN_POINT('Ctrl Pts',(1.398463589,2.142857143,-7.36846657));
#119103=CARTESIAN_POINT('Ctrl Pts',(1.118546742,2.187438859,-7.421592076));
#119104=CARTESIAN_POINT('Ctrl Pts',(0.835406142,2.232664075,-7.45332788600001));
#119105=CARTESIAN_POINT('Ctrl Pts',(1.357655845,2.103262031,-7.121746317));
#119106=CARTESIAN_POINT('Ctrl Pts',(1.237939671,2.123129682,-7.14456843900001));
#119107=CARTESIAN_POINT('Ctrl Pts',(1.117524075,2.142857143,-7.163353959));
#119108=CARTESIAN_POINT('Ctrl Pts',(0.845399144,2.187438859,-7.205807));
#119109=CARTESIAN_POINT('Ctrl Pts',(0.570837696,2.232664075,-7.227492257));
#119110=CARTESIAN_POINT('Ctrl Pts',(0.570837704799485,2.23266407355057,
-7.22749225630501));
#119111=CARTESIAN_POINT('Ctrl Pts',(0.719120844582198,2.20823916949319,
-7.21578064104272));
#119112=CARTESIAN_POINT('Ctrl Pts',(0.866702658605281,2.18398288628028,
-7.19952837926755));
#119113=CARTESIAN_POINT('Ctrl Pts',(1.01317800933121,2.15996093704372,-7.17885578073409));
#119114=CARTESIAN_POINT('Ctrl Pts',(1.04802432438135,2.15424614334589,-7.17393779366096));
#119115=CARTESIAN_POINT('Ctrl Pts',(1.08280810605537,2.14854459495148,-7.16876984815762));
#119116=CARTESIAN_POINT('Ctrl Pts',(1.11752407577372,2.14285714287763,-7.16335395890305));
#119117=CARTESIAN_POINT('Ctrl Pts',(1.19609409852967,2.12998516356796,-7.15109658704414));
#119118=CARTESIAN_POINT('Ctrl Pts',(1.2746081595671,2.11704095627861,-7.13752346249769));
#119119=CARTESIAN_POINT('Ctrl Pts',(1.35300068233045,2.10403448759796,-7.12263217854009));
#119120=CARTESIAN_POINT('Ctrl Pts',(0.345002067,2.232664075,-7.492060703));
#119121=CARTESIAN_POINT('Ctrl Pts',(-0.061489915,2.168401865,-7.510779261));
#119122=CARTESIAN_POINT('Ctrl Pts',(-0.467620938,2.103255924,-7.485407848));
#119123=CARTESIAN_POINT('Ctrl Pts',(0.570837696,2.232664075,-7.227492257));
#119124=CARTESIAN_POINT('Ctrl Pts',(0.178700236,2.168401865,-7.258463836));
#119125=CARTESIAN_POINT('Ctrl Pts',(-0.214486235,2.103255924,-7.246826592));
#119126=CARTESIAN_POINT('',(-0.209787091421739,2.10403448613548,-7.24696414904864));
#119127=CARTESIAN_POINT('Origin',(0.0199483692145396,2.01791774013504,0.19401068436918));
#119128=CARTESIAN_POINT('Ctrl Pts',(-0.219224279818263,2.14301213120524,
-7.49679536283724));
#119129=CARTESIAN_POINT('Ctrl Pts',(-0.217673919736163,2.13706111995674,
-7.45661297729562));
#119130=CARTESIAN_POINT('Ctrl Pts',(-0.216076931763984,2.13073653540574,
-7.41488367955731));
#119131=CARTESIAN_POINT('Ctrl Pts',(-0.212876114293857,2.11752978377184,
-7.3301734731909));
#119132=CARTESIAN_POINT('Ctrl Pts',(-0.211320895472153,2.11086978240037,
-7.28854146381932));
#119133=CARTESIAN_POINT('Ctrl Pts',(-0.209787090011732,2.10403448647094,
-7.2469641490455));
#119134=CARTESIAN_POINT('Ctrl Pts',(0.033860313,2.103262031,-7.499923565));
#119135=CARTESIAN_POINT('Ctrl Pts',(-0.092213001,2.123129682,-7.500492755));
#119136=CARTESIAN_POINT('Ctrl Pts',(-0.218234215,2.142857143,-7.496824249));
#119137=CARTESIAN_POINT('Ctrl Pts',(-0.503027175,2.187438859,-7.488533863));
#119138=CARTESIAN_POINT('Ctrl Pts',(-0.786370366,2.232664075,-7.458660848));
#119139=CARTESIAN_POINT('Ctrl Pts',(-0.205050335,2.103262031,-7.247099721));
#119140=CARTESIAN_POINT('Ctrl Pts',(-0.326873693,2.123129682,-7.243652835));
#119141=CARTESIAN_POINT('Ctrl Pts',(-0.448512371,2.142857143,-7.236113367));
#119142=CARTESIAN_POINT('Ctrl Pts',(-0.723401321,2.187438859,-7.21907506300001));
#119143=CARTESIAN_POINT('Ctrl Pts',(-0.996205364,2.232664075,-7.181230735));
#119144=CARTESIAN_POINT('Ctrl Pts',(-0.996205355809929,2.23266407364226,
-7.18123073613615));
#119145=CARTESIAN_POINT('Ctrl Pts',(-0.848871309784289,2.20823916417171,
-7.20166942852254));
#119146=CARTESIAN_POINT('Ctrl Pts',(-0.701246087786972,2.18398287560745,
-7.21752286603136));
#119147=CARTESIAN_POINT('Ctrl Pts',(-0.553751218670259,2.15996092105231,
-7.22882145264826));
#119148=CARTESIAN_POINT('Ctrl Pts',(-0.518662401800881,2.15424613267169,
-7.23150937012673));
#119149=CARTESIAN_POINT('Ctrl Pts',(-0.483580922611584,2.14854458956584,
-7.23393973070297));
#119150=CARTESIAN_POINT('Ctrl Pts',(-0.448512369351866,2.14285714274861,
-7.23611336720714));
#119151=CARTESIAN_POINT('Ctrl Pts',(-0.369144296888193,2.12998516335947,
-7.2410327977486));
#119152=CARTESIAN_POINT('Ctrl Pts',(-0.289548030983509,2.11704095615912,
-7.24465520746409));
#119153=CARTESIAN_POINT('Ctrl Pts',(-0.209787096109261,2.10403448751812,
-7.24696414920313));
#119154=CARTESIAN_POINT('Ctrl Pts',(-1.273635477,2.232664075,-7.391065733));
#119155=CARTESIAN_POINT('Ctrl Pts',(-1.674647839,2.168401865,-7.321962901));
#119156=CARTESIAN_POINT('Ctrl Pts',(-2.065829641,2.103255924,-7.209878494));
#119157=CARTESIAN_POINT('Ctrl Pts',(-0.996205363999999,2.232664075,-7.181230735));
#119158=CARTESIAN_POINT('Ctrl Pts',(-1.385832842,2.168401865,-7.127180253));
#119159=CARTESIAN_POINT('Ctrl Pts',(-1.767325168,2.103255924,-7.031291613));
#119160=CARTESIAN_POINT('',(-1.76276545949674,2.10403448615187,-7.03243613115166));
#119161=CARTESIAN_POINT('Origin',(0.0611885772422269,2.01791773077624,0.185186671872305));
#119162=CARTESIAN_POINT('Ctrl Pts',(-1.82568833719172,2.14301213121992,
-7.27439771327462));
#119163=CARTESIAN_POINT('Ctrl Pts',(-1.81553619967466,2.13706112066952,
-7.23548805575916));
#119164=CARTESIAN_POINT('Ctrl Pts',(-1.80500598344183,2.13073653646983,
-7.19507767308385));
#119165=CARTESIAN_POINT('Ctrl Pts',(-1.78366980731394,2.11752978372427,
-7.11303601874195));
#119166=CARTESIAN_POINT('Ctrl Pts',(-1.77320129741869,2.11086978243029,
-7.07271166924485));
#119167=CARTESIAN_POINT('Ctrl Pts',(-1.76276545739217,2.10403448650513,
-7.03243613163703));
#119168=CARTESIAN_POINT('Ctrl Pts',(-1.579193193,2.103262031,-7.331858486));
#119169=CARTESIAN_POINT('Ctrl Pts',(-1.702441341,2.123129682,-7.305312333));
#119170=CARTESIAN_POINT('Ctrl Pts',(-1.824727629,2.142857143,-7.274638759));
#119171=CARTESIAN_POINT('Ctrl Pts',(-2.1010801,2.187438859,-7.20532013));
#119172=CARTESIAN_POINT('Ctrl Pts',(-2.37137707,2.232664075,-7.115235119));
#119173=CARTESIAN_POINT('Ctrl Pts',(-1.758168589,2.103262031,-7.03358679600001));
#119174=CARTESIAN_POINT('Ctrl Pts',(-1.876402807,2.123129682,-7.004032076));
#119175=CARTESIAN_POINT('Ctrl Pts',(-1.993576877,2.142857143,-6.970520155));
#119176=CARTESIAN_POINT('Ctrl Pts',(-2.258376345,2.187438859,-6.894787199));
#119177=CARTESIAN_POINT('Ctrl Pts',(-2.516666969,2.232664075,-6.799182846));
#119178=CARTESIAN_POINT('Ctrl Pts',(-2.51666696086751,2.23266407357605,
-6.79918284901019));
#119179=CARTESIAN_POINT('Ctrl Pts',(-2.37717117474474,2.20823915657027,
-6.85081617631785));
#119180=CARTESIAN_POINT('Ctrl Pts',(-2.23640532564656,2.18398286067009,
-6.89803404054907));
#119181=CARTESIAN_POINT('Ctrl Pts',(-2.09478762344738,2.15996089904969,
-6.94077551930649));
#119182=CARTESIAN_POINT('Ctrl Pts',(-2.06109702949982,2.15424611804273,
-6.95094363941559));
#119183=CARTESIAN_POINT('Ctrl Pts',(-2.02735823470697,2.14854458228384,
-6.96085864743894));
#119184=CARTESIAN_POINT('Ctrl Pts',(-1.99357687567617,2.14285714278373,
-6.97052015543815));
#119185=CARTESIAN_POINT('Ctrl Pts',(-1.91712191750664,2.12998516346973,
-6.99238636286277));
#119186=CARTESIAN_POINT('Ctrl Pts',(-1.8401652780448,2.11704095609638,-7.01303492728226));
#119187=CARTESIAN_POINT('Ctrl Pts',(-1.76276546417599,2.10403448765243,
-7.0324361299985));
#119188=CARTESIAN_POINT('Ctrl Pts',(-2.832719242,2.232664075,-6.94447274400001));
#119189=CARTESIAN_POINT('Ctrl Pts',(-3.209501092,2.168401865,-6.790779694));
#119190=CARTESIAN_POINT('Ctrl Pts',(-3.567442445,2.103255924,-6.597223234));
#119191=CARTESIAN_POINT('Ctrl Pts',(-2.516666969,2.232664075,-6.79918284600001));
#119192=CARTESIAN_POINT('Ctrl Pts',(-2.885565917,2.168401865,-6.662637643));
#119193=CARTESIAN_POINT('Ctrl Pts',(-3.237525941,2.103255924,-6.486981253));
#119194=CARTESIAN_POINT('',(-3.23331887357527,2.10403448611767,-6.48907921541247));
#119195=CARTESIAN_POINT('Origin',(0.0995677333265954,2.01791771040135,0.167703467424962));
#119196=CARTESIAN_POINT('Ctrl Pts',(-3.34678523697546,2.14301213127202,
-6.71185731172976));
#119197=CARTESIAN_POINT('Ctrl Pts',(-3.32850605734533,2.13706113135863,
-6.67603981394334));
#119198=CARTESIAN_POINT('Ctrl Pts',(-3.30953490584366,2.13073651740591,
-6.63883771552103));
#119199=CARTESIAN_POINT('Ctrl Pts',(-3.2710610826908,2.11752978374566,-6.56330090580391));
#119200=CARTESIAN_POINT('Ctrl Pts',(-3.25216877742398,2.11086978240132,
-6.52616973707515));
#119201=CARTESIAN_POINT('Ctrl Pts',(-3.23331887183686,2.10403448644393,
-6.48907921623583));
#119202=CARTESIAN_POINT('Ctrl Pts',(-3.11840538,2.103262031,-6.820963853));
#119203=CARTESIAN_POINT('Ctrl Pts',(-3.233065417,2.123129682,-6.768543626));
#119204=CARTESIAN_POINT('Ctrl Pts',(-3.345898807,2.142857143,-6.712299246));
#119205=CARTESIAN_POINT('Ctrl Pts',(-3.600888855,2.187438859,-6.585193635));
#119206=CARTESIAN_POINT('Ctrl Pts',(-3.845500817,2.232664075,-6.439108903));
#119207=CARTESIAN_POINT('Ctrl Pts',(-3.229076835,2.103262031,-6.491191169));
#119208=CARTESIAN_POINT('Ctrl Pts',(-3.33819341,2.123129682,-6.436910561));
#119209=CARTESIAN_POINT('Ctrl Pts',(-3.445423944,2.142857143,-6.378993169));
#119210=CARTESIAN_POINT('Ctrl Pts',(-3.6877522,2.187438859,-6.248106749));
#119211=CARTESIAN_POINT('Ctrl Pts',(-3.919452023,2.232664075,-6.09921272300001));
#119212=CARTESIAN_POINT('Ctrl Pts',(-3.91945201577089,2.23266407358896,
-6.09921272764555));
#119213=CARTESIAN_POINT('Ctrl Pts',(-3.79431723693095,2.20823916327371,
-6.17962634524914));
#119214=CARTESIAN_POINT('Ctrl Pts',(-3.66699289525697,2.18398287387826,
-6.25600075962498));
#119215=CARTESIAN_POINT('Ctrl Pts',(-3.53787432629011,2.15996091850635,
-6.32818656929695));
#119216=CARTESIAN_POINT('Ctrl Pts',(-3.50715721036665,2.15424613097601,
-6.34535946628199));
#119217=CARTESIAN_POINT('Ctrl Pts',(-3.47633860863562,2.14854458871641,
-6.36229553001448));
#119218=CARTESIAN_POINT('Ctrl Pts',(-3.44542394254845,2.14285714274096,
-6.37899316990622));
#119219=CARTESIAN_POINT('Ctrl Pts',(-3.37545704587549,2.12998516332753,
-6.41678371346767));
#119220=CARTESIAN_POINT('Ctrl Pts',(-3.3047384418402,2.11704095611477,-6.45349292782825));
#119221=CARTESIAN_POINT('Ctrl Pts',(-3.23331887791259,2.1040344875398,-6.48907921306364));
#119222=CARTESIAN_POINT('Ctrl Pts',(-4.259348203,2.232664075,-6.173163928));
#119223=CARTESIAN_POINT('Ctrl Pts',(-4.59428164,2.168401865,-5.942067176));
#119224=CARTESIAN_POINT('Ctrl Pts',(-4.902245606,2.103255924,-5.676089148));
#119225=CARTESIAN_POINT('Ctrl Pts',(-3.919452023,2.232664075,-6.09921272300001));
#119226=CARTESIAN_POINT('Ctrl Pts',(-4.250373136,2.168401865,-5.886557502));
#119227=CARTESIAN_POINT('Ctrl Pts',(-4.5563436,2.103255924,-5.639346859));
#119228=CARTESIAN_POINT('',(-4.55268589075539,2.10403448616461,-5.64230016800444));
#119229=CARTESIAN_POINT('Origin',(0.133291235478736,2.017917758889,0.142378628454944));
#119230=CARTESIAN_POINT('Ctrl Pts',(-4.71139017880313,2.14301213124691,
-5.8354779218392));
#119231=CARTESIAN_POINT('Ctrl Pts',(-4.68583860689175,2.13706112064235,
-5.80442724467249));
#119232=CARTESIAN_POINT('Ctrl Pts',(-4.65931375765888,2.13073653525099,
-5.77217329178188));
#119233=CARTESIAN_POINT('Ctrl Pts',(-4.60550117740287,2.11752978380513,
-5.70667313699972));
#119234=CARTESIAN_POINT('Ctrl Pts',(-4.57906846021973,2.11086978249623,
-5.67447136160385));
#119235=CARTESIAN_POINT('Ctrl Pts',(-4.55268588945731,2.1040344865579,-5.6423001689854));
#119236=CARTESIAN_POINT('Ctrl Pts',(-4.511804397,2.103262031,-5.99112853100001));
#119237=CARTESIAN_POINT('Ctrl Pts',(-4.612514947,2.123129682,-5.915285341));
#119238=CARTESIAN_POINT('Ctrl Pts',(-4.710619476,2.142857143,-5.83610008));
#119239=CARTESIAN_POINT('Ctrl Pts',(-4.93232405,2.187438859,-5.657150805));
#119240=CARTESIAN_POINT('Ctrl Pts',(-5.139813221,2.232664075,-5.461897111));
#119241=CARTESIAN_POINT('Ctrl Pts',(-4.548997036,2.103262031,-5.64527465800001));
#119242=CARTESIAN_POINT('Ctrl Pts',(-4.6438938,2.123129682,-5.568806262));
#119243=CARTESIAN_POINT('Ctrl Pts',(-4.736166816,2.142857143,-5.489191552));
#119244=CARTESIAN_POINT('Ctrl Pts',(-4.944692861,2.187438859,-5.309271772));
#119245=CARTESIAN_POINT('Ctrl Pts',(-5.138967857,2.232664075,-5.114050192));
#119246=CARTESIAN_POINT('Ctrl Pts',(-5.13896785074891,2.23266407354481,
-5.11405019828154));
#119247=CARTESIAN_POINT('Ctrl Pts',(-5.03404520691936,2.20823916389876,
-5.21948406613815));
#119248=CARTESIAN_POINT('Ctrl Pts',(-4.92611588207458,2.18398287519858,
-5.32144385596657));
#119249=CARTESIAN_POINT('Ctrl Pts',(-4.81553385235499,2.15996092059238,
-5.41969867423203));
#119250=CARTESIAN_POINT('Ctrl Pts',(-4.7892265476722,2.15424613238941,-5.4430733531669));
#119251=CARTESIAN_POINT('Ctrl Pts',(-4.76276921770239,2.14854458946511,
-5.46623855226876));
#119252=CARTESIAN_POINT('Ctrl Pts',(-4.73616681522128,2.14285714283382,
-5.48919155269031));
#119253=CARTESIAN_POINT('Ctrl Pts',(-4.67595955624502,2.12998516351878,
-5.54113938823304));
#119254=CARTESIAN_POINT('Ctrl Pts',(-4.61478570966966,2.11704095624726,
-5.59219277144713));
#119255=CARTESIAN_POINT('Ctrl Pts',(-4.55268589439775,2.10403448758647,
-5.6423001647471));
#119256=CARTESIAN_POINT('Ctrl Pts',(-5.486814776,2.232664075,-5.11320482800001));
#119257=CARTESIAN_POINT('Ctrl Pts',(-5.764238685,2.168401865,-4.815510201));
#119258=CARTESIAN_POINT('Ctrl Pts',(-6.007825211,2.103255924,-4.489547442));
#119259=CARTESIAN_POINT('Ctrl Pts',(-5.138967857,2.232664075,-5.114050192));
#119260=CARTESIAN_POINT('Ctrl Pts',(-5.416437632,2.168401865,-4.835228475));
#119261=CARTESIAN_POINT('Ctrl Pts',(-5.662111695,2.103255924,-4.528022874));
#119262=CARTESIAN_POINT('',(-5.65917437505436,2.10403448616662,-4.53169343530542));
#119263=CARTESIAN_POINT('Origin',(0.160781923469345,2.01791774637,0.110395999616852));
#119264=CARTESIAN_POINT('Ctrl Pts',(-5.85569575257519,2.14301213124708,
-4.68623807016988));
#119265=CARTESIAN_POINT('Ctrl Pts',(-5.82406658291385,2.13706112033571,
-4.66140617195806));
#119266=CARTESIAN_POINT('Ctrl Pts',(-5.79122822973611,2.1307365362573,-4.63560836239601));
#119267=CARTESIAN_POINT('Ctrl Pts',(-5.72459315521941,2.11752978376544,
-4.5832076747887));
#119268=CARTESIAN_POINT('Ctrl Pts',(-5.69185599037294,2.11086978245082,
-4.5574410118544));
#119269=CARTESIAN_POINT('Ctrl Pts',(-5.65917437376922,2.10403448653929,
-4.53169343683771));
#119270=CARTESIAN_POINT('Ctrl Pts',(-5.694236456,2.103262031,-4.881154698));
#119271=CARTESIAN_POINT('Ctrl Pts',(-5.776288404,2.123129682,-4.785434889));
#119272=CARTESIAN_POINT('Ctrl Pts',(-5.855076814,2.142857143,-4.687011361));
#119273=CARTESIAN_POINT('Ctrl Pts',(-6.033129253,2.187438859,-4.464585891));
#119274=CARTESIAN_POINT('Ctrl Pts',(-6.19379367,2.232664075,-4.229293082));
#119275=CARTESIAN_POINT('Ctrl Pts',(-5.656211191,2.103262031,-4.535391379));
#119276=CARTESIAN_POINT('Ctrl Pts',(-5.732450877,2.123129682,-4.440310772));
#119277=CARTESIAN_POINT('Ctrl Pts',(-5.805451792,2.142857143,-4.342721438));
#119278=CARTESIAN_POINT('Ctrl Pts',(-5.97042518,2.187438859,-4.122181147));
#119279=CARTESIAN_POINT('Ctrl Pts',(-6.118191265,2.232664075,-3.889760358));
#119280=CARTESIAN_POINT('Ctrl Pts',(-6.11819126023038,2.23266407354021,
-3.88976036550212));
#119281=CARTESIAN_POINT('Ctrl Pts',(-6.038386802732,2.20823916020164,-4.01528453383383));
#119282=CARTESIAN_POINT('Ctrl Pts',(-5.95489913341043,2.18398286787429,
-4.13806219287367));
#119283=CARTESIAN_POINT('Ctrl Pts',(-5.86802431742651,2.15996090971641,
-4.25779175283678));
#119284=CARTESIAN_POINT('Ctrl Pts',(-5.84735694074199,2.15424612514592,
-4.28627521939729));
#119285=CARTESIAN_POINT('Ctrl Pts',(-5.82649801453941,2.14854458583761,
-4.31458635487229));
#119286=CARTESIAN_POINT('Ctrl Pts',(-5.80545179132039,2.14285714280396,
-4.34272143928787));
#119287=CARTESIAN_POINT('Ctrl Pts',(-5.75781939364538,2.12998516349468,
-4.40639754486088));
#119288=CARTESIAN_POINT('Ctrl Pts',(-5.70905072577705,2.11704095625527,
-4.469407896851));
#119289=CARTESIAN_POINT('Ctrl Pts',(-5.65917437799496,2.10403448764214,
-4.53169343152591));
#119290=CARTESIAN_POINT('Ctrl Pts',(-6.45772398800001,2.232664075,-3.814157953));
#119291=CARTESIAN_POINT('Ctrl Pts',(-6.664666336,2.168401865,-3.463785321));
#119292=CARTESIAN_POINT('Ctrl Pts',(-6.832485586,2.103255924,-3.093079487));
#119293=CARTESIAN_POINT('Ctrl Pts',(-6.118191265,2.232664075,-3.889760358));
#119294=CARTESIAN_POINT('Ctrl Pts',(-6.329235524,2.168401865,-3.557809538));
#119295=CARTESIAN_POINT('Ctrl Pts',(-6.503125741,2.103255924,-3.204973572));
#119296=CARTESIAN_POINT('',(-6.50104615573101,2.10403448617462,-3.20918975457166));
#119297=CARTESIAN_POINT('Origin',(0.180754841449393,2.01791773564785,0.0732516632395214));
#119298=CARTESIAN_POINT('Ctrl Pts',(-6.72619550123132,2.14301213123526,
-3.31787493432136));
#119299=CARTESIAN_POINT('Ctrl Pts',(-6.68996775205999,2.13706113217375,
-3.30042296334979));
#119300=CARTESIAN_POINT('Ctrl Pts',(-6.65235119062877,2.1307365168745,-3.28228747872196));
#119301=CARTESIAN_POINT('Ctrl Pts',(-6.57600906312516,2.11752970468666,
-3.24543629492975));
#119302=CARTESIAN_POINT('Ctrl Pts',(-6.53849844888826,2.11086974369859,
-3.22730968301239));
#119303=CARTESIAN_POINT('Ctrl Pts',(-6.50104615485299,2.10403448649296,
-3.20918975626637));
#119304=CARTESIAN_POINT('Ctrl Pts',(-6.61041234600001,2.103262031,-3.542943496));
#119305=CARTESIAN_POINT('Ctrl Pts',(-6.669969036,2.123129682,-3.431822819));
#119306=CARTESIAN_POINT('Ctrl Pts',(-6.725757268,2.142857143,-3.3187632));
#119307=CARTESIAN_POINT('Ctrl Pts',(-6.851832038,2.187438859,-3.063261902));
#119308=CARTESIAN_POINT('Ctrl Pts',(-6.95815921200001,2.232664075,-2.798932008));
#119309=CARTESIAN_POINT('Ctrl Pts',(-6.49894719800001,2.103262031,-3.213438239));
#119310=CARTESIAN_POINT('Ctrl Pts',(-6.552964923,2.123129682,-3.104191285));
#119311=CARTESIAN_POINT('Ctrl Pts',(-6.603280295,2.142857143,-2.993190497));
#119312=CARTESIAN_POINT('Ctrl Pts',(-6.716987053,2.187438859,-2.742341913));
#119313=CARTESIAN_POINT('Ctrl Pts',(-6.81133485,2.232664075,-2.483589653));
#119314=CARTESIAN_POINT('Ctrl Pts',(-6.81133484702938,2.23266407357604,
-2.48358966114703));
#119315=CARTESIAN_POINT('Ctrl Pts',(-6.76038013566595,2.20823914906342,
-2.62333480722537));
#119316=CARTESIAN_POINT('Ctrl Pts',(-6.7052379020462,2.1839828457863,-2.7611894355538));
#119317=CARTESIAN_POINT('Ctrl Pts',(-6.64613245686244,2.15996087693181,
-2.89679536201218));
#119318=CARTESIAN_POINT('Ctrl Pts',(-6.63207140127089,2.15424610330256,
-2.92905571407529));
#119319=CARTESIAN_POINT('Ctrl Pts',(-6.61778622926372,2.14854457488727,
-2.96118894202542));
#119320=CARTESIAN_POINT('Ctrl Pts',(-6.60328029421641,2.14285714269277,
-2.99319049872867));
#119321=CARTESIAN_POINT('Ctrl Pts',(-6.57044999596232,2.12998516336823,
-3.06561744956076));
#119322=CARTESIAN_POINT('Ctrl Pts',(-6.5363668754193,2.11704095610237,-3.13763847664814));
#119323=CARTESIAN_POINT('Ctrl Pts',(-6.50104615793019,2.10403448763485,
-3.20918974991449));
#119324=CARTESIAN_POINT('Ctrl Pts',(-7.126677204,2.232664075,-2.336765291));
#119325=CARTESIAN_POINT('Ctrl Pts',(-7.253461596,2.168401865,-1.950097689));
#119326=CARTESIAN_POINT('Ctrl Pts',(-7.337666529,2.103255924,-1.551982574));
#119327=CARTESIAN_POINT('Ctrl Pts',(-6.81133485,2.232664075,-2.483589653));
#119328=CARTESIAN_POINT('Ctrl Pts',(-6.946085397,2.168401865,-2.114031381));
#119329=CARTESIAN_POINT('Ctrl Pts',(-7.040060855,2.103255924,-1.732063268));
#119330=CARTESIAN_POINT('',(-7.03893624373328,2.10403448613602,-1.73662792757353));
#119331=CARTESIAN_POINT('Origin',(0.19227601318856,2.01791769717493,0.032682179817278));
#119332=CARTESIAN_POINT('Ctrl Pts',(-7.28218582306869,2.14301213122963,
-1.7943716548747));
#119333=CARTESIAN_POINT('Ctrl Pts',(-7.24305332634239,2.13706112086173,
-1.7851155788767));
#119334=CARTESIAN_POINT('Ctrl Pts',(-7.20241782122318,2.13073653615391,
-1.77549058655946));
#119335=CARTESIAN_POINT('Ctrl Pts',(-7.11993850864511,2.11752970689892,
-1.7559122383386));
#119336=CARTESIAN_POINT('Ctrl Pts',(-7.07940817845469,2.11086974474719,
-1.74627308796845));
#119337=CARTESIAN_POINT('Ctrl Pts',(-7.03893624340029,2.10403448644561,
-1.7366279295276));
#119338=CARTESIAN_POINT('Ctrl Pts',(-7.217492702,2.103262031,-2.039068194));
#119339=CARTESIAN_POINT('Ctrl Pts',(-7.251769329,2.123129682,-1.917742529));
#119340=CARTESIAN_POINT('Ctrl Pts',(-7.281948786,2.142857143,-1.79533336));
#119341=CARTESIAN_POINT('Ctrl Pts',(-7.350150772,2.187438859,-1.518703192));
#119342=CARTESIAN_POINT('Ctrl Pts',(-7.397168962,2.232664075,-1.237695984));
#119343=CARTESIAN_POINT('Ctrl Pts',(-7.03779965700001,2.103262031,-1.741228298));
#119344=CARTESIAN_POINT('Ctrl Pts',(-7.067069611,2.123129682,-1.622923263));
#119345=CARTESIAN_POINT('Ctrl Pts',(-7.09234675,2.142857143,-1.503701295));
#119346=CARTESIAN_POINT('Ctrl Pts',(-7.149470077,2.187438859,-1.234273819));
#119347=CARTESIAN_POINT('Ctrl Pts',(-7.18598798700001,2.232664075,-0.961289056));
#119348=CARTESIAN_POINT('Ctrl Pts',(-7.18598798581391,2.23266407353109,
-0.961289064866521));
#119349=CARTESIAN_POINT('Ctrl Pts',(-7.16626565124671,2.20823915894989,
-1.1087207436533));
#119350=CARTESIAN_POINT('Ctrl Pts',(-7.14204729433149,2.18398286543511,
-1.25520629864654));
#119351=CARTESIAN_POINT('Ctrl Pts',(-7.1134749823763,2.15996090615119,-1.40034769983849));
#119352=CARTESIAN_POINT('Ctrl Pts',(-7.10667767780776,2.15424612276782,
-1.43487659308848));
#119353=CARTESIAN_POINT('Ctrl Pts',(-7.09963416776281,2.14854458464336,
-1.46932951247662));
#119354=CARTESIAN_POINT('Ctrl Pts',(-7.09234674973051,2.14285714278968,
-1.50370129627107));
#119355=CARTESIAN_POINT('Ctrl Pts',(-7.07585365867762,2.12998516347851,
-1.58149248822485));
#119356=CARTESIAN_POINT('Ctrl Pts',(-7.05804977456917,2.11704095615068,
-1.65915656746971));
#119357=CARTESIAN_POINT('Ctrl Pts',(-7.03893624466465,2.10403448753363,
-1.73662792249327));
#119358=CARTESIAN_POINT('Ctrl Pts',(-7.462394915,2.232664075,-0.750108081));
#119359=CARTESIAN_POINT('Ctrl Pts',(-7.503093053,2.168401865,-0.345225657));
#119360=CARTESIAN_POINT('Ctrl Pts',(-7.49974634,2.103255924,0.0616833200000001));
#119361=CARTESIAN_POINT('Ctrl Pts',(-7.185987987,2.232664075,-0.961289056000001));
#119362=CARTESIAN_POINT('Ctrl Pts',(-7.238144037,2.168401865,-0.571403467));
#119363=CARTESIAN_POINT('Ctrl Pts',(-7.247810547,2.103255924,-0.17816361));
#119364=CARTESIAN_POINT('',(-7.24769349611018,2.10403448614893,-0.182863309005228));
#119365=CARTESIAN_POINT('Origin',(0.194806409965016,2.01791775247604,-0.00941555982621519));
#119366=CARTESIAN_POINT('Ctrl Pts',(-7.49766922992161,2.14301213117218,
-0.186965550243363));
#119367=CARTESIAN_POINT('Ctrl Pts',(-7.45746192152156,2.1370611319295,-0.186338207433853));
#119368=CARTESIAN_POINT('Ctrl Pts',(-7.41570717295776,2.13073651822537,
-0.185673671629014));
#119369=CARTESIAN_POINT('Ctrl Pts',(-7.33094802269037,2.11752978372598,
-0.18428367832303));
#119370=CARTESIAN_POINT('Ctrl Pts',(-7.28929287292505,2.11086978243035,
-0.183582704619183));
#119371=CARTESIAN_POINT('Ctrl Pts',(-7.24769349602953,2.10403448649871,
-0.182863310345257));
#119372=CARTESIAN_POINT('Ctrl Pts',(-7.487091121,2.103262031,-0.43984833));
#119373=CARTESIAN_POINT('Ctrl Pts',(-7.494484947,2.123129682,-0.313990729));
#119374=CARTESIAN_POINT('Ctrl Pts',(-7.497644473,2.142857143,-0.187955727));
#119375=CARTESIAN_POINT('Ctrl Pts',(-7.504784626,2.187438859,0.0968683920000001));
#119376=CARTESIAN_POINT('Ctrl Pts',(-7.490295313,2.232664075,0.381413328));
#119377=CARTESIAN_POINT('Ctrl Pts',(-7.247572426,2.103262031,-0.187600458));
#119378=CARTESIAN_POINT('Ctrl Pts',(-7.25072598,2.123129682,-0.065769154));
#119379=CARTESIAN_POINT('Ctrl Pts',(-7.249782953,2.142857143,0.056099309));
#119380=CARTESIAN_POINT('Ctrl Pts',(-7.247651826,2.187438859,0.331507546));
#119381=CARTESIAN_POINT('Ctrl Pts',(-7.224632313,2.232664075,0.605960349000001));
#119382=CARTESIAN_POINT('Ctrl Pts',(-7.22463231372479,2.23266407357604,
0.605960340358616));
#119383=CARTESIAN_POINT('Ctrl Pts',(-7.23706452836554,2.20823916065962,
0.457735822982831));
#119384=CARTESIAN_POINT('Ctrl Pts',(-7.2449024470062,2.18398286877176,0.309468797995694));
#119385=CARTESIAN_POINT('Ctrl Pts',(-7.24819925090731,2.15996091108634,
0.161578529878988));
#119386=CARTESIAN_POINT('Ctrl Pts',(-7.24898355524294,2.15424612606176,
0.126395673403131));
#119387=CARTESIAN_POINT('Ctrl Pts',(-7.24951107796628,2.14854458630384,
0.0912340876929665));
#119388=CARTESIAN_POINT('Ctrl Pts',(-7.24978295323504,2.14285714282549,
0.056099307698734));
#119389=CARTESIAN_POINT('Ctrl Pts',(-7.25039826940105,2.12998516354546,
-0.0234186967996028));
#119390=CARTESIAN_POINT('Ctrl Pts',(-7.2497061112786,2.11704095613262,-0.103094342054953));
#119391=CARTESIAN_POINT('Ctrl Pts',(-7.2476934961534,2.10403448751907,-0.182863304051553));
#119392=CARTESIAN_POINT('Ctrl Pts',(-7.449179333,2.232664075,0.871623349000001));
#119393=CARTESIAN_POINT('Ctrl Pts',(-7.401888218,2.168401865,1.275788744));
#119394=CARTESIAN_POINT('Ctrl Pts',(-7.311146348,2.103255924,1.672464971));
#119395=CARTESIAN_POINT('Ctrl Pts',(-7.224632313,2.232664075,0.605960349000001));
#119396=CARTESIAN_POINT('Ctrl Pts',(-7.191755107,2.168401865,0.997942639));
#119397=CARTESIAN_POINT('Ctrl Pts',(-7.116660674,2.103255924,1.38406678));
#119398=CARTESIAN_POINT('',(-7.11755665582389,2.10403448616646,1.37945179518342));
#119399=CARTESIAN_POINT('Origin',(0.188227755794577,2.01791772706583,-0.0510730378310159));
#119400=CARTESIAN_POINT('Ctrl Pts',(-7.36256995640569,2.14301213123507,
1.42918285531713));
#119401=CARTESIAN_POINT('Ctrl Pts',(-7.32316781099792,2.13706113177995,
1.42115214801647));
#119402=CARTESIAN_POINT('Ctrl Pts',(-7.28224641026556,2.13073651812043,
1.41282511087366));
#119403=CARTESIAN_POINT('Ctrl Pts',(-7.19917007545252,2.11752978377754,
1.39596189507937));
#119404=CARTESIAN_POINT('Ctrl Pts',(-7.15833811113647,2.11086978244974,
1.38769185434603));
#119405=CARTESIAN_POINT('Ctrl Pts',(-7.11755665617418,2.1040344865323,1.37945179314629));
#119406=CARTESIAN_POINT('Ctrl Pts',(-7.40660148,2.103262031,1.179938354));
#119407=CARTESIAN_POINT('Ctrl Pts',(-7.386766779,2.123129682,1.304442928));
#119408=CARTESIAN_POINT('Ctrl Pts',(-7.362758637,2.142857143,1.428210506));
#119409=CARTESIAN_POINT('Ctrl Pts',(-7.308503091,2.187438859,1.707910518));
#119410=CARTESIAN_POINT('Ctrl Pts',(-7.23318378,2.232664075,1.982688177));
#119411=CARTESIAN_POINT('Ctrl Pts',(-7.118456763,2.103262031,1.374799371));
#119412=CARTESIAN_POINT('Ctrl Pts',(-7.095346459,2.123129682,1.494460248));
#119413=CARTESIAN_POINT('Ctrl Pts',(-7.068227363,2.142857143,1.613276771));
#119414=CARTESIAN_POINT('Ctrl Pts',(-7.00694143000001,2.187438859,1.881787987));
#119415=CARTESIAN_POINT('Ctrl Pts',(-6.925460861,2.232664075,2.144875721));
#119416=CARTESIAN_POINT('Ctrl Pts',(-6.92546086356549,2.23266407357604,
2.14487571271646));
#119417=CARTESIAN_POINT('Ctrl Pts',(-6.96946627562099,2.20823917943093,
2.00278927011421));
#119418=CARTESIAN_POINT('Ctrl Pts',(-7.00899394941072,2.18398290596486,
1.85967367665201));
#119419=CARTESIAN_POINT('Ctrl Pts',(-7.04400569229374,2.15996096621933,
1.71594982672751));
#119420=CARTESIAN_POINT('Ctrl Pts',(-7.05233496260397,2.1542461627551,1.68175801856626));
#119421=CARTESIAN_POINT('Ctrl Pts',(-7.06040888047637,2.14854460463559,
1.64753178316994));
#119422=CARTESIAN_POINT('Ctrl Pts',(-7.06822736368688,2.14285714288217,
1.61327676996052));
#119423=CARTESIAN_POINT('Ctrl Pts',(-7.08592231393104,2.12998516356634,
1.53575012699934));
#119424=CARTESIAN_POINT('Ctrl Pts',(-7.10237424704962,2.1170409562774,1.45778846079541));
#119425=CARTESIAN_POINT('Ctrl Pts',(-7.11755665457197,2.10403448768129,
1.37945180024277));
#119426=CARTESIAN_POINT('Ctrl Pts',(-7.087648405,2.232664075,2.45259864));
#119427=CARTESIAN_POINT('Ctrl Pts',(-6.954579317,2.168401865,2.837148681));
#119428=CARTESIAN_POINT('Ctrl Pts',(-6.780685278,2.103255924,3.205044018));
#119429=CARTESIAN_POINT('Ctrl Pts',(-6.925460861,2.232664075,2.144875721));
#119430=CARTESIAN_POINT('Ctrl Pts',(-6.809087701,2.168401865,2.520626056));
#119431=CARTESIAN_POINT('Ctrl Pts',(-6.652743657,2.103255924,2.881579746));
#119432=CARTESIAN_POINT('',(-6.65461077679171,2.10403448616333,2.8772652662477));
#119433=CARTESIAN_POINT('Origin',(0.172847689192316,2.01791773293874,-0.0903423007010168));
#119434=CARTESIAN_POINT('Ctrl Pts',(-6.8832050949221,2.1430121312801,2.97850425893303));
#119435=CARTESIAN_POINT('Ctrl Pts',(-6.84645051598016,2.13706113205809,
2.96219100944993));
#119436=CARTESIAN_POINT('Ctrl Pts',(-6.80827589352981,2.13073651702508,
2.94526175870189));
#119437=CARTESIAN_POINT('Ctrl Pts',(-6.73076693640448,2.11752978374688,
2.91093384222074));
#119438=CARTESIAN_POINT('Ctrl Pts',(-6.69266741499653,2.11086978242154,
2.89407948519025));
#119439=CARTESIAN_POINT('Ctrl Pts',(-6.65461077734004,2.1040344865073,2.8772652648668));
#119440=CARTESIAN_POINT('Ctrl Pts',(-6.979787386,2.103262031,2.744552431));
#119441=CARTESIAN_POINT('Ctrl Pts',(-6.933651607,2.123129682,2.861882283));
#119442=CARTESIAN_POINT('Ctrl Pts',(-6.883598391,2.142857143,2.977595203));
#119443=CARTESIAN_POINT('Ctrl Pts',(-6.770484074,2.187438859,3.239092645));
#119444=CARTESIAN_POINT('Ctrl Pts',(-6.63785661200001,2.232664075,3.491254731));
#119445=CARTESIAN_POINT('Ctrl Pts',(-6.656489974,2.103262031,2.87291511));
#119446=CARTESIAN_POINT('Ctrl Pts',(-6.608196425,2.123129682,2.98481035));
#119447=CARTESIAN_POINT('Ctrl Pts',(-6.556169318,2.142857143,3.095019205));
#119448=CARTESIAN_POINT('Ctrl Pts',(-6.438594242,2.187438859,3.344078114));
#119449=CARTESIAN_POINT('Ctrl Pts',(-6.302462557,2.232664075,3.583499089));
#119450=CARTESIAN_POINT('Ctrl Pts',(-6.30246256128625,2.23266407357604,
3.58349908146159));
#119451=CARTESIAN_POINT('Ctrl Pts',(-6.37598361868775,2.20823915216313,
3.45419425947911));
#119452=CARTESIAN_POINT('Ctrl Pts',(-6.44535285159381,2.18398285191355,
3.32292176254641));
#119453=CARTESIAN_POINT('Ctrl Pts',(-6.51044248130645,2.15996088600698,
3.19008443517309));
#119454=CARTESIAN_POINT('Ctrl Pts',(-6.5259271713798,2.15424610934197,3.15848270608615));
#119455=CARTESIAN_POINT('Ctrl Pts',(-6.54116988211619,2.14854457790376,
3.12679246227866));
#119456=CARTESIAN_POINT('Ctrl Pts',(-6.55616931878926,2.14285714270073,
3.09501920332812));
#119457=CARTESIAN_POINT('Ctrl Pts',(-6.59011650761173,2.12998516340818,
3.02310898135356));
#119458=CARTESIAN_POINT('Ctrl Pts',(-6.62294325708969,2.11704095609677,
2.95050669476758));
#119459=CARTESIAN_POINT('Ctrl Pts',(-6.65461077492281,2.10403448753761,
2.87726527063246));
#119460=CARTESIAN_POINT('Ctrl Pts',(-6.39470691500001,2.232664075,3.918893144));
#119461=CARTESIAN_POINT('Ctrl Pts',(-6.182082017,2.168401865,4.265846698));
#119462=CARTESIAN_POINT('Ctrl Pts',(-5.933166901,2.103255924,4.58775876899999));
#119463=CARTESIAN_POINT('Ctrl Pts',(-6.302462557,2.232664075,3.583499089));
#119464=CARTESIAN_POINT('Ctrl Pts',(-6.108034921,2.168401865,3.9254478));
#119465=CARTESIAN_POINT('Ctrl Pts',(-5.877751741,2.103255924,4.244353245));
#119466=CARTESIAN_POINT('',(-5.88050269387236,2.10403448615122,4.24054101112135));
#119467=CARTESIAN_POINT('Origin',(0.149385849193904,2.01791769792684,-0.125387414436151));
#119468=CARTESIAN_POINT('Ctrl Pts',(-6.08198921328939,2.14301213123481,
4.38855411340676));
#119469=CARTESIAN_POINT('Ctrl Pts',(-6.04960074080206,2.13706112071591,
4.36472106532138));
#119470=CARTESIAN_POINT('Ctrl Pts',(-6.01595806662983,2.13073653570991,
4.33998131233119));
#119471=CARTESIAN_POINT('Ctrl Pts',(-5.94764061628231,2.1175297837157,4.28979375773196));
#119472=CARTESIAN_POINT('Ctrl Pts',(-5.91405502901557,2.11086978238005,
4.26514317521297));
#119473=CARTESIAN_POINT('Ctrl Pts',(-5.88050269485777,2.10403448647498,
4.2405410096875));
#119474=CARTESIAN_POINT('Ctrl Pts',(-6.226606191,2.103262031,4.180834288));
#119475=CARTESIAN_POINT('Ctrl Pts',(-6.156326591,2.123129682,4.285503204));
#119476=CARTESIAN_POINT('Ctrl Pts',(-6.082568734,2.142857143,4.387750858));
#119477=CARTESIAN_POINT('Ctrl Pts',(-5.915884747,2.187438859,4.618818401));
#119478=CARTESIAN_POINT('Ctrl Pts',(-5.732150647,2.232664075,4.836574093));
#119479=CARTESIAN_POINT('Ctrl Pts',(-5.883273111,2.103262031,4.236696531));
#119480=CARTESIAN_POINT('Ctrl Pts',(-5.81205447,2.123129682,4.335594037));
#119481=CARTESIAN_POINT('Ctrl Pts',(-5.737552082,2.142857143,4.43204198));
#119482=CARTESIAN_POINT('Ctrl Pts',(-5.569185542,2.187438859,4.650002864));
#119483=CARTESIAN_POINT('Ctrl Pts',(-5.384768108,2.232664075,4.854562022));
#119484=CARTESIAN_POINT('Ctrl Pts',(-5.38476811398704,2.23266407353178,
4.85456201535907));
#119485=CARTESIAN_POINT('Ctrl Pts',(-5.48436695112432,2.20823916515672,
4.74408518097743));
#119486=CARTESIAN_POINT('Ctrl Pts',(-5.58033402759021,2.18398287769443,
4.6307941581107));
#119487=CARTESIAN_POINT('Ctrl Pts',(-5.67245795214641,2.15996092427026,
4.51505490397573));
#119488=CARTESIAN_POINT('Ctrl Pts',(-5.69437410617214,2.15424613483007,
4.4875206957593));
#119489=CARTESIAN_POINT('Ctrl Pts',(-5.71607296529475,2.14854459067243,
4.45984802322099));
#119490=CARTESIAN_POINT('Ctrl Pts',(-5.73755208278728,2.14285714281209,
4.43204197907132));
#119491=CARTESIAN_POINT('Ctrl Pts',(-5.78616417716126,2.12998516349167,
4.36911062020453));
#119492=CARTESIAN_POINT('Ctrl Pts',(-5.83383080093272,2.11704095618126,
4.30526251552709));
#119493=CARTESIAN_POINT('Ctrl Pts',(-5.88050269069905,2.10403448751903,
4.24054101494961));
#119494=CARTESIAN_POINT('Ctrl Pts',(-5.402756036,2.232664075,5.201944561));
#119495=CARTESIAN_POINT('Ctrl Pts',(-5.120517432,2.168401865,5.49507846600001));
#119496=CARTESIAN_POINT('Ctrl Pts',(-4.808220234,2.103255924,5.755955019));
#119497=CARTESIAN_POINT('Ctrl Pts',(-5.38476810800001,2.232664075,4.854562022));
#119498=CARTESIAN_POINT('Ctrl Pts',(-5.121377218,2.168401865,5.14671996700001));
#119499=CARTESIAN_POINT('Ctrl Pts',(-4.827922686,2.103255924,5.408665504));
#119500=CARTESIAN_POINT('',(-4.83142884100588,2.10403448617778,5.40553377166433));
#119501=CARTESIAN_POINT('Origin',(0.118938734844523,2.01791776995071,-0.154569479146689));
#119502=CARTESIAN_POINT('Ctrl Pts',(-4.99638627563914,2.14301213125791,
5.5934000559955));
#119503=CARTESIAN_POINT('Ctrl Pts',(-4.96987847844244,2.13706113193449,
5.56316170396712));
#119504=CARTESIAN_POINT('Ctrl Pts',(-4.94234053791621,2.13073651703642,
5.53176802477778));
#119505=CARTESIAN_POINT('Ctrl Pts',(-4.88640923164154,2.11752978377236,
5.46806768500414));
#119506=CARTESIAN_POINT('Ctrl Pts',(-4.85890800332318,2.11086978245107,
5.43677351095245));
#119507=CARTESIAN_POINT('Ctrl Pts',(-4.83142884221226,2.10403448652669,
5.40553377052683));
#119508=CARTESIAN_POINT('Ctrl Pts',(-5.182275811,2.103262031,5.421624979));
#119509=CARTESIAN_POINT('Ctrl Pts',(-5.091138586,2.123129682,5.508738758));
#119510=CARTESIAN_POINT('Ctrl Pts',(-4.997124924,2.142857143,5.59274016));
#119511=CARTESIAN_POINT('Ctrl Pts',(-4.784665224,2.187438859,5.782573342));
#119512=CARTESIAN_POINT('Ctrl Pts',(-4.558415688,2.232664075,5.955740627));
#119513=CARTESIAN_POINT('Ctrl Pts',(-4.834960937,2.103262031,5.402374731));
#119514=CARTESIAN_POINT('Ctrl Pts',(-4.744147307,2.123129682,5.483650165));
#119515=CARTESIAN_POINT('Ctrl Pts',(-4.650653287,2.142857143,5.561827398));
#119516=CARTESIAN_POINT('Ctrl Pts',(-4.439367916,2.187438859,5.738498649));
#119517=CARTESIAN_POINT('Ctrl Pts',(-4.215287887,2.232664075,5.89863103));
#119518=CARTESIAN_POINT('Ctrl Pts',(-4.21528789435224,2.23266407351613,
5.89863102474593));
#119519=CARTESIAN_POINT('Ctrl Pts',(-4.3363073888234,2.20823917136867,5.81214790559146));
#119520=CARTESIAN_POINT('Ctrl Pts',(-4.45438500029938,2.18398289002927,
5.72213567242712));
#119521=CARTESIAN_POINT('Ctrl Pts',(-4.56923560956039,2.15996094257694,
5.62890628343251));
#119522=CARTESIAN_POINT('Ctrl Pts',(-4.59655844647514,2.15424614701044,
5.6067271116584));
#119523=CARTESIAN_POINT('Ctrl Pts',(-4.62369883406465,2.14854459675296,
5.58436600038853));
#119524=CARTESIAN_POINT('Ctrl Pts',(-4.65065328800589,2.142857142822,5.56182739730908));
#119525=CARTESIAN_POINT('Ctrl Pts',(-4.71165724029445,2.12998516349101,
5.51081750162112));
#119526=CARTESIAN_POINT('Ctrl Pts',(-4.77193490002844,2.11704095622126,
5.45870904546891));
#119527=CARTESIAN_POINT('Ctrl Pts',(-4.83142883691819,2.10403448756895,
5.40553377475842));
#119528=CARTESIAN_POINT('Ctrl Pts',(-4.15817829,2.232664075,6.24175883100001));
#119529=CARTESIAN_POINT('Ctrl Pts',(-3.819523143,2.168401865,6.467366471));
#119530=CARTESIAN_POINT('Ctrl Pts',(-3.458446532,2.103255924,6.65500921));
#119531=CARTESIAN_POINT('Ctrl Pts',(-4.215287887,2.232664075,5.89863103));
#119532=CARTESIAN_POINT('Ctrl Pts',(-3.895249607,2.168401865,6.127337229));
#119533=CARTESIAN_POINT('Ctrl Pts',(-3.552345332,2.103255924,6.320074576));
#119534=CARTESIAN_POINT('',(-3.55644274485985,2.10403448617125,6.31776978103635));
#119535=CARTESIAN_POINT('Origin',(0.082930208574552,2.01791772973768,-0.176524146984284));
#119536=CARTESIAN_POINT('Ctrl Pts',(-3.67715786822644,2.14301213123246,
6.53670482815667));
#119537=CARTESIAN_POINT('Ctrl Pts',(-3.65777016219678,2.1370611324582,6.50147504250649));
#119538=CARTESIAN_POINT('Ctrl Pts',(-3.63762475105466,2.13073651583364,
6.46489547691489));
#119539=CARTESIAN_POINT('Ctrl Pts',(-3.59669478159521,2.11752978378474,
6.39066084503437));
#119540=CARTESIAN_POINT('Ctrl Pts',(-3.57656383913306,2.1108697824456,6.35418636013881));
#119541=CARTESIAN_POINT('Ctrl Pts',(-3.55644274658363,2.10403448654469,
6.31776978008171));
#119542=CARTESIAN_POINT('Ctrl Pts',(-3.895627974,2.103262031,6.408906513));
#119543=CARTESIAN_POINT('Ctrl Pts',(-3.787894599,2.123129682,6.47439181));
#119544=CARTESIAN_POINT('Ctrl Pts',(-3.678021106,2.142857143,6.536219148));
#119545=CARTESIAN_POINT('Ctrl Pts',(-3.429720073,2.187438859,6.67594158));
#119546=CARTESIAN_POINT('Ctrl Pts',(-3.171534278,2.232664075,6.796423348));
#119547=CARTESIAN_POINT('Ctrl Pts',(-3.560571363,2.103262031,6.315443893));
#119548=CARTESIAN_POINT('Ctrl Pts',(-3.45440909,2.123129682,6.375296907));
#119549=CARTESIAN_POINT('Ctrl Pts',(-3.346295113,2.142857143,6.431547949));
#119550=CARTESIAN_POINT('Ctrl Pts',(-3.101970381,2.187438859,6.558668615));
#119551=CARTESIAN_POINT('Ctrl Pts',(-2.84870549,2.232664075,6.666886607));
#119552=CARTESIAN_POINT('Ctrl Pts',(-2.84870549797434,2.23266407357603,
6.66688660359263));
#119553=CARTESIAN_POINT('Ctrl Pts',(-2.98548704572222,2.20823915222455,
6.60844097999876));
#119554=CARTESIAN_POINT('Ctrl Pts',(-3.12015414092708,2.18398285202096,
6.54591632681462));
#119555=CARTESIAN_POINT('Ctrl Pts',(-3.25236126881296,2.15996088615698,
6.47955601744561));
#119556=CARTESIAN_POINT('Ctrl Pts',(-3.28381307499604,2.1542461094534,6.46376903514065));
#119557=CARTESIAN_POINT('Ctrl Pts',(-3.31512580993533,2.14854457797663,
6.44776514722032));
#119558=CARTESIAN_POINT('Ctrl Pts',(-3.34629511470663,2.14285714273527,
6.43154794832585));
#119559=CARTESIAN_POINT('Ctrl Pts',(-3.41683844901538,2.12998516343135,
6.39484468235121));
#119560=CARTESIAN_POINT('Ctrl Pts',(-3.48690862792303,2.11704095624996,
6.35691240809715));
#119561=CARTESIAN_POINT('Ctrl Pts',(-3.55644274019248,2.10403448765571,
6.317769783299));
#119562=CARTESIAN_POINT('Ctrl Pts',(-2.719168749,2.232664075,6.989715396));
#119563=CARTESIAN_POINT('Ctrl Pts',(-2.339932197,2.168401865,7.137247609));
#119564=CARTESIAN_POINT('Ctrl Pts',(-1.946959715,2.103255924,7.242882566));
#119565=CARTESIAN_POINT('Ctrl Pts',(-2.84870549,2.232664075,6.666886607));
#119566=CARTESIAN_POINT('Ctrl Pts',(-2.486984455,2.168401865,6.821447013));
#119567=CARTESIAN_POINT('Ctrl Pts',(-2.110664259,2.103255924,6.935963984));
#119568=CARTESIAN_POINT('',(-2.11516133921097,2.10403448613605,6.93459389680005));
#119569=CARTESIAN_POINT('Origin',(0.0430438123248453,2.01791774548237,-0.190224481398423));
#119570=CARTESIAN_POINT('Ctrl Pts',(-2.18598964688697,2.14301213127581,
7.17436054715705));
#119571=CARTESIAN_POINT('Ctrl Pts',(-2.17462855492618,2.13706112079029,
7.13578655461992));
#119572=CARTESIAN_POINT('Ctrl Pts',(-2.16281771494847,2.13073653523302,
7.09573172665891));
#119573=CARTESIAN_POINT('Ctrl Pts',(-2.13880288145904,2.11752978374283,
7.01443380632184));
#119574=CARTESIAN_POINT('Ctrl Pts',(-2.12698352521162,2.11086978238224,
6.97448451705866));
#119575=CARTESIAN_POINT('Ctrl Pts',(-2.11516134064851,2.10403448644958,
6.93459389632029));
#119576=CARTESIAN_POINT('Ctrl Pts',(-2.426824903,2.103262031,7.0965147));
#119577=CARTESIAN_POINT('Ctrl Pts',(-2.307532871,2.123129682,7.137309497));
#119578=CARTESIAN_POINT('Ctrl Pts',(-2.186937109,2.142857143,7.174071792));
#119579=CARTESIAN_POINT('Ctrl Pts',(-1.914405023,2.187438859,7.25715021));
#119580=CARTESIAN_POINT('Ctrl Pts',(-1.63635545,2.232664075,7.319312867));
#119581=CARTESIAN_POINT('Ctrl Pts',(-2.119693429,2.103262031,6.933209918));
#119582=CARTESIAN_POINT('Ctrl Pts',(-2.003146542,2.123129682,6.968841851));
#119583=CARTESIAN_POINT('Ctrl Pts',(-1.885467899,2.142857143,7.000536465));
#119584=CARTESIAN_POINT('Ctrl Pts',(-1.619528158,2.187438859,7.072162525));
#119585=CARTESIAN_POINT('Ctrl Pts',(-1.34892079,2.232664075,7.12340597600001));
#119586=CARTESIAN_POINT('Ctrl Pts',(-1.34892079852034,2.23266407357604,
7.12340597438655));
#119587=CARTESIAN_POINT('Ctrl Pts',(-1.49506844498092,2.20823916996667,
7.09573078629201));
#119588=CARTESIAN_POINT('Ctrl Pts',(-1.64002794687247,2.18398288716985,
7.06361739593309));
#119589=CARTESIAN_POINT('Ctrl Pts',(-1.78340954923378,2.15996093828879,
7.0272292105977));
#119590=CARTESIAN_POINT('Ctrl Pts',(-1.81751986821592,2.15424614416311,
7.01857250298299));
#119591=CARTESIAN_POINT('Ctrl Pts',(-1.85154099512468,2.1485445953398,7.00967406320081));
#119592=CARTESIAN_POINT('Ctrl Pts',(-1.88546790014525,2.1428571428359,7.00053646483213));
#119593=CARTESIAN_POINT('Ctrl Pts',(-1.96225208760458,2.12998516346518,
6.97985603268479));
#119594=CARTESIAN_POINT('Ctrl Pts',(-2.03883838298836,2.11704095611587,
6.95787361101836));
#119595=CARTESIAN_POINT('Ctrl Pts',(-2.11516133429163,2.10403448747751,
6.93459389798712));
#119596=CARTESIAN_POINT('Ctrl Pts',(-1.153013899,2.232664075,7.410840637));
#119597=CARTESIAN_POINT('Ctrl Pts',(-0.750928622,2.168401865,7.47339898));
#119598=CARTESIAN_POINT('Ctrl Pts',(-0.344435225,2.103255924,7.492086784));
#119599=CARTESIAN_POINT('Ctrl Pts',(-1.34892079,2.232664075,7.123405976));
#119600=CARTESIAN_POINT('Ctrl Pts',(-0.962430673,2.168401865,7.19659351500001));
#119601=CARTESIAN_POINT('Ctrl Pts',(-0.57029087,2.103255924,7.227535425));
#119602=CARTESIAN_POINT('',(-0.574977339844184,2.10403448631433,7.22716410899259));
#119603=CARTESIAN_POINT('Origin',(0.00114484907014038,2.01791774551872,
-0.195030425692181));
#119604=CARTESIAN_POINT('Ctrl Pts',(-0.592606977972668,2.14301213123161,
7.47655114138138));
#119605=CARTESIAN_POINT('Ctrl Pts',(-0.58980377572683,2.13706113256072,
7.43643676802673));
#119606=CARTESIAN_POINT('Ctrl Pts',(-0.58687965707151,2.13073651668701,
7.3947792195583));
#119607=CARTESIAN_POINT('Ctrl Pts',(-0.580902935316097,2.11752978377134,
7.31021963858121));
#119608=CARTESIAN_POINT('Ctrl Pts',(-0.577947825397008,2.11086978246525,
7.26866352942372));
#119609=CARTESIAN_POINT('Ctrl Pts',(-0.574977341364854,2.10403448656429,
7.22716410884257));
#119610=CARTESIAN_POINT('Ctrl Pts',(-0.844546196,2.103262031,7.452297748));
#119611=CARTESIAN_POINT('Ctrl Pts',(-0.71927347,2.123129682,7.46649452400001));
#119612=CARTESIAN_POINT('Ctrl Pts',(-0.593594363,2.142857143,7.476472814));
#119613=CARTESIAN_POINT('Ctrl Pts',(-0.309574522,2.187438859,7.499022561));
#119614=CARTESIAN_POINT('Ctrl Pts',(-0.02466246,2.232664075,7.499959451));
#119615=CARTESIAN_POINT('Ctrl Pts',(-0.579700987,2.103262031,7.226786752));
#119616=CARTESIAN_POINT('Ctrl Pts',(-0.458219089,2.123129682,7.236531495));
#119617=CARTESIAN_POINT('Ctrl Pts',(-0.336478302,2.142857143,7.242187677));
#119618=CARTESIAN_POINT('Ctrl Pts',(-0.061358598,2.187438859,7.254969977));
#119619=CARTESIAN_POINT('Ctrl Pts',(0.213937947,2.232664075,7.24684279900001));
#119620=CARTESIAN_POINT('Ctrl Pts',(0.213937946177155,2.232664075,7.24684279987291));
#119621=CARTESIAN_POINT('Ctrl Pts',(0.0652582714129358,2.2082392481818,
7.25123205215457));
#119622=CARTESIAN_POINT('Ctrl Pts',(-0.0832151217912876,2.18398304100009,
7.25103147792061));
#119623=CARTESIAN_POINT('Ctrl Pts',(-0.231066464265715,2.15996116639334,
7.24631687763066));
#119624=CARTESIAN_POINT('Ctrl Pts',(-0.266240708327531,2.15424629586123,
7.2451952611578));
#119625=CARTESIAN_POINT('Ctrl Pts',(-0.301379809906624,2.1485446709918,
7.24381838362196));
#119626=CARTESIAN_POINT('Ctrl Pts',(-0.336478303285617,2.14285714284189,
7.24218767723706));
#119627=CARTESIAN_POINT('Ctrl Pts',(-0.415913000634215,2.12998516353286,
7.23849707277838));
#119628=CARTESIAN_POINT('Ctrl Pts',(-0.49543432170632,2.11704095620001,
7.23349237724681));
#119629=CARTESIAN_POINT('Ctrl Pts',(-0.574977334691461,2.10403448761162,
7.22716410912341));
#119630=CARTESIAN_POINT('Ctrl Pts',(-1.353927101,3.785444214,7.122456136));
#119631=CARTESIAN_POINT('Ctrl Pts',(-0.968373059999999,3.720864611,7.195747154));
#119632=CARTESIAN_POINT('Ctrl Pts',(-0.577160368,3.655724827,7.2269901));
#119633=CARTESIAN_POINT('Ctrl Pts',(-1.641499383,3.785444214,7.318160956));
#119634=CARTESIAN_POINT('Ctrl Pts',(-1.245351414,3.720864611,7.407018888));
#119635=CARTESIAN_POINT('Ctrl Pts',(-0.841926282,3.655724827,7.452594188));
#119636=CARTESIAN_POINT('',(-1.34934427538633,3.78467661253199,7.12332577179078));
#119637=CARTESIAN_POINT('Origin',(0.0106253979274054,3.6250144669058,-0.197552907747238));
#119638=CARTESIAN_POINT('Ctrl Pts',(-1.39775963841221,3.74576903859142,
7.3686001377517));
#119639=CARTESIAN_POINT('Ctrl Pts',(-1.39215392831734,3.75001846750314,
7.34045544110582));
#119640=CARTESIAN_POINT('Ctrl Pts',(-1.38653968409124,3.75433282935595,
7.31232213507245));
#119641=CARTESIAN_POINT('Ctrl Pts',(-1.38096227129015,3.75872286883793,
7.28419340331767));
#119642=CARTESIAN_POINT('Ctrl Pts',(-1.37564367939182,3.76290918770205,
7.25736999071461));
#119643=CARTESIAN_POINT('Ctrl Pts',(-1.37034856584378,3.76716275954374,
7.23055231415295));
#119644=CARTESIAN_POINT('Ctrl Pts',(-1.36507845944258,3.77148708937521,
7.20374123248363));
#119645=CARTESIAN_POINT('Ctrl Pts',(-1.35980819818422,3.77581154627309,
7.17692936299568));
#119646=CARTESIAN_POINT('Ctrl Pts',(-1.35456290478237,3.78020679563467,
7.15012388873262));
#119647=CARTESIAN_POINT('Ctrl Pts',(-1.34934427553073,3.78467661261598,
7.12332577112288));
#119648=CARTESIAN_POINT('Ctrl Pts',(-2.117255923,3.655724827,6.933954669));
#119649=CARTESIAN_POINT('Ctrl Pts',(-1.84081698,3.703213228,7.018364219));
#119650=CARTESIAN_POINT('Ctrl Pts',(-1.558535692,3.75,7.080499029));
#119651=CARTESIAN_POINT('Ctrl Pts',(-1.451936835,3.76766825,7.103963212));
#119652=CARTESIAN_POINT('Ctrl Pts',(-1.344679932,3.785449891,7.124207737));
#119653=CARTESIAN_POINT('Ctrl Pts',(-1.953843178,3.655724827,7.241028714));
#119654=CARTESIAN_POINT('Ctrl Pts',(-1.665161983,3.703213228,7.318923417));
#119655=CARTESIAN_POINT('Ctrl Pts',(-1.371195932,3.75,7.373589473));
#119656=CARTESIAN_POINT('Ctrl Pts',(-1.260184519,3.76766825,7.39423320399999));
#119657=CARTESIAN_POINT('Ctrl Pts',(-1.148601964,3.785449891,7.411525722));
#119658=CARTESIAN_POINT('Ctrl Pts',(-2.11725591807228,3.65572482784652,
6.93395467050466));
#119659=CARTESIAN_POINT('Ctrl Pts',(-1.9749657670162,3.68016831499129,6.97740241147478));
#119660=CARTESIAN_POINT('Ctrl Pts',(-1.83165561670273,3.70444732820564,
7.01636901394677));
#119661=CARTESIAN_POINT('Ctrl Pts',(-1.68774656448177,3.72849594166796,
7.05081637380165));
#119662=CARTESIAN_POINT('Ctrl Pts',(-1.64472605968218,3.73568508977861,
7.06111414720158));
#119663=CARTESIAN_POINT('Ctrl Pts',(-1.6016520313209,3.74285367318542,7.07100840506992));
#119664=CARTESIAN_POINT('Ctrl Pts',(-1.55853569152624,3.75000000007635,
7.08049902912192));
#119665=CARTESIAN_POINT('Ctrl Pts',(-1.48913063931403,3.76150355506906,
7.09577623651641));
#119666=CARTESIAN_POINT('Ctrl Pts',(-1.41938586396231,3.77306479256719,
7.11005806111148));
#119667=CARTESIAN_POINT('Ctrl Pts',(-1.34934427541734,3.7846766123156,7.12332577109486));
#119668=CARTESIAN_POINT('Ctrl Pts',(-2.853390569,3.785444214,6.664882764));
#119669=CARTESIAN_POINT('Ctrl Pts',(-2.492605969,3.720864611,6.819343002));
#119670=CARTESIAN_POINT('Ctrl Pts',(-2.117255923,3.655724827,6.933954669));
#119671=CARTESIAN_POINT('Ctrl Pts',(-3.176310322,3.785444214,6.794192575));
#119672=CARTESIAN_POINT('Ctrl Pts',(-2.808525901,3.720864611,6.96613316000001));
#119673=CARTESIAN_POINT('Ctrl Pts',(-2.424329967,3.655724827,7.097367414));
#119674=CARTESIAN_POINT('',(-2.84910183335486,3.7846766124451,6.6667172411859));
#119675=CARTESIAN_POINT('Origin',(0.0528447207396793,3.62501418821225,-0.190649488831013));
#119676=CARTESIAN_POINT('Ctrl Pts',(-2.94911201019669,3.74576903853266,
6.89584935663054));
#119677=CARTESIAN_POINT('Ctrl Pts',(-2.93758708077133,3.75001846748317,
6.86956772922826));
#119678=CARTESIAN_POINT('Ctrl Pts',(-2.92605626518708,3.75433282933,6.84329906083679));
#119679=CARTESIAN_POINT('Ctrl Pts',(-2.91456240336134,3.75872286881353,
6.81702694207654));
#119680=CARTESIAN_POINT('Ctrl Pts',(-2.90360191637789,3.76290918768055,
6.79197398598008));
#119681=CARTESIAN_POINT('Ctrl Pts',(-2.89266559197175,3.76716275952688,
6.76692158464856));
#119682=CARTESIAN_POINT('Ctrl Pts',(-2.88175510775647,3.77148708936756,
6.74187024814746));
#119683=CARTESIAN_POINT('Ctrl Pts',(-2.87084430300772,3.77581154625049,
6.71681817567609));
#119684=CARTESIAN_POINT('Ctrl Pts',(-2.85995925715714,3.78020679560255,
6.69176698148066));
#119685=CARTESIAN_POINT('Ctrl Pts',(-2.84910183346196,3.78467661243857,
6.66671724045537));
#119686=CARTESIAN_POINT('Ctrl Pts',(-3.558350943,3.655724827,6.316695225));
#119687=CARTESIAN_POINT('Ctrl Pts',(-3.306520548,3.703213228,6.458557527));
#119688=CARTESIAN_POINT('Ctrl Pts',(-3.044195986,3.75,6.579921793));
#119689=CARTESIAN_POINT('Ctrl Pts',(-2.945133458,3.76766825,6.625752999));
#119690=CARTESIAN_POINT('Ctrl Pts',(-2.844736136,3.785449891,6.668581282));
#119691=CARTESIAN_POINT('Ctrl Pts',(-3.46477054,3.655724827,6.651718958));
#119692=CARTESIAN_POINT('Ctrl Pts',(-3.19958361,3.703213228,6.78985045));
#119693=CARTESIAN_POINT('Ctrl Pts',(-2.924241908,3.75,6.906432456));
#119694=CARTESIAN_POINT('Ctrl Pts',(-2.820263672,3.76766825,6.95045772));
#119695=CARTESIAN_POINT('Ctrl Pts',(-2.715007236,3.785449891,6.991332899));
#119696=CARTESIAN_POINT('Ctrl Pts',(-3.55835093856568,3.65572482783619,
6.31669522749796));
#119697=CARTESIAN_POINT('Ctrl Pts',(-3.42872747054081,3.68016830784389,
6.38971533905775));
#119698=CARTESIAN_POINT('Ctrl Pts',(-3.29714453855422,3.70444731404074,
6.45857835112766));
#119699=CARTESIAN_POINT('Ctrl Pts',(-3.16400520355533,3.72849592062057,
6.52315652692829));
#119700=CARTESIAN_POINT('Ctrl Pts',(-3.12420417265987,3.73568507575255,
6.54246170049126));
#119701=CARTESIAN_POINT('Ctrl Pts',(-3.08426412533397,3.74285366614081,
6.56138429775543));
#119702=CARTESIAN_POINT('Ctrl Pts',(-3.04419598618343,3.74999999996728,
6.57992179291514));
#119703=CARTESIAN_POINT('Ctrl Pts',(-2.97969773445506,3.76150355493518,
6.60976186182413));
#119704=CARTESIAN_POINT('Ctrl Pts',(-2.91465372285346,3.77306479257878,
6.63870285047732));
#119705=CARTESIAN_POINT('Ctrl Pts',(-2.84910183331928,3.78467661222203,
6.66671724047858));
#119706=CARTESIAN_POINT('Ctrl Pts',(-4.219432665,3.785444214,5.895666882));
#119707=CARTESIAN_POINT('Ctrl Pts',(-3.900287394,3.720864611,6.124073949));
#119708=CARTESIAN_POINT('Ctrl Pts',(-3.558350943,3.655724827,6.316695225));
#119709=CARTESIAN_POINT('Ctrl Pts',(-4.56260052,3.785444214,5.9525353));
#119710=CARTESIAN_POINT('Ctrl Pts',(-4.240376838,3.720864611,6.199518789));
#119711=CARTESIAN_POINT('Ctrl Pts',(-3.893374677,3.655724827,6.41027562800001));
#119712=CARTESIAN_POINT('',(-4.21563855624423,3.78467661244694,5.89838042167661));
#119713=CARTESIAN_POINT('Origin',(0.0925935034102404,3.6250141983369,-0.174832560614677));
#119714=CARTESIAN_POINT('Ctrl Pts',(-4.36256718214553,3.74576903864837,
6.10065632342285));
#119715=CARTESIAN_POINT('Ctrl Pts',(-4.34566192601587,3.75001846755915,
6.07746666510329));
#119716=CARTESIAN_POINT('Ctrl Pts',(-4.32875370718208,3.75433282938854,
6.05429092807439));
#119717=CARTESIAN_POINT('Ctrl Pts',(-4.31188083645845,3.75872286886535,
6.03110387735168));
#119718=CARTESIAN_POINT('Ctrl Pts',(-4.29579095460153,3.76290918770143,
6.00899282625375));
#119719=CARTESIAN_POINT('Ctrl Pts',(-4.27972478969674,3.76716275952398,
5.98687712269222));
#119720=CARTESIAN_POINT('Ctrl Pts',(-4.2636840897836,3.7714870893529,5.96475690416098));
#119721=CARTESIAN_POINT('Ctrl Pts',(-4.24764291863144,3.77581154622073,
5.94263603578839));
#119722=CARTESIAN_POINT('Ctrl Pts',(-4.23162709297523,3.78020679556982,
5.92051048772824));
#119723=CARTESIAN_POINT('Ctrl Pts',(-4.21563855622686,3.78467661242271,
5.89838042089163));
#119724=CARTESIAN_POINT('Ctrl Pts',(-4.833061429,3.655724827,5.404074132));
#119725=CARTESIAN_POINT('Ctrl Pts',(-4.61761489,3.703213228,5.596755863));
#119726=CARTESIAN_POINT('Ctrl Pts',(-4.38751306,3.75,5.771674726));
#119727=CARTESIAN_POINT('Ctrl Pts',(-4.300618913,3.76766825,5.83772994));
#119728=CARTESIAN_POINT('Ctrl Pts',(-4.21177564,3.785449891,5.901139378));
#119729=CARTESIAN_POINT('Ctrl Pts',(-4.813689083,3.655724827,5.751382217));
#119730=CARTESIAN_POINT('Ctrl Pts',(-4.584396264,3.703213228,5.943291623));
#119731=CARTESIAN_POINT('Ctrl Pts',(-4.340553583,3.75,6.116338332));
#119732=CARTESIAN_POINT('Ctrl Pts',(-4.24847043,3.76766825,6.181686558));
#119733=CARTESIAN_POINT('Ctrl Pts',(-4.154461786,3.785449891,6.244233121));
#119734=CARTESIAN_POINT('Ctrl Pts',(-4.83306142520631,3.6557248278362,5.40407413539284));
#119735=CARTESIAN_POINT('Ctrl Pts',(-4.72216563184353,3.68016831124059,
5.50325230504341));
#119736=CARTESIAN_POINT('Ctrl Pts',(-4.60846253156385,3.70444732075457,
5.59879179157711));
#119737=CARTESIAN_POINT('Ctrl Pts',(-4.4923183023693,3.72849593057745,5.69048119835488));
#119738=CARTESIAN_POINT('Ctrl Pts',(-4.45759785485245,3.73568508238464,
5.71789105985171));
#119739=CARTESIAN_POINT('Ctrl Pts',(-4.42265939864353,3.74285366946605,
5.74495717419604));
#119740=CARTESIAN_POINT('Ctrl Pts',(-4.38751305994637,3.75000000000682,
5.77167472617292));
#119741=CARTESIAN_POINT('Ctrl Pts',(-4.33093747394232,3.7615035549861,5.81468236902783));
#119742=CARTESIAN_POINT('Ctrl Pts',(-4.27363561251273,3.77306479258905,
5.85692927332391));
#119743=CARTESIAN_POINT('Ctrl Pts',(-4.2156385560841,3.78467661217519,5.89838042094478));
#119744=CARTESIAN_POINT('Ctrl Pts',(-5.388178779,3.785444214,4.85077617));
#119745=CARTESIAN_POINT('Ctrl Pts',(-5.125595715,3.720864611,5.142450006));
#119746=CARTESIAN_POINT('Ctrl Pts',(-4.83306142900001,3.655724827,5.404074132));
#119747=CARTESIAN_POINT('Ctrl Pts',(-5.735548589,3.785444214,4.83254409));
#119748=CARTESIAN_POINT('Ctrl Pts',(-5.473952467,3.720864611,5.143021809));
#119749=CARTESIAN_POINT('Ctrl Pts',(-5.180369514,3.655724827,5.423446478));
#119750=CARTESIAN_POINT('',(-5.38505670423473,3.78467661256409,4.85424188857806));
#119751=CARTESIAN_POINT('Origin',(0.128012373723314,3.62501421072075,-0.15084001019758));
#119752=CARTESIAN_POINT('Ctrl Pts',(-5.57203356107251,3.74576903855143,
5.02020338136684));
#119753=CARTESIAN_POINT('Ctrl Pts',(-5.55053844964326,3.7500184675163,5.00119001457086));
#119754=CARTESIAN_POINT('Ctrl Pts',(-5.52904343725189,3.75433282935624,
4.98219088070486));
#119755=CARTESIAN_POINT('Ctrl Pts',(-5.50758051440555,3.75872286883733,
4.96317309889155));
#119756=CARTESIAN_POINT('Ctrl Pts',(-5.48711358252958,3.76290918771084,
4.94503784081921));
#119757=CARTESIAN_POINT('Ctrl Pts',(-5.46666881295276,3.76716275956891,
4.92689294063437));
#119758=CARTESIAN_POINT('Ctrl Pts',(-5.44624794248302,3.77148708941655,
4.90873815689551));
#119759=CARTESIAN_POINT('Ctrl Pts',(-5.42582647195078,3.77581154633361,
4.89058283968258));
#119760=CARTESIAN_POINT('Ctrl Pts',(-5.40542874841309,3.78020679571413,
4.87241750373948));
#119761=CARTESIAN_POINT('Ctrl Pts',(-5.38505670397224,3.78467661270115,
4.85424188794923));
#119762=CARTESIAN_POINT('Ctrl Pts',(-5.881783334,3.655724827,4.238764539));
#119763=CARTESIAN_POINT('Ctrl Pts',(-5.712794691,3.703213228,4.473256116));
#119764=CARTESIAN_POINT('Ctrl Pts',(-5.5256749,3.75,4.693550565));
#119765=CARTESIAN_POINT('Ctrl Pts',(-5.455012208,3.76766825,4.776741117));
#119766=CARTESIAN_POINT('Ctrl Pts',(-5.381877196,3.785449891,4.857766756));
#119767=CARTESIAN_POINT('Ctrl Pts',(-5.937524875,3.655724827,4.582117236));
#119768=CARTESIAN_POINT('Ctrl Pts',(-5.75484764300001,3.703213228,4.818831084));
#119769=CARTESIAN_POINT('Ctrl Pts',(-5.553905796,3.75,5.040251027));
#119770=CARTESIAN_POINT('Ctrl Pts',(-5.478023433,3.76766825,5.123866603));
#119771=CARTESIAN_POINT('Ctrl Pts',(-5.399658321,3.785449891,5.205159941));
#119772=CARTESIAN_POINT('Ctrl Pts',(-5.88178333102439,3.65572482783619,
4.23876454312901));
#119773=CARTESIAN_POINT('Ctrl Pts',(-5.79480058251351,3.68016831447287,
4.35946331600408));
#119774=CARTESIAN_POINT('Ctrl Pts',(-5.70429395042422,3.7044473271979,4.47721196332595));
#119775=CARTESIAN_POINT('Ctrl Pts',(-5.61057560779318,3.72849594018888,
4.59172531338442));
#119776=CARTESIAN_POINT('Ctrl Pts',(-5.58255922733452,3.73568508878181,
4.62595820198196));
#119777=CARTESIAN_POINT('Ctrl Pts',(-5.55425603991417,3.74285367266895,
4.65990224573283));
#119778=CARTESIAN_POINT('Ctrl Pts',(-5.52567489984892,3.75000000003778,
4.69355056517787));
#119779=CARTESIAN_POINT('Ctrl Pts',(-5.47966739129328,3.76150355502565,
4.74771479136725));
#119780=CARTESIAN_POINT('Ctrl Pts',(-5.43278705104974,3.77306479261622,
4.80129219296576));
#119781=CARTESIAN_POINT('Ctrl Pts',(-5.38505670388047,3.78467661243118,
4.8542418879857));
#119782=CARTESIAN_POINT('Ctrl Pts',(-6.304979642,3.785444214,3.579068554));
#119783=CARTESIAN_POINT('Ctrl Pts',(-6.11123687700001,3.720864611,3.920370815));
#119784=CARTESIAN_POINT('Ctrl Pts',(-5.881783334,3.655724827,4.238764539));
#119785=CARTESIAN_POINT('Ctrl Pts',(-6.640308781,3.785444214,3.48658849));
#119786=CARTESIAN_POINT('Ctrl Pts',(-6.451572163,3.720864611,3.846042846));
#119787=CARTESIAN_POINT('Ctrl Pts',(-6.22513603100001,3.655724827,4.183022998));
#119788=CARTESIAN_POINT('',(-6.30267558725977,3.78467661246027,3.58312440082087));
#119789=CARTESIAN_POINT('Origin',(0.15744564959693,3.62501421946758,-0.119794573750415));
#119790=CARTESIAN_POINT('Ctrl Pts',(-6.52095784396231,3.7457690385946,3.70501130873339));
#119791=CARTESIAN_POINT('Ctrl Pts',(-6.49587796423671,3.75001846753171,
3.6910632775486));
#119792=CARTESIAN_POINT('Ctrl Pts',(-6.47080124111466,3.75433282936697,
3.67712912506813));
#119793=CARTESIAN_POINT('Ctrl Pts',(-6.44575184852869,3.75872286883072,
3.66316986236309));
#119794=CARTESIAN_POINT('Ctrl Pts',(-6.42186487777182,3.76290918767787,
3.64985838189991));
#119795=CARTESIAN_POINT('Ctrl Pts',(-6.3979974783993,3.76716275950069,3.63653272053864));
#119796=CARTESIAN_POINT('Ctrl Pts',(-6.37415129467673,3.77148708931986,
3.62319226906006));
#119797=CARTESIAN_POINT('Ctrl Pts',(-6.35030441032532,3.77581154619291,
3.60985142562337));
#119798=CARTESIAN_POINT('Ctrl Pts',(-6.32647856400905,3.78020679553667,
3.59649569275204));
#119799=CARTESIAN_POINT('Ctrl Pts',(-6.30267558683402,3.78467661244032,
3.58312440024228));
#119800=CARTESIAN_POINT('Ctrl Pts',(-6.655479587,3.655724827,2.875255027));
#119801=CARTESIAN_POINT('Ctrl Pts',(-6.540850562,3.703213228,3.140591884));
#119802=CARTESIAN_POINT('Ctrl Pts',(-6.405462322,3.75,3.395961195));
#119803=CARTESIAN_POINT('Ctrl Pts',(-6.354335194,3.76766825,3.492397189));
#119804=CARTESIAN_POINT('Ctrl Pts',(-6.300328155,3.785449891,3.587250358));
#119805=CARTESIAN_POINT('Ctrl Pts',(-6.783728602,3.655724827,3.198597545));
#119806=CARTESIAN_POINT('Ctrl Pts',(-6.656208743,3.703213228,3.46904736));
#119807=CARTESIAN_POINT('Ctrl Pts',(-6.507563547,3.75,3.728487185));
#119808=CARTESIAN_POINT('Ctrl Pts',(-6.451430149,3.76766825,3.82646034));
#119809=CARTESIAN_POINT('Ctrl Pts',(-6.392372834,3.785449891,3.922699268));
#119810=CARTESIAN_POINT('Ctrl Pts',(-6.65547958491555,3.65572482786355,
2.87525503182498));
#119811=CARTESIAN_POINT('Ctrl Pts',(-6.59647713513738,3.68016830533402,
3.01183060287484));
#119812=CARTESIAN_POINT('Ctrl Pts',(-6.53339900144488,3.70444730902973,
3.14628255331846));
#119813=CARTESIAN_POINT('Ctrl Pts',(-6.46648875464711,3.72849591317344,
3.27826527057431));
#119814=CARTESIAN_POINT('Ctrl Pts',(-6.44648641654104,3.73568507080001,
3.3177205567383));
#119815=CARTESIAN_POINT('Ctrl Pts',(-6.42614188288712,3.7428536636702,3.35695540555018));
#119816=CARTESIAN_POINT('Ctrl Pts',(-6.40546232214056,3.74999999996442,
3.39596119492824));
#119817=CARTESIAN_POINT('Ctrl Pts',(-6.37217415113294,3.76150355492965,
3.45874934637612));
#119818=CARTESIAN_POINT('Ctrl Pts',(-6.33790740515646,3.77306479242226,
3.5211520252893));
#119819=CARTESIAN_POINT('Ctrl Pts',(-6.3026755867305,3.78467661218534,3.58312440034133));
#119820=CARTESIAN_POINT('Ctrl Pts',(-6.926966664,3.785444214,2.140007671));
#119821=CARTESIAN_POINT('Ctrl Pts',(-6.811123395,3.720864611,2.514979442));
#119822=CARTESIAN_POINT('Ctrl Pts',(-6.655479587,3.655724827,2.875255027));
#119823=CARTESIAN_POINT('Ctrl Pts',(-7.234575514,3.785444214,1.977603887));
#119824=CARTESIAN_POINT('Ctrl Pts',(-7.127523515,3.720864611,2.369227193));
#119825=CARTESIAN_POINT('Ctrl Pts',(-6.978822105,3.655724827,2.747006012));
#119826=CARTESIAN_POINT('',(-6.92558836415996,3.78467661244452,2.1444639974593));
#119827=CARTESIAN_POINT('Origin',(0.179517066360537,3.62501419796814,-0.083147728267117));
#119828=CARTESIAN_POINT('Ctrl Pts',(-7.16496938531577,3.74576903859088,
2.21657702476992));
#119829=CARTESIAN_POINT('Ctrl Pts',(-7.13747744483996,3.75001846753709,
2.20834652356073));
#119830=CARTESIAN_POINT('Ctrl Pts',(-7.10999157065178,3.75433282938089,
2.20012889801899));
#119831=CARTESIAN_POINT('Ctrl Pts',(-7.08252699007823,3.75872286885859,
2.19188087402488));
#119832=CARTESIAN_POINT('Ctrl Pts',(-7.05633690862041,3.76290918771448,
2.18401560116213));
#119833=CARTESIAN_POINT('Ctrl Pts',(-7.03016289250742,3.76716275954892,
2.17613227165504));
#119834=CARTESIAN_POINT('Ctrl Pts',(-7.00400641660713,3.77148708937527,
2.16822993708759));
#119835=CARTESIAN_POINT('Ctrl Pts',(-6.97784917217286,3.7758115462598,2.16032737033241));
#119836=CARTESIAN_POINT('Ctrl Pts',(-6.95170927313872,3.78020679561047,
2.15240573970377));
#119837=CARTESIAN_POINT('Ctrl Pts',(-6.92558836364052,3.78467661253422,
2.14446399698953));
#119838=CARTESIAN_POINT('Ctrl Pts',(-7.117973011,3.655724827,1.377301786));
#119839=CARTESIAN_POINT('Ctrl Pts',(-7.063063531,3.703213228,1.661077066));
#119840=CARTESIAN_POINT('Ctrl Pts',(-6.985737446,3.75,1.939580454));
#119841=CARTESIAN_POINT('Ctrl Pts',(-6.95653653,3.76766825,2.044752649));
#119842=CARTESIAN_POINT('Ctrl Pts',(-6.924182773,3.785449891,2.148998121));
#119843=CARTESIAN_POINT('Ctrl Pts',(-7.312732719,3.655724827,1.665514988));
#119844=CARTESIAN_POINT('Ctrl Pts',(-7.24633292000001,3.703213228,1.957054837));
#119845=CARTESIAN_POINT('Ctrl Pts',(-7.156934859,3.75,2.242383426));
#119846=CARTESIAN_POINT('Ctrl Pts',(-7.123175161,3.76766825,2.350133045));
#119847=CARTESIAN_POINT('Ctrl Pts',(-7.086187098,3.785449891,2.456817537));
#119848=CARTESIAN_POINT('Ctrl Pts',(-7.11797301003313,3.65572482783619,
1.37730179099681));
#119849=CARTESIAN_POINT('Ctrl Pts',(-7.08970970895861,3.68016831136589,
1.52336811954265));
#119850=CARTESIAN_POINT('Ctrl Pts',(-7.05700949318934,3.70444732101029,
1.66823662756823));
#119851=CARTESIAN_POINT('Ctrl Pts',(-7.02003594244959,3.72849593099671,
1.81151742205105));
#119852=CARTESIAN_POINT('Ctrl Pts',(-7.00898297661549,3.73568508267999,
1.85435014150631));
#119853=CARTESIAN_POINT('Ctrl Pts',(-6.99754842866315,3.74285366964143,
1.89704113948066));
#119854=CARTESIAN_POINT('Ctrl Pts',(-6.98573744594291,3.75000000006696,
1.93958045449333));
#119855=CARTESIAN_POINT('Ctrl Pts',(-6.96672513038322,3.76150355507051,
2.00805662662846));
#119856=CARTESIAN_POINT('Ctrl Pts',(-6.94667425285339,3.77306479261547,
2.07636670287174));
#119857=CARTESIAN_POINT('Ctrl Pts',(-6.92558836356273,3.78467661226242,
2.1444639970924));
#119858=CARTESIAN_POINT('Ctrl Pts',(-7.225056424,3.785444214,0.600882408));
#119859=CARTESIAN_POINT('Ctrl Pts',(-7.192529353,3.720864611,0.991990426));
#119860=CARTESIAN_POINT('Ctrl Pts',(-7.117973011,3.655724827,1.377301786));
#119861=CARTESIAN_POINT('Ctrl Pts',(-7.490561537,3.785444214,0.376148724));
#119862=CARTESIAN_POINT('Ctrl Pts',(-7.470199788,3.720864611,0.781629111));
#119863=CARTESIAN_POINT('Ctrl Pts',(-7.406186214,3.655724827,1.182542078));
#119864=CARTESIAN_POINT('',(-7.22466832603432,3.78467661248487,0.605530842000411));
#119865=CARTESIAN_POINT('Origin',(0.193194190418122,3.62501420910875,-0.042612894957625));
#119866=CARTESIAN_POINT('Ctrl Pts',(-7.47395492118949,3.74576903857413,
0.624498063269066));
#119867=CARTESIAN_POINT('Ctrl Pts',(-7.44533641265202,3.75001846749754,
0.622369941210292));
#119868=CARTESIAN_POINT('Ctrl Pts',(-7.41672659636916,3.75433282935662,
0.620253089576217));
#119869=CARTESIAN_POINT('Ctrl Pts',(-7.38813104109206,3.75872286884412,
0.618101972734711));
#119870=CARTESIAN_POINT('Ctrl Pts',(-7.36086246801177,3.76290918771187,
0.616050678880527));
#119871=CARTESIAN_POINT('Ctrl Pts',(-7.33360570302689,3.76716275955502,
0.61397829698979));
#119872=CARTESIAN_POINT('Ctrl Pts',(-7.30636198266434,3.77148708938627,
0.611883583750487));
#119873=CARTESIAN_POINT('Ctrl Pts',(-7.2791174617877,3.77581154628119,0.609788808961313));
#119874=CARTESIAN_POINT('Ctrl Pts',(-7.25188578263253,3.78020679563828,
0.607671687265006));
#119875=CARTESIAN_POINT('Ctrl Pts',(-7.22466832542905,3.7846766125672,0.605530841610901));
#119876=CARTESIAN_POINT('Ctrl Pts',(-7.247637929,3.655724827,-0.185052556));
#119877=CARTESIAN_POINT('Ctrl Pts',(-7.255015499,3.703213228,0.103892131));
#119878=CARTESIAN_POINT('Ctrl Pts',(-7.23936725,3.75,0.392507087));
#119879=CARTESIAN_POINT('Ctrl Pts',(-7.233457948,3.76766825,0.501497748));
#119880=CARTESIAN_POINT('Ctrl Pts',(-7.2242703,3.785449891,0.610261121));
#119881=CARTESIAN_POINT('Ctrl Pts',(-7.499801582,3.655724827,0.054554802));
#119882=CARTESIAN_POINT('Ctrl Pts',(-7.497626623,3.703213228,0.353552605));
#119883=CARTESIAN_POINT('Ctrl Pts',(-7.471655851,3.75,0.651428311));
#119884=CARTESIAN_POINT('Ctrl Pts',(-7.461848419,3.76766825,0.76391614));
#119885=CARTESIAN_POINT('Ctrl Pts',(-7.448659129,3.785449891,0.876057748));
#119886=CARTESIAN_POINT('Ctrl Pts',(-7.24763792912991,3.65572482783619,
-0.18505255091221));
#119887=CARTESIAN_POINT('Ctrl Pts',(-7.25143535144642,3.68016831243512,
-0.0363253910426296));
#119888=CARTESIAN_POINT('Ctrl Pts',(-7.2506420949807,3.70444732310703,0.112185757815467));
#119889=CARTESIAN_POINT('Ctrl Pts',(-7.24533410011286,3.72849593402264,
0.260064953471494));
#119890=CARTESIAN_POINT('Ctrl Pts',(-7.24374731512805,3.73568508466364,
0.304272322369906));
#119891=CARTESIAN_POINT('Ctrl Pts',(-7.24175740340817,3.7428536705816,0.348423312034834));
#119892=CARTESIAN_POINT('Ctrl Pts',(-7.23936725054934,3.74999999996199,
0.392507087363699));
#119893=CARTESIAN_POINT('Ctrl Pts',(-7.23551978532587,3.76150355491796,
0.46346941028073));
#119894=CARTESIAN_POINT('Ctrl Pts',(-7.23062233359156,3.77306479251089,
0.534492781363057));
#119895=CARTESIAN_POINT('Ctrl Pts',(-7.2246683253825,3.78467661233474,0.605530841717469));
#119896=CARTESIAN_POINT('Ctrl Pts',(-7.185310576,3.785444214,-0.966339449));
#119897=CARTESIAN_POINT('Ctrl Pts',(-7.237620632,3.720864611,-0.57738296));
#119898=CARTESIAN_POINT('Ctrl Pts',(-7.24763792900001,3.655724827,-0.185052556));
#119899=CARTESIAN_POINT('Ctrl Pts',(-7.39629722700001,3.785444214,-1.242894736));
#119900=CARTESIAN_POINT('Ctrl Pts',(-7.463577823,3.720864611,-0.842517081));
#119901=CARTESIAN_POINT('Ctrl Pts',(-7.48724528700001,3.655724827,-0.437216209));
#119902=CARTESIAN_POINT('',(-7.18593082770886,3.7846766124854,-0.961716263426633));
#119903=CARTESIAN_POINT('Origin',(0.197837913337127,3.62501423301475,-8.55908097693869E-5));
#119904=CARTESIAN_POINT('Ctrl Pts',(-7.43346663201529,3.74576903857242,
-0.996781734613965));
#119905=CARTESIAN_POINT('Ctrl Pts',(-7.40505972491877,3.7500184674993,-0.992707968931452));
#119906=CARTESIAN_POINT('Ctrl Pts',(-7.37666372970027,3.75433282934856,
-0.988625064820828));
#119907=CARTESIAN_POINT('Ctrl Pts',(-7.34827429605646,3.75872286884045,
-0.98457869056506));
#119908=CARTESIAN_POINT('Ctrl Pts',(-7.32120227962763,3.76290918769198,
-0.980720089097213));
#119909=CARTESIAN_POINT('Ctrl Pts',(-7.29413726191584,3.7671627595281,-0.976884621059635));
#119910=CARTESIAN_POINT('Ctrl Pts',(-7.26708018324357,3.77148708936403,
-0.973073766491055));
#119911=CARTESIAN_POINT('Ctrl Pts',(-7.24002230959502,3.77581154625505,
-0.969262799954033));
#119912=CARTESIAN_POINT('Ctrl Pts',(-7.2129721734837,3.78020679562023,-0.965476418463916));
#119913=CARTESIAN_POINT('Ctrl Pts',(-7.18593082702751,3.78467661255006,
-0.961716263674782));
#119914=CARTESIAN_POINT('Ctrl Pts',(-7.038411352,3.655724827,-1.738754046));
#119915=CARTESIAN_POINT('Ctrl Pts',(-7.107731005,3.703213228,-1.458150685));
#119916=CARTESIAN_POINT('Ctrl Pts',(-7.154492288,3.75,-1.172919475));
#119917=CARTESIAN_POINT('Ctrl Pts',(-7.172150913,3.76766825,-1.06520663));
#119918=CARTESIAN_POINT('Ctrl Pts',(-7.186558977,3.785449891,-0.957011012));
#119919=CARTESIAN_POINT('Ctrl Pts',(-7.336188059,3.655724827,-1.558956307));
#119920=CARTESIAN_POINT('Ctrl Pts',(-7.39833963800001,3.703213228,-1.266481354));
#119921=CARTESIAN_POINT('Ctrl Pts',(-7.43701052,3.75,-0.969986869));
#119922=CARTESIAN_POINT('Ctrl Pts',(-7.451613939,3.76766825,-0.858020634));
#119923=CARTESIAN_POINT('Ctrl Pts',(-7.462840138,3.785449891,-0.745665527));
#119924=CARTESIAN_POINT('Ctrl Pts',(-7.03841135322059,3.65572482783619,
-1.73875404105908));
#119925=CARTESIAN_POINT('Ctrl Pts',(-7.07409192112379,3.68016830162473,
-1.59432043712552));
#119926=CARTESIAN_POINT('Ctrl Pts',(-7.10524270618244,3.70444730165851,
-1.44911093398924));
#119927=CARTESIAN_POINT('Ctrl Pts',(-7.13184845739956,3.72849590219442,
-1.30354807414556));
#119928=CARTESIAN_POINT('Ctrl Pts',(-7.13980206105466,3.73568506349874,
-1.26003307302222));
#119929=CARTESIAN_POINT('Ctrl Pts',(-7.14734984176541,3.74285366002429,
-1.21648647257524));
#119930=CARTESIAN_POINT('Ctrl Pts',(-7.15449228842347,3.74999999994902,
-1.17291947497001));
#119931=CARTESIAN_POINT('Ctrl Pts',(-7.16598957666898,3.76150355491072,
-1.10278912066276));
#119932=CARTESIAN_POINT('Ctrl Pts',(-7.17647455002868,3.77306479254669,
-1.03237342918396));
#119933=CARTESIAN_POINT('Ctrl Pts',(-7.18593082700197,3.78467661229154,
-0.961716263551076));
#119934=CARTESIAN_POINT('Ctrl Pts',(-6.809587591,3.785444214,-2.488376347));
#119935=CARTESIAN_POINT('Ctrl Pts',(-6.944288814,3.720864611,-2.119758561));
#119936=CARTESIAN_POINT('Ctrl Pts',(-7.038411352,3.655724827,-1.738754046));
#119937=CARTESIAN_POINT('Ctrl Pts',(-6.95619028,3.785444214,-2.803821818));
#119938=CARTESIAN_POINT('Ctrl Pts',(-7.107967253,3.720864611,-2.42726811));
#119939=CARTESIAN_POINT('Ctrl Pts',(-7.218209092,3.655724827,-2.036530753));
#119940=CARTESIAN_POINT('',(-6.81118718954655,3.78467661249988,-2.48399458494427));
#119941=CARTESIAN_POINT('Origin',(0.193231149625587,3.62501425022595,0.0424457680865267));
#119942=CARTESIAN_POINT('Ctrl Pts',(-7.04539770492945,3.74576903854636,
-2.57145312545179));
#119943=CARTESIAN_POINT('Ctrl Pts',(-7.01853067466861,3.75001846749528,
-2.56136795692049));
#119944=CARTESIAN_POINT('Ctrl Pts',(-6.99167626573214,3.75433282934435,
-2.55127620925497));
#119945=CARTESIAN_POINT('Ctrl Pts',(-6.96482041212457,3.75872286883609,
-2.54122154794212));
#119946=CARTESIAN_POINT('Ctrl Pts',(-6.93921080960062,3.76290918769569,
-2.5316334751332));
#119947=CARTESIAN_POINT('Ctrl Pts',(-6.91360306916377,3.76716275953997,
-2.52206949942425));
#119948=CARTESIAN_POINT('Ctrl Pts',(-6.88799779097978,3.77148708938402,
-2.51253126837146));
#119949=CARTESIAN_POINT('Ctrl Pts',(-6.86239176050391,3.77581154627836,
-2.50299275708217));
#119950=CARTESIAN_POINT('Ctrl Pts',(-6.83678800159914,3.78020679564683,
-2.49347991937481));
#119951=CARTESIAN_POINT('Ctrl Pts',(-6.81118718888813,3.78467661260747,
-2.48399458499447));
#119952=CARTESIAN_POINT('Ctrl Pts',(-6.500076484,3.655724827,-3.21115333));
#119953=CARTESIAN_POINT('Ctrl Pts',(-6.62809690900001,3.703213228,-2.952011995));
#119954=CARTESIAN_POINT('Ctrl Pts',(-6.735081219,3.75,-2.683501626));
#119955=CARTESIAN_POINT('Ctrl Pts',(-6.775482072,3.76766825,-2.58210313));
#119956=CARTESIAN_POINT('Ctrl Pts',(-6.812812143,3.785449891,-2.479534373));
#119957=CARTESIAN_POINT('Ctrl Pts',(-6.829542535,3.655724827,-3.099572351));
#119958=CARTESIAN_POINT('Ctrl Pts',(-6.953114514,3.703213228,-2.827296052));
#119959=CARTESIAN_POINT('Ctrl Pts',(-7.054618843,3.75,-2.54604654));
#119960=CARTESIAN_POINT('Ctrl Pts',(-7.092950272,3.76766825,-2.439837317));
#119961=CARTESIAN_POINT('Ctrl Pts',(-7.128067036,3.785449891,-2.332522311));
#119962=CARTESIAN_POINT('Ctrl Pts',(-6.50007648625421,3.65572482783619,
-3.21115332543699));
#119963=CARTESIAN_POINT('Ctrl Pts',(-6.5659718131589,3.68016830013526,-3.07776677391967));
#119964=CARTESIAN_POINT('Ctrl Pts',(-6.62761005750583,3.70444729873061,
-2.94264869413223));
#119965=CARTESIAN_POINT('Ctrl Pts',(-6.68488549041593,3.72849589790548,
-2.80620847119841));
#119966=CARTESIAN_POINT('Ctrl Pts',(-6.70200758579652,3.73568506065677,
-2.76542060819808));
#119967=CARTESIAN_POINT('Ctrl Pts',(-6.71874013893801,3.74285365862559,
-2.72451464466946));
#119968=CARTESIAN_POINT('Ctrl Pts',(-6.73508121915812,3.74999999998921,
-2.68350162598332));
#119969=CARTESIAN_POINT('Ctrl Pts',(-6.76138565968406,3.76150355498974,
-2.61748245745513));
#119970=CARTESIAN_POINT('Ctrl Pts',(-6.7867627926547,3.77306479254987,-2.55096700510787));
#119971=CARTESIAN_POINT('Ctrl Pts',(-6.81118718887542,3.78467661225419,
-2.48399458486229));
#119972=CARTESIAN_POINT('Ctrl Pts',(-6.115455858,3.785444214,-3.894059533));
#119973=CARTESIAN_POINT('Ctrl Pts',(-6.32624977,3.720864611,-3.563016607));
#119974=CARTESIAN_POINT('Ctrl Pts',(-6.500076484,3.655724827,-3.21115333));
#119975=CARTESIAN_POINT('Ctrl Pts',(-6.19081960600001,3.785444214,-4.233645309));
#119976=CARTESIAN_POINT('Ctrl Pts',(-6.419996035,3.720864611,-3.898522779));
#119977=CARTESIAN_POINT('Ctrl Pts',(-6.611657462,3.655724827,-3.540619381));
#119978=CARTESIAN_POINT('',(-6.11796000880229,3.78467661249981,-3.89012408040951));
#119979=CARTESIAN_POINT('Origin',(0.179589055403488,3.62501418376288,0.0829924647008767));
#119980=CARTESIAN_POINT('Ctrl Pts',(-6.32789381133271,3.74576903857982,
-4.02588622635888));
#119981=CARTESIAN_POINT('Ctrl Pts',(-6.30382293047905,3.75001846750999,
-4.01026122619376));
#119982=CARTESIAN_POINT('Ctrl Pts',(-6.27976579010809,3.75433282935617,
-3.99463251394156));
#119983=CARTESIAN_POINT('Ctrl Pts',(-6.25569926639655,3.75872286883614,
-3.97903971039016));
#119984=CARTESIAN_POINT('Ctrl Pts',(-6.23274955436762,3.76290918768585,
-3.96417049390017));
#119985=CARTESIAN_POINT('Ctrl Pts',(-6.20979648073913,3.76716275951515,
-3.94932521141505));
#119986=CARTESIAN_POINT('Ctrl Pts',(-6.18684027743799,3.77148708934838,
-3.93450560102785));
#119987=CARTESIAN_POINT('Ctrl Pts',(-6.16388339968018,3.77581154623106,
-3.91968555523829));
#119988=CARTESIAN_POINT('Ctrl Pts',(-6.140923221305,3.78020679559228,-3.90489107114311));
#119989=CARTESIAN_POINT('Ctrl Pts',(-6.11796000806892,3.78467661247508,
-3.89012408036331));
#119990=CARTESIAN_POINT('Ctrl Pts',(-5.657805263,3.655724827,-4.533402653));
#119991=CARTESIAN_POINT('Ctrl Pts',(-5.838540369,3.703213228,-4.307840506));
#119992=CARTESIAN_POINT('Ctrl Pts',(-6.000745237,3.75,-4.068606224));
#119993=CARTESIAN_POINT('Ctrl Pts',(-6.06199922,3.76766825,-3.978263357));
#119994=CARTESIAN_POINT('Ctrl Pts',(-6.120505785,3.785449891,-3.886117463));
#119995=CARTESIAN_POINT('Ctrl Pts',(-6.003555193,3.655724827,-4.495255837));
#119996=CARTESIAN_POINT('Ctrl Pts',(-6.182769484,3.703213228,-4.25590953));
#119997=CARTESIAN_POINT('Ctrl Pts',(-6.342361029,3.75,-4.003055905));
#119998=CARTESIAN_POINT('Ctrl Pts',(-6.402628134,3.76766825,-3.907569919));
#119999=CARTESIAN_POINT('Ctrl Pts',(-6.45999344200001,3.785449891,-3.810312944));
#120000=CARTESIAN_POINT('Ctrl Pts',(-5.65780526618243,3.65572482783619,
-4.53340264902825));
#120001=CARTESIAN_POINT('Ctrl Pts',(-5.75083422362151,3.68016831608079,
-4.41730007290052));
#120002=CARTESIAN_POINT('Ctrl Pts',(-5.84007784835361,3.70444733035584,
-4.29859130048564));
#120003=CARTESIAN_POINT('Ctrl Pts',(-5.92534487833161,3.72849594483852,
-4.17765341767066));
#120004=CARTESIAN_POINT('Ctrl Pts',(-5.95083479653685,3.73568509187778,
-4.14149997428622));
#120005=CARTESIAN_POINT('Ctrl Pts',(-5.97596966945381,3.74285367421748,
-4.10514745230995));
#120006=CARTESIAN_POINT('Ctrl Pts',(-6.00074523716432,3.75000000004653,
-4.06860622376149));
#120007=CARTESIAN_POINT('Ctrl Pts',(-6.04062686442943,3.76150355502397,
-4.00978522352873));
#120008=CARTESIAN_POINT('Ctrl Pts',(-6.07970954977572,3.77306479253944,
-3.95028019920642));
#120009=CARTESIAN_POINT('Ctrl Pts',(-6.11796000811214,3.78467661228328,
-3.89012408023804));
#120010=CARTESIAN_POINT('Ctrl Pts',(-5.135372207,3.785444214,-5.117660823));
#120011=CARTESIAN_POINT('Ctrl Pts',(-5.41240231700001,3.720864611,-4.839671956));
#120012=CARTESIAN_POINT('Ctrl Pts',(-5.657805263,3.655724827,-4.533402653));
#120013=CARTESIAN_POINT('Ctrl Pts',(-5.135973089,3.785444214,-5.46550825000001));
#120014=CARTESIAN_POINT('Ctrl Pts',(-5.431832937,3.720864611,-5.187486857));
#120015=CARTESIAN_POINT('Ctrl Pts',(-5.695952078,3.655724827,-4.879152583));
#120016=CARTESIAN_POINT('',(-5.13866381757032,3.78467661250474,-5.11435569747235));
#120017=CARTESIAN_POINT('Origin',(0.157549562756596,3.62501420442123,0.119658603587385));
#120018=CARTESIAN_POINT('Ctrl Pts',(-5.31450463650428,3.74576903856886,
-5.29207336192223));
#120019=CARTESIAN_POINT('Ctrl Pts',(-5.29435543258093,3.75001846751486,
-5.27163913767389));
#120020=CARTESIAN_POINT('Ctrl Pts',(-5.27422044602485,3.75433282934707,
-5.25120424192238));
#120021=CARTESIAN_POINT('Ctrl Pts',(-5.25406857613353,3.75872286882774,
-5.23080239827387));
#120022=CARTESIAN_POINT('Ctrl Pts',(-5.23485185760006,3.76290918769074,
-5.21134730606298));
#120023=CARTESIAN_POINT('Ctrl Pts',(-5.21562671092685,3.76716275954088,
-5.19191486568245));
#120024=CARTESIAN_POINT('Ctrl Pts',(-5.1963929890299,3.77148708939095,-5.17250682437492));
#120025=CARTESIAN_POINT('Ctrl Pts',(-5.17715870205999,3.77581154628672,
-5.15309821287304));
#120026=CARTESIAN_POINT('Ctrl Pts',(-5.15791569665113,3.78020679565695,
-5.13371385587399));
#120027=CARTESIAN_POINT('Ctrl Pts',(-5.13866381689417,3.78467661259413,
-5.11435569730711));
#120028=CARTESIAN_POINT('Ctrl Pts',(-4.550981356,3.655724827,-5.643675106));
#120029=CARTESIAN_POINT('Ctrl Pts',(-4.77598017,3.703213228,-5.462239182));
#120030=CARTESIAN_POINT('Ctrl Pts',(-4.985821077,3.75,-5.263467316));
#120031=CARTESIAN_POINT('Ctrl Pts',(-5.065064022,3.76766825,-5.188404412));
#120032=CARTESIAN_POINT('Ctrl Pts',(-5.14201138,3.785449891,-5.110990019));
#120033=CARTESIAN_POINT('Ctrl Pts',(-4.896848283,3.655724827,-5.680746157));
#120034=CARTESIAN_POINT('Ctrl Pts',(-5.123325024,3.703213228,-5.485521408));
#120035=CARTESIAN_POINT('Ctrl Pts',(-5.333541463,3.75,-5.272886825));
#120036=CARTESIAN_POINT('Ctrl Pts',(-5.41292622100001,3.76766825,-5.192588894));
#120037=CARTESIAN_POINT('Ctrl Pts',(-5.489857734,3.785449891,-5.109937579));
#120038=CARTESIAN_POINT('Ctrl Pts',(-4.55098135996182,3.65572482783619,
-5.64367510280524));
#120039=CARTESIAN_POINT('Ctrl Pts',(-4.66679394937079,3.68016831085496,
-5.55028543631377));
#120040=CARTESIAN_POINT('Ctrl Pts',(-4.77946996131795,3.7044473199498,-5.45353677174798));
#120041=CARTESIAN_POINT('Ctrl Pts',(-4.88874154317296,3.7284959293042,-5.35375626322254));
#120042=CARTESIAN_POINT('Ctrl Pts',(-4.9214074667792,3.7356850815309,-5.32392762513062));
#120043=CARTESIAN_POINT('Ctrl Pts',(-4.95376944141401,3.74285366902422,
-5.29382823817083));
#120044=CARTESIAN_POINT('Ctrl Pts',(-4.98582107706216,3.74999999996854,
-5.26346731613916));
#120045=CARTESIAN_POINT('Ctrl Pts',(-5.03741507037547,3.76150355490328,
-5.21459489019404));
#120046=CARTESIAN_POINT('Ctrl Pts',(-5.08837584583837,3.77306479260976,
-5.16488268167932));
#120047=CARTESIAN_POINT('Ctrl Pts',(-5.13866381694153,3.78467661224474,
-5.11435569717934));
#120048=CARTESIAN_POINT('Ctrl Pts',(-3.915164259,3.785444214,-6.101965981));
#120049=CARTESIAN_POINT('Ctrl Pts',(-4.245476948,3.720864611,-5.89002962400001));
#120050=CARTESIAN_POINT('Ctrl Pts',(-4.550981356,3.655724827,-5.643675106));
#120051=CARTESIAN_POINT('Ctrl Pts',(-3.840974177,3.785444214,-6.4418101));
#120052=CARTESIAN_POINT('Ctrl Pts',(-4.189683368,3.720864611,-6.233889815));
#120053=CARTESIAN_POINT('Ctrl Pts',(-4.513910305,3.655724827,-5.989542033));
#120054=CARTESIAN_POINT('',(-3.91908941653677,3.78467661230451,-6.09944572553291));
#120055=CARTESIAN_POINT('Origin',(0.128142893896167,3.62501424720021,0.150729317702604));
#120056=CARTESIAN_POINT('Ctrl Pts',(-4.05261513068026,3.74576903858172,
-6.31080902862542));
#120057=CARTESIAN_POINT('Ctrl Pts',(-4.03732975837536,3.75001846748708,
-6.2865210619541));
#120058=CARTESIAN_POINT('Ctrl Pts',(-4.02205841514173,3.75433282933544,
-6.26223549580967));
#120059=CARTESIAN_POINT('Ctrl Pts',(-4.00676347813404,3.758722868824,-6.23797857957129));
#120060=CARTESIAN_POINT('Ctrl Pts',(-3.99217830559993,3.76290918769149,
-6.21484731016465));
#120061=CARTESIAN_POINT('Ctrl Pts',(-3.9775800325423,3.7671627595409,-6.19173635117419));
#120062=CARTESIAN_POINT('Ctrl Pts',(-3.96296813980594,3.77148708935365,
-6.16864737757532));
#120063=CARTESIAN_POINT('Ctrl Pts',(-3.94835581754222,3.77581154628328,
-6.14555772525904));
#120064=CARTESIAN_POINT('Ctrl Pts',(-3.93372976681854,3.78020679564855,
-6.12248988635496));
#120065=CARTESIAN_POINT('Ctrl Pts',(-3.91908941594345,3.78467661291491,
-6.0994457254675));
#120066=CARTESIAN_POINT('Ctrl Pts',(-3.231358619,3.655724827,-6.490055583));
#120067=CARTESIAN_POINT('Ctrl Pts',(-3.490100446,3.703213228,-6.361229625));
#120068=CARTESIAN_POINT('Ctrl Pts',(-3.737765465,3.75,-6.212214527));
#120069=CARTESIAN_POINT('Ctrl Pts',(-3.831292059,3.76766825,-6.155941442));
#120070=CARTESIAN_POINT('Ctrl Pts',(-3.923082237,3.785449891,-6.096878362));
#120071=CARTESIAN_POINT('Ctrl Pts',(-3.561170189,3.655724827,-6.600611099));
#120072=CARTESIAN_POINT('Ctrl Pts',(-3.82431958,3.703213228,-6.458636401));
#120073=CARTESIAN_POINT('Ctrl Pts',(-4.075331425,3.75,-6.296163417));
#120074=CARTESIAN_POINT('Ctrl Pts',(-4.170121894,3.76766825,-6.23480818400001));
#120075=CARTESIAN_POINT('Ctrl Pts',(-4.26302238,3.785449891,-6.170627212));
#120076=CARTESIAN_POINT('Ctrl Pts',(-3.23135862351649,3.65572482782894,
-6.49005558075127));
#120077=CARTESIAN_POINT('Ctrl Pts',(-3.36453956354981,3.68016830479105,
-6.42374561295059));
#120078=CARTESIAN_POINT('Ctrl Pts',(-3.49537934446265,3.70444730795221,
-6.35348090887989));
#120079=CARTESIAN_POINT('Ctrl Pts',(-3.62354604724397,3.72849591153848,
-6.27952339325455));
#120080=CARTESIAN_POINT('Ctrl Pts',(-3.66186056706451,3.73568506971114,
-6.25741432251455));
#120081=CARTESIAN_POINT('Ctrl Pts',(-3.6999364466945,3.7428536631213,-6.2349754922436));
#120082=CARTESIAN_POINT('Ctrl Pts',(-3.73776546478839,3.74999999994898,
-6.21221452717703));
#120083=CARTESIAN_POINT('Ctrl Pts',(-3.79865934571585,3.76150355489174,
-6.17557589430039));
#120084=CARTESIAN_POINT('Ctrl Pts',(-3.85911534157287,3.77306479252643,
-6.1379809899611));
#120085=CARTESIAN_POINT('Ctrl Pts',(-3.91908941579481,3.78467661229662,
-6.09944572494293));
#120086=CARTESIAN_POINT('Ctrl Pts',(-2.511887581,3.785444214,-6.800949991));
#120087=CARTESIAN_POINT('Ctrl Pts',(-2.880037795,3.720864611,-6.664976053));
#120088=CARTESIAN_POINT('Ctrl Pts',(-3.231358619,3.655724827,-6.490055583));
#120089=CARTESIAN_POINT('Ctrl Pts',(-2.366375582,3.785444214,-7.11690007));
#120090=CARTESIAN_POINT('Ctrl Pts',(-2.751628862,3.720864611,-6.988803013));
#120091=CARTESIAN_POINT('Ctrl Pts',(-3.120803103,3.655724827,-6.819867154));
#120092=CARTESIAN_POINT('',(-2.51626275117737,3.78467661244294,-6.79933245108693));
#120093=CARTESIAN_POINT('Origin',(0.0927445870603161,3.62501424977788,0.174752169069451));
#120094=CARTESIAN_POINT('Ctrl Pts',(-2.60122984628958,3.74576903855236,
-7.03445827945423));
#120095=CARTESIAN_POINT('Ctrl Pts',(-2.59152303216242,3.75001846749456,
-7.00745224865496));
#120096=CARTESIAN_POINT('Ctrl Pts',(-2.58182940328144,3.7543328293346,-6.98045157812523));
#120097=CARTESIAN_POINT('Ctrl Pts',(-2.57210657331077,3.75872286882143,
-6.95347381572861));
#120098=CARTESIAN_POINT('Ctrl Pts',(-2.56283493314422,3.76290918767733,
-6.92774796161051));
#120099=CARTESIAN_POINT('Ctrl Pts',(-2.55354613256455,3.76716275952044,
-6.90203912684389));
#120100=CARTESIAN_POINT('Ctrl Pts',(-2.5442393045101,3.77148708932044,-6.87634883570633));
#120101=CARTESIAN_POINT('Ctrl Pts',(-2.53493220283023,3.77581154625792,
-6.85065778926127));
#120102=CARTESIAN_POINT('Ctrl Pts',(-2.52560700440847,3.78020679562409,
-6.82498509510151));
#120103=CARTESIAN_POINT('Ctrl Pts',(-2.51626275052791,3.78467661289218,
-6.79933245031635));
#120104=CARTESIAN_POINT('Ctrl Pts',(-1.760641144,3.655724827,-7.032968275));
#120105=CARTESIAN_POINT('Ctrl Pts',(-2.041027504,3.703213228,-6.96277604));
#120106=CARTESIAN_POINT('Ctrl Pts',(-2.314936093,3.75,-6.870485491));
#120107=CARTESIAN_POINT('Ctrl Pts',(-2.418373138,3.76766825,-6.835633493));
#120108=CARTESIAN_POINT('Ctrl Pts',(-2.520714129,3.785449891,-6.79768345));
#120109=CARTESIAN_POINT('Ctrl Pts',(-2.058975735,3.655724827,-7.211838803));
#120110=CARTESIAN_POINT('Ctrl Pts',(-2.346493203,3.703213228,-7.129752735));
#120111=CARTESIAN_POINT('Ctrl Pts',(-2.62656342,3.75,-7.025038406));
#120112=CARTESIAN_POINT('Ctrl Pts',(-2.732327301,3.76766825,-6.98549477199999));
#120113=CARTESIAN_POINT('Ctrl Pts',(-2.836852838,3.785449891,-6.94278517400001));
#120114=CARTESIAN_POINT('Ctrl Pts',(-1.76064114857457,3.65572482777479,
-7.03296827385479));
#120115=CARTESIAN_POINT('Ctrl Pts',(-1.90496309768958,3.6801683085245,-6.99683855557638));
#120116=CARTESIAN_POINT('Ctrl Pts',(-2.04784877368294,3.70444731544377,
-6.95634327951747));
#120117=CARTESIAN_POINT('Ctrl Pts',(-2.18891771140563,3.72849592276323,
-6.91166689384207));
#120118=CARTESIAN_POINT('Ctrl Pts',(-2.23108923368116,3.73568507719821,
-6.89831121665249));
#120119=CARTESIAN_POINT('Ctrl Pts',(-2.27309858376271,3.74285366689624,
-6.88458218934028));
#120120=CARTESIAN_POINT('Ctrl Pts',(-2.31493609343746,3.75000000004083,
-6.8704854910179));
#120121=CARTESIAN_POINT('Ctrl Pts',(-2.3822825332196,3.76150355503787,-6.84779383358611));
#120122=CARTESIAN_POINT('Ctrl Pts',(-2.44940689466729,3.77306479265215,
-6.82407412937982));
#120123=CARTESIAN_POINT('Ctrl Pts',(-2.51626275101608,3.78467661239246,
-6.79933245062732));
#120124=CARTESIAN_POINT('Ctrl Pts',(-0.991157832000001,3.785444214,-7.181929139));
#120125=CARTESIAN_POINT('Ctrl Pts',(-1.379931276,3.720864611,-7.12827561));
#120126=CARTESIAN_POINT('Ctrl Pts',(-1.760641144,3.655724827,-7.032968275));
#120127=CARTESIAN_POINT('Ctrl Pts',(-0.781127895000001,3.785444214,-7.459211702));
#120128=CARTESIAN_POINT('Ctrl Pts',(-1.184911248,3.720864611,-7.41692755));
#120129=CARTESIAN_POINT('Ctrl Pts',(-1.581770616,3.655724827,-7.331302866));
#120130=CARTESIAN_POINT('',(-0.995778437273178,3.78467661247787,-7.18128994900401));
#120131=CARTESIAN_POINT('Origin',(0.0530096971896153,3.62501423314348,0.190603709598965));
#120132=CARTESIAN_POINT('Ctrl Pts',(-1.02821394493559,3.74576903859535,
-7.42918407887292));
#120133=CARTESIAN_POINT('Ctrl Pts',(-1.02453956940242,3.7500184674844,-7.40072275602811));
#120134=CARTESIAN_POINT('Ctrl Pts',(-1.02087691824179,3.75433282933031,
-7.37226950252932));
#120135=CARTESIAN_POINT('Ctrl Pts',(-1.01718082414336,3.75872286881798,
-7.34383234421332));
#120136=CARTESIAN_POINT('Ctrl Pts',(-1.01365624800282,3.76290918767842,
-7.31671481770127));
#120137=CARTESIAN_POINT('Ctrl Pts',(-1.01011125400241,3.76716275952209,
-7.28961022365669));
#120138=CARTESIAN_POINT('Ctrl Pts',(-1.00654466763215,3.77148708935972,
-7.26251986408723));
#120139=CARTESIAN_POINT('Ctrl Pts',(-1.00297797646616,3.77581154625761,
-7.23542870853134));
#120140=CARTESIAN_POINT('Ctrl Pts',(-0.999389666409323,3.78020679562356,
-7.20835158568946));
#120141=CARTESIAN_POINT('Ctrl Pts',(-0.995778436939607,3.78467661259395,
-7.18128994843103));
#120142=CARTESIAN_POINT('Ctrl Pts',(-0.207598047,3.655724827,-7.247027187));
#120143=CARTESIAN_POINT('Ctrl Pts',(-0.496518385,3.703213228,-7.238750787));
#120144=CARTESIAN_POINT('Ctrl Pts',(-0.783862884,3.75,-7.207500189));
#120145=CARTESIAN_POINT('Ctrl Pts',(-0.892373777000001,3.76766825,-7.19569891800001));
#120146=CARTESIAN_POINT('Ctrl Pts',(-1.00048023,3.785449891,-7.18063641400001));
#120147=CARTESIAN_POINT('Ctrl Pts',(-0.460505865,3.655724827,-7.48584894));
#120148=CARTESIAN_POINT('Ctrl Pts',(-0.758947412,3.703213228,-7.467489755));
#120149=CARTESIAN_POINT('Ctrl Pts',(-1.054980228,3.75,-7.425430406));
#120150=CARTESIAN_POINT('Ctrl Pts',(-1.166772121,3.76766825,-7.409547389));
#120151=CARTESIAN_POINT('Ctrl Pts',(-1.27803521,3.785449891,-7.390306218));
#120152=CARTESIAN_POINT('Ctrl Pts',(-0.207598052087366,3.65572482783619,
-7.24702718685427));
#120153=CARTESIAN_POINT('Ctrl Pts',(-0.356312633948643,3.68016830504614,
-7.2427671150157));
#120154=CARTESIAN_POINT('Ctrl Pts',(-0.504562987970137,3.70444730845298,
-7.23393479450269));
#120155=CARTESIAN_POINT('Ctrl Pts',(-0.651937893342154,3.72849591226242,
-7.2206285727237));
#120156=CARTESIAN_POINT('Ctrl Pts',(-0.695994566083915,3.73568507018081,
-7.21665077299676));
#120157=CARTESIAN_POINT('Ctrl Pts',(-0.73997311729786,3.74285366333655,
-7.21227348925494));
#120158=CARTESIAN_POINT('Ctrl Pts',(-0.783862883953297,3.74999999990936,
-7.20750018947045));
#120159=CARTESIAN_POINT('Ctrl Pts',(-0.854512836360514,3.76150355485184,
-7.19981654407829));
#120160=CARTESIAN_POINT('Ctrl Pts',(-0.92516690338793,3.77306479249498,
-7.19108114729756));
#120161=CARTESIAN_POINT('Ctrl Pts',(-0.995778437045702,3.78467661227579,
-7.18128994836432));
#120162=CARTESIAN_POINT('Ctrl Pts',(0.575917356,3.785444214,-7.227089262));
#120163=CARTESIAN_POINT('Ctrl Pts',(0.184699296,3.720864611,-7.258264921));
#120164=CARTESIAN_POINT('Ctrl Pts',(-0.207598047,3.655724827,-7.247027187));
#120165=CARTESIAN_POINT('Ctrl Pts',(0.840644464,3.785444214,-7.452738885));
#120166=CARTESIAN_POINT('Ctrl Pts',(0.437211499,3.720864611,-7.498244798));
#120167=CARTESIAN_POINT('Ctrl Pts',(0.031223706,3.655724827,-7.499935005));
#120168=CARTESIAN_POINT('',(0.571267371189336,3.78467661250746,-7.22745830975374));
#120169=CARTESIAN_POINT('Origin',(0.0107961935969751,3.62501419796389,0.197543322221929));
#120170=CARTESIAN_POINT('Ctrl Pts',(0.592880097666729,3.74576903859534,
-7.47652948817413));
#120171=CARTESIAN_POINT('Ctrl Pts',(0.590350225508585,3.75001846753542,
-7.44794369301283));
#120172=CARTESIAN_POINT('Ctrl Pts',(0.587810637439167,3.75433282936884,
-7.4193682990325));
#120173=CARTESIAN_POINT('Ctrl Pts',(0.585307170438767,3.75872286884618,
-7.39080143468898));
#120174=CARTESIAN_POINT('Ctrl Pts',(0.582919877304075,3.76290918770063,
-7.36356022115747));
#120175=CARTESIAN_POINT('Ctrl Pts',(0.580555304784233,3.7671627595402,-7.336327248497));
#120176=CARTESIAN_POINT('Ctrl Pts',(0.578214879801036,3.77148708937742,
-7.30910353575974));
#120177=CARTESIAN_POINT('Ctrl Pts',(0.575874386056288,3.77581154626321,
-7.28187902319138));
#120178=CARTESIAN_POINT('Ctrl Pts',(0.573558022377638,3.78020679562105,
-7.2546635678004));
#120179=CARTESIAN_POINT('Ctrl Pts',(0.571267371386615,3.7846766125698,-7.22745830916289));
#120180=CARTESIAN_POINT('Ctrl Pts',(1.355152105,3.655724827,-7.122223162));
#120181=CARTESIAN_POINT('Ctrl Pts',(1.071207382,3.703213228,-7.176249592));
#120182=CARTESIAN_POINT('Ctrl Pts',(0.783862884,3.75,-7.207500189));
#120183=CARTESIAN_POINT('Ctrl Pts',(0.67535199,3.76766825,-7.21930146));
#120184=CARTESIAN_POINT('Ctrl Pts',(0.566535013,3.785449891,-7.22783080000001));
#120185=CARTESIAN_POINT('Ctrl Pts',(1.159496749,3.655724827,-7.4098291));
#120186=CARTESIAN_POINT('Ctrl Pts',(0.864085917,3.703213228,-7.456055254));
#120187=CARTESIAN_POINT('Ctrl Pts',(0.565932667,3.75,-7.478617534));
#120188=CARTESIAN_POINT('Ctrl Pts',(0.453340027,3.76766825,-7.487137805));
#120189=CARTESIAN_POINT('Ctrl Pts',(0.340541924,3.785449891,-7.492264758));
#120190=CARTESIAN_POINT('Ctrl Pts',(1.3551521000723,3.65572482782414,-7.1222231629376));
#120191=CARTESIAN_POINT('Ctrl Pts',(1.20899854655521,3.68016831274631,-7.15003193717776));
#120192=CARTESIAN_POINT('Ctrl Pts',(1.06231546936486,3.70444732374593,-7.17327556105714));
#120193=CARTESIAN_POINT('Ctrl Pts',(0.915525617098543,3.72849593500173,
-7.19196168252318));
#120194=CARTESIAN_POINT('Ctrl Pts',(0.871643901735247,3.73568508532593,
-7.19754775711046));
#120195=CARTESIAN_POINT('Ctrl Pts',(0.827752604260194,3.7428536709306,-7.20272689443133));
#120196=CARTESIAN_POINT('Ctrl Pts',(0.78386288387654,3.75000000000168,-7.20750018914185));
#120197=CARTESIAN_POINT('Ctrl Pts',(0.71321293074891,3.76150355496809,-7.21518383469371));
#120198=CARTESIAN_POINT('Ctrl Pts',(0.642332865126122,3.77306479247657,
-7.22184120228829));
#120199=CARTESIAN_POINT('Ctrl Pts',(0.571267371253685,3.78467661219437,
-7.2274583091124));
#120200=CARTESIAN_POINT('Ctrl Pts',(2.116063288,3.785444214,-6.93431872400001));
#120201=CARTESIAN_POINT('Ctrl Pts',(1.740693535,3.720864611,-7.048865831));
#120202=CARTESIAN_POINT('Ctrl Pts',(1.355152105,3.655724827,-7.122223162));
#120203=CARTESIAN_POINT('Ctrl Pts',(2.423109222,3.785444214,-7.097784281));
#120204=CARTESIAN_POINT('Ctrl Pts',(2.038890722,3.720864611,-7.228952453));
#120205=CARTESIAN_POINT('Ctrl Pts',(1.642758043,3.655724827,-7.31787851900001));
#120206=CARTESIAN_POINT('',(2.11160135187181,3.78467661255684,-6.93567875264863));
#120207=CARTESIAN_POINT('Origin',(-0.0319222393415766,3.62501423866122,
0.195245911636008));
#120208=CARTESIAN_POINT('Ctrl Pts',(2.18625172552362,3.74576903864184,-7.17428068773664));
#120209=CARTESIAN_POINT('Ctrl Pts',(2.17763589926571,3.75001846753479,-7.14690706044628));
#120210=CARTESIAN_POINT('Ctrl Pts',(2.16901282041789,3.75433282937659,-7.11954567964758));
#120211=CARTESIAN_POINT('Ctrl Pts',(2.16042685174653,3.75872286886273,-7.09218486411846));
#120212=CARTESIAN_POINT('Ctrl Pts',(2.15223931659581,3.76290918772571,-7.06609373247429));
#120213=CARTESIAN_POINT('Ctrl Pts',(2.14407574238575,3.76716275957337,-7.04000576478655));
#120214=CARTESIAN_POINT('Ctrl Pts',(2.13593774173399,3.7714870894253,-7.01392164950441));
#120215=CARTESIAN_POINT('Ctrl Pts',(2.12779950200521,3.77581154631678,-6.98783676792682));
#120216=CARTESIAN_POINT('Ctrl Pts',(2.11968677518882,3.78020679568715,-6.96175554450415));
#120217=CARTESIAN_POINT('Ctrl Pts',(2.11160135209104,3.78467661264949,-6.93567875210078));
#120218=CARTESIAN_POINT('Ctrl Pts',(2.85453685,3.655724827,-6.664391898));
#120219=CARTESIAN_POINT('Ctrl Pts',(2.588844683,3.703213228,-6.778194942));
#120220=CARTESIAN_POINT('Ctrl Pts',(2.314936093,3.75,-6.870485491));
#120221=CARTESIAN_POINT('Ctrl Pts',(2.211499049,3.76766825,-6.905337489));
#120222=CARTESIAN_POINT('Ctrl Pts',(2.107059708,3.785449891,-6.937059852));
#120223=CARTESIAN_POINT('Ctrl Pts',(2.725282582,3.655724827,-6.987333887));
#120224=CARTESIAN_POINT('Ctrl Pts',(2.446715548,3.703213228,-7.095983895));
#120225=CARTESIAN_POINT('Ctrl Pts',(2.160383179,3.75,-7.182112817));
#120226=CARTESIAN_POINT('Ctrl Pts',(2.052254499,3.76766825,-7.21463797899999));
#120227=CARTESIAN_POINT('Ctrl Pts',(1.943195696,3.785449891,-7.243893324));
#120228=CARTESIAN_POINT('Ctrl Pts',(2.85453684561659,3.65572482778347,-6.66439189987753));
#120229=CARTESIAN_POINT('Ctrl Pts',(2.71777836705026,3.68016830890369,-6.72296920496374));
#120230=CARTESIAN_POINT('Ctrl Pts',(2.57952137248556,3.70444731614839,-6.77720192375549));
#120231=CARTESIAN_POINT('Ctrl Pts',(2.44018037091755,3.72849592370944,-6.82700664690812));
#120232=CARTESIAN_POINT('Ctrl Pts',(2.39852540482211,3.73568507780856,-6.84189540205534));
#120233=CARTESIAN_POINT('Ctrl Pts',(2.35677360102747,3.7428536671656,-6.85638879336383));
#120234=CARTESIAN_POINT('Ctrl Pts',(2.31493609318094,3.74999999996342,-6.87048549099486));
#120235=CARTESIAN_POINT('Ctrl Pts',(2.24758965425263,3.76150355491197,-6.89317714831988));
#120236=CARTESIAN_POINT('Ctrl Pts',(2.17979786166445,3.77306479259842,-6.91491598961235));
#120237=CARTESIAN_POINT('Ctrl Pts',(2.11160135195229,3.78467661222486,-6.93567875207102));
#120238=CARTESIAN_POINT('Ctrl Pts',(3.557264453,3.785444214,-6.317307149));
#120239=CARTESIAN_POINT('Ctrl Pts',(3.215294878,3.720864611,-6.50986961));
#120240=CARTESIAN_POINT('Ctrl Pts',(2.85453685,3.655724827,-6.664391898));
#120241=CARTESIAN_POINT('Ctrl Pts',(3.892272087,3.785444214,-6.410945172));
#120242=CARTESIAN_POINT('Ctrl Pts',(3.545233681,3.720864611,-6.621642326));
#120243=CARTESIAN_POINT('Ctrl Pts',(3.177478839,3.655724827,-6.79364616600001));
#120244=CARTESIAN_POINT('',(3.5531991999166,3.78467661247843,-6.31959456523331));
#120245=CARTESIAN_POINT('Origin',(-0.0731479704522126,3.62501422279194,
0.183818735359169));
#120246=CARTESIAN_POINT('Ctrl Pts',(3.67739665301007,3.74576903856647,-6.53657049633276));
#120247=CARTESIAN_POINT('Ctrl Pts',(3.66309773951716,3.7500184675244,-6.51168899697415));
#120248=CARTESIAN_POINT('Ctrl Pts',(3.64879437539399,3.75433282937531,-6.48682101708142));
#120249=CARTESIAN_POINT('Ctrl Pts',(3.63452737529612,3.75872286886363,-6.46194561166964));
#120250=CARTESIAN_POINT('Ctrl Pts',(3.620922438067,3.76290918772969,-6.43822455420455));
#120251=CARTESIAN_POINT('Ctrl Pts',(3.6073415817108,3.76716275957753,-6.41450143583751));
#120252=CARTESIAN_POINT('Ctrl Pts',(3.59378652917745,3.77148708941549,-6.39077658231892));
#120253=CARTESIAN_POINT('Ctrl Pts',(3.58023107836183,3.77581154631337,-6.36705103170317));
#120254=CARTESIAN_POINT('Ctrl Pts',(3.56670133038181,3.78020679567546,-6.34332356926532));
#120255=CARTESIAN_POINT('Ctrl Pts',(3.55319919983689,3.78467661264265,-6.31959456457597));
#120256=CARTESIAN_POINT('Ctrl Pts',(4.220446625,3.655724827,-5.894941076));
#120257=CARTESIAN_POINT('Ctrl Pts',(3.985430483,3.703213228,-6.06319943));
#120258=CARTESIAN_POINT('Ctrl Pts',(3.737765465,3.75,-6.212214527));
#120259=CARTESIAN_POINT('Ctrl Pts',(3.64423887,3.76766825,-6.268487612));
#120260=CARTESIAN_POINT('Ctrl Pts',(3.549060633,3.785449891,-6.321919694));
#120261=CARTESIAN_POINT('Ctrl Pts',(4.163637232,3.655724827,-6.238118707));
#120262=CARTESIAN_POINT('Ctrl Pts',(3.91493948,3.703213228,-6.404112217));
#120263=CARTESIAN_POINT('Ctrl Pts',(3.653816575,3.75,-6.549780488));
#120264=CARTESIAN_POINT('Ctrl Pts',(3.555207832,3.76766825,-6.60478969900001));
#120265=CARTESIAN_POINT('Ctrl Pts',(3.454987798,3.785449891,-6.656805489));
#120266=CARTESIAN_POINT('Ctrl Pts',(4.22044662086179,3.65572482783619,-5.89494107896272));
#120267=CARTESIAN_POINT('Ctrl Pts',(4.09947783216379,3.68016831624432,-5.98154793527608));
#120268=CARTESIAN_POINT('Ctrl Pts',(3.97611160334085,3.70444733067044,-6.06423391356302));
#120269=CARTESIAN_POINT('Ctrl Pts',(3.85073482196067,3.7284959452959,-6.14282844728115));
#120270=CARTESIAN_POINT('Ctrl Pts',(3.81325440525329,3.7356850921816,-6.16632367376766));
#120271=CARTESIAN_POINT('Ctrl Pts',(3.77559442370857,3.74285367436812,-6.18945359777217));
#120272=CARTESIAN_POINT('Ctrl Pts',(3.73776546476096,3.75000000004461,-6.21221452715368));
#120273=CARTESIAN_POINT('Ctrl Pts',(3.67687158297574,3.76150355501617,-6.24885316009497));
#120274=CARTESIAN_POINT('Ctrl Pts',(3.61533793358737,3.77306479254825,-6.28465699023988));
#120275=CARTESIAN_POINT('Ctrl Pts',(3.55319919971644,3.78467661230877,-6.31959456458162));
#120276=CARTESIAN_POINT('Ctrl Pts',(4.83213188600001,3.785444214,-5.404905313));
#120277=CARTESIAN_POINT('Ctrl Pts',(4.539552606,3.720864611,-5.66647912100001));
#120278=CARTESIAN_POINT('Ctrl Pts',(4.220446625,3.655724827,-5.894941076));
#120279=CARTESIAN_POINT('Ctrl Pts',(5.179436634,3.785444214,-5.424337393));
#120280=CARTESIAN_POINT('Ctrl Pts',(4.885805454,3.720864611,-5.704711563));
#120281=CARTESIAN_POINT('Ctrl Pts',(4.563624257,3.655724827,-5.951750469));
#120282=CARTESIAN_POINT('',(4.82865340266755,3.78467661231159,-5.40801315903628));
#120283=CARTESIAN_POINT('Origin',(-0.110953360283951,3.62501423096888,0.163796429963448));
#120284=CARTESIAN_POINT('Ctrl Pts',(4.99659059962423,3.74576903861156,-5.5932175331691));
#120285=CARTESIAN_POINT('Ctrl Pts',(4.97727719960564,3.75001846750351,-5.57199159346776));
#120286=CARTESIAN_POINT('Ctrl Pts',(4.95796235959718,3.75433282936886,-5.55077981355134));
#120287=CARTESIAN_POINT('Ctrl Pts',(4.93868143718509,3.75872286886735,-5.52955296453581));
#120288=CARTESIAN_POINT('Ctrl Pts',(4.92029524972338,3.76290918773003,-5.50931115157272));
#120289=CARTESIAN_POINT('Ctrl Pts',(4.90193213712422,3.76716275957218,-5.48906214921159));
#120290=CARTESIAN_POINT('Ctrl Pts',(4.88359385225733,3.77148708938566,-5.46880590528075));
#120291=CARTESIAN_POINT('Ctrl Pts',(4.86525502831547,3.77581154631779,-5.44854906589434));
#120292=CARTESIAN_POINT('Ctrl Pts',(4.84694089549697,3.78020679569389,-5.4282848341132));
#120293=CARTESIAN_POINT('Ctrl Pts',(4.82865340282906,3.78467661285823,-5.4080131584029));
#120294=CARTESIAN_POINT('Ctrl Pts',(5.389013006,3.655724827,-4.84984936));
#120295=CARTESIAN_POINT('Ctrl Pts',(5.195661984,3.703213228,-5.06469545100001));
#120296=CARTESIAN_POINT('Ctrl Pts',(4.985821077,3.75,-5.263467316));
#120297=CARTESIAN_POINT('Ctrl Pts',(4.906578131,3.76766825,-5.338530221));
#120298=CARTESIAN_POINT('Ctrl Pts',(4.825111428,3.785449891,-5.411173598));
#120299=CARTESIAN_POINT('Ctrl Pts',(5.407304832,3.655724827,-5.19721603));
#120300=CARTESIAN_POINT('Ctrl Pts',(5.200105193,3.703213228,-5.412791369));
#120301=CARTESIAN_POINT('Ctrl Pts',(4.976401568,3.75,-5.611187702));
#120302=CARTESIAN_POINT('Ctrl Pts',(4.891923597,3.76766825,-5.686108794));
#120303=CARTESIAN_POINT('Ctrl Pts',(4.805228509,3.785449891,-5.75845282800001));
#120304=CARTESIAN_POINT('Ctrl Pts',(5.38901300259543,3.65572482783619,-4.84984936378305));
#120305=CARTESIAN_POINT('Ctrl Pts',(5.2894903402649,3.68016830914952,-4.96043608174435));
#120306=CARTESIAN_POINT('Ctrl Pts',(5.18678341734772,3.70444731657778,-5.06770897050535));
#120307=CARTESIAN_POINT('Ctrl Pts',(5.08123340919572,3.72849592434171,-5.17141828174666));
#120308=CARTESIAN_POINT('Ctrl Pts',(5.04968001283305,3.73568507824166,-5.20242141534551));
#120309=CARTESIAN_POINT('Ctrl Pts',(5.01787272000543,3.74285366740273,-5.23310638753778));
#120310=CARTESIAN_POINT('Ctrl Pts',(4.98582107694877,3.75000000000868,-5.26346731649106));
#120311=CARTESIAN_POINT('Ctrl Pts',(4.93422708289128,3.76150355498014,-5.31233974326661));
#120312=CARTESIAN_POINT('Ctrl Pts',(4.88182882144562,3.77306479250486,-5.36053441520924));
#120313=CARTESIAN_POINT('Ctrl Pts',(4.82865340234207,3.78467661251199,-5.40801315826926));
#120314=CARTESIAN_POINT('Ctrl Pts',(5.881054202,3.785444214,-4.239776111));
#120315=CARTESIAN_POINT('Ctrl Pts',(5.6515459,3.720864611,-4.558130366));
#120316=CARTESIAN_POINT('Ctrl Pts',(5.389013006,3.655724827,-4.84984936));
#120317=CARTESIAN_POINT('Ctrl Pts',(6.224416481,3.785444214,-4.184093626));
#120318=CARTESIAN_POINT('Ctrl Pts',(5.997922393,3.720864611,-4.521034827));
#120319=CARTESIAN_POINT('Ctrl Pts',(5.736379676,3.655724827,-4.831557535));
#120320=CARTESIAN_POINT('',(5.87832514029295,3.7846766124525,-4.24355907006547));
#120321=CARTESIAN_POINT('Origin',(-0.143570501109366,3.62501422270825,0.136115116627182));
#120322=CARTESIAN_POINT('Ctrl Pts',(6.08214952361695,3.74576903857924,-4.38833193459805));
#120323=CARTESIAN_POINT('Ctrl Pts',(6.05872471075178,3.75001846754309,-4.37175405532135));
#120324=CARTESIAN_POINT('Ctrl Pts',(6.03530153526747,3.75433282939705,-4.35519031474441));
#120325=CARTESIAN_POINT('Ctrl Pts',(6.01190824498433,3.75872286888058,-4.33860456609077));
#120326=CARTESIAN_POINT('Ctrl Pts',(5.98960052494431,3.76290918771721,-4.32278848237012));
#120327=CARTESIAN_POINT('Ctrl Pts',(5.96731379477278,3.76716275953038,-4.30696041691506));
#120328=CARTESIAN_POINT('Ctrl Pts',(5.94504975494914,3.77148708934424,-4.29111994183739));
#120329=CARTESIAN_POINT('Ctrl Pts',(5.92278506103885,3.77581154620093,-4.2752790013885));
#120330=CARTESIAN_POINT('Ctrl Pts',(5.90054289164115,3.78020679553293,-4.25942553337721));
#120331=CARTESIAN_POINT('Ctrl Pts',(5.87832513993511,3.78467661242694,-4.24355906945344));
#120332=CARTESIAN_POINT('Ctrl Pts',(6.305595129,3.655724827,-3.577984079));
#120333=CARTESIAN_POINT('Ctrl Pts',(6.162950104,3.703213228,-3.829371942));
#120334=CARTESIAN_POINT('Ctrl Pts',(6.000745237,3.75,-4.068606224));
#120335=CARTESIAN_POINT('Ctrl Pts',(5.939491253,3.76766825,-4.158949091));
#120336=CARTESIAN_POINT('Ctrl Pts',(5.875545374,3.785449891,-4.247407039));
#120337=CARTESIAN_POINT('Ctrl Pts',(6.398132867,3.655724827,-3.913297307));
#120338=CARTESIAN_POINT('Ctrl Pts',(6.242119767,3.703213228,-4.168374412));
#120339=CARTESIAN_POINT('Ctrl Pts',(6.066295556,3.75,-4.410222016));
#120340=CARTESIAN_POINT('Ctrl Pts',(5.99989845300001,3.76766825,-4.501551761));
#120341=CARTESIAN_POINT('Ctrl Pts',(5.930782076,3.785449891,-4.590841313));
#120342=CARTESIAN_POINT('Ctrl Pts',(6.30559512632834,3.65572482788943,-3.57798408370835));
#120343=CARTESIAN_POINT('Ctrl Pts',(6.23217209691088,3.68016831800515,-3.70737982273348));
#120344=CARTESIAN_POINT('Ctrl Pts',(6.15492687539684,3.70444733414286,-3.83422372830123));
#120345=CARTESIAN_POINT('Ctrl Pts',(6.07413897226622,3.72849595049746,-3.95819854833682));
#120346=CARTESIAN_POINT('Ctrl Pts',(6.04998806253253,3.73568509565773,-3.99525984801047));
#120347=CARTESIAN_POINT('Ctrl Pts',(6.0255207977836,3.74285367613321,-4.03206500559797));
#120348=CARTESIAN_POINT('Ctrl Pts',(6.00074523661453,3.75000000011495,-4.06860622465582));
#120349=CARTESIAN_POINT('Ctrl Pts',(5.9608636085474,3.76150355512892,-4.12742722500174));
#120350=CARTESIAN_POINT('Ctrl Pts',(5.92005081953396,3.77306479251279,-4.18575920929946));
#120351=CARTESIAN_POINT('Ctrl Pts',(5.87832513980401,3.78467661209925,-4.2435590695447));
#120352=CARTESIAN_POINT('Ctrl Pts',(6.65498496000001,3.785444214,-2.876399691));
#120353=CARTESIAN_POINT('Ctrl Pts',(6.499279189,3.720864611,-3.236648501));
#120354=CARTESIAN_POINT('Ctrl Pts',(6.305595129,3.655724827,-3.577984079));
#120355=CARTESIAN_POINT('Ctrl Pts',(6.978349531,3.785444214,-2.748206291));
#120356=CARTESIAN_POINT('Ctrl Pts',(6.829583148,3.720864611,-3.125959528));
#120357=CARTESIAN_POINT('Ctrl Pts',(6.640908357,3.655724827,-3.485446341));
#120358=CARTESIAN_POINT('',(6.65313292495336,3.78467661232429,-2.88068087308594));
#120359=CARTESIAN_POINT('Origin',(-0.169474684097664,3.62501422942962,0.102069408652304));
#120360=CARTESIAN_POINT('Ctrl Pts',(6.8833138953662,3.74576903858391,-2.97825281206827));
#120361=CARTESIAN_POINT('Ctrl Pts',(6.85687298764022,3.75001846751913,-2.96709815684438));
#120362=CARTESIAN_POINT('Ctrl Pts',(6.83043671842893,3.75433282937008,-2.95595695765276));
#120363=CARTESIAN_POINT('Ctrl Pts',(6.80402490463526,3.75872286884989,-2.9447878404987));
#120364=CARTESIAN_POINT('Ctrl Pts',(6.7788387361469,3.76290918770224,-2.93413702837705));
#120365=CARTESIAN_POINT('Ctrl Pts',(6.75367049107894,3.76716275953069,-2.92347000246075));
#120366=CARTESIAN_POINT('Ctrl Pts',(6.72852173843565,3.77148708931287,-2.9127859794265));
#120367=CARTESIAN_POINT('Ctrl Pts',(6.70337224640891,3.77581154623209,-2.90210164227767));
#120368=CARTESIAN_POINT('Ctrl Pts',(6.67824205949415,3.78020679557677,-2.89140022848748));
#120369=CARTESIAN_POINT('Ctrl Pts',(6.65313292455553,3.78467661284088,-2.88068087237092));
#120370=CARTESIAN_POINT('Ctrl Pts',(6.927334631,3.655724827,-2.138816239));
#120371=CARTESIAN_POINT('Ctrl Pts',(6.842065528,3.703213228,-2.414991257));
#120372=CARTESIAN_POINT('Ctrl Pts',(6.735081219,3.75,-2.683501626));
#120373=CARTESIAN_POINT('Ctrl Pts',(6.69468036500001,3.76766825,-2.784900123));
#120374=CARTESIAN_POINT('Ctrl Pts',(6.651245349,3.785449891,-2.885036447));
#120375=CARTESIAN_POINT('Ctrl Pts',(7.089791321,3.655724827,-2.446397152));
#120376=CARTESIAN_POINT('Ctrl Pts',(6.992259758,3.703213228,-2.7290489));
#120377=CARTESIAN_POINT('Ctrl Pts',(6.872536305,3.75,-3.00303925));
#120378=CARTESIAN_POINT('Ctrl Pts',(6.827324725,3.76766825,-3.106507171));
#120379=CARTESIAN_POINT('Ctrl Pts',(6.779018865,3.785449891,-3.208567161));
#120380=CARTESIAN_POINT('Ctrl Pts',(6.92733462964675,3.65572482775366,-2.138816243383));
#120381=CARTESIAN_POINT('Ctrl Pts',(6.88344445138572,3.68016831674824,-2.28097055623012));
#120382=CARTESIAN_POINT('Ctrl Pts',(6.83527287313895,3.70444733170435,-2.42145435399876));
#120383=CARTESIAN_POINT('Ctrl Pts',(6.78302467103386,3.72849594680057,-2.55989771550699));
#120384=CARTESIAN_POINT('Ctrl Pts',(6.76740547750231,3.73568509318686,-2.60128428134912));
#120385=CARTESIAN_POINT('Ctrl Pts',(6.75142226205709,3.74285367487235,-2.64248870044474));
#120386=CARTESIAN_POINT('Ctrl Pts',(6.73508121889342,3.75000000004661,-2.68350162626749));
#120387=CARTESIAN_POINT('Ctrl Pts',(6.70877677764511,3.76150355499729,-2.74952079523594));
#120388=CARTESIAN_POINT('Ctrl Pts',(6.68145782078675,3.77306479247725,-2.81526255334838));
#120389=CARTESIAN_POINT('Ctrl Pts',(6.65313292417658,3.7846766123365,-2.88068087229939));
#120390=CARTESIAN_POINT('Ctrl Pts',(7.117736018,3.785444214,-1.378526018));
#120391=CARTESIAN_POINT('Ctrl Pts',(7.043113406,3.720864611,-1.763824549));
#120392=CARTESIAN_POINT('Ctrl Pts',(6.927334631,3.655724827,-2.138816239));
#120393=CARTESIAN_POINT('Ctrl Pts',(7.405982713,3.785444214,-1.183815884));
#120394=CARTESIAN_POINT('Ctrl Pts',(7.341900185,3.720864611,-1.584717836));
#120395=CARTESIAN_POINT('Ctrl Pts',(7.234915544,3.655724827,-1.976359549));
#120396=CARTESIAN_POINT('',(7.11684761125436,3.78467661242663,-1.38310524218956));
#120397=CARTESIAN_POINT('Origin',(-0.187454685946141,3.62501420012553,0.0632511407711575));
#120398=CARTESIAN_POINT('Ctrl Pts',(7.3626221596976,3.74576903850582,-1.42891389841415));
#120399=CARTESIAN_POINT('Ctrl Pts',(7.33440150456421,3.75001846745712,-1.42370404627908));
#120400=CARTESIAN_POINT('Ctrl Pts',(7.30618827216532,3.75433282931056,-1.41850633850769));
#120401=CARTESIAN_POINT('Ctrl Pts',(7.27799292189132,3.75872286879844,-1.41327610827669));
#120402=CARTESIAN_POINT('Ctrl Pts',(7.25110598229676,3.76290918765531,-1.40828858789053));
#120403=CARTESIAN_POINT('Ctrl Pts',(7.22423306159013,3.76716275949081,-1.4032813797772));
#120404=CARTESIAN_POINT('Ctrl Pts',(7.19737552341408,3.77148708932007,-1.39825338164923));
#120405=CARTESIAN_POINT('Ctrl Pts',(7.17051719618115,3.77581154619532,-1.39322523580198));
#120406=CARTESIAN_POINT('Ctrl Pts',(7.14367405144934,3.78020679553876,-1.38817626253347));
#120407=CARTESIAN_POINT('Ctrl Pts',(7.1168476107115,3.78467661246488,-1.38310524176854));
#120408=CARTESIAN_POINT('Ctrl Pts',(7.225159666,3.655724827,-0.599639729));
#120409=CARTESIAN_POINT('Ctrl Pts',(7.201253572,3.703213228,-0.887688265));
#120410=CARTESIAN_POINT('Ctrl Pts',(7.154492288,3.75,-1.172919475));
#120411=CARTESIAN_POINT('Ctrl Pts',(7.136833664,3.76766825,-1.28063232));
#120412=CARTESIAN_POINT('Ctrl Pts',(7.11594048400001,3.785449891,-1.387764758));
#120413=CARTESIAN_POINT('Ctrl Pts',(7.449939012,3.655724827,-0.865106183999999));
#120414=CARTESIAN_POINT('Ctrl Pts',(7.41544945400001,3.703213228,-1.162116095));
#120415=CARTESIAN_POINT('Ctrl Pts',(7.357424895,3.75,-1.455437707));
#120416=CARTESIAN_POINT('Ctrl Pts',(7.335512881,3.76766825,-1.566205758));
#120417=CARTESIAN_POINT('Ctrl Pts',(7.310276266,3.785449891,-1.676263974));
#120418=CARTESIAN_POINT('Ctrl Pts',(7.22515966557906,3.65572482783619,-0.599639734072013));
#120419=CARTESIAN_POINT('Ctrl Pts',(7.2128545925476,3.68016831230712,-0.74790562150211));
#120420=CARTESIAN_POINT('Ctrl Pts',(7.19600910650006,3.70444732281126,-0.895460424408708));
#120421=CARTESIAN_POINT('Ctrl Pts',(7.17474367395376,3.72849593352359,-1.04189884946702));
#120422=CARTESIAN_POINT('Ctrl Pts',(7.16838653326402,3.73568508433717,-1.08567551229546));
#120423=CARTESIAN_POINT('Ctrl Pts',(7.16163472464087,3.7428536704232,-1.12935254070576));
#120424=CARTESIAN_POINT('Ctrl Pts',(7.15449228824709,3.74999999996714,-1.17291947509793));
#120425=CARTESIAN_POINT('Ctrl Pts',(7.14299500075388,3.76150355489508,-1.24304982931552));
#120426=CARTESIAN_POINT('Ctrl Pts',(7.13044728075292,3.7730647925216,-1.31312735085109));
#120427=CARTESIAN_POINT('Ctrl Pts',(7.11684761062354,3.78467661208736,-1.38310524190111));
#120428=CARTESIAN_POINT('Ctrl Pts',(7.24766965,3.785444214,0.183805999));
#120429=CARTESIAN_POINT('Ctrl Pts',(7.257619468,3.720864611,-0.208526122));
#120430=CARTESIAN_POINT('Ctrl Pts',(7.225159666,3.655724827,-0.599639729));
#120431=CARTESIAN_POINT('Ctrl Pts',(7.487320375,3.785444214,0.435928437));
#120432=CARTESIAN_POINT('Ctrl Pts',(7.510918129,3.720864611,0.030623501));
#120433=CARTESIAN_POINT('Ctrl Pts',(7.490626122,3.655724827,-0.374860382));
#120434=CARTESIAN_POINT('',(7.24778641184,3.78467661246146,0.179142853532766));
#120435=CARTESIAN_POINT('Origin',(-0.196669441527031,3.62501419190378,0.0214751493333531));
#120436=CARTESIAN_POINT('Ctrl Pts',(7.49766239486428,3.74576903859026,0.187239441344393));
#120437=CARTESIAN_POINT('Ctrl Pts',(7.46898155867307,3.75001846754567,0.186260883320056));
#120438=CARTESIAN_POINT('Ctrl Pts',(7.44031058236322,3.75433282937421,0.185272060355488));
#120439=CARTESIAN_POINT('Ctrl Pts',(7.41165007873406,3.75872286885703,0.184318843757048));
#120440=CARTESIAN_POINT('Ctrl Pts',(7.38431957143929,3.76290918769016,0.18340986136322));
#120441=CARTESIAN_POINT('Ctrl Pts',(7.35699852299701,3.76716275951432,0.182523120145202));
#120442=CARTESIAN_POINT('Ctrl Pts',(7.32968802821128,3.77148708934581,0.18165998977544));
#120443=CARTESIAN_POINT('Ctrl Pts',(7.30237673105925,3.77581154622358,0.180796834047416));
#120444=CARTESIAN_POINT('Ctrl Pts',(7.27507578416942,3.78020679558335,0.179957282699222));
#120445=CARTESIAN_POINT('Ctrl Pts',(7.24778641118233,3.78467661245961,0.179142853867999));
#120446=CARTESIAN_POINT('Ctrl Pts',(7.185144264,3.655724827,0.967575269));
#120447=CARTESIAN_POINT('Ctrl Pts',(7.223719002,3.703213228,0.681122044));
#120448=CARTESIAN_POINT('Ctrl Pts',(7.23936725,3.75,0.392507087));
#120449=CARTESIAN_POINT('Ctrl Pts',(7.245276552,3.76766825,0.283516426));
#120450=CARTESIAN_POINT('Ctrl Pts',(7.247902151,3.785449891,0.17439727));
#120451=CARTESIAN_POINT('Ctrl Pts',(7.461735836,3.655724827,0.756636186000001));
#120452=CARTESIAN_POINT('Ctrl Pts',(7.491900975,3.703213228,0.459155966));
#120453=CARTESIAN_POINT('Ctrl Pts',(7.498288474,3.75,0.160218487));
#120454=CARTESIAN_POINT('Ctrl Pts',(7.500700607,3.76766825,0.047329695));
#120455=CARTESIAN_POINT('Ctrl Pts',(7.49971327400001,3.785449891,-0.065580547));
#120456=CARTESIAN_POINT('Ctrl Pts',(7.18514426467923,3.65572482783619,0.967575263956075));
#120457=CARTESIAN_POINT('Ctrl Pts',(7.20499965519742,3.68016830563138,0.820130563806539));
#120458=CARTESIAN_POINT('Ctrl Pts',(7.220267925519,3.70444730961,0.672404268532776));
#120459=CARTESIAN_POINT('Ctrl Pts',(7.23097959932907,3.72849591398212,0.524818092604028));
#120460=CARTESIAN_POINT('Ctrl Pts',(7.23418177719071,3.7356850713341,0.480698266550486));
#120461=CARTESIAN_POINT('Ctrl Pts',(7.23697709503498,3.74285366392681,0.436590903575513));
#120462=CARTESIAN_POINT('Ctrl Pts',(7.23936725006134,3.7499999999406,0.392507087293556));
#120463=CARTESIAN_POINT('Ctrl Pts',(7.24321471544561,3.76150355488793,0.321544764621282));
#120464=CARTESIAN_POINT('Ctrl Pts',(7.24602495025561,3.77306479248825,0.250408227808213));
#120465=CARTESIAN_POINT('Ctrl Pts',(7.24778641115059,3.78467661224106,0.179142853732049));
#120466=CARTESIAN_POINT('Ctrl Pts',(7.038710305,3.785444214,1.737543452));
#120467=CARTESIAN_POINT('Ctrl Pts',(7.132767311,3.720864611,1.356522755));
#120468=CARTESIAN_POINT('Ctrl Pts',(7.18514426400001,3.655724827,0.967575269));
#120469=CARTESIAN_POINT('Ctrl Pts',(7.21855925700001,3.785444214,2.03528923));
#120470=CARTESIAN_POINT('Ctrl Pts',(7.32873389,3.720864611,1.644532917));
#120471=CARTESIAN_POINT('Ctrl Pts',(7.396083347,3.655724827,1.24416684));
#120472=CARTESIAN_POINT('',(7.03982677465566,3.78467661254277,1.73301442877743));
#120473=CARTESIAN_POINT('Origin',(-0.196687510874572,3.6250142158557,-0.0213049642278113));
#120474=CARTESIAN_POINT('Ctrl Pts',(7.2821202695864,3.7457690385624,1.7946376730135));
#120475=CARTESIAN_POINT('Ctrl Pts',(7.25432033648699,3.7500184675284,1.78751646127483));
#120476=CARTESIAN_POINT('Ctrl Pts',(7.22653223946043,3.75433282935617,1.78038734412676));
#120477=CARTESIAN_POINT('Ctrl Pts',(7.19874671596483,3.75872286883388,1.7732952521629));
#120478=CARTESIAN_POINT('Ctrl Pts',(7.17225058499085,3.76290918769164,1.76653227008039));
#120479=CARTESIAN_POINT('Ctrl Pts',(7.14575891054067,3.76716275953878,1.75979304253155));
#120480=CARTESIAN_POINT('Ctrl Pts',(7.11927246741103,3.77148708938777,1.75307914252952));
#120481=CARTESIAN_POINT('Ctrl Pts',(7.09278524606327,3.77581154629315,1.74636504526135));
#120482=CARTESIAN_POINT('Ctrl Pts',(7.06630305878795,3.7802067956747,1.73967622549821));
#120483=CARTESIAN_POINT('Ctrl Pts',(7.03982677401824,3.78467661262501,1.73301442899937));
#120484=CARTESIAN_POINT('Ctrl Pts',(6.809159503,3.655724827,2.489547522));
#120485=CARTESIAN_POINT('Ctrl Pts',(6.908411361,3.703213228,2.218083843));
#120486=CARTESIAN_POINT('Ctrl Pts',(6.985737446,3.75,1.939580454));
#120487=CARTESIAN_POINT('Ctrl Pts',(7.014938362,3.76766825,1.83440826));
#120488=CARTESIAN_POINT('Ctrl Pts',(7.040959969,3.785449891,1.728404675));
#120489=CARTESIAN_POINT('Ctrl Pts',(7.124630184,3.655724827,2.34299909));
#120490=CARTESIAN_POINT('Ctrl Pts',(7.218039533,3.703213228,2.058958406));
#120491=CARTESIAN_POINT('Ctrl Pts',(7.288540418,3.75,1.768383042));
#120492=CARTESIAN_POINT('Ctrl Pts',(7.31516391,3.76766825,1.658652065));
#120493=CARTESIAN_POINT('Ctrl Pts',(7.338472024,3.785449891,1.548169354));
#120494=CARTESIAN_POINT('Ctrl Pts',(6.80915950467478,3.65572482780133,2.4895475174193));
#120495=CARTESIAN_POINT('Ctrl Pts',(6.86024694711263,3.68016830932062,2.34981829336983));
#120496=CARTESIAN_POINT('Ctrl Pts',(6.90691504685433,3.70444731696092,2.20882796211418));
#120497=CARTESIAN_POINT('Ctrl Pts',(6.94910295791911,3.72849592491557,2.06699494043432));
#120498=CARTESIAN_POINT('Ctrl Pts',(6.9617147222808,3.7356850786114,2.02459500635401));
#120499=CARTESIAN_POINT('Ctrl Pts',(6.97392645999889,3.74285366756795,1.9821197811675));
#120500=CARTESIAN_POINT('Ctrl Pts',(6.98573744594791,3.74999999996848,1.93958045418761));
#120501=CARTESIAN_POINT('Ctrl Pts',(7.00474976135324,3.76150355491264,1.87110428296099));
#120502=CARTESIAN_POINT('Ctrl Pts',(7.0227865466034,3.77306479262606,1.80223499602672));
#120503=CARTESIAN_POINT('Ctrl Pts',(7.03982677400277,3.78467661236402,1.73301442888571));
#120504=CARTESIAN_POINT('Ctrl Pts',(6.500628688,3.785444214,3.210035304));
#120505=CARTESIAN_POINT('Ctrl Pts',(6.674394881,3.720864611,2.858142135));
#120506=CARTESIAN_POINT('Ctrl Pts',(6.809159503,3.655724827,2.489547522));
#120507=CARTESIAN_POINT('Ctrl Pts',(6.61226633200001,3.785444214,3.53948216));
#120508=CARTESIAN_POINT('Ctrl Pts',(6.803866199,3.720864611,3.181545802));
#120509=CARTESIAN_POINT('Ctrl Pts',(6.955707935,3.655724827,2.805018204));
#120510=CARTESIAN_POINT('',(6.50269266208612,3.78467661244381,3.20585217509439));
#120511=CARTESIAN_POINT('Origin',(-0.187509038755996,3.62501423310757,-0.063088837505566));
#120512=CARTESIAN_POINT('Ctrl Pts',(6.72607429382293,3.74576903860098,3.31812064141916));
#120513=CARTESIAN_POINT('Ctrl Pts',(6.70045515785978,3.75001846751968,3.30518975552696));
#120514=CARTESIAN_POINT('Ctrl Pts',(6.67484928050536,3.75433282935375,3.29225369376685));
#120515=CARTESIAN_POINT('Ctrl Pts',(6.64923795717537,3.75872286883744,3.27935434482528));
#120516=CARTESIAN_POINT('Ctrl Pts',(6.62481513221521,3.76290918769716,3.26705359264465));
#120517=CARTESIAN_POINT('Ctrl Pts',(6.60039155305013,3.76716275954495,3.25477699767267));
#120518=CARTESIAN_POINT('Ctrl Pts',(6.57596763822924,3.77148708938579,3.24252626267529));
#120519=CARTESIAN_POINT('Ctrl Pts',(6.55154300579018,3.77581154628315,3.23027516772947));
#120520=CARTESIAN_POINT('Ctrl Pts',(6.52711785581645,3.78020679564801,3.21804984148404));
#120521=CARTESIAN_POINT('Ctrl Pts',(6.5026926613042,3.78467661251154,3.2058521752322));
#120522=CARTESIAN_POINT('Ctrl Pts',(6.114786011,3.655724827,3.895111301));
#120523=CARTESIAN_POINT('Ctrl Pts',(6.270074082,3.703213228,3.651330506));
#120524=CARTESIAN_POINT('Ctrl Pts',(6.405462322,3.75,3.395961195));
#120525=CARTESIAN_POINT('Ctrl Pts',(6.45658945,3.76766825,3.299525202));
#120526=CARTESIAN_POINT('Ctrl Pts',(6.504790324,3.785449891,3.201593798));
#120527=CARTESIAN_POINT('Ctrl Pts',(6.454384744,3.655724827,3.819805961));
#120528=CARTESIAN_POINT('Ctrl Pts',(6.606670585,3.703213228,3.562486238));
#120529=CARTESIAN_POINT('Ctrl Pts',(6.737988312,3.75,3.293859971));
#120530=CARTESIAN_POINT('Ctrl Pts',(6.787578278,3.76766825,3.192417707));
#120531=CARTESIAN_POINT('Ctrl Pts',(6.834091979,3.785449891,3.089528577));
#120532=CARTESIAN_POINT('Ctrl Pts',(6.11478601373434,3.65572482783619,3.89511129670746));
#120533=CARTESIAN_POINT('Ctrl Pts',(6.19471672344615,3.68016831260846,3.76963113674948));
#120534=CARTESIAN_POINT('Ctrl Pts',(6.27060251193692,3.70444732345577,3.64196932547167));
#120535=CARTESIAN_POINT('Ctrl Pts',(6.34229400865791,3.72849593454659,3.51252141730028));
#120536=CARTESIAN_POINT('Ctrl Pts',(6.3637256395827,3.73568508501387,3.47382394383685));
#120537=CARTESIAN_POINT('Ctrl Pts',(6.38478278197638,3.74285367075939,3.43496694581494));
#120538=CARTESIAN_POINT('Ctrl Pts',(6.40546232230385,3.74999999996872,3.39596119504962));
#120539=CARTESIAN_POINT('Ctrl Pts',(6.43875049341836,3.76150355492492,3.33317304420941));
#120540=CARTESIAN_POINT('Ctrl Pts',(6.47117044971429,3.77306479256857,3.26979125879157));
#120541=CARTESIAN_POINT('Ctrl Pts',(6.5026926613336,3.78467661235723,3.20585217511677));
#120542=CARTESIAN_POINT('Ctrl Pts',(5.6585849,3.785444214,4.532429474));
#120543=CARTESIAN_POINT('Ctrl Pts',(5.903935165,3.720864611,4.226117966));
#120544=CARTESIAN_POINT('Ctrl Pts',(6.114786011,3.655724827,3.895111301));
#120545=CARTESIAN_POINT('Ctrl Pts',(5.696791181,3.785444214,4.878172838));
#120546=CARTESIAN_POINT('Ctrl Pts',(5.960857287,3.720864611,4.56979314100001));
#120547=CARTESIAN_POINT('Ctrl Pts',(6.190091351,3.655724827,4.234710034));
#120548=CARTESIAN_POINT('',(5.66149986688143,3.78467661242999,4.52878783667046));
#120549=CARTESIAN_POINT('Origin',(-0.169563074774411,3.62501420262947,-0.101922854223928));
#120550=CARTESIAN_POINT('Ctrl Pts',(5.85552455969347,3.74576903856604,4.68645197658526));
#120551=CARTESIAN_POINT('Ctrl Pts',(5.8332841429803,3.75001846752245,4.66831605084936));
#120552=CARTESIAN_POINT('Ctrl Pts',(5.81105778769237,3.75433282936489,4.65017792033751));
#120553=CARTESIAN_POINT('Ctrl Pts',(5.78881822167272,3.75872286883866,4.63207447348692));
#120554=CARTESIAN_POINT('Ctrl Pts',(5.76761068695466,3.76290918769358,4.61481112053925));
#120555=CARTESIAN_POINT('Ctrl Pts',(5.74639722263548,3.7671627595273,4.59757119782373));
#120556=CARTESIAN_POINT('Ctrl Pts',(5.72517787158082,3.77148708931804,4.58035645850533));
#120557=CARTESIAN_POINT('Ctrl Pts',(5.70395789665028,3.77581154624956,4.56314121305174));
#120558=CARTESIAN_POINT('Ctrl Pts',(5.68273187698867,3.78020679560976,4.54595102275112));
#120559=CARTESIAN_POINT('Ctrl Pts',(5.66149986605684,3.78467661289658,4.52878783714528));
#120560=CARTESIAN_POINT('Ctrl Pts',(5.134491921,3.655724827,5.118544003));
#120561=CARTESIAN_POINT('Ctrl Pts',(5.338555108,3.703213228,4.913845014));
#120562=CARTESIAN_POINT('Ctrl Pts',(5.5256749,3.75,4.693550565));
#120563=CARTESIAN_POINT('Ctrl Pts',(5.596337592,3.76766825,4.610360012));
#120564=CARTESIAN_POINT('Ctrl Pts',(5.664463913,3.785449891,4.525079953));
#120565=CARTESIAN_POINT('Ctrl Pts',(5.482339447,3.655724827,5.11800295));
#120566=CARTESIAN_POINT('Ctrl Pts',(5.686381063,3.703213228,4.899436174));
#120567=CARTESIAN_POINT('Ctrl Pts',(5.872375362,3.75,4.665319669));
#120568=CARTESIAN_POINT('Ctrl Pts',(5.94261303000001,3.76766825,4.57690944600001));
#120569=CARTESIAN_POINT('Ctrl Pts',(6.010157388,3.785449891,4.486424876));
#120570=CARTESIAN_POINT('Ctrl Pts',(5.1344919245932,3.65572482783619,5.11854399939561));
#120571=CARTESIAN_POINT('Ctrl Pts',(5.23952844189472,3.68016831678484,5.01318021847078));
#120572=CARTESIAN_POINT('Ctrl Pts',(5.34108359530637,3.70444733171498,4.90481625233483));
#120573=CARTESIAN_POINT('Ctrl Pts',(5.43892647385379,3.7284959468036,4.79380629735723));
#120574=CARTESIAN_POINT('Ctrl Pts',(5.46817584118771,3.73568509318852,4.76062073496305));
#120575=CARTESIAN_POINT('Ctrl Pts',(5.4970937687556,3.74285367487428,4.72719887388563));
#120576=CARTESIAN_POINT('Ctrl Pts',(5.52567490020155,3.7500000000504,4.69355056476271));
#120577=CARTESIAN_POINT('Ctrl Pts',(5.57168240855751,3.76150355498939,4.63938633814908));
#120578=CARTESIAN_POINT('Ctrl Pts',(5.61696961380205,3.77306479247568,4.58445571633938));
#120579=CARTESIAN_POINT('Ctrl Pts',(5.66149986636746,3.78467661236143,4.52878783624501));
#120580=CARTESIAN_POINT('Ctrl Pts',(4.55195197,3.785444214,5.642892278));
#120581=CARTESIAN_POINT('Ctrl Pts',(4.857414002,3.720864611,5.39648521799999));
#120582=CARTESIAN_POINT('Ctrl Pts',(5.134491921,3.655724827,5.118544003));
#120583=CARTESIAN_POINT('Ctrl Pts',(4.514940407,3.785444214,5.988765576));
#120584=CARTESIAN_POINT('Ctrl Pts',(4.839125312,3.720864611,5.744362032));
#120585=CARTESIAN_POINT('Ctrl Pts',(5.135032975,3.655724827,5.466391529));
#120586=CARTESIAN_POINT('',(4.55558163233989,3.78467661243338,5.63996241300083));
#120587=CARTESIAN_POINT('Origin',(-0.143688241515189,3.62501423950758,-0.135990833085079));
#120588=CARTESIAN_POINT('Ctrl Pts',(4.7111770047759,3.7457690385862,5.83565002581625));
#120589=CARTESIAN_POINT('Ctrl Pts',(4.69335524483929,3.75001846749632,5.81315707568708));
#120590=CARTESIAN_POINT('Ctrl Pts',(4.6755476913489,3.75433282933081,5.7906649951772));
#120591=CARTESIAN_POINT('Ctrl Pts',(4.65771977994644,3.75872286880854,5.76820394759314));
#120592=CARTESIAN_POINT('Ctrl Pts',(4.64071917619361,3.76290918766191,5.74678520923227));
#120593=CARTESIAN_POINT('Ctrl Pts',(4.62370774462027,3.7671627594984,5.72538807866446));
#120594=CARTESIAN_POINT('Ctrl Pts',(4.60668515011344,3.77148708932264,5.70401427703497));
#120595=CARTESIAN_POINT('Ctrl Pts',(4.58966205543604,3.77581154620756,5.68263984738451));
#120596=CARTESIAN_POINT('Ctrl Pts',(4.57262767108181,3.78020679555432,5.66128858746507));
#120597=CARTESIAN_POINT('Ctrl Pts',(4.5555816317836,3.78467661248386,5.6399624126005));
#120598=CARTESIAN_POINT('Ctrl Pts',(3.914114695,3.655724827,6.102639278));
#120599=CARTESIAN_POINT('Ctrl Pts',(4.157411231,3.703213228,5.94659359));
#120600=CARTESIAN_POINT('Ctrl Pts',(4.38751306,3.75,5.771674726));
#120601=CARTESIAN_POINT('Ctrl Pts',(4.474407207,3.76766825,5.705619513));
#120602=CARTESIAN_POINT('Ctrl Pts',(4.559273465,3.785449891,5.636978399));
#120603=CARTESIAN_POINT('Ctrl Pts',(4.25394605,3.655724827,6.176887809));
#120604=CARTESIAN_POINT('Ctrl Pts',(4.500202683,3.703213228,6.007293919));
#120605=CARTESIAN_POINT('Ctrl Pts',(4.732176666,3.75,5.818634204));
#120606=CARTESIAN_POINT('Ctrl Pts',(4.819777801,3.76766825,5.747389985));
#120607=CARTESIAN_POINT('Ctrl Pts',(4.905194518,3.785449891,5.67354093500001));
#120608=CARTESIAN_POINT('Ctrl Pts',(3.91411469962435,3.65572482790262,6.10263927503403));
#120609=CARTESIAN_POINT('Ctrl Pts',(4.03934556802192,3.68016830661403,6.02231862036379));
#120610=CARTESIAN_POINT('Ctrl Pts',(4.16182141836033,3.7044473115228,5.93831953563007));
#120611=CARTESIAN_POINT('Ctrl Pts',(4.28124059665187,3.7284959168111,5.85093829710996));
#120612=CARTESIAN_POINT('Ctrl Pts',(4.31694009517294,3.73568507320295,5.82481630866601));
#120613=CARTESIAN_POINT('Ctrl Pts',(4.35236669927942,3.74285366484134,5.79839229546968));
#120614=CARTESIAN_POINT('Ctrl Pts',(4.38751306021334,3.7499999999068,5.77167472643996));
#120615=CARTESIAN_POINT('Ctrl Pts',(4.44408864624166,3.76150355484585,5.7286670844108));
#120616=CARTESIAN_POINT('Ctrl Pts',(4.50012552270294,3.77306479247613,5.68475612009858));
#120617=CARTESIAN_POINT('Ctrl Pts',(4.55558163185474,3.78467661218761,5.63996241248155));
#120618=CARTESIAN_POINT('Ctrl Pts',(3.232474826,3.785444214,6.489499711));
#120619=CARTESIAN_POINT('Ctrl Pts',(3.583765559,3.720864611,6.31451881899999));
#120620=CARTESIAN_POINT('Ctrl Pts',(3.914114695,3.655724827,6.102639278));
#120621=CARTESIAN_POINT('Ctrl Pts',(3.121976037,3.785444214,6.81933029100001));
#120622=CARTESIAN_POINT('Ctrl Pts',(3.491121217,3.720864611,6.650330939));
#120623=CARTESIAN_POINT('Ctrl Pts',(3.839866164,3.655724827,6.442470632));
#120624=CARTESIAN_POINT('',(3.23664946277011,3.78467661248022,6.48741861533793));
#120625=CARTESIAN_POINT('Origin',(-0.111094888332385,3.6250142351479,-0.163700176824847));
#120626=CARTESIAN_POINT('Ctrl Pts',(3.34654004953935,3.74576903858902,6.71197956579666));
#120627=CARTESIAN_POINT('Ctrl Pts',(3.33397027170812,3.75001846752048,6.68618133683447));
#120628=CARTESIAN_POINT('Ctrl Pts',(3.32141418136731,3.75433282935661,6.66038701106181));
#120629=CARTESIAN_POINT('Ctrl Pts',(3.30883153794991,3.75872286883258,6.63461861631273));
#120630=CARTESIAN_POINT('Ctrl Pts',(3.29683279451946,3.76290918768263,6.61004600887627));
#120631=CARTESIAN_POINT('Ctrl Pts',(3.28481883139786,3.76716275951602,6.58549217638448));
#120632=CARTESIAN_POINT('Ctrl Pts',(3.2727889512392,3.77148708935664,6.560958727682));
#120633=CARTESIAN_POINT('Ctrl Pts',(3.26075871765674,3.77581154624101,6.53642455821551));
#120634=CARTESIAN_POINT('Ctrl Pts',(3.24871247748031,3.78020679560717,6.51191058980696));
#120635=CARTESIAN_POINT('Ctrl Pts',(3.2366494621999,3.78467661255436,6.48741861492866));
#120636=CARTESIAN_POINT('Ctrl Pts',(2.510717817,3.655724827,6.801381922));
#120637=CARTESIAN_POINT('Ctrl Pts',(2.781871425,3.703213228,6.70128605900001));
#120638=CARTESIAN_POINT('Ctrl Pts',(3.044195986,3.75,6.579921793));
#120639=CARTESIAN_POINT('Ctrl Pts',(3.143258515,3.76766825,6.534090586));
#120640=CARTESIAN_POINT('Ctrl Pts',(3.240896457,3.785449891,6.485298001));
#120641=CARTESIAN_POINT('Ctrl Pts',(2.826642864,3.655724827,6.94694826000001));
#120642=CARTESIAN_POINT('Ctrl Pts',(3.103599827,3.703213228,6.834257277));
#120643=CARTESIAN_POINT('Ctrl Pts',(3.370706649,3.75,6.699875871));
#120644=CARTESIAN_POINT('Ctrl Pts',(3.47157512,3.76766825,6.649128957));
#120645=CARTESIAN_POINT('Ctrl Pts',(3.570870203,3.785449891,6.59536852600001));
#120646=CARTESIAN_POINT('Ctrl Pts',(2.51071782177452,3.65572482783619,6.80138192023749));
#120647=CARTESIAN_POINT('Ctrl Pts',(2.65028748540186,3.68016831654245,6.74986003173072));
#120648=CARTESIAN_POINT('Ctrl Pts',(2.78795729369265,3.70444733127152,6.69415346213049));
#120649=CARTESIAN_POINT('Ctrl Pts',(2.92336895432209,3.72849594620015,6.63448671431067));
#120650=CARTESIAN_POINT('Ctrl Pts',(2.96384921821405,3.73568509279227,6.61664980361853));
#120651=CARTESIAN_POINT('Ctrl Pts',(3.00412789473792,3.74285367468743,6.59845926607656));
#120652=CARTESIAN_POINT('Ctrl Pts',(3.04419598642018,3.75000000007494,6.57992179280561));
#120653=CARTESIAN_POINT('Ctrl Pts',(3.10869423890095,3.76150355506134,6.55008172319584));
#120654=CARTESIAN_POINT('Ctrl Pts',(3.17286056324773,3.77306479246515,6.51924364565036));
#120655=CARTESIAN_POINT('Ctrl Pts',(3.23664946229233,3.78467661220444,6.48741861481928));
#120656=CARTESIAN_POINT('Ctrl Pts',(1.761850751,3.785444214,7.03266535));
#120657=CARTESIAN_POINT('Ctrl Pts',(2.142544221,3.720864611,6.937292538));
#120658=CARTESIAN_POINT('Ctrl Pts',(2.510717817,3.655724827,6.801381922));
#120659=CARTESIAN_POINT('Ctrl Pts',(1.583031538,3.785444214,7.331030702));
#120660=CARTESIAN_POINT('Ctrl Pts',(1.979876174,3.720864611,7.245337762));
#120661=CARTESIAN_POINT('Ctrl Pts',(2.365151479,3.655724827,7.11730696800001));
#120662=CARTESIAN_POINT('',(1.76637516134309,3.78467661248993,7.03153033211043));
#120663=CARTESIAN_POINT('Origin',(-0.0733069003038278,3.62501423486551,
-0.183755265501093));
#120664=CARTESIAN_POINT('Ctrl Pts',(1.8254226014359,3.7457690386059,7.27446440098778));
#120665=CARTESIAN_POINT('Ctrl Pts',(1.81869255493101,3.7500184674834,7.24656718951097));
#120666=CARTESIAN_POINT('Ctrl Pts',(1.81197503635231,3.75433282934033,7.2186767325143));
#120667=CARTESIAN_POINT('Ctrl Pts',(1.80522601115336,3.75872286882405,7.19080589214298));
#120668=CARTESIAN_POINT('Ctrl Pts',(1.79879017574622,3.76290918769458,7.1642284033945));
#120669=CARTESIAN_POINT('Ctrl Pts',(1.79233544045292,3.76716275954058,7.13766597884808));
#120670=CARTESIAN_POINT('Ctrl Pts',(1.78586077837975,3.77148708937977,7.11112003987493));
#120671=CARTESIAN_POINT('Ctrl Pts',(1.77938592606624,3.77581154627763,7.08457332092151));
#120672=CARTESIAN_POINT('Ctrl Pts',(1.77289109879307,3.78020679564289,7.05804288983037));
#120673=CARTESIAN_POINT('Ctrl Pts',(1.76637516089216,3.78467661258282,7.03153033156102));
#120674=CARTESIAN_POINT('Ctrl Pts',(0.989922564,3.655724827,7.18209950600001));
#120675=CARTESIAN_POINT('Ctrl Pts',(1.276254403,3.703213228,7.142633839));
#120676=CARTESIAN_POINT('Ctrl Pts',(1.558535692,3.75,7.080499029));
#120677=CARTESIAN_POINT('Ctrl Pts',(1.665134548,3.76766825,7.057034846));
#120678=CARTESIAN_POINT('Ctrl Pts',(1.770978732,3.785449891,7.030372275));
#120679=CARTESIAN_POINT('Ctrl Pts',(1.267168999,3.655724827,7.39217713));
#120680=CARTESIAN_POINT('Ctrl Pts',(1.561876092,3.703213228,7.341658361));
#120681=CARTESIAN_POINT('Ctrl Pts',(1.851626136,3.75,7.267838788));
#120682=CARTESIAN_POINT('Ctrl Pts',(1.961045444,3.76766825,7.23996204900001));
#120683=CARTESIAN_POINT('Ctrl Pts',(2.069575967,3.785449891,7.208804014));
#120684=CARTESIAN_POINT('Ctrl Pts',(0.989922569042201,3.65572482783626,
7.18209950530503));
#120685=CARTESIAN_POINT('Ctrl Pts',(1.13730475520406,3.68016830007153,7.16178553557222));
#120686=CARTESIAN_POINT('Ctrl Pts',(1.28373108860322,3.70444729863585,7.136976313866));
#120687=CARTESIAN_POINT('Ctrl Pts',(1.4288033920426,3.72849589780304,7.10781407124424));
#120688=CARTESIAN_POINT('Ctrl Pts',(1.47217175613058,3.73568506058438,7.09909622003723));
#120689=CARTESIAN_POINT('Ctrl Pts',(1.51541926466407,3.74285365858513,7.08998967248929));
#120690=CARTESIAN_POINT('Ctrl Pts',(1.55853569203865,3.74999999998231,7.08049902911643));
#120691=CARTESIAN_POINT('Ctrl Pts',(1.62794074349579,3.76150355498248,7.06522182162138));
#120692=CARTESIAN_POINT('Ctrl Pts',(1.69723617000859,3.77306479253841,7.04889858360392));
#120693=CARTESIAN_POINT('Ctrl Pts',(1.76637516099065,3.78467661232633,7.03153033149357));
#120694=CARTESIAN_POINT('Ctrl Pts',(0.208844493,3.785444214,7.246991374));
#120695=CARTESIAN_POINT('Ctrl Pts',(0.601139897,3.720864611,7.235686168));
#120696=CARTESIAN_POINT('Ctrl Pts',(0.989922564,3.655724827,7.182099506));
#120697=CARTESIAN_POINT('Ctrl Pts',(-0.029933757,3.785444214,7.499940264));
#120698=CARTESIAN_POINT('Ctrl Pts',(0.376054321,3.720864611,7.501560644));
#120699=CARTESIAN_POINT('Ctrl Pts',(0.77984494,3.655724827,7.459345941));
#120700=CARTESIAN_POINT('',(0.213507120844762,3.78467661246786,7.24685550681245));
#120701=CARTESIAN_POINT('Origin',(-0.0320910878355247,3.62501421661864,
-0.19521798448639));
#120702=CARTESIAN_POINT('Ctrl Pts',(0.218950420658305,3.74576903856463,
7.49680336600003));
#120703=CARTESIAN_POINT('Ctrl Pts',(0.218374794353158,3.75001846750272,
7.46811161477292));
#120704=CARTESIAN_POINT('Ctrl Pts',(0.217809951500075,3.75433282935218,
7.43942915323723));
#120705=CARTESIAN_POINT('Ctrl Pts',(0.217210121623312,3.75872286883286,
7.41075907670793));
#120706=CARTESIAN_POINT('Ctrl Pts',(0.216638126966634,3.76290918769233,
7.38341944055992));
#120707=CARTESIAN_POINT('Ctrl Pts',(0.216044435932847,3.76716275952922,
7.35609045350274));
#120708=CARTESIAN_POINT('Ctrl Pts',(0.215427740108189,3.7714870893588,7.32877328291361));
#120709=CARTESIAN_POINT('Ctrl Pts',(0.214811026164153,3.77581154624318,
7.30145530970816));
#120710=CARTESIAN_POINT('Ctrl Pts',(0.214171302877491,3.7802067955946,7.27414894952492));
#120711=CARTESIAN_POINT('Ctrl Pts',(0.213507120496326,3.78467661249255,
7.24685550621309));
#120712=CARTESIAN_POINT('Ctrl Pts',(-0.577160368,3.655724827,7.2269901));
#120713=CARTESIAN_POINT('Ctrl Pts',(-0.289038857,3.703213228,7.25000000000001));
#120714=CARTESIAN_POINT('Ctrl Pts',(0.,3.75,7.25));
#120715=CARTESIAN_POINT('Ctrl Pts',(0.10915074,3.76766825,7.25));
#120716=CARTESIAN_POINT('Ctrl Pts',(0.218252011,3.785449891,7.246714156));
#120717=CARTESIAN_POINT('Ctrl Pts',(-0.35155628,3.655724827,7.491756015));
#120718=CARTESIAN_POINT('Ctrl Pts',(-0.052879233,3.703213228,7.505771659));
#120719=CARTESIAN_POINT('Ctrl Pts',(0.245965642,3.75,7.495965642));
#120720=CARTESIAN_POINT('Ctrl Pts',(0.358819462,3.76766825,7.492262562));
#120721=CARTESIAN_POINT('Ctrl Pts',(0.471510658,3.785449891,7.48516383900001));
#120722=CARTESIAN_POINT('Ctrl Pts',(-0.577160365809908,3.655724827,7.22699010257026));
#120723=CARTESIAN_POINT('Ctrl Pts',(-0.428857240241091,3.68016825824677,
7.23883385462487));
#120724=CARTESIAN_POINT('Ctrl Pts',(-0.280521273726523,3.7044472163737,
7.24608198666862));
#120725=CARTESIAN_POINT('Ctrl Pts',(-0.132571908922941,3.72849577568566,
7.24878780841957));
#120726=CARTESIAN_POINT('Ctrl Pts',(-0.0883431417441284,3.73568497945282,
7.24959670111343));
#120727=CARTESIAN_POINT('Ctrl Pts',(-0.0441488467817412,3.74285361818873,
7.25000000004411));
#120728=CARTESIAN_POINT('Ctrl Pts',(2.36530813326477E-10,3.75000000003403,
7.25000000002632));
#120729=CARTESIAN_POINT('Ctrl Pts',(0.0710665482390681,3.76150355500044,
7.24999999999768));
#120730=CARTESIAN_POINT('Ctrl Pts',(0.142250900143361,3.77306479256824,
7.24895485867233));
#120731=CARTESIAN_POINT('Ctrl Pts',(0.213507120622118,3.78467661225502,
7.24685550617113));
#120732=CARTESIAN_POINT('Ctrl Pts',(0.209270709,2.233426833,7.246979079));
#120733=CARTESIAN_POINT('Ctrl Pts',(0.602449449,2.169174758,7.235625273));
#120734=CARTESIAN_POINT('Ctrl Pts',(0.992091961,2.104034486,7.18180016));
#120735=CARTESIAN_POINT('Ctrl Pts',(-0.029492665,2.233426833,7.499942012));
#120736=CARTESIAN_POINT('Ctrl Pts',(0.377410366,2.169174758,7.501542112));
#120737=CARTESIAN_POINT('Ctrl Pts',(0.782098092,2.104034486,7.45911003900001));
#120738=CARTESIAN_POINT('',(0.221277496030376,2.19371102278168,7.49673504087804));
#120739=CARTESIAN_POINT('',(0.782098084443547,2.10403448602304,7.45911003971491));
#120740=CARTESIAN_POINT('Origin',(-0.0334709911476522,2.01789494501912,
-0.18672642780092));
#120741=CARTESIAN_POINT('',(0.887095018906516,2.10403448477417,7.32045510042018));
#120742=CARTESIAN_POINT('Ctrl Pts',(0.221277495100879,2.19371102279664,
7.49673504090519));
#120743=CARTESIAN_POINT('Ctrl Pts',(0.220158920792203,2.19989438507272,
7.45504412804595));
#120744=CARTESIAN_POINT('Ctrl Pts',(0.218990649590036,2.20622738122548,
7.41335239673016));
#120745=CARTESIAN_POINT('Ctrl Pts',(0.216548003071353,2.2192010688388,7.33006921341966));
#120746=CARTESIAN_POINT('Ctrl Pts',(0.21527218294975,2.22584946938312,7.28842824146336));
#120747=CARTESIAN_POINT('Ctrl Pts',(0.213937948795667,2.23266407510067,
7.24684279883278));
#120748=CARTESIAN_POINT('Ctrl Pts',(0.984221732802958,2.10273945758871,
7.18288735118082));
#120749=CARTESIAN_POINT('Ctrl Pts',(0.988156846901479,2.10338697179435,
7.18234375559041));
#120750=CARTESIAN_POINT('Ctrl Pts',(0.992091961000001,2.104034486,7.18180016));
#120751=CARTESIAN_POINT('Ctrl Pts',(1.110469927,2.123513315,7.16544746));
#120752=CARTESIAN_POINT('Ctrl Pts',(1.228244647,2.142857143,7.145202243));
#120753=CARTESIAN_POINT('Ctrl Pts',(1.502027081,2.18782435,7.098139641));
#120754=CARTESIAN_POINT('Ctrl Pts',(1.77140546,2.233445087,7.030264767));
#120755=CARTESIAN_POINT('Ctrl Pts',(1.26130148850622,2.10273945758871,7.39318511227826));
#120756=CARTESIAN_POINT('Ctrl Pts',(1.26535166425311,2.10338697179435,7.39248957063913));
#120757=CARTESIAN_POINT('Ctrl Pts',(1.26940184,2.104034486,7.39179402900001));
#120758=CARTESIAN_POINT('Ctrl Pts',(1.391241145,2.123513315,7.370870416));
#120759=CARTESIAN_POINT('Ctrl Pts',(1.51232468,2.142857143,7.345942694));
#120760=CARTESIAN_POINT('Ctrl Pts',(1.793798878,2.18782435,7.287995009));
#120761=CARTESIAN_POINT('Ctrl Pts',(2.070013524,2.233445087,7.208678382));
#120762=CARTESIAN_POINT('',(1.26940183221411,2.10403448602285,7.39179403024986));
#120763=CARTESIAN_POINT('',(1.82768058314702,2.19371102273794,7.27389742077111));
#120764=CARTESIAN_POINT('Ctrl Pts',(1.26940183226555,2.10403448479508,7.39179403014459));
#120765=CARTESIAN_POINT('Ctrl Pts',(1.35075679015265,2.11704095516579,7.37782284375772));
#120766=CARTESIAN_POINT('Ctrl Pts',(1.43175196247422,2.12998516342569,7.36253036882388));
#120767=CARTESIAN_POINT('Ctrl Pts',(1.51232468132839,2.14285714321222,7.34594269372652));
#120768=CARTESIAN_POINT('Ctrl Pts',(1.61770521265512,2.15969232100109,7.32424778213805));
#120769=CARTESIAN_POINT('Ctrl Pts',(1.72287450736513,2.17665108707963,7.30023158799395));
#120770=CARTESIAN_POINT('Ctrl Pts',(1.82768058353484,2.19371102295844,7.27389742079628));
#120771=CARTESIAN_POINT('Ctrl Pts',(1.76679318445803,2.23266407503808,7.03142530635304));
#120772=CARTESIAN_POINT('Ctrl Pts',(1.77703575218887,2.22584954505362,7.07175123545953));
#120773=CARTESIAN_POINT('Ctrl Pts',(1.78723319543015,2.21920122285034,7.11214388952697));
#120774=CARTESIAN_POINT('Ctrl Pts',(1.80752239779132,2.20622738127396,7.19295582045961));
#120775=CARTESIAN_POINT('Ctrl Pts',(1.81762584542517,2.19989438509207,7.23342167862178));
#120776=CARTESIAN_POINT('Ctrl Pts',(1.82768058214188,2.19371102275407,7.27389742102327));
#120777=CARTESIAN_POINT('',(1.13074689248641,2.10403448732041,7.28679709574353));
#120778=CARTESIAN_POINT('Origin',(2.88506198098393E-13,2.19479107899967,
1.24553145575135E-12));
#120779=CARTESIAN_POINT('',(1.82046088170416,2.01370168037458,7.27570767520946));
#120780=CARTESIAN_POINT('Origin',(-0.0461554580507678,2.0178579971655,-0.187186739991818));
#120781=CARTESIAN_POINT('',(2.36730123479692,2.10403448602304,7.11659222239181));
#120782=CARTESIAN_POINT('Origin',(-0.0234499208926006,1.87510628711794,
-0.184916550569142));
#120783=CARTESIAN_POINT('Origin',(-0.0728291832817074,2.01789495839557,
-0.175165815870086));
#120784=CARTESIAN_POINT('Ctrl Pts',(1.762264358,2.233426833,7.032561719));
#120785=CARTESIAN_POINT('Ctrl Pts',(2.143810065,2.169174758,6.936951552));
#120786=CARTESIAN_POINT('Ctrl Pts',(2.512772145,2.104034486,6.800623218));
#120787=CARTESIAN_POINT('Ctrl Pts',(1.583462693,2.233426833,7.330937587));
#120788=CARTESIAN_POINT('Ctrl Pts',(1.981196531,2.169174758,7.245028153));
#120789=CARTESIAN_POINT('Ctrl Pts',(2.367301242,2.104034486,7.11659222000001));
#120790=CARTESIAN_POINT('',(2.44003668628186,2.10403448477417,6.95860772153105));
#120791=CARTESIAN_POINT('Ctrl Pts',(2.50531963238596,2.10273945758871,6.80337685771357));
#120792=CARTESIAN_POINT('Ctrl Pts',(2.50904588869298,2.10338697179435,6.80200003785678));
#120793=CARTESIAN_POINT('Ctrl Pts',(2.512772145,2.104034486,6.80062321800001));
#120794=CARTESIAN_POINT('Ctrl Pts',(2.624867152,2.123513315,6.759205071));
#120795=CARTESIAN_POINT('Ctrl Pts',(2.735536241,2.142857143,6.714115092));
#120796=CARTESIAN_POINT('Ctrl Pts',(2.992800725,2.18782435,6.60929765800001));
#120797=CARTESIAN_POINT('Ctrl Pts',(3.241290096,2.233445087,6.485101272));
#120798=CARTESIAN_POINT('Ctrl Pts',(2.82112921903791,2.10273945758871,6.94919401667824));
#120799=CARTESIAN_POINT('Ctrl Pts',(2.82493518301896,2.10338697179435,6.94764406833912));
#120800=CARTESIAN_POINT('Ctrl Pts',(2.828741147,2.104034486,6.94609412));
#120801=CARTESIAN_POINT('Ctrl Pts',(2.943233958,2.123513315,6.89946784));
#120802=CARTESIAN_POINT('Ctrl Pts',(3.056127904,2.142857143,6.849093534));
#120803=CARTESIAN_POINT('Ctrl Pts',(3.318564352,2.18782435,6.731992001));
#120804=CARTESIAN_POINT('Ctrl Pts',(3.571270523,2.233445087,6.595151768));
#120805=CARTESIAN_POINT('',(2.82874113964746,2.10403448602284,6.94609412285167));
#120806=CARTESIAN_POINT('',(3.34862335744545,2.19371102277393,6.71094044162914));
#120807=CARTESIAN_POINT('Ctrl Pts',(2.82874113969246,2.10403448479508,6.9460941227805));
#120808=CARTESIAN_POINT('Ctrl Pts',(2.90519067147956,2.11704095516575,6.91496066358089));
#120809=CARTESIAN_POINT('Ctrl Pts',(2.98100479150848,2.12998516342585,6.88261415040418));
#120810=CARTESIAN_POINT('Ctrl Pts',(3.05612790518021,2.14285714325508,6.84909353320588));
#120811=CARTESIAN_POINT('Ctrl Pts',(3.15438093342072,2.1596923211117,6.80525213688257));
#120812=CARTESIAN_POINT('Ctrl Pts',(3.2519286566968,2.1766510870814,6.75918913885246));
#120813=CARTESIAN_POINT('Ctrl Pts',(3.34862335742491,2.19371102292536,6.71094044145691));
#120814=CARTESIAN_POINT('Ctrl Pts',(3.23703513543889,2.23266407512044,6.4872261814177));
#120815=CARTESIAN_POINT('Ctrl Pts',(3.25570709552928,2.22584955417931,6.52440741393398));
#120816=CARTESIAN_POINT('Ctrl Pts',(3.27434932678514,2.2192012413584,6.56166350465828));
#120817=CARTESIAN_POINT('Ctrl Pts',(3.31153637344353,2.20622739343214,6.63622455513787));
#120818=CARTESIAN_POINT('Ctrl Pts',(3.3301025323744,2.19989440977418,6.6735723221256));
#120819=CARTESIAN_POINT('Ctrl Pts',(3.34862335692001,2.1937110227988,6.71094044189368));
#120820=CARTESIAN_POINT('',(2.67075663844113,2.1040344873204,6.87335867193713));
#120821=CARTESIAN_POINT('Origin',(1.10154940724527E-13,2.19479107899989,
1.74773390204663E-13));
#120822=CARTESIAN_POINT('',(3.34196159990719,2.01370168036029,6.71426039577534));
#120823=CARTESIAN_POINT('Origin',(-0.0853159245424984,2.01785799516844,
-0.172888221673519));
#120824=CARTESIAN_POINT('',(3.84181201039925,2.10403448602304,6.4413104627498));
#120825=CARTESIAN_POINT('Origin',(-0.0626532618141579,1.87510632037829,
-0.175552255440798));
#120826=CARTESIAN_POINT('Origin',(-0.108781860044905,2.01789497339341,-0.155414262569433));
#120827=CARTESIAN_POINT('Ctrl Pts',(3.232856486,2.233426833,6.489309589));
#120828=CARTESIAN_POINT('Ctrl Pts',(3.584928506,2.169174758,6.313913686));
#120829=CARTESIAN_POINT('Ctrl Pts',(3.915957895,2.104034486,6.101456692));
#120830=CARTESIAN_POINT('Ctrl Pts',(3.122377096,2.233426833,6.81914666800001));
#120831=CARTESIAN_POINT('Ctrl Pts',(3.492344149,2.169174758,6.649744731));
#120832=CARTESIAN_POINT('Ctrl Pts',(3.841812017,2.104034486,6.441310459));
#120833=CARTESIAN_POINT('',(3.87888494949472,2.10403448477417,6.27138357952356));
#120834=CARTESIAN_POINT('Ctrl Pts',(3.90927156911326,2.10273945758871,6.1057480230819));
#120835=CARTESIAN_POINT('Ctrl Pts',(3.91261473205663,2.10338697179435,6.10360235754095));
#120836=CARTESIAN_POINT('Ctrl Pts',(3.915957895,2.104034486,6.101456692));
#120837=CARTESIAN_POINT('Ctrl Pts',(4.016528506,2.123513315,6.036909765));
#120838=CARTESIAN_POINT('Ctrl Pts',(4.114917201,2.142857143,5.969083383));
#120839=CARTESIAN_POINT('Ctrl Pts',(4.343634335,2.18782435,5.811412262));
#120840=CARTESIAN_POINT('Ctrl Pts',(4.55961561000001,2.233445087,5.636701649));
#120841=CARTESIAN_POINT('Ctrl Pts',(4.24904408282165,2.10273945758871,6.18026633229042));
#120842=CARTESIAN_POINT('Ctrl Pts',(4.25242787241083,2.10338697179435,6.17793445114522));
#120843=CARTESIAN_POINT('Ctrl Pts',(4.255811662,2.104034486,6.17560257000001));
#120844=CARTESIAN_POINT('Ctrl Pts',(4.357604423,2.123513315,6.105453817));
#120845=CARTESIAN_POINT('Ctrl Pts',(4.457029984,2.142857143,6.031988372));
#120846=CARTESIAN_POINT('Ctrl Pts',(4.68815744500001,2.18782435,5.86120852900001));
#120847=CARTESIAN_POINT('Ctrl Pts',(4.905538882,2.233445087,5.673243189));
#120848=CARTESIAN_POINT('',(4.25581165537718,2.10403448602284,6.17560257428551));
#120849=CARTESIAN_POINT('',(4.71298822490245,2.19371102275907,5.83418734600645));
#120850=CARTESIAN_POINT('Ctrl Pts',(4.25581165546101,2.10403448479508,6.17560257428641));
#120851=CARTESIAN_POINT('Ctrl Pts',(4.32378106640512,2.11704095516577,6.12876260887064));
#120852=CARTESIAN_POINT('Ctrl Pts',(4.39086915015339,2.12998516342558,6.080874544256));
#120853=CARTESIAN_POINT('Ctrl Pts',(4.45702998493875,2.14285714318264,6.03198837130636));
#120854=CARTESIAN_POINT('Ctrl Pts',(4.54356130742803,2.15969232094174,5.96805046617741));
#120855=CARTESIAN_POINT('Ctrl Pts',(4.62892623627878,2.17665108709072,5.90209451773462));
#120856=CARTESIAN_POINT('Ctrl Pts',(4.71298822516702,2.19371102296318,5.83418734583089));
#120857=CARTESIAN_POINT('Ctrl Pts',(4.55591692076068,2.2326640751634,5.63969156977356));
#120858=CARTESIAN_POINT('Ctrl Pts',(4.58214553279196,2.22584946947947,5.6719900080537));
#120859=CARTESIAN_POINT('Ctrl Pts',(4.6083612467119,2.21920106896372,5.70436800343796));
#120860=CARTESIAN_POINT('Ctrl Pts',(4.66070659567174,2.20622739621349,5.7691908669884));
#120861=CARTESIAN_POINT('Ctrl Pts',(4.68686734132964,2.19989441540384,5.8016742728421));
#120862=CARTESIAN_POINT('Ctrl Pts',(4.71298822419491,2.19371102277413,5.83418734657775));
#120863=CARTESIAN_POINT('',(4.08588477174921,2.10403448732041,6.13852963549342));
#120864=CARTESIAN_POINT('Origin',(-9.68843061333047E-13,2.19479107900022,
-1.23252102968152E-12));
#120865=CARTESIAN_POINT('',(4.70719590771126,2.013701680375,5.83886176247297));
#120866=CARTESIAN_POINT('Origin',(-0.120487294631751,2.01785797603456,-0.150505974900553));
#120867=CARTESIAN_POINT('',(5.13668392641915,2.10403448602304,5.46484018414439));
#120868=CARTESIAN_POINT('Origin',(-0.0989268749541183,1.87510626229254,
-0.157979202217122));
#120869=CARTESIAN_POINT('Origin',(-0.139648184984119,2.01789496832727,-0.128396010934203));
#120870=CARTESIAN_POINT('Ctrl Pts',(4.552283837,2.233426833,5.642624555));
#120871=CARTESIAN_POINT('Ctrl Pts',(4.858419675,2.169174758,5.395644234));
#120872=CARTESIAN_POINT('Ctrl Pts',(5.136037807,2.104034486,5.116992833));
#120873=CARTESIAN_POINT('Ctrl Pts',(4.515292615,2.233426833,5.988500029));
#120874=CARTESIAN_POINT('Ctrl Pts',(4.84019363500001,2.169174758,5.74352663500001));
#120875=CARTESIAN_POINT('Ctrl Pts',(5.136683932,2.104034486,5.464840179));
#120876=CARTESIAN_POINT('',(5.13636086401175,2.10403448477417,5.29091651132793));
#120877=CARTESIAN_POINT('Ctrl Pts',(5.13043031307457,2.10273945758871,5.12262119754958));
#120878=CARTESIAN_POINT('Ctrl Pts',(5.13323406003728,2.10338697179435,5.11980701527479));
#120879=CARTESIAN_POINT('Ctrl Pts',(5.136037807,2.104034486,5.11699283300001));
#120880=CARTESIAN_POINT('Ctrl Pts',(5.220381451,2.123513315,5.032335269));
#120881=CARTESIAN_POINT('Ctrl Pts',(5.301889206,2.142857143,4.944943968));
#120882=CARTESIAN_POINT('Ctrl Pts',(5.49136443000001,2.18782435,4.741791688));
#120883=CARTESIAN_POINT('Ctrl Pts',(5.664738566,2.233445087,4.524736122));
#120884=CARTESIAN_POINT('Ctrl Pts',(5.47827836712804,2.10273945758871,5.12235626254307));
#120885=CARTESIAN_POINT('Ctrl Pts',(5.48108176006402,2.10338697179435,5.11935148477153));
#120886=CARTESIAN_POINT('Ctrl Pts',(5.483885153,2.104034486,5.116346707));
#120887=CARTESIAN_POINT('Ctrl Pts',(5.568218147,2.123513315,5.025955559));
#120888=CARTESIAN_POINT('Ctrl Pts',(5.649526295,2.142857143,4.932834139));
#120889=CARTESIAN_POINT('Ctrl Pts',(5.838537507,2.18782435,4.71636146100001));
#120890=CARTESIAN_POINT('Ctrl Pts',(6.010429695,2.233445087,4.486060063));
#120891=CARTESIAN_POINT('',(5.48388515162104,2.10403448644943,5.11634671002942));
#120892=CARTESIAN_POINT('',(5.85697900152487,2.19371102277848,4.68463413472096));
#120893=CARTESIAN_POINT('Ctrl Pts',(5.48388515081103,2.10403448555181,5.11634670908027));
#120894=CARTESIAN_POINT('Ctrl Pts',(5.5401962652435,2.11704095566781,5.05599042349386));
#120895=CARTESIAN_POINT('Ctrl Pts',(5.59542134742777,2.12998516367539,4.9948000018663));
#120896=CARTESIAN_POINT('Ctrl Pts',(5.64952629587031,2.14285714323533,4.93283413787128));
#120897=CARTESIAN_POINT('Ctrl Pts',(5.72028980490418,2.1596923210693,4.85178938829458));
#120898=CARTESIAN_POINT('Ctrl Pts',(5.78948036981908,2.17665108709428,4.76902451731539));
#120899=CARTESIAN_POINT('Ctrl Pts',(5.85697900143682,2.19371102292441,4.68463413468002));
#120900=CARTESIAN_POINT('Ctrl Pts',(5.66176909438834,2.2326640750986,4.52845124925428));
#120901=CARTESIAN_POINT('Ctrl Pts',(5.69432770564971,2.22584946943075,4.55435619166373));
#120902=CARTESIAN_POINT('Ctrl Pts',(5.72689082273297,2.21920106893194,4.58034160385709));
#120903=CARTESIAN_POINT('Ctrl Pts',(5.79194737442727,2.20622739455584,4.63239624867638));
#120904=CARTESIAN_POINT('Ctrl Pts',(5.8244794777516,2.19989441206853,4.65849643099321));
#120905=CARTESIAN_POINT('Ctrl Pts',(5.85697900107028,2.19371102279883,4.68463413529101));
#120906=CARTESIAN_POINT('',(5.30996147437299,2.10403448732041,5.11666977583958));
#120907=CARTESIAN_POINT('Origin',(8.50014503228635E-14,2.19479107899956,
-6.0281640790194E-14));
#120908=CARTESIAN_POINT('',(5.85232696648488,2.01370168039118,4.69044444290746));
#120909=CARTESIAN_POINT('Origin',(-0.150024755449846,2.01785801005925,-0.121086082215633));
#120910=CARTESIAN_POINT('',(6.19137021059321,2.10403448602304,4.23284005318077));
#120911=CARTESIAN_POINT('Origin',(-0.130574934157813,1.87510630182543,-0.133019420198138));
#120912=CARTESIAN_POINT('Origin',(-0.163984545083379,2.01789498312784,-0.0953738858012115));
#120913=CARTESIAN_POINT('Ctrl Pts',(5.658851455,2.233426833,4.532096669));
#120914=CARTESIAN_POINT('Ctrl Pts',(5.904736539,2.169174758,4.225080454));
#120915=CARTESIAN_POINT('Ctrl Pts',(6.115962299,2.104034486,3.893264076));
#120916=CARTESIAN_POINT('Ctrl Pts',(5.697078071,2.233426833,4.877837785));
#120917=CARTESIAN_POINT('Ctrl Pts',(5.961721047,2.169174758,4.568747618));
#120918=CARTESIAN_POINT('Ctrl Pts',(6.191370215,2.104034486,4.232840047));
#120919=CARTESIAN_POINT('',(6.15366625278541,2.10403448477417,4.06305206788318));
#120920=CARTESIAN_POINT('Ctrl Pts',(6.11169583714959,2.10273945758871,3.89996629798646));
#120921=CARTESIAN_POINT('Ctrl Pts',(6.1138290680748,2.10338697179435,3.89661518699323));
#120922=CARTESIAN_POINT('Ctrl Pts',(6.115962299,2.104034486,3.893264076));
#120923=CARTESIAN_POINT('Ctrl Pts',(6.180135162,2.123513315,3.792454368));
#120924=CARTESIAN_POINT('Ctrl Pts',(6.240950764,2.142857143,3.68958447));
#120925=CARTESIAN_POINT('Ctrl Pts',(6.382324428,2.18782435,3.450450204));
#120926=CARTESIAN_POINT('Ctrl Pts',(6.504984643,2.233445087,3.201198963));
#120927=CARTESIAN_POINT('Ctrl Pts',(6.45135444343917,2.10273945758871,3.82493050776523));
#120928=CARTESIAN_POINT('Ctrl Pts',(6.45344635621958,2.10338697179435,3.82139333338262));
#120929=CARTESIAN_POINT('Ctrl Pts',(6.455538269,2.104034486,3.817856159));
#120930=CARTESIAN_POINT('Ctrl Pts',(6.51846818000001,2.123513315,3.711449204));
#120931=CARTESIAN_POINT('Ctrl Pts',(6.577857036,2.142857143,3.603026063));
#120932=CARTESIAN_POINT('Ctrl Pts',(6.71591404400001,2.18782435,3.350982573));
#120933=CARTESIAN_POINT('Ctrl Pts',(6.834279495,2.233445087,3.089113754));
#120934=CARTESIAN_POINT('',(6.45553826687932,2.10403448645287,3.81785616360662));
#120935=CARTESIAN_POINT('',(6.72710394928449,2.19371102277434,3.31603263760013));
#120936=CARTESIAN_POINT('Ctrl Pts',(6.45553826486484,2.10403448479514,3.81785616563568));
#120937=CARTESIAN_POINT('Ctrl Pts',(6.49755804059041,2.11704095516578,3.74680574940807));
#120938=CARTESIAN_POINT('Ctrl Pts',(6.53833786010976,2.1299851634258,3.67517416401284));
#120939=CARTESIAN_POINT('Ctrl Pts',(6.57785703661758,2.14285714324141,3.60302606167866));
#120940=CARTESIAN_POINT('Ctrl Pts',(6.62954390864494,2.15969232108233,3.50866403078514));
#120941=CARTESIAN_POINT('Ctrl Pts',(6.67932483578951,2.17665108709007,3.41296023049362));
#120942=CARTESIAN_POINT('Ctrl Pts',(6.72710394921967,2.19371102294551,3.31603263741837));
#120943=CARTESIAN_POINT('Ctrl Pts',(6.50288323742489,2.23266407508744,3.20546558167077));
#120944=CARTESIAN_POINT('Ctrl Pts',(6.54024908133438,2.22584953542554,3.22376556438151));
#120945=CARTESIAN_POINT('Ctrl Pts',(6.57763657488875,2.21920120319565,3.24214314013562));
#120946=CARTESIAN_POINT('Ctrl Pts',(6.65236312620955,2.20622739415915,3.27899592300733));
#120947=CARTESIAN_POINT('Ctrl Pts',(6.68974541749201,2.19989441124867,3.29749245826285));
#120948=CARTESIAN_POINT('Ctrl Pts',(6.72710394898493,2.1937110227962,3.31603263821102));
#120949=CARTESIAN_POINT('',(6.28575027975988,2.10403448732041,3.8555601244127));
#120950=CARTESIAN_POINT('Origin',(-4.78783679369599E-13,2.19479107899967,
-2.39391839684799E-13));
#120951=CARTESIAN_POINT('',(6.72380972100024,2.01370168038612,3.32270715385081));
#120952=CARTESIAN_POINT('Origin',(-0.172547194246069,2.01785801023315,-0.0860042763948671));
#120953=CARTESIAN_POINT('',(6.95655490512516,2.10403448602304,2.80291702502399));
#120954=CARTESIAN_POINT('Origin',(-0.156117583468591,1.87510627379371,-0.101839827848934));
#120955=CARTESIAN_POINT('Origin',(-0.180653106157236,2.01789493165625,-0.0578921944339506));
#120956=CARTESIAN_POINT('Ctrl Pts',(6.500817468,2.233426833,3.209652979));
#120957=CARTESIAN_POINT('Ctrl Pts',(6.674954485,2.169174758,2.856956608));
#120958=CARTESIAN_POINT('Ctrl Pts',(6.809911191,2.104034486,2.487490617));
#120959=CARTESIAN_POINT('Ctrl Pts',(6.612474487,2.233426833,3.539093268));
#120960=CARTESIAN_POINT('Ctrl Pts',(6.804485009,2.169174758,3.180339039));
#120961=CARTESIAN_POINT('Ctrl Pts',(6.956554908,2.104034486,2.802917018));
#120962=CARTESIAN_POINT('',(6.88323304675614,2.10403448477417,2.64520382463995));
#120963=CARTESIAN_POINT('Ctrl Pts',(6.80718525625549,2.10273945758871,2.49495330789937));
#120964=CARTESIAN_POINT('Ctrl Pts',(6.80854822362774,2.10338697179435,2.49122196244969));
#120965=CARTESIAN_POINT('Ctrl Pts',(6.809911191,2.104034486,2.487490617));
#120966=CARTESIAN_POINT('Ctrl Pts',(6.850912621,2.123513315,2.375242516));
#120967=CARTESIAN_POINT('Ctrl Pts',(6.888192401,2.142857143,2.261704102));
#120968=CARTESIAN_POINT('Ctrl Pts',(6.974854028,2.18782435,1.997769504));
#120969=CARTESIAN_POINT('Ctrl Pts',(7.041064867,2.233445087,1.727977298));
#120970=CARTESIAN_POINT('Ctrl Pts',(7.1227723568037,2.10273945758871,2.34865525323209));
#120971=CARTESIAN_POINT('Ctrl Pts',(7.12405497390185,2.10338697179435,2.34475107661605));
#120972=CARTESIAN_POINT('Ctrl Pts',(7.125337591,2.104034486,2.3408469));
#120973=CARTESIAN_POINT('Ctrl Pts',(7.163921886,2.123513315,2.22339961));
#120974=CARTESIAN_POINT('Ctrl Pts',(7.198614493,2.142857143,2.104744493));
#120975=CARTESIAN_POINT('Ctrl Pts',(7.279261905,2.18782435,1.828915464));
#120976=CARTESIAN_POINT('Ctrl Pts',(7.338565982,2.233445087,1.547723919));
#120977=CARTESIAN_POINT('',(7.12533758978023,2.10403448645145,2.34084690533364));
#120978=CARTESIAN_POINT('',(7.28267699335155,2.19371102276864,1.7923771396886));
#120979=CARTESIAN_POINT('Ctrl Pts',(7.125337588388,2.10403448479513,2.34084690736949));
#120980=CARTESIAN_POINT('Ctrl Pts',(7.15110122605881,2.11704095516579,2.26242460083382));
#120981=CARTESIAN_POINT('Ctrl Pts',(7.17552896264762,2.12998516342569,2.18370126632093));
#120982=CARTESIAN_POINT('Ctrl Pts',(7.19861449338138,2.14285714321265,2.1047444916956));
#120983=CARTESIAN_POINT('Ctrl Pts',(7.22880790787021,2.15969232101418,2.00147744319749));
#120984=CARTESIAN_POINT('Ctrl Pts',(7.25685149639181,2.17665108709078,1.8973097164389));
#120985=CARTESIAN_POINT('Ctrl Pts',(7.28267699333017,2.1937110229533,1.79237713946812));
#120986=CARTESIAN_POINT('Ctrl Pts',(7.03992978818633,2.23266407510364,1.73259590538724));
#120987=CARTESIAN_POINT('Ctrl Pts',(7.08035593384536,2.22584954571016,1.74243547782734));
#120988=CARTESIAN_POINT('Ctrl Pts',(7.12081989475702,2.21920122410525,1.75234617281721));
#120989=CARTESIAN_POINT('Ctrl Pts',(7.20172176572101,2.20622739487872,1.77227338946031));
#120990=CARTESIAN_POINT('Ctrl Pts',(7.24220628307591,2.19989441271045,1.78230139712961));
#120991=CARTESIAN_POINT('Ctrl Pts',(7.2826769931679,2.19371102278755,1.79237714043786));
#120992=CARTESIAN_POINT('',(6.96762438834504,2.10403448732041,2.41416876616258));
#120993=CARTESIAN_POINT('Origin',(-5.96311194867027E-13,2.194791079001,
-9.15066633577766E-14));
#120994=CARTESIAN_POINT('',(7.28089460575536,2.01370168035532,1.79960377154688));
#120995=CARTESIAN_POINT('Origin',(-0.187001519079321,2.01785800852069,-0.0469009978311266));
#120996=CARTESIAN_POINT('',(7.39645882446895,2.10403448602304,1.24193271243861));
#120997=CARTESIAN_POINT('Origin',(-0.174359959711083,1.87510632648327,-0.0658981560518858));
#120998=CARTESIAN_POINT('Origin',(-0.188874785710973,2.01789494957119,-0.0177036690202756));
#120999=CARTESIAN_POINT('Ctrl Pts',(7.038812482,2.233426833,1.737129483));
#121000=CARTESIAN_POINT('Ctrl Pts',(7.133058978,2.169174758,1.355244646));
#121001=CARTESIAN_POINT('Ctrl Pts',(7.185436205,2.104034486,0.965404863000001));
#121002=CARTESIAN_POINT('Ctrl Pts',(7.218678946,2.233426833,2.034864682));
#121003=CARTESIAN_POINT('Ctrl Pts',(7.329078814,2.169174758,1.643221342));
#121004=CARTESIAN_POINT('Ctrl Pts',(7.39645882600001,2.104034486,1.241932705));
#121005=CARTESIAN_POINT('',(7.29094751435517,2.10403448477417,1.10366879156288));
#121006=CARTESIAN_POINT('Ctrl Pts',(7.18437825902062,2.10273945758871,0.973279075776289));
#121007=CARTESIAN_POINT('Ctrl Pts',(7.18490723201031,2.10338697179435,0.969341969388144));
#121008=CARTESIAN_POINT('Ctrl Pts',(7.185436205,2.104034486,0.965404863));
#121009=CARTESIAN_POINT('Ctrl Pts',(7.201349021,2.123513315,0.846966964));
#121010=CARTESIAN_POINT('Ctrl Pts',(7.213349817,2.142857143,0.728068964));
#121011=CARTESIAN_POINT('Ctrl Pts',(7.241247207,2.18782435,0.451675322));
#121012=CARTESIAN_POINT('Ctrl Pts',(7.24791272300001,2.233445087,0.173957335));
#121013=CARTESIAN_POINT('Ctrl Pts',(7.46113735175124,2.10273945758871,0.762559489829848));
#121014=CARTESIAN_POINT('Ctrl Pts',(7.46155069937562,2.10338697179435,0.758470865914925));
#121015=CARTESIAN_POINT('Ctrl Pts',(7.461964047,2.104034486,0.754382242));
#121016=CARTESIAN_POINT('Ctrl Pts',(7.474398566,2.123513315,0.631386321));
#121017=CARTESIAN_POINT('Ctrl Pts',(7.482772737,2.142857143,0.50804741));
#121018=CARTESIAN_POINT('Ctrl Pts',(7.50223956900001,2.18782435,0.221330301));
#121019=CARTESIAN_POINT('Ctrl Pts',(7.49970928,2.233445087,-0.066035765));
#121020=CARTESIAN_POINT('Ctrl Pts',(7.24779704645756,2.23266407511293,0.178711969599128));
#121021=CARTESIAN_POINT('Ctrl Pts',(7.28939373424232,2.22584946942467,0.179631082645235));
#121022=CARTESIAN_POINT('Ctrl Pts',(7.33104270738621,2.21920106891639,0.180611530318155));
#121023=CARTESIAN_POINT('Ctrl Pts',(7.4143359909464,2.20622738129719,0.182681326636278));
#121024=CARTESIAN_POINT('Ctrl Pts',(7.45602982682077,2.19989438512088,0.183771913550348));
#121025=CARTESIAN_POINT('Ctrl Pts',(7.49772015495655,2.19371102281662,0.184912080174598));
#121026=CARTESIAN_POINT('',(7.32370012505434,2.10403448732041,0.859893560554172));
#121027=CARTESIAN_POINT('Ctrl Pts',(7.247680448,2.233426833,0.183379743));
#121028=CARTESIAN_POINT('Ctrl Pts',(7.257629561,2.169174758,-0.209837049));
#121029=CARTESIAN_POINT('Ctrl Pts',(7.224978208,2.104034486,-0.601822151));
#121030=CARTESIAN_POINT('Ctrl Pts',(7.487346,2.233426833,0.435488086));
#121031=CARTESIAN_POINT('Ctrl Pts',(7.510973039,2.169174758,0.029268441));
#121032=CARTESIAN_POINT('Ctrl Pts',(7.490512549,2.104034486,-0.377123002));
#121033=CARTESIAN_POINT('',(7.35774537900773,2.10403448477417,-0.489472568867835));
#121034=CARTESIAN_POINT('Ctrl Pts',(7.22563771925764,2.10273945758871,-0.593904605882857));
#121035=CARTESIAN_POINT('Ctrl Pts',(7.22530796362882,2.10338697179435,-0.597863378441428));
#121036=CARTESIAN_POINT('Ctrl Pts',(7.224978208,2.104034486,-0.601822151));
#121037=CARTESIAN_POINT('Ctrl Pts',(7.215058343,2.123513315,-0.720911822));
#121038=CARTESIAN_POINT('Ctrl Pts',(7.201219013,2.142857143,-0.839609869));
#121039=CARTESIAN_POINT('Ctrl Pts',(7.169047714,2.18782435,-1.115538695));
#121040=CARTESIAN_POINT('Ctrl Pts',(7.115856237,2.233445087,-1.38819668));
#121041=CARTESIAN_POINT('Ctrl Pts',(7.45062785596414,2.10273945758871,-0.859192708687909));
#121042=CARTESIAN_POINT('Ctrl Pts',(7.45015260648208,2.10338697179435,-0.863274600343954));
#121043=CARTESIAN_POINT('Ctrl Pts',(7.449677357,2.104034486,-0.867356492));
#121044=CARTESIAN_POINT('Ctrl Pts',(7.435380677,2.123513315,-0.99014989));
#121045=CARTESIAN_POINT('Ctrl Pts',(7.417044844,2.142857143,-1.112405405));
#121046=CARTESIAN_POINT('Ctrl Pts',(7.37442085,2.18782435,-1.396604021));
#121047=CARTESIAN_POINT('Ctrl Pts',(7.310174507,2.233445087,-1.676707691));
#121048=CARTESIAN_POINT('',(7.44967735805002,2.10403448645287,-0.86735648699064));
#121049=CARTESIAN_POINT('',(7.36217825550271,2.19371102279854,-1.43119926446366));
#121050=CARTESIAN_POINT('Ctrl Pts',(7.44967735772419,2.10403448479508,-0.867356484214936));
#121051=CARTESIAN_POINT('Ctrl Pts',(7.44013112972914,2.11704095516576,-0.94934851233994));
#121052=CARTESIAN_POINT('Ctrl Pts',(7.42924607263757,2.12998516342571,-1.03105281584612));
#121053=CARTESIAN_POINT('Ctrl Pts',(7.41704484379483,2.14285714321645,-1.11240540636801));
#121054=CARTESIAN_POINT('Ctrl Pts',(7.40108693653606,2.15969232103061,-1.21880592696433));
#121055=CARTESIAN_POINT('Ctrl Pts',(7.38279971496218,2.17665108712091,-1.32512119247307));
#121056=CARTESIAN_POINT('Ctrl Pts',(7.36217825556157,2.19371102302331,-1.43119926485229));
#121057=CARTESIAN_POINT('Ctrl Pts',(7.11676536986912,2.2326640751513,-1.3835283379909));
#121058=CARTESIAN_POINT('Ctrl Pts',(7.15758669679708,2.22584954216184,-1.39157268591327));
#121059=CARTESIAN_POINT('Ctrl Pts',(7.19847221067012,2.21920121681727,-1.39956836349629));
#121060=CARTESIAN_POINT('Ctrl Pts',(7.28026402078548,2.20622738133191,-1.41545273276343));
#121061=CARTESIAN_POINT('Ctrl Pts',(7.32121752195779,2.19989438514916,-1.42335058539379));
#121062=CARTESIAN_POINT('Ctrl Pts',(7.36217825570581,2.19371102281618,-1.43119926341763));
#121063=CARTESIAN_POINT('',(7.33732778330786,2.10403448732041,-0.734589313430841));
#121064=CARTESIAN_POINT('Origin',(-4.32379826387219E-13,2.19479107899978,
7.35089072945172E-14));
#121065=CARTESIAN_POINT('',(7.36359498823949,2.01370168036158,-1.42389214627152));
#121066=CARTESIAN_POINT('Origin',(-0.189411173610758,2.01785802215147,0.0359537117828659));
#121067=CARTESIAN_POINT('',(7.23431823199796,2.10403448602304,-1.97854484767787));
#121068=CARTESIAN_POINT('Origin',(-0.185914974555001,1.8751063385133,0.0134043706131987));
#121069=CARTESIAN_POINT('Origin',(-0.178851690633703,2.01789495737722,0.0632390566086299));
#121070=CARTESIAN_POINT('Ctrl Pts',(7.11765493,2.233426833,-1.37894463));
#121071=CARTESIAN_POINT('Ctrl Pts',(7.042841452,2.169174758,-1.765106997));
#121072=CARTESIAN_POINT('Ctrl Pts',(6.926688259,2.104034486,-2.140908629));
#121073=CARTESIAN_POINT('Ctrl Pts',(7.405913077,2.233426833,-1.184251449));
#121074=CARTESIAN_POINT('Ctrl Pts',(7.341662513,2.169174758,-1.586053019));
#121075=CARTESIAN_POINT('Ctrl Pts',(7.23431823,2.104034486,-1.978544855));
#121076=CARTESIAN_POINT('',(7.08050324663655,2.10403448477417,-2.05972673465542));
#121077=CARTESIAN_POINT('Ctrl Pts',(6.92903438933913,2.10273945758871,-2.13331796710826));
#121078=CARTESIAN_POINT('Ctrl Pts',(6.92786132416957,2.10338697179435,-2.13711329805413));
#121079=CARTESIAN_POINT('Ctrl Pts',(6.926688259,2.104034486,-2.140908629));
#121080=CARTESIAN_POINT('Ctrl Pts',(6.891399557,2.123513315,-2.255081572));
#121081=CARTESIAN_POINT('Ctrl Pts',(6.852367211,2.142857143,-2.368029478));
#121082=CARTESIAN_POINT('Ctrl Pts',(6.761631518,2.18782435,-2.630591364));
#121083=CARTESIAN_POINT('Ctrl Pts',(6.65107022100001,2.233445087,-2.88544016));
#121084=CARTESIAN_POINT('Ctrl Pts',(7.09173528189306,2.10273945758871,-2.44077001058573));
#121085=CARTESIAN_POINT('Ctrl Pts',(7.09039365744652,2.10338697179435,-2.44465430529287));
#121086=CARTESIAN_POINT('Ctrl Pts',(7.089052033,2.104034486,-2.4485386));
#121087=CARTESIAN_POINT('Ctrl Pts',(7.048692651,2.123513315,-2.565387793));
#121088=CARTESIAN_POINT('Ctrl Pts',(7.004504177,2.142857143,-2.68084338));
#121089=CARTESIAN_POINT('Ctrl Pts',(6.901782407,2.18782435,-2.949234692));
#121090=CARTESIAN_POINT('Ctrl Pts',(6.778824099,2.233445087,-3.208978629));
#121091=CARTESIAN_POINT('',(7.08905203541496,2.10403448602284,-2.44853859249194));
#121092=CARTESIAN_POINT('',(6.88238908334387,2.19371102272824,-2.98038932157766));
#121093=CARTESIAN_POINT('Ctrl Pts',(7.08905203538081,2.10403448479508,-2.44853859255263));
#121094=CARTESIAN_POINT('Ctrl Pts',(7.06210313077159,2.11704095516578,-2.52656153578999));
#121095=CARTESIAN_POINT('Ctrl Pts',(7.03390855006303,2.1299851634255,-2.60401567259929));
#121096=CARTESIAN_POINT('Ctrl Pts',(7.00450417663004,2.14285714316195,-2.68084338096663));
#121097=CARTESIAN_POINT('Ctrl Pts',(6.96604638994939,2.15969232088389,-2.78132583779706));
#121098=CARTESIAN_POINT('Ctrl Pts',(6.92533207396718,2.1766510870693,-2.88122430014084));
#121099=CARTESIAN_POINT('Ctrl Pts',(6.88238908322556,2.19371102292877,-2.98038932185199));
#121100=CARTESIAN_POINT('Ctrl Pts',(6.65296165455413,2.23266407514811,-2.88107639833952));
#121101=CARTESIAN_POINT('Ctrl Pts',(6.69109930720342,2.22584954166836,-2.89770805379725));
#121102=CARTESIAN_POINT('Ctrl Pts',(6.72931010913872,2.21920121582914,-2.91430597519197));
#121103=CARTESIAN_POINT('Ctrl Pts',(6.80577491209313,2.20622739563285,-2.94740175930617));
#121104=CARTESIAN_POINT('Ctrl Pts',(6.84407304226061,2.1998944142384,-2.96391871576311));
#121105=CARTESIAN_POINT('Ctrl Pts',(6.88238908369198,2.19371102274336,-2.98038932077352));
#121106=CARTESIAN_POINT('',(7.00787014852359,2.1040344873204,-2.2947236067932));
#121107=CARTESIAN_POINT('Origin',(-9.86190296092815E-13,2.19479107899967,
4.562322741819E-13));
#121108=CARTESIAN_POINT('',(6.88534350783936,2.01370168036146,-2.97355759565002));
#121109=CARTESIAN_POINT('Origin',(-0.177253920966249,2.01785798996329,0.0758309605004354));
#121110=CARTESIAN_POINT('',(6.63985523530347,2.10403448602304,-3.48745214416206));
#121111=CARTESIAN_POINT('Origin',(-0.178686657155458,1.87510628692599,0.0530570999994617));
#121112=CARTESIAN_POINT('Origin',(-0.161075815931262,2.01789495313179,0.100208434369154));
#121113=CARTESIAN_POINT('Ctrl Pts',(6.654815779,2.233426833,-2.876791084));
#121114=CARTESIAN_POINT('Ctrl Pts',(6.498737904,2.169174758,-3.237842504));
#121115=CARTESIAN_POINT('Ctrl Pts',(6.304514067,2.104034486,-3.579888599));
#121116=CARTESIAN_POINT('Ctrl Pts',(6.97818789,2.233426833,-2.748616702));
#121117=CARTESIAN_POINT('Ctrl Pts',(6.829064008,2.169174758,-3.127212403));
#121118=CARTESIAN_POINT('Ctrl Pts',(6.639855232,2.104034486,-3.487452151));
#121119=CARTESIAN_POINT('',(6.47218465316547,2.10403448477417,-3.53367036828643));
#121120=CARTESIAN_POINT('Ctrl Pts',(6.30843711407222,2.10273945758871,-3.5729797511861));
#121121=CARTESIAN_POINT('Ctrl Pts',(6.30647559053612,2.10338697179435,-3.57643417509305));
#121122=CARTESIAN_POINT('Ctrl Pts',(6.30451406700001,2.104034486,-3.579888599));
#121123=CARTESIAN_POINT('Ctrl Pts',(6.245506587,2.123513315,-3.683806215));
#121124=CARTESIAN_POINT('Ctrl Pts',(6.183106334,2.142857143,-3.785722661));
#121125=CARTESIAN_POINT('Ctrl Pts',(6.038048947,2.18782435,-4.022640503));
#121126=CARTESIAN_POINT('Ctrl Pts',(5.875287554,2.233445087,-4.247763666));
#121127=CARTESIAN_POINT('Ctrl Pts',(6.4012410481422,2.10273945758871,-3.90821961906406));
#121128=CARTESIAN_POINT('Ctrl Pts',(6.39909578157111,2.10338697179435,-3.91172469153203));
#121129=CARTESIAN_POINT('Ctrl Pts',(6.39695051500001,2.104034486,-3.915229764));
#121130=CARTESIAN_POINT('Ctrl Pts',(6.33241559,2.123513315,-4.020671014));
#121131=CARTESIAN_POINT('Ctrl Pts',(6.264440681,2.142857143,-4.123928098));
#121132=CARTESIAN_POINT('Ctrl Pts',(6.10642429,2.18782435,-4.363962426));
#121133=CARTESIAN_POINT('Ctrl Pts',(5.93050341,2.233445087,-4.591201292));
#121134=CARTESIAN_POINT('',(6.39695051908625,2.10403448602285,-3.91522975725624));
#121135=CARTESIAN_POINT('',(6.08078704656053,2.19371102280142,-4.39021968642618));
#121136=CARTESIAN_POINT('Ctrl Pts',(6.39695051892612,2.10403448479508,-3.91522975723856));
#121137=CARTESIAN_POINT('Ctrl Pts',(6.35385903796573,2.11704095516575,-3.98563534974328));
#121138=CARTESIAN_POINT('Ctrl Pts',(6.30967328131607,2.12998516342593,-4.055217650617));
#121139=CARTESIAN_POINT('Ctrl Pts',(6.26444067997456,2.14285714327577,-4.12392809923762));
#121140=CARTESIAN_POINT('Ctrl Pts',(6.20528125616144,2.15969232116965,-4.2137940452781));
#121141=CARTESIAN_POINT('Ctrl Pts',(6.14404360261655,2.17665108712213,-4.3026045618202));
#121142=CARTESIAN_POINT('Ctrl Pts',(6.08078704643701,2.1937110230209,-4.39021968677865));
#121143=CARTESIAN_POINT('Ctrl Pts',(5.87807284688596,2.23266407510804,-4.24390852932449));
#121144=CARTESIAN_POINT('Ctrl Pts',(5.91174353685336,2.22584954390413,-4.26834980573084));
#121145=CARTESIAN_POINT('Ctrl Pts',(5.94549291609518,2.21920122043011,-4.29277386055344));
#121146=CARTESIAN_POINT('Ctrl Pts',(6.0130554977416,2.20622738131649,-4.34153362698864));
#121147=CARTESIAN_POINT('Ctrl Pts',(6.04690766649077,2.19989438513347,-4.36589745271608));
#121148=CARTESIAN_POINT('Ctrl Pts',(6.0807870471606,2.19371102281822,-4.3902196855946));
#121149=CARTESIAN_POINT('',(6.35073229512134,2.10403448732041,-3.74755917451584));
#121150=CARTESIAN_POINT('Origin',(-9.68843061333047E-13,2.194791079,6.74807432154978E-13));
#121151=CARTESIAN_POINT('',(6.08514101776743,2.01370168035776,-4.3841827961962));
#121152=CARTESIAN_POINT('Origin',(-0.15680816817603,2.01785800931407,0.112162256881573));
#121153=CARTESIAN_POINT('',(5.7349199867538,2.10403448602304,-4.83329005408069));
#121154=CARTESIAN_POINT('Origin',(-0.163103671603423,1.87510627865103,0.0902292551797146));
#121155=CARTESIAN_POINT('Origin',(-0.135768119198344,2.01789496108694,0.13249216721638));
#121156=CARTESIAN_POINT('Ctrl Pts',(5.880804839,2.233426833,-4.240121985));
#121157=CARTESIAN_POINT('Ctrl Pts',(5.650760595,2.169174758,-4.559180094));
#121158=CARTESIAN_POINT('Ctrl Pts',(5.38754780300001,2.104034486,-4.851476957));
#121159=CARTESIAN_POINT('Ctrl Pts',(6.224170392,2.233426833,-4.184459694));
#121160=CARTESIAN_POINT('Ctrl Pts',(5.997146059,2.169174758,-4.522146811));
#121161=CARTESIAN_POINT('Ctrl Pts',(5.734919982,2.104034486,-4.83329006));
#121162=CARTESIAN_POINT('',(5.56123389752302,2.10403448477417,-4.84238350273132));
#121163=CARTESIAN_POINT('Ctrl Pts',(5.39286432943003,2.10273945758871,-4.84557297336042));
#121164=CARTESIAN_POINT('Ctrl Pts',(5.39020606621502,2.10338697179435,-4.84852496518022));
#121165=CARTESIAN_POINT('Ctrl Pts',(5.387547803,2.104034486,-4.851476957));
#121166=CARTESIAN_POINT('Ctrl Pts',(5.30758067,2.123513315,-4.940280173));
#121167=CARTESIAN_POINT('Ctrl Pts',(5.224730277,2.142857143,-5.026399659));
#121168=CARTESIAN_POINT('Ctrl Pts',(5.032133918,2.18782435,-5.22659544400001));
#121169=CARTESIAN_POINT('Ctrl Pts',(4.82478297,2.233445087,-5.411466464));
#121170=CARTESIAN_POINT('Ctrl Pts',(5.41143189778815,2.10273945758871,-5.19292522215096));
#121171=CARTESIAN_POINT('Ctrl Pts',(5.40858329939408,2.10338697179435,-5.19588717907548));
#121172=CARTESIAN_POINT('Ctrl Pts',(5.405734701,2.104034486,-5.198849136));
#121173=CARTESIAN_POINT('Ctrl Pts',(5.320041815,2.123513315,-5.28795212699999));
#121174=CARTESIAN_POINT('Ctrl Pts',(5.2314589,2.142857143,-5.374182522));
#121175=CARTESIAN_POINT('Ctrl Pts',(5.02553655899999,2.18782435,-5.574636127));
#121176=CARTESIAN_POINT('Ctrl Pts',(4.804878973,2.233445087,-5.758744486));
#121177=CARTESIAN_POINT('',(5.40573470643701,2.10403448602284,-5.19884913028904));
#121178=CARTESIAN_POINT('',(4.9948541657922,2.19371102276988,-5.59476825811766));
#121179=CARTESIAN_POINT('Ctrl Pts',(5.40573470628783,2.10403448479508,-5.19884913024064));
#121180=CARTESIAN_POINT('Ctrl Pts',(5.34851555915554,2.11704095516575,-5.25834528453067));
#121181=CARTESIAN_POINT('Ctrl Pts',(5.29040470290504,2.12998516342573,-5.31680215845702));
#121182=CARTESIAN_POINT('Ctrl Pts',(5.23145889897971,2.14285714322178,-5.37418252274678));
#121183=CARTESIAN_POINT('Ctrl Pts',(5.15436406791138,2.15969232103608,-5.44922992492733));
#121184=CARTESIAN_POINT('Ctrl Pts',(5.07546648035821,2.17665108709335,-5.52279981598171));
#121185=CARTESIAN_POINT('Ctrl Pts',(4.99485416557968,2.1937110229587,-5.59476825821744));
#121186=CARTESIAN_POINT('Ctrl Pts',(4.82833188497325,2.2326640750528,-5.40830021369509));
#121187=CARTESIAN_POINT('Ctrl Pts',(4.85596119964846,2.22584954915282,-5.43940824552606));
#121188=CARTESIAN_POINT('Ctrl Pts',(4.88367106275028,2.21920123117121,-5.47051637100757));
#121189=CARTESIAN_POINT('Ctrl Pts',(4.93917214762191,2.2062273950432,-5.53266010496482));
#121190=CARTESIAN_POINT('Ctrl Pts',(4.96699530202773,2.1998944130555,-5.56373145926826));
#121191=CARTESIAN_POINT('Ctrl Pts',(4.9948541663831,2.1937110227882,-5.59476825759091));
#121192=CARTESIAN_POINT('',(5.39664125752638,2.10403448732041,-5.02516304056509));
#121193=CARTESIAN_POINT('Origin',(2.53703308361608E-13,2.19479107899989,
-1.61762964134837E-13));
#121194=CARTESIAN_POINT('',(5.00040409668657,2.01370168037898,-5.58980848202957));
#121195=CARTESIAN_POINT('Origin',(-0.129030496864432,2.01785801116634,0.143249073428582));
#121196=CARTESIAN_POINT('',(4.56182625396996,2.10403448602304,-5.95312869231247));
#121197=CARTESIAN_POINT('Origin',(-0.139893566805733,1.87510629126109,0.123181968685396));
#121198=CARTESIAN_POINT('Origin',(-0.104112042392351,2.01789493571883,0.158580727431307));
#121199=CARTESIAN_POINT('Ctrl Pts',(4.831814,2.233426833,-5.405189494));
#121200=CARTESIAN_POINT('Ctrl Pts',(4.538560001,2.169174758,-5.667335489));
#121201=CARTESIAN_POINT('Ctrl Pts',(4.218665792,2.104034486,-5.896215645));
#121202=CARTESIAN_POINT('Ctrl Pts',(5.179117605,2.233426833,-5.424642001));
#121203=CARTESIAN_POINT('Ctrl Pts',(4.884808226,2.169174758,-5.70563066));
#121204=CARTESIAN_POINT('Ctrl Pts',(4.561826248,2.104034486,-5.953128697));
#121205=CARTESIAN_POINT('',(4.39024602614564,2.10403448477417,-5.92467216644601));
#121206=CARTESIAN_POINT('Ctrl Pts',(4.2251272029383,2.10273945758871,-5.89159258926902));
#121207=CARTESIAN_POINT('Ctrl Pts',(4.22189649746915,2.10338697179435,-5.89390411713451));
#121208=CARTESIAN_POINT('Ctrl Pts',(4.218665792,2.104034486,-5.896215645));
#121209=CARTESIAN_POINT('Ctrl Pts',(4.12147818,2.123513315,-5.965752121));
#121210=CARTESIAN_POINT('Ctrl Pts',(4.022051639,2.142857143,-6.032047796));
#121211=CARTESIAN_POINT('Ctrl Pts',(3.7909219,2.18782435,-6.186160591));
#121212=CARTESIAN_POINT('Ctrl Pts',(3.548676898,2.233445087,-6.322135104));
#121213=CARTESIAN_POINT('Ctrl Pts',(4.16859020585149,2.10273945758871,-6.2348154138769));
#121214=CARTESIAN_POINT('Ctrl Pts',(4.16517147292575,2.10338697179435,-6.23709575743844));
#121215=CARTESIAN_POINT('Ctrl Pts',(4.16175274,2.104034486,-6.239376101));
#121216=CARTESIAN_POINT('Ctrl Pts',(4.058908797,2.123513315,-6.307974476));
#121217=CARTESIAN_POINT('Ctrl Pts',(3.953859916,2.142857143,-6.373146144));
#121218=CARTESIAN_POINT('Ctrl Pts',(3.709660325,2.18782435,-6.52464603900001));
#121219=CARTESIAN_POINT('Ctrl Pts',(3.454583735,2.233445087,-6.657015188));
#121220=CARTESIAN_POINT('',(4.16175274651115,2.10403448602285,-6.23937609655172));
#121221=CARTESIAN_POINT('',(3.67536745575486,2.19371102277769,-6.53771168431448));
#121222=CARTESIAN_POINT('Ctrl Pts',(4.1617527464023,2.10403448479508,-6.23937609651201));
#121223=CARTESIAN_POINT('Ctrl Pts',(4.093081436751,2.11704095516575,-6.28518083842335));
#121224=CARTESIAN_POINT('Ctrl Pts',(4.02376268037025,2.12998516342593,-6.32977890670614));
#121225=CARTESIAN_POINT('Ctrl Pts',(3.9538599145795,2.14285714327501,-6.37314614456156));
#121226=CARTESIAN_POINT('Ctrl Pts',(3.86243454430784,2.15969232116114,-6.42986587055072));
#121227=CARTESIAN_POINT('Ctrl Pts',(3.76956618710414,2.17665108709805,-6.48475508920061));
#121228=CARTESIAN_POINT('Ctrl Pts',(3.67536745552681,2.19371102296706,-6.5377116843956));
#121229=CARTESIAN_POINT('Ctrl Pts',(3.55282349131177,2.23266407508749,-6.31980579090035));
#121230=CARTESIAN_POINT('Ctrl Pts',(3.57311955964696,2.2258495427368,-6.35612605452519));
#121231=CARTESIAN_POINT('Ctrl Pts',(3.5934942760525,2.21920121809161,-6.39246372980776));
#121232=CARTESIAN_POINT('Ctrl Pts',(3.63433866877511,2.20622739519198,-6.46508559643128));
#121233=CARTESIAN_POINT('Ctrl Pts',(3.65483191001531,2.19989441336666,-6.50141167452851));
#121234=CARTESIAN_POINT('Ctrl Pts',(3.67536745646046,2.19371102279552,-6.53771168391835));
#121235=CARTESIAN_POINT('',(4.19020927267301,2.10403448732041,-6.06779586839186));
#121236=CARTESIAN_POINT('Origin',(8.17054757185076E-13,2.194791079,-1.56038376664114E-12));
#121237=CARTESIAN_POINT('',(3.68185383757781,2.01370168038203,-6.53406093588962));
#121238=CARTESIAN_POINT('Origin',(-0.0952194678829571,2.0178580037239,0.167637656801262));
#121239=CARTESIAN_POINT('',(3.17542659582,2.10403448602304,-6.79460564966676));
#121240=CARTESIAN_POINT('Origin',(-0.110142518719101,1.87510629248459,0.150375150613581));
#121241=CARTESIAN_POINT('Origin',(-0.0675876867919295,2.01789496007953,
0.177253998031647));
#121242=CARTESIAN_POINT('Ctrl Pts',(3.556892909,2.233426833,-6.31751635));
#121243=CARTESIAN_POINT('Ctrl Pts',(3.214141385,2.169174758,-6.510492576));
#121244=CARTESIAN_POINT('Ctrl Pts',(2.852523658,2.104034486,-6.665253842));
#121245=CARTESIAN_POINT('Ctrl Pts',(3.891895034,2.233426833,-6.411174077));
#121246=CARTESIAN_POINT('Ctrl Pts',(3.54406219,2.169174758,-6.622325561));
#121247=CARTESIAN_POINT('Ctrl Pts',(3.175426589,2.104034486,-6.794605653));
#121248=CARTESIAN_POINT('',(3.01397513048093,2.10403448477417,-6.72992974437362));
#121249=CARTESIAN_POINT('Ctrl Pts',(2.85982782510034,2.10273945758871,-6.66212788310327));
#121250=CARTESIAN_POINT('Ctrl Pts',(2.85617574155017,2.10338697179435,-6.66369086255163));
#121251=CARTESIAN_POINT('Ctrl Pts',(2.852523658,2.104034486,-6.66525384200001));
#121252=CARTESIAN_POINT('Ctrl Pts',(2.742659951,2.123513315,-6.71227213));
#121253=CARTESIAN_POINT('Ctrl Pts',(2.631306337,2.142857143,-6.755644082));
#121254=CARTESIAN_POINT('Ctrl Pts',(2.372450588,2.18782435,-6.856467744));
#121255=CARTESIAN_POINT('Ctrl Pts',(2.106638638,2.233445087,-6.937187734));
#121256=CARTESIAN_POINT('Ctrl Pts',(2.73082986964227,2.10273945758871,-6.98517256627893));
#121257=CARTESIAN_POINT('Ctrl Pts',(2.72700085832114,2.10338697179435,-6.98666467013946));
#121258=CARTESIAN_POINT('Ctrl Pts',(2.723171847,2.104034486,-6.98815677400001));
#121259=CARTESIAN_POINT('Ctrl Pts',(2.607985715,2.123513315,-7.033042949));
#121260=CARTESIAN_POINT('Ctrl Pts',(2.491382836,2.142857143,-7.074108535));
#121261=CARTESIAN_POINT('Ctrl Pts',(2.220324497,2.18782435,-7.169570753));
#121262=CARTESIAN_POINT('Ctrl Pts',(1.942756002,2.233445087,-7.244011259));
#121263=CARTESIAN_POINT('',(2.72317185035002,2.10403448644945,-6.98815677381845));
#121264=CARTESIAN_POINT('',(2.18402464846601,2.19371102276864,-7.17495897777774));
#121265=CARTESIAN_POINT('Ctrl Pts',(2.72317184977156,2.1040344855469,-6.98815677272572));
#121266=CARTESIAN_POINT('Ctrl Pts',(2.6462593728704,2.11704095566462,-7.0181283226553));
#121267=CARTESIAN_POINT('Ctrl Pts',(2.56897398538449,2.12998516367377,-7.04678222845144));
#121268=CARTESIAN_POINT('Ctrl Pts',(2.4913828346596,2.14285714322954,-7.07410853538889));
#121269=CARTESIAN_POINT('Ctrl Pts',(2.38990187464735,2.15969232105421,-7.10984843377403));
#121270=CARTESIAN_POINT('Ctrl Pts',(2.28740516825367,2.17665108710236,-7.14349042110731));
#121271=CARTESIAN_POINT('Ctrl Pts',(2.18402464850465,2.19371102292762,-7.17495897781848));
#121272=CARTESIAN_POINT('Ctrl Pts',(2.11118901954595,2.2326640751888,-6.93580427336281));
#121273=CARTESIAN_POINT('Ctrl Pts',(2.12320280378213,2.22584953741119,-6.97563847567611));
#121274=CARTESIAN_POINT('Ctrl Pts',(2.13528965577598,2.21920120713672,-7.01550659406681));
#121275=CARTESIAN_POINT('Ctrl Pts',(2.15956758010625,2.20622738131793,-7.09521095647696));
#121276=CARTESIAN_POINT('Ctrl Pts',(2.17177269769327,2.19989438511491,-7.13509328890588));
#121277=CARTESIAN_POINT('Ctrl Pts',(2.18402464940508,2.19371102278408,-7.17495897749153));
#121278=CARTESIAN_POINT('',(2.78784776000761,2.10403448732041,-6.82670530493409));
#121279=CARTESIAN_POINT('Origin',(1.07444435293313E-13,2.19479107900022,
-2.87096735274162E-13));
#121280=CARTESIAN_POINT('',(2.1911441852037,2.01370168036753,-7.1727879625103));
#121281=CARTESIAN_POINT('Origin',(-0.0569562509952645,2.01785797429459,
0.184188081689782));
#121282=CARTESIAN_POINT('',(1.64054751841348,2.10403448602304,-7.31837439837307));
#121283=CARTESIAN_POINT('Origin',(-0.0752411761825214,1.87510627598791,
0.17053664232371));
#121284=CARTESIAN_POINT('Origin',(-0.0279031774344973,2.01789493616642,
0.187639359023223));
#121285=CARTESIAN_POINT('Ctrl Pts',(2.115655458,2.233426833,-6.934443163));
#121286=CARTESIAN_POINT('Ctrl Pts',(1.739433091,2.169174758,-7.049226266));
#121287=CARTESIAN_POINT('Ctrl Pts',(1.353000687,2.104034486,-7.122632178));
#121288=CARTESIAN_POINT('Ctrl Pts',(2.422691778,2.233426833,-7.097926778));
#121289=CARTESIAN_POINT('Ctrl Pts',(2.037599744,2.169174758,-7.229367878));
#121290=CARTESIAN_POINT('Ctrl Pts',(1.640547511,2.104034486,-7.3183744));
#121291=CARTESIAN_POINT('',(1.49677410648981,2.10403448477417,-7.22050328744741));
#121292=CARTESIAN_POINT('Ctrl Pts',(1.36080607551578,2.10273945758871,-7.12114948230861));
#121293=CARTESIAN_POINT('Ctrl Pts',(1.35690338125789,2.10338697179435,-7.12189083015431));
#121294=CARTESIAN_POINT('Ctrl Pts',(1.353000687,2.104034486,-7.12263217800001));
#121295=CARTESIAN_POINT('Ctrl Pts',(1.23559799,2.123513315,-7.144933755));
#121296=CARTESIAN_POINT('Ctrl Pts',(1.117524075,2.142857143,-7.163353959));
#121297=CARTESIAN_POINT('Ctrl Pts',(0.843046122000001,2.18782435,-7.206174085));
#121298=CARTESIAN_POINT('Ctrl Pts',(0.566096296,2.233445087,-7.227865175));
#121299=CARTESIAN_POINT('Ctrl Pts',(1.16537896377316,2.10273945758871,-7.40891081180722));
#121300=CARTESIAN_POINT('Ctrl Pts',(1.16131871438658,2.10338697179435,-7.40954490690361));
#121301=CARTESIAN_POINT('Ctrl Pts',(1.157258465,2.104034486,-7.410179002));
#121302=CARTESIAN_POINT('Ctrl Pts',(1.03511612,2.123513315,-7.429254151));
#121303=CARTESIAN_POINT('Ctrl Pts',(0.912411464,2.142857143,-7.444293474));
#121304=CARTESIAN_POINT('Ctrl Pts',(0.627168763000001,2.18782435,-7.47925430800001));
#121305=CARTESIAN_POINT('Ctrl Pts',(0.340087157,2.233445087,-7.492285414));
#121306=CARTESIAN_POINT('',(1.15725847007385,2.10403448645287,-7.41017900172129));
#121307=CARTESIAN_POINT('',(0.59055927596526,2.19371102275364,-7.47671316452157));
#121308=CARTESIAN_POINT('Ctrl Pts',(1.15725847269504,2.10403448479508,-7.41017900061506));
#121309=CARTESIAN_POINT('Ctrl Pts',(1.07570116794104,2.11704095516578,-7.42291592453183));
#121310=CARTESIAN_POINT('Ctrl Pts',(0.994062925427622,2.12998516342565,
-7.43428584478598));
#121311=CARTESIAN_POINT('Ctrl Pts',(0.91241146271857,2.14285714320201,-7.44429347415706));
#121312=CARTESIAN_POINT('Ctrl Pts',(0.805620049540351,2.15969232098381,
-7.4573823870384));
#121313=CARTESIAN_POINT('Ctrl Pts',(0.698287626122133,2.17665108708032,
-7.46820408109766));
#121314=CARTESIAN_POINT('Ctrl Pts',(0.590559275733128,2.19371102293932,
-7.47671316449973));
#121315=CARTESIAN_POINT('Ctrl Pts',(0.570837695248524,2.23266407508929,
-7.22749225713458));
#121316=CARTESIAN_POINT('Ctrl Pts',(0.574007422813354,2.22584954795846,
-7.26897770171532));
#121317=CARTESIAN_POINT('Ctrl Pts',(0.577241217928545,2.21920122871194,
-7.31051196769929));
#121318=CARTESIAN_POINT('Ctrl Pts',(0.583817460117917,2.20622739501542,
-7.3935719730685));
#121319=CARTESIAN_POINT('Ctrl Pts',(0.58716369802571,2.19989441300601,-7.43514551846265));
#121320=CARTESIAN_POINT('Ctrl Pts',(0.590559276757404,2.19371102277163,
-7.47671316445954));
#121321=CARTESIAN_POINT('',(1.25512958399116,2.10403448732041,-7.26640558861968));
#121322=CARTESIAN_POINT('Origin',(-1.06953156183906E-13,2.19479107900022,
-1.30104260698261E-15));
#121323=CARTESIAN_POINT('',(0.597979065930106,2.01370168036969,-7.47612339603309));
#121324=CARTESIAN_POINT('Origin',(-0.0160296328144827,2.01785795518985,
0.192125553256562));
#121325=CARTESIAN_POINT('',(0.0289582635899551,2.10403448602304,-7.4999440940205));
#121326=CARTESIAN_POINT('Origin',(-0.0368217379804399,1.87510631679366,
0.18272430212099));
#121327=CARTESIAN_POINT('Origin',(0.0130861037075583,2.01789498920075,0.189250678432509));
#121328=CARTESIAN_POINT('Ctrl Pts',(0.57549231,2.233426833,-7.227123121));
#121329=CARTESIAN_POINT('Ctrl Pts',(0.183390838,2.169174758,-7.258345971));
#121330=CARTESIAN_POINT('Ctrl Pts',(-0.209787092,2.104034486,-7.246964149));
#121331=CARTESIAN_POINT('Ctrl Pts',(0.840206146,2.233426833,-7.452788313));
#121332=CARTESIAN_POINT('Ctrl Pts',(0.4358614,2.169174758,-7.498372989));
#121333=CARTESIAN_POINT('Ctrl Pts',(0.028958256,2.104034486,-7.499944094));
#121334=CARTESIAN_POINT('',(-0.0904144103515404,2.10403448477418,-7.37345412159379));
#121335=CARTESIAN_POINT('Ctrl Pts',(-0.201845453451927,2.10273945758871,
-7.24719404571963));
#121336=CARTESIAN_POINT('Ctrl Pts',(-0.205816272725964,2.10338697179435,
-7.24707909735982));
#121337=CARTESIAN_POINT('Ctrl Pts',(-0.209787092,2.104034486,-7.246964149));
#121338=CARTESIAN_POINT('Ctrl Pts',(-0.329239158,2.123513315,-7.24350621800001));
#121339=CARTESIAN_POINT('Ctrl Pts',(-0.448512371,2.142857143,-7.236113367));
#121340=CARTESIAN_POINT('Ctrl Pts',(-0.725778243,2.18782435,-7.21892773600001));
#121341=CARTESIAN_POINT('Ctrl Pts',(-1.000916079,2.233445087,-7.180575673));
#121342=CARTESIAN_POINT('Ctrl Pts',(-0.454563767573315,2.10273945758871,
-7.48621662364792));
#121343=CARTESIAN_POINT('Ctrl Pts',(-0.458665402286658,2.10338697179435,
-7.48596306032396));
#121344=CARTESIAN_POINT('Ctrl Pts',(-0.462767037,2.104034486,-7.48570949700001));
#121345=CARTESIAN_POINT('Ctrl Pts',(-0.586154355,2.123513315,-7.478081685));
#121346=CARTESIAN_POINT('Ctrl Pts',(-0.709223254,2.142857143,-7.466391523));
#121347=CARTESIAN_POINT('Ctrl Pts',(-0.995312685000001,2.18782435,-7.439216243));
#121348=CARTESIAN_POINT('Ctrl Pts',(-1.278483785,2.233445087,-7.39022863000001));
#121349=CARTESIAN_POINT('',(-0.462767031955311,2.10403448645287,-7.48570949779066));
#121350=CARTESIAN_POINT('',(-1.03051999194114,2.19371102277752,-7.42886455274631));
#121351=CARTESIAN_POINT('Ctrl Pts',(-0.462767029187143,2.10403448479507,
-7.48570949730166));
#121352=CARTESIAN_POINT('Ctrl Pts',(-0.545155631601333,2.11704095516578,
-7.48061622867985));
#121353=CARTESIAN_POINT('Ctrl Pts',(-0.627329414052753,2.12998516342569,
-7.47417051724953));
#121354=CARTESIAN_POINT('Ctrl Pts',(-0.709223255345179,2.14285714321143,
-7.46639152287222));
#121355=CARTESIAN_POINT('Ctrl Pts',(-0.816331674104039,2.15969232101307,
-7.45621742708153));
#121356=CARTESIAN_POINT('Ctrl Pts',(-0.923481069260558,2.17665108708536,
-7.44371281763971));
#121357=CARTESIAN_POINT('Ctrl Pts',(-1.030519991955,2.19371102293018,-7.42886455253598));
#121358=CARTESIAN_POINT('Ctrl Pts',(-0.996205364718836,2.23266407509814,
-7.1812307344084));
#121359=CARTESIAN_POINT('Ctrl Pts',(-1.00202789610967,2.2258495383401,-7.2224277285144));
#121360=CARTESIAN_POINT('Ctrl Pts',(-1.00779835385358,2.21920120912754,
-7.26368618337483));
#121361=CARTESIAN_POINT('Ctrl Pts',(-1.01923129090295,2.2062273932737,-7.34621787628459));
#121362=CARTESIAN_POINT('Ctrl Pts',(-1.02490037136756,2.19989440942399,
-7.38753881040581));
#121363=CARTESIAN_POINT('Ctrl Pts',(-1.03051999137907,2.19371102280297,
-7.42886455282655));
#121364=CARTESIAN_POINT('',(-0.336277056398938,2.10403448732041,-7.36633682336982));
#121365=CARTESIAN_POINT('Origin',(4.82741017299171E-14,2.19479107899978,
2.63677968348475E-13));
#121366=CARTESIAN_POINT('',(-1.02314689010353,2.01370168036372,-7.42988360835676));
#121367=CARTESIAN_POINT('Origin',(0.025646473847156,2.0178579822224,0.19107986823753));
#121368=CARTESIAN_POINT('',(-1.58398504857694,2.10403448602304,-7.3308247395824));
#121369=CARTESIAN_POINT('Origin',(0.00331945828723729,1.8751062980361,0.186367960182877));
#121370=CARTESIAN_POINT('Origin',(0.0534634732188782,2.01789498208132,0.182013091687114));
#121371=CARTESIAN_POINT('Ctrl Pts',(-0.991580219,2.233426833,-7.181870833));
#121372=CARTESIAN_POINT('Ctrl Pts',(-1.381226566,2.169174758,-7.128073485));
#121373=CARTESIAN_POINT('Ctrl Pts',(-1.76276546,2.104034486,-7.032436131));
#121374=CARTESIAN_POINT('Ctrl Pts',(-0.781566591,2.233426833,-7.459165749));
#121375=CARTESIAN_POINT('Ctrl Pts',(-1.18625734,2.169174758,-7.416762512));
#121376=CARTESIAN_POINT('Ctrl Pts',(-1.583985056,2.104034486,-7.330824738));
#121377=CARTESIAN_POINT('',(-1.67337525055052,2.10403448477417,-7.18163043623579));
#121378=CARTESIAN_POINT('Ctrl Pts',(-1.75505891355549,2.10273945758871,
-7.03436787041624));
#121379=CARTESIAN_POINT('Ctrl Pts',(-1.75891218677774,2.10338697179435,
-7.03340200070812));
#121380=CARTESIAN_POINT('Ctrl Pts',(-1.76276546,2.104034486,-7.032436131));
#121381=CARTESIAN_POINT('Ctrl Pts',(-1.87868145,2.123513315,-7.003380381));
#121382=CARTESIAN_POINT('Ctrl Pts',(-1.993576877,2.142857143,-6.970520155));
#121383=CARTESIAN_POINT('Ctrl Pts',(-2.260666024,2.18782435,-6.894132348));
#121384=CARTESIAN_POINT('Ctrl Pts',(-2.521126731,2.233445087,-6.797530434));
#121385=CARTESIAN_POINT('Ctrl Pts',(-2.05325160269057,2.10273945758871,
-7.21347526574446));
#121386=CARTESIAN_POINT('Ctrl Pts',(-2.05720283484529,2.10338697179435,
-7.21234590037223));
#121387=CARTESIAN_POINT('Ctrl Pts',(-2.061154067,2.104034486,-7.211216535));
#121388=CARTESIAN_POINT('Ctrl Pts',(-2.180016904,2.123513315,-7.177242431));
#121389=CARTESIAN_POINT('Ctrl Pts',(-2.297695481,2.142857143,-7.139369403));
#121390=CARTESIAN_POINT('Ctrl Pts',(-2.571254418,2.18782435,-7.05132869600001));
#121391=CARTESIAN_POINT('Ctrl Pts',(-2.837274247,2.233445087,-6.94261297));
#121392=CARTESIAN_POINT('',(-2.06115405937038,2.10403448602285,-7.2112165369986));
#121393=CARTESIAN_POINT('',(-2.6034132904615,2.19371102279527,-7.03365049153161));
#121394=CARTESIAN_POINT('Ctrl Pts',(-2.06115405943465,2.10403448479507,
-7.21121653697413));
#121395=CARTESIAN_POINT('Ctrl Pts',(-2.14052155993136,2.11704095516577,
-7.18853123205384));
#121396=CARTESIAN_POINT('Ctrl Pts',(-2.2193885275124,2.12998516342558,-7.16457128357355));
#121397=CARTESIAN_POINT('Ctrl Pts',(-2.29769548211535,2.14285714318334,
-7.13936940264104));
#121398=CARTESIAN_POINT('Ctrl Pts',(-2.40011263545933,2.15969232095406,
-7.10640802805374));
#121399=CARTESIAN_POINT('Ctrl Pts',(-2.50206881644122,2.17665108712062,
-7.07116181681474));
#121400=CARTESIAN_POINT('Ctrl Pts',(-2.60341329084455,2.19371102302222,
-7.03365049150481));
#121401=CARTESIAN_POINT('Ctrl Pts',(-2.51666696932107,2.23266407506185,
-6.79918284486745));
#121402=CARTESIAN_POINT('Ctrl Pts',(-2.53120951025225,2.22584953775784,
-6.8381650071174));
#121403=CARTESIAN_POINT('Ctrl Pts',(-2.54571440735249,2.21920120797771,
-6.87721838802777));
#121404=CARTESIAN_POINT('Ctrl Pts',(-2.57462194694882,2.20622738131974,
-6.95536285752602));
#121405=CARTESIAN_POINT('Ctrl Pts',(-2.58904129656605,2.19989438514245,
-6.99449912828361));
#121406=CARTESIAN_POINT('Ctrl Pts',(-2.60341328946789,2.19371102281277,
-7.03365049189911));
#121407=CARTESIAN_POINT('',(-1.91195975566783,2.10403448732041,-7.12182633510266));
#121408=CARTESIAN_POINT('Origin',(3.30247981739085E-13,2.19479107899967,
1.03172678733721E-12));
#121409=CARTESIAN_POINT('',(-2.59643163431786,2.01370168038089,-7.03623072141384));
#121410=CARTESIAN_POINT('Origin',(0.0661234049200093,2.01785800203912,0.181099350435265));
#121411=CARTESIAN_POINT('',(-3.12286297908654,2.10403448602304,-6.81892416813213));
#121412=CARTESIAN_POINT('Origin',(0.0433053581726939,1.87510630668807,0.181296946708333));
#121413=CARTESIAN_POINT('Origin',(0.0913409759321476,2.01789493322103,0.166264684052931));
#121414=CARTESIAN_POINT('Ctrl Pts',(-2.512287559,2.233426833,-6.800802248));
#121415=CARTESIAN_POINT('Ctrl Pts',(-2.881259352,2.169174758,-6.664500205));
#121416=CARTESIAN_POINT('Ctrl Pts',(-3.233318874,2.104034486,-6.489079215));
#121417=CARTESIAN_POINT('Ctrl Pts',(-2.366794143,2.233426833,-7.116760884));
#121418=CARTESIAN_POINT('Ctrl Pts',(-2.752908005,2.169174758,-6.988352463));
#121419=CARTESIAN_POINT('Ctrl Pts',(-3.122862986,2.104034486,-6.81892416500001));
#121420=CARTESIAN_POINT('',(-3.17809092309783,2.10403448477417,-6.65400169329663));
#121421=CARTESIAN_POINT('Ctrl Pts',(-3.22620776921482,2.10273945758871,
-6.49262247109658));
#121422=CARTESIAN_POINT('Ctrl Pts',(-3.22976332160741,2.10338697179435,
-6.4908508430483));
#121423=CARTESIAN_POINT('Ctrl Pts',(-3.233318874,2.104034486,-6.489079215));
#121424=CARTESIAN_POINT('Ctrl Pts',(-3.340278685,2.123513315,-6.435784261));
#121425=CARTESIAN_POINT('Ctrl Pts',(-3.445423944,2.142857143,-6.378993169));
#121426=CARTESIAN_POINT('Ctrl Pts',(-3.689847575,2.18782435,-6.246974995));
#121427=CARTESIAN_POINT('Ctrl Pts',(-3.923452299,2.233445087,-6.096640227));
#121428=CARTESIAN_POINT('Ctrl Pts',(-3.5559316742459,2.10273945758871,-6.60343982105814));
#121429=CARTESIAN_POINT('Ctrl Pts',(-3.55954774862295,2.10338697179435,
-6.60148746152907));
#121430=CARTESIAN_POINT('Ctrl Pts',(-3.563163823,2.104034486,-6.599535102));
#121431=CARTESIAN_POINT('Ctrl Pts',(-3.671944285,2.123513315,-6.540803298));
#121432=CARTESIAN_POINT('Ctrl Pts',(-3.778730021,2.142857143,-6.478518305));
#121433=CARTESIAN_POINT('Ctrl Pts',(-4.026967153,2.18782435,-6.333728855));
#121434=CARTESIAN_POINT('Ctrl Pts',(-4.263396918,2.233445087,-6.170368443));
#121435=CARTESIAN_POINT('',(-3.56316381608928,2.10403448602284,-6.59953510579737));
#121436=CARTESIAN_POINT('',(-4.0545738770561,2.19371102273927,-6.30955075083422));
#121437=CARTESIAN_POINT('Ctrl Pts',(-3.56316381603591,2.10403448479508,
-6.5995351055543));
#121438=CARTESIAN_POINT('Ctrl Pts',(-3.63579907860376,2.11704095516575,
-6.56031850441903));
#121439=CARTESIAN_POINT('Ctrl Pts',(-3.7076714997741,2.1299851634257,-6.51996465977361));
#121440=CARTESIAN_POINT('Ctrl Pts',(-3.77873002219237,2.14285714321599,
-6.47851830430452));
#121441=CARTESIAN_POINT('Ctrl Pts',(-3.87166699851752,2.15969232101281,
-6.42431088745251));
#121442=CARTESIAN_POINT('Ctrl Pts',(-3.96366260665177,2.17665108707702,
-6.36797114815556));
#121443=CARTESIAN_POINT('Ctrl Pts',(-4.05457387729845,2.19371102294006,
-6.3095507506677));
#121444=CARTESIAN_POINT('Ctrl Pts',(-3.91945202306782,2.23266407511321,
-6.09921272201927));
#121445=CARTESIAN_POINT('Ctrl Pts',(-3.94203458296659,2.22584953691232,
-6.13415729112328));
#121446=CARTESIAN_POINT('Ctrl Pts',(-3.96459568950821,2.2192012061956,-6.16917950680068));
#121447=CARTESIAN_POINT('Ctrl Pts',(-4.00962608213548,2.20622739562724,
-6.23928264841866));
#121448=CARTESIAN_POINT('Ctrl Pts',(-4.03212140082664,2.19989441423173,
-6.27440411284586));
#121449=CARTESIAN_POINT('Ctrl Pts',(-4.05457387632248,2.19371102275467,
-6.30955075130558));
#121450=CARTESIAN_POINT('',(-3.39824134130296,2.10403448732041,-6.54430716223719));
#121451=CARTESIAN_POINT('Origin',(8.03393809811759E-13,2.19479107900055,
1.33096658694321E-12));
#121452=CARTESIAN_POINT('',(-4.04831012106117,2.01370168036841,-6.31357150582532));
#121453=CARTESIAN_POINT('Origin',(0.103508509358519,2.0178580184687,0.162650835382203));
#121454=CARTESIAN_POINT('',(-4.51571930876562,2.10403448602304,-5.98817828133842));
#121455=CARTESIAN_POINT('Origin',(0.0812663913473916,1.87510629006869,0.167748984339933));
#121456=CARTESIAN_POINT('Origin',(0.124947457768929,2.01789494613023,0.14274189675082));
#121457=CARTESIAN_POINT('Ctrl Pts',(-3.915523125,2.233426833,-6.101735708));
#121458=CARTESIAN_POINT('Ctrl Pts',(-4.246567652,2.169174758,-5.889302302));
#121459=CARTESIAN_POINT('Ctrl Pts',(-4.552685891,2.104034486,-5.642300168));
#121460=CARTESIAN_POINT('Ctrl Pts',(-3.841353031,2.233426833,-6.441584191));
#121461=CARTESIAN_POINT('Ctrl Pts',(-4.190835751,2.169174758,-6.233174821));
#121462=CARTESIAN_POINT('Ctrl Pts',(-4.515719315,2.104034486,-5.988178277));
#121463=CARTESIAN_POINT('',(-4.53420259696787,2.10403448477417,-5.81523922720332));
#121464=CARTESIAN_POINT('Ctrl Pts',(-4.54650273517165,2.10273945758871,
-5.64728926211416));
#121465=CARTESIAN_POINT('Ctrl Pts',(-4.54959431308582,2.10338697179435,
-5.64479471505708));
#121466=CARTESIAN_POINT('Ctrl Pts',(-4.552685891,2.104034486,-5.64230016800001));
#121467=CARTESIAN_POINT('Ctrl Pts',(-4.645688202,2.123513315,-5.567258022));
#121468=CARTESIAN_POINT('Ctrl Pts',(-4.736166816,2.142857143,-5.489191552));
#121469=CARTESIAN_POINT('Ctrl Pts',(-4.946495953,2.18782435,-5.30771603400001));
#121470=CARTESIAN_POINT('Ctrl Pts',(-5.142321598,2.233445087,-5.110677899));
#121471=CARTESIAN_POINT('Ctrl Pts',(-4.89234033307211,2.10273945758871,
-5.6846348711734));
#121472=CARTESIAN_POINT('Ctrl Pts',(-4.89545216603606,2.10338697179435,
-5.6819508075867));
#121473=CARTESIAN_POINT('Ctrl Pts',(-4.898563999,2.104034486,-5.679266744));
#121474=CARTESIAN_POINT('Ctrl Pts',(-4.992175632,2.123513315,-5.598523472));
#121475=CARTESIAN_POINT('Ctrl Pts',(-5.083075345,2.142857143,-5.514738891));
#121476=CARTESIAN_POINT('Ctrl Pts',(-5.29438337900001,2.18782435,-5.319970893));
#121477=CARTESIAN_POINT('Ctrl Pts',(-5.490167888,2.233445087,-5.109604345));
#121478=CARTESIAN_POINT('',(-4.89856399292584,2.10403448602284,-5.67926674903035));
#121479=CARTESIAN_POINT('',(-5.31614709538626,2.19371102275033,-5.29042342922392));
#121480=CARTESIAN_POINT('Ctrl Pts',(-4.89856399296279,2.10403448479507,
-5.67926674896828));
#121481=CARTESIAN_POINT('Ctrl Pts',(-4.9610706731201,2.11704095516573,-5.62535257504612));
#121482=CARTESIAN_POINT('Ctrl Pts',(-5.02258787329021,2.12998516342565,
-5.57049173451762));
#121483=CARTESIAN_POINT('Ctrl Pts',(-5.08307534592545,2.14285714320276,
-5.51473889011978));
#121484=CARTESIAN_POINT('Ctrl Pts',(-5.16218651501869,2.15969232098375,
-5.44182011015275));
#121485=CARTESIAN_POINT('Ctrl Pts',(-5.23991993861851,2.17665108708914,
-5.36702122616938));
#121486=CARTESIAN_POINT('Ctrl Pts',(-5.31614709572608,2.19371102297335,
-5.29042342904008));
#121487=CARTESIAN_POINT('Ctrl Pts',(-5.1389678569471,2.23266407517315,-5.11405019133426));
#121488=CARTESIAN_POINT('Ctrl Pts',(-5.16853448282782,2.22584954056946,
-5.14332317738498));
#121489=CARTESIAN_POINT('Ctrl Pts',(-5.19809684655265,2.21920121356828,
-5.17267660435743));
#121490=CARTESIAN_POINT('Ctrl Pts',(-5.25714465533372,2.20622738130656,
-5.23146066835532));
#121491=CARTESIAN_POINT('Ctrl Pts',(-5.28666419622672,2.19989438510761,
-5.26092525794062));
#121492=CARTESIAN_POINT('Ctrl Pts',(-5.31614709465043,2.1937110227668,-5.29042342996282));
#121493=CARTESIAN_POINT('',(-4.72562493877461,2.10403448732041,-5.66078346119696));
#121494=CARTESIAN_POINT('Origin',(-1.26201132877313E-13,2.19479107899967,
-2.07299455379228E-13));
#121495=CARTESIAN_POINT('',(-5.31089412610488,2.01370168037457,-5.29569670366414));
#121496=CARTESIAN_POINT('Origin',(0.136053719833905,2.0178579893417,0.136596925122779));
#121497=CARTESIAN_POINT('',(-5.69742562195829,2.10403448602304,-4.87743183267503));
#121498=CARTESIAN_POINT('Origin',(0.115427610369099,1.87510627655157,0.146357328943851));
#121499=CARTESIAN_POINT('Origin',(0.152711537184925,2.01789496111607,0.11254465378285));
#121500=CARTESIAN_POINT('Ctrl Pts',(-5.135673182,2.233426833,-5.117358788));
#121501=CARTESIAN_POINT('Ctrl Pts',(-5.413311169,2.169174758,-4.83872717));
#121502=CARTESIAN_POINT('Ctrl Pts',(-5.659174375,2.104034486,-4.531693435));
#121503=CARTESIAN_POINT('Ctrl Pts',(-5.136294521,2.233426833,-5.46520618));
#121504=CARTESIAN_POINT('Ctrl Pts',(-5.432804675,2.169174758,-5.186540851));
#121505=CARTESIAN_POINT('Ctrl Pts',(-5.697425627,2.104034486,-4.877431827));
#121506=CARTESIAN_POINT('',(-5.67829999611998,2.10403448477417,-4.70456263689009));
#121507=CARTESIAN_POINT('Ctrl Pts',(-5.65420828564301,2.10273945758871,
-4.53789508252579));
#121508=CARTESIAN_POINT('Ctrl Pts',(-5.6566913303215,2.10338697179435,-4.5347942587629));
#121509=CARTESIAN_POINT('Ctrl Pts',(-5.659174375,2.104034486,-4.531693435));
#121510=CARTESIAN_POINT('Ctrl Pts',(-5.733870501,2.123513315,-4.438412986));
#121511=CARTESIAN_POINT('Ctrl Pts',(-5.805451792,2.142857143,-4.342721438));
#121512=CARTESIAN_POINT('Ctrl Pts',(-5.971851679,2.18782435,-4.12027417));
#121513=CARTESIAN_POINT('Ctrl Pts',(-6.120741654,2.233445087,-3.885745952));
#121514=CARTESIAN_POINT('Ctrl Pts',(-5.99998859553901,2.10273945758871,
-4.50002271153911));
#121515=CARTESIAN_POINT('Ctrl Pts',(-6.00245068126951,2.10338697179435,
-4.49673244776956));
#121516=CARTESIAN_POINT('Ctrl Pts',(-6.004912767,2.104034486,-4.493442184));
#121517=CARTESIAN_POINT('Ctrl Pts',(-6.078978396,2.123513315,-4.394462911));
#121518=CARTESIAN_POINT('Ctrl Pts',(-6.149741715,2.142857143,-4.293096416));
#121519=CARTESIAN_POINT('Ctrl Pts',(-6.314240122,2.18782435,-4.057457004));
#121520=CARTESIAN_POINT('Ctrl Pts',(-6.460224709,2.233445087,-3.809920827));
#121521=CARTESIAN_POINT('',(-6.00491276435706,2.10403448645287,-4.49344218835448));
#121522=CARTESIAN_POINT('',(-6.32914318402187,2.19371102275985,-4.02392178800931));
#121523=CARTESIAN_POINT('Ctrl Pts',(-6.00491276217198,2.10403448479507,
-4.49344219014995));
#121524=CARTESIAN_POINT('Ctrl Pts',(-6.05436811763821,2.11704095516577,
-4.42735141118761));
#121525=CARTESIAN_POINT('Ctrl Pts',(-6.10265362072263,2.12998516342579,
-4.36054880719136));
#121526=CARTESIAN_POINT('Ctrl Pts',(-6.14974171586987,2.14285714323779,
-4.29309641475394));
#121527=CARTESIAN_POINT('Ctrl Pts',(-6.21132792766173,2.15969232106977,
-4.20487587204554));
#121528=CARTESIAN_POINT('Ctrl Pts',(-6.27116443763095,2.17665108708656,
-4.11511535646212));
#121529=CARTESIAN_POINT('Ctrl Pts',(-6.32914318408443,2.19371102294831,
-4.02392178778338));
#121530=CARTESIAN_POINT('Ctrl Pts',(-6.11819126499426,2.23266407510997,
-3.8897603574231));
#121531=CARTESIAN_POINT('Ctrl Pts',(-6.15335945352216,2.22584954299481,
-3.9119929986438));
#121532=CARTESIAN_POINT('Ctrl Pts',(-6.18854077009955,2.21920121859506,
-3.93430511501348));
#121533=CARTESIAN_POINT('Ctrl Pts',(-6.25884486332238,2.20622739499845,
-3.97902127689778));
#121534=CARTESIAN_POINT('Ctrl Pts',(-6.29400818557493,2.19989441296563,
-4.00145111797627));
#121535=CARTESIAN_POINT('Ctrl Pts',(-6.32914318359895,2.19371102277812,
-4.02392178867561));
#121536=CARTESIAN_POINT('',(-5.83204356603735,2.10403448732041,-4.51256781591374));
#121537=CARTESIAN_POINT('Origin',(-9.6710833785707E-14,2.19479107899956,
-6.91720986045752E-14));
#121538=CARTESIAN_POINT('',(-6.32514662437653,2.01370168036548,-4.03020100929145));
#121539=CARTESIAN_POINT('Origin',(0.162236843553594,2.0178579794846,0.104155616411823));
#121540=CARTESIAN_POINT('',(-6.61272664530214,2.10403448602304,-3.53862209262939));
#121541=CARTESIAN_POINT('Origin',(0.144191659737194,1.87510624665707,0.118122165376416));
#121542=CARTESIAN_POINT('Origin',(0.17333485522942,2.01789499684262,0.0770848752727871));
#121543=CARTESIAN_POINT('Ctrl Pts',(-6.115684868,2.233426833,-3.893699859));
#121544=CARTESIAN_POINT('Ctrl Pts',(-6.326934271,2.169174758,-3.561898533));
#121545=CARTESIAN_POINT('Ctrl Pts',(-6.501046156,2.104034486,-3.209189754));
#121546=CARTESIAN_POINT('Ctrl Pts',(-6.191068588,2.233426833,-4.233281202));
#121547=CARTESIAN_POINT('Ctrl Pts',(-6.420741691,2.169174758,-3.897389996));
#121548=CARTESIAN_POINT('Ctrl Pts',(-6.61272664900001,2.104034486,-3.538622086));
#121549=CARTESIAN_POINT('',(-6.55688639900026,2.10403448477417,-3.37390592680144));
#121550=CARTESIAN_POINT('Ctrl Pts',(-6.49752934201089,2.10273945758871,
-3.21631397286633));
#121551=CARTESIAN_POINT('Ctrl Pts',(-6.49928774900544,2.10338697179435,
-3.21275186343316));
#121552=CARTESIAN_POINT('Ctrl Pts',(-6.50104615600001,2.104034486,-3.209189754));
#121553=CARTESIAN_POINT('Ctrl Pts',(-6.553943388,2.123513315,-3.102032691));
#121554=CARTESIAN_POINT('Ctrl Pts',(-6.603280295,2.142857143,-2.993190497));
#121555=CARTESIAN_POINT('Ctrl Pts',(-6.71797025700001,2.18782435,-2.740172865));
#121556=CARTESIAN_POINT('Ctrl Pts',(-6.812962634,2.233445087,-2.479120843));
#121557=CARTESIAN_POINT('Ctrl Pts',(-6.82708405989073,2.10273945758871,
-3.1049944917374));
#121558=CARTESIAN_POINT('Ctrl Pts',(-6.82878127394536,2.10338697179435,
-3.1012518768687));
#121559=CARTESIAN_POINT('Ctrl Pts',(-6.830478488,2.104034486,-3.097509262));
#121560=CARTESIAN_POINT('Ctrl Pts',(-6.881534885,2.123513315,-2.984922149));
#121561=CARTESIAN_POINT('Ctrl Pts',(-6.928852998,2.142857143,-2.870713524));
#121562=CARTESIAN_POINT('Ctrl Pts',(-7.038850015,2.18782435,-2.605220935));
#121563=CARTESIAN_POINT('Ctrl Pts',(-7.128208603,2.233445087,-2.332089646));
#121564=CARTESIAN_POINT('',(-6.83047848457064,2.10403448602288,-3.09750926910287));
#121565=CARTESIAN_POINT('',(-7.04619557178843,2.1937110227552,-2.56926603626331));
#121566=CARTESIAN_POINT('Ctrl Pts',(-6.83047848460633,2.10403448479516,
-3.09750926904382));
#121567=CARTESIAN_POINT('Ctrl Pts',(-6.86457003691931,2.11704095516579,
-3.02233221654642));
#121568=CARTESIAN_POINT('Ctrl Pts',(-6.89736606667674,2.12998516342585,
-2.94671146444441));
#121569=CARTESIAN_POINT('Ctrl Pts',(-6.92885299821979,2.14285714325619,
-2.87071352264051));
#121570=CARTESIAN_POINT('Ctrl Pts',(-6.97003454902749,2.1596923211106,-2.77131631200742));
#121571=CARTESIAN_POINT('Ctrl Pts',(-7.00917625783354,2.17665108708345,
-2.67079126633463));
#121572=CARTESIAN_POINT('Ctrl Pts',(-7.04619557181963,2.19371102294448,
-2.56926603602451));
#121573=CARTESIAN_POINT('Ctrl Pts',(-6.81133484948218,2.23266407509841,
-2.48358965246892));
#121574=CARTESIAN_POINT('Ctrl Pts',(-6.85046022076444,2.22584953695752,
-2.49774239831446));
#121575=CARTESIAN_POINT('Ctrl Pts',(-6.88961550288228,2.21920120628502,
-2.51196994118742));
#121576=CARTESIAN_POINT('Ctrl Pts',(-6.96788850361665,2.20622739510165,
-2.54052733481638));
#121577=CARTESIAN_POINT('Ctrl Pts',(-7.00705147916311,2.19989441314747,
-2.55487370363071));
#121578=CARTESIAN_POINT('Ctrl Pts',(-7.04619557151431,2.19371102277301,
-2.56926603701651));
#121579=CARTESIAN_POINT('',(-6.66576231853214,2.10403448732041,-3.15334951533061));
#121580=CARTESIAN_POINT('Origin',(-6.08020578329871E-13,2.19479107900044,
-2.8275992658422E-13));
#121581=CARTESIAN_POINT('',(-7.04364229628566,2.01370168036341,-2.57625759529277));
#121582=CARTESIAN_POINT('Origin',(0.180834155255899,2.01785799584734,0.0668443661232415));
#121583=CARTESIAN_POINT('',(-7.21882391984097,2.10403448602303,-2.0343503172764));
#121584=CARTESIAN_POINT('Origin',(0.166213305598615,1.8751063277391,0.0843635730378581));
#121585=CARTESIAN_POINT('Origin',(0.185853546571361,2.01789499323372,0.0380208633381401));
#121586=CARTESIAN_POINT('Ctrl Pts',(-6.809733927,2.233426833,-2.487975852));
#121587=CARTESIAN_POINT('Ctrl Pts',(-6.94471696,2.169174758,-2.118519479));
#121588=CARTESIAN_POINT('Ctrl Pts',(-7.03893624400001,2.104034486,-1.736627927));
#121589=CARTESIAN_POINT('Ctrl Pts',(-6.956355169,2.233426833,-2.8034127));
#121590=CARTESIAN_POINT('Ctrl Pts',(-7.108451961,2.169174758,-2.426001516));
#121591=CARTESIAN_POINT('Ctrl Pts',(-7.218823922,2.104034486,-2.03435031));
#121592=CARTESIAN_POINT('',(-7.12888008104419,2.10403448477417,-1.88548912589476));
#121593=CARTESIAN_POINT('Ctrl Pts',(-7.03703314764056,2.10273945758871,
-1.74434159666193));
#121594=CARTESIAN_POINT('Ctrl Pts',(-7.03798469582028,2.10338697179435,
-1.74048476183097));
#121595=CARTESIAN_POINT('Ctrl Pts',(-7.038936244,2.104034486,-1.736627927));
#121596=CARTESIAN_POINT('Ctrl Pts',(-7.067561167,2.123513315,-1.620604795));
#121597=CARTESIAN_POINT('Ctrl Pts',(-7.09234675,2.142857143,-1.503701295));
#121598=CARTESIAN_POINT('Ctrl Pts',(-7.149964013,2.18782435,-1.231944122));
#121599=CARTESIAN_POINT('Ctrl Pts',(-7.18661705200001,2.233445087,-0.956574799));
#121600=CARTESIAN_POINT('Ctrl Pts',(-7.33495266083656,2.10273945758871,
-1.5647801799305));
#121601=CARTESIAN_POINT('Ctrl Pts',(-7.33580564341827,2.10338697179435,
-1.56076021446525));
#121602=CARTESIAN_POINT('Ctrl Pts',(-7.33665862600001,2.104034486,-1.556740249));
#121603=CARTESIAN_POINT('Ctrl Pts',(-7.362318452,2.123513315,-1.435809744));
#121604=CARTESIAN_POINT('Ctrl Pts',(-7.383978815,2.142857143,-1.314099258));
#121605=CARTESIAN_POINT('Ctrl Pts',(-7.43433110500001,2.18782435,-1.031167631));
#121606=CARTESIAN_POINT('Ctrl Pts',(-7.462885385,2.233445087,-0.745212545));
#121607=CARTESIAN_POINT('',(-7.33665862544321,2.10403448645287,-1.55674025405362));
#121608=CARTESIAN_POINT('',(-7.43377568585854,2.19371102273836,-0.994474260409655));
#121609=CARTESIAN_POINT('Ctrl Pts',(-7.3366586242005,2.10403448479508,-1.55674025660878));
#121610=CARTESIAN_POINT('Ctrl Pts',(-7.35379229118596,2.11704095516578,
-1.47599212581495));
#121611=CARTESIAN_POINT('Ctrl Pts',(-7.36956534162783,2.12998516342583,
-1.39508916805695));
#121612=CARTESIAN_POINT('Ctrl Pts',(-7.38397881522071,2.1428571432493,-1.31409925646942));
#121613=CARTESIAN_POINT('Ctrl Pts',(-7.40283010283332,2.15969232108844,
-1.20817308110037));
#121614=CARTESIAN_POINT('Ctrl Pts',(-7.41944678640928,2.17665108707894,
-1.10158394513924));
#121615=CARTESIAN_POINT('Ctrl Pts',(-7.43377568598252,2.19371102295089,
-0.994474260071402));
#121616=CARTESIAN_POINT('Ctrl Pts',(-7.18598798653499,2.23266407510434,
-0.961289055387706));
#121617=CARTESIAN_POINT('Ctrl Pts',(-7.22724102058186,2.22584954186998,
-0.96670011587034));
#121618=CARTESIAN_POINT('Ctrl Pts',(-7.26853934111409,2.21920121629529,
-0.972177793950064));
#121619=CARTESIAN_POINT('Ctrl Pts',(-7.35112150980201,2.20622738128115,
-0.983241170647898));
#121620=CARTESIAN_POINT('Ctrl Pts',(-7.39245302161804,2.19989438508059,
-0.98883326110024));
#121621=CARTESIAN_POINT('Ctrl Pts',(-7.43377568572892,2.19371102275314,
-0.994474261375388));
#121622=CARTESIAN_POINT('',(-7.18779743318908,2.10403448732041,-1.64668409590472));
#121623=CARTESIAN_POINT('Origin',(-6.24934132220645E-13,2.19479107899956,
-4.32596666821716E-14));
#121624=CARTESIAN_POINT('',(-7.43278508299951,2.01370168036821,-1.0018512392213));
#121625=CARTESIAN_POINT('Origin',(0.190975910079478,2.01785797598412,0.0264075854711586));
#121626=CARTESIAN_POINT('',(-7.48737701144199,2.10403448602304,-0.434954581570202));
#121627=CARTESIAN_POINT('Origin',(0.18046278998651,1.87510630430002,0.046660235261801));
#121628=CARTESIAN_POINT('Origin',(0.189681877241171,2.0178949369342,-0.00282105850883979));
#121629=CARTESIAN_POINT('Ctrl Pts',(-7.185367396,2.233426833,-0.965916859000001));
#121630=CARTESIAN_POINT('Ctrl Pts',(-7.237772401,2.169174758,-0.576080809));
#121631=CARTESIAN_POINT('Ctrl Pts',(-7.247693496,2.104034486,-0.182863309));
#121632=CARTESIAN_POINT('Ctrl Pts',(-7.396370313,2.233426833,-1.242459737));
#121633=CARTESIAN_POINT('Ctrl Pts',(-7.463778918,2.169174758,-0.841175901));
#121634=CARTESIAN_POINT('Ctrl Pts',(-7.487377012,2.104034486,-0.434954574));
#121635=CARTESIAN_POINT('',(-7.36753525367957,2.10403448477417,-0.30890894914232));
#121636=CARTESIAN_POINT('Ctrl Pts',(-7.24749310390195,2.10273945758871,
-0.190805746883936));
#121637=CARTESIAN_POINT('Ctrl Pts',(-7.24759329995098,2.10338697179435,
-0.186834527941968));
#121638=CARTESIAN_POINT('Ctrl Pts',(-7.247693496,2.104034486,-0.182863309));
#121639=CARTESIAN_POINT('Ctrl Pts',(-7.250707641,2.123513315,-0.06339922));
#121640=CARTESIAN_POINT('Ctrl Pts',(-7.249782953,2.142857143,0.056099309));
#121641=CARTESIAN_POINT('Ctrl Pts',(-7.247633398,2.18782435,0.333888958));
#121642=CARTESIAN_POINT('Ctrl Pts',(-7.224233245,2.233445087,0.61069962));
#121643=CARTESIAN_POINT('Ctrl Pts',(-7.49984702782103,2.10273945758871,
0.0486015141103503));
#121644=CARTESIAN_POINT('Ctrl Pts',(-7.49981589441051,2.10338697179435,
0.0527108610551751));
#121645=CARTESIAN_POINT('Ctrl Pts',(-7.499784761,2.104034486,0.056820208));
#121646=CARTESIAN_POINT('Ctrl Pts',(-7.498848191,2.123513315,0.180439529));
#121647=CARTESIAN_POINT('Ctrl Pts',(-7.49383799,2.142857143,0.303960829));
#121648=CARTESIAN_POINT('Ctrl Pts',(-7.482191134,2.18782435,0.591101925));
#121649=CARTESIAN_POINT('Ctrl Pts',(-7.44860594,2.233445087,0.876509867));
#121650=CARTESIAN_POINT('',(-7.49978476100023,2.10403448602285,0.0568202001146768));
#121651=CARTESIAN_POINT('',(-7.4737607105466,2.19371102281187,0.626818027942189));
#121652=CARTESIAN_POINT('Ctrl Pts',(-7.49978476087731,2.10403448481428,
0.0568202003041735));
#121653=CARTESIAN_POINT('Ctrl Pts',(-7.49915939127319,2.11704095516578,
0.139363716427324));
#121654=CARTESIAN_POINT('Ctrl Pts',(-7.49717193224029,2.12998516342591,
0.221765947480715));
#121655=CARTESIAN_POINT('Ctrl Pts',(-7.49383798972033,2.14285714327001,
0.30396083051117));
#121656=CARTESIAN_POINT('Ctrl Pts',(-7.4894775475308,2.15969232121401,0.41146298053867));
#121657=CARTESIAN_POINT('Ctrl Pts',(-7.48279222887186,2.17665108720123,
0.519132217772847));
#121658=CARTESIAN_POINT('Ctrl Pts',(-7.47376071040789,2.19371102307763,
0.626818027888455));
#121659=CARTESIAN_POINT('Ctrl Pts',(-7.22463231248959,2.23266407510154,
0.605960349779416));
#121660=CARTESIAN_POINT('Ctrl Pts',(-7.26608408384316,2.22584954313154,
0.609543979184151));
#121661=CARTESIAN_POINT('Ctrl Pts',(-7.30759440260203,2.21920121886999,
0.613072283660542));
#121662=CARTESIAN_POINT('Ctrl Pts',(-7.39062361859046,2.20622746610293,
0.620020243728127));
#121663=CARTESIAN_POINT('Ctrl Pts',(-7.43219034000722,2.19989455756702,
0.623443897837998));
#121664=CARTESIAN_POINT('Ctrl Pts',(-7.47376071067519,2.19371102281321,
0.626818026360383));
#121665=CARTESIAN_POINT('',(-7.3737391284307,2.10403448732041,-0.0630215586092022));
#121666=CARTESIAN_POINT('Ctrl Pts',(-7.225021072,2.233426833,0.601307333));
#121667=CARTESIAN_POINT('Ctrl Pts',(-7.19239765,2.169174758,0.993294759999999));
#121668=CARTESIAN_POINT('Ctrl Pts',(-7.117556656,2.104034486,1.379451795));
#121669=CARTESIAN_POINT('Ctrl Pts',(-7.490539402,2.233426833,0.376589264));
#121670=CARTESIAN_POINT('Ctrl Pts',(-7.470107869,2.169174758,0.782982164));
#121671=CARTESIAN_POINT('Ctrl Pts',(-7.405828674,2.104034486,1.184779155));
#121672=CARTESIAN_POINT('',(-7.40582866653834,2.10403448559146,1.18477915314357));
#121673=CARTESIAN_POINT('Origin',(0.184637716951742,2.01789546140875,-0.043530754871078));
#121674=CARTESIAN_POINT('',(-7.26169266632994,2.10403448477417,1.28211546746747));
#121675=CARTESIAN_POINT('Origin',(1.42160588856299E-12,2.19479107900078,
3.61174848709234E-15));
#121676=CARTESIAN_POINT('',(-7.47437910004272,2.01370168037301,0.619400567520569));
#121677=CARTESIAN_POINT('Origin',(0.192188080730424,2.01785800239135,-0.0152639928727116));
#121678=CARTESIAN_POINT('Origin',(0.186271580860661,1.87510603428352,0.00677543665428812));
#121679=CARTESIAN_POINT('Ctrl Pts',(-7.11906833833695,2.10273945758871,
1.37165196852683));
#121680=CARTESIAN_POINT('Ctrl Pts',(-7.11831249716848,2.10338697179435,
1.37555188176341));
#121681=CARTESIAN_POINT('Ctrl Pts',(-7.11755665600001,2.104034486,1.379451795));
#121682=CARTESIAN_POINT('Ctrl Pts',(-7.094819084,2.123513315,1.496770832));
#121683=CARTESIAN_POINT('Ctrl Pts',(-7.068227363,2.142857143,1.613276771));
#121684=CARTESIAN_POINT('Ctrl Pts',(-7.006411501,2.18782435,1.884109762));
#121685=CARTESIAN_POINT('Ctrl Pts',(-6.92405232,2.233445087,2.149418403));
#121686=CARTESIAN_POINT('Ctrl Pts',(-7.3140568833428,2.10273945758871,1.65971065413927));
#121687=CARTESIAN_POINT('Ctrl Pts',(-7.3131430896714,2.10338697179435,1.66371723406964));
#121688=CARTESIAN_POINT('Ctrl Pts',(-7.31222929600001,2.104034486,1.667723814));
#121689=CARTESIAN_POINT('Ctrl Pts',(-7.284740122,2.123513315,1.788251649));
#121690=CARTESIAN_POINT('Ctrl Pts',(-7.253293629,2.142857143,1.907808045));
#121691=CARTESIAN_POINT('Ctrl Pts',(-7.180192223,2.18782435,2.185732212));
#121692=CARTESIAN_POINT('Ctrl Pts',(-7.086037961,2.233445087,2.457247651));
#121693=CARTESIAN_POINT('',(-7.31222929770186,2.10403448602284,1.66772380630061));
#121694=CARTESIAN_POINT('',(-7.21489297767554,2.1040344873204,1.52358779656554));
#121695=CARTESIAN_POINT('',(-7.16428099143325,2.19371102282214,2.21880099966736));
#121696=CARTESIAN_POINT('Ctrl Pts',(-7.31222929756165,2.10403448479508,
1.66772380633891));
#121697=CARTESIAN_POINT('Ctrl Pts',(-7.29387413230456,2.11704095516578,
1.74820306499409));
#121698=CARTESIAN_POINT('Ctrl Pts',(-7.27421909503796,2.12998516342588,
1.82825153285545));
#121699=CARTESIAN_POINT('Ctrl Pts',(-7.25329362833213,2.14285714326307,
1.90780804624363));
#121700=CARTESIAN_POINT('Ctrl Pts',(-7.22592534663195,2.15969232114706,
2.01185948903283));
#121701=CARTESIAN_POINT('Ctrl Pts',(-7.19625062404025,2.17665108713607,
2.11557433372164));
#121702=CARTESIAN_POINT('Ctrl Pts',(-7.16428099143183,2.19371102304242,
2.21880100004067));
#121703=CARTESIAN_POINT('Ctrl Pts',(-6.92546086042238,2.23266407511715,
2.14487572194143));
#121704=CARTESIAN_POINT('Ctrl Pts',(-6.96517311709716,2.22584954676187,
2.15728646692895));
#121705=CARTESIAN_POINT('Ctrl Pts',(-7.00495444262849,2.21920122623209,
2.169655765656));
#121706=CARTESIAN_POINT('Ctrl Pts',(-7.08454944101889,2.20622738134269,
2.19429028818731));
#121707=CARTESIAN_POINT('Ctrl Pts',(-7.12440896293867,2.19989438516438,
2.20656969562189));
#121708=CARTESIAN_POINT('Ctrl Pts',(-7.16428099173822,2.19371102283936,
2.21880099868191));
#121709=CARTESIAN_POINT('Origin',(-8.89045781438114E-14,2.19479107900022,
1.4734307524078E-13));
#121710=CARTESIAN_POINT('',(-6.97799202168079,2.10403448602303,2.74911391989858));
#121711=CARTESIAN_POINT('Origin',(0.170966029185567,2.0178949611216,-0.0822056528557094));
#121712=CARTESIAN_POINT('',(-7.16647945764014,2.01370168037485,2.21168989156015));
#121713=CARTESIAN_POINT('Origin',(0.184413421002589,2.01785795354705,-0.0562218673240203));
#121714=CARTESIAN_POINT('Origin',(0.183375927438085,1.87510628547333,-0.0334267439278485));
#121715=CARTESIAN_POINT('Ctrl Pts',(-6.926840792,2.233426833,2.140415062));
#121716=CARTESIAN_POINT('Ctrl Pts',(-6.810714378,2.169174758,2.516224969));
#121717=CARTESIAN_POINT('Ctrl Pts',(-6.654610777,2.104034486,2.877265266));
#121718=CARTESIAN_POINT('Ctrl Pts',(-7.234459193,2.233426833,1.978029369));
#121719=CARTESIAN_POINT('Ctrl Pts',(-7.127142877,2.169174758,2.370528853));
#121720=CARTESIAN_POINT('Ctrl Pts',(-6.977992019,2.104034486,2.749113927));
#121721=CARTESIAN_POINT('',(-6.81630140091813,2.10403448477417,2.81318958942943));
#121722=CARTESIAN_POINT('Ctrl Pts',(-6.65776384915911,2.10273945758871,
2.86997276216926));
#121723=CARTESIAN_POINT('Ctrl Pts',(-6.65618731307956,2.10338697179435,
2.87361901408463));
#121724=CARTESIAN_POINT('Ctrl Pts',(-6.654610777,2.104034486,2.877265266));
#121725=CARTESIAN_POINT('Ctrl Pts',(-6.60718467200001,2.123513315,2.986953543));
#121726=CARTESIAN_POINT('Ctrl Pts',(-6.556169318,2.142857143,3.095019205));
#121727=CARTESIAN_POINT('Ctrl Pts',(-6.437577588,2.18782435,3.346231687));
#121728=CARTESIAN_POINT('Ctrl Pts',(-6.300110404,2.233445087,3.58763277));
#121729=CARTESIAN_POINT('Ctrl Pts',(-6.78626956786007,2.10273945758871,
3.19321356957691));
#121730=CARTESIAN_POINT('Ctrl Pts',(-6.78451584193003,2.10338697179435,
3.19693003928845));
#121731=CARTESIAN_POINT('Ctrl Pts',(-6.782762116,2.104034486,3.200646509));
#121732=CARTESIAN_POINT('Ctrl Pts',(-6.730005702,2.123513315,3.312447111));
#121733=CARTESIAN_POINT('Ctrl Pts',(-6.673593319,2.142857143,3.422448278));
#121734=CARTESIAN_POINT('Ctrl Pts',(-6.542455503,2.18782435,3.678160091));
#121735=CARTESIAN_POINT('Ctrl Pts',(-6.392134722,2.233445087,3.923087266));
#121736=CARTESIAN_POINT('',(-6.78276211930204,2.10403448602284,3.20064650183925));
#121737=CARTESIAN_POINT('',(-6.51980745556354,2.19371102277151,3.7070353038849));
#121738=CARTESIAN_POINT('Ctrl Pts',(-6.78276211917204,2.10403448479508,
3.20064650185367));
#121739=CARTESIAN_POINT('Ctrl Pts',(-6.74753542590802,2.11704095516576,
3.27529838263622));
#121740=CARTESIAN_POINT('Ctrl Pts',(-6.71113185801136,2.12998516342577,
3.34925010984637));
#121741=CARTESIAN_POINT('Ctrl Pts',(-6.67359331829007,2.14285714323346,
3.42244827924652));
#121742=CARTESIAN_POINT('Ctrl Pts',(-6.62449690776747,2.15969232106281,
3.5181836857061));
#121743=CARTESIAN_POINT('Ctrl Pts',(-6.57322033755702,2.17665108710102,
3.61309454621992));
#121744=CARTESIAN_POINT('Ctrl Pts',(-6.51980745545966,2.19371102298407,
3.70703530422561));
#121745=CARTESIAN_POINT('Ctrl Pts',(-6.30246255588908,2.23266407512598,
3.58349908979831));
#121746=CARTESIAN_POINT('Ctrl Pts',(-6.33857882852142,2.22584946944336,
3.60415687408536));
#121747=CARTESIAN_POINT('Ctrl Pts',(-6.37477152369063,2.21920106892251,
3.62478905923907));
#121748=CARTESIAN_POINT('Ctrl Pts',(-6.44720906296556,2.20622738129678,
3.66595771293647));
#121749=CARTESIAN_POINT('Ctrl Pts',(-6.48349698183141,2.19989438510489,
3.68651865357025));
#121750=CARTESIAN_POINT('Ctrl Pts',(-6.51980745604546,2.19371102278678,
3.7070353030366));
#121751=CARTESIAN_POINT('',(-6.71868644984205,2.1040344873204,3.03895588011123));
#121752=CARTESIAN_POINT('Origin',(-9.28510740516586E-13,2.19479107900033,
5.17164436275586E-13));
#121753=CARTESIAN_POINT('',(-6.52348320100087,2.01370168036228,3.70056305468784));
#121754=CARTESIAN_POINT('Origin',(0.168016078881957,2.01785801084683,-0.0945509464054189));
#121755=CARTESIAN_POINT('',(-6.22387221623701,2.10403448602303,4.18490318070215));
#121756=CARTESIAN_POINT('Origin',(0.171902718429249,1.87510629435436,-0.0720655236513112));
#121757=CARTESIAN_POINT('Origin',(0.149296957399963,2.01789501609392,-0.117036249363178));
#121758=CARTESIAN_POINT('Ctrl Pts',(-6.304769136,2.233426833,3.579439362));
#121759=CARTESIAN_POINT('Ctrl Pts',(-6.110569671,2.169174758,3.921499296));
#121760=CARTESIAN_POINT('Ctrl Pts',(-5.880502694,2.104034486,4.240541011));
#121761=CARTESIAN_POINT('Ctrl Pts',(-6.640103713,2.233426833,3.486979019));
#121762=CARTESIAN_POINT('Ctrl Pts',(-6.450920607,2.169174758,3.847232247));
#121763=CARTESIAN_POINT('Ctrl Pts',(-6.223872212,2.104034486,4.184903187));
#121764=CARTESIAN_POINT('',(-6.05218745737027,2.10403448477406,4.21272209272149));
#121765=CARTESIAN_POINT('Ctrl Pts',(-5.8851497218288,2.10273945758871,4.23409681912444));
#121766=CARTESIAN_POINT('Ctrl Pts',(-5.8828262079144,2.10338697179435,4.23731891506222));
#121767=CARTESIAN_POINT('Ctrl Pts',(-5.880502694,2.104034486,4.240541011));
#121768=CARTESIAN_POINT('Ctrl Pts',(-5.810605648,2.123513315,4.337469627));
#121769=CARTESIAN_POINT('Ctrl Pts',(-5.737552082,2.142857143,4.43204198));
#121770=CARTESIAN_POINT('Ctrl Pts',(-5.567729703,2.18782435,4.651887538));
#121771=CARTESIAN_POINT('Ctrl Pts',(-5.381582328,2.233445087,4.85809341700001));
#121772=CARTESIAN_POINT('Ctrl Pts',(-5.94116382984549,2.10273945758871,
4.57740536707451));
#121773=CARTESIAN_POINT('Ctrl Pts',(-5.93865217392275,2.10338697179435,
4.58065794853725));
#121774=CARTESIAN_POINT('Ctrl Pts',(-5.936140518,2.104034486,4.58391053));
#121775=CARTESIAN_POINT('Ctrl Pts',(-5.860583695,2.123513315,4.681756226));
#121776=CARTESIAN_POINT('Ctrl Pts',(-5.781843203,2.142857143,4.777058632));
#121777=CARTESIAN_POINT('Ctrl Pts',(-5.598800835,2.18782435,4.998601291));
#121778=CARTESIAN_POINT('Ctrl Pts',(-5.399342368,2.233445087,5.205487681));
#121779=CARTESIAN_POINT('',(-5.93614052278719,2.10403448602287,4.58391052373464));
#121780=CARTESIAN_POINT('',(-5.57047496931209,2.19371102277816,5.02193275707079));
#121781=CARTESIAN_POINT('Ctrl Pts',(-5.93614052263355,2.1040344847952,4.58391052370258));
#121782=CARTESIAN_POINT('Ctrl Pts',(-5.88568946219855,2.11704095516577,
4.64924438689608));
#121783=CARTESIAN_POINT('Ctrl Pts',(-5.83423955417546,2.12998516342584,
4.71364147262295));
#121784=CARTESIAN_POINT('Ctrl Pts',(-5.78184320195303,2.14285714325256,
4.77705863309712));
#121785=CARTESIAN_POINT('Ctrl Pts',(-5.713314355531,2.15969232111075,4.86000152207673));
#121786=CARTESIAN_POINT('Ctrl Pts',(-5.6428335737432,2.17665108710259,4.94167047258073));
#121787=CARTESIAN_POINT('Ctrl Pts',(-5.57047496910811,2.19371102297666,
5.02193275725284));
#121788=CARTESIAN_POINT('Ctrl Pts',(-5.38476810723808,2.23266407504934,
4.85456202239123));
#121789=CARTESIAN_POINT('Ctrl Pts',(-5.41559884105151,2.22584954617779,
4.88250045523468));
#121790=CARTESIAN_POINT('Ctrl Pts',(-5.44650966311776,2.21920122513509,
4.91043027399371));
#121791=CARTESIAN_POINT('Ctrl Pts',(-5.50840428648849,2.20622739557511,
4.96620896750364));
#121792=CARTESIAN_POINT('Ctrl Pts',(-5.53942374179524,2.19989441414187,
4.99408996540044));
#121793=CARTESIAN_POINT('Ctrl Pts',(-5.57047496988285,2.19371102279481,
5.02193275643796));
#121794=CARTESIAN_POINT('',(-5.90832161085208,2.10403448732034,4.41222576400268));
#121795=CARTESIAN_POINT('Origin',(5.00034041950315E-13,2.19479107899967,
-5.16513914972094E-13));
#121796=CARTESIAN_POINT('',(-5.57545611979481,2.01370168035743,5.01640200242529));
#121797=CARTESIAN_POINT('Origin',(0.143762228792316,2.01785801671927,-0.128458831064288));
#121798=CARTESIAN_POINT('',(-5.17873106354523,2.10403448602303,5.42501101981358));
#121799=CARTESIAN_POINT('Origin',(0.152391677768917,1.87510625869217,-0.107334577256234));
#121800=CARTESIAN_POINT('Origin',(0.120647118062397,2.017894964074,-0.146394430512981));
#121801=CARTESIAN_POINT('Ctrl Pts',(-5.387893482,2.233426833,4.851093055));
#121802=CARTESIAN_POINT('Ctrl Pts',(-5.124701518,2.169174758,5.143408673));
#121803=CARTESIAN_POINT('Ctrl Pts',(-4.831428841,2.104034486,5.405533772));
#121804=CARTESIAN_POINT('Ctrl Pts',(-5.735264364,2.233426833,4.832881405));
#121805=CARTESIAN_POINT('Ctrl Pts',(-5.473060458,2.169174758,5.144043338));
#121806=CARTESIAN_POINT('Ctrl Pts',(-5.178731058,2.104034486,5.425011025));
#121807=CARTESIAN_POINT('',(-5.00507995511935,2.10403448477372,5.41527239330631));
#121808=CARTESIAN_POINT('Ctrl Pts',(-4.83735253472086,2.10273945758871,
5.40023921543883));
#121809=CARTESIAN_POINT('Ctrl Pts',(-4.83439068786043,2.10338697179435,
5.40288649371942));
#121810=CARTESIAN_POINT('Ctrl Pts',(-4.83142884100001,2.104034486,5.405533772));
#121811=CARTESIAN_POINT('Ctrl Pts',(-4.742329161,2.123513315,5.485170451));
#121812=CARTESIAN_POINT('Ctrl Pts',(-4.650653287,2.142857143,5.561827398));
#121813=CARTESIAN_POINT('Ctrl Pts',(-4.437540965,2.18782435,5.740026298));
#121814=CARTESIAN_POINT('Ctrl Pts',(-4.211417444,2.233445087,5.90139501400001));
#121815=CARTESIAN_POINT('Ctrl Pts',(-4.81825587435657,2.10273945758871,
5.74756277776072));
#121816=CARTESIAN_POINT('Ctrl Pts',(-4.81510373067829,2.10338697179435,
5.75019938388036));
#121817=CARTESIAN_POINT('Ctrl Pts',(-4.81195158700001,2.104034486,5.75283599));
#121818=CARTESIAN_POINT('Ctrl Pts',(-4.717127308,2.123513315,5.832151624));
#121819=CARTESIAN_POINT('Ctrl Pts',(-4.619740525,2.142857143,5.908299035));
#121820=CARTESIAN_POINT('Ctrl Pts',(-4.393352463,2.18782435,6.085313451));
#121821=CARTESIAN_POINT('Ctrl Pts',(-4.154082765,2.233445087,6.244485277));
#121822=CARTESIAN_POINT('',(-4.81195159151963,2.10403448645145,5.75283598686443));
#121823=CARTESIAN_POINT('',(-4.36067326450885,2.19371102278376,6.10201021640601));
#121824=CARTESIAN_POINT('Ctrl Pts',(-4.81195159287894,2.10403448479521,
5.75283598484611));
#121825=CARTESIAN_POINT('Ctrl Pts',(-4.74863520074105,2.11704095516583,
5.80579689162016));
#121826=CARTESIAN_POINT('Ctrl Pts',(-4.68454469311788,2.12998516342591,
5.85762819990044));
#121827=CARTESIAN_POINT('Ctrl Pts',(-4.61974052367469,2.14285714327157,
5.90829903559918));
#121828=CARTESIAN_POINT('Ctrl Pts',(-4.53498357418592,2.15969232115578,
5.97457108920442));
#121829=CARTESIAN_POINT('Ctrl Pts',(-4.44859418376242,2.17665108710306,
6.03917938074946));
#121830=CARTESIAN_POINT('Ctrl Pts',(-4.36067326428603,2.19371102297454,
6.10201021650341));
#121831=CARTESIAN_POINT('Ctrl Pts',(-4.21528788658319,2.23266407510532,
5.89863103047213));
#121832=CARTESIAN_POINT('Ctrl Pts',(-4.23939186650286,2.22584954934901,
5.93254395921881));
#121833=CARTESIAN_POINT('Ctrl Pts',(-4.26357591243212,2.21920123154142,
5.96646568966808));
#121834=CARTESIAN_POINT('Ctrl Pts',(-4.3120327286523,2.2062273952247,6.03424585800495));
#121835=CARTESIAN_POINT('Ctrl Pts',(-4.3363333774625,2.19989441341491,6.06814328174801));
#121836=CARTESIAN_POINT('Ctrl Pts',(-4.36067326516774,2.19371102280167,
6.10201021593574));
#121837=CARTESIAN_POINT('',(-4.82169022013528,2.10403448732032,5.57918487569773));
#121838=CARTESIAN_POINT('Origin',(2.21610924056037E-13,2.19479107900044,
-2.77555756156289E-13));
#121839=CARTESIAN_POINT('',(-4.36672690753537,2.01370168035468,6.09767956787779));
#121840=CARTESIAN_POINT('Origin',(0.112786245340395,2.01785802450165,-0.156360098587847));
#121841=CARTESIAN_POINT('',(-3.89143820237535,2.10403448602303,6.41145137387601));
#121842=CARTESIAN_POINT('Origin',(0.125755312133621,1.87510628134173,-0.137585200689151));
#121843=CARTESIAN_POINT('Origin',(0.0863561570362009,2.01789497217148,-0.168907619351457));
#121844=CARTESIAN_POINT('Ctrl Pts',(-4.219085917,2.233426833,5.895915029));
#121845=CARTESIAN_POINT('Ctrl Pts',(-3.899208018,2.169174758,6.12481797800001));
#121846=CARTESIAN_POINT('Ctrl Pts',(-3.556442745,2.104034486,6.317769781));
#121847=CARTESIAN_POINT('Ctrl Pts',(-4.562250427,2.233426833,5.952803629));
#121848=CARTESIAN_POINT('Ctrl Pts',(-4.239286085,2.169174758,6.200324679));
#121849=CARTESIAN_POINT('Ctrl Pts',(-3.891438196,2.104034486,6.411451378));
#121850=CARTESIAN_POINT('',(-3.72394047710203,2.10403448477417,6.36461057563715));
#121851=CARTESIAN_POINT('Ctrl Pts',(-3.56336611914592,2.10273945758871,
6.31387242722715));
#121852=CARTESIAN_POINT('Ctrl Pts',(-3.55990443207296,2.10338697179435,
6.31582110411357));
#121853=CARTESIAN_POINT('Ctrl Pts',(-3.556442745,2.104034486,6.317769781));
#121854=CARTESIAN_POINT('Ctrl Pts',(-3.452306635,2.123513315,6.376390802));
#121855=CARTESIAN_POINT('Ctrl Pts',(-3.346295113,2.142857143,6.431547949));
#121856=CARTESIAN_POINT('Ctrl Pts',(-3.099857743,2.18782435,6.559767807));
#121857=CARTESIAN_POINT('Ctrl Pts',(-2.84433136,2.233445087,6.66875394));
#121858=CARTESIAN_POINT('Ctrl Pts',(-3.47005162939066,2.10273945758871,
6.64897053993112));
#121859=CARTESIAN_POINT('Ctrl Pts',(-3.46640638869533,2.10338697179435,
6.65086788596556));
#121860=CARTESIAN_POINT('Ctrl Pts',(-3.462761148,2.104034486,6.652765232));
#121861=CARTESIAN_POINT('Ctrl Pts',(-3.353103291,2.123513315,6.709842094));
#121862=CARTESIAN_POINT('Ctrl Pts',(-3.241623914,2.142857143,6.763273941));
#121863=CARTESIAN_POINT('Ctrl Pts',(-2.982475812,2.18782435,6.887483117));
#121864=CARTESIAN_POINT('Ctrl Pts',(-2.71458287,2.233445087,6.991497682));
#121865=CARTESIAN_POINT('',(-3.46276115129472,2.10403448644941,6.65276523147423));
#121866=CARTESIAN_POINT('',(-2.94697132435592,2.19371102277444,6.89676445962475));
#121867=CARTESIAN_POINT('Ctrl Pts',(-3.46276115059833,2.10403448555034,
6.65276523044313));
#121868=CARTESIAN_POINT('Ctrl Pts',(-3.38954003234906,2.11704095566684,
6.69087678746824));
#121869=CARTESIAN_POINT('Ctrl Pts',(-3.31580572724131,2.12998516367491,
6.72771874325727));
#121870=CARTESIAN_POINT('Ctrl Pts',(-3.24162391269829,2.14285714324092,
6.76327394139065));
#121871=CARTESIAN_POINT('Ctrl Pts',(-3.14460200116611,2.15969232108241,
6.80977635259009));
#121872=CARTESIAN_POINT('Ctrl Pts',(-3.04634347358902,2.17665108710011,
6.85430297270454));
#121873=CARTESIAN_POINT('Ctrl Pts',(-2.94697132436812,2.19371102292601,
6.89676445959237));
#121874=CARTESIAN_POINT('Ctrl Pts',(-2.84870548848617,2.23266407512427,
6.66688660753919));
#121875=CARTESIAN_POINT('Ctrl Pts',(-2.86495564567119,2.22584955275781,
6.70518829479386));
#121876=CARTESIAN_POINT('Ctrl Pts',(-2.88128210347658,2.21920123846776,
6.74351578719786));
#121877=CARTESIAN_POINT('Ctrl Pts',(-2.91403531030025,2.20622739559012,
6.82012811461766));
#121878=CARTESIAN_POINT('Ctrl Pts',(-2.93048087823981,2.19989441416818,
6.85845695408517));
#121879=CARTESIAN_POINT('Ctrl Pts',(-2.94697132514375,2.19371102279083,
6.89676445928825));
#121880=CARTESIAN_POINT('',(-3.50960195363171,2.10403448732032,6.48526750264057));
#121881=CARTESIAN_POINT('Origin',(2.78423117894278E-13,2.19479107900055,
-7.29451221648247E-13));
#121882=CARTESIAN_POINT('',(-2.95381439771729,2.01370168036686,6.89383641367547));
#121883=CARTESIAN_POINT('Origin',(0.0765365434508686,2.01785800296307,-0.176950156993154));
#121884=CARTESIAN_POINT('',(-2.42218601520132,2.10403448602303,7.0980993866009));
#121885=CARTESIAN_POINT('Origin',(0.0932382937642756,1.87510628672111,-0.161401769551879));
#121886=CARTESIAN_POINT('Origin',(0.0480269101018865,2.01789493634255,-0.183522341499351));
#121887=CARTESIAN_POINT('Ctrl Pts',(-2.852998583,2.233426833,6.665050569));
#121888=CARTESIAN_POINT('Ctrl Pts',(-2.491391884,2.169174758,6.819837601));
#121889=CARTESIAN_POINT('Ctrl Pts',(-2.115161339,2.104034486,6.934593897));
#121890=CARTESIAN_POINT('Ctrl Pts',(-3.175910731,2.233426833,6.79437937));
#121891=CARTESIAN_POINT('Ctrl Pts',(-2.807287406,2.169174758,6.96668573000001));
#121892=CARTESIAN_POINT('Ctrl Pts',(-2.422186008,2.104034486,7.098099389));
#121893=CARTESIAN_POINT('',(-2.26867368077852,2.1040344847741,7.01634664064656));
#121894=CARTESIAN_POINT('Ctrl Pts',(-2.12276066440802,2.10273945758871,
6.93227598202678));
#121895=CARTESIAN_POINT('Ctrl Pts',(-2.11896100170401,2.10338697179436,
6.93343493951339));
#121896=CARTESIAN_POINT('Ctrl Pts',(-2.115161339,2.104034486,6.934593897));
#121897=CARTESIAN_POINT('Ctrl Pts',(-2.000858086,2.123513315,6.969458205));
#121898=CARTESIAN_POINT('Ctrl Pts',(-1.885467899,2.142857143,7.000536465));
#121899=CARTESIAN_POINT('Ctrl Pts',(-1.617228618,2.18782435,7.072781865));
#121900=CARTESIAN_POINT('Ctrl Pts',(-1.344247503,2.233445087,7.124289344));
#121901=CARTESIAN_POINT('Ctrl Pts',(-1.95959162658564,2.10273945758871,
7.23947982964323));
#121902=CARTESIAN_POINT('Ctrl Pts',(-1.95562373629282,2.10338697179436,
7.24054919782161));
#121903=CARTESIAN_POINT('Ctrl Pts',(-1.951655846,2.104034486,7.241618566));
#121904=CARTESIAN_POINT('Ctrl Pts',(-1.832291891,2.123513315,7.273787806));
#121905=CARTESIAN_POINT('Ctrl Pts',(-1.711932572,2.142857143,7.302005674));
#121906=CARTESIAN_POINT('Ctrl Pts',(-1.432141907,2.18782435,7.367601728));
#121907=CARTESIAN_POINT('Ctrl Pts',(-1.148152096,2.233445087,7.411595426));
#121908=CARTESIAN_POINT('',(-1.95165585101424,2.10403448645285,7.24161856517329));
#121909=CARTESIAN_POINT('',(-1.39547228056022,2.19371102271546,7.36903366209712));
#121910=CARTESIAN_POINT('Ctrl Pts',(-1.95165585349977,2.10403448479518,
7.241618563791));
#121911=CARTESIAN_POINT('Ctrl Pts',(-1.87195374484221,2.11704095516582,
7.26309871897641));
#121912=CARTESIAN_POINT('Ctrl Pts',(-1.79202337387582,2.12998516342552,
7.28322863460931));
#121913=CARTESIAN_POINT('Ctrl Pts',(-1.71193257096122,2.14285714316695,
7.30200567424354));
#121914=CARTESIAN_POINT('Ctrl Pts',(-1.60718233439155,2.15969232089214,
7.32656404244406));
#121915=CARTESIAN_POINT('Ctrl Pts',(-1.50164912869463,2.17665108706648,
7.3489269758674));
#121916=CARTESIAN_POINT('Ctrl Pts',(-1.39547228022281,2.19371102293117,
7.36903366220398));
#121917=CARTESIAN_POINT('Ctrl Pts',(-1.34892078850231,2.23266407510437,
7.12340597657611));
#121918=CARTESIAN_POINT('Ctrl Pts',(-1.35655729175984,2.22584955593532,
7.1643054758536));
#121919=CARTESIAN_POINT('Ctrl Pts',(-1.36426276392943,2.21920124492997,
7.20524657681581));
#121920=CARTESIAN_POINT('Ctrl Pts',(-1.37978085812241,2.20622738124446,
7.28710885303433));
#121921=CARTESIAN_POINT('Ctrl Pts',(-1.38760239028112,2.19989438504379,
7.32807699882485));
#121922=CARTESIAN_POINT('Ctrl Pts',(-1.39547228150767,2.19371102272976,
7.36903366191723));
#121923=CARTESIAN_POINT('',(-2.03340860029468,2.10403448732034,7.0881062292639));
#121924=CARTESIAN_POINT('Origin',(2.7451999007333E-13,2.19479107900011,
-1.07466119336763E-12));
#121925=CARTESIAN_POINT('',(-1.40278480996379,2.0137016803479,7.36764513069795));
#121926=CARTESIAN_POINT('Origin',(0.036708161759855,2.01785799579938,-0.189266476262751));
#121927=CARTESIAN_POINT('',(-0.839675102517359,2.10403448602304,7.4528481619308));
#121928=CARTESIAN_POINT('Origin',(0.0563618769601583,1.87510629880602,-0.177672048156901));
#121929=CARTESIAN_POINT('Origin',(0.00745225203801603,2.01789496330402,
-0.189556365350569));
#121930=CARTESIAN_POINT('Ctrl Pts',(-1.353508207,2.233426833,7.122535752));
#121931=CARTESIAN_POINT('Ctrl Pts',(-0.967081035,2.169174758,7.195969198));
#121932=CARTESIAN_POINT('Ctrl Pts',(-0.574977339,2.104034486,7.227164109));
#121933=CARTESIAN_POINT('Ctrl Pts',(-1.641068979,2.233426833,7.318257484));
#121934=CARTESIAN_POINT('Ctrl Pts',(-1.244023089,2.169174758,7.407292298));
#121935=CARTESIAN_POINT('Ctrl Pts',(-0.839675095000001,2.104034486,7.452848163));
#121936=CARTESIAN_POINT('',(-0.707326224613765,2.10403448477417,7.34000613526629));
#121937=CARTESIAN_POINT('Origin',(8.67361737988404E-16,2.19479107900078,
3.20056481317721E-13));
#121938=CARTESIAN_POINT('',(0.213837435912966,2.01370168036516,7.4969509500413));
#121939=CARTESIAN_POINT('',(-0.349293291499008,2.10403448645148,7.49186186523539));
#121940=CARTESIAN_POINT('Origin',(-0.00483675568053087,2.01785801767571,
-0.192732460490868));
#121941=CARTESIAN_POINT('Origin',(0.0168499294777102,1.87510630843667,-0.185634169925616));
#121942=CARTESIAN_POINT('Ctrl Pts',(-0.349293293799583,2.10403448479561,
7.49186186445147));
#121943=CARTESIAN_POINT('Ctrl Pts',(-0.266836977566266,2.11704095516595,
7.49570622743379));
#121944=CARTESIAN_POINT('Ctrl Pts',(-0.184447997517407,2.12998516342579,
7.49818284972337));
#121945=CARTESIAN_POINT('Ctrl Pts',(-0.102193164471361,2.14285714323922,
7.49930373802083));
#121946=CARTESIAN_POINT('Ctrl Pts',(0.00538739360841867,2.15969232107956,
7.50076974064817));
#121947=CARTESIAN_POINT('Ctrl Pts',(0.113260660248663,2.17665108710564,
7.49992332144283));
#121948=CARTESIAN_POINT('Ctrl Pts',(0.221277496359257,2.19371102298715,
7.4967350409221));
#121949=CARTESIAN_POINT('Ctrl Pts',(-0.58289727953186,2.10273945758871,
7.2265340158684));
#121950=CARTESIAN_POINT('Ctrl Pts',(-0.57893730926593,2.10338697179435,
7.2268490624342));
#121951=CARTESIAN_POINT('Ctrl Pts',(-0.574977339,2.104034486,7.227164109));
#121952=CARTESIAN_POINT('Ctrl Pts',(-0.455851638000001,2.123513315,7.236641489));
#121953=CARTESIAN_POINT('Ctrl Pts',(-0.336478302,2.142857143,7.242187677));
#121954=CARTESIAN_POINT('Ctrl Pts',(-0.0589796810000001,2.18782435,7.255080503));
#121955=CARTESIAN_POINT('Ctrl Pts',(0.218691873,2.233445087,7.246700895));
#121956=CARTESIAN_POINT('Ctrl Pts',(-0.357503297558422,2.10273945758871,
7.49147908942938));
#121957=CARTESIAN_POINT('Ctrl Pts',(-0.353398291779211,2.10338697179435,
7.49167047721469));
#121958=CARTESIAN_POINT('Ctrl Pts',(-0.349293286,2.104034486,7.491861865));
#121959=CARTESIAN_POINT('Ctrl Pts',(-0.225804558,2.123513315,7.497619283));
#121960=CARTESIAN_POINT('Ctrl Pts',(-0.102193166,2.142857143,7.499303738));
#121961=CARTESIAN_POINT('Ctrl Pts',(0.185157361,2.18782435,7.50321947));
#121962=CARTESIAN_POINT('Ctrl Pts',(0.471964993,2.233445087,7.485135206));
#121963=CARTESIAN_POINT('',(-0.462135320593557,2.10403448732041,7.35951298649177));
#121964=CARTESIAN_POINT('Ctrl Pts',(-1.153454472,3.784676613,7.410772077));
#121965=CARTESIAN_POINT('Ctrl Pts',(-0.75228298,3.720089779,7.473212677));
#121966=CARTESIAN_POINT('Ctrl Pts',(-0.346715327,3.654947264,7.491981613));
#121967=CARTESIAN_POINT('Ctrl Pts',(-1.349344274,3.784676613,7.12332577));
#121968=CARTESIAN_POINT('Ctrl Pts',(-0.963733275,3.720089779,7.196370583));
#121969=CARTESIAN_POINT('Ctrl Pts',(-0.572490449,3.654947264,7.22736153));
#121970=CARTESIAN_POINT('',(-0.595569424151332,3.69493258270807,7.47631574084745));
#121971=CARTESIAN_POINT('Ctrl Pts',(-0.595569427165582,3.69493258262019,
7.47631574064059));
#121972=CARTESIAN_POINT('Ctrl Pts',(-0.592533546838534,3.6887188543259,
7.43471764119767));
#121973=CARTESIAN_POINT('Ctrl Pts',(-0.589480876022489,3.68234999899509,
7.3931195546627));
#121974=CARTESIAN_POINT('Ctrl Pts',(-0.583346580461599,3.66929201047644,
7.31002507177171));
#121975=CARTESIAN_POINT('Ctrl Pts',(-0.580261328340382,3.66259515856785,
7.26847951121063));
#121976=CARTESIAN_POINT('Ctrl Pts',(-0.577160368804072,3.65572482644946,
7.22699010136305));
#121977=CARTESIAN_POINT('',(-1.15345447430354,3.78467661255986,7.41077207811034));
#121978=CARTESIAN_POINT('Origin',(0.0039120167552463,3.62502539284573,-0.190456296094067));
#121979=CARTESIAN_POINT('',(-1.25139938100297,3.78467661169947,7.26704892212187));
#121980=CARTESIAN_POINT('Ctrl Pts',(-2.428996377,3.654941533,7.095771741));
#121981=CARTESIAN_POINT('Ctrl Pts',(-2.143769523,3.702826767,7.193409464));
#121982=CARTESIAN_POINT('Ctrl Pts',(-1.851626136,3.75,7.267838788));
#121983=CARTESIAN_POINT('Ctrl Pts',(-1.744586692,3.767283967,7.29510921));
#121984=CARTESIAN_POINT('Ctrl Pts',(-1.636790581,3.784676613,7.319215572));
#121985=CARTESIAN_POINT('Ctrl Pts',(-2.121814945,3.654941533,6.932560951));
#121986=CARTESIAN_POINT('Ctrl Pts',(-1.843148632,3.702826767,7.01785098300001));
#121987=CARTESIAN_POINT('Ctrl Pts',(-1.558535692,3.75,7.080499029));
#121988=CARTESIAN_POINT('Ctrl Pts',(-1.454255355,3.767283967,7.103452867));
#121989=CARTESIAN_POINT('Ctrl Pts',(-1.349344274,3.784676613,7.12332577));
#121990=CARTESIAN_POINT('',(-1.63679058102371,3.78467661265395,7.31921557283982));
#121991=CARTESIAN_POINT('',(-1.49306742272831,3.78467661221161,7.2212706719866));
#121992=CARTESIAN_POINT('',(-2.18883222389661,3.69493258295591,7.17349381339529));
#121993=CARTESIAN_POINT('Ctrl Pts',(-1.63679058234593,3.78467661270495,
7.3192155712621));
#121994=CARTESIAN_POINT('Ctrl Pts',(-1.70875829796881,3.77306479305815,
7.30312148604201));
#121995=CARTESIAN_POINT('Ctrl Pts',(-1.78038472622913,3.76150355535518,
7.28598895022121));
#121996=CARTESIAN_POINT('Ctrl Pts',(-1.85162613527264,3.750000000057,7.26783878785067));
#121997=CARTESIAN_POINT('Ctrl Pts',(-1.9644656106393,3.73177948540332,7.23909069274917));
#121998=CARTESIAN_POINT('Ctrl Pts',(-2.07693173261751,3.71341418930112,
7.20763776133147));
#121999=CARTESIAN_POINT('Ctrl Pts',(-2.18883221719789,3.69493258478878,
7.17349381504735));
#122000=CARTESIAN_POINT('Ctrl Pts',(-2.11725592328059,3.6557248262931,6.93395466940919));
#122001=CARTESIAN_POINT('Ctrl Pts',(-2.12920338773,3.66259516242469,6.97380748842239));
#122002=CARTESIAN_POINT('Ctrl Pts',(-2.14114758426415,3.66929201878043,
7.01371852726311));
#122003=CARTESIAN_POINT('Ctrl Pts',(-2.16500130557688,3.68234999887378,
7.09355156358785));
#122004=CARTESIAN_POINT('Ctrl Pts',(-2.17692496583076,3.68871885430259,
7.13352087664977));
#122005=CARTESIAN_POINT('Ctrl Pts',(-2.18883223082714,3.6949325826302,7.17349381138143));
#122006=CARTESIAN_POINT('Ctrl Pts',(-2.719584283,3.784676613,6.989553729));
#122007=CARTESIAN_POINT('Ctrl Pts',(-2.341214841,3.720089779,7.136774514));
#122008=CARTESIAN_POINT('Ctrl Pts',(-1.949163901,3.654947264,7.242289699));
#122009=CARTESIAN_POINT('Ctrl Pts',(-2.849101831,3.784676613,6.66671724));
#122010=CARTESIAN_POINT('Ctrl Pts',(-2.488208678,3.720089779,6.820949271));
#122011=CARTESIAN_POINT('Ctrl Pts',(-2.11277503,3.654947264,6.93532131));
#122012=CARTESIAN_POINT('',(-2.71958428550801,3.78467661255987,6.98955372957205));
#122013=CARTESIAN_POINT('Origin',(0.0447630885962563,3.62502541599822,-0.185162737300266));
#122014=CARTESIAN_POINT('',(-2.78434306451961,3.78467661169947,6.82813548143369));
#122015=CARTESIAN_POINT('Origin',(2.03504747775529E-13,3.87542691999989,
-7.01261965163624E-13));
#122016=CARTESIAN_POINT('',(-2.18502660827734,3.87435041278773,7.17465390913854));
#122017=CARTESIAN_POINT('Origin',(0.015141183425918,3.62514700711987,-0.184193113378951));
#122018=CARTESIAN_POINT('Origin',(0.0318996984283249,4.01774292436015,-0.183314131582852));
#122019=CARTESIAN_POINT('Ctrl Pts',(-3.897588966,3.654941533,6.40771412100001));
#122020=CARTESIAN_POINT('Ctrl Pts',(-3.640019782,3.702826767,6.56438447000001));
#122021=CARTESIAN_POINT('Ctrl Pts',(-3.370706649,3.75,6.699875871));
#122022=CARTESIAN_POINT('Ctrl Pts',(-3.272032063,3.767283967,6.74951904200001));
#122023=CARTESIAN_POINT('Ctrl Pts',(-3.17193832,3.784676613,6.796234788));
#122024=CARTESIAN_POINT('Ctrl Pts',(-3.56250377,3.654941533,6.314354036));
#122025=CARTESIAN_POINT('Ctrl Pts',(-3.308687357,3.702826767,6.457555054));
#122026=CARTESIAN_POINT('Ctrl Pts',(-3.044195986,3.75,6.579921793));
#122027=CARTESIAN_POINT('Ctrl Pts',(-2.947288063,3.767283967,6.62475617200001));
#122028=CARTESIAN_POINT('Ctrl Pts',(-2.849101831,3.784676613,6.66671724));
#122029=CARTESIAN_POINT('',(-3.17193832006988,3.78467661264219,6.79623478881948));
#122030=CARTESIAN_POINT('',(-3.01052007105196,3.78467661221161,6.7314760159893));
#122031=CARTESIAN_POINT('',(-3.67974766537335,3.69493258296101,6.53524728790441));
#122032=CARTESIAN_POINT('Ctrl Pts',(-3.17193832115586,3.78467661270495,
6.79623478699001));
#122033=CARTESIAN_POINT('Ctrl Pts',(-3.23876371927838,3.77306479305815,
6.76504604108857));
#122034=CARTESIAN_POINT('Ctrl Pts',(-3.30503257260356,3.76150355535501,
6.73291648968132));
#122035=CARTESIAN_POINT('Ctrl Pts',(-3.37070664861055,3.75000000000425,
6.69987587087807));
#122036=CARTESIAN_POINT('Ctrl Pts',(-3.47472800982055,3.73177948527608,
6.6475427381026));
#122037=CARTESIAN_POINT('Ctrl Pts',(-3.57780328498725,3.71341418931372,
6.59264826720419));
#122038=CARTESIAN_POINT('Ctrl Pts',(-3.67974765917455,3.69493258479731,
6.53524729096345));
#122039=CARTESIAN_POINT('Ctrl Pts',(-3.55835094392697,3.65572482629106,
6.31669522493169));
#122040=CARTESIAN_POINT('Ctrl Pts',(-3.5785862593756,3.66259516175953,6.35304795193743));
#122041=CARTESIAN_POINT('Ctrl Pts',(-3.59883089848927,3.66929201740613,
6.3894582395044));
#122042=CARTESIAN_POINT('Ctrl Pts',(-3.63928868009484,3.68234999884861,
6.46229698630405));
#122043=CARTESIAN_POINT('Ctrl Pts',(-3.65952579260872,3.68871885429276,
6.49876860462018));
#122044=CARTESIAN_POINT('Ctrl Pts',(-3.67974767172092,3.69493258263467,
6.53524728444124));
#122045=CARTESIAN_POINT('Ctrl Pts',(-4.158549356,3.784676613,6.241511616));
#122046=CARTESIAN_POINT('Ctrl Pts',(-3.820674098,3.720089779,6.466628707));
#122047=CARTESIAN_POINT('Ctrl Pts',(-3.460471736,3.654947264,6.653956369));
#122048=CARTESIAN_POINT('Ctrl Pts',(-4.215638554,3.784676613,5.898380421));
#122049=CARTESIAN_POINT('Ctrl Pts',(-3.89633821,3.720089779,6.126587953));
#122050=CARTESIAN_POINT('Ctrl Pts',(-3.554268599,3.654947264,6.318993173));
#122051=CARTESIAN_POINT('',(-4.15854935856325,3.78467661255987,6.24151161603186));
#122052=CARTESIAN_POINT('Origin',(0.0835210236929956,3.62502542756177,-0.171210912967148));
#122053=CARTESIAN_POINT('',(-4.18709396168464,3.78467661169947,6.06994601388889));
#122054=CARTESIAN_POINT('Origin',(-1.94939550612894E-13,3.87542691999978,
3.09214459592866E-13));
#122055=CARTESIAN_POINT('',(-3.67628040958875,3.87435041277305,6.53719835590231));
#122056=CARTESIAN_POINT('Origin',(0.0543832873474687,3.62514703295402,-0.176631898517006));
#122057=CARTESIAN_POINT('Origin',(0.070561184785547,4.01774295255202,-0.172171126850401));
#122058=CARTESIAN_POINT('Ctrl Pts',(-5.183934627,3.654941533,5.42003891));
#122059=CARTESIAN_POINT('Ctrl Pts',(-4.966066761,3.702826767,5.62841615400001));
#122060=CARTESIAN_POINT('Ctrl Pts',(-4.732176666,3.75,5.818634204));
#122061=CARTESIAN_POINT('Ctrl Pts',(-4.646480852,3.767283967,5.888328864));
#122062=CARTESIAN_POINT('Ctrl Pts',(-4.558769749,3.784676613,5.95546961800001));
#122063=CARTESIAN_POINT('Ctrl Pts',(-4.836613879,3.654941533,5.400894943));
#122064=CARTESIAN_POINT('Ctrl Pts',(-4.619515538,3.702826767,5.59531102800001));
#122065=CARTESIAN_POINT('Ctrl Pts',(-4.38751306,3.75,5.771674726));
#122066=CARTESIAN_POINT('Ctrl Pts',(-4.302508856,3.767283967,5.836293242));
#122067=CARTESIAN_POINT('Ctrl Pts',(-4.215638554,3.784676613,5.898380421));
#122068=CARTESIAN_POINT('',(-4.55876974925585,3.784676612643,5.95546961878348));
#122069=CARTESIAN_POINT('',(-4.38720414758359,3.78467661221161,5.92692502239899));
#122070=CARTESIAN_POINT('',(-4.99860219645893,3.69493258290123,5.59141986218738));
#122071=CARTESIAN_POINT('Ctrl Pts',(-4.55876974991172,3.78467661270495,
5.95546961676514));
#122072=CARTESIAN_POINT('Ctrl Pts',(-4.6173281493066,3.77306479305815,5.91064456103513));
#122073=CARTESIAN_POINT('Ctrl Pts',(-4.67514076981802,3.76150355535487,
5.86502033620042));
#122074=CARTESIAN_POINT('Ctrl Pts',(-4.73217666580034,3.74999999996496,
5.81863420380783));
#122075=CARTESIAN_POINT('Ctrl Pts',(-4.82251598914285,3.73177948513261,
5.74516307240019));
#122076=CARTESIAN_POINT('Ctrl Pts',(-4.91138073268572,3.71341418923768,
5.66939386676725));
#122077=CARTESIAN_POINT('Ctrl Pts',(-4.99860219118283,3.69493258469624,
5.59141986640992));
#122078=CARTESIAN_POINT('Ctrl Pts',(-4.83306143014278,3.65572482629796,
5.404074131136));
#122079=CARTESIAN_POINT('Ctrl Pts',(-4.86063842297878,3.66259516332046,
5.43522696430087));
#122080=CARTESIAN_POINT('Ctrl Pts',(-4.88823689646622,3.66929202062442,
5.46643400910792));
#122081=CARTESIAN_POINT('Ctrl Pts',(-4.94340696137908,3.68234999884373,
5.52887258421955));
#122082=CARTESIAN_POINT('Ctrl Pts',(-4.97101126117534,3.6887188542611,5.56014113531008));
#122083=CARTESIAN_POINT('Ctrl Pts',(-4.9986022017914,3.6949325825822,5.59141985754699));
#122084=CARTESIAN_POINT('Ctrl Pts',(-5.403065283,3.784676613,5.201623357));
#122085=CARTESIAN_POINT('Ctrl Pts',(-5.121482881,3.720089779,5.494110528));
#122086=CARTESIAN_POINT('Ctrl Pts',(-4.80997176,3.654947264,5.754491434));
#122087=CARTESIAN_POINT('Ctrl Pts',(-5.385056702,3.784676613,4.854241888));
#122088=CARTESIAN_POINT('Ctrl Pts',(-5.122279297,3.720089779,5.145754191));
#122089=CARTESIAN_POINT('Ctrl Pts',(-4.829568519,3.654947264,5.407195939));
#122090=CARTESIAN_POINT('',(-5.40306528551253,3.78467661255987,5.2016233564748));
#122091=CARTESIAN_POINT('Origin',(0.118373689425329,3.62502544195215,-0.149253603691564));
#122092=CARTESIAN_POINT('',(-5.3940609980371,3.78467661169947,5.02793261655969));
#122093=CARTESIAN_POINT('Origin',(1.72171304990698E-13,3.87542691999967,
-5.76795555762288E-14));
#122094=CARTESIAN_POINT('',(-4.99563542483049,3.87435041277173,5.59407067324547));
#122095=CARTESIAN_POINT('Origin',(0.0910824517895525,3.62514697033697,-0.160811540126664));
#122096=CARTESIAN_POINT('Origin',(0.10592302656507,4.0177429632892,-0.152977109250126));
#122097=CARTESIAN_POINT('Ctrl Pts',(-6.227885267,3.654941533,4.178928703));
#122098=CARTESIAN_POINT('Ctrl Pts',(-6.05990597900001,3.702826767,4.429269354));
#122099=CARTESIAN_POINT('Ctrl Pts',(-5.872375362,3.75,4.665319669));
#122100=CARTESIAN_POINT('Ctrl Pts',(-5.803665359,3.767283967,4.751806974));
#122101=CARTESIAN_POINT('Ctrl Pts',(-5.732438171,3.784676613,4.836233308));
#122102=CARTESIAN_POINT('Ctrl Pts',(-5.884569297,3.654941533,4.234896006));
#122103=CARTESIAN_POINT('Ctrl Pts',(-5.714340306,3.702826767,4.471436477));
#122104=CARTESIAN_POINT('Ctrl Pts',(-5.5256749,3.75,4.693550565));
#122105=CARTESIAN_POINT('Ctrl Pts',(-5.456549118,3.767283967,4.774931727));
#122106=CARTESIAN_POINT('Ctrl Pts',(-5.385056702,3.784676613,4.854241888));
#122107=CARTESIAN_POINT('',(-5.73243817153119,3.78467661265427,4.8362333086525));
#122108=CARTESIAN_POINT('',(-5.55874743329835,3.78467661221161,4.84523760167313));
#122109=CARTESIAN_POINT('',(-6.08372764417876,3.69493258299157,4.38614385873408));
#122110=CARTESIAN_POINT('Ctrl Pts',(-5.73243817162459,3.78467661270495,
4.83623330659804));
#122111=CARTESIAN_POINT('Ctrl Pts',(-5.77999144574589,3.77306479305815,
4.7798679114699));
#122112=CARTESIAN_POINT('Ctrl Pts',(-5.8266445798002,3.76150355535494,4.72288235128597));
#122113=CARTESIAN_POINT('Ctrl Pts',(-5.87237536131112,3.74999999998527,
4.66531966898717));
#122114=CARTESIAN_POINT('Ctrl Pts',(-5.94480847923997,3.73177948523852,
4.57414596793933));
#122115=CARTESIAN_POINT('Ctrl Pts',(-6.01530747597372,3.71341418934238,
4.48104491092565));
#122116=CARTESIAN_POINT('Ctrl Pts',(-6.08372763978926,3.69493258484955,
4.38614386417697));
#122117=CARTESIAN_POINT('Ctrl Pts',(-5.88178333421816,3.65572482624985,
4.23876453771841));
#122118=CARTESIAN_POINT('Ctrl Pts',(-5.91541252772084,3.66259516269456,
4.26326079454881));
#122119=CARTESIAN_POINT('Ctrl Pts',(-5.94907435307606,3.6692920193845,4.28780537752084));
#122120=CARTESIAN_POINT('Ctrl Pts',(-6.01637702712757,3.68234999888808,
4.33692424506331));
#122121=CARTESIAN_POINT('Ctrl Pts',(-6.05005776801226,3.68871885432269,
4.36152764636592));
#122122=CARTESIAN_POINT('Ctrl Pts',(-6.08372764853543,3.69493258266148,
4.38614385285839));
#122123=CARTESIAN_POINT('Ctrl Pts',(-6.394939882,3.784676613,3.918512972));
#122124=CARTESIAN_POINT('Ctrl Pts',(-6.182816816,3.720089779,4.264693848));
#122125=CARTESIAN_POINT('Ctrl Pts',(-5.93456285000001,3.654947264,4.585952876));
#122126=CARTESIAN_POINT('Ctrl Pts',(-6.30267558499999,3.784676613,3.583124401));
#122127=CARTESIAN_POINT('Ctrl Pts',(-6.108708297,3.720089779,3.924310682));
#122128=CARTESIAN_POINT('Ctrl Pts',(-5.879043182,3.654947264,4.242564232));
#122129=CARTESIAN_POINT('',(-6.39493988502584,3.78467661255746,3.91851296839459));
#122130=CARTESIAN_POINT('Origin',(0.147691334653877,3.62502544960019,-0.120317321946553));
#122131=CARTESIAN_POINT('',(-6.34880773763066,3.78467661169947,3.75081867950825));
#122132=CARTESIAN_POINT('Origin',(6.5746019739521E-13,3.87542692000089,
-4.11129463806503E-13));
#122133=CARTESIAN_POINT('',(-6.08140007977474,3.87435041276949,4.38937046332155));
#122134=CARTESIAN_POINT('Origin',(0.123522468772804,3.62514698942111,-0.137471620475743));
#122135=CARTESIAN_POINT('Origin',(0.136332299683514,4.01774292398868,-0.126630361102386));
#122136=CARTESIAN_POINT('Ctrl Pts',(-6.980626913,3.654941533,2.742416435));
#122137=CARTESIAN_POINT('Ctrl Pts',(-6.87039072700001,3.702826767,3.023014843));
#122138=CARTESIAN_POINT('Ctrl Pts',(-6.737988312,3.75,3.293859971));
#122139=CARTESIAN_POINT('Ctrl Pts',(-6.689476925,3.767283967,3.39309587));
#122140=CARTESIAN_POINT('Ctrl Pts',(-6.638064156,3.784676613,3.490860104));
#122141=CARTESIAN_POINT('Ctrl Pts',(-6.657368796,3.654941533,2.870878039));
#122142=CARTESIAN_POINT('Ctrl Pts',(-6.541968873,3.702826767,3.138482526));
#122143=CARTESIAN_POINT('Ctrl Pts',(-6.405462322,3.75,3.395961195));
#122144=CARTESIAN_POINT('Ctrl Pts',(-6.355447207,3.767283967,3.49029971));
#122145=CARTESIAN_POINT('Ctrl Pts',(-6.302675585,3.784676613,3.583124401));
#122146=CARTESIAN_POINT('',(-6.63806415663382,3.78467661265215,3.49086010454012));
#122147=CARTESIAN_POINT('',(-6.47036986816281,3.78467661221161,3.53699225677551));
#122148=CARTESIAN_POINT('',(-6.8843847484949,3.69493258292739,2.9757766430664));
#122149=CARTESIAN_POINT('Ctrl Pts',(-6.63806415630895,3.78467661270495,
3.49086010249646));
#122150=CARTESIAN_POINT('Ctrl Pts',(-6.67238876700937,3.77306479305815,
3.42558995016941));
#122151=CARTESIAN_POINT('Ctrl Pts',(-6.70570096541578,3.76150355535494,
3.35990763583552));
#122152=CARTESIAN_POINT('Ctrl Pts',(-6.73798831140227,3.74999999998515,
3.29385997111107));
#122153=CARTESIAN_POINT('Ctrl Pts',(-6.78912833275206,3.73177948520444,
3.18924688147208));
#122154=CARTESIAN_POINT('Ctrl Pts',(-6.83796512675053,3.71341418927237,
3.0831672751429));
#122155=CARTESIAN_POINT('Ctrl Pts',(-6.88438474544995,3.69493258474057,
2.97577664917517));
#122156=CARTESIAN_POINT('Ctrl Pts',(-6.65547958725748,3.6557248262485,2.87525502630231));
#122157=CARTESIAN_POINT('Ctrl Pts',(-6.69358851777076,3.66259516228845,
2.89194929059024));
#122158=CARTESIAN_POINT('Ctrl Pts',(-6.73173970549951,3.66929201854781,
2.90868373622512));
#122159=CARTESIAN_POINT('Ctrl Pts',(-6.80802798946081,3.68234999883,2.94218614845776));
#122160=CARTESIAN_POINT('Ctrl Pts',(-6.84621029730883,3.68871885426788,
2.95897397227035));
#122161=CARTESIAN_POINT('Ctrl Pts',(-6.88438475141514,3.69493258260516,
2.97577663655099));
#122162=CARTESIAN_POINT('Ctrl Pts',(-7.0877942,3.784676613,2.452177274));
#122163=CARTESIAN_POINT('Ctrl Pts',(-6.955049108,3.720089779,2.835864823));
#122164=CARTESIAN_POINT('Ctrl Pts',(-6.781660377,3.654947264,3.202980258));
#122165=CARTESIAN_POINT('Ctrl Pts',(-6.925588362,3.784676613,2.144463998));
#122166=CARTESIAN_POINT('Ctrl Pts',(-6.809500887,3.720089779,2.519370767));
#122167=CARTESIAN_POINT('Ctrl Pts',(-6.65362032,3.654947264,2.879554937));
#122168=CARTESIAN_POINT('',(-7.0877942021837,3.78467661255747,2.45217726983537));
#122169=CARTESIAN_POINT('Origin',(0.170103244611084,3.62502542055922,-0.0857551768533432));
#122170=CARTESIAN_POINT('',(-7.00669128353107,3.78467661169947,2.29832062828375));
#122171=CARTESIAN_POINT('Origin',(-1.05991604382183E-12,3.87542691999911,
5.15212872365112E-13));
#122172=CARTESIAN_POINT('',(-6.88280522652425,3.87435041281037,2.97942816863292));
#122173=CARTESIAN_POINT('Origin',(0.150187169775698,3.62514698409845,-0.107704045563386));
#122174=CARTESIAN_POINT('Origin',(0.160366692848825,4.01774291427557,-0.0943623854139694));
#122175=CARTESIAN_POINT('Ctrl Pts',(-7.406962203,3.654941533,1.177671822));
#122176=CARTESIAN_POINT('Ctrl Pts',(-7.359623641,3.702826767,1.475407516));
#122177=CARTESIAN_POINT('Ctrl Pts',(-7.288540418,3.75,1.768383042));
#122178=CARTESIAN_POINT('Ctrl Pts',(-7.262495985,3.767283967,1.875727375));
#122179=CARTESIAN_POINT('Ctrl Pts',(-7.23330163800001,3.784676613,1.982258161));
#122180=CARTESIAN_POINT('Ctrl Pts',(-7.118877129,3.654941533,1.372621005));
#122181=CARTESIAN_POINT('Ctrl Pts',(-7.063702247,3.702826767,1.65877662));
#122182=CARTESIAN_POINT('Ctrl Pts',(-6.985737446,3.75,1.939580454));
#122183=CARTESIAN_POINT('Ctrl Pts',(-6.957171648,3.767283967,2.042465159));
#122184=CARTESIAN_POINT('Ctrl Pts',(-6.92558836200001,3.784676613,2.144463998));
#122185=CARTESIAN_POINT('',(-7.23330163873809,3.78467661265248,1.98225816138796));
#122186=CARTESIAN_POINT('',(-7.07944499863657,3.78467661221161,2.06336108417798));
#122187=CARTESIAN_POINT('',(-7.36313567399622,3.69493258296679,1.42626541837353));
#122188=CARTESIAN_POINT('Ctrl Pts',(-7.23330163797819,3.78467661270495,
1.98225815946538));
#122189=CARTESIAN_POINT('Ctrl Pts',(-7.25279260523575,3.77306479305815,
1.9111352104377));
#122190=CARTESIAN_POINT('Ctrl Pts',(-7.27120622711416,3.76150355535477,
1.83982737421093));
#122191=CARTESIAN_POINT('Ctrl Pts',(-7.28854041727107,3.74999999993373,
1.76838304205702));
#122192=CARTESIAN_POINT('Ctrl Pts',(-7.31599609085907,3.73177948507314,
1.65522215470338));
#122193=CARTESIAN_POINT('Ctrl Pts',(-7.3408871284668,3.71341418929527,1.54112416376592));
#122194=CARTESIAN_POINT('Ctrl Pts',(-7.36313567231283,3.69493258480758,
1.42626542509399));
#122195=CARTESIAN_POINT('Ctrl Pts',(-7.11797301180835,3.65572482627641,
1.37730178494789));
#122196=CARTESIAN_POINT('Ctrl Pts',(-7.15877975551595,3.66259516323431,
1.38541345409399));
#122197=CARTESIAN_POINT('Ctrl Pts',(-7.19963640720115,3.66929202046406,
1.39355528123289));
#122198=CARTESIAN_POINT('Ctrl Pts',(-7.28134313014978,3.68234999887737,
1.40987469711569));
#122199=CARTESIAN_POINT('Ctrl Pts',(-7.32224164272322,3.68871885430734,
1.41806196326326));
#122200=CARTESIAN_POINT('Ctrl Pts',(-7.3631356754694,3.69493258263972,1.42626541127745));
#122201=CARTESIAN_POINT('Ctrl Pts',(-7.449231138,3.784676613,0.871180493));
#122202=CARTESIAN_POINT('Ctrl Pts',(-7.402071035,3.720089779,1.274433911));
#122203=CARTESIAN_POINT('Ctrl Pts',(-7.311655002,3.654947264,1.670239842));
#122204=CARTESIAN_POINT('Ctrl Pts',(-7.224668324,3.784676613,0.605530843));
#122205=CARTESIAN_POINT('Ctrl Pts',(-7.191888783,3.720089779,0.996627876));
#122206=CARTESIAN_POINT('Ctrl Pts',(-7.117081567,3.654947264,1.381900854));
#122207=CARTESIAN_POINT('',(-7.44923113925812,3.78467661255747,0.871180488487826));
#122208=CARTESIAN_POINT('Origin',(0.184560763367131,3.6250254182926,-0.0471830310168703));
#122209=CARTESIAN_POINT('',(-7.33694973181313,3.78467661169947,0.738355659920048));
#122210=CARTESIAN_POINT('Origin',(-9.93129189996722E-13,3.87542691999967,
2.2253249590265E-13));
#122211=CARTESIAN_POINT('',(-7.36237804979258,3.87435041279178,1.43017112447896));
#122212=CARTESIAN_POINT('Origin',(0.169829105002478,3.62514697679868,-0.072900190738982));
#122213=CARTESIAN_POINT('Origin',(0.176902520092889,4.01774291269509,-0.0576821437523266));
#122214=CARTESIAN_POINT('Ctrl Pts',(-7.486956173,3.654941533,-0.442139416));
#122215=CARTESIAN_POINT('Ctrl Pts',(-7.504728734,3.702826767,-0.141188225));
#122216=CARTESIAN_POINT('Ctrl Pts',(-7.498288474,3.75,0.160218487));
#122217=CARTESIAN_POINT('Ctrl Pts',(-7.49592880400001,3.767283967,0.270651952));
#122218=CARTESIAN_POINT('Ctrl Pts',(-7.490317975,3.784676613,0.380968029));
#122219=CARTESIAN_POINT('Ctrl Pts',(-7.247514679,3.654941533,-0.189818262));
#122220=CARTESIAN_POINT('Ctrl Pts',(-7.255144754,3.702826767,0.101508163));
#122221=CARTESIAN_POINT('Ctrl Pts',(-7.23936725,3.75,0.392507087));
#122222=CARTESIAN_POINT('Ctrl Pts',(-7.23358647600001,3.767283967,0.499127207));
#122223=CARTESIAN_POINT('Ctrl Pts',(-7.224668324,3.784676613,0.605530843));
#122224=CARTESIAN_POINT('',(-7.49031797580076,3.78467661265198,0.380968029226118));
#122225=CARTESIAN_POINT('',(-7.35749314917407,3.78467661221161,0.493249440861707));
#122226=CARTESIAN_POINT('',(-7.49759455824446,3.69493258292492,-0.189936391004461));
#122227=CARTESIAN_POINT('Ctrl Pts',(-7.49031797464904,3.78467661270495,
0.380968027505726));
#122228=CARTESIAN_POINT('Ctrl Pts',(-7.49406392197607,3.77306479305815,
0.307317911724217));
#122229=CARTESIAN_POINT('Ctrl Pts',(-7.49671796648463,3.76150355535484,
0.233718828824487));
#122230=CARTESIAN_POINT('Ctrl Pts',(-7.49828847349936,3.7499999999552,0.16021848716836));
#122231=CARTESIAN_POINT('Ctrl Pts',(-7.50077600364447,3.73177948513637,
0.04380108050615));
#122232=CARTESIAN_POINT('Ctrl Pts',(-7.50055740678639,3.71341418928101,
-0.0729801998009269));
#122233=CARTESIAN_POINT('Ctrl Pts',(-7.49759455804428,3.69493258473592,
-0.189936384188764));
#122234=CARTESIAN_POINT('Ctrl Pts',(-7.24763792913635,3.65572482635196,
-0.185052557384502));
#122235=CARTESIAN_POINT('Ctrl Pts',(-7.28923440487671,3.66259516360214,
-0.185902778062423));
#122236=CARTESIAN_POINT('Ctrl Pts',(-7.33088610520975,3.66929202115375,
-0.186734274564594));
#122237=CARTESIAN_POINT('Ctrl Pts',(-7.4141907581793,3.68234999887337,-0.188360927321621));
#122238=CARTESIAN_POINT('Ctrl Pts',(-7.45589310641358,3.68871885428542,
-0.189157045999112));
#122239=CARTESIAN_POINT('Ctrl Pts',(-7.49759455815914,3.69493258260301,
-0.189936398136369));
#122240=CARTESIAN_POINT('Ctrl Pts',(-7.462350308,3.784676613,-0.750551720000001));
#122241=CARTESIAN_POINT('Ctrl Pts',(-7.502980346,3.720089779,-0.346588114));
#122242=CARTESIAN_POINT('Ctrl Pts',(-7.49976476500001,3.654947264,0.059400869));
#122243=CARTESIAN_POINT('Ctrl Pts',(-7.185930826,3.784676613,-0.961716262));
#122244=CARTESIAN_POINT('Ctrl Pts',(-7.237991953,3.720089779,-0.572716228));
#122245=CARTESIAN_POINT('Ctrl Pts',(-7.24775599,3.654947264,-0.180369377));
#122246=CARTESIAN_POINT('',(-7.46235030922085,3.78467661255987,-0.750551722266326));
#122247=CARTESIAN_POINT('Origin',(0.190388983462796,3.62502540451372,-0.0064048087139305));
#122248=CARTESIAN_POINT('',(-7.32414056605717,3.78467661169947,-0.856133999065892));
#122249=CARTESIAN_POINT('Origin',(1.04343617080005E-12,3.87542692000022,
-3.97089045672816E-14));
#122250=CARTESIAN_POINT('',(-7.49769425871509,3.87435041278221,-0.185959132095994));
#122251=CARTESIAN_POINT('Origin',(0.18153000267657,3.62514693102631,-0.0346875952443603));
#122252=CARTESIAN_POINT('Origin',(0.185166703032014,4.01774291708685,-0.0183047507880639));
#122253=CARTESIAN_POINT('Ctrl Pts',(-7.216868393,3.654941533,-2.041276707));
#122254=CARTESIAN_POINT('Ctrl Pts',(-7.298921051,3.702826767,-1.751182163));
#122255=CARTESIAN_POINT('Ctrl Pts',(-7.357424895,3.75,-1.455437707));
#122256=CARTESIAN_POINT('Ctrl Pts',(-7.37886032399999,3.767283967,-1.347078855));
#122257=CARTESIAN_POINT('Ctrl Pts',(-7.397095368,3.784676613,-1.238135744));
#122258=CARTESIAN_POINT('Ctrl Pts',(-7.037266498,3.654941533,-1.743381837));
#122259=CARTESIAN_POINT('Ctrl Pts',(-7.10734475600001,3.702826767,-1.460506703));
#122260=CARTESIAN_POINT('Ctrl Pts',(-7.154492288,3.75,-1.172919475));
#122261=CARTESIAN_POINT('Ctrl Pts',(-7.171766839,3.767283967,-1.067549379));
#122262=CARTESIAN_POINT('Ctrl Pts',(-7.185930826,3.784676613,-0.961716262));
#122263=CARTESIAN_POINT('',(-7.39709536883232,3.78467661265234,-1.23813574395619));
#122264=CARTESIAN_POINT('',(-7.29151309772682,3.78467661221161,-1.09992599818185));
#122265=CARTESIAN_POINT('',(-7.28147425473844,3.69493258302597,-1.79725698725771));
#122266=CARTESIAN_POINT('Ctrl Pts',(-7.39709536733601,3.78467661270495,
-1.23813574538389));
#122267=CARTESIAN_POINT('Ctrl Pts',(-7.38492113915177,3.77306479305815,
-1.31086923046358));
#122268=CARTESIAN_POINT('Ctrl Pts',(-7.37169150633935,3.76150355535505,
-1.38331814913354));
#122269=CARTESIAN_POINT('Ctrl Pts',(-7.35742489468756,3.75000000001838,
-1.45543770641804));
#122270=CARTESIAN_POINT('Ctrl Pts',(-7.33482796656171,3.73177948531458,
-1.5696680836393));
#122271=CARTESIAN_POINT('Ctrl Pts',(-7.30950995692274,3.71341418935042,
-1.68367209139032));
#122272=CARTESIAN_POINT('Ctrl Pts',(-7.28147425606393,3.69493258490811,
-1.79725698030097));
#122273=CARTESIAN_POINT('Ctrl Pts',(-7.03841135207602,3.65572482629248,
-1.73875404728258));
#122274=CARTESIAN_POINT('Ctrl Pts',(-7.07885255327227,3.66259516359781,
-1.74852640327108));
#122275=CARTESIAN_POINT('Ctrl Pts',(-7.11935171309557,3.66929202120471,
-1.75829234449999));
#122276=CARTESIAN_POINT('Ctrl Pts',(-7.20035906707951,3.6823499989136,-1.77778900530806));
#122277=CARTESIAN_POINT('Ctrl Pts',(-7.24091529565991,3.68871885434777,
-1.78753128353635));
#122278=CARTESIAN_POINT('Ctrl Pts',(-7.28147425305936,3.69493258269165,
-1.79725699447353));
#122279=CARTESIAN_POINT('Ctrl Pts',(-7.126538271,3.784676613,-2.337188968));
#122280=CARTESIAN_POINT('Ctrl Pts',(-7.253058636,3.720089779,-1.951404065));
#122281=CARTESIAN_POINT('Ctrl Pts',(-7.337193864,3.654947264,-1.554215624));
#122282=CARTESIAN_POINT('Ctrl Pts',(-6.811187188,3.784676613,-2.483994583));
#122283=CARTESIAN_POINT('Ctrl Pts',(-6.945654664,3.720089779,-2.115280757));
#122284=CARTESIAN_POINT('Ctrl Pts',(-7.039533398,3.654947264,-1.734205737));
#122285=CARTESIAN_POINT('',(-7.12653827171353,3.78467661255986,-2.33718897046504));
#122286=CARTESIAN_POINT('Origin',(0.187314493622497,3.62502543456919,0.0346729102936216));
#122287=CARTESIAN_POINT('',(-6.96886272684527,3.78467661169947,-2.41059178317464));
#122288=CARTESIAN_POINT('Origin',(-7.80625564189563E-15,3.87542691999945,
-1.14925430283463E-14));
#122289=CARTESIAN_POINT('',(-7.2824266169875,3.87435041280466,-1.79339414632136));
#122290=CARTESIAN_POINT('Origin',(0.184742667813114,3.62514698225076,0.00514695786445446));
#122291=CARTESIAN_POINT('Origin',(0.184772441726333,4.01774288341306,0.0219285383710868));
#122292=CARTESIAN_POINT('Ctrl Pts',(-6.609327869,3.654941533,-3.544966167));
#122293=CARTESIAN_POINT('Ctrl Pts',(-6.75182393300001,3.702826767,-3.279292768));
#122294=CARTESIAN_POINT('Ctrl Pts',(-6.872536305,3.75,-3.00303925));
#122295=CARTESIAN_POINT('Ctrl Pts',(-6.916764535,3.767283967,-2.901821752));
#122296=CARTESIAN_POINT('Ctrl Pts',(-6.957992803,3.784676613,-2.799345666));
#122297=CARTESIAN_POINT('Ctrl Pts',(-6.497963557,3.654941533,-3.215426816));
#122298=CARTESIAN_POINT('Ctrl Pts',(-6.62721321600001,3.702826767,-2.954229899));
#122299=CARTESIAN_POINT('Ctrl Pts',(-6.735081219,3.75,-2.683501626));
#122300=CARTESIAN_POINT('Ctrl Pts',(-6.77460335600001,3.767283967,-2.584308542));
#122301=CARTESIAN_POINT('Ctrl Pts',(-6.811187188,3.784676613,-2.483994583));
#122302=CARTESIAN_POINT('',(-6.95799280382198,3.78467661265224,-2.79934566613447));
#122303=CARTESIAN_POINT('',(-6.88458999724559,3.78467661221161,-2.64167011995074));
#122304=CARTESIAN_POINT('',(-6.72488030715598,3.69493258291181,-3.3205398430634));
#122305=CARTESIAN_POINT('Ctrl Pts',(-6.95799280205389,3.78467661270495,
-2.79934566720847));
#122306=CARTESIAN_POINT('Ctrl Pts',(-6.93046765080907,3.77306479305815,
-2.86776158452025));
#122307=CARTESIAN_POINT('Ctrl Pts',(-6.90197294353504,3.76150355535485,
-2.9356727074718));
#122308=CARTESIAN_POINT('Ctrl Pts',(-6.87253630462734,3.74999999995688,
-3.00303924964273));
#122309=CARTESIAN_POINT('Ctrl Pts',(-6.82591152545913,3.73177948512204,
-3.10974131322218));
#122310=CARTESIAN_POINT('Ctrl Pts',(-6.77667794548035,3.71341418925438,
-3.21563734638589));
#122311=CARTESIAN_POINT('Ctrl Pts',(-6.72488030982493,3.69493258471435,
-3.32053983682491));
#122312=CARTESIAN_POINT('Ctrl Pts',(-6.5000764830721,3.65572482634468,-3.21115333069244));
#122313=CARTESIAN_POINT('Ctrl Pts',(-6.53747141465312,3.6625951619445,-3.22939087267071));
#122314=CARTESIAN_POINT('Ctrl Pts',(-6.57492432725294,3.66929201774574,
-3.24763460849258));
#122315=CARTESIAN_POINT('Ctrl Pts',(-6.64984658820229,3.68234999883056,
-3.28408964402176));
#122316=CARTESIAN_POINT('Ctrl Pts',(-6.68736033292733,3.68871885425686,
-3.30232254341066));
#122317=CARTESIAN_POINT('Ctrl Pts',(-6.7248803040988,3.69493258259148,-3.32053984946918));
#122318=CARTESIAN_POINT('Ctrl Pts',(-6.457497225,3.784676613,-3.814541858));
#122319=CARTESIAN_POINT('Ctrl Pts',(-6.663991964,3.720089779,-3.46497453));
#122320=CARTESIAN_POINT('Ctrl Pts',(-6.83154393200001,3.654947264,-3.095158721));
#122321=CARTESIAN_POINT('Ctrl Pts',(-6.117960008,3.784676613,-3.890124078));
#122322=CARTESIAN_POINT('Ctrl Pts',(-6.328546282,3.720089779,-3.558937109));
#122323=CARTESIAN_POINT('Ctrl Pts',(-6.502150048,3.654947264,-3.206952564));
#122324=CARTESIAN_POINT('',(-6.45749722517541,3.78467661255985,-3.8145418605538));
#122325=CARTESIAN_POINT('Origin',(0.175481749935874,3.62502544254973,0.0741294711214169));
#122326=CARTESIAN_POINT('',(-6.28772861225752,3.78467661169946,-3.85233297492452));
#122327=CARTESIAN_POINT('Origin',(-2.54136989230602E-13,3.87542692000067,
-1.61762964134837E-13));
#122328=CARTESIAN_POINT('',(-6.72664080054465,3.87435041277593,-3.3169720436542));
#122329=CARTESIAN_POINT('Origin',(0.179317325669673,3.62514694770728,0.0447409567355106));
#122330=CARTESIAN_POINT('Origin',(0.175738402230885,4.01774290648807,0.0611363810192611));
#122331=CARTESIAN_POINT('Ctrl Pts',(-5.692742518,3.654941533,-4.882896949));
#122332=CARTESIAN_POINT('Ctrl Pts',(-5.889019031,3.702826767,-4.654067289));
#122333=CARTESIAN_POINT('Ctrl Pts',(-6.066295556,3.75,-4.410222016));
#122334=CARTESIAN_POINT('Ctrl Pts',(-6.131248525,3.767283967,-4.320878689));
#122335=CARTESIAN_POINT('Ctrl Pts',(-6.193542228,3.784676613,-4.229661295));
#122336=CARTESIAN_POINT('Ctrl Pts',(-5.654823062,3.654941533,-4.53712201));
#122337=CARTESIAN_POINT('Ctrl Pts',(-5.837200552,3.702826767,-4.309816588));
#122338=CARTESIAN_POINT('Ctrl Pts',(-6.000745237,3.75,-4.068606224));
#122339=CARTESIAN_POINT('Ctrl Pts',(-6.06066694900001,3.767283967,-3.98022831));
#122340=CARTESIAN_POINT('Ctrl Pts',(-6.117960008,3.784676613,-3.890124078));
#122341=CARTESIAN_POINT('',(-6.19354222877282,3.78467661265299,-4.22966129531913));
#122342=CARTESIAN_POINT('',(-6.15575112068274,3.78467661221161,-4.05989268243235));
#122343=CARTESIAN_POINT('',(-5.8538384305328,3.69493258295246,-4.68855794658045));
#122344=CARTESIAN_POINT('Ctrl Pts',(-6.1935422268163,3.78467661270495,-4.22966129597718));
#122345=CARTESIAN_POINT('Ctrl Pts',(-6.15195319866575,3.77306479305815,
-4.29056059385924));
#122346=CARTESIAN_POINT('Ctrl Pts',(-6.10952579781268,3.76150355535484,
-4.35075847299217));
#122347=CARTESIAN_POINT('Ctrl Pts',(-6.06629555573076,3.74999999995653,
-4.41022201567284));
#122348=CARTESIAN_POINT('Ctrl Pts',(-5.99782304821393,3.73177948514419,
-4.50440649522614));
#122349=CARTESIAN_POINT('Ctrl Pts',(-5.92697600490363,3.71341418929997,
-4.59724297326434));
#122350=CARTESIAN_POINT('Ctrl Pts',(-5.85383843453696,3.69493258478171,
-4.68855794097464));
#122351=CARTESIAN_POINT('Ctrl Pts',(-5.6578052618491,3.65572482628151,-4.53340265369335));
#122352=CARTESIAN_POINT('Ctrl Pts',(-5.69040539293398,3.66259516290112,
-4.5592526205251));
#122353=CARTESIAN_POINT('Ctrl Pts',(-5.72306081877124,3.66929201977292,
-4.58512110127768));
#122354=CARTESIAN_POINT('Ctrl Pts',(-5.78839467372621,3.68234999888282,
-4.63682990164374));
#122355=CARTESIAN_POINT('Ctrl Pts',(-5.82111183342389,3.6887188543046,-4.66270087208794));
#122356=CARTESIAN_POINT('Ctrl Pts',(-5.85383842610379,3.69493258262724,
-4.68855795226429));
#122357=CARTESIAN_POINT('Ctrl Pts',(-5.486510786,3.784676613,-5.11353101));
#122358=CARTESIAN_POINT('Ctrl Pts',(-5.763324435,3.720089779,-4.816526637));
#122359=CARTESIAN_POINT('Ctrl Pts',(-6.006458598,3.654947264,-4.491375636));
#122360=CARTESIAN_POINT('Ctrl Pts',(-5.138663817,3.784676613,-5.114355695));
#122361=CARTESIAN_POINT('Ctrl Pts',(-5.41552211,3.720089779,-4.836181517));
#122362=CARTESIAN_POINT('Ctrl Pts',(-5.660733389,3.654947264,-4.529745854));
#122363=CARTESIAN_POINT('',(-5.48651078539378,3.78467661259838,-5.11353101337042));
#122364=CARTESIAN_POINT('Origin',(0.155443362235889,3.62502545473262,0.110119686174778));
#122365=CARTESIAN_POINT('',(-5.31258729586815,3.78467661169946,-5.11394335885062));
#122366=CARTESIAN_POINT('Origin',(4.09828421199521E-13,3.87542691999967,
3.73832909073002E-13));
#122367=CARTESIAN_POINT('',(-5.85632473619676,3.8743504128077,-4.68545201434567));
#122368=CARTESIAN_POINT('Origin',(0.165506588395413,3.62514705308022,0.0822425757635481));
#122369=CARTESIAN_POINT('Origin',(0.158487625325135,4.01774296008671,0.0974859321624588));
#122370=CARTESIAN_POINT('Ctrl Pts',(-4.509970855,3.654941533,-5.992508897));
#122371=CARTESIAN_POINT('Ctrl Pts',(-4.75085014500001,3.702826767,-5.811222796));
#122372=CARTESIAN_POINT('Ctrl Pts',(-4.976401568,3.75,-5.611187702));
#122373=CARTESIAN_POINT('Ctrl Pts',(-5.059042148,3.767283967,-5.537896141));
#122374=CARTESIAN_POINT('Ctrl Pts',(-5.139488502,3.784676613,-5.462202664));
#122375=CARTESIAN_POINT('Ctrl Pts',(-4.54726932600001,3.654941533,-5.646666422));
#122376=CARTESIAN_POINT('Ctrl Pts',(-4.77424687800001,3.702826767,-5.463881043));
#122377=CARTESIAN_POINT('Ctrl Pts',(-4.985821077,3.75,-5.263467316));
#122378=CARTESIAN_POINT('Ctrl Pts',(-5.063340492,3.767283967,-5.190037026));
#122379=CARTESIAN_POINT('Ctrl Pts',(-5.138663817,3.784676613,-5.114355695));
#122380=CARTESIAN_POINT('',(-5.13948850268994,3.78467661265216,-5.46220266446606));
#122381=CARTESIAN_POINT('',(-5.13907616299444,3.78467661221161,-5.28827917610415));
#122382=CARTESIAN_POINT('',(-4.70907757523346,3.6949325829312,-5.83734429200579));
#122383=CARTESIAN_POINT('Ctrl Pts',(-5.13948850063391,3.78467661270495,
-5.46220266469957));
#122384=CARTESIAN_POINT('Ctrl Pts',(-5.0857802520988,3.77306479305815,-5.51273775897462));
#122385=CARTESIAN_POINT('Ctrl Pts',(-5.03140401545385,3.76150355535523,
-5.56240760790579));
#122386=CARTESIAN_POINT('Ctrl Pts',(-4.97640156835124,3.75000000007195,
-5.61118770142894));
#122387=CARTESIAN_POINT('Ctrl Pts',(-4.88928303217232,3.73177948542768,
-5.68845063510256));
#122388=CARTESIAN_POINT('Ctrl Pts',(-4.80013525362314,3.71341418927266,
-5.76388662848969));
#122389=CARTESIAN_POINT('Ctrl Pts',(-4.70907758031102,3.69493258474665,
-5.83734428743019));
#122390=CARTESIAN_POINT('Ctrl Pts',(-4.55098135569828,3.65572482635055,
-5.64367510635039));
#122391=CARTESIAN_POINT('Ctrl Pts',(-4.5772623290225,3.66259516142306,-5.67592877291498));
#122392=CARTESIAN_POINT('Ctrl Pts',(-4.60359332345062,3.66929201666084,
-5.70821240602175));
#122393=CARTESIAN_POINT('Ctrl Pts',(-4.65628385779129,3.6823499988366,-5.77275714643303));
#122394=CARTESIAN_POINT('Ctrl Pts',(-4.68267461454173,3.68871885427104,
-5.80505649036733));
#122395=CARTESIAN_POINT('Ctrl Pts',(-4.70907756972931,3.69493258260853,
-5.83734429656885));
#122396=CARTESIAN_POINT('Ctrl Pts',(-4.2589812,3.784676613,-6.173417136));
#122397=CARTESIAN_POINT('Ctrl Pts',(-4.593170261,3.720089779,-5.942863312));
#122398=CARTESIAN_POINT('Ctrl Pts',(-4.900517936,3.654947264,-5.677580819));
#122399=CARTESIAN_POINT('Ctrl Pts',(-3.919089417,3.784676613,-6.09944572399999));
#122400=CARTESIAN_POINT('Ctrl Pts',(-4.249274143,3.720089779,-5.887291453));
#122401=CARTESIAN_POINT('Ctrl Pts',(-4.554627128,3.654947264,-5.640733261));
#122402=CARTESIAN_POINT('',(-4.25898119661183,3.78467661255747,-6.1734171392271));
#122403=CARTESIAN_POINT('Origin',(0.128136702922485,3.62502543316226,0.140960870947283));
#122404=CARTESIAN_POINT('',(-4.08903530174211,3.78467661169946,-6.13643143450315));
#122405=CARTESIAN_POINT('Origin',(7.28150179041265E-13,3.87542691999978,
8.21391565875018E-13));
#122406=CARTESIAN_POINT('',(-4.71217343633271,3.87435041277489,-5.83484545661085));
#122407=CARTESIAN_POINT('Origin',(0.143957591579971,3.62514698264479,0.115899004331725));
#122408=CARTESIAN_POINT('Origin',(0.133825468097622,4.01774292011938,0.129276663896634));
#122409=CARTESIAN_POINT('Ctrl Pts',(-3.116317967,3.654941533,-6.82191779));
#122410=CARTESIAN_POINT('Ctrl Pts',(-3.390536786,3.702826767,-6.69665198300001));
#122411=CARTESIAN_POINT('Ctrl Pts',(-3.653816575,3.75,-6.549780488));
#122412=CARTESIAN_POINT('Ctrl Pts',(-3.750280582,3.767283967,-6.495967724));
#122413=CARTESIAN_POINT('Ctrl Pts',(-3.845118005,3.784676613,-6.439337507));
#122414=CARTESIAN_POINT('Ctrl Pts',(-3.22709033,3.654941533,-6.492178987));
#122415=CARTESIAN_POINT('Ctrl Pts',(-3.488054726,3.702826767,-6.362460494));
#122416=CARTESIAN_POINT('Ctrl Pts',(-3.737765465,3.75,-6.212214527));
#122417=CARTESIAN_POINT('Ctrl Pts',(-3.82925786,3.767283967,-6.157165379));
#122418=CARTESIAN_POINT('Ctrl Pts',(-3.919089417,3.784676613,-6.099445724));
#122419=CARTESIAN_POINT('',(-3.84511800556879,3.7846766126528,-6.43933750761177));
#122420=CARTESIAN_POINT('',(-3.88210371514274,3.78467661221161,-6.26939161293474));
#122421=CARTESIAN_POINT('',(-3.34412548649015,3.69493258295384,-6.71318290578519));
#122422=CARTESIAN_POINT('Ctrl Pts',(-3.8451180035154,3.78467661270495,-6.43933750738985));
#122423=CARTESIAN_POINT('Ctrl Pts',(-3.78180187253579,3.77306479305815,
-6.4771454331204));
#122424=CARTESIAN_POINT('Ctrl Pts',(-3.71801937323458,3.76150355535473,
-6.51396474519606));
#122425=CARTESIAN_POINT('Ctrl Pts',(-3.65381657476172,3.74999999992168,
-6.54978048744424));
#122426=CARTESIAN_POINT('Ctrl Pts',(-3.55212557335821,3.73177948505058,
-6.60650914605142));
#122427=CARTESIAN_POINT('Ctrl Pts',(-3.44884551331829,3.71341418929757,
-6.6610173506864));
#122428=CARTESIAN_POINT('Ctrl Pts',(-3.34412549248534,3.69493258478546,
-6.71318290238093));
#122429=CARTESIAN_POINT('Ctrl Pts',(-3.23135861816428,3.6557248262122,-6.49005558377445));
#122430=CARTESIAN_POINT('Ctrl Pts',(-3.2500915766167,3.66259516294686,-6.52720481884039));
#122431=CARTESIAN_POINT('Ctrl Pts',(-3.26886694552431,3.66929201994454,
-6.56439407440542));
#122432=CARTESIAN_POINT('Ctrl Pts',(-3.30645038375794,3.68234999883342,
-6.63875668313945));
#122433=CARTESIAN_POINT('Ctrl Pts',(-3.32528073514068,3.68871885427786,
-6.6759741189413));
#122434=CARTESIAN_POINT('Ctrl Pts',(-3.34412548007839,3.69493258262837,
-6.71318290908683));
#122435=CARTESIAN_POINT('Ctrl Pts',(-2.832306387,3.784676613,-6.944641137));
#122436=CARTESIAN_POINT('Ctrl Pts',(-3.208244551,3.720089779,-6.791318303));
#122437=CARTESIAN_POINT('Ctrl Pts',(-3.565434502,3.654947264,-6.598308633));
#122438=CARTESIAN_POINT('Ctrl Pts',(-2.516262752,3.784676613,-6.79933245));
#122439=CARTESIAN_POINT('Ctrl Pts',(-2.884334839,3.720089779,-6.663118183));
#122440=CARTESIAN_POINT('Ctrl Pts',(-3.235551564,3.654947264,-6.487966251));
#122441=CARTESIAN_POINT('',(-2.83230638302414,3.78467661255746,-6.94464113943562));
#122442=CARTESIAN_POINT('Origin',(0.0948385248949762,3.62502540108089,0.165210910142309));
#122443=CARTESIAN_POINT('',(-2.67428456193206,3.78467661169946,-6.87198679644513));
#122444=CARTESIAN_POINT('Origin',(-2.3787395664332E-13,3.87542691999945,
-7.92768628521401E-13));
#122445=CARTESIAN_POINT('',(-3.34768614346571,3.87435041276815,-6.71140801018691));
#122446=CARTESIAN_POINT('Origin',(0.115677207989847,3.62514695239622,0.144136193356513));
#122447=CARTESIAN_POINT('Origin',(0.102905937121066,4.01774294932997,0.155022531962715));
#122448=CARTESIAN_POINT('Ctrl Pts',(-1.576949515,3.654941533,-7.332341388));
#122449=CARTESIAN_POINT('Ctrl Pts',(-1.871685696,3.702826767,-7.268953167));
#122450=CARTESIAN_POINT('Ctrl Pts',(-2.160383179,3.75,-7.182112817));
#122451=CARTESIAN_POINT('Ctrl Pts',(-2.266160065,3.767283967,-7.150295076));
#122452=CARTESIAN_POINT('Ctrl Pts',(-2.370954065,3.784676613,-7.115376084));
#122453=CARTESIAN_POINT('Ctrl Pts',(-1.756016176,3.654941533,-7.034124479));
#122454=CARTESIAN_POINT('Ctrl Pts',(-2.038765011,3.702826767,-6.96353836300001));
#122455=CARTESIAN_POINT('Ctrl Pts',(-2.314936093,3.75,-6.870485491));
#122456=CARTESIAN_POINT('Ctrl Pts',(-2.416123388,3.767283967,-6.836391522));
#122457=CARTESIAN_POINT('Ctrl Pts',(-2.516262752,3.784676613,-6.79933245));
#122458=CARTESIAN_POINT('',(-2.37095406541212,3.78467661265402,-7.11537608473225));
#122459=CARTESIAN_POINT('',(-2.44360841309735,3.78467661221161,-6.95735426538529));
#122460=CARTESIAN_POINT('',(-1.82280580688747,3.69493258293707,-7.27512054808345));
#122461=CARTESIAN_POINT('Ctrl Pts',(-2.37095406346643,3.78467661270495,
-7.11537608406131));
#122462=CARTESIAN_POINT('Ctrl Pts',(-2.30099064162556,3.77306479305815,
-7.13868898533261));
#122463=CARTESIAN_POINT('Ctrl Pts',(-2.23078427769843,3.76150355535498,
-7.16093613044395));
#122464=CARTESIAN_POINT('Ctrl Pts',(-2.16038317911554,3.749999999997,-7.18211281673554));
#122465=CARTESIAN_POINT('Ctrl Pts',(-2.04887467270013,3.73177948523619,
-7.21565463245062));
#122466=CARTESIAN_POINT('Ctrl Pts',(-1.93629158990197,3.71341418927889,
-7.24668630494625));
#122467=CARTESIAN_POINT('Ctrl Pts',(-1.82280581343427,3.69493258475776,
-7.27512054606235));
#122468=CARTESIAN_POINT('Ctrl Pts',(-1.76064114319113,3.65572482631164,
-7.03296827586369));
#122469=CARTESIAN_POINT('Ctrl Pts',(-1.77095014868274,3.66259516333785,
-7.07327601647927));
#122470=CARTESIAN_POINT('Ctrl Pts',(-1.78129196996794,3.66929202064669,
-7.11363195929011));
#122471=CARTESIAN_POINT('Ctrl Pts',(-1.8020109648606,3.68234999887879,-7.19433533590008));
#122472=CARTESIAN_POINT('Ctrl Pts',(-1.81240042463632,3.68871885429569,
-7.2347306175881));
#122473=CARTESIAN_POINT('Ctrl Pts',(-1.8228057999587,3.69493258261361,-7.27512054991822));
#122474=CARTESIAN_POINT('Ctrl Pts',(-1.273196075,3.784676613,-7.391141438));
#122475=CARTESIAN_POINT('Ctrl Pts',(-1.673304891,3.720089779,-7.322218799));
#122476=CARTESIAN_POINT('Ctrl Pts',(-2.063635314,3.654947264,-7.210506868));
#122477=CARTESIAN_POINT('Ctrl Pts',(-0.995778438,3.784676613,-7.181289947));
#122478=CARTESIAN_POINT('Ctrl Pts',(-1.384527244,3.720089779,-7.127384913));
#122479=CARTESIAN_POINT('Ctrl Pts',(-1.765185206,3.654947264,-7.03182915));
#122480=CARTESIAN_POINT('',(-1.27319607054881,3.78467661255747,-7.39114143949019));
#122481=CARTESIAN_POINT('Origin',(0.0571057823865292,3.62502542317003,0.181735794487139));
#122482=CARTESIAN_POINT('',(-1.13448724847587,3.78467661169946,-7.28621569374938));
#122483=CARTESIAN_POINT('Origin',(1.40078920685127E-13,3.87542691999967,
2.1163626406917E-13));
#122484=CARTESIAN_POINT('',(-1.82666476757934,3.8743504127621,-7.27415258434626));
#122485=CARTESIAN_POINT('Origin',(0.0819875193912198,3.62514702744759,0.165632892872857));
#122486=CARTESIAN_POINT('Origin',(0.0671748843628595,4.01774297204972,0.173520298462304));
#122487=CARTESIAN_POINT('Ctrl Pts',(0.036155345,3.654941533,-7.499912852));
#122488=CARTESIAN_POINT('Ctrl Pts',(-0.265316662,3.702826767,-7.501366179));
#122489=CARTESIAN_POINT('Ctrl Pts',(-0.565932667,3.75,-7.478617534));
#122490=CARTESIAN_POINT('Ctrl Pts',(-0.676076422,3.767283967,-7.470282578));
#122491=CARTESIAN_POINT('Ctrl Pts',(-0.785926947,3.784676613,-7.458707585));
#122492=CARTESIAN_POINT('Ctrl Pts',(-0.202832658,3.654941533,-7.247162128));
#122493=CARTESIAN_POINT('Ctrl Pts',(-0.494144911,3.702826767,-7.23900891800001));
#122494=CARTESIAN_POINT('Ctrl Pts',(-0.783862884,3.75,-7.207500189));
#122495=CARTESIAN_POINT('Ctrl Pts',(-0.890013671,3.767283967,-7.195955596));
#122496=CARTESIAN_POINT('Ctrl Pts',(-0.995778438,3.784676613,-7.18128994700001));
#122497=CARTESIAN_POINT('',(-0.890852697336977,3.78467661221161,-7.31999876541133));
#122498=CARTESIAN_POINT('Ctrl Pts',(-0.20759804596496,3.65572482631731,
-7.24702718706223));
#122499=CARTESIAN_POINT('Ctrl Pts',(-0.209001059456919,3.66259516224294,
-7.2886086799602));
#122500=CARTESIAN_POINT('Ctrl Pts',(-0.210425759463657,3.66929201838331,
-7.33024430135007));
#122501=CARTESIAN_POINT('Ctrl Pts',(-0.213311515592496,3.68234999884975,
-7.4135148635547));
#122502=CARTESIAN_POINT('Ctrl Pts',(-0.214774283997655,3.68871885431118,
-7.45519915301341));
#122503=CARTESIAN_POINT('Ctrl Pts',(-0.216253745842927,3.69493258264677,
-7.49688163937647));
#122504=CARTESIAN_POINT('Ctrl Pts',(0.34544747,3.784676613,-7.49204017899999));
#122505=CARTESIAN_POINT('Ctrl Pts',(-0.060123354,3.720089779,-7.510740481));
#122506=CARTESIAN_POINT('Ctrl Pts',(-0.465342831,3.654947264,-7.485549816));
#122507=CARTESIAN_POINT('Ctrl Pts',(0.57126737,3.784676613,-7.227458308));
#122508=CARTESIAN_POINT('Ctrl Pts',(0.180019305,3.720089779,-7.258383046));
#122509=CARTESIAN_POINT('Ctrl Pts',(-0.212280749,3.654947264,-7.246891532));
#122510=CARTESIAN_POINT('',(0.458357428105106,3.78467661169946,-7.35974924299523));
#122511=CARTESIAN_POINT('Ctrl Pts',(1.64756962,3.654941533,-7.316796727));
#122512=CARTESIAN_POINT('Ctrl Pts',(1.353458284,3.702826767,-7.383023646));
#122513=CARTESIAN_POINT('Ctrl Pts',(1.054980228,3.75,-7.425430406));
#122514=CARTESIAN_POINT('Ctrl Pts',(0.945619802999998,3.767283967,-7.440967968));
#122515=CARTESIAN_POINT('Ctrl Pts',(0.835849241000001,3.784676613,-7.453278208));
#122516=CARTESIAN_POINT('Ctrl Pts',(1.35983509,3.654941533,-7.121330531));
#122517=CARTESIAN_POINT('Ctrl Pts',(1.073580856,3.702826767,-7.175991461));
#122518=CARTESIAN_POINT('Ctrl Pts',(0.783862884,3.75,-7.207500189));
#122519=CARTESIAN_POINT('Ctrl Pts',(0.677712097,3.767283967,-7.21904478299999));
#122520=CARTESIAN_POINT('Ctrl Pts',(0.57126737,3.784676613,-7.227458308));
#122521=CARTESIAN_POINT('',(0.835849240921721,3.78467661265316,-7.45327820883271));
#122522=CARTESIAN_POINT('',(0.703558300649563,3.78467661221161,-7.3403682584649));
#122523=CARTESIAN_POINT('',(1.40041008554965,3.69493258292194,-7.36809687647276));
#122524=CARTESIAN_POINT('Ctrl Pts',(0.835849242417206,3.78467661270495,
-7.45327820741139));
#122525=CARTESIAN_POINT('Ctrl Pts',(0.909135157053171,3.77306479305815,
-7.44505954502045));
#122526=CARTESIAN_POINT('Ctrl Pts',(0.982194061001742,3.76150355535505,
-7.43577161989865));
#122527=CARTESIAN_POINT('Ctrl Pts',(1.05498022756045,3.7500000000188,-7.42543040575917));
#122528=CARTESIAN_POINT('Ctrl Pts',(1.17026644958751,3.73177948530145,-7.40905092646273));
#122529=CARTESIAN_POINT('Ctrl Pts',(1.28547394979438,3.71341418927964,-7.38994210007725));
#122530=CARTESIAN_POINT('Ctrl Pts',(1.4004100787995,3.69493258473014,-7.36809687737378));
#122531=CARTESIAN_POINT('Ctrl Pts',(1.35515210599328,3.65572482629701,-7.12222316244251));
#122532=CARTESIAN_POINT('Ctrl Pts',(1.36272068683348,3.66259516309388,-7.163134114624));
#122533=CARTESIAN_POINT('Ctrl Pts',(1.37027972438359,3.66929202016128,-7.20410259268216));
#122534=CARTESIAN_POINT('Ctrl Pts',(1.38536214280068,3.68234999884869,-7.28604667629));
#122535=CARTESIAN_POINT('Ctrl Pts',(1.39289446304458,3.68871885427417,-7.32707086185062));
#122536=CARTESIAN_POINT('Ctrl Pts',(1.40041009256457,3.69493258260044,-7.36809687523637));
#122537=CARTESIAN_POINT('Ctrl Pts',(1.947938275,3.784676613,-7.242619448));
#122538=CARTESIAN_POINT('Ctrl Pts',(1.555869484,3.720089779,-7.348068286));
#122539=CARTESIAN_POINT('Ctrl Pts',(1.154708565,3.654947264,-7.410576774));
#122540=CARTESIAN_POINT('Ctrl Pts',(2.11160135,3.784676613,-6.935678751));
#122541=CARTESIAN_POINT('Ctrl Pts',(1.736148353,3.720089779,-7.049987254));
#122542=CARTESIAN_POINT('Ctrl Pts',(1.35054972,3.654947264,-7.123097322));
#122543=CARTESIAN_POINT('',(1.94793827739633,3.78467661255984,-7.24261944886446));
#122544=CARTESIAN_POINT('Origin',(-0.0244810821294403,3.62502541707946,
0.188917070851253));
#122545=CARTESIAN_POINT('',(2.0297698203071,3.78467661169946,-7.08914909726467));
#122546=CARTESIAN_POINT('Origin',(-9.24824453130135E-14,3.87542691999989,
-1.16226472890446E-13));
#122547=CARTESIAN_POINT('',(1.39650135063367,3.8743504127644,-7.36883871276101));
#122548=CARTESIAN_POINT('Origin',(0.00486236478177832,3.62514700919744,
0.184750327287636));
#122549=CARTESIAN_POINT('Origin',(-0.0118929950341548,4.01774294200309,
0.185688624677329));
#122550=CARTESIAN_POINT('Ctrl Pts',(3.181945371,3.654941533,-6.791555319));
#122551=CARTESIAN_POINT('Ctrl Pts',(2.908947024,3.702826767,-6.919459133));
#122552=CARTESIAN_POINT('Ctrl Pts',(2.62656342,3.75,-7.025038406));
#122553=CARTESIAN_POINT('Ctrl Pts',(2.523099898,3.767283967,-7.063721967));
#122554=CARTESIAN_POINT('Ctrl Pts',(2.418542048,3.784676613,-7.09934182600001));
#122555=CARTESIAN_POINT('Ctrl Pts',(2.85891846,3.654941533,-6.662513432));
#122556=CARTESIAN_POINT('Ctrl Pts',(2.591107176,3.702826767,-6.777432619));
#122557=CARTESIAN_POINT('Ctrl Pts',(2.314936093,3.75,-6.870485491));
#122558=CARTESIAN_POINT('Ctrl Pts',(2.213748799,3.767283967,-6.90457946));
#122559=CARTESIAN_POINT('Ctrl Pts',(2.11160135,3.784676613,-6.935678751));
#122560=CARTESIAN_POINT('',(2.41854204810109,3.78467661265302,-7.09934182683003));
#122561=CARTESIAN_POINT('',(2.26507169436299,3.78467661221163,-7.0175102899967));
#122562=CARTESIAN_POINT('',(2.95159230542166,3.69493258288868,-6.89478809371964));
#122563=CARTESIAN_POINT('Ctrl Pts',(2.4185420492583,3.78467661270494,-7.09934182512084));
#122564=CARTESIAN_POINT('Ctrl Pts',(2.48834781076507,3.77306479305814,-7.07556100546958));
#122565=CARTESIAN_POINT('Ctrl Pts',(2.55770200877317,3.76150355535497,-7.050784722334));
#122566=CARTESIAN_POINT('Ctrl Pts',(2.62656341956181,3.74999999999367,-7.0250384057497));
#122567=CARTESIAN_POINT('Ctrl Pts',(2.73563320979076,3.73177948519891,-6.98425873926709));
#122568=CARTESIAN_POINT('Ctrl Pts',(2.84403938978583,3.71341418922258,-6.94083045977405));
#122569=CARTESIAN_POINT('Ctrl Pts',(2.95159229910395,3.69493258467529,-6.8947880960262));
#122570=CARTESIAN_POINT('Ctrl Pts',(2.85453685143343,3.65572482630255,-6.66439189757751));
#122571=CARTESIAN_POINT('Ctrl Pts',(2.87072312912744,3.66259516339516,-6.70271935502675));
#122572=CARTESIAN_POINT('Ctrl Pts',(2.88691245315828,3.66929202076924,-6.74110504524683));
#122573=CARTESIAN_POINT('Ctrl Pts',(2.91925780735638,3.68234999885248,-6.81789104437783));
#122574=CARTESIAN_POINT('Ctrl Pts',(2.93543301341889,3.68871885426192,-6.85633688116857));
#122575=CARTESIAN_POINT('Ctrl Pts',(2.95159231192568,3.69493258257117,-6.8947880910376));
#122576=CARTESIAN_POINT('Ctrl Pts',(3.459345652,3.784676613,-6.654541882));
#122577=CARTESIAN_POINT('Ctrl Pts',(3.099111595,3.720089779,-6.84180858500001));
#122578=CARTESIAN_POINT('Ctrl Pts',(2.720767072,3.654947264,-6.989093399));
#122579=CARTESIAN_POINT('Ctrl Pts',(3.553199198,3.784676613,-6.319594564));
#122580=CARTESIAN_POINT('Ctrl Pts',(3.211097032,3.720089779,-6.511941894));
#122581=CARTESIAN_POINT('Ctrl Pts',(2.850229985,3.654947264,-6.66623499700001));
#122582=CARTESIAN_POINT('',(3.45934565454573,3.78467661255985,-6.65454188230779));
#122583=CARTESIAN_POINT('Origin',(-0.0645203334186512,3.62502544807729,
0.179237618766572));
#122584=CARTESIAN_POINT('',(3.50627243214405,3.78467661169946,-6.48706821913863));
#122585=CARTESIAN_POINT('Origin',(7.61109925084824E-14,3.87542692,-1.89518539750466E-13));
#122586=CARTESIAN_POINT('',(2.94793442701482,3.8743504127991,-6.89635284844599));
#122587=CARTESIAN_POINT('Origin',(-0.0349672952314722,3.62514694700665,
0.181476572229583));
#122588=CARTESIAN_POINT('Origin',(-0.0515325411352557,4.01774291754067,
0.178790762305159));
#122589=CARTESIAN_POINT('Ctrl Pts',(4.567536894,3.654941533,-5.948748333));
#122590=CARTESIAN_POINT('Ctrl Pts',(4.328416635,3.702826767,-6.13234840100001));
#122591=CARTESIAN_POINT('Ctrl Pts',(4.075331425,3.75,-6.296163417));
#122592=CARTESIAN_POINT('Ctrl Pts',(3.98260264499999,3.767283967,-6.356184177));
#122593=CARTESIAN_POINT('Ctrl Pts',(3.888146516,3.784676613,-6.41344811100001));
#122594=CARTESIAN_POINT('Ctrl Pts',(4.224321981,3.654941533,-5.892164611));
#122595=CARTESIAN_POINT('Ctrl Pts',(3.987476203,3.702826767,-6.061968561));
#122596=CARTESIAN_POINT('Ctrl Pts',(3.737765465,3.75,-6.212214527));
#122597=CARTESIAN_POINT('Ctrl Pts',(3.646273069,3.767283967,-6.267263675));
#122598=CARTESIAN_POINT('Ctrl Pts',(3.553199198,3.784676613,-6.319594564));
#122599=CARTESIAN_POINT('',(3.88814651615013,3.78467661264165,-6.41344811180752));
#122600=CARTESIAN_POINT('',(3.72067285279307,3.78467661221161,-6.36652133995858));
#122601=CARTESIAN_POINT('',(4.36476134892142,3.69493258293937,-6.09908668245247));
#122602=CARTESIAN_POINT('Ctrl Pts',(3.88814651703987,3.78467661270495,-6.41344810987096));
#122603=CARTESIAN_POINT('Ctrl Pts',(3.95120808549809,3.77306479305815,-6.37521709697566));
#122604=CARTESIAN_POINT('Ctrl Pts',(4.01361465239844,3.76150355535501,-6.33611096684481));
#122605=CARTESIAN_POINT('Ctrl Pts',(4.075331424686,3.75000000000677,-6.29616341695445));
#122606=CARTESIAN_POINT('Ctrl Pts',(4.17308480125791,3.7317794852682,-6.23289037585193));
#122607=CARTESIAN_POINT('Ctrl Pts',(4.26962070823788,3.71341418928686,-6.16717330105097));
#122608=CARTESIAN_POINT('Ctrl Pts',(4.36476134313645,3.69493258476044,-6.09908668613228));
#122609=CARTESIAN_POINT('Ctrl Pts',(4.22044662611337,3.65572482627337,-5.89494107521926));
#122610=CARTESIAN_POINT('Ctrl Pts',(4.24449374406195,3.66259516224952,-5.92889288124631));
#122611=CARTESIAN_POINT('Ctrl Pts',(4.26855635478161,3.6692920184403,-5.96290090268654));
#122612=CARTESIAN_POINT('Ctrl Pts',(4.3166522209443,3.68234999883244,-6.03093840455968));
#122613=CARTESIAN_POINT('Ctrl Pts',(4.34071397816382,3.68871885427257,-6.0650082078822));
#122614=CARTESIAN_POINT('Ctrl Pts',(4.3647613548088,3.69493258261569,-6.09908667835707));
#122615=CARTESIAN_POINT('Ctrl Pts',(4.808997871,3.784676613,-5.755305333));
#122616=CARTESIAN_POINT('Ctrl Pts',(4.497442691,3.720089779,-6.015633519));
#122617=CARTESIAN_POINT('Ctrl Pts',(4.159605534,3.654947264,-6.240807784));
#122618=CARTESIAN_POINT('Ctrl Pts',(4.828653401,3.784676613,-5.408013159));
#122619=CARTESIAN_POINT('Ctrl Pts',(4.535898384,3.720089779,-5.669405369));
#122620=CARTESIAN_POINT('Ctrl Pts',(4.216636664,3.654947264,-5.897666932));
#122621=CARTESIAN_POINT('',(4.80899787355245,3.78467661255986,-5.75530533275323));
#122622=CARTESIAN_POINT('Origin',(-0.10154261991247,3.6250254170349,0.161177119320642));
#122623=CARTESIAN_POINT('',(4.81882564214694,3.78467661169946,-5.58165924069315));
#122624=CARTESIAN_POINT('Origin',(-8.1380215066762E-13,3.87542692000056,
1.09287578986539E-12));
#122625=CARTESIAN_POINT('',(4.36152536599514,3.8743504127714,-6.10140118956461));
#122626=CARTESIAN_POINT('Origin',(-0.0731616365008658,3.6251470099273,0.169716425061738));
#122627=CARTESIAN_POINT('Origin',(-0.0887624311096608,4.01774290295748,
0.163532712363043));
#122628=CARTESIAN_POINT('Ctrl Pts',(5.739555467,3.654941533,-4.827784486));
#122629=CARTESIAN_POINT('Ctrl Pts',(5.54549429500001,3.702826767,-5.05849587400001));
#122630=CARTESIAN_POINT('Ctrl Pts',(5.333541463,3.75,-5.272886825));
#122631=CARTESIAN_POINT('Ctrl Pts',(5.255883319,3.767283967,-5.351438279));
#122632=CARTESIAN_POINT('Ctrl Pts',(5.175945575,3.784676613,-5.42766869));
#122633=CARTESIAN_POINT('Ctrl Pts',(5.392200901,3.654941533,-4.846304721));
#122634=CARTESIAN_POINT('Ctrl Pts',(5.197395276,3.702826767,-5.06305359));
#122635=CARTESIAN_POINT('Ctrl Pts',(4.985821077,3.75,-5.263467316));
#122636=CARTESIAN_POINT('Ctrl Pts',(4.908301662,3.767283967,-5.336897607));
#122637=CARTESIAN_POINT('Ctrl Pts',(4.828653401,3.784676613,-5.40801315900001));
#122638=CARTESIAN_POINT('',(5.17594557543062,3.78467661265236,-5.4276686907134));
#122639=CARTESIAN_POINT('',(5.00229948441995,3.78467661221161,-5.41784092780546));
#122640=CARTESIAN_POINT('',(5.57383900329526,3.69493258294351,-5.01819875675396));
#122641=CARTESIAN_POINT('Ctrl Pts',(5.17594557577235,3.78467661270495,-5.42766868867377));
#122642=CARTESIAN_POINT('Ctrl Pts',(5.22931426206921,3.77306479305815,-5.37677512226711));
#122643=CARTESIAN_POINT('Ctrl Pts',(5.28185513625994,3.76150355535484,-5.32516770467289));
#122644=CARTESIAN_POINT('Ctrl Pts',(5.33354146241084,3.7499999999535,-5.27288682476706));
#122645=CARTESIAN_POINT('Ctrl Pts',(5.41540758530399,3.73177948512943,-5.19007898539102));
#122646=CARTESIAN_POINT('Ctrl Pts',(5.49555930847529,3.71341418928853,-5.10514597349467));
#122647=CARTESIAN_POINT('Ctrl Pts',(5.57383899842944,3.69493258476864,-5.01819876160287));
#122648=CARTESIAN_POINT('Ctrl Pts',(5.38901300709273,3.65572482636599,-4.84984936019253));
#122649=CARTESIAN_POINT('Ctrl Pts',(5.41979654877931,3.66259516170139,-4.87783796967264));
#122650=CARTESIAN_POINT('Ctrl Pts',(5.45060730516922,3.66929201721005,-4.90587814937095));
#122651=CARTESIAN_POINT('Ctrl Pts',(5.51220477454759,3.68234999884185,-4.96198578808013));
#122652=CARTESIAN_POINT('Ctrl Pts',(5.5430279819644,3.68871885427849,-4.99008649180989));
#122653=CARTESIAN_POINT('Ctrl Pts',(5.57383900817425,3.69493258261921,-5.01819875147828));
#122654=CARTESIAN_POINT('Ctrl Pts',(5.93378669400001,3.784676613,-4.586957103));
#122655=CARTESIAN_POINT('Ctrl Pts',(5.685478366,3.720089779,-4.908174115));
#122656=CARTESIAN_POINT('Ctrl Pts',(5.403945465,3.654947264,-5.200708934));
#122657=CARTESIAN_POINT('Ctrl Pts',(5.878325138,3.784676613,-4.24355907));
#122658=CARTESIAN_POINT('Ctrl Pts',(5.648606168,3.720089779,-4.56177375));
#122659=CARTESIAN_POINT('Ctrl Pts',(5.385878098,3.654947264,-4.853330517));
#122660=CARTESIAN_POINT('',(5.93378669740299,3.7846766125581,-4.58695709980869));
#122661=CARTESIAN_POINT('Origin',(-0.133816982094878,3.62502543110219,0.135580259674121));
#122662=CARTESIAN_POINT('',(5.90605592085549,3.78467661170132,-4.41525808000507));
#122663=CARTESIAN_POINT('Origin',(1.24466409401336E-12,3.875426919999,-1.06685493772574E-12));
#122664=CARTESIAN_POINT('',(5.57117622608685,3.87435041281487,-5.02115479259927));
#122665=CARTESIAN_POINT('Origin',(-0.107935379660555,3.62514703452631,0.150021153177837));
#122666=CARTESIAN_POINT('Origin',(-0.121841914116984,4.01774292735558,0.140628110217738));
#122667=CARTESIAN_POINT('Ctrl Pts',(6.643198806,3.654941533,-3.481078802));
#122668=CARTESIAN_POINT('Ctrl Pts',(6.503270805,3.702826767,-3.748113702));
#122669=CARTESIAN_POINT('Ctrl Pts',(6.342361029,3.75,-4.003055905));
#122670=CARTESIAN_POINT('Ctrl Pts',(6.28340473,3.767283967,-4.096465076));
#122671=CARTESIAN_POINT('Ctrl Pts',(6.221723171,3.784676613,-4.188097513));
#122672=CARTESIAN_POINT('Ctrl Pts',(6.307946499,3.654941533,-3.573837008));
#122673=CARTESIAN_POINT('Ctrl Pts',(6.164289921,3.702826767,-3.82739586));
#122674=CARTESIAN_POINT('Ctrl Pts',(6.000745237,3.75,-4.068606224));
#122675=CARTESIAN_POINT('Ctrl Pts',(5.940823524,3.767283967,-4.156984138));
#122676=CARTESIAN_POINT('Ctrl Pts',(5.87832513800001,3.784676613,-4.24355907));
#122677=CARTESIAN_POINT('',(6.22172317159642,3.78467661265403,-4.1880975135927));
#122678=CARTESIAN_POINT('',(6.05002415171423,3.78467661221161,-4.21582829549779));
#122679=CARTESIAN_POINT('',(6.52229014041628,3.69493258292203,-3.70266543424931));
#122680=CARTESIAN_POINT('Ctrl Pts',(6.22172317147013,3.78467661270495,-4.18809751153862));
#122681=CARTESIAN_POINT('Ctrl Pts',(6.26290351519349,3.77306479305815,-4.12692111936028));
#122682=CARTESIAN_POINT('Ctrl Pts',(6.30312194364033,3.76150355535514,-4.06522551979907));
#122683=CARTESIAN_POINT('Ctrl Pts',(6.34236102849552,3.75000000004468,-4.003055905309));
#122684=CARTESIAN_POINT('Ctrl Pts',(6.40451192965349,3.73177948536437,-3.90458527148364));
#122685=CARTESIAN_POINT('Ctrl Pts',(6.46453166289258,3.71341418927574,-3.80440769392256));
#122686=CARTESIAN_POINT('Ctrl Pts',(6.52229013673516,3.69493258473157,-3.70266543998151));
#122687=CARTESIAN_POINT('Ctrl Pts',(6.30559512923655,3.65572482628442,-3.5779840780076));
#122688=CARTESIAN_POINT('Ctrl Pts',(6.34167569982709,3.66259516300955,-3.59870078211737));
#122689=CARTESIAN_POINT('Ctrl Pts',(6.37779393621342,3.66929202000516,-3.61946200121221));
#122690=CARTESIAN_POINT('Ctrl Pts',(6.45001275926347,3.68234999884121,-3.66101623074809));
#122691=CARTESIAN_POINT('Ctrl Pts',(6.48615615776691,3.68871885426855,-3.68183387725921));
#122692=CARTESIAN_POINT('Ctrl Pts',(6.52229014401681,3.69493258260042,-3.70266542809982));
#122693=CARTESIAN_POINT('Ctrl Pts',(6.781118246,3.784676613,-3.204127858));
#122694=CARTESIAN_POINT('Ctrl Pts',(6.607667391,3.720089779,-3.571213945));
#122695=CARTESIAN_POINT('Ctrl Pts',(6.395602912,3.654947264,-3.917430713));
#122696=CARTESIAN_POINT('Ctrl Pts',(6.653132924,3.784676613,-2.880680874));
#122697=CARTESIAN_POINT('Ctrl Pts',(6.497191406,3.720089779,-3.24083866));
#122698=CARTESIAN_POINT('Ctrl Pts',(6.303281859,3.654947264,-3.582057761));
#122699=CARTESIAN_POINT('',(6.78111824863517,3.78467661255781,-3.20412785413918));
#122700=CARTESIAN_POINT('Origin',(-0.159834164648105,3.62502540404964,0.103643783894751));
#122701=CARTESIAN_POINT('',(6.71712558834799,3.78467661170044,-3.04240435860819));
#122702=CARTESIAN_POINT('Origin',(6.63965410430123E-13,3.87542691999967,
-2.56955914879065E-13));
#122703=CARTESIAN_POINT('',(6.52032507813851,3.87435041281238,-3.70612477802144));
#122704=CARTESIAN_POINT('Origin',(-0.137661888874591,3.62514700884721,0.12331075786046));
#122705=CARTESIAN_POINT('Origin',(-0.149224008936868,4.01774292818933,0.111147792207484));
#122706=CARTESIAN_POINT('Ctrl Pts',(7.236213552,3.654941533,-1.971601742));
#122707=CARTESIAN_POINT('Ctrl Pts',(7.1569616,3.702826767,-2.262473898));
#122708=CARTESIAN_POINT('Ctrl Pts',(7.054618843,3.75,-2.54604654));
#122709=CARTESIAN_POINT('Ctrl Pts',(7.01712112,3.767283967,-2.649945718));
#122710=CARTESIAN_POINT('Ctrl Pts',(6.976579907,3.784676613,-2.752695552));
#122711=CARTESIAN_POINT('Ctrl Pts',(6.92873953,3.654941533,-2.134260649));
#122712=CARTESIAN_POINT('Ctrl Pts',(6.84294922100001,3.702826767,-2.412773354));
#122713=CARTESIAN_POINT('Ctrl Pts',(6.735081219,3.75,-2.683501626));
#122714=CARTESIAN_POINT('Ctrl Pts',(6.695559082,3.767283967,-2.78269471));
#122715=CARTESIAN_POINT('Ctrl Pts',(6.653132924,3.784676613,-2.880680874));
#122716=CARTESIAN_POINT('',(6.97657990769681,3.78467661265293,-2.75269555246126));
#122717=CARTESIAN_POINT('',(6.81485641363876,3.78467661221161,-2.81668821750318));
#122718=CARTESIAN_POINT('',(7.16576624024253,3.69493258298315,-2.21399959103629));
#122719=CARTESIAN_POINT('Ctrl Pts',(6.97657990714416,3.78467661270495,-2.75269555047203));
#122720=CARTESIAN_POINT('Ctrl Pts',(7.003646361286,3.77306479305815,-2.68409687135126));
#122721=CARTESIAN_POINT('Ctrl Pts',(7.02966177503315,3.76150355535505,-2.61519790717972));
#122722=CARTESIAN_POINT('Ctrl Pts',(7.05461884248965,3.7500000000164,-2.54604654030279));
#122723=CARTESIAN_POINT('Ctrl Pts',(7.09414841436022,3.73177948530313,-2.43651748824419));
#122724=CARTESIAN_POINT('Ctrl Pts',(7.13122970190591,3.713414189321,-2.32577953856128));
#122725=CARTESIAN_POINT('Ctrl Pts',(7.16576623782883,3.69493258483551,-2.21399959757585));
#122726=CARTESIAN_POINT('Ctrl Pts',(6.92733463179486,3.65572482628702,-2.13881623762723));
#122727=CARTESIAN_POINT('Ctrl Pts',(6.96702513999574,3.66259516342404,-2.15129234134254));
#122728=CARTESIAN_POINT('Ctrl Pts',(7.00676200318601,3.66929202084997,-2.16380382232231));
#122729=CARTESIAN_POINT('Ctrl Pts',(7.0862253164602,3.68234999889486,-2.1888616232306));
#122730=CARTESIAN_POINT('Ctrl Pts',(7.12599888104864,3.68871885432242,-2.20142280235593));
#122731=CARTESIAN_POINT('Ctrl Pts',(7.16576624248811,3.69493258265407,-2.21399958409845));
#122732=CARTESIAN_POINT('Ctrl Pts',(7.311372246,3.784676613,-1.671477154));
#122733=CARTESIAN_POINT('Ctrl Pts',(7.220889234,3.720089779,-2.067267779));
#122734=CARTESIAN_POINT('Ctrl Pts',(7.088209075,3.654947264,-2.450977787));
#122735=CARTESIAN_POINT('Ctrl Pts',(7.116847609,3.784676613,-1.383105243));
#122736=CARTESIAN_POINT('Ctrl Pts',(7.041975195,3.720089779,-1.768365556));
#122737=CARTESIAN_POINT('Ctrl Pts',(6.925951166,3.654947264,-2.143291965));
#122738=CARTESIAN_POINT('',(7.3113722477471,3.78467661255746,-1.67147714966288));
#122739=CARTESIAN_POINT('Origin',(-0.178377525387388,3.62502544882287,0.0668609742983872));
#122740=CARTESIAN_POINT('',(7.21410992918197,3.78467661169946,-1.52729119055528));
#122741=CARTESIAN_POINT('Origin',(-1.86786350275803E-12,3.87542691999978,
5.44269490587723E-13));
#122742=CARTESIAN_POINT('',(7.16459077629712,3.87435041280689,-2.21780048786891));
#122743=CARTESIAN_POINT('Origin',(-0.160951713076786,3.62514696513198,0.0908346270462984));
#122744=CARTESIAN_POINT('Origin',(-0.169628826863583,4.01774292196974,0.0764704926359777));
#122745=CARTESIAN_POINT('Ctrl Pts',(7.490870995,3.654941533,-0.369934777));
#122746=CARTESIAN_POINT('Ctrl Pts',(7.476000825,3.702826767,-0.67104333));
#122747=CARTESIAN_POINT('Ctrl Pts',(7.43701052,3.75,-0.969986869));
#122748=CARTESIAN_POINT('Ctrl Pts',(7.422724725,3.767283967,-1.079517843));
#122749=CARTESIAN_POINT('Ctrl Pts',(7.40521952,3.784676613,-1.188580606));
#122750=CARTESIAN_POINT('Ctrl Pts',(7.225552402,3.654941533,-0.594888634));
#122751=CARTESIAN_POINT('Ctrl Pts',(7.201639821,3.702826767,-0.885332247));
#122752=CARTESIAN_POINT('Ctrl Pts',(7.154492288,3.75,-1.172919475));
#122753=CARTESIAN_POINT('Ctrl Pts',(7.137217738,3.767283967,-1.278289571));
#122754=CARTESIAN_POINT('Ctrl Pts',(7.116847609,3.784676613,-1.383105243));
#122755=CARTESIAN_POINT('',(7.40521952078668,3.78467661265378,-1.18858060629129));
#122756=CARTESIAN_POINT('',(7.26103356365033,3.78467661221161,-1.28584292929801));
#122757=CARTESIAN_POINT('',(7.47417907411976,3.69493258291695,-0.621809588034605));
#122758=CARTESIAN_POINT('Ctrl Pts',(7.40521951981189,3.78467661270495,-1.18858060447705));
#122759=CARTESIAN_POINT('Ctrl Pts',(7.41690648710047,3.77306479305815,-1.11576723638085));
#122760=CARTESIAN_POINT('Ctrl Pts',(7.4275024342893,3.76150355535484,-1.04288654688099));
#122761=CARTESIAN_POINT('Ctrl Pts',(7.43701051966161,3.749999999954,-0.969986868978883));
#122762=CARTESIAN_POINT('Ctrl Pts',(7.45207040391301,3.73177948512167,-0.854520854919855));
#122763=CARTESIAN_POINT('Ctrl Pts',(7.46447936555569,3.71341418926482,-0.738400517224669));
#122764=CARTESIAN_POINT('Ctrl Pts',(7.47417907318899,3.69493258472366,-0.621809594771243));
#122765=CARTESIAN_POINT('Ctrl Pts',(7.22515966610095,3.65572482629693,-0.599639727402921));
#122766=CARTESIAN_POINT('Ctrl Pts',(7.26660422586383,3.66259516346406,-0.603291860843454));
#122767=CARTESIAN_POINT('Ctrl Pts',(7.30810166197504,3.66929202091486,-0.606968579461314));
#122768=CARTESIAN_POINT('Ctrl Pts',(7.39109385304935,3.68234999886983,-0.614358279513562));
#122769=CARTESIAN_POINT('Ctrl Pts',(7.43263781594534,3.68871885428331,-0.618075644577407));
#122770=CARTESIAN_POINT('Ctrl Pts',(7.47417907480425,3.69493258259591,-0.621809580953705));
#122771=CARTESIAN_POINT('Ctrl Pts',(7.499754606,3.784676613,-0.060670037));
#122772=CARTESIAN_POINT('Ctrl Pts',(7.496470321,3.720089779,-0.46665847));
#122773=CARTESIAN_POINT('Ctrl Pts',(7.449378459,3.654947264,-0.869919863));
#122774=CARTESIAN_POINT('Ctrl Pts',(7.24778641,3.784676613,0.179142852));
#122775=CARTESIAN_POINT('Ctrl Pts',(7.25748405,3.720089779,-0.213205645));
#122776=CARTESIAN_POINT('Ctrl Pts',(7.22477069400001,3.654947264,-0.604308219));
#122777=CARTESIAN_POINT('',(7.4997546067426,3.78467661255817,-0.0606700323674423));
#122778=CARTESIAN_POINT('Origin',(-0.188580229804709,3.6250254421705,0.0269519150140703));
#122779=CARTESIAN_POINT('',(7.37377050793487,3.78467661170154,0.0592364156075977));
#122780=CARTESIAN_POINT('Origin',(-1.06685493772574E-12,3.87542692000011,
1.41617132517341E-13));
#122781=CARTESIAN_POINT('',(7.47384817270334,3.87435041278447,-0.6257743120038));
#122782=CARTESIAN_POINT('Origin',(-0.176715334483249,3.62514697594731,0.0541110863649678));
#122783=CARTESIAN_POINT('Origin',(-0.182101924228347,4.01774293762491,0.0382174800455872));
#122784=CARTESIAN_POINT('Ctrl Pts',(7.395263635,3.654941533,1.249029928));
#122785=CARTESIAN_POINT('Ctrl Pts',(7.44547056,3.702826767,0.951764478));
#122786=CARTESIAN_POINT('Ctrl Pts',(7.471655851,3.75,0.651428311));
#122787=CARTESIAN_POINT('Ctrl Pts',(7.481249972,3.767283967,0.541387086));
#122788=CARTESIAN_POINT('Ctrl Pts',(7.487599299,3.784676613,0.431111049));
#122789=CARTESIAN_POINT('Ctrl Pts',(7.184506474,3.654941533,0.972299712));
#122790=CARTESIAN_POINT('Ctrl Pts',(7.223589747,3.702826767,0.683506012));
#122791=CARTESIAN_POINT('Ctrl Pts',(7.23936725,3.75,0.392507087));
#122792=CARTESIAN_POINT('Ctrl Pts',(7.245148025,3.767283967,0.285886968));
#122793=CARTESIAN_POINT('Ctrl Pts',(7.24778641,3.784676613,0.179142852));
#122794=CARTESIAN_POINT('',(7.48759929982812,3.78467661265328,0.43111104887842));
#122795=CARTESIAN_POINT('',(7.36769285470162,3.78467661221161,0.305126945631554));
#122796=CARTESIAN_POINT('',(7.43310760180177,3.69493258296357,0.999455540430897));
#122797=CARTESIAN_POINT('Ctrl Pts',(7.48759929848919,3.78467661270495,0.431111050447227));
#122798=CARTESIAN_POINT('Ctrl Pts',(7.48336030927576,3.77306479305815,0.504734434406425));
#122799=CARTESIAN_POINT('Ctrl Pts',(7.47804133512577,3.76150355535511,0.578189029261445));
#122800=CARTESIAN_POINT('Ctrl Pts',(7.47165585077238,3.75000000003437,0.651428310506225));
#122801=CARTESIAN_POINT('Ctrl Pts',(7.46154186354479,3.73177948533219,0.767432222086782));
#122802=CARTESIAN_POINT('Ctrl Pts',(7.4486982702273,3.71341418929205,0.883505291650194));
#122803=CARTESIAN_POINT('Ctrl Pts',(7.43310760235171,3.69493258480238,0.999455533532112));
#122804=CARTESIAN_POINT('Ctrl Pts',(7.18514426466047,3.65572482627106,0.967575270075688));
#122805=CARTESIAN_POINT('Ctrl Pts',(7.22640497355284,3.66259516332048,0.97291787694699));
#122806=CARTESIAN_POINT('Ctrl Pts',(7.26772260757813,3.66929202065056,0.978247840087374));
#122807=CARTESIAN_POINT('Ctrl Pts',(7.35036305591922,3.68234999887543,0.988871775223886));
#122808=CARTESIAN_POINT('Ctrl Pts',(7.3917348676734,3.68871885430748,0.994172044021346));
#122809=CARTESIAN_POINT('Ctrl Pts',(7.43310760093298,3.69493258263685,0.999455547618201));
#122810=CARTESIAN_POINT('Ctrl Pts',(7.337456775,3.784676613,1.552973944));
#122811=CARTESIAN_POINT('Ctrl Pts',(7.421524787,3.720089779,1.15577127));
#122812=CARTESIAN_POINT('Ctrl Pts',(7.462223187,3.654947264,0.751814547));
#122813=CARTESIAN_POINT('Ctrl Pts',(7.039826773,3.784676613,1.733014427));
#122814=CARTESIAN_POINT('Ctrl Pts',(7.133641018,3.720089779,1.351923526));
#122815=CARTESIAN_POINT('Ctrl Pts',(7.18576797400001,3.654947264,0.962932308));
#122816=CARTESIAN_POINT('',(7.33745677598408,3.7846766125602,1.55297394635713));
#122817=CARTESIAN_POINT('Origin',(-0.189965454764864,3.62502539034957,-0.0142174262418361));
#122818=CARTESIAN_POINT('',(7.18864177219204,3.78467661170049,1.64299419341043));
#122819=CARTESIAN_POINT('Origin',(1.69742692124331E-12,3.875426919999,2.83952548973954E-13));
#122820=CARTESIAN_POINT('',(7.43363673487299,3.87435041278443,0.995512375213104));
#122821=CARTESIAN_POINT('Origin',(-0.184216316489234,3.62514695593933,0.0148574046262219));
#122822=CARTESIAN_POINT('Origin',(-0.186060340080447,4.01774294148807,-0.00182259763174569));
#122823=CARTESIAN_POINT('Ctrl Pts',(6.953861968,3.654941533,2.809591382));
#122824=CARTESIAN_POINT('Ctrl Pts',(7.06679836700001,3.702826767,2.530068838));
#122825=CARTESIAN_POINT('Ctrl Pts',(7.156934859,3.75,2.242383426));
#122826=CARTESIAN_POINT('Ctrl Pts',(7.189960285,3.767283967,2.136977356));
#122827=CARTESIAN_POINT('Ctrl Pts',(7.219867256,3.784676613,2.030644429));
#122828=CARTESIAN_POINT('Ctrl Pts',(6.807521008,3.654941533,2.494024404));
#122829=CARTESIAN_POINT('Ctrl Pts',(6.907772645,3.702826767,2.220384289));
#122830=CARTESIAN_POINT('Ctrl Pts',(6.985737446,3.75,1.939580454));
#122831=CARTESIAN_POINT('Ctrl Pts',(7.014303243,3.767283967,1.83669575));
#122832=CARTESIAN_POINT('Ctrl Pts',(7.039826773,3.784676613,1.733014427));
#122833=CARTESIAN_POINT('',(7.21986725684003,3.78467661265474,2.03064442908069));
#122834=CARTESIAN_POINT('',(7.12984701574349,3.78467661221161,1.88182942328867));
#122835=CARTESIAN_POINT('',(7.04447227901576,3.69493258292078,2.57398723862445));
#122836=CARTESIAN_POINT('Ctrl Pts',(7.21986725519049,3.78467661270495,2.03064443030433));
#122837=CARTESIAN_POINT('Ctrl Pts',(7.1999005202516,3.77306479305815,2.10163528313903));
#122838=CARTESIAN_POINT('Ctrl Pts',(7.17891533445251,3.76150355535492,2.17222912823678));
#122839=CARTESIAN_POINT('Ctrl Pts',(7.15693485866925,3.74999999998004,2.24238342560418));
#122840=CARTESIAN_POINT('Ctrl Pts',(7.12211991836894,3.73177948519665,2.35350102255827));
#122841=CARTESIAN_POINT('Ctrl Pts',(7.08462432257388,3.71341418927471,2.46409937521361));
#122842=CARTESIAN_POINT('Ctrl Pts',(7.04447228100107,3.69493258472953,2.57398723211122));
#122843=CARTESIAN_POINT('Ctrl Pts',(6.80915950283612,3.65572482629022,2.48954752285279));
#122844=CARTESIAN_POINT('Ctrl Pts',(6.8483070455585,3.66259516136376,2.503635051298));
#122845=CARTESIAN_POINT('Ctrl Pts',(6.88751289855184,3.66929201659142,2.5177224682113));
#122846=CARTESIAN_POINT('Ctrl Pts',(6.96593745121808,3.68234999882244,2.54586328409005));
#122847=CARTESIAN_POINT('Ctrl Pts',(7.00520261193498,3.6887188542613,2.55993335229255));
#122848=CARTESIAN_POINT('Ctrl Pts',(7.04447227666092,3.69493258259933,2.57398724534652));
#122849=CARTESIAN_POINT('Ctrl Pts',(6.832067621,3.784676613,3.094002589));
#122850=CARTESIAN_POINT('Ctrl Pts',(6.999557003,3.720089779,2.724158431));
#122851=CARTESIAN_POINT('Ctrl Pts',(7.126142651,3.654947264,2.338394944));
#122852=CARTESIAN_POINT('Ctrl Pts',(6.502692661,3.784676613,3.205852173));
#122853=CARTESIAN_POINT('Ctrl Pts',(6.676236859,3.720089779,2.853838255));
#122854=CARTESIAN_POINT('Ctrl Pts',(6.810766729,3.654947264,2.48514719));
#122855=CARTESIAN_POINT('',(6.8320676214468,3.78467661256008,3.09400259152216));
#122856=CARTESIAN_POINT('Origin',(-0.182467702143871,3.62502542581436,-0.0547219315056946));
#122857=CARTESIAN_POINT('',(6.66738013753278,3.78467661170011,3.14992738833899));
#122858=CARTESIAN_POINT('Origin',(-1.01091010562548E-12,3.87542692000078,
-3.56485674313234E-13));
#122859=CARTESIAN_POINT('',(7.04583670518564,3.87435041281413,2.57025001060989));
#122860=CARTESIAN_POINT('Origin',(-0.183103012010924,3.62514699798789,-0.0250909105996028));
#122861=CARTESIAN_POINT('Origin',(-0.181318334342333,4.0177429538234,-0.0417773652865977));
#122862=CARTESIAN_POINT('Ctrl Pts',(6.187305443,3.654941533,4.238779465));
#122863=CARTESIAN_POINT('Ctrl Pts',(6.357690537,3.702826767,3.99006999));
#122864=CARTESIAN_POINT('Ctrl Pts',(6.507563547,3.75,3.728487185));
#122865=CARTESIAN_POINT('Ctrl Pts',(6.562476046,3.767283967,3.632644941));
#122866=CARTESIAN_POINT('Ctrl Pts',(6.614542245,3.784676613,3.535227133));
#122867=CARTESIAN_POINT('Ctrl Pts',(6.112223425,3.654941533,3.899131288));
#122868=CARTESIAN_POINT('Ctrl Pts',(6.268955771,3.702826767,3.653439864));
#122869=CARTESIAN_POINT('Ctrl Pts',(6.405462322,3.75,3.395961195));
#122870=CARTESIAN_POINT('Ctrl Pts',(6.455477438,3.767283967,3.30162268));
#122871=CARTESIAN_POINT('Ctrl Pts',(6.502692661,3.784676613,3.205852173));
#122872=CARTESIAN_POINT('',(6.61454224581363,3.78467661264356,3.53522713313392));
#122873=CARTESIAN_POINT('',(6.55861745522635,3.78467661221192,3.37053964866783));
#122874=CARTESIAN_POINT('',(6.32644526234173,3.69493258293484,4.02816215414154));
#122875=CARTESIAN_POINT('Ctrl Pts',(6.61454224392794,3.78467661270466,3.53522713410086));
#122876=CARTESIAN_POINT('Ctrl Pts',(6.57978138511409,3.77306479305805,3.60026600275559));
#122877=CARTESIAN_POINT('Ctrl Pts',(6.5441112313165,3.76150355535493,3.66469820841077));
#122878=CARTESIAN_POINT('Ctrl Pts',(6.50756354677996,3.74999999998162,3.72848718457547));
#122879=CARTESIAN_POINT('Ctrl Pts',(6.4496755619513,3.73177948520058,3.82952273065416));
#122880=CARTESIAN_POINT('Ctrl Pts',(6.38928121584586,3.71341418928213,3.92947491035372));
#122881=CARTESIAN_POINT('Ctrl Pts',(6.32644526570093,3.69493258475378,4.02816214817663));
#122882=CARTESIAN_POINT('Ctrl Pts',(6.11478601007337,3.65572482633407,3.89511130188058));
#122883=CARTESIAN_POINT('Ctrl Pts',(6.14998991154971,3.66259516307394,3.91728504138573));
#122884=CARTESIAN_POINT('Ctrl Pts',(6.18525078550877,3.66929202007563,3.93947120792721));
#122885=CARTESIAN_POINT('Ctrl Pts',(6.25579235404782,3.6823499988899,3.98381305591855));
#122886=CARTESIAN_POINT('Ctrl Pts',(6.29111486838206,3.68871885430092,4.00599502244057));
#122887=CARTESIAN_POINT('Ctrl Pts',(6.32644525857656,3.69493258261167,4.02816216023313));
#122888=CARTESIAN_POINT('Ctrl Pts',(6.007218578,3.784676613,4.490359112));
#122889=CARTESIAN_POINT('Ctrl Pts',(6.250297713,3.720089779,4.165166971));
#122890=CARTESIAN_POINT('Ctrl Pts',(6.456851606,3.654947264,3.815634592));
#122891=CARTESIAN_POINT('Ctrl Pts',(5.661499867,3.784676613,4.528787835));
#122892=CARTESIAN_POINT('Ctrl Pts',(5.906659286,3.720089779,4.222310679));
#122893=CARTESIAN_POINT('Ctrl Pts',(6.117301603,3.654947264,3.891159352));
#122894=CARTESIAN_POINT('',(6.00721857789413,3.78467661255989,4.49035911456038));
#122895=CARTESIAN_POINT('Origin',(-0.166438120794062,3.62502543736376,-0.0926677379736934));
#122896=CARTESIAN_POINT('',(5.834359217534,3.78467661169954,4.50957347992487));
#122897=CARTESIAN_POINT('Origin',(-4.28043017697277E-13,3.87542691999933,
-2.07733136248223E-13));
#122898=CARTESIAN_POINT('',(6.32858118252462,3.87435041281544,4.02480561184882));
#122899=CARTESIAN_POINT('Origin',(-0.173428612544835,3.62514700340954,-0.0638661794404793));
#122900=CARTESIAN_POINT('Origin',(-0.168098172405629,4.01774290969785,-0.0797786309649051));
#122901=CARTESIAN_POINT('Ctrl Pts',(5.131437393,3.654941533,5.469766932));
#122902=CARTESIAN_POINT('Ctrl Pts',(5.351304163,3.702826767,5.263499904));
#122903=CARTESIAN_POINT('Ctrl Pts',(5.553905796,3.75,5.040251027));
#122904=CARTESIAN_POINT('Ctrl Pts',(5.62813772100001,3.767283967,4.958454085));
#122905=CARTESIAN_POINT('Ctrl Pts',(5.69992859,3.784676613,4.874506546));
#122906=CARTESIAN_POINT('Ctrl Pts',(5.131125069,3.654941533,5.121919125));
#122907=CARTESIAN_POINT('Ctrl Pts',(5.337009493,3.702826767,4.915664652));
#122908=CARTESIAN_POINT('Ctrl Pts',(5.5256749,3.75,4.693550565));
#122909=CARTESIAN_POINT('Ctrl Pts',(5.594800682,3.767283967,4.612169403));
#122910=CARTESIAN_POINT('Ctrl Pts',(5.661499867,3.784676613,4.528787835));
#122911=CARTESIAN_POINT('',(5.69992859076987,3.78467661264248,4.87450654629026));
#122912=CARTESIAN_POINT('',(5.68071423160659,3.78467661221167,4.7016471867465));
#122913=CARTESIAN_POINT('',(5.31260069589747,3.69493258285852,5.2939846841393));
#122914=CARTESIAN_POINT('Ctrl Pts',(5.69992858871736,3.7846766127049,4.87450654684343));
#122915=CARTESIAN_POINT('Ctrl Pts',(5.65199898542052,3.77306479305813,4.93055228505985));
#122916=CARTESIAN_POINT('Ctrl Pts',(5.60331176036077,3.76150355535504,4.98581007269591));
#122917=CARTESIAN_POINT('Ctrl Pts',(5.55390579601133,3.75000000001507,5.04025102627296));
#122918=CARTESIAN_POINT('Ctrl Pts',(5.47565154445195,3.73177948527118,5.12648021133348));
#122919=CARTESIAN_POINT('Ctrl Pts',(5.395182420043,3.7134141892243,5.21111256605488));
#122920=CARTESIAN_POINT('Ctrl Pts',(5.31260070032299,3.69493258462341,5.29398467918044));
#122921=CARTESIAN_POINT('Ctrl Pts',(5.13449192012045,3.65572482626041,5.11854400406274));
#122922=CARTESIAN_POINT('Ctrl Pts',(5.16410607726281,3.66259516344758,5.14776713409778));
#122923=CARTESIAN_POINT('Ctrl Pts',(5.19377320384533,3.66929202093393,5.17701464831315));
#122924=CARTESIAN_POINT('Ctrl Pts',(5.25313335869222,3.68234999880056,5.23548415631472));
#122925=CARTESIAN_POINT('Ctrl Pts',(5.2828615851379,3.68871885422111,5.26474081721335));
#122926=CARTESIAN_POINT('Ctrl Pts',(5.31260069105651,3.69493258254474,5.29398468912891));
#122927=CARTESIAN_POINT('Ctrl Pts',(4.901478671,3.784676613,5.67675143300001));
#122928=CARTESIAN_POINT('Ctrl Pts',(5.208781448,3.720089779,5.41141693200001));
#122929=CARTESIAN_POINT('Ctrl Pts',(5.485645355,3.654947264,5.11445940800001));
#122930=CARTESIAN_POINT('Ctrl Pts',(4.555581632,3.784676613,5.639962411));
#122931=CARTESIAN_POINT('Ctrl Pts',(4.860892888,3.720089779,5.393352549));
#122932=CARTESIAN_POINT('Ctrl Pts',(5.137798252,3.654947264,5.115225227));
#122933=CARTESIAN_POINT('',(4.90147867036157,3.78467661255985,5.67675143547201));
#122934=CARTESIAN_POINT('Origin',(-0.142626193212273,3.62502542072744,-0.126280622329832));
#122935=CARTESIAN_POINT('',(4.72853014526859,3.78467661169946,5.65835692720741));
#122936=CARTESIAN_POINT('Origin',(6.89552581700781E-14,3.87542691999978,
4.59701721133854E-14));
#122937=CARTESIAN_POINT('',(5.31540823698528,3.87435041276596,5.29116577603125));
#122938=CARTESIAN_POINT('Origin',(-0.155644556110387,3.62514698104704,-0.0996550053936607));
#122939=CARTESIAN_POINT('Origin',(-0.14701820053967,4.01774292527244,-0.114049714748815));
#122940=CARTESIAN_POINT('Ctrl Pts',(3.835629033,3.654941533,6.444994175));
#122941=CARTESIAN_POINT('Ctrl Pts',(4.094696754,3.702826767,6.290814413));
#122942=CARTESIAN_POINT('Ctrl Pts',(4.340553583,3.75,6.116338332));
#122943=CARTESIAN_POINT('Ctrl Pts',(4.430633931,3.767283967,6.052411428));
#122944=CARTESIAN_POINT('Ctrl Pts',(4.518792609,3.784676613,5.98585945));
#122945=CARTESIAN_POINT('Ctrl Pts',(3.910101007,3.654941533,6.105211717));
#122946=CARTESIAN_POINT('Ctrl Pts',(4.155510583,3.702826767,5.948038425));
#122947=CARTESIAN_POINT('Ctrl Pts',(4.38751306,3.75,5.771674726));
#122948=CARTESIAN_POINT('Ctrl Pts',(4.472517264,3.767283967,5.707056211));
#122949=CARTESIAN_POINT('Ctrl Pts',(4.555581632,3.784676613,5.639962411));
#122950=CARTESIAN_POINT('',(4.51879260962801,3.7846766126534,5.98585945055455));
#122951=CARTESIAN_POINT('',(4.53718712434111,3.78467661221161,5.81291092750187));
#122952=CARTESIAN_POINT('',(4.05034482615765,3.69493258293517,6.31226637490125));
#122953=CARTESIAN_POINT('Ctrl Pts',(4.51879260756625,3.78467661270495,5.98585945054807));
#122954=CARTESIAN_POINT('Ctrl Pts',(4.45993539460359,3.77306479305815,6.03029142297988));
#122955=CARTESIAN_POINT('Ctrl Pts',(4.4005076589704,3.76150355535495,6.07379099976697));
#122956=CARTESIAN_POINT('Ctrl Pts',(4.34055358297325,3.74999999998799,6.11633833178121));
#122957=CARTESIAN_POINT('Ctrl Pts',(4.24559214605223,3.73177948520062,6.18372917663367));
#122958=CARTESIAN_POINT('Ctrl Pts',(4.14881089109748,3.71341418926484,6.24908438995837));
#122959=CARTESIAN_POINT('Ctrl Pts',(4.05034483171224,3.6949325847545,6.31226637089826));
#122960=CARTESIAN_POINT('Ctrl Pts',(3.91411469426839,3.65572482628045,6.10263927833785));
#122961=CARTESIAN_POINT('Ctrl Pts',(3.93675437896973,3.66259516319504,6.13754535472069));
#122962=CARTESIAN_POINT('Ctrl Pts',(3.95944055256593,3.66929202038164,6.17248663184647));
#122963=CARTESIAN_POINT('Ctrl Pts',(4.00484368630039,3.68234999886763,6.24234983720333));
#122964=CARTESIAN_POINT('Ctrl Pts',(4.02758756605168,3.68871885428794,6.27731318362012));
#122965=CARTESIAN_POINT('Ctrl Pts',(4.05034482018178,3.69493258261195,6.31226637884947));
#122966=CARTESIAN_POINT('Ctrl Pts',(3.566551069,3.784676613,6.597705167));
#122967=CARTESIAN_POINT('Ctrl Pts',(3.923708353,3.720089779,6.40463505300001));
#122968=CARTESIAN_POINT('Ctrl Pts',(4.257936425,3.654947264,6.174137786));
#122969=CARTESIAN_POINT('Ctrl Pts',(3.236649463,3.784676613,6.487418613));
#122970=CARTESIAN_POINT('Ctrl Pts',(3.587836542,3.720089779,6.312207247));
#122971=CARTESIAN_POINT('Ctrl Pts',(3.918057165,3.654947264,6.100108856));
#122972=CARTESIAN_POINT('',(3.56655106527544,3.78467661255747,6.5977051698394));
#122973=CARTESIAN_POINT('Origin',(-0.112144915021962,3.62502542437372,-0.15398841209647));
#122974=CARTESIAN_POINT('',(3.40160025879484,3.78467661169946,6.5425618937461));
#122975=CARTESIAN_POINT('Origin',(3.88144377749811E-14,3.87542691999956,
7.80625564189563E-14));
#122976=CARTESIAN_POINT('',(4.05369271029252,3.87435041278445,6.31011690930621));
#122977=CARTESIAN_POINT('Origin',(-0.130582748923885,3.62514698298211,-0.13078403823463));
#122978=CARTESIAN_POINT('Origin',(-0.119063806199796,4.01774296137409,-0.142988065470824));
#122979=CARTESIAN_POINT('Ctrl Pts',(2.360470923,3.654941533,7.118860655));
#122980=CARTESIAN_POINT('Ctrl Pts',(2.646625875,3.702826767,7.023977432));
#122981=CARTESIAN_POINT('Ctrl Pts',(2.924241908,3.75,6.906432456));
#122982=CARTESIAN_POINT('Ctrl Pts',(3.025958623,3.767283967,6.86336473800001));
#122983=CARTESIAN_POINT('Ctrl Pts',(3.126362908,3.784676613,6.81732021900001));
#122984=CARTESIAN_POINT('Ctrl Pts',(2.506244968,3.654941533,6.803031395));
#122985=CARTESIAN_POINT('Ctrl Pts',(2.779704616,3.702826767,6.702288531));
#122986=CARTESIAN_POINT('Ctrl Pts',(3.044195986,3.75,6.579921793));
#122987=CARTESIAN_POINT('Ctrl Pts',(3.14110391,3.767283967,6.53508741300001));
#122988=CARTESIAN_POINT('Ctrl Pts',(3.236649463,3.784676613,6.487418613));
#122989=CARTESIAN_POINT('',(3.12636290849546,3.78467661265307,6.81732021967232));
#122990=CARTESIAN_POINT('',(3.18150618989289,3.78467661221213,6.65236941389909));
#122991=CARTESIAN_POINT('',(2.59869933355453,3.6949325829309,7.03539350480189));
#122992=CARTESIAN_POINT('Ctrl Pts',(3.12636290647896,3.78467661270444,6.81732021922853));
#122993=CARTESIAN_POINT('Ctrl Pts',(3.05933018184786,3.77306479305799,6.84806083524092));
#122994=CARTESIAN_POINT('Ctrl Pts',(2.99194071024776,3.76150355535498,6.87776820981747));
#122995=CARTESIAN_POINT('Ctrl Pts',(2.92424190825284,3.74999999999723,6.90643245527431));
#122996=CARTESIAN_POINT('Ctrl Pts',(2.81701357788189,3.73177948525387,6.95183383669016));
#122997=CARTESIAN_POINT('Ctrl Pts',(2.70844557548394,3.71341418929348,6.99485597339471));
#122998=CARTESIAN_POINT('Ctrl Pts',(2.5986993398269,3.69493258474626,7.03539350208781));
#122999=CARTESIAN_POINT('Ctrl Pts',(2.51071781620878,3.65572482632389,6.8013819220982));
#123000=CARTESIAN_POINT('Ctrl Pts',(2.52532442071916,3.66259516218778,6.84033877095559));
#123001=CARTESIAN_POINT('Ctrl Pts',(2.53996885977681,3.66929201826815,6.87933999028188));
#123002=CARTESIAN_POINT('Ctrl Pts',(2.56929197403464,3.682349998848,6.95733017684901));
#123003=CARTESIAN_POINT('Ctrl Pts',(2.58398802850682,3.68871885427552,6.99636536148919));
#123004=CARTESIAN_POINT('Ctrl Pts',(2.59869932688208,3.69493258260825,7.03539350736838));
#123005=CARTESIAN_POINT('Ctrl Pts',(2.064855503,3.784676613,7.21015754));
#123006=CARTESIAN_POINT('Ctrl Pts',(2.455167015,3.720089779,7.09837955600001));
#123007=CARTESIAN_POINT('Ctrl Pts',(2.83113112,3.654947264,6.945120343));
#123008=CARTESIAN_POINT('Ctrl Pts',(1.766375162,3.784676613,7.03153033));
#123009=CARTESIAN_POINT('Ctrl Pts',(2.147016947,3.720089779,6.935910151));
#123010=CARTESIAN_POINT('Ctrl Pts',(2.51511208,3.654947264,6.799758174));
#123011=CARTESIAN_POINT('',(2.06485549874544,3.78467661255747,7.21015754196833));
#123012=CARTESIAN_POINT('Origin',(-0.0764201343107868,3.62502544448452,
-0.174496270778641));
#123013=CARTESIAN_POINT('',(1.915615324658,3.78467661169946,7.12084393710962));
#123014=CARTESIAN_POINT('Origin',(-1.23599047663348E-14,3.87542691999956,
3.963843142607E-13));
#123015=CARTESIAN_POINT('',(2.60243101765054,3.87435041278084,7.0340139887341));
#123016=CARTESIAN_POINT('Origin',(-0.0994150821283607,3.62514695328514,
-0.155797783113337));
#123017=CARTESIAN_POINT('Origin',(-0.0855418496423702,4.01774292338515,
-0.165239972260454));
#123018=CARTESIAN_POINT('Ctrl Pts',(0.774939815,3.654941533,7.459857122));
#123019=CARTESIAN_POINT('Ctrl Pts',(1.074801713,3.702826767,7.428707072));
#123020=CARTESIAN_POINT('Ctrl Pts',(1.371195932,3.75,7.373589473));
#123021=CARTESIAN_POINT('Ctrl Pts',(1.479792853,3.767283967,7.353394742));
#123022=CARTESIAN_POINT('Ctrl Pts',(1.587747952,3.784676613,7.330010671));
#123023=CARTESIAN_POINT('Ctrl Pts',(0.9851997,3.654941533,7.182748885));
#123024=CARTESIAN_POINT('Ctrl Pts',(1.273922751,3.702826767,7.14314707500001));
#123025=CARTESIAN_POINT('Ctrl Pts',(1.558535692,3.75,7.080499029));
#123026=CARTESIAN_POINT('Ctrl Pts',(1.662816028,3.767283967,7.057545191));
#123027=CARTESIAN_POINT('Ctrl Pts',(1.766375162,3.784676613,7.03153033));
#123028=CARTESIAN_POINT('',(1.58774795233273,3.78467661265383,7.33001067177046));
#123029=CARTESIAN_POINT('',(1.67706156174498,3.78467661221161,7.18077049939182));
#123030=CARTESIAN_POINT('',(1.02554154841774,3.694932582952,7.42955345417115));
#123031=CARTESIAN_POINT('Ctrl Pts',(1.58774795046899,3.78467661270495,7.3300106708948));
#123032=CARTESIAN_POINT('Ctrl Pts',(1.51567409001811,3.77306479305815,7.3456225344741));
#123033=CARTESIAN_POINT('Ctrl Pts',(1.44347393947909,3.76150355535514,7.3601486227396));
#123034=CARTESIAN_POINT('Ctrl Pts',(1.37119593248388,3.7500000000441,7.37358947262491));
#123035=CARTESIAN_POINT('Ctrl Pts',(1.25671458624729,3.73177948536409,7.39487847406491));
#123036=CARTESIAN_POINT('Ctrl Pts',(1.14143635549968,3.71341418929291,7.41355586531108));
#123037=CARTESIAN_POINT('Ctrl Pts',(1.02554155518139,3.69493258478233,7.42955345286027));
#123038=CARTESIAN_POINT('Ctrl Pts',(0.989922562716053,3.65572482627746,
7.18209950661361));
#123039=CARTESIAN_POINT('Ctrl Pts',(0.995813103393928,3.66259516373845,
7.22328556359935));
#123040=CARTESIAN_POINT('Ctrl Pts',(1.00173105597368,3.66929202150471,7.26452308866619));
#123041=CARTESIAN_POINT('Ctrl Pts',(1.01360302452885,3.68234999887928,7.34699349048117));
#123042=CARTESIAN_POINT('Ctrl Pts',(1.01956408260669,3.6887188543024,7.3882752714801));
#123043=CARTESIAN_POINT('Ctrl Pts',(1.02554154129235,3.69493258262675,7.42955345525194));
#123044=CARTESIAN_POINT('Ctrl Pts',(0.466609588,3.784676613,7.48547096));
#123045=CARTESIAN_POINT('Ctrl Pts',(0.871824797,3.720089779,7.460211721));
#123046=CARTESIAN_POINT('Ctrl Pts',(1.27194527,3.654947264,7.391356792));
#123047=CARTESIAN_POINT('Ctrl Pts',(0.213507122,3.784676613,7.246855505));
#123048=CARTESIAN_POINT('Ctrl Pts',(0.605805226,3.720089779,7.23529760400001));
#123049=CARTESIAN_POINT('Ctrl Pts',(0.994563149000001,3.654947264,7.181458358));
#123050=CARTESIAN_POINT('',(0.466609583418929,3.78467661255747,7.485470961005));
#123051=CARTESIAN_POINT('Origin',(-0.037121924407804,3.62502541058654,-0.186844580745509));
#123052=CARTESIAN_POINT('',(0.340058346887876,3.78467661169947,7.36616323287449));
#123053=CARTESIAN_POINT('Origin',(1.22352215164989E-13,3.87542692000033,
9.23306570088656E-13));
#123054=CARTESIAN_POINT('',(1.0294825429063,3.87435041278135,7.42900839215867));
#123055=CARTESIAN_POINT('Origin',(-0.0635989656444805,3.62514698225777,
-0.173527014489177));
#123056=CARTESIAN_POINT('Origin',(-0.0480202374533851,4.0177429109103,-0.179765932794114));
#123057=CARTESIAN_POINT('Origin',(-1.14342671615753E-13,3.87542691999933,
1.13884596197877E-12));
#123058=CARTESIAN_POINT('',(-0.0251083328437495,3.784676612654,7.49995797182608));
#123059=CARTESIAN_POINT('Ctrl Pts',(-0.0251083344734971,3.78467661270495,
7.4999579705691));
#123060=CARTESIAN_POINT('Ctrl Pts',(-0.0988532380978356,3.77306479305815,
7.49971108777196));
#123061=CARTESIAN_POINT('Ctrl Pts',(-0.172488069042823,3.76150355535486,
7.49837666610599));
#123062=CARTESIAN_POINT('Ctrl Pts',(-0.245965641750855,3.74999999995948,
7.49596564148352));
#123063=CARTESIAN_POINT('Ctrl Pts',(-0.362346987351099,3.73177948469136,
7.49214681183236));
#123064=CARTESIAN_POINT('Ctrl Pts',(-0.478945166289772,3.71341418839415,
7.48560612447644));
#123065=CARTESIAN_POINT('Ctrl Pts',(-0.595569421730545,3.69493258345309,
7.4763157408961));
#123066=CARTESIAN_POINT('',(-0.591603389574171,3.87435041291099,7.47663061978449));
#123067=CARTESIAN_POINT('Origin',(-0.0248088887967525,3.62514697597139,
-0.183141684594958));
#123068=CARTESIAN_POINT('Origin',(-0.00825320893698786,4.0177429119903,
-0.185885846195389));
#123069=CARTESIAN_POINT('Ctrl Pts',(-0.846826616,3.654941533,7.452038961));
#123070=CARTESIAN_POINT('Ctrl Pts',(-0.547278984,3.702826767,7.48607862600001));
#123071=CARTESIAN_POINT('Ctrl Pts',(-0.245965642,3.75,7.495965642));
#123072=CARTESIAN_POINT('Ctrl Pts',(-0.135566387,3.767283967,7.49958818));
#123073=CARTESIAN_POINT('Ctrl Pts',(-0.025108333,3.784676613,7.499957971));
#123074=CARTESIAN_POINT('Ctrl Pts',(-0.581912411,3.654941533,7.226609021));
#123075=CARTESIAN_POINT('Ctrl Pts',(-0.291426326,3.702826767,7.25));
#123076=CARTESIAN_POINT('Ctrl Pts',(0.,3.75,7.25));
#123077=CARTESIAN_POINT('Ctrl Pts',(0.106776717,3.767283967,7.25));
#123078=CARTESIAN_POINT('Ctrl Pts',(0.213507122,3.784676613,7.246855505));
#123079=CARTESIAN_POINT('',(0.094199399372222,3.78467661221161,7.37340673793775));
#123080=CARTESIAN_POINT('Ctrl Pts',(-0.037636821,1.973534152,7.499905564));
#123081=CARTESIAN_POINT('Ctrl Pts',(0.373348407,2.039276147,7.501968014));
#123082=CARTESIAN_POINT('Ctrl Pts',(0.782098092,2.104034486,7.459110039));
#123083=CARTESIAN_POINT('Ctrl Pts',(0.201401104,1.973534152,7.247202053));
#123084=CARTESIAN_POINT('Ctrl Pts',(0.598538503,2.039276147,7.23616553));
#123085=CARTESIAN_POINT('Ctrl Pts',(0.992091961000001,2.104034486,7.18180016));
#123086=CARTESIAN_POINT('',(0.206148885799383,1.97432008506241,7.24706856114906));
#123087=CARTESIAN_POINT('Origin',(0.0109862546629633,1.8750787904931,-0.193835066307506));
#123088=CARTESIAN_POINT('Ctrl Pts',(0.206148889272356,1.97432008582198,
7.24706856091956));
#123089=CARTESIAN_POINT('Ctrl Pts',(0.207389323391247,1.98121389469559,
7.28865544780864));
#123090=CARTESIAN_POINT('Ctrl Pts',(0.20865216717907,1.98793719438241,7.33029549705021));
#123091=CARTESIAN_POINT('Ctrl Pts',(0.211215736360714,2.00105345756954,
7.41357575940194));
#123092=CARTESIAN_POINT('Ctrl Pts',(0.212517943973008,2.00745398499083,
7.45526404173224));
#123093=CARTESIAN_POINT('Ctrl Pts',(0.213837435628797,2.01370168115021,
7.49695094993264));
#123094=CARTESIAN_POINT('Ctrl Pts',(1.24240846169613,2.10851071898521,7.39695738032139));
#123095=CARTESIAN_POINT('Ctrl Pts',(1.25618820682232,2.10627260249257,7.39459004978026));
#123096=CARTESIAN_POINT('Ctrl Pts',(1.26996795194848,2.104034486,7.39222271923915));
#123097=CARTESIAN_POINT('Ctrl Pts',(1.67129990201488,2.038849851,7.32327475439542));
#123098=CARTESIAN_POINT('Ctrl Pts',(2.06280841283434,1.973541827,7.21128260348006));
#123099=CARTESIAN_POINT('Ctrl Pts',(0.965316962563659,2.10851071898521,
7.18549885113338));
#123100=CARTESIAN_POINT('Ctrl Pts',(0.978704461781823,2.10627260249257,
7.18364950556676));
#123101=CARTESIAN_POINT('Ctrl Pts',(0.992091961,2.104034486,7.18180016));
#123102=CARTESIAN_POINT('Ctrl Pts',(1.381999838,2.038849851,7.12793839));
#123103=CARTESIAN_POINT('Ctrl Pts',(1.763784701,1.973541827,7.032180567));
#123104=CARTESIAN_POINT('',(1.75923475770139,1.97432008459303,7.03332020118504));
#123105=CARTESIAN_POINT('Origin',(-0.04140142794191,2.0178567362601,-0.195280406556874));
#123106=CARTESIAN_POINT('Ctrl Pts',(1.82046088137077,2.01370168116173,7.27570767517235));
#123107=CARTESIAN_POINT('Ctrl Pts',(1.81021078533883,2.00745398478552,7.23527903401856));
#123108=CARTESIAN_POINT('Ctrl Pts',(1.79997727388742,2.00105345715051,7.19484533535441));
#123109=CARTESIAN_POINT('Ctrl Pts',(1.77957084490069,1.98793719393146,7.11406321064706));
#123110=CARTESIAN_POINT('Ctrl Pts',(1.76938614485983,1.98121389346264,7.07366815198737));
#123111=CARTESIAN_POINT('Ctrl Pts',(1.75923476045435,1.97432008482154,7.03332020138535));
#123112=CARTESIAN_POINT('Ctrl Pts',(1.575501108,1.973534152,7.33265274399999));
#123113=CARTESIAN_POINT('Ctrl Pts',(1.977321095,2.039276147,7.246317299));
#123114=CARTESIAN_POINT('Ctrl Pts',(2.367301242,2.104034486,7.11659222000001));
#123115=CARTESIAN_POINT('Ctrl Pts',(1.754626674,1.973534152,7.034471212));
#123116=CARTESIAN_POINT('Ctrl Pts',(2.140106694,2.039276147,6.938319916));
#123117=CARTESIAN_POINT('Ctrl Pts',(2.512772145,2.104034486,6.80062321800001));
#123118=CARTESIAN_POINT('Origin',(-0.0309385540210372,1.87507850637468,
-0.191662857044855));
#123119=CARTESIAN_POINT('Ctrl Pts',(2.8034888261742,2.10851071909229,6.95693953369873));
#123120=CARTESIAN_POINT('Ctrl Pts',(2.81643750274181,2.10627260254611,6.95166531203499));
#123121=CARTESIAN_POINT('Ctrl Pts',(2.82938617930937,2.104034486,6.94639109037137));
#123122=CARTESIAN_POINT('Ctrl Pts',(3.20651343716099,2.038849851,6.79278058485507));
#123123=CARTESIAN_POINT('Ctrl Pts',(3.56479369392208,1.973541827,6.59924399066095));
#123124=CARTESIAN_POINT('Ctrl Pts',(2.48741823987845,2.10851071909229,6.80999126923477));
#123125=CARTESIAN_POINT('Ctrl Pts',(2.50009519243922,2.10627260254611,6.80530724361737));
#123126=CARTESIAN_POINT('Ctrl Pts',(2.512772145,2.104034486,6.800623218));
#123127=CARTESIAN_POINT('Ctrl Pts',(2.881985503,2.038849851,6.664202038));
#123128=CARTESIAN_POINT('Ctrl Pts',(3.234259347,1.973541827,6.48861052));
#123129=CARTESIAN_POINT('',(3.23006076639947,1.97432008459905,6.49070161271792));
#123130=CARTESIAN_POINT('Origin',(-0.0824129386066702,2.0178567697538,-0.181814627491717));
#123131=CARTESIAN_POINT('Ctrl Pts',(3.34196159965903,2.01370168113681,6.71426039576969));
#123132=CARTESIAN_POINT('Ctrl Pts',(3.32326018235616,2.00745398477792,6.67698042153999));
#123133=CARTESIAN_POINT('Ctrl Pts',(3.30457387463032,2.00105345714848,6.63969194278597));
#123134=CARTESIAN_POINT('Ctrl Pts',(3.26727876750594,1.98793719395234,6.56518523846705));
#123135=CARTESIAN_POINT('Ctrl Pts',(3.24864843637574,1.98121389347921,6.52792400329991));
#123136=CARTESIAN_POINT('Ctrl Pts',(3.23006076876782,1.97432008483358,6.49070161298074));
#123137=CARTESIAN_POINT('Ctrl Pts',(3.114970356,1.973534152,6.822533231));
#123138=CARTESIAN_POINT('Ctrl Pts',(3.488836447,2.039276147,6.651836841));
#123139=CARTESIAN_POINT('Ctrl Pts',(3.841812017,2.104034486,6.441310459));
#123140=CARTESIAN_POINT('Ctrl Pts',(3.22580785,1.973534152,6.492816316));
#123141=CARTESIAN_POINT('Ctrl Pts',(3.581605876,2.039276147,6.316046174));
#123142=CARTESIAN_POINT('Ctrl Pts',(3.915957895,2.104034486,6.101456692));
#123143=CARTESIAN_POINT('Origin',(-0.071416952844599,1.87507855779732,-0.180530784418701));
#123144=CARTESIAN_POINT('Ctrl Pts',(4.23348117064494,2.10851071892058,6.19162292591988));
#123145=CARTESIAN_POINT('Ctrl Pts',(4.24499331214195,2.10627260246026,6.18368843020217));
#123146=CARTESIAN_POINT('Ctrl Pts',(4.25650545363899,2.104034486,6.17575393448443));
#123147=CARTESIAN_POINT('Ctrl Pts',(4.59179396738482,2.038849851,5.94466354376879));
#123148=CARTESIAN_POINT('Ctrl Pts',(4.90009318391161,1.973541827,5.67863206376884));
#123149=CARTESIAN_POINT('Ctrl Pts',(3.89321060504381,2.10851071892058,6.11605606300682));
#123150=CARTESIAN_POINT('Ctrl Pts',(3.9045842500219,2.10627260246026,6.10875637750341));
#123151=CARTESIAN_POINT('Ctrl Pts',(3.915957895,2.104034486,6.101456692));
#123152=CARTESIAN_POINT('Ctrl Pts',(4.247212729,2.038849851,5.88885500499999));
#123153=CARTESIAN_POINT('Ctrl Pts',(4.55350362,1.973541827,5.64164025600001));
#123154=CARTESIAN_POINT('',(4.54985272407125,1.97432008460192,5.64458503122448));
#123155=CARTESIAN_POINT('Origin',(-0.11957089886817,2.01785677029382,-0.159847509292501));
#123156=CARTESIAN_POINT('Ctrl Pts',(4.70719590746652,2.0137016811724,5.83886176251772));
#123157=CARTESIAN_POINT('Ctrl Pts',(4.68091762642383,2.00745398479891,5.80647362523456));
#123158=CARTESIAN_POINT('Ctrl Pts',(4.65465227342763,2.00105345713783,5.7740739340661));
#123159=CARTESIAN_POINT('Ctrl Pts',(4.60221236624691,1.98793719392138,5.709326500652));
#123160=CARTESIAN_POINT('Ctrl Pts',(4.57600753795865,1.98121389346668,5.67694138305711));
#123161=CARTESIAN_POINT('Ctrl Pts',(4.54985272626207,1.97432008483703,5.64458503070716));
#123162=CARTESIAN_POINT('Ctrl Pts',(4.508787052,1.973534152,5.993399646));
#123163=CARTESIAN_POINT('Ctrl Pts',(4.837217683,2.039276147,5.746323886));
#123164=CARTESIAN_POINT('Ctrl Pts',(5.136683932,2.104034486,5.464840179));
#123165=CARTESIAN_POINT('Ctrl Pts',(4.546153837,1.973534152,5.647564545));
#123166=CARTESIAN_POINT('Ctrl Pts',(4.855633147,2.039276147,5.398441132));
#123167=CARTESIAN_POINT('Ctrl Pts',(5.136037807,2.104034486,5.11699283300001));
#123168=CARTESIAN_POINT('Origin',(-0.108556179717638,1.87507852096226,-0.160957689532432));
#123169=CARTESIAN_POINT('Ctrl Pts',(5.4655206391911,2.10851071889853,5.13679291131898));
#123170=CARTESIAN_POINT('Ctrl Pts',(5.47505795112589,2.10627260244923,5.12656914964515));
#123171=CARTESIAN_POINT('Ctrl Pts',(5.48459526306069,2.104034486,5.11634538797148));
#123172=CARTESIAN_POINT('Ctrl Pts',(5.76236731444896,2.038849851,4.81858064331117));
#123173=CARTESIAN_POINT('Ctrl Pts',(6.00626976343028,1.973541827,4.49249361300632));
#123174=CARTESIAN_POINT('Ctrl Pts',(5.11696076933579,2.10851071889853,5.13614087365377));
#123175=CARTESIAN_POINT('Ctrl Pts',(5.12649928816785,2.10627260244923,5.12656685332694));
#123176=CARTESIAN_POINT('Ctrl Pts',(5.136037807,2.104034486,5.116992833));
#123177=CARTESIAN_POINT('Ctrl Pts',(5.413845009,2.038849851,4.838151658));
#123178=CARTESIAN_POINT('Ctrl Pts',(5.659831125,1.973541827,4.530873164));
#123179=CARTESIAN_POINT('',(5.65689862469295,1.97432008458259,4.53453392705498));
#123180=CARTESIAN_POINT('Origin',(-0.15113806033607,2.01785671859312,-0.130406290041515));
#123181=CARTESIAN_POINT('Ctrl Pts',(5.85232696622083,2.01370168119811,4.690444443045));
#123182=CARTESIAN_POINT('Ctrl Pts',(5.81970056460916,2.00745398481113,4.66446257602344));
#123183=CARTESIAN_POINT('Ctrl Pts',(5.78708430510987,2.00105345714669,4.63846664610439));
#123184=CARTESIAN_POINT('Ctrl Pts',(5.72195162961054,1.98793719392437,4.58650600150808));
#123185=CARTESIAN_POINT('Ctrl Pts',(5.68939761284271,1.98121389349597,4.56051129344533));
#123186=CARTESIAN_POINT('Ctrl Pts',(5.65689862700698,1.97432008489497,4.53453392596363));
#123187=CARTESIAN_POINT('Ctrl Pts',(5.691777876,1.973534152,4.884021356));
#123188=CARTESIAN_POINT('Ctrl Pts',(5.959415997,2.039276147,4.57211921199999));
#123189=CARTESIAN_POINT('Ctrl Pts',(6.191370215,2.104034486,4.232840047));
#123190=CARTESIAN_POINT('Ctrl Pts',(5.653926723,1.973534152,4.538238933));
#123191=CARTESIAN_POINT('Ctrl Pts',(5.902616409,2.039276147,4.228410983));
#123192=CARTESIAN_POINT('Ctrl Pts',(6.115962299,2.104034486,3.893264076));
#123193=CARTESIAN_POINT('Origin',(-0.140619339003883,1.87507853779743,-0.133858214553792));
#123194=CARTESIAN_POINT('Ctrl Pts',(6.44199843682638,2.10851071890015,3.84177217007522));
#123195=CARTESIAN_POINT('Ctrl Pts',(6.44911496517792,2.10627260245004,3.82973719410629));
#123196=CARTESIAN_POINT('Ctrl Pts',(6.45623149352946,2.104034486,3.81770221813728));
#123197=CARTESIAN_POINT('Ctrl Pts',(6.6634987709102,2.038849851,3.46718626721084));
#123198=CARTESIAN_POINT('Ctrl Pts',(6.83159984383339,1.973541827,3.09629115331911));
#123199=CARTESIAN_POINT('Ctrl Pts',(6.10144753458863,2.10851071890015,3.91606544531126));
#123200=CARTESIAN_POINT('Ctrl Pts',(6.10870491679432,2.10627260245004,3.90466476065566));
#123201=CARTESIAN_POINT('Ctrl Pts',(6.115962299,2.104034486,3.893264076));
#123202=CARTESIAN_POINT('Ctrl Pts',(6.327331913,2.038849851,3.561221716));
#123203=CARTESIAN_POINT('Ctrl Pts',(6.501511218,1.973541827,3.208247479));
#123204=CARTESIAN_POINT('',(6.49943423274117,1.97432008456978,3.21245305639565));
#123205=CARTESIAN_POINT('Origin',(-0.175638016403146,2.01785677543793,-0.0948672503717496));
#123206=CARTESIAN_POINT('Ctrl Pts',(6.72380972081394,2.01370168119116,3.32270715395686));
#123207=CARTESIAN_POINT('Ctrl Pts',(6.6863607730789,2.00745398482567,3.30434644058282));
#123208=CARTESIAN_POINT('Ctrl Pts',(6.64891870713716,2.00105345717049,3.28596981283331));
#123209=CARTESIAN_POINT('Ctrl Pts',(6.57413879473958,1.98793719396562,3.24922557947126));
#123210=CARTESIAN_POINT('Ctrl Pts',(6.53675777860832,1.98121389349064,3.23083676460714));
#123211=CARTESIAN_POINT('Ctrl Pts',(6.49943423450967,1.9743200848467,3.21245305497854));
#123212=CARTESIAN_POINT('Ctrl Pts',(6.608627494,1.973534152,3.546271655));
#123213=CARTESIAN_POINT('Ctrl Pts',(6.802958642,2.039276147,3.184127325));
#123214=CARTESIAN_POINT('Ctrl Pts',(6.956554908,2.104034486,2.802917018));
#123215=CARTESIAN_POINT('Ctrl Pts',(6.49732827900001,1.973534152,3.216710312));
#123216=CARTESIAN_POINT('Ctrl Pts',(6.67359988800001,2.039276147,2.860665037));
#123217=CARTESIAN_POINT('Ctrl Pts',(6.809911191,2.104034486,2.487490617));
#123218=CARTESIAN_POINT('Origin',(-0.166107150153769,1.87507854227463,-0.10049961351814));
#123219=CARTESIAN_POINT('Ctrl Pts',(7.11725554807123,2.10851071887221,2.36711443152886));
#123220=CARTESIAN_POINT('Ctrl Pts',(7.12161853182935,2.10627260243607,2.35383098346935));
#123221=CARTESIAN_POINT('Ctrl Pts',(7.12598151558734,2.104034486,2.34054753540986));
#123222=CARTESIAN_POINT('Ctrl Pts',(7.2530524307518,2.038849851,1.95367011503003));
#123223=CARTESIAN_POINT('Ctrl Pts',(7.33749190763721,1.973541827,1.55530956171743));
#123224=CARTESIAN_POINT('Ctrl Pts',(6.80063739414221,2.10851071887221,2.5128791480281));
#123225=CARTESIAN_POINT('Ctrl Pts',(6.80527429257119,2.10627260243607,2.50018488251402));
#123226=CARTESIAN_POINT('Ctrl Pts',(6.809911191,2.104034486,2.487490617));
#123227=CARTESIAN_POINT('Ctrl Pts',(6.944959809,2.038849851,2.117773005));
#123228=CARTESIAN_POINT('Ctrl Pts',(7.039187871,1.973541827,1.735607707));
#123229=CARTESIAN_POINT('',(7.03806351987006,1.97432008460083,1.74016145090013));
#123230=CARTESIAN_POINT('Origin',(-0.191925213452907,2.01785676680825,-0.0548922832922177));
#123231=CARTESIAN_POINT('Ctrl Pts',(7.28089460562994,2.01370168114298,1.7996037715632));
#123232=CARTESIAN_POINT('Ctrl Pts',(7.24037418281004,2.00745398477847,1.78972273822671));
#123233=CARTESIAN_POINT('Ctrl Pts',(7.19985705962638,2.0010534570977,1.77982468312593));
#123234=CARTESIAN_POINT('Ctrl Pts',(7.11892653610712,1.98793719390642,1.76001497998512));
#123235=CARTESIAN_POINT('Ctrl Pts',(7.07846641611887,1.98121389348972,1.75009189878342));
#123236=CARTESIAN_POINT('Ctrl Pts',(7.03806352196428,1.97432008490095,1.74016144855234));
#123237=CARTESIAN_POINT('Ctrl Pts',(7.216465034,1.973534152,2.042702233));
#123238=CARTESIAN_POINT('Ctrl Pts',(7.328402503,2.039276147,1.647249183));
#123239=CARTESIAN_POINT('Ctrl Pts',(7.39645882600001,2.104034486,1.241932705));
#123240=CARTESIAN_POINT('Ctrl Pts',(7.036921987,1.973534152,1.744771892));
#123241=CARTESIAN_POINT('Ctrl Pts',(7.132533254,2.039276147,1.359157572));
#123242=CARTESIAN_POINT('Ctrl Pts',(7.185436205,2.104034486,0.965404863));
#123243=CARTESIAN_POINT('Origin',(-0.183828099314221,1.87507853001457,-0.0624418681352172));
#123244=CARTESIAN_POINT('Ctrl Pts',(7.45971770060335,2.1085107188556,0.781773053483733));
#123245=CARTESIAN_POINT('Ctrl Pts',(7.46112313152621,2.10627260242776,0.767862252559916));
#123246=CARTESIAN_POINT('Ctrl Pts',(7.46252856244921,2.104034486,0.753951451636089));
#123247=CARTESIAN_POINT('Ctrl Pts',(7.50346142036284,2.038849851,0.348802519468778));
#123248=CARTESIAN_POINT('Ctrl Pts',(7.50029100568184,1.973541827,-0.0583965774922585));
#123249=CARTESIAN_POINT('Ctrl Pts',(7.18183700810203,2.1085107188556,0.992193416474425));
#123250=CARTESIAN_POINT('Ctrl Pts',(7.18363660655107,2.10627260242776,0.978799139737212));
#123251=CARTESIAN_POINT('Ctrl Pts',(7.185436205,2.104034486,0.965404863000001));
#123252=CARTESIAN_POINT('Ctrl Pts',(7.237849103,2.038849851,0.575299581));
#123253=CARTESIAN_POINT('Ctrl Pts',(7.247719923,1.973541827,0.181812848));
#123254=CARTESIAN_POINT('',(7.24760077907989,1.97432008459269,0.186501829852585));
#123255=CARTESIAN_POINT('Origin',(-0.199238328473579,2.01785675377979,-0.0123506811088942));
#123256=CARTESIAN_POINT('Ctrl Pts',(7.49753295086213,2.01370168117945,0.192352917068669));
#123257=CARTESIAN_POINT('Ctrl Pts',(7.45583574284584,2.00745398481533,0.191413589910291));
#123258=CARTESIAN_POINT('Ctrl Pts',(7.41413809829081,2.0010534571559,0.190456929640095));
#123259=CARTESIAN_POINT('Ctrl Pts',(7.33084118470819,1.98793719395886,0.18850803665614));
#123260=CARTESIAN_POINT('Ctrl Pts',(7.28919383066974,1.98121389353883,0.187514681429552));
#123261=CARTESIAN_POINT('Ctrl Pts',(7.24760078045297,1.97432008494145,0.186501827635298));
#123262=CARTESIAN_POINT('Ctrl Pts',(7.48686869,1.973534152,0.443618325));
#123263=CARTESIAN_POINT('Ctrl Pts',(7.511178407,2.039276147,0.033347501));
#123264=CARTESIAN_POINT('Ctrl Pts',(7.490512549,2.104034486,-0.377123002));
#123265=CARTESIAN_POINT('Ctrl Pts',(7.247477043,1.973534152,0.191249878));
#123266=CARTESIAN_POINT('Ctrl Pts',(7.257957291,2.039276147,-0.20590259));
#123267=CARTESIAN_POINT('Ctrl Pts',(7.224978208,2.104034486,-0.601822151));
#123268=CARTESIAN_POINT('Origin',(-0.192953490786607,1.87507854258771,-0.0214644009727091));
#123269=CARTESIAN_POINT('Ctrl Pts',(7.4533717437585,2.10851071889274,-0.840123164227433));
#123270=CARTESIAN_POINT('Ctrl Pts',(7.45175390547986,2.10627260244634,-0.854010864545254));
#123271=CARTESIAN_POINT('Ctrl Pts',(7.45013606720136,2.104034486,-0.867898564863071));
#123272=CARTESIAN_POINT('Ctrl Pts',(7.40301689346621,2.038849851,-1.27237469374659));
#123273=CARTESIAN_POINT('Ctrl Pts',(7.31238483253978,1.973541827,-1.6693721570991));
#123274=CARTESIAN_POINT('Ctrl Pts',(7.22722190550252,2.10851071889274,-0.574886177926066));
#123275=CARTESIAN_POINT('Ctrl Pts',(7.2261000567513,2.10627260244633,-0.588354164463037));
#123276=CARTESIAN_POINT('Ctrl Pts',(7.224978208,2.104034486,-0.601822151));
#123277=CARTESIAN_POINT('Ctrl Pts',(7.192304617,2.038849851,-0.994074210999999));
#123278=CARTESIAN_POINT('Ctrl Pts',(7.117356647,1.973541827,-1.380483378));
#123279=CARTESIAN_POINT('',(7.11824828114546,1.9743200846023,-1.37587840931435));
#123280=CARTESIAN_POINT('Origin',(-0.197235680099277,2.0178567977005,0.0307684671074535));
#123281=CARTESIAN_POINT('Ctrl Pts',(7.36359498822142,2.01370168115123,-1.42389214575026));
#123282=CARTESIAN_POINT('Ctrl Pts',(7.32267071009206,2.00745398477611,-1.41584584484626));
#123283=CARTESIAN_POINT('Ctrl Pts',(7.28174227990175,2.00105345716874,-1.40781637803124));
#123284=CARTESIAN_POINT('Ctrl Pts',(7.19997384729897,1.98793719396908,-1.39181333278929));
#123285=CARTESIAN_POINT('Ctrl Pts',(7.15908664290256,1.98121389351294,-1.38383051380209));
#123286=CARTESIAN_POINT('Ctrl Pts',(7.11824828113933,1.97432008488866,-1.37587841117222));
#123287=CARTESIAN_POINT('Ctrl Pts',(7.407194687,1.973534152,-1.176208683));
#123288=CARTESIAN_POINT('Ctrl Pts',(7.342739956,2.039276147,-1.582113474));
#123289=CARTESIAN_POINT('Ctrl Pts',(7.23431823,2.104034486,-1.978544855));
#123290=CARTESIAN_POINT('Ctrl Pts',(7.119148127,1.973534152,-1.371214768));
#123291=CARTESIAN_POINT('Ctrl Pts',(7.044007313,2.039276147,-1.761334976));
#123292=CARTESIAN_POINT('Ctrl Pts',(6.926688259,2.104034486,-2.140908629));
#123293=CARTESIAN_POINT('Origin',(-0.19305672921978,1.87507853802671,0.0205167763710182));
#123294=CARTESIAN_POINT('Ctrl Pts',(7.09851440741733,2.10851071884374,-2.42273615646732));
#123295=CARTESIAN_POINT('Ctrl Pts',(7.09394894829215,2.10627260242184,-2.43595138254796));
#123296=CARTESIAN_POINT('Ctrl Pts',(7.08938348916698,2.104034486,-2.44916660862854));
#123297=CARTESIAN_POINT('Ctrl Pts',(6.95641552388265,2.038849851,-2.83405708175071));
#123298=CARTESIAN_POINT('Ctrl Pts',(6.78255967079359,1.973541827,-3.20228974984045));
#123299=CARTESIAN_POINT('Ctrl Pts',(6.93466993796179,2.10851071884374,-2.1150847329012));
#123300=CARTESIAN_POINT('Ctrl Pts',(6.93067909848083,2.10627260242184,-2.12799668095063));
#123301=CARTESIAN_POINT('Ctrl Pts',(6.926688259,2.104034486,-2.140908629));
#123302=CARTESIAN_POINT('Ctrl Pts',(6.810455961,2.038849851,-2.516966198));
#123303=CARTESIAN_POINT('Ctrl Pts',(6.654193685,1.973541827,-2.878229735));
#123304=CARTESIAN_POINT('',(6.65605440469576,1.97432008458747,-2.87392410309619));
#123305=CARTESIAN_POINT('Origin',(-0.186009880413163,2.01785677534532,0.0724488708947763));
#123306=CARTESIAN_POINT('Ctrl Pts',(6.88534350778262,2.01370168114798,-2.97355759548525));
#123307=CARTESIAN_POINT('Ctrl Pts',(6.84710573362344,2.00745398479343,-2.95690190251033));
#123308=CARTESIAN_POINT('Ctrl Pts',(6.80886028528214,2.00105345714027,-2.94026175731253));
#123309=CARTESIAN_POINT('Ctrl Pts',(6.73244373526343,1.98793719394154,-2.90705505827984));
#123310=CARTESIAN_POINT('Ctrl Pts',(6.69422852120976,1.98121389346513,-2.89046933272022));
#123311=CARTESIAN_POINT('Ctrl Pts',(6.65605440477926,1.97432008481482,-2.8739241051104));
#123312=CARTESIAN_POINT('Ctrl Pts',(6.981168493,1.973534152,-2.741037481));
#123313=CARTESIAN_POINT('Ctrl Pts',(6.830963147,2.039276147,-3.123596581));
#123314=CARTESIAN_POINT('Ctrl Pts',(6.639855232,2.104034486,-3.487452151));
#123315=CARTESIAN_POINT('Ctrl Pts',(6.657935758,1.973534152,-2.869562936));
#123316=CARTESIAN_POINT('Ctrl Pts',(6.500687381,2.039276147,-3.234409296));
#123317=CARTESIAN_POINT('Ctrl Pts',(6.30451406700001,2.104034486,-3.579888599));
#123318=CARTESIAN_POINT('Origin',(-0.184132620718572,1.87507855398852,0.0615385729578144));
#123319=CARTESIAN_POINT('Ctrl Pts',(6.41173842758946,2.10851071904183,-3.89206469701236));
#123320=CARTESIAN_POINT('Ctrl Pts',(6.40443882310531,2.10627260252088,-3.90398952022805));
#123321=CARTESIAN_POINT('Ctrl Pts',(6.39713921862116,2.104034486,-3.9159143434438));
#123322=CARTESIAN_POINT('Ctrl Pts',(6.18453989704751,2.038849851,-4.26322210937211));
#123323=CARTESIAN_POINT('Ctrl Pts',(5.93558955777856,1.973541827,-4.5854718333146));
#123324=CARTESIAN_POINT('Ctrl Pts',(6.31786051367224,2.10851071904183,-3.55638427522397));
#123325=CARTESIAN_POINT('Ctrl Pts',(6.31118729033618,2.10627260252088,-3.56813643711199));
#123326=CARTESIAN_POINT('Ctrl Pts',(6.304514067,2.104034486,-3.579888599));
#123327=CARTESIAN_POINT('Ctrl Pts',(6.11015795399999,2.038849851,-3.922167643));
#123328=CARTESIAN_POINT('Ctrl Pts',(5.879888021,1.973541827,-4.241393269));
#123329=CARTESIAN_POINT('',(5.88263082204013,1.9743200845952,-4.23758830006517));
#123330=CARTESIAN_POINT('Origin',(-0.166086502365517,2.01785676854295,0.110741551565458));
#123331=CARTESIAN_POINT('Ctrl Pts',(6.08514101783681,2.01370168113767,-4.38418279590154));
#123332=CARTESIAN_POINT('Ctrl Pts',(6.05137770310302,2.0074539847697,-4.3596965126326));
#123333=CARTESIAN_POINT('Ctrl Pts',(6.01760355145,2.00105345713783,-4.33522376406238));
#123334=CARTESIAN_POINT('Ctrl Pts',(5.95011203634988,1.98793719393057,-4.28636611987748));
#123335=CARTESIAN_POINT('Ctrl Pts',(5.9163557133816,1.98121389345838,-4.26195301803478));
#123336=CARTESIAN_POINT('Ctrl Pts',(5.88263082133317,1.97432008481336,-4.23758830206259));
#123337=CARTESIAN_POINT('Ctrl Pts',(6.22871062,1.973534152,-4.177698412));
#123338=CARTESIAN_POINT('Ctrl Pts',(5.999778092,2.039276147,-4.519023783));
#123339=CARTESIAN_POINT('Ctrl Pts',(5.734919982,2.104034486,-4.83329006));
#123340=CARTESIAN_POINT('Ctrl Pts',(5.885405712,1.973534152,-4.23373353));
#123341=CARTESIAN_POINT('Ctrl Pts',(5.653402532,2.039276147,-4.556246232));
#123342=CARTESIAN_POINT('Ctrl Pts',(5.387547803,2.104034486,-4.85147695700001));
#123343=CARTESIAN_POINT('Origin',(-0.166598777824842,1.87507851971097,0.0996829389749004));
#123344=CARTESIAN_POINT('Ctrl Pts',(5.42515668504128,2.1085107190361,-5.17940461950462));
#123345=CARTESIAN_POINT('Ctrl Pts',(5.41546425676681,2.10627260251802,-5.18948144778066));
#123346=CARTESIAN_POINT('Ctrl Pts',(5.40577182849224,2.104034486,-5.19955827605677));
#123347=CARTESIAN_POINT('Ctrl Pts',(5.12348205749383,2.038849851,-5.49304360974979));
#123348=CARTESIAN_POINT('Ctrl Pts',(4.81107787356319,1.973541827,-5.75424235046432));
#123349=CARTESIAN_POINT('Ctrl Pts',(5.40563495191362,2.1085107190361,-4.83139124279361));
#123350=CARTESIAN_POINT('Ctrl Pts',(5.39659137745674,2.10627260251802,-4.84143409989687));
#123351=CARTESIAN_POINT('Ctrl Pts',(5.38754780300001,2.104034486,-4.851476957));
#123352=CARTESIAN_POINT('Ctrl Pts',(5.124155752,2.038849851,-5.143972888));
#123353=CARTESIAN_POINT('Ctrl Pts',(4.830645328,1.973541827,-5.406233968));
#123354=CARTESIAN_POINT('',(4.83414196006164,1.97432008459502,-5.40310757779746));
#123355=CARTESIAN_POINT('Origin',(-0.138397360010162,2.01785674122855,0.14385621189966));
#123356=CARTESIAN_POINT('Ctrl Pts',(5.00040409687359,2.01370168117331,-5.58980848170412));
#123357=CARTESIAN_POINT('Ctrl Pts',(4.9726939767263,2.00745398480132,-5.5586365595206));
#123358=CARTESIAN_POINT('Ctrl Pts',(4.94497036347981,2.00105345717066,-5.52747552602794));
#123359=CARTESIAN_POINT('Ctrl Pts',(4.88955971169157,1.98793719396736,-5.46525146592909));
#123360=CARTESIAN_POINT('Ctrl Pts',(4.86184068816398,1.98121389354149,-5.43415251759514));
#123361=CARTESIAN_POINT('Ctrl Pts',(4.83414195911806,1.9743200849399,-5.40310758066947));
#123362=CARTESIAN_POINT('Ctrl Pts',(5.18500516,1.973534152,-5.419014808));
#123363=CARTESIAN_POINT('Ctrl Pts',(4.88805008300001,2.039276147,-5.703146456));
#123364=CARTESIAN_POINT('Ctrl Pts',(4.561826248,2.104034486,-5.953128697));
#123365=CARTESIAN_POINT('Ctrl Pts',(4.837680637,1.973534152,-5.39993945));
#123366=CARTESIAN_POINT('Ctrl Pts',(4.541770865,2.039276147,-5.66503815800001));
#123367=CARTESIAN_POINT('Ctrl Pts',(4.218665792,2.104034486,-5.896215645));
#123368=CARTESIAN_POINT('Origin',(-0.14127475023858,1.87507852894051,0.133166015454209));
#123369=CARTESIAN_POINT('Ctrl Pts',(4.18490064535655,2.10851071908492,-6.22456133880191));
#123370=CARTESIAN_POINT('Ctrl Pts',(4.17326860033842,2.10627260254242,-6.23231899093966));
#123371=CARTESIAN_POINT('Ctrl Pts',(4.16163655532026,2.104034486,-6.24007664307739));
#123372=CARTESIAN_POINT('Ctrl Pts',(3.82285589111545,2.038849851,-6.46601649628373));
#123373=CARTESIAN_POINT('Ctrl Pts',(3.46160553536181,1.973541827,-6.65395088997058));
#123374=CARTESIAN_POINT('Ctrl Pts',(4.24064790846959,2.10851071908492,-5.88048772585869));
#123375=CARTESIAN_POINT('Ctrl Pts',(4.22965685023479,2.10627260254242,-5.88835168542928));
#123376=CARTESIAN_POINT('Ctrl Pts',(4.218665792,2.104034486,-5.89621564500001));
#123377=CARTESIAN_POINT('Ctrl Pts',(3.898553722,2.038849851,-6.125251678));
#123378=CARTESIAN_POINT('Ctrl Pts',(3.555527029,1.973541827,-6.31828517400001));
#123379=CARTESIAN_POINT('',(3.55961399279641,1.97432008460497,-6.31598355033228));
#123380=CARTESIAN_POINT('Origin',(-0.104236902038956,2.01785675819182,0.170244306810112));
#123381=CARTESIAN_POINT('Ctrl Pts',(3.68185383783361,2.0137016811815,-6.53406093560932));
#123382=CARTESIAN_POINT('Ctrl Pts',(3.66149260672337,2.00745398479605,-6.49766093882905));
#123383=CARTESIAN_POINT('Ctrl Pts',(3.64111585723233,2.00105345715233,-6.46126867554373));
#123384=CARTESIAN_POINT('Ctrl Pts',(3.60037700929709,1.987937193926,-6.38858772696064));
#123385=CARTESIAN_POINT('Ctrl Pts',(3.57999139574734,1.9812138934833,-6.35225708390207));
#123386=CARTESIAN_POINT('Ctrl Pts',(3.55961399137252,1.97432008486823,-6.31598355218539));
#123387=CARTESIAN_POINT('Ctrl Pts',(3.898854622,1.973534152,-6.406944095));
#123388=CARTESIAN_POINT('Ctrl Pts',(3.547762284,2.039276147,-6.620596339));
#123389=CARTESIAN_POINT('Ctrl Pts',(3.175426589,2.104034486,-6.794605653));
#123390=CARTESIAN_POINT('Ctrl Pts',(3.563750991,1.973534152,-6.313650202));
#123391=CARTESIAN_POINT('Ctrl Pts',(3.217771039,2.039276147,-6.508939196));
#123392=CARTESIAN_POINT('Ctrl Pts',(2.852523658,2.104034486,-6.66525384200001));
#123393=CARTESIAN_POINT('Origin',(-0.109345230970199,1.87507853275137,0.160422895055139));
#123394=CARTESIAN_POINT('Ctrl Pts',(2.74896330201779,2.10851071888029,-6.97866448860505));
#123395=CARTESIAN_POINT('Ctrl Pts',(2.73593554242207,2.10627260244012,-6.9837402250486));
#123396=CARTESIAN_POINT('Ctrl Pts',(2.72290778282633,2.104034486,-6.98881596149228));
#123397=CARTESIAN_POINT('Ctrl Pts',(2.34347723180894,2.038849851,-7.13664563715395));
#123398=CARTESIAN_POINT('Ctrl Pts',(1.95027237023958,1.973541827,-7.24252808156075));
#123399=CARTESIAN_POINT('Ctrl Pts',(2.87737288146855,2.1085107188803,-6.65461913855489));
#123400=CARTESIAN_POINT('Ctrl Pts',(2.8649482697343,2.10627260244012,-6.65993649027745));
#123401=CARTESIAN_POINT('Ctrl Pts',(2.852523658,2.104034486,-6.665253842));
#123402=CARTESIAN_POINT('Ctrl Pts',(2.490659652,2.038849851,-6.820120508));
#123403=CARTESIAN_POINT('Ctrl Pts',(2.114156238,1.973541827,-6.934900389));
#123404=CARTESIAN_POINT('',(2.11864243188274,1.97432008458627,-6.93353115165319));
#123405=CARTESIAN_POINT('Origin',(-0.0652023946488164,2.01785671755945,
0.188671929289841));
#123406=CARTESIAN_POINT('Ctrl Pts',(2.19114418540924,2.01370168115789,-7.17278796232453));
#123407=CARTESIAN_POINT('Ctrl Pts',(2.17908391196442,2.00745398478866,-7.13286191455669));
#123408=CARTESIAN_POINT('Ctrl Pts',(2.16700682047428,2.00105345714571,-7.09294008337231));
#123409=CARTESIAN_POINT('Ctrl Pts',(2.14284467989806,1.98793719393754,-7.01320072699691));
#123410=CARTESIAN_POINT('Ctrl Pts',(2.13074568506423,1.98121389346194,-6.97333716964254));
#123411=CARTESIAN_POINT('Ctrl Pts',(2.11864243027874,1.97432008481779,-6.93353115313861));
#123412=CARTESIAN_POINT('Ctrl Pts',(2.430397975,1.973534152,-7.095291797));
#123413=CARTESIAN_POINT('Ctrl Pts',(2.041585064,2.039276147,-7.228474496));
#123414=CARTESIAN_POINT('Ctrl Pts',(1.640547511,2.104034486,-7.31837440000001));
#123415=CARTESIAN_POINT('Ctrl Pts',(2.12318431,1.973534152,-6.932141688));
#123416=CARTESIAN_POINT('Ctrl Pts',(1.743311816,2.039276147,-7.04848947199999));
#123417=CARTESIAN_POINT('Ctrl Pts',(1.353000687,2.104034486,-7.12263217800001));
#123418=CARTESIAN_POINT('Origin',(-0.0723025749741271,1.87507854736493,
0.180178118841089));
#123419=CARTESIAN_POINT('Ctrl Pts',(1.18448749191198,2.10851071904162,-7.40645304119193));
#123420=CARTESIAN_POINT('Ctrl Pts',(1.17067318028706,2.10627260252078,-7.40860952663705));
#123421=CARTESIAN_POINT('Ctrl Pts',(1.15685886866217,2.104034486,-7.4107660120822));
#123422=CARTESIAN_POINT('Ctrl Pts',(0.754520182233737,2.038849851,-7.47357316055654));
#123423=CARTESIAN_POINT('Ctrl Pts',(0.347746635845483,1.973541827,-7.4924527102599));
#123424=CARTESIAN_POINT('Ctrl Pts',(1.37955509720262,2.10851071904162,-7.1175879563888));
#123425=CARTESIAN_POINT('Ctrl Pts',(1.36627789210132,2.10627260252078,-7.12011006719445));
#123426=CARTESIAN_POINT('Ctrl Pts',(1.353000687,2.104034486,-7.122632178));
#123427=CARTESIAN_POINT('Ctrl Pts',(0.966305106,2.038849851,-7.196088082));
#123428=CARTESIAN_POINT('Ctrl Pts',(0.57392985,1.973541827,-7.22724736900001));
#123429=CARTESIAN_POINT('',(0.578605504968936,1.974320084601,-7.22687454289004));
#123430=CARTESIAN_POINT('Origin',(-0.0231191456018464,2.01785675782624,
0.198277636829115));
#123431=CARTESIAN_POINT('Ctrl Pts',(0.597979066411303,2.01370168115889,
-7.47612339587755));
#123432=CARTESIAN_POINT('Ctrl Pts',(0.594783675462212,2.00745398478028,
-7.4345381945658));
#123433=CARTESIAN_POINT('Ctrl Pts',(0.591570953207994,2.00105345716446,
-7.3929534961251));
#123434=CARTESIAN_POINT('Ctrl Pts',(0.585115314289111,1.98793719394626,
-7.30988425562794));
#123435=CARTESIAN_POINT('Ctrl Pts',(0.581868673498223,1.98121389348095,
-7.26835175999199));
#123436=CARTESIAN_POINT('Ctrl Pts',(0.57860550267337,1.97432008484254,-7.22687454419911));
#123437=CARTESIAN_POINT('Ctrl Pts',(0.84829862,1.973534152,-7.45187154));
#123438=CARTESIAN_POINT('Ctrl Pts',(0.439945595,2.039276147,-7.498357219));
#123439=CARTESIAN_POINT('Ctrl Pts',(0.028958256,2.104034486,-7.499944094));
#123440=CARTESIAN_POINT('Ctrl Pts',(0.58333989,1.973534152,-7.226493934));
#123441=CARTESIAN_POINT('Ctrl Pts',(0.18733727,2.039276147,-7.258460213));
#123442=CARTESIAN_POINT('Ctrl Pts',(-0.209787092,2.104034486,-7.246964149));
#123443=CARTESIAN_POINT('Origin',(-0.0318792104160436,1.87507852637965,
0.191508478928001));
#123444=CARTESIAN_POINT('Ctrl Pts',(-0.435373639053406,2.10851071889989,
-7.48792408298776));
#123445=CARTESIAN_POINT('Ctrl Pts',(-0.449328559925206,2.10627260244991,
-7.48706048234279));
#123446=CARTESIAN_POINT('Ctrl Pts',(-0.463283480797019,2.104034486,-7.4861968816978));
#123447=CARTESIAN_POINT('Ctrl Pts',(-0.869717392453361,2.038849851,-7.46104470839085));
#123448=CARTESIAN_POINT('Ctrl Pts',(-1.27103934506489,1.973541827,-7.39203857617524));
#123449=CARTESIAN_POINT('Ctrl Pts',(-0.182769151482024,2.10851071889989,
-7.24774627167939));
#123450=CARTESIAN_POINT('Ctrl Pts',(-0.196278121741014,2.10627260244991,
-7.24735521033965));
#123451=CARTESIAN_POINT('Ctrl Pts',(-0.209787092,2.104034486,-7.246964149));
#123452=CARTESIAN_POINT('Ctrl Pts',(-0.603232793,2.038849851,-7.235574576));
#123453=CARTESIAN_POINT('Ctrl Pts',(-0.993132859,1.973541827,-7.18165629400001));
#123454=CARTESIAN_POINT('',(-0.988486371605164,1.97432008459582,-7.18229731209575));
#123455=CARTESIAN_POINT('Origin',(0.0200451930811343,2.01785676284002,0.198611868378687));
#123456=CARTESIAN_POINT('Ctrl Pts',(-1.02314688972635,2.01370168116698,
-7.42988360828839));
#123457=CARTESIAN_POINT('Ctrl Pts',(-1.01732798509792,2.00745398479636,
-7.38858373133107));
#123458=CARTESIAN_POINT('Ctrl Pts',(-1.01152611461238,2.00105345715369,
-7.34728061954436));
#123459=CARTESIAN_POINT('Ctrl Pts',(-0.999973392743274,1.98793719394499,
-7.26476572021039));
#123460=CARTESIAN_POINT('Ctrl Pts',(-0.99421586977725,1.9812138934727,-7.22350629936079));
#123461=CARTESIAN_POINT('Ctrl Pts',(-0.988486373856812,1.97432008483443,
-7.18229731246988));
#123462=CARTESIAN_POINT('Ctrl Pts',(-0.773466236,1.973534152,-7.460010052));
#123463=CARTESIAN_POINT('Ctrl Pts',(-1.182265241,2.039276147,-7.417625092));
#123464=CARTESIAN_POINT('Ctrl Pts',(-1.583985056,2.104034486,-7.330824738));
#123465=CARTESIAN_POINT('Ctrl Pts',(-0.983780854,1.973534152,-7.182943354));
#123466=CARTESIAN_POINT('Ctrl Pts',(-1.377396959,2.039276147,-7.129033422));
#123467=CARTESIAN_POINT('Ctrl Pts',(-1.76276546,2.104034486,-7.032436131));
#123468=CARTESIAN_POINT('Origin',(0.010034762528979,1.87507853927421,0.193884179309698));
#123469=CARTESIAN_POINT('Ctrl Pts',(-2.03487718223917,2.10851071886228,
-7.21926811592231));
#123470=CARTESIAN_POINT('Ctrl Pts',(-2.04832019608257,2.1062726024311,-7.21542481034134));
#123471=CARTESIAN_POINT('Ctrl Pts',(-2.0617632099259,2.104034486,-7.21158150476034));
#123472=CARTESIAN_POINT('Ctrl Pts',(-2.45328794854016,2.038849851,-7.09964609871615));
#123473=CARTESIAN_POINT('Ctrl Pts',(-2.83039293831185,1.973541827,-6.9459809348642));
#123474=CARTESIAN_POINT('Ctrl Pts',(-1.73654731743755,2.10851071886228,
-7.03900802662101));
#123475=CARTESIAN_POINT('Ctrl Pts',(-1.74965638871877,2.1062726024311,-7.03572207881043));
#123476=CARTESIAN_POINT('Ctrl Pts',(-1.76276546,2.104034486,-7.032436131));
#123477=CARTESIAN_POINT('Ctrl Pts',(-2.144564197,2.038849851,-6.936733644));
#123478=CARTESIAN_POINT('Ctrl Pts',(-2.51375778,1.973541827,-6.800258953));
#123479=CARTESIAN_POINT('',(-2.50935772461844,1.97432008459731,-6.80188384142906));
#123480=CARTESIAN_POINT('Origin',(0.0622722465869113,2.01785673676985,0.189659333559888));
#123481=CARTESIAN_POINT('Ctrl Pts',(-2.59643163413031,2.01370168117248,
-7.03623072135717));
#123482=CARTESIAN_POINT('Ctrl Pts',(-2.58187051952417,2.00745398481506,
-6.99714730511095));
#123483=CARTESIAN_POINT('Ctrl Pts',(-2.56732534538734,2.0010534571731,-6.95805706773284));
#123484=CARTESIAN_POINT('Ctrl Pts',(-2.53830445549343,1.98793719398528,
-6.87995481461199));
#123485=CARTESIAN_POINT('Ctrl Pts',(-2.52381198434064,1.98121389351532,
-6.84089771329464));
#123486=CARTESIAN_POINT('Ctrl Pts',(-2.50935772681519,1.97432008487983,
-6.80188384184303));
#123487=CARTESIAN_POINT('Ctrl Pts',(-2.35906467,1.973534152,-7.119326786));
#123488=CARTESIAN_POINT('Ctrl Pts',(-2.749194668,2.039276147,-6.990053061));
#123489=CARTESIAN_POINT('Ctrl Pts',(-3.122862986,2.104034486,-6.81892416500001));
#123490=CARTESIAN_POINT('Ctrl Pts',(-2.504901099,1.973534152,-6.80352632700001));
#123491=CARTESIAN_POINT('Ctrl Pts',(-2.877725636,2.039276147,-6.666260952));
#123492=CARTESIAN_POINT('Ctrl Pts',(-3.233318874,2.104034486,-6.489079215));
#123493=CARTESIAN_POINT('Origin',(0.0514794804254071,1.87507852070844,0.187194023090833));
#123494=CARTESIAN_POINT('Ctrl Pts',(-3.53923212928303,2.1085107188304,-6.61304719479122));
#123495=CARTESIAN_POINT('Ctrl Pts',(-3.5515346557452,2.10627260241517,-6.60640389301813));
#123496=CARTESIAN_POINT('Ctrl Pts',(-3.56383718220737,2.104034486,-6.59976059124501));
#123497=CARTESIAN_POINT('Ctrl Pts',(-3.92214548626936,2.038849851,-6.40627592782908));
#123498=CARTESIAN_POINT('Ctrl Pts',(-4.25740050355622,1.973541827,-6.17513694492405));
#123499=CARTESIAN_POINT('Ctrl Pts',(-3.20912646050364,2.10851071883041,
-6.50113358894312));
#123500=CARTESIAN_POINT('Ctrl Pts',(-3.22122266725182,2.10627260241517,
-6.4951064019715));
#123501=CARTESIAN_POINT('Ctrl Pts',(-3.233318874,2.104034486,-6.489079215));
#123502=CARTESIAN_POINT('Ctrl Pts',(-3.585618163,2.038849851,-6.313538756));
#123503=CARTESIAN_POINT('Ctrl Pts',(-3.91684218,1.973541827,-6.100889061));
#123504=CARTESIAN_POINT('',(-3.91289429922261,1.97432008459373,-6.10342184278226));
#123505=CARTESIAN_POINT('Origin',(0.10158756789478,2.01785674361773,0.171838632592149));
#123506=CARTESIAN_POINT('Ctrl Pts',(-4.04831012087656,2.01370168115928,
-6.31357150580349));
#123507=CARTESIAN_POINT('Ctrl Pts',(-4.02568765781778,2.00745398480099,
-6.27853204729133));
#123508=CARTESIAN_POINT('Ctrl Pts',(-4.00307929618702,2.00105345714537,
-6.24348250033079));
#123509=CARTESIAN_POINT('Ctrl Pts',(-3.95794722285307,1.98793719394509,
-6.1734448678984));
#123510=CARTESIAN_POINT('Ctrl Pts',(-3.93539745539647,1.98121389347014,
-6.13841635280565));
#123511=CARTESIAN_POINT('Ctrl Pts',(-3.91289430129604,1.97432008482122,
-6.10342184208376));
#123512=CARTESIAN_POINT('Ctrl Pts',(-3.834355862,1.973534152,-6.445751711));
#123513=CARTESIAN_POINT('Ctrl Pts',(-4.187574808,2.039276147,-6.235633917));
#123514=CARTESIAN_POINT('Ctrl Pts',(-4.515719315,2.104034486,-5.988178277));
#123515=CARTESIAN_POINT('Ctrl Pts',(-3.908894953,1.973534152,-6.10598397));
#123516=CARTESIAN_POINT('Ctrl Pts',(-4.243495061,2.039276147,-5.891781529));
#123517=CARTESIAN_POINT('Ctrl Pts',(-4.552685891,2.104034486,-5.64230016800001));
#123518=CARTESIAN_POINT('Origin',(0.0905172887651684,1.87507854014182,0.171751205712217));
#123519=CARTESIAN_POINT('Ctrl Pts',(-4.87809651566979,2.10851071879243,
-5.69760753822029));
#123520=CARTESIAN_POINT('Ctrl Pts',(-4.88868330231458,2.10627260239619,
-5.68847487366332));
#123521=CARTESIAN_POINT('Ctrl Pts',(-4.89927008895948,2.104034486,-5.67934220910619));
#123522=CARTESIAN_POINT('Ctrl Pts',(-5.20760786104499,2.038849851,-5.41335541469936));
#123523=CARTESIAN_POINT('Ctrl Pts',(-5.48533675284584,1.973541827,-5.11555041405222));
#123524=CARTESIAN_POINT('Ctrl Pts',(-4.53165041691484,2.10851071879244,
-5.65927337102369));
#123525=CARTESIAN_POINT('Ctrl Pts',(-4.54216815395742,2.10627260239619,
-5.65078676951184));
#123526=CARTESIAN_POINT('Ctrl Pts',(-4.552685891,2.104034486,-5.642300168));
#123527=CARTESIAN_POINT('Ctrl Pts',(-4.859012609,2.038849851,-5.395129814));
#123528=CARTESIAN_POINT('Ctrl Pts',(-5.136779394,1.973541827,-5.116248377));
#123529=CARTESIAN_POINT('',(-5.13346828566157,1.97432008459591,-5.11957062092842));
#123530=CARTESIAN_POINT('Origin',(0.136152707978381,2.01785677842596,0.145982787016607));
#123531=CARTESIAN_POINT('Ctrl Pts',(-5.31089412599479,2.01370168116644,
-5.29569670360671));
#123532=CARTESIAN_POINT('Ctrl Pts',(-5.28126811575688,2.00745398480778,
-5.26633960900817));
#123533=CARTESIAN_POINT('Ctrl Pts',(-5.2516537084966,2.0010534571446,-5.23696963039117));
#123534=CARTESIAN_POINT('Ctrl Pts',(-5.19252077725244,1.98793719395353,
-5.17827150052631));
#123535=CARTESIAN_POINT('Ctrl Pts',(-5.16296811547313,1.98121389348676,
-5.1489094660589));
#123536=CARTESIAN_POINT('Ctrl Pts',(-5.1334682871504,1.97432008485722,-5.11957062045771));
#123537=CARTESIAN_POINT('Ctrl Pts',(-5.130356836,1.973534152,-5.470780451));
#123538=CARTESIAN_POINT('Ctrl Pts',(-5.430148604,2.039276147,-5.189643461));
#123539=CARTESIAN_POINT('Ctrl Pts',(-5.69742562700001,2.104034486,-4.877431827));
#123540=CARTESIAN_POINT('Ctrl Pts',(-5.130113223,1.973534152,-5.122932589));
#123541=CARTESIAN_POINT('Ctrl Pts',(-5.41084337400001,2.039276147,-4.841808949));
#123542=CARTESIAN_POINT('Ctrl Pts',(-5.659174375,2.104034486,-4.531693435));
#123543=CARTESIAN_POINT('Origin',(0.125322351826307,1.87507854796951,0.148277099444511));
#123544=CARTESIAN_POINT('Ctrl Pts',(-5.98886652981042,2.10851071902134,
-4.51575408564252));
#123545=CARTESIAN_POINT('Ctrl Pts',(-5.99724255079195,2.10627260251063,
-4.50455909097158));
#123546=CARTESIAN_POINT('Ctrl Pts',(-6.00561857177351,2.104034486,-4.49336409630082));
#123547=CARTESIAN_POINT('Ctrl Pts',(-6.24956828030743,2.038849851,-4.16731241937841));
#123548=CARTESIAN_POINT('Ctrl Pts',(-6.45678475223118,1.973541827,-3.81676643166152));
#123549=CARTESIAN_POINT('Ctrl Pts',(-5.64227943465445,2.10851071902134,
-4.55279182017937));
#123550=CARTESIAN_POINT('Ctrl Pts',(-5.65072690482716,2.10627260251063,
-4.5422426275897));
#123551=CARTESIAN_POINT('Ctrl Pts',(-5.659174375,2.104034486,-4.531693435));
#123552=CARTESIAN_POINT('Ctrl Pts',(-5.905205025,2.038849851,-4.224450597));
#123553=CARTESIAN_POINT('Ctrl Pts',(-6.116526512,1.973541827,-3.892377606));
#123554=CARTESIAN_POINT('',(-6.11400699946281,1.97432008458578,-3.89633396849977));
#123555=CARTESIAN_POINT('Origin',(0.164351554709555,2.01785674952642,0.113301003398673));
#123556=CARTESIAN_POINT('Ctrl Pts',(-6.32514662409162,2.01370168115646,
-4.03020100952011));
#123557=CARTESIAN_POINT('Ctrl Pts',(-6.28990234594244,2.00745398478208,
-4.0078989838217));
#123558=CARTESIAN_POINT('Ctrl Pts',(-6.25466663006614,2.00105345714523,
-3.98558188120025));
#123559=CARTESIAN_POINT('Ctrl Pts',(-6.18429783112559,1.98793719392257,
-3.9409679131739));
#123560=CARTESIAN_POINT('Ctrl Pts',(-6.14912412478396,1.98121389345093,
-3.91864529551827));
#123561=CARTESIAN_POINT('Ctrl Pts',(-6.11400700156398,1.97432008480395,
-3.89633396700648));
#123562=CARTESIAN_POINT('Ctrl Pts',(-6.18646802600001,1.973534152,-4.240001576));
#123563=CARTESIAN_POINT('Ctrl Pts',(-6.418814686,2.039276147,-3.900991045));
#123564=CARTESIAN_POINT('Ctrl Pts',(-6.612726649,2.104034486,-3.538622086));
#123565=CARTESIAN_POINT('Ctrl Pts',(-6.111453101,1.973534152,-3.900338574));
#123566=CARTESIAN_POINT('Ctrl Pts',(-6.325186664,2.039276147,-3.565438765));
#123567=CARTESIAN_POINT('Ctrl Pts',(-6.50104615600001,2.104034486,-3.209189754));
#123568=CARTESIAN_POINT('Origin',(0.154267558917515,1.87507849351964,0.117869865208854));
#123569=CARTESIAN_POINT('Ctrl Pts',(-6.81960380217781,2.1085107190505,-3.12274899058748));
#123570=CARTESIAN_POINT('Ctrl Pts',(-6.82537740354237,2.10627260252522,
-3.11001513168578));
#123571=CARTESIAN_POINT('Ctrl Pts',(-6.83115100490693,2.104034486,-3.09728127278417));
#123572=CARTESIAN_POINT('Ctrl Pts',(-6.99930583212112,2.038849851,-2.72641052709678));
#123573=CARTESIAN_POINT('Ctrl Pts',(-7.12632067321807,1.973541827,-2.33951469307138));
#123574=CARTESIAN_POINT('Ctrl Pts',(-6.48908173904204,2.1085107190505,-3.23342678355775));
#123575=CARTESIAN_POINT('Ctrl Pts',(-6.49506394752096,2.10627260252522,
-3.22130826877888));
#123576=CARTESIAN_POINT('Ctrl Pts',(-6.501046156,2.104034486,-3.209189754));
#123577=CARTESIAN_POINT('Ctrl Pts',(-6.675276618,2.038849851,-2.856240766));
#123578=CARTESIAN_POINT('Ctrl Pts',(-6.810271649,1.973541827,-2.486503584));
#123579=CARTESIAN_POINT('',(-6.80866154187226,1.97432008459362,-2.49090906853672));
#123580=CARTESIAN_POINT('Origin',(0.184865071285617,2.01785679395891,0.0753211970401979));
#123581=CARTESIAN_POINT('Ctrl Pts',(-7.04364229597177,2.0137016811527,-2.57625759581218));
#123582=CARTESIAN_POINT('Ctrl Pts',(-7.00442773317143,2.00745398478086,
-2.56205345706551));
#123583=CARTESIAN_POINT('Ctrl Pts',(-6.96521829159588,2.00105345718054,
-2.54783275332503));
#123584=CARTESIAN_POINT('Ctrl Pts',(-6.8869039917953,1.98793719395232,-2.51938904670658));
#123585=CARTESIAN_POINT('Ctrl Pts',(-6.8477539241966,1.98121389345868,-2.50514962650101));
#123586=CARTESIAN_POINT('Ctrl Pts',(-6.80866154374563,1.97432008478381,
-2.49090906776778));
#123587=CARTESIAN_POINT('Ctrl Pts',(-6.953306846,1.973534152,-2.810964941));
#123588=CARTESIAN_POINT('Ctrl Pts',(-7.107344128,2.039276147,-2.429932623));
#123589=CARTESIAN_POINT('Ctrl Pts',(-7.21882392200001,2.104034486,-2.03435031));
#123590=CARTESIAN_POINT('Ctrl Pts',(-6.807028224,1.973534152,-2.495369062));
#123591=CARTESIAN_POINT('Ctrl Pts',(-6.943771255,2.039276147,-2.122352626));
#123592=CARTESIAN_POINT('Ctrl Pts',(-7.038936244,2.104034486,-1.736627927));
#123593=CARTESIAN_POINT('Origin',(0.175999427533899,1.87507851689146,0.0819511757973274));
#123594=CARTESIAN_POINT('Ctrl Pts',(-7.33146397982346,2.10851071905646,
-1.58372762280809));
#123595=CARTESIAN_POINT('Ctrl Pts',(-7.33436519435819,2.10627260252819,
-1.57005032079825));
#123596=CARTESIAN_POINT('Ctrl Pts',(-7.33726640889282,2.104034486,-1.55637301878848));
#123597=CARTESIAN_POINT('Ctrl Pts',(-7.4217636225605,2.038849851,-1.1580247075818));
#123598=CARTESIAN_POINT('Ctrl Pts',(-7.46263775903092,1.973541827,-0.752869847803945));
#123599=CARTESIAN_POINT('Ctrl Pts',(-7.03246179338692,2.10851071905645,
-1.7628703042967));
#123600=CARTESIAN_POINT('Ctrl Pts',(-7.03569901869346,2.10627260252819,
-1.74974911564838));
#123601=CARTESIAN_POINT('Ctrl Pts',(-7.03893624400001,2.104034486,-1.736627927));
#123602=CARTESIAN_POINT('Ctrl Pts',(-7.13321969499999,2.038849851,-1.354476291));
#123603=CARTESIAN_POINT('Ctrl Pts',(-7.185576052,1.973541827,-0.964363417));
#123604=CARTESIAN_POINT('',(-7.1849506379579,1.97432008461106,-0.969012030082719));
#123605=CARTESIAN_POINT('Origin',(0.196735211445732,2.01785674944065,0.0338197687879882));
#123606=CARTESIAN_POINT('Ctrl Pts',(-7.43278508283959,2.01370168115849,
-1.00185123952923));
#123607=CARTESIAN_POINT('Ctrl Pts',(-7.39143386477347,2.00745398478806,
-0.996409157496566));
#123608=CARTESIAN_POINT('Ctrl Pts',(-7.35008408696195,2.00105345715456,
-0.990949796784439));
#123609=CARTESIAN_POINT('Ctrl Pts',(-7.26748617586181,1.98793719395952,
-0.980006347682499));
#123610=CARTESIAN_POINT('Ctrl Pts',(-7.22619036093368,1.98121389353513,
-0.97451594447279));
#123611=CARTESIAN_POINT('Ctrl Pts',(-7.18495063964874,1.97432008493794,
-0.969012028304344));
#123612=CARTESIAN_POINT('Ctrl Pts',(-7.395016767,1.973534152,-1.250490709));
#123613=CARTESIAN_POINT('Ctrl Pts',(-7.463542058,2.039276147,-0.845253253));
#123614=CARTESIAN_POINT('Ctrl Pts',(-7.487377012,2.104034486,-0.434954574));
#123615=CARTESIAN_POINT('Ctrl Pts',(-7.18431427300001,1.973534152,-0.973718867));
#123616=CARTESIAN_POINT('Ctrl Pts',(-7.237672821,2.039276147,-0.580027638));
#123617=CARTESIAN_POINT('Ctrl Pts',(-7.247693496,2.104034486,-0.182863309));
#123618=CARTESIAN_POINT('Origin',(0.189501763679538,1.87507855285121,0.0422005216901355));
#123619=CARTESIAN_POINT('Ctrl Pts',(-7.50051305040893,2.10851071891129,
0.029347089545044));
#123620=CARTESIAN_POINT('Ctrl Pts',(-7.50040622050944,2.10627260245561,
0.043328298730679));
#123621=CARTESIAN_POINT('Ctrl Pts',(-7.50029939060997,2.104034486,0.0573095079163131));
#123622=CARTESIAN_POINT('Ctrl Pts',(-7.4971879939768,2.038849851,0.464509059725814));
#123623=CARTESIAN_POINT('Ctrl Pts',(-7.45001019763226,1.973541827,0.868978355344865));
#123624=CARTESIAN_POINT('Ctrl Pts',(-7.24701174985858,2.10851071891129,
-0.209883968783856));
#123625=CARTESIAN_POINT('Ctrl Pts',(-7.24735262292936,2.10627260245561,
-0.196373638891925));
#123626=CARTESIAN_POINT('Ctrl Pts',(-7.247693496,2.104034486,-0.182863309));
#123627=CARTESIAN_POINT('Ctrl Pts',(-7.257621347,2.038849851,0.21062199));
#123628=CARTESIAN_POINT('Ctrl Pts',(-7.224890905,1.973541827,0.60286931));
#123629=CARTESIAN_POINT('',(-7.22527942719973,1.97432008458926,0.598194933891309));
#123630=CARTESIAN_POINT('Origin',(0.199405651581389,2.01785674870612,-0.00926317386782061));
#123631=CARTESIAN_POINT('Ctrl Pts',(-7.47437909993499,2.01370168117242,
0.619400567375759));
#123632=CARTESIAN_POINT('Ctrl Pts',(-7.43282476363654,2.00745398479686,
0.615826126927519));
#123633=CARTESIAN_POINT('Ctrl Pts',(-7.39126811926572,2.00105345711966,
0.612268870771427));
#123634=CARTESIAN_POINT('Ctrl Pts',(-7.30824878339747,1.98793719390629,
0.605200358586722));
#123635=CARTESIAN_POINT('Ctrl Pts',(-7.26673816734005,1.98121389347822,
0.601685019581431));
#123636=CARTESIAN_POINT('Ctrl Pts',(-7.22527942859502,1.97432008487502,
0.598194936057672));
#123637=CARTESIAN_POINT('Ctrl Pts',(-7.49094392300001,1.973534152,0.368455079));
#123638=CARTESIAN_POINT('Ctrl Pts',(-7.470753056,2.039276147,0.77894922));
#123639=CARTESIAN_POINT('Ctrl Pts',(-7.405828674,2.104034486,1.184779155));
#123640=CARTESIAN_POINT('Ctrl Pts',(-7.22566977100001,1.973534152,0.593461341));
#123641=CARTESIAN_POINT('Ctrl Pts',(-7.193148849,2.039276147,0.989418798));
#123642=CARTESIAN_POINT('Ctrl Pts',(-7.11755665600001,2.104034486,1.379451795));
#123643=CARTESIAN_POINT('Origin',(0.194143031294935,1.8750785217705,0.000476651582254073));
#123644=CARTESIAN_POINT('Ctrl Pts',(-7.31884646687648,2.10851071898058,
1.6410495620188));
#123645=CARTESIAN_POINT('Ctrl Pts',(-7.31573658785984,2.10627260249025,
1.65468093326815));
#123646=CARTESIAN_POINT('Ctrl Pts',(-7.3126267088431,2.104034486,1.6683123045175));
#123647=CARTESIAN_POINT('Ctrl Pts',(-7.22205218804354,2.038849851,2.06532289950042));
#123648=CARTESIAN_POINT('Ctrl Pts',(-7.08902844015126,1.973541827,2.45019409568082));
#123649=CARTESIAN_POINT('Ctrl Pts',(-7.12269949194147,2.10851071898057,
1.35291630753869));
#123650=CARTESIAN_POINT('Ctrl Pts',(-7.12012807397073,2.10627260249025,
1.36618405126933));
#123651=CARTESIAN_POINT('Ctrl Pts',(-7.117556656,2.104034486,1.379451795));
#123652=CARTESIAN_POINT('Ctrl Pts',(-7.042664691,2.038849851,1.765871821));
#123653=CARTESIAN_POINT('Ctrl Pts',(-6.92637789,1.973541827,2.141912539));
#123654=CARTESIAN_POINT('',(-6.92776218145332,1.97432008456834,2.13743096775303));
#123655=CARTESIAN_POINT('Origin',(0.192752513283734,2.01785674458455,-0.0519129632658388));
#123656=CARTESIAN_POINT('Ctrl Pts',(-7.16647945765253,2.01370168118037,
2.21168989111538));
#123657=CARTESIAN_POINT('Ctrl Pts',(-7.12666503765107,2.00745398480427,
2.19926606514373));
#123658=CARTESIAN_POINT('Ctrl Pts',(-7.08684466969444,2.00105345716807,
2.18685852563209));
#123659=CARTESIAN_POINT('Ctrl Pts',(-7.00728580085381,1.98793719394073,
2.16210856820885));
#123660=CARTESIAN_POINT('Ctrl Pts',(-6.96750137361793,1.9812138934618,2.14975186042709));
#123661=CARTESIAN_POINT('Ctrl Pts',(-6.92776218168722,1.97432008480815,
2.13743096977317));
#123662=CARTESIAN_POINT('Ctrl Pts',(-7.236602866,1.973534152,1.970172316));
#123663=CARTESIAN_POINT('Ctrl Pts',(-7.128639944,2.039276147,2.366728893));
#123664=CARTESIAN_POINT('Ctrl Pts',(-6.977992019,2.104034486,2.749113927));
#123665=CARTESIAN_POINT('Ctrl Pts',(-6.929160981,1.973534152,2.132891956));
#123666=CARTESIAN_POINT('Ctrl Pts',(-6.812281231,2.039276147,2.512601111));
#123667=CARTESIAN_POINT('Ctrl Pts',(-6.654610777,2.104034486,2.877265266));
#123668=CARTESIAN_POINT('Origin',(0.189706688252155,1.87507854824575,-0.0412695740778762));
#123669=CARTESIAN_POINT('Ctrl Pts',(-6.79495875646654,2.10851071886654,
3.17601838304026));
#123670=CARTESIAN_POINT('Ctrl Pts',(-6.78899124297289,2.10627260243327,
3.18866252798723));
#123671=CARTESIAN_POINT('Ctrl Pts',(-6.78302372947934,2.104034486,3.20130667293425));
#123672=CARTESIAN_POINT('Ctrl Pts',(-6.6092212484499,2.038849851,3.56956453521749));
#123673=CARTESIAN_POINT('Ctrl Pts',(-6.39657159139358,1.973541827,3.91684148375803));
#123674=CARTESIAN_POINT('Ctrl Pts',(-6.66533772140354,2.10851071886654,
2.85245572181685));
#123675=CARTESIAN_POINT('Ctrl Pts',(-6.65997424920171,2.10627260243327,
2.86486049390841));
#123676=CARTESIAN_POINT('Ctrl Pts',(-6.654610777,2.104034486,2.877265266));
#123677=CARTESIAN_POINT('Ctrl Pts',(-6.49840086199999,2.038849851,3.238551448));
#123678=CARTESIAN_POINT('Ctrl Pts',(-6.303995142,1.973541827,3.580802319));
#123679=CARTESIAN_POINT('',(-6.30631047548681,1.97432008458569,3.57672310566895));
#123680=CARTESIAN_POINT('Origin',(0.177086448535698,2.01785677518475,-0.0921354177511241));
#123681=CARTESIAN_POINT('Ctrl Pts',(-6.52348320097802,2.01370168114992,
3.70056305449002));
#123682=CARTESIAN_POINT('Ctrl Pts',(-6.48727037534077,2.00745398478357,
3.67987076733538));
#123683=CARTESIAN_POINT('Ctrl Pts',(-6.45104823951118,2.00105345713091,
3.65919310715007));
#123684=CARTESIAN_POINT('Ctrl Pts',(-6.37866992196166,1.98793719393924,
3.61791898507919));
#123685=CARTESIAN_POINT('Ctrl Pts',(-6.34247195938141,1.98121389348754,
3.59729869452439));
#123686=CARTESIAN_POINT('Ctrl Pts',(-6.30631047486903,1.97432008487082,
3.57672310798306));
#123687=CARTESIAN_POINT('Ctrl Pts',(-6.643886303,1.973534152,3.479766486));
#123688=CARTESIAN_POINT('Ctrl Pts',(-6.453199552,2.039276147,3.843842954));
#123689=CARTESIAN_POINT('Ctrl Pts',(-6.223872212,2.104034486,4.184903187));
#123690=CARTESIAN_POINT('Ctrl Pts',(-6.308652325,1.973534152,3.572590914));
#123691=CARTESIAN_POINT('Ctrl Pts',(-6.112878915,2.039276147,3.918296989));
#123692=CARTESIAN_POINT('Ctrl Pts',(-5.880502694,2.104034486,4.240541011));
#123693=CARTESIAN_POINT('Origin',(0.176399700379388,1.87507855895761,-0.0810860420883436));
#123694=CARTESIAN_POINT('Ctrl Pts',(-5.95334632705935,2.10851071891587,
4.56248011285926));
#123695=CARTESIAN_POINT('Ctrl Pts',(-5.94480021321551,2.1062726024579,4.57354580585008));
#123696=CARTESIAN_POINT('Ctrl Pts',(-5.93625409937179,2.104034486,4.58461149884087));
#123697=CARTESIAN_POINT('Ctrl Pts',(-5.68735046899805,2.038849851,4.90689730129712));
#123698=CARTESIAN_POINT('Ctrl Pts',(-5.40501816371079,1.973541827,5.20034171741082));
#123699=CARTESIAN_POINT('Ctrl Pts',(-5.89631216717291,2.10851071891587,
4.21861747586753));
#123700=CARTESIAN_POINT('Ctrl Pts',(-5.88840743058648,2.1062726024579,4.2295792434338));
#123701=CARTESIAN_POINT('Ctrl Pts',(-5.880502694,2.104034486,4.240541011));
#123702=CARTESIAN_POINT('Ctrl Pts',(-5.650279031,2.038849851,4.559800009));
#123703=CARTESIAN_POINT('Ctrl Pts',(-5.386844588,1.973541827,4.852257761));
#123704=CARTESIAN_POINT('',(-5.3899827002885,1.97432008460163,4.84877164614663));
#123705=CARTESIAN_POINT('Origin',(0.153139825866802,2.01785673863234,-0.128049668616968));
#123706=CARTESIAN_POINT('Ctrl Pts',(-5.57545611982729,2.0137016811512,5.01640200221225));
#123707=CARTESIAN_POINT('Ctrl Pts',(-5.5445381600034,2.00745398477771,4.98840880214805));
#123708=CARTESIAN_POINT('Ctrl Pts',(-5.51360796327672,2.00105345711284,
4.96042788561598));
#123709=CARTESIAN_POINT('Ctrl Pts',(-5.45179452686102,1.98793719392029,
4.90455953070735));
#123710=CARTESIAN_POINT('Ctrl Pts',(-5.4208756055621,1.98121389347575,4.87663983909214));
#123711=CARTESIAN_POINT('Ctrl Pts',(-5.3899826994675,1.97432008486875,4.84877164802182));
#123712=CARTESIAN_POINT('Ctrl Pts',(-5.740508999,1.973534152,4.826650643));
#123713=CARTESIAN_POINT('Ctrl Pts',(-5.476014721,2.039276147,5.14122319));
#123714=CARTESIAN_POINT('Ctrl Pts',(-5.17873105800001,2.104034486,5.42501102500001));
#123715=CARTESIAN_POINT('Ctrl Pts',(-5.393158098,1.973534152,4.845239491));
#123716=CARTESIAN_POINT('Ctrl Pts',(-5.127645174,2.039276147,5.140777654));
#123717=CARTESIAN_POINT('Ctrl Pts',(-4.831428841,2.104034486,5.405533772));
#123718=CARTESIAN_POINT('Origin',(0.154844449314781,1.87507851562995,-0.117110982067028));
#123719=CARTESIAN_POINT('Ctrl Pts',(-4.83336204015693,2.10851071895189,
5.73560534432582));
#123720=CARTESIAN_POINT('Ctrl Pts',(-4.82263693273945,2.10627260247597,
5.744575165774));
#123721=CARTESIAN_POINT('Ctrl Pts',(-4.81191182532195,2.104034486,5.75354498722217));
#123722=CARTESIAN_POINT('Ctrl Pts',(-4.49954550307968,2.038849851,6.01478900351599));
#123723=CARTESIAN_POINT('Ctrl Pts',(-4.16073209479057,1.973541827,6.24067975220858));
#123724=CARTESIAN_POINT('Ctrl Pts',(-4.85158160963388,2.10851071895189,
5.38752136625703));
#123725=CARTESIAN_POINT('Ctrl Pts',(-4.84150522531699,2.10627260247597,
5.39652756912856));
#123726=CARTESIAN_POINT('Ctrl Pts',(-4.83142884100001,2.104034486,5.405533772));
#123727=CARTESIAN_POINT('Ctrl Pts',(-4.537956432,2.038849851,5.667837389));
#123728=CARTESIAN_POINT('Ctrl Pts',(-4.217811169,1.973541827,5.896827024));
#123729=CARTESIAN_POINT('',(-4.22162532483266,1.9743200846106,5.89409701316203));
#123730=CARTESIAN_POINT('Origin',(0.122032535617409,2.01785676375151,-0.157976378280066));
#123731=CARTESIAN_POINT('Ctrl Pts',(-4.36672690769356,2.01370168112843,
6.09767956762301));
#123732=CARTESIAN_POINT('Ctrl Pts',(-4.34254950320055,2.00745398476853,
6.06369438560014));
#123733=CARTESIAN_POINT('Ctrl Pts',(-4.31835750742411,2.00105345714589,
6.02971856953371));
#123734=CARTESIAN_POINT('Ctrl Pts',(-4.26999927977852,1.98793719394933,
5.96186832408102));
#123735=CARTESIAN_POINT('Ctrl Pts',(-4.24580513408982,1.98121389347898,
5.92795472514188));
#123736=CARTESIAN_POINT('Ctrl Pts',(-4.22162532432222,1.97432008483649,
5.8940970152098));
#123737=CARTESIAN_POINT('Ctrl Pts',(-4.568711876,1.973534152,5.94784598));
#123738=CARTESIAN_POINT('Ctrl Pts',(-4.242777527,2.039276147,6.198205544));
#123739=CARTESIAN_POINT('Ctrl Pts',(-3.891438196,2.104034486,6.411451378));
#123740=CARTESIAN_POINT('Ctrl Pts',(-4.225485793,1.973534152,5.891330055));
#123741=CARTESIAN_POINT('Ctrl Pts',(-3.902648444,2.039276147,6.122881269));
#123742=CARTESIAN_POINT('Ctrl Pts',(-3.556442745,2.104034486,6.317769781));
#123743=CARTESIAN_POINT('Origin',(0.126048906359134,1.87507854154913,-0.147660019429458));
#123744=CARTESIAN_POINT('Ctrl Pts',(-3.48737511637751,2.10851071898316,
6.64054004366626));
#123745=CARTESIAN_POINT('Ctrl Pts',(-3.4749725094299,2.10627260249161,6.64699457467313));
#123746=CARTESIAN_POINT('Ctrl Pts',(-3.46256990248223,2.104034486,6.65344910567988));
#123747=CARTESIAN_POINT('Ctrl Pts',(-3.10134678922284,2.038849851,6.84143585675025));
#123748=CARTESIAN_POINT('Ctrl Pts',(-2.72189481628282,1.973541827,6.98921053722634));
#123749=CARTESIAN_POINT('Ctrl Pts',(-3.57999648804651,2.10851071898316,
6.30451074476264));
#123750=CARTESIAN_POINT('Ctrl Pts',(-3.56821961652325,2.10627260249161,
6.31114026288136));
#123751=CARTESIAN_POINT('Ctrl Pts',(-3.556442745,2.104034486,6.317769781));
#123752=CARTESIAN_POINT('Ctrl Pts',(-3.213444034,2.038849851,6.510852992));
#123753=CARTESIAN_POINT('Ctrl Pts',(-2.851557586,1.973541827,6.665667208));
#123754=CARTESIAN_POINT('',(-2.85586944075241,1.97432008458678,6.66382095471484));
#123755=CARTESIAN_POINT('Origin',(0.0852192425560599,2.01785676144799,-0.180516398354523));
#123756=CARTESIAN_POINT('Ctrl Pts',(-2.95381439782471,2.01370168116074,
6.89383641350064));
#123757=CARTESIAN_POINT('Ctrl Pts',(-2.93750805711261,2.00745398478963,
6.8554483588014));
#123758=CARTESIAN_POINT('Ctrl Pts',(-2.92118545276571,2.00105345712332,
6.81706631419646));
#123759=CARTESIAN_POINT('Ctrl Pts',(-2.8885436106362,1.98793719391023,6.74040678021258));
#123760=CARTESIAN_POINT('Ctrl Pts',(-2.87220553189679,1.98121389345132,
6.70208503629584));
#123761=CARTESIAN_POINT('Ctrl Pts',(-2.85586943938469,1.97432008482102,
6.66382095653845));
#123762=CARTESIAN_POINT('Ctrl Pts',(-3.183286862,1.973534152,6.790926649));
#123763=CARTESIAN_POINT('Ctrl Pts',(-2.811152772,2.039276147,6.965366696));
#123764=CARTESIAN_POINT('Ctrl Pts',(-2.422186008,2.104034486,7.098099389));
#123765=CARTESIAN_POINT('Ctrl Pts',(-2.860234467,1.973534152,6.661948573));
#123766=CARTESIAN_POINT('Ctrl Pts',(-2.495168211,2.039276147,6.818685762));
#123767=CARTESIAN_POINT('Ctrl Pts',(-2.115161339,2.104034486,6.93459389700001));
#123768=CARTESIAN_POINT('Origin',(0.0913593601730348,1.87507851176375,-0.171304427570849));
#123769=CARTESIAN_POINT('Ctrl Pts',(-1.97832240692608,2.10851071887184,
7.23497047157778));
#123770=CARTESIAN_POINT('Ctrl Pts',(-1.96482223300216,2.10627260243589,
7.23860790526074));
#123771=CARTESIAN_POINT('Ctrl Pts',(-1.95132205907823,2.104034486,7.24224533894379));
#123772=CARTESIAN_POINT('Ctrl Pts',(-1.55813254688159,2.038849851,7.34818477228274));
#123773=CARTESIAN_POINT('Ctrl Pts',(-1.15578476260228,1.973541827,7.41093360613812));
#123774=CARTESIAN_POINT('Ctrl Pts',(-2.14101470886305,2.10851071887184,
6.92670820836453));
#123775=CARTESIAN_POINT('Ctrl Pts',(-2.12808802393157,2.10627260243589,
6.93065105268227));
#123776=CARTESIAN_POINT('Ctrl Pts',(-2.115161339,2.104034486,6.93459389700001));
#123777=CARTESIAN_POINT('Ctrl Pts',(-1.738674564,2.038849851,7.049428346));
#123778=CARTESIAN_POINT('Ctrl Pts',(-1.35196834,1.973541827,7.122828203));
#123779=CARTESIAN_POINT('',(-1.35657627667434,1.97432008457408,7.12195203495116));
#123780=CARTESIAN_POINT('Origin',(0.0444211629499514,2.01785670642679,-0.194615624344407));
#123781=CARTESIAN_POINT('Ctrl Pts',(-1.40278481009805,2.01370168113039,
7.36764513055357));
#123782=CARTESIAN_POINT('Ctrl Pts',(-1.39511199963778,2.00745398477036,
7.32664918607161));
#123783=CARTESIAN_POINT('Ctrl Pts',(-1.38742201379162,2.0010534571221,7.28565561499032));
#123784=CARTESIAN_POINT('Ctrl Pts',(-1.37202285368925,1.98793719394712,
7.20377130722825));
#123785=CARTESIAN_POINT('Ctrl Pts',(-1.36430479237323,1.98121389349783,
7.16283330034612));
#123786=CARTESIAN_POINT('Ctrl Pts',(-1.35657627478824,1.97432008488557,
7.12195203641865));
#123787=CARTESIAN_POINT('Ctrl Pts',(-1.649014893,1.973534152,7.31647113600001));
#123788=CARTESIAN_POINT('Ctrl Pts',(-1.248081637,2.039276147,7.406835042));
#123789=CARTESIAN_POINT('Ctrl Pts',(-0.839675095000001,2.104034486,7.452848163));
#123790=CARTESIAN_POINT('Ctrl Pts',(-1.361241758,1.973534152,7.12106178));
#123791=CARTESIAN_POINT('Ctrl Pts',(-0.971016684,2.039276147,7.195656087));
#123792=CARTESIAN_POINT('Ctrl Pts',(-0.574977339,2.104034486,7.227164109));
#123793=CARTESIAN_POINT('Origin',(0.05239802991064,1.87507856101189,-0.186939026512341));
#123794=CARTESIAN_POINT('Ctrl Pts',(-0.376765541919947,2.10851071897258,
7.49110172164174));
#123795=CARTESIAN_POINT('Ctrl Pts',(-0.362799053543135,2.10627260248626,
7.4917519758376));
#123796=CARTESIAN_POINT('Ctrl Pts',(-0.348832565166325,2.104034486,7.49240223003331));
#123797=CARTESIAN_POINT('Ctrl Pts',(0.0579382408491217,2.038849851,7.51134073598938));
#123798=CARTESIAN_POINT('Ctrl Pts',(0.464368502441386,1.973541827,7.48612965584813));
#123799=CARTESIAN_POINT('Ctrl Pts',(-0.601921461974099,2.10851071897258,
7.22502049361022));
#123800=CARTESIAN_POINT('Ctrl Pts',(-0.588449400487053,2.10627260248626,
7.22609230130511));
#123801=CARTESIAN_POINT('Ctrl Pts',(-0.574977339,2.104034486,7.227164109));
#123802=CARTESIAN_POINT('Ctrl Pts',(-0.182606604,2.038849851,7.258380265));
#123803=CARTESIAN_POINT('Ctrl Pts',(0.210837442,1.973541827,7.246933667));
#123804=CARTESIAN_POINT('Origin',(0.00154614941171419,2.01785680179854,
-0.199616151906485));
#123805=CARTESIAN_POINT('Ctrl Pts',(-1.35704670638058,3.78339966801642,
7.12186672777107));
#123806=CARTESIAN_POINT('Ctrl Pts',(-1.35319549019029,3.78403814050821,
7.12259624888554));
#123807=CARTESIAN_POINT('Ctrl Pts',(-1.349344274,3.784676613,7.12332577));
#123808=CARTESIAN_POINT('Ctrl Pts',(-0.962175844,3.848863192,7.196665601));
#123809=CARTESIAN_POINT('Ctrl Pts',(-0.569339312,3.914045302,7.227610445));
#123810=CARTESIAN_POINT('Ctrl Pts',(-1.16146771926858,3.78339966801642,
7.40952484987452));
#123811=CARTESIAN_POINT('Ctrl Pts',(-1.15746109563429,3.78403814050821,
7.41014846343727));
#123812=CARTESIAN_POINT('Ctrl Pts',(-1.153454472,3.784676613,7.410772077));
#123813=CARTESIAN_POINT('Ctrl Pts',(-0.750662703,3.848863192,7.473464866));
#123814=CARTESIAN_POINT('Ctrl Pts',(-0.343448839,3.914045302,7.492132066));
#123815=CARTESIAN_POINT('',(-0.574036075380877,3.91326598488409,7.2272389368462));
#123816=CARTESIAN_POINT('Ctrl Pts',(-0.574036076308431,3.91326598386019,
7.22723893873903));
#123817=CARTESIAN_POINT('Ctrl Pts',(-0.576049247025033,3.90857186132774,
7.2558036048112));
#123818=CARTESIAN_POINT('Ctrl Pts',(-0.57805430305433,3.90396299771727,
7.28438297799801));
#123819=CARTESIAN_POINT('Ctrl Pts',(-0.580051625069697,3.89943471856325,
7.31297553246098));
#123820=CARTESIAN_POINT('Ctrl Pts',(-0.581955575986403,3.89511812805851,
7.34023143804963));
#123821=CARTESIAN_POINT('Ctrl Pts',(-0.583844230084641,3.89087604513709,
7.36750030135324));
#123822=CARTESIAN_POINT('Ctrl Pts',(-0.585765722797521,3.88669712984843,
7.39477643667835));
#123823=CARTESIAN_POINT('Ctrl Pts',(-0.587687262853223,3.88251811159729,
7.42205324404827));
#123824=CARTESIAN_POINT('Ctrl Pts',(-0.589633671771024,3.87840354548757,
7.44933825566685));
#123825=CARTESIAN_POINT('Ctrl Pts',(-0.59160338941931,3.87435041354706,
7.47663061988905));
#123826=CARTESIAN_POINT('Origin',(-0.00201954687480965,4.01777100458333,
-0.19381601599339));
#123827=CARTESIAN_POINT('Ctrl Pts',(-2.118772315,3.914032935,6.933491464));
#123828=CARTESIAN_POINT('Ctrl Pts',(-2.056341304,3.90342418,6.952569456));
#123829=CARTESIAN_POINT('Ctrl Pts',(-1.993576877,3.892857143,6.970520155));
#123830=CARTESIAN_POINT('Ctrl Pts',(-1.674952964,3.839213527,7.061646965));
#123831=CARTESIAN_POINT('Ctrl Pts',(-1.349344274,3.784676613,7.12332577));
#123832=CARTESIAN_POINT('Ctrl Pts',(-1.34543222082607,3.78402137462933,
7.12406681522476));
#123833=CARTESIAN_POINT('Ctrl Pts',(-1.34152016765215,3.78336613625867,
7.12480786044952));
#123834=CARTESIAN_POINT('Ctrl Pts',(-2.42588209,3.914032935,7.096837048));
#123835=CARTESIAN_POINT('Ctrl Pts',(-2.361980272,3.90342418,7.118680339));
#123836=CARTESIAN_POINT('Ctrl Pts',(-2.297695481,3.892857143,7.139369403));
#123837=CARTESIAN_POINT('Ctrl Pts',(-1.971353434,3.839213527,7.244397537));
#123838=CARTESIAN_POINT('Ctrl Pts',(-1.636790581,3.784676613,7.319215572));
#123839=CARTESIAN_POINT('Ctrl Pts',(-1.6327709472766,3.78402137462933,7.32011447961603));
#123840=CARTESIAN_POINT('Ctrl Pts',(-1.6287513135532,3.78336613625867,7.32101338723207));
#123841=CARTESIAN_POINT('',(-2.11425816854035,3.91326598495297,6.93486931335475));
#123842=CARTESIAN_POINT('Ctrl Pts',(-2.1142581686341,3.91326598528019,6.93486931384458));
#123843=CARTESIAN_POINT('Ctrl Pts',(-2.07409799250755,3.90644394825061,
6.9471130886998));
#123844=CARTESIAN_POINT('Ctrl Pts',(-2.03386770757442,3.89964051877146,
6.95899693099171));
#123845=CARTESIAN_POINT('Ctrl Pts',(-1.99357687675307,3.89285714287914,
6.97052015546677));
#123846=CARTESIAN_POINT('Ctrl Pts',(-1.85161574205348,3.86895652430184,
7.01112120550672));
#123847=CARTESIAN_POINT('Ctrl Pts',(-1.7079233848003,3.84480664668525,7.04752157904651));
#123848=CARTESIAN_POINT('Ctrl Pts',(-1.56288052588263,3.82047224755234,
7.07954126122991));
#123849=CARTESIAN_POINT('Ctrl Pts',(-1.49200829878732,3.80858174101899,
7.09518702417306));
#123850=CARTESIAN_POINT('Ctrl Pts',(-1.42081403974305,3.79664724067556,
7.109787527585));
#123851=CARTESIAN_POINT('Ctrl Pts',(-1.34934427548489,3.78467661296572,
7.12332577119014));
#123852=CARTESIAN_POINT('Ctrl Pts',(-2.18502660812532,3.87435041326576,
7.17465390925577));
#123853=CARTESIAN_POINT('Ctrl Pts',(-2.17685404271359,3.87860220111518,
7.14713740763035));
#123854=CARTESIAN_POINT('Ctrl Pts',(-2.1687082656535,3.88292159126619,7.11962328841485));
#123855=CARTESIAN_POINT('Ctrl Pts',(-2.16059124855501,3.8873120745959,7.0921121225464));
#123856=CARTESIAN_POINT('Ctrl Pts',(-2.15285368017845,3.89149731463637,
7.06588702970225));
#123857=CARTESIAN_POINT('Ctrl Pts',(-2.14514798794445,3.8957461849516,7.03966258355752));
#123858=CARTESIAN_POINT('Ctrl Pts',(-2.13742892265818,3.90006996195599,
7.01345452121582));
#123859=CARTESIAN_POINT('Ctrl Pts',(-2.12970964348895,3.90439385876533,
6.98724573269059));
#123860=CARTESIAN_POINT('Ctrl Pts',(-2.12198607104547,3.90879118062969,
6.96105020924954));
#123861=CARTESIAN_POINT('Ctrl Pts',(-2.1142581719554,3.91326598407097,6.93486931282839));
#123862=CARTESIAN_POINT('Ctrl Pts',(-2.85631053383156,3.78339966801642,
6.66363651409478));
#123863=CARTESIAN_POINT('Ctrl Pts',(-2.85270618241578,3.78403814050821,
6.66517687704739));
#123864=CARTESIAN_POINT('Ctrl Pts',(-2.849101831,3.784676613,6.66671724));
#123865=CARTESIAN_POINT('Ctrl Pts',(-2.48675108,3.848863192,6.82157219400001));
#123866=CARTESIAN_POINT('Ctrl Pts',(-2.109751075,3.914045302,6.936241807));
#123867=CARTESIAN_POINT('Ctrl Pts',(-2.72714206803972,3.78339966801642,
6.98661305006529));
#123868=CARTESIAN_POINT('Ctrl Pts',(-2.72336317551986,3.78403814050821,
6.98808338953264));
#123869=CARTESIAN_POINT('Ctrl Pts',(-2.719584283,3.784676613,6.989553729));
#123870=CARTESIAN_POINT('Ctrl Pts',(-2.339686658,3.848863192,7.137369119));
#123871=CARTESIAN_POINT('Ctrl Pts',(-1.946006124,3.914045302,7.243138834));
#123872=CARTESIAN_POINT('Origin',(0.0396917695066523,4.01777116282268,-0.189717473787636));
#123873=CARTESIAN_POINT('Ctrl Pts',(-3.559732308,3.914032935,6.315916869));
#123874=CARTESIAN_POINT('Ctrl Pts',(-3.502862104,3.90342418,6.347969651));
#123875=CARTESIAN_POINT('Ctrl Pts',(-3.445423944,3.892857143,6.378993169));
#123876=CARTESIAN_POINT('Ctrl Pts',(-3.153838851,3.839213527,6.536484208));
#123877=CARTESIAN_POINT('Ctrl Pts',(-2.849101831,3.784676613,6.66671724));
#123878=CARTESIAN_POINT('Ctrl Pts',(-2.84544054227241,3.78402137462933,
6.66828193578925));
#123879=CARTESIAN_POINT('Ctrl Pts',(-2.84177925354481,3.78336613625867,
6.66984663157849));
#123880=CARTESIAN_POINT('Ctrl Pts',(-3.894776499,3.914032935,6.409424001));
#123881=CARTESIAN_POINT('Ctrl Pts',(-3.837064332,3.90342418,6.44449361));
#123882=CARTESIAN_POINT('Ctrl Pts',(-3.778730021,3.892857143,6.478518305));
#123883=CARTESIAN_POINT('Ctrl Pts',(-3.482595614,3.839213527,6.651244833));
#123884=CARTESIAN_POINT('Ctrl Pts',(-3.17193832,3.784676613,6.796234788));
#123885=CARTESIAN_POINT('Ctrl Pts',(-3.16820590163919,3.78402137462933,
6.79797678209003));
#123886=CARTESIAN_POINT('Ctrl Pts',(-3.16447348327838,3.78336613625867,
6.79971877618007));
#123887=CARTESIAN_POINT('',(-3.55561989781354,3.9132659848605,6.31823291263059));
#123888=CARTESIAN_POINT('Ctrl Pts',(-3.55561990133067,3.9132659850464,6.31823290990407));
#123889=CARTESIAN_POINT('Ctrl Pts',(-3.500785581,3.903042157,6.349091223));
#123890=CARTESIAN_POINT('Ctrl Pts',(-3.445423944,3.892857143,6.378993169));
#123891=CARTESIAN_POINT('Ctrl Pts',(-3.153838851037,3.83921352752391,6.5364842076699));
#123892=CARTESIAN_POINT('Ctrl Pts',(-2.84910183343416,3.7846766127594,6.66671724052467));
#123893=CARTESIAN_POINT('Ctrl Pts',(-3.67628040946578,3.87435041322476,
6.53719835604485));
#123894=CARTESIAN_POINT('Ctrl Pts',(-3.66238367936974,3.87860220111933,
6.51208203505423));
#123895=CARTESIAN_POINT('Ctrl Pts',(-3.64851362369141,3.88292159127308,
6.48696228194705));
#123896=CARTESIAN_POINT('Ctrl Pts',(-3.63467229045904,3.8873120746017,6.46183923059982));
#123897=CARTESIAN_POINT('Ctrl Pts',(-3.62147800234562,3.89149731463765,
6.43789061436477));
#123898=CARTESIAN_POINT('Ctrl Pts',(-3.60831498411576,3.89574618495018,
6.41393577729978));
#123899=CARTESIAN_POINT('Ctrl Pts',(-3.59514242756216,3.90006996193851,
6.38999981577969));
#123900=CARTESIAN_POINT('Ctrl Pts',(-3.58196950601821,3.90439385873175,
6.3660631910326));
#123901=CARTESIAN_POINT('Ctrl Pts',(-3.56879524322248,3.90879118056604,
6.34214044413692));
#123902=CARTESIAN_POINT('Ctrl Pts',(-3.55561990060165,3.91326598374165,
6.31823291137695));
#123903=CARTESIAN_POINT('Ctrl Pts',(-4.22201645637774,3.78339966801642,
5.893822062747));
#123904=CARTESIAN_POINT('Ctrl Pts',(-4.21882750518887,3.78403814050821,
5.8961012418735));
#123905=CARTESIAN_POINT('Ctrl Pts',(-4.215638554,3.784676613,5.898380421));
#123906=CARTESIAN_POINT('Ctrl Pts',(-3.895048599,3.848863192,6.127509652));
#123907=CARTESIAN_POINT('Ctrl Pts',(-3.551513221,3.914045302,6.320542211));
#123908=CARTESIAN_POINT('Ctrl Pts',(-4.16529828519659,3.78339966801642,
6.23701498812772));
#123909=CARTESIAN_POINT('Ctrl Pts',(-4.16192382059829,3.78403814050821,
6.23926330206386));
#123910=CARTESIAN_POINT('Ctrl Pts',(-4.158549356,3.784676613,6.241511616));
#123911=CARTESIAN_POINT('Ctrl Pts',(-3.819309465,3.848863192,6.467537924));
#123912=CARTESIAN_POINT('Ctrl Pts',(-3.457570326,3.914045302,6.65546448));
#123913=CARTESIAN_POINT('Origin',(0.0795475392719219,4.01777120008797,-0.176749585716738));
#123914=CARTESIAN_POINT('Ctrl Pts',(-4.834243174,3.914032935,5.403017021));
#123915=CARTESIAN_POINT('Ctrl Pts',(-4.785592964,3.90342418,5.446545839));
#123916=CARTESIAN_POINT('Ctrl Pts',(-4.736166816,3.892857143,5.489191552));
#123917=CARTESIAN_POINT('Ctrl Pts',(-4.485254739,3.839213527,5.705682713));
#123918=CARTESIAN_POINT('Ctrl Pts',(-4.215638554,3.784676613,5.898380421));
#123919=CARTESIAN_POINT('Ctrl Pts',(-4.21239922751805,3.78402137462933,
5.90069560392768));
#123920=CARTESIAN_POINT('Ctrl Pts',(-4.20915990103609,3.78336613625867,
5.90301078685534));
#123921=CARTESIAN_POINT('Ctrl Pts',(-5.181555488,3.914032935,5.422313411));
#123922=CARTESIAN_POINT('Ctrl Pts',(-5.13273152800001,3.90342418,5.468969522));
#123923=CARTESIAN_POINT('Ctrl Pts',(-5.083075345,3.892857143,5.514738891));
#123924=CARTESIAN_POINT('Ctrl Pts',(-4.830995493,3.839213527,5.747087313));
#123925=CARTESIAN_POINT('Ctrl Pts',(-4.558769749,3.784676613,5.955469618));
#123926=CARTESIAN_POINT('Ctrl Pts',(-4.5554990697505,3.78402137462933,5.95797324484628));
#123927=CARTESIAN_POINT('Ctrl Pts',(-4.552228390501,3.78336613625867,5.96047687169255));
#123928=CARTESIAN_POINT('',(-4.83072479043724,3.91326598487081,5.40616296424982));
#123929=CARTESIAN_POINT('Ctrl Pts',(-4.83072479322977,3.9132659850464,5.40616296074057));
#123930=CARTESIAN_POINT('Ctrl Pts',(-4.783806095,3.903042157,5.448087581));
#123931=CARTESIAN_POINT('Ctrl Pts',(-4.736166816,3.892857143,5.489191552));
#123932=CARTESIAN_POINT('Ctrl Pts',(-4.48525473952604,3.83921352756829,
5.70568271291834));
#123933=CARTESIAN_POINT('Ctrl Pts',(-4.21563855621441,3.78467661274867,
5.89838042096646));
#123934=CARTESIAN_POINT('Ctrl Pts',(-4.99563542474069,3.87435041323828,
5.59407067341434));
#123935=CARTESIAN_POINT('Ctrl Pts',(-4.97666432598813,3.87860220109873,
5.57252894419364));
#123936=CARTESIAN_POINT('Ctrl Pts',(-4.95771854011772,3.88292159124263,
5.55097812899301));
#123937=CARTESIAN_POINT('Ctrl Pts',(-4.93880009614804,3.88731207456726,
5.52941791819073));
#123938=CARTESIAN_POINT('Ctrl Pts',(-4.92076603853602,3.89149731460856,
5.50886558923815));
#123939=CARTESIAN_POINT('Ctrl Pts',(-4.90276118250714,3.89574618491636,
5.48830046273151));
#123940=CARTESIAN_POINT('Ctrl Pts',(-4.88475106888788,3.90006996189442,
5.46775582088404));
#123941=CARTESIAN_POINT('Ctrl Pts',(-4.86674045623729,3.90439385867739,
5.44721060977753));
#123942=CARTESIAN_POINT('Ctrl Pts',(-4.84873151701053,3.90879118050781,
5.42667924040515));
#123943=CARTESIAN_POINT('Ctrl Pts',(-4.83072479286557,3.91326598389372,
5.4061629624153));
#123944=CARTESIAN_POINT('Ctrl Pts',(-5.39030558027708,3.78339966801642,
4.84841904112145));
#123945=CARTESIAN_POINT('Ctrl Pts',(-5.38768114113854,3.78403814050821,
4.85133046456072));
#123946=CARTESIAN_POINT('Ctrl Pts',(-5.385056702,3.784676613,4.854241888));
#123947=CARTESIAN_POINT('Ctrl Pts',(-5.121217974,3.848863192,5.14693157));
#123948=CARTESIAN_POINT('Ctrl Pts',(-4.827210557,3.914045302,5.409301086));
#123949=CARTESIAN_POINT('Ctrl Pts',(-5.40868978391049,3.78339966801642,
5.19578103749289));
#123950=CARTESIAN_POINT('Ctrl Pts',(-5.40587753345524,3.78403814050821,
5.19870219724644));
#123951=CARTESIAN_POINT('Ctrl Pts',(-5.40306528300001,3.784676613,5.201623357));
#123952=CARTESIAN_POINT('Ctrl Pts',(-5.120345607,3.848863192,5.495291845));
#123953=CARTESIAN_POINT('Ctrl Pts',(-4.807462382,3.914045302,5.756588004));
#123954=CARTESIAN_POINT('Origin',(0.115683568884218,4.01777114530414,-0.155516752860486));
#123955=CARTESIAN_POINT('Ctrl Pts',(-5.88271020300001,3.914032935,4.237478103));
#123956=CARTESIAN_POINT('Ctrl Pts',(-5.844554817,3.90342418,4.290447598));
#123957=CARTESIAN_POINT('Ctrl Pts',(-5.805451792,3.892857143,4.342721438));
#123958=CARTESIAN_POINT('Ctrl Pts',(-5.6069451,3.839213527,4.608089836));
#123959=CARTESIAN_POINT('Ctrl Pts',(-5.385056702,3.784676613,4.854241888));
#123960=CARTESIAN_POINT('Ctrl Pts',(-5.38239080505588,3.78402137462933,
4.85719930266942));
#123961=CARTESIAN_POINT('Ctrl Pts',(-5.37972490811174,3.78336613625867,
4.86015671733883));
#123962=CARTESIAN_POINT('Ctrl Pts',(-6.22605070100001,3.914032935,4.181661472));
#123963=CARTESIAN_POINT('Ctrl Pts',(-6.188397903,3.90342418,4.237722498));
#123964=CARTESIAN_POINT('Ctrl Pts',(-6.149741715,3.892857143,4.293096416));
#123965=CARTESIAN_POINT('Ctrl Pts',(-5.953503393,3.839213527,4.574202378));
#123966=CARTESIAN_POINT('Ctrl Pts',(-5.732438171,3.784676613,4.836233308));
#123967=CARTESIAN_POINT('Ctrl Pts',(-5.72978216417362,3.78402137462933,
4.83938150079354));
#123968=CARTESIAN_POINT('Ctrl Pts',(-5.72712615734723,3.78336613625867,
4.84252969358708));
#123969=CARTESIAN_POINT('',(-5.87995036158964,3.91326598496052,4.24130684423531));
#123970=CARTESIAN_POINT('Ctrl Pts',(-5.87995036176124,3.91326598532877,
4.24130684443286));
#123971=CARTESIAN_POINT('Ctrl Pts',(-5.85538874095779,3.90644394830579,
4.27535793159474));
#123972=CARTESIAN_POINT('Ctrl Pts',(-5.8305534848299,3.89964051880999,4.30916490723401));
#123973=CARTESIAN_POINT('Ctrl Pts',(-5.80545179213163,3.89285714291852,
4.34272143834066));
#123974=CARTESIAN_POINT('Ctrl Pts',(-5.71700827329339,3.86895653713759,
4.46095480768064));
#123975=CARTESIAN_POINT('Ctrl Pts',(-5.62464440301594,3.84480667252569,
4.57689174154322));
#123976=CARTESIAN_POINT('Ctrl Pts',(-5.52855433006173,3.82047228658325,
4.69015852906592));
#123977=CARTESIAN_POINT('Ctrl Pts',(-5.48160180434346,3.80858176712922,
4.74550411878901));
#123978=CARTESIAN_POINT('Ctrl Pts',(-5.43376034511521,3.79664725376609,
4.80021246869245));
#123979=CARTESIAN_POINT('Ctrl Pts',(-5.38505670397552,3.78467661297329,
4.85424188801248));
#123980=CARTESIAN_POINT('Ctrl Pts',(-6.08140007972271,3.87435041321968,
4.38937046350253));
#123981=CARTESIAN_POINT('Ctrl Pts',(-6.05824167964873,3.87860220110466,
4.37241059342075));
#123982=CARTESIAN_POINT('Ctrl Pts',(-6.03510604752354,3.88292159125114,
4.35543640811372));
#123983=CARTESIAN_POINT('Ctrl Pts',(-6.01199509829652,3.88731207457891,
4.33844716915637));
#123984=CARTESIAN_POINT('Ctrl Pts',(-5.98996452384717,3.89149731460825,
4.32225213147051));
#123985=CARTESIAN_POINT('Ctrl Pts',(-5.96795971712769,3.89574618491864,
4.30603831801684));
#123986=CARTESIAN_POINT('Ctrl Pts',(-5.94595417929557,3.90006996191496,
4.2898456405848));
#123987=CARTESIAN_POINT('Ctrl Pts',(-5.92394803172508,3.90439385871625,
4.27365251447949));
#123988=CARTESIAN_POINT('Ctrl Pts',(-5.90194649400798,3.90879118057332,
4.25747254677785));
#123989=CARTESIAN_POINT('Ctrl Pts',(-5.87995036393221,3.91326598396042,
4.24130684150133));
#123990=CARTESIAN_POINT('Ctrl Pts',(-6.30655000747555,3.78339966801642,
3.57630933537954));
#123991=CARTESIAN_POINT('Ctrl Pts',(-6.30461279623777,3.78403814050821,
3.57971686818977));
#123992=CARTESIAN_POINT('Ctrl Pts',(-6.302675585,3.784676613,3.583124401));
#123993=CARTESIAN_POINT('Ctrl Pts',(-6.107924889,3.848863192,3.925688688));
#123994=CARTESIAN_POINT('Ctrl Pts',(-5.87719289300001,3.914045302,4.245127054));
#123995=CARTESIAN_POINT('Ctrl Pts',(-6.39917695920962,3.78339966801642,
3.91159814126253));
#123996=CARTESIAN_POINT('Ctrl Pts',(-6.39705842060482,3.78403814050821,
3.91505555663127));
#123997=CARTESIAN_POINT('Ctrl Pts',(-6.394939882,3.784676613,3.918512972));
#123998=CARTESIAN_POINT('Ctrl Pts',(-6.181960079,3.848863192,4.266092026));
#123999=CARTESIAN_POINT('Ctrl Pts',(-5.93256284,3.914045302,4.588539871));
#124000=CARTESIAN_POINT('Origin',(0.146410461703627,4.01777117749663,-0.127012326547644));
#124001=CARTESIAN_POINT('Ctrl Pts',(-6.65610824,3.914032935,2.873799418));
#124002=CARTESIAN_POINT('Ctrl Pts',(-6.630231782,3.90342418,2.933732796));
#124003=CARTESIAN_POINT('Ctrl Pts',(-6.603280295,3.892857143,2.993190497));
#124004=CARTESIAN_POINT('Ctrl Pts',(-6.46646094,3.839213527,3.2950278));
#124005=CARTESIAN_POINT('Ctrl Pts',(-6.30267558499999,3.784676613,3.583124401));
#124006=CARTESIAN_POINT('Ctrl Pts',(-6.30070777198533,3.78402137462933,
3.58658576200464));
#124007=CARTESIAN_POINT('Ctrl Pts',(-6.29873995897067,3.78336613625867,
3.59004712300929));
#124008=CARTESIAN_POINT('Ctrl Pts',(-6.979422703,3.914032935,2.745479691));
#124009=CARTESIAN_POINT('Ctrl Pts',(-6.95470167,3.90342418,2.808324279));
#124010=CARTESIAN_POINT('Ctrl Pts',(-6.928852998,3.892857143,2.870713524));
#124011=CARTESIAN_POINT('Ctrl Pts',(-6.797632091,3.839213527,3.187432823));
#124012=CARTESIAN_POINT('Ctrl Pts',(-6.638064156,3.784676613,3.490860104));
#124013=CARTESIAN_POINT('Ctrl Pts',(-6.63614701353499,3.78402137462933,
3.49450565675749));
#124014=CARTESIAN_POINT('Ctrl Pts',(-6.63422987106999,3.78336613625867,
3.49815120951497));
#124015=CARTESIAN_POINT('',(-6.65423598880558,3.91326598476628,2.87813192909408));
#124016=CARTESIAN_POINT('Ctrl Pts',(-6.6542359888712,3.91326598544311,2.8781319292423));
#124017=CARTESIAN_POINT('Ctrl Pts',(-6.63756858305185,3.90644394855885,
2.91666694270274));
#124018=CARTESIAN_POINT('Ctrl Pts',(-6.62058146189084,3.8996405190235,2.95502237632601));
#124019=CARTESIAN_POINT('Ctrl Pts',(-6.60328029523313,3.8928571430914,2.9931904964857));
#124020=CARTESIAN_POINT('Ctrl Pts',(-6.5423212091965,3.86895653485097,3.12767239143726));
#124021=CARTESIAN_POINT('Ctrl Pts',(-6.47703976156619,3.84480666772173,
3.26075429956098));
#124022=CARTESIAN_POINT('Ctrl Pts',(-6.40754522474049,3.82047227927594,
3.39202951081633));
#124023=CARTESIAN_POINT('Ctrl Pts',(-6.37358809548747,3.80858176224409,
3.45617454321643));
#124024=CARTESIAN_POINT('Ctrl Pts',(-6.33862582826106,3.79664725133354,
3.51988832868173));
#124025=CARTESIAN_POINT('Ctrl Pts',(-6.30267558687012,3.78467661302513,
3.58312440037351));
#124026=CARTESIAN_POINT('Ctrl Pts',(-6.88280522651749,3.87435041325227,
2.97942816881733));
#124027=CARTESIAN_POINT('Ctrl Pts',(-6.8565423860806,3.87860220116035,2.96784318262581));
#124028=CARTESIAN_POINT('Ctrl Pts',(-6.83029870404635,3.88292159130352,
2.95623932143671));
#124029=CARTESIAN_POINT('Ctrl Pts',(-6.80407589172509,3.88731207462835,
2.94461545246392));
#124030=CARTESIAN_POINT('Ctrl Pts',(-6.77907892536439,3.89149731466413,
2.933534968108));
#124031=CARTESIAN_POINT('Ctrl Pts',(-6.75410308807489,3.89574618496796,
2.92243060758178));
#124032=CARTESIAN_POINT('Ctrl Pts',(-6.72913108036634,3.90006996195947,
2.91134704614054));
#124033=CARTESIAN_POINT('Ctrl Pts',(-6.70415838072343,3.90439385875593,
2.90026317759156));
#124034=CARTESIAN_POINT('Ctrl Pts',(-6.6791930118057,3.90879118061045,2.88919116886928));
#124035=CARTESIAN_POINT('Ctrl Pts',(-6.65423599044422,3.91326598379351,
2.87813192527154));
#124036=CARTESIAN_POINT('Ctrl Pts',(-6.92790716496715,3.78339966801642,
2.13697537852514));
#124037=CARTESIAN_POINT('Ctrl Pts',(-6.92674776348357,3.78403814050821,
2.14071968826257));
#124038=CARTESIAN_POINT('Ctrl Pts',(-6.92558836200001,3.784676613,2.144463998));
#124039=CARTESIAN_POINT('Ctrl Pts',(-6.809032025,3.848863192,2.520884965));
#124040=CARTESIAN_POINT('Ctrl Pts',(-6.65236422,3.914045302,2.882455599));
#124041=CARTESIAN_POINT('Ctrl Pts',(-7.09044573248517,3.78339966801642,
2.44451326180714));
#124042=CARTESIAN_POINT('Ctrl Pts',(-7.08911996624259,3.78403814050821,
2.44834526790357));
#124043=CARTESIAN_POINT('Ctrl Pts',(-7.0877942,3.784676613,2.452177274));
#124044=CARTESIAN_POINT('Ctrl Pts',(-6.954512969,3.848863192,2.837414485));
#124045=CARTESIAN_POINT('Ctrl Pts',(-6.780263254,3.914045302,3.205936713));
#124046=CARTESIAN_POINT('Origin',(0.170291314417856,4.01777096736017,-0.0925688634418695));
#124047=CARTESIAN_POINT('Ctrl Pts',(-7.118274054,3.914032935,1.375745066));
#124048=CARTESIAN_POINT('Ctrl Pts',(-7.105886478,3.90342418,1.439839908));
#124049=CARTESIAN_POINT('Ctrl Pts',(-7.09234675,3.892857143,1.503701295));
#124050=CARTESIAN_POINT('Ctrl Pts',(-7.02361225300001,3.839213527,1.827893927));
#124051=CARTESIAN_POINT('Ctrl Pts',(-6.925588362,3.784676613,2.144463998));
#124052=CARTESIAN_POINT('Ctrl Pts',(-6.92441064566231,3.78402137462933,
2.14826745592069));
#124053=CARTESIAN_POINT('Ctrl Pts',(-6.92323292932462,3.78336613625867,
2.15207091384138));
#124054=CARTESIAN_POINT('Ctrl Pts',(-7.406444656,3.914032935,1.180922331));
#124055=CARTESIAN_POINT('Ctrl Pts',(-7.395811316,3.90342418,1.247611939));
#124056=CARTESIAN_POINT('Ctrl Pts',(-7.383978815,3.892857143,1.314099258));
#124057=CARTESIAN_POINT('Ctrl Pts',(-7.323911067,3.839213527,1.651622452));
#124058=CARTESIAN_POINT('Ctrl Pts',(-7.233301638,3.784676613,1.982258161));
#124059=CARTESIAN_POINT('Ctrl Pts',(-7.23221300334376,3.78402137462933,
1.98623061171932));
#124060=CARTESIAN_POINT('Ctrl Pts',(-7.23112436868752,3.78336613625867,
1.99020306243863));
#124061=CARTESIAN_POINT('',(-7.11737693701566,3.91326598488478,1.38037876392498));
#124062=CARTESIAN_POINT('Ctrl Pts',(-7.11737693714267,3.9132659850464,1.38037875906925));
#124063=CARTESIAN_POINT('Ctrl Pts',(-7.105396986,3.903042157,1.442148645));
#124064=CARTESIAN_POINT('Ctrl Pts',(-7.09234675,3.892857143,1.503701295));
#124065=CARTESIAN_POINT('Ctrl Pts',(-7.02361225412372,3.83921352757512,
1.82789392608951));
#124066=CARTESIAN_POINT('Ctrl Pts',(-6.92558836366604,3.78467661276937,
2.14446399703795));
#124067=CARTESIAN_POINT('Ctrl Pts',(-7.36237804982059,3.87435041323098,
1.43017112466086));
#124068=CARTESIAN_POINT('Ctrl Pts',(-7.33423879050147,3.87860220114459,
1.42450272340496));
#124069=CARTESIAN_POINT('Ctrl Pts',(-7.30611418400067,3.8829215913066,1.4188117698809));
#124070=CARTESIAN_POINT('Ctrl Pts',(-7.27800565822947,3.88731207464986,
1.41309678996559));
#124071=CARTESIAN_POINT('Ctrl Pts',(-7.2512111305266,3.89149731469153,1.40764897000845));
#124072=CARTESIAN_POINT('Ctrl Pts',(-7.22443210526551,3.89574618499422,
1.40217328992509));
#124073=CARTESIAN_POINT('Ctrl Pts',(-7.19766129125643,3.9000699619737,1.39671709932097));
#124074=CARTESIAN_POINT('Ctrl Pts',(-7.17088973547094,3.90439385875811,
1.39126075753454));
#124075=CARTESIAN_POINT('Ctrl Pts',(-7.14412788854292,3.90879118059815,
1.38581442237808));
#124076=CARTESIAN_POINT('Ctrl Pts',(-7.11737693823209,3.91326598397551,
1.38037876113061));
#124077=CARTESIAN_POINT('Ctrl Pts',(-7.22532308280471,3.78339966801642,
0.597718829193276));
#124078=CARTESIAN_POINT('Ctrl Pts',(-7.22499570340235,3.78403814050821,
0.601624836096638));
#124079=CARTESIAN_POINT('Ctrl Pts',(-7.224668324,3.784676613,0.605530843000001));
#124080=CARTESIAN_POINT('Ctrl Pts',(-7.191756391,3.848863192,0.998207464));
#124081=CARTESIAN_POINT('Ctrl Pts',(-7.116478391,3.914045302,1.385003724));
#124082=CARTESIAN_POINT('Ctrl Pts',(-7.45017314305326,3.78339966801642,
0.863125660047407));
#124083=CARTESIAN_POINT('Ctrl Pts',(-7.44970214052664,3.78403814050821,
0.867153076523704));
#124084=CARTESIAN_POINT('Ctrl Pts',(-7.449231138,3.784676613,0.871180493));
#124085=CARTESIAN_POINT('Ctrl Pts',(-7.401880561,3.848863192,1.276062597));
#124086=CARTESIAN_POINT('Ctrl Pts',(-7.31092609300001,3.914045302,1.673427518));
#124087=CARTESIAN_POINT('Origin',(0.186209394296897,4.01777117271173,-0.0537970715760096));
#124088=CARTESIAN_POINT('Ctrl Pts',(-7.24759728500001,3.914032935,-0.186637596));
#124089=CARTESIAN_POINT('Ctrl Pts',(-7.24927782,3.90342418,-0.121378293));
#124090=CARTESIAN_POINT('Ctrl Pts',(-7.249782953,3.892857143,-0.056099309));
#124091=CARTESIAN_POINT('Ctrl Pts',(-7.25234726400001,3.839213527,0.275289764));
#124092=CARTESIAN_POINT('Ctrl Pts',(-7.224668324,3.784676613,0.605530843));
#124093=CARTESIAN_POINT('Ctrl Pts',(-7.22433577303191,3.78402137462933,
0.609498552403771));
#124094=CARTESIAN_POINT('Ctrl Pts',(-7.22400322206382,3.78336613625867,
0.613466261807543));
#124095=CARTESIAN_POINT('Ctrl Pts',(-7.487149489,3.914032935,-0.438853645));
#124096=CARTESIAN_POINT('Ctrl Pts',(-7.491101045,3.90342418,-0.37143735));
#124097=CARTESIAN_POINT('Ctrl Pts',(-7.49383799,3.892857143,-0.303960829));
#124098=CARTESIAN_POINT('Ctrl Pts',(-7.507732102,3.839213527,0.038584051));
#124099=CARTESIAN_POINT('Ctrl Pts',(-7.490317975,3.784676613,0.380968029));
#124100=CARTESIAN_POINT('Ctrl Pts',(-7.49010875149677,3.78402137462933,
0.385081630291895));
#124101=CARTESIAN_POINT('Ctrl Pts',(-7.48989952799356,3.78336613625867,
0.389195231583791));
#124102=CARTESIAN_POINT('',(-7.24771724987847,3.91326598491533,-0.181919377610948));
#124103=CARTESIAN_POINT('Ctrl Pts',(-7.24771724884897,3.9132659850464,-0.181919382176649));
#124104=CARTESIAN_POINT('Ctrl Pts',(-7.249296082,3.903042157,-0.119018306));
#124105=CARTESIAN_POINT('Ctrl Pts',(-7.249782953,3.892857143,-0.056099309));
#124106=CARTESIAN_POINT('Ctrl Pts',(-7.25234726369774,3.83921352753372,
0.275289763730124));
#124107=CARTESIAN_POINT('Ctrl Pts',(-7.22466832546219,3.78467661278774,
0.605530841650099));
#124108=CARTESIAN_POINT('Ctrl Pts',(-7.49769425876845,3.8743504132083,-0.185959131938337));
#124109=CARTESIAN_POINT('Ctrl Pts',(-7.46899434101961,3.87860220112769,
-0.185445900076303));
#124110=CARTESIAN_POINT('Ctrl Pts',(-7.44030388546657,3.88292159126831,
-0.184957843287825));
#124111=CARTESIAN_POINT('Ctrl Pts',(-7.41162396971045,3.88731207458993,
-0.18449670805495));
#124112=CARTESIAN_POINT('Ctrl Pts',(-7.38428476285018,3.89149731462924,
-0.184057129653488));
#124113=CARTESIAN_POINT('Ctrl Pts',(-7.3569547068799,3.89574618493294,-0.183648092579244));
#124114=CARTESIAN_POINT('Ctrl Pts',(-7.32963685985538,3.90006996193835,
-0.183221786705205));
#124115=CARTESIAN_POINT('Ctrl Pts',(-7.3023182558969,3.90439385874872,-0.182795469018913));
#124116=CARTESIAN_POINT('Ctrl Pts',(-7.27501128494097,3.90879118062685,
-0.182361465698886));
#124117=CARTESIAN_POINT('Ctrl Pts',(-7.24771725040738,3.913265984062,-0.181919380376777));
#124118=CARTESIAN_POINT('Ctrl Pts',(-7.18489092487628,3.78339966801642,
-0.969486389062758));
#124119=CARTESIAN_POINT('Ctrl Pts',(-7.18541087543814,3.78403814050821,
-0.965601325531379));
#124120=CARTESIAN_POINT('Ctrl Pts',(-7.18593082600001,3.784676613,-0.961716262));
#124121=CARTESIAN_POINT('Ctrl Pts',(-7.23820222100001,3.848863192,-0.571145109));
#124122=CARTESIAN_POINT('Ctrl Pts',(-7.24783394100001,3.914045302,-0.177209386));
#124123=CARTESIAN_POINT('Ctrl Pts',(-7.46153873851908,3.78339966801642,
-0.758620738679522));
#124124=CARTESIAN_POINT('Ctrl Pts',(-7.46194452325954,3.78403814050821,
-0.754586229339761));
#124125=CARTESIAN_POINT('Ctrl Pts',(-7.462350308,3.784676613,-0.750551720000001));
#124126=CARTESIAN_POINT('Ctrl Pts',(-7.503144445,3.848863192,-0.34495656));
#124127=CARTESIAN_POINT('Ctrl Pts',(-7.499738154,3.914045302,0.062670712));
#124128=CARTESIAN_POINT('Origin',(0.193420885555706,4.01777118640439,-0.0125098067846215));
#124129=CARTESIAN_POINT('Ctrl Pts',(-7.038030922,3.914032935,-1.740293292));
#124130=CARTESIAN_POINT('Ctrl Pts',(-7.053700988,3.90342418,-1.67692098));
#124131=CARTESIAN_POINT('Ctrl Pts',(-7.068227363,3.892857143,-1.613276771));
#124132=CARTESIAN_POINT('Ctrl Pts',(-7.141970577,3.839213527,-1.290186641));
#124133=CARTESIAN_POINT('Ctrl Pts',(-7.185930826,3.784676613,-0.961716262));
#124134=CARTESIAN_POINT('Ctrl Pts',(-7.18645899013354,3.78402137462933,
-0.957769826821296));
#124135=CARTESIAN_POINT('Ctrl Pts',(-7.18698715426708,3.78336613625867,
-0.953823391642592));
#124136=CARTESIAN_POINT('Ctrl Pts',(-7.21776353400001,3.914032935,-2.038109313));
#124137=CARTESIAN_POINT('Ctrl Pts',(-7.236115215,3.90342418,-1.97311864));
#124138=CARTESIAN_POINT('Ctrl Pts',(-7.253293629,3.892857143,-1.907808045));
#124139=CARTESIAN_POINT('Ctrl Pts',(-7.340499928,3.839213527,-1.576258498));
#124140=CARTESIAN_POINT('Ctrl Pts',(-7.397095368,3.784676613,-1.238135744));
#124141=CARTESIAN_POINT('Ctrl Pts',(-7.39777533870557,3.78402137462933,
-1.23407333954463));
#124142=CARTESIAN_POINT('Ctrl Pts',(-7.39845530941115,3.78336613625867,
-1.23001093508926));
#124143=CARTESIAN_POINT('',(-7.03916235933143,3.91326598489301,-1.73571117188066));
#124144=CARTESIAN_POINT('Ctrl Pts',(-7.03916235763906,3.91326598504639,
-1.73571117593494));
#124145=CARTESIAN_POINT('Ctrl Pts',(-7.05422615,3.903042157,-1.674620094));
#124146=CARTESIAN_POINT('Ctrl Pts',(-7.068227363,3.892857143,-1.613276771));
#124147=CARTESIAN_POINT('Ctrl Pts',(-7.14197057734831,3.83921352753312,
-1.29018664159581));
#124148=CARTESIAN_POINT('Ctrl Pts',(-7.18593082707106,3.78467661278557,
-0.96171626364151));
#124149=CARTESIAN_POINT('Ctrl Pts',(-7.28242661707377,3.87435041323117,
-1.79339414618054));
#124150=CARTESIAN_POINT('Ctrl Pts',(-7.25450801706575,3.87860220116321,
-1.78672327941277));
#124151=CARTESIAN_POINT('Ctrl Pts',(-7.22659324614468,3.88292159131356,
-1.78007903323408));
#124152=CARTESIAN_POINT('Ctrl Pts',(-7.19868298126388,3.88731207464196,
-1.77346334495166));
#124153=CARTESIAN_POINT('Ctrl Pts',(-7.17207744626437,3.8914973146731,-1.76715692231842));
#124154=CARTESIAN_POINT('Ctrl Pts',(-7.14547428273653,3.89574618497195,
-1.76088229411127));
#124155=CARTESIAN_POINT('Ctrl Pts',(-7.1188867549914,3.90006996196626,-1.75459342542347));
#124156=CARTESIAN_POINT('Ctrl Pts',(-7.09229849054837,3.90439385876552,
-1.74830438248117));
#124157=CARTESIAN_POINT('Ctrl Pts',(-7.06572323930961,3.90879118062557,
-1.74201033436876));
#124158=CARTESIAN_POINT('Ctrl Pts',(-7.03916235886328,3.91326598396044,
-1.73571117489821));
#124159=CARTESIAN_POINT('Ctrl Pts',(-6.80850125154208,3.78339966801642,
-2.49135950079383));
#124160=CARTESIAN_POINT('Ctrl Pts',(-6.80984421977104,3.78403814050821,
-2.48767704189692));
#124161=CARTESIAN_POINT('Ctrl Pts',(-6.811187188,3.784676613,-2.483994583));
#124162=CARTESIAN_POINT('Ctrl Pts',(-6.94619776,3.848863192,-2.113791572));
#124163=CARTESIAN_POINT('Ctrl Pts',(-7.040288831,3.914045302,-1.731136382));
#124164=CARTESIAN_POINT('Ctrl Pts',(-7.12401107506173,3.78339966801642,
-2.34489487403908));
#124165=CARTESIAN_POINT('Ctrl Pts',(-7.12527467303087,3.78403814050821,
-2.34104192101954));
#124166=CARTESIAN_POINT('Ctrl Pts',(-7.126538271,3.784676613,-2.337188968));
#124167=CARTESIAN_POINT('Ctrl Pts',(-7.253569634,3.848863192,-1.949845932));
#124168=CARTESIAN_POINT('Ctrl Pts',(-7.337870794,3.914045302,-1.551016507));
#124169=CARTESIAN_POINT('Origin',(0.191588194309098,4.01777119498489,0.0293624839387421));
#124170=CARTESIAN_POINT('Ctrl Pts',(-6.499374055,3.914032935,-3.212574807));
#124171=CARTESIAN_POINT('Ctrl Pts',(-6.528300937,3.90342418,-3.154052706));
#124172=CARTESIAN_POINT('Ctrl Pts',(-6.556169318,3.892857143,-3.095019205));
#124173=CARTESIAN_POINT('Ctrl Pts',(-6.697643284,3.839213527,-2.795335353));
#124174=CARTESIAN_POINT('Ctrl Pts',(-6.811187188,3.784676613,-2.483994583));
#124175=CARTESIAN_POINT('Ctrl Pts',(-6.81255137084789,3.78402137462933,
-2.48025395295892));
#124176=CARTESIAN_POINT('Ctrl Pts',(-6.81391555369579,3.78336613625867,
-2.47651332291784));
#124177=CARTESIAN_POINT('Ctrl Pts',(-6.610882977,3.914032935,-3.542065254));
#124178=CARTESIAN_POINT('Ctrl Pts',(-6.64277668,3.90342418,-3.482539096));
#124179=CARTESIAN_POINT('Ctrl Pts',(-6.673593319,3.892857143,-3.422448278));
#124180=CARTESIAN_POINT('Ctrl Pts',(-6.830034135,3.839213527,-3.117396951));
#124181=CARTESIAN_POINT('Ctrl Pts',(-6.957992803,3.784676613,-2.799345666));
#124182=CARTESIAN_POINT('Ctrl Pts',(-6.95953017325041,3.78402137462933,
-2.7955244119083));
#124183=CARTESIAN_POINT('Ctrl Pts',(-6.96106754350082,3.78336613625867,
-2.7917031578166));
#124184=CARTESIAN_POINT('',(-6.50146406065124,3.91326598485366,-3.20834304064166));
#124185=CARTESIAN_POINT('Ctrl Pts',(-6.50146405798387,3.91326598504639,
-3.20834304420609));
#124186=CARTESIAN_POINT('Ctrl Pts',(-6.529308444,3.903042157,-3.151918508));
#124187=CARTESIAN_POINT('Ctrl Pts',(-6.556169318,3.892857143,-3.095019205));
#124188=CARTESIAN_POINT('Ctrl Pts',(-6.69764328314188,3.83921352754265,
-2.79533535427979));
#124189=CARTESIAN_POINT('Ctrl Pts',(-6.81118718892826,3.78467661279769,
-2.48399458497579));
#124190=CARTESIAN_POINT('Ctrl Pts',(-6.72664080068503,3.874350413243,-3.31697204352362));
#124191=CARTESIAN_POINT('Ctrl Pts',(-6.70080896102677,3.87860220111571,
-3.3044554644234));
#124192=CARTESIAN_POINT('Ctrl Pts',(-6.67497513854352,3.88292159126161,
-3.29196570633432));
#124193=CARTESIAN_POINT('Ctrl Pts',(-6.64913957764185,3.88731207458674,
-3.27950480713943));
#124194=CARTESIAN_POINT('Ctrl Pts',(-6.62451175980179,3.89149731461202,
-3.26762642150409));
#124195=CARTESIAN_POINT('Ctrl Pts',(-6.59987942312048,3.89574618490558,
-3.25577959675733));
#124196=CARTESIAN_POINT('Ctrl Pts',(-6.57526541791268,3.90006996188385,
-3.24392222576582));
#124197=CARTESIAN_POINT('Ctrl Pts',(-6.55065073069009,3.90439385866708,
-3.23206452622549));
#124198=CARTESIAN_POINT('Ctrl Pts',(-6.52604982838253,3.90879118050865,
-3.22020473601112));
#124199=CARTESIAN_POINT('Ctrl Pts',(-6.50146405949151,3.91326598380885,
-3.20834304338909));
#124200=CARTESIAN_POINT('Ctrl Pts',(-6.1137536276454,3.78339966801642,-3.8967394111811));
#124201=CARTESIAN_POINT('Ctrl Pts',(-6.11585681782271,3.78403814050821,
-3.89343174459055));
#124202=CARTESIAN_POINT('Ctrl Pts',(-6.117960008,3.784676613,-3.890124078));
#124203=CARTESIAN_POINT('Ctrl Pts',(-6.329396811,3.848863192,-3.557599489));
#124204=CARTESIAN_POINT('Ctrl Pts',(-6.503547641,3.914045302,-3.204117364));
#124205=CARTESIAN_POINT('Ctrl Pts',(-6.45337257147076,3.78339966801642,
-3.82152433181391));
#124206=CARTESIAN_POINT('Ctrl Pts',(-6.45543489823538,3.78403814050821,
-3.81803309490696));
#124207=CARTESIAN_POINT('Ctrl Pts',(-6.457497225,3.784676613,-3.814541858));
#124208=CARTESIAN_POINT('Ctrl Pts',(-6.664825969,3.848863192,-3.463562675));
#124209=CARTESIAN_POINT('Ctrl Pts',(-6.832892752,3.914045302,-3.092179918));
#124210=CARTESIAN_POINT('Origin',(0.180796726433546,4.01777118709131,0.0698617078634745));
#124211=CARTESIAN_POINT('Ctrl Pts',(-5.656813681,3.914032935,-4.53463989500001));
#124212=CARTESIAN_POINT('Ctrl Pts',(-5.697644791,3.90342418,-4.483704433));
#124213=CARTESIAN_POINT('Ctrl Pts',(-5.737552082,3.892857143,-4.43204198));
#124214=CARTESIAN_POINT('Ctrl Pts',(-5.940141634,3.839213527,-4.169777291));
#124215=CARTESIAN_POINT('Ctrl Pts',(-6.117960008,3.784676613,-3.890124078));
#124216=CARTESIAN_POINT('Ctrl Pts',(-6.12009642190956,3.78402137462933,
-3.88676416079535));
#124217=CARTESIAN_POINT('Ctrl Pts',(-6.12223283581911,3.78336613625867,
-3.8834042435907));
#124218=CARTESIAN_POINT('Ctrl Pts',(-5.69488488000001,3.914032935,-4.88039816));
#124219=CARTESIAN_POINT('Ctrl Pts',(-5.73882929,3.90342418,-4.82911989400001));
#124220=CARTESIAN_POINT('Ctrl Pts',(-5.781843203,3.892857143,-4.777058632));
#124221=CARTESIAN_POINT('Ctrl Pts',(-6.000203538,3.839213527,-4.512769388));
#124222=CARTESIAN_POINT('Ctrl Pts',(-6.193542228,3.784676613,-4.229661295));
#124223=CARTESIAN_POINT('Ctrl Pts',(-6.19586511206018,3.78402137462933,
-4.22625986884708));
#124224=CARTESIAN_POINT('Ctrl Pts',(-6.19818799612036,3.78336613625867,
-4.22285844269416));
#124225=CARTESIAN_POINT('',(-5.65976452842113,3.91326598494767,-4.53095635412661));
#124226=CARTESIAN_POINT('Ctrl Pts',(-5.65976452843428,3.91326598549518,
-4.53095635402317));
#124227=CARTESIAN_POINT('Ctrl Pts',(-5.68600352383997,3.90644394849667,
-4.49818037437931));
#124228=CARTESIAN_POINT('Ctrl Pts',(-5.71193410056366,3.89964051894245,
-4.46520603921559));
#124229=CARTESIAN_POINT('Ctrl Pts',(-5.73755208191494,3.89285714302252,
-4.43204198011011));
#124230=CARTESIAN_POINT('Ctrl Pts',(-5.82781467713491,3.86895654227978,
-4.31519147509118));
#124231=CARTESIAN_POINT('Ctrl Pts',(-5.91481573894974,3.84480668268621,
-4.19517787889522));
#124232=CARTESIAN_POINT('Ctrl Pts',(-5.99824711819163,3.82047230181262,
-4.07228824113556));
#124233=CARTESIAN_POINT('Ctrl Pts',(-6.03901424766822,3.80858177735024,
-4.01224059695898));
#124234=CARTESIAN_POINT('Ctrl Pts',(-6.07892954915294,3.79664725893554,
-3.95150690003611));
#124235=CARTESIAN_POINT('Ctrl Pts',(-6.11796000820442,3.78467661307154,
-3.89012408033314));
#124236=CARTESIAN_POINT('Ctrl Pts',(-5.85632473635433,3.87435041325547,
-4.68545201425032));
#124237=CARTESIAN_POINT('Ctrl Pts',(-5.83378752536501,3.87860220116027,
-4.66767498378072));
#124238=CARTESIAN_POINT('Ctrl Pts',(-5.81124261200345,3.88292159132248,
-4.64992372110351));
#124239=CARTESIAN_POINT('Ctrl Pts',(-5.78868979708449,3.88731207466434,
-4.63220026889469));
#124240=CARTESIAN_POINT('Ctrl Pts',(-5.76719126574319,3.8914973146917,-4.61530534051627));
#124241=CARTESIAN_POINT('Ctrl Pts',(-5.74568153657525,3.89574618498683,
-4.59844026372362));
#124242=CARTESIAN_POINT('Ctrl Pts',(-5.72419197744197,3.9000699619644,-4.58156882796319));
#124243=CARTESIAN_POINT('Ctrl Pts',(-5.70270182286743,3.90439385874691,
-4.56469692472231));
#124244=CARTESIAN_POINT('Ctrl Pts',(-5.68122558035583,3.90879118058365,
-4.54782594303456));
#124245=CARTESIAN_POINT('Ctrl Pts',(-5.65976452598906,3.91326598372246,
-4.53095635732969));
#124246=CARTESIAN_POINT('Ctrl Pts',(-5.13313367838099,3.78339966801642,
-5.11991211792546));
#124247=CARTESIAN_POINT('Ctrl Pts',(-5.13589874769049,3.78403814050821,
-5.11713390646273));
#124248=CARTESIAN_POINT('Ctrl Pts',(-5.13866381700001,3.784676613,-5.114355695));
#124249=CARTESIAN_POINT('Ctrl Pts',(-5.416640303,3.848863192,-4.835058009));
#124250=CARTESIAN_POINT('Ctrl Pts',(-5.662707791,3.914045302,-4.52727738));
#124251=CARTESIAN_POINT('Ctrl Pts',(-5.48098153912164,3.78339966801642,
-5.11946355990375));
#124252=CARTESIAN_POINT('Ctrl Pts',(-5.48374616256082,3.78403814050821,
-5.11649728545188));
#124253=CARTESIAN_POINT('Ctrl Pts',(-5.486510786,3.784676613,-5.113531011));
#124254=CARTESIAN_POINT('Ctrl Pts',(-5.76444244800001,3.848863192,-4.815327076));
#124255=CARTESIAN_POINT('Ctrl Pts',(-6.008416238,3.914045302,-4.488756433));
#124256=CARTESIAN_POINT('Origin',(0.161551797490415,4.01777118461528,0.107094516475824));
#124257=CARTESIAN_POINT('Ctrl Pts',(-4.549746986,3.914032935,-5.644670262));
#124258=CARTESIAN_POINT('Ctrl Pts',(-4.600573106,3.90342418,-5.603703124));
#124259=CARTESIAN_POINT('Ctrl Pts',(-4.650653287,3.892857143,-5.561827398));
#124260=CARTESIAN_POINT('Ctrl Pts',(-4.904885564,3.839213527,-5.349245077));
#124261=CARTESIAN_POINT('Ctrl Pts',(-5.138663817,3.784676613,-5.114355695));
#124262=CARTESIAN_POINT('Ctrl Pts',(-5.14147256561369,3.78402137462933,
-5.11153359663286));
#124263=CARTESIAN_POINT('Ctrl Pts',(-5.14428131422739,3.78336613625867,
-5.10871149826573));
#124264=CARTESIAN_POINT('Ctrl Pts',(-4.512600295,3.914032935,-5.99052907300001));
#124265=CARTESIAN_POINT('Ctrl Pts',(-4.566540621,3.90342418,-5.949896413));
#124266=CARTESIAN_POINT('Ctrl Pts',(-4.619740525,3.892857143,-5.908299035));
#124267=CARTESIAN_POINT('Ctrl Pts',(-4.889810092,3.839213527,-5.697129743));
#124268=CARTESIAN_POINT('Ctrl Pts',(-5.139488502,3.784676613,-5.462202664));
#124269=CARTESIAN_POINT('Ctrl Pts',(-5.14248828439617,3.78402137462933,
-5.45938011271906));
#124270=CARTESIAN_POINT('Ctrl Pts',(-5.14548806679234,3.78336613625867,
-5.45655756143813));
#124271=CARTESIAN_POINT('',(-4.55342069631209,3.91326598487342,-5.64170718412929));
#124272=CARTESIAN_POINT('Ctrl Pts',(-4.55342069208161,3.91326598504639,
-5.64170718634669));
#124273=CARTESIAN_POINT('Ctrl Pts',(-4.602383621,3.903042157,-5.602189219));
#124274=CARTESIAN_POINT('Ctrl Pts',(-4.650653287,3.892857143,-5.561827398));
#124275=CARTESIAN_POINT('Ctrl Pts',(-4.90488556315104,3.83921352756483,
-5.34924507770047));
#124276=CARTESIAN_POINT('Ctrl Pts',(-5.13866381694183,3.78467661279893,
-5.114355697307));
#124277=CARTESIAN_POINT('Ctrl Pts',(-4.71217343650642,3.87435041320727,
-5.83484545654915));
#124278=CARTESIAN_POINT('Ctrl Pts',(-4.69398466915291,3.87860220113085,
-5.81263920890565));
#124279=CARTESIAN_POINT('Ctrl Pts',(-4.6757828400969,3.8829215912813,-5.79045647096184));
#124280=CARTESIAN_POINT('Ctrl Pts',(-4.65756731577416,3.88731207461094,
-5.76829919469483));
#124281=CARTESIAN_POINT('Ctrl Pts',(-4.64020331825134,3.89149731464626,
-5.74717771153595));
#124282=CARTESIAN_POINT('Ctrl Pts',(-4.62282196747897,3.89574618494989,
-5.72608297484968));
#124283=CARTESIAN_POINT('Ctrl Pts',(-4.60546168216947,3.90006996193938,
-5.70498636382479));
#124284=CARTESIAN_POINT('Ctrl Pts',(-4.58810091583424,3.90439385873382,
-5.68388916824655));
#124285=CARTESIAN_POINT('Ctrl Pts',(-4.57075353820189,3.90879118058493,
-5.66279586335939));
#124286=CARTESIAN_POINT('Ctrl Pts',(-4.55342069426683,3.91326598388217,
-5.64170718630607));
#124287=CARTESIAN_POINT('Ctrl Pts',(-3.91249410326131,3.78339966801642,
-6.10368342451692));
#124288=CARTESIAN_POINT('Ctrl Pts',(-3.91579176013065,3.78403814050821,
-6.10156457425846));
#124289=CARTESIAN_POINT('Ctrl Pts',(-3.919089417,3.784676613,-6.09944572400001));
#124290=CARTESIAN_POINT('Ctrl Pts',(-4.250607714,3.848863192,-5.88643459));
#124291=CARTESIAN_POINT('Ctrl Pts',(-4.55708601800001,3.914045302,-5.63874693700001));
#124292=CARTESIAN_POINT('Ctrl Pts',(-4.25230590117908,3.78339966801642,
-6.17802236055207));
#124293=CARTESIAN_POINT('Ctrl Pts',(-4.25564355058954,3.78403814050821,
-6.17571974827603));
#124294=CARTESIAN_POINT('Ctrl Pts',(-4.2589812,3.784676613,-6.173417136));
#124295=CARTESIAN_POINT('Ctrl Pts',(-4.594520006,3.848863192,-5.941932136));
#124296=CARTESIAN_POINT('Ctrl Pts',(-4.90299285900001,3.914045302,-5.675443685));
#124297=CARTESIAN_POINT('Origin',(0.134752179725973,4.0177709926056,0.139318973597412));
#124298=CARTESIAN_POINT('Ctrl Pts',(-3.229939179,3.914032935,-6.49076212));
#124299=CARTESIAN_POINT('Ctrl Pts',(-3.288383736,3.90342418,-6.461678884));
#124300=CARTESIAN_POINT('Ctrl Pts',(-3.346295113,3.892857143,-6.431547949));
#124301=CARTESIAN_POINT('Ctrl Pts',(-3.640282496,3.839213527,-6.278588109));
#124302=CARTESIAN_POINT('Ctrl Pts',(-3.919089417,3.784676613,-6.09944572399999));
#124303=CARTESIAN_POINT('Ctrl Pts',(-3.92243916635777,3.78402137462933,
-6.09729340264818));
#124304=CARTESIAN_POINT('Ctrl Pts',(-3.92578891571553,3.78336613625867,
-6.09514108129637));
#124305=CARTESIAN_POINT('Ctrl Pts',(-3.119311536,3.914032935,-6.820549504));
#124306=CARTESIAN_POINT('Ctrl Pts',(-3.180725587,3.90342418,-6.792462389));
#124307=CARTESIAN_POINT('Ctrl Pts',(-3.241623914,3.892857143,-6.763273941));
#124308=CARTESIAN_POINT('Ctrl Pts',(-3.55077456,3.839213527,-6.615098643));
#124309=CARTESIAN_POINT('Ctrl Pts',(-3.845118005,3.784676613,-6.439337507));
#124310=CARTESIAN_POINT('Ctrl Pts',(-3.84865441924078,3.78402137462933,
-6.43722580995057));
#124311=CARTESIAN_POINT('Ctrl Pts',(-3.85219083348155,3.78336613625867,
-6.43511411290114));
#124312=CARTESIAN_POINT('',(-3.234163974001,3.91326598471179,-6.4886580577403));
#124313=CARTESIAN_POINT('Ctrl Pts',(-3.23416396978397,3.91326598504639,
-6.48865805903995));
#124314=CARTESIAN_POINT('Ctrl Pts',(-3.290477367,3.903042157,-6.460589581));
#124315=CARTESIAN_POINT('Ctrl Pts',(-3.346295113,3.892857143,-6.431547949));
#124316=CARTESIAN_POINT('Ctrl Pts',(-3.64028249503674,3.83921352754219,
-6.27858810986231));
#124317=CARTESIAN_POINT('Ctrl Pts',(-3.91908941581858,3.78467661181153,
-6.09944572483374));
#124318=CARTESIAN_POINT('Ctrl Pts',(-3.3476861436547,3.87435041322755,-6.71140801016537));
#124319=CARTESIAN_POINT('Ctrl Pts',(-3.33469630621779,3.87860220110384,
-6.68581088513763));
#124320=CARTESIAN_POINT('Ctrl Pts',(-3.32168865877955,3.88292159125227,
-6.66023391214072));
#124321=CARTESIAN_POINT('Ctrl Pts',(-3.30866216274858,3.8873120745777,-6.63467886147286));
#124322=CARTESIAN_POINT('Ctrl Pts',(-3.29624462038394,3.89149731461195,
-6.61031844071623));
#124323=CARTESIAN_POINT('Ctrl Pts',(-3.28380438072982,3.89574618490461,
-6.58598041070877));
#124324=CARTESIAN_POINT('Ctrl Pts',(-3.27138511704215,3.90006996189716,
-6.56164507859973));
#124325=CARTESIAN_POINT('Ctrl Pts',(-3.2589655092365,3.90439385869467,-6.53730907219747));
#124326=CARTESIAN_POINT('Ctrl Pts',(-3.24655814078464,3.90879118056004,
-6.51297974367115));
#124327=CARTESIAN_POINT('Ctrl Pts',(-3.23416397113967,3.91326598383281,
-6.48865805919438));
#124328=CARTESIAN_POINT('Ctrl Pts',(-2.50891065267966,3.78339966801642,
-6.80205327793971));
#124329=CARTESIAN_POINT('Ctrl Pts',(-2.51258670233983,3.78403814050821,
-6.80069286396985));
#124330=CARTESIAN_POINT('Ctrl Pts',(-2.516262752,3.784676613,-6.79933245));
#124331=CARTESIAN_POINT('Ctrl Pts',(-2.885821433,3.848863192,-6.662568032));
#124332=CARTESIAN_POINT('Ctrl Pts',(-3.238379968,3.914045302,-6.486554955));
#124333=CARTESIAN_POINT('Ctrl Pts',(-2.82479716579741,3.78339966801642,
-6.94770370202509));
#124334=CARTESIAN_POINT('Ctrl Pts',(-2.8285517763987,3.78403814050821,-6.94617241951255));
#124335=CARTESIAN_POINT('Ctrl Pts',(-2.832306387,3.784676613,-6.944641137));
#124336=CARTESIAN_POINT('Ctrl Pts',(-3.209762915,3.848863192,-6.790699053));
#124337=CARTESIAN_POINT('Ctrl Pts',(-3.568310983,3.914045302,-6.596753499));
#124338=CARTESIAN_POINT('Origin',(0.101652530173353,4.01777101481532,0.165030098550536));
#124339=CARTESIAN_POINT('Ctrl Pts',(-1.759103005,3.914032935,-7.033353156));
#124340=CARTESIAN_POINT('Ctrl Pts',(-1.822433198,3.90342418,-7.017513722));
#124341=CARTESIAN_POINT('Ctrl Pts',(-1.885467899,3.892857143,-7.000536465));
#124342=CARTESIAN_POINT('Ctrl Pts',(-2.205463864,3.839213527,-6.914351339));
#124343=CARTESIAN_POINT('Ctrl Pts',(-2.516262752,3.784676613,-6.79933245));
#124344=CARTESIAN_POINT('Ctrl Pts',(-2.51999687155391,3.78402137462933,
-6.79795054581994));
#124345=CARTESIAN_POINT('Ctrl Pts',(-2.52373099110783,3.78336613625867,
-6.79656864163989));
#124346=CARTESIAN_POINT('Ctrl Pts',(-1.580167237,3.914032935,-7.331648621));
#124347=CARTESIAN_POINT('Ctrl Pts',(-1.646183361,3.90342418,-7.317420373));
#124348=CARTESIAN_POINT('Ctrl Pts',(-1.711932572,3.892857143,-7.302005674));
#124349=CARTESIAN_POINT('Ctrl Pts',(-2.045708757,3.839213527,-7.223752884));
#124350=CARTESIAN_POINT('Ctrl Pts',(-2.370954065,3.784676613,-7.115376084));
#124351=CARTESIAN_POINT('Ctrl Pts',(-2.37486175229012,3.78402137462933,
-7.11407398176059));
#124352=CARTESIAN_POINT('Ctrl Pts',(-2.37876943958024,3.78336613625867,
-7.11277187952119));
#124353=CARTESIAN_POINT('',(-1.76368133860213,3.91326598469372,-7.03220649149698));
#124354=CARTESIAN_POINT('Ctrl Pts',(-1.76368133412727,3.91326598504639,
-7.03220649202675));
#124355=CARTESIAN_POINT('Ctrl Pts',(-1.824712048,3.903042157,-7.016899955));
#124356=CARTESIAN_POINT('Ctrl Pts',(-1.885467899,3.892857143,-7.000536465));
#124357=CARTESIAN_POINT('Ctrl Pts',(-2.2054638634848,3.83921352755012,-6.91435133898436));
#124358=CARTESIAN_POINT('Ctrl Pts',(-2.51626275037259,3.78467661195553,
-6.79933245013235));
#124359=CARTESIAN_POINT('Ctrl Pts',(-1.82666476776869,3.87435041321898,
-7.27415258436543));
#124360=CARTESIAN_POINT('Ctrl Pts',(-1.81948125070448,3.87860220108891,
-7.24636147483946));
#124361=CARTESIAN_POINT('Ctrl Pts',(-1.81227600790523,3.88292159123251,
-7.21858621756027));
#124362=CARTESIAN_POINT('Ctrl Pts',(-1.80504764454275,3.88731207455456,
-7.19082831818905));
#124363=CARTESIAN_POINT('Ctrl Pts',(-1.79815718774571,3.89149731457801,
-7.16436802603133));
#124364=CARTESIAN_POINT('Ctrl Pts',(-1.79123975117751,3.89574618489468,
-7.13792472184617));
#124365=CARTESIAN_POINT('Ctrl Pts',(-1.7843422201044,3.90006996189343,-7.11148856171909));
#124366=CARTESIAN_POINT('Ctrl Pts',(-1.77744449791178,3.9043938586971,-7.08505166908842));
#124367=CARTESIAN_POINT('Ctrl Pts',(-1.77055729322819,3.90879118054189,
-7.05862392934173));
#124368=CARTESIAN_POINT('Ctrl Pts',(-1.76368133504616,3.91326598374363,
-7.03220649222192));
#124369=CARTESIAN_POINT('Ctrl Pts',(-0.988013329107109,3.78339966801642,
-7.18236667945575));
#124370=CARTESIAN_POINT('Ctrl Pts',(-0.991895883553554,3.78403814050821,
-7.18182831322788));
#124371=CARTESIAN_POINT('Ctrl Pts',(-0.995778438,3.784676613,-7.181289947));
#124372=CARTESIAN_POINT('Ctrl Pts',(-1.386097349,3.848863192,-7.12716719800001));
#124373=CARTESIAN_POINT('Ctrl Pts',(-1.76825087,3.914045302,-7.031058872));
#124374=CARTESIAN_POINT('Ctrl Pts',(-1.26520405425852,3.78339966801642,
-7.39251814139622));
#124375=CARTESIAN_POINT('Ctrl Pts',(-1.26920006462926,3.78403814050821,
-7.39182978969811));
#124376=CARTESIAN_POINT('Ctrl Pts',(-1.273196075,3.784676613,-7.39114143800001));
#124377=CARTESIAN_POINT('Ctrl Pts',(-1.674920877,3.848863192,-7.321940429));
#124378=CARTESIAN_POINT('Ctrl Pts',(-2.066778852,3.914045302,-7.209606451));
#124379=CARTESIAN_POINT('Origin',(0.0637993348120211,4.01777099075444,0.183023921145155));
#124380=CARTESIAN_POINT('Ctrl Pts',(-0.206013131,3.914032935,-7.247072415));
#124381=CARTESIAN_POINT('Ctrl Pts',(-0.271267708,3.90342418,-7.245217418));
#124382=CARTESIAN_POINT('Ctrl Pts',(-0.336478302,3.892857143,-7.242187677));
#124383=CARTESIAN_POINT('Ctrl Pts',(-0.667520194,3.839213527,-7.226807185));
#124384=CARTESIAN_POINT('Ctrl Pts',(-0.995778438,3.784676613,-7.181289947));
#124385=CARTESIAN_POINT('Ctrl Pts',(-0.999722324464786,3.78402137462933,
-7.18074307629029));
#124386=CARTESIAN_POINT('Ctrl Pts',(-1.00366621092957,3.78336613625867,
-7.18019620558059));
#124387=CARTESIAN_POINT('Ctrl Pts',(0.032863927,3.914032935,-7.499927997));
#124388=CARTESIAN_POINT('Ctrl Pts',(-0.03466743,3.90342418,-7.500223913));
#124389=CARTESIAN_POINT('Ctrl Pts',(-0.102193166,3.892857143,-7.499303738));
#124390=CARTESIAN_POINT('Ctrl Pts',(-0.444987886,3.839213527,-7.494632467));
#124391=CARTESIAN_POINT('Ctrl Pts',(-0.785926947,3.784676613,-7.458707585));
#124392=CARTESIAN_POINT('Ctrl Pts',(-0.790023188214264,3.78402137462933,
-7.45827596246361));
#124393=CARTESIAN_POINT('Ctrl Pts',(-0.794119429428528,3.78336613625867,
-7.4578443399272));
#124394=CARTESIAN_POINT('',(-0.210730925048304,3.91326598495388,-7.24693676499616));
#124395=CARTESIAN_POINT('Ctrl Pts',(-0.210730925117643,3.91326598525536,
-7.24693676569531));
#124396=CARTESIAN_POINT('Ctrl Pts',(-0.341742803026686,3.89196925411006,
-7.24312712114134));
#124397=CARTESIAN_POINT('Ctrl Pts',(-0.472587783383507,3.87079710536095,
-7.23576926099415));
#124398=CARTESIAN_POINT('Ctrl Pts',(-0.668801818713384,3.83867883707161,
-7.21938563561741));
#124399=CARTESIAN_POINT('Ctrl Pts',(-0.734255518074978,3.82792484001174,
-7.21302242832566));
#124400=CARTESIAN_POINT('Ctrl Pts',(-0.8323440796812,3.81174904512853,-7.20213774459991));
#124401=CARTESIAN_POINT('Ctrl Pts',(-0.865052750424345,3.80634502469735,
-7.19828232153745));
#124402=CARTESIAN_POINT('Ctrl Pts',(-0.91408637592218,3.79822878950977,
-7.1921636313569));
#124403=CARTESIAN_POINT('Ctrl Pts',(-0.93043242491259,3.795520612997,-7.19006725232141));
#124404=CARTESIAN_POINT('Ctrl Pts',(-0.954943348359991,3.79145592368764,
-7.18683874599003));
#124405=CARTESIAN_POINT('Ctrl Pts',(-0.963113831538947,3.79010036834645,
-7.18574837480559));
#124406=CARTESIAN_POINT('Ctrl Pts',(-0.979077887758595,3.78745055926263,
-7.18359021558888));
#124407=CARTESIAN_POINT('Ctrl Pts',(-0.983007263997672,3.7867984191769,
-7.18306083599155));
#124408=CARTESIAN_POINT('Ctrl Pts',(-0.995778437250238,3.78467661296255,
-7.18128994825785));
#124409=CARTESIAN_POINT('Ctrl Pts',(-0.220230577341825,3.87435041326975,
-7.49676586842818));
#124410=CARTESIAN_POINT('Ctrl Pts',(-0.219189274043534,3.87860220113651,
-7.46808025586321));
#124411=CARTESIAN_POINT('Ctrl Pts',(-0.218123345138543,3.8829215912762,
-7.43940545450373));
#124412=CARTESIAN_POINT('Ctrl Pts',(-0.217031104751613,3.88731207459202,
-7.41074263500273));
#124413=CARTESIAN_POINT('Ctrl Pts',(-0.215989923663363,3.89149731462842,
-7.38341972517652));
#124414=CARTESIAN_POINT('Ctrl Pts',(-0.214918741528663,3.89574618493874,
-7.3561076063082));
#124415=CARTESIAN_POINT('Ctrl Pts',(-0.213865463789634,3.90006996194319,
-7.32880674356716));
#124416=CARTESIAN_POINT('Ctrl Pts',(-0.21281215686596,3.9043938587526,-7.30150512436279));
#124417=CARTESIAN_POINT('Ctrl Pts',(-0.211767154034762,3.90879118062038,
-7.27421470500944));
#124418=CARTESIAN_POINT('Ctrl Pts',(-0.210730921496787,3.91326598402241,
-7.24693676549611));
#124419=CARTESIAN_POINT('Ctrl Pts',(0.579082400613263,3.78339966801642,
-7.22684059819051));
#124420=CARTESIAN_POINT('Ctrl Pts',(0.575174885306631,3.78403814050821,
-7.22714945309525));
#124421=CARTESIAN_POINT('Ctrl Pts',(0.57126737,3.784676613,-7.22745830800001));
#124422=CARTESIAN_POINT('Ctrl Pts',(0.178439107,3.848863192,-7.258507946));
#124423=CARTESIAN_POINT('Ctrl Pts',(-0.215440326,3.914045302,-7.246798291));
#124424=CARTESIAN_POINT('Ctrl Pts',(0.353548592258207,3.78339966801642,
-7.49166664761222));
#124425=CARTESIAN_POINT('Ctrl Pts',(0.349498031129104,3.78403814050821,
-7.49185341330611));
#124426=CARTESIAN_POINT('Ctrl Pts',(0.34544747,3.784676613,-7.492040179));
#124427=CARTESIAN_POINT('Ctrl Pts',(-0.0617614,3.848863192,-7.51081600900001));
#124428=CARTESIAN_POINT('Ctrl Pts',(-0.468606438,3.914045302,-7.485346218));
#124429=CARTESIAN_POINT('Origin',(0.0229630490407847,4.01777116662245,0.192459969041543));
#124430=CARTESIAN_POINT('Ctrl Pts',(1.356709689,3.914032935,-7.121926623));
#124431=CARTESIAN_POINT('Ctrl Pts',(1.292581958,3.90342418,-7.134142799));
#124432=CARTESIAN_POINT('Ctrl Pts',(1.228244647,3.892857143,-7.145202243));
#124433=CARTESIAN_POINT('Ctrl Pts',(0.901635979,3.839213527,-7.201345559));
#124434=CARTESIAN_POINT('Ctrl Pts',(0.57126737,3.784676613,-7.227458308));
#124435=CARTESIAN_POINT('Ctrl Pts',(0.567298128376246,3.78402137462933,
-7.22777204183371));
#124436=CARTESIAN_POINT('Ctrl Pts',(0.563328886752492,3.78336613625867,
-7.22808577566744));
#124437=CARTESIAN_POINT('Ctrl Pts',(1.64435841,3.914032935,-7.317519076));
#124438=CARTESIAN_POINT('Ctrl Pts',(1.578469512,3.90342418,-7.332325318));
#124439=CARTESIAN_POINT('Ctrl Pts',(1.51232468,3.892857143,-7.345942694));
#124440=CARTESIAN_POINT('Ctrl Pts',(1.176540125,3.839213527,-7.415071367));
#124441=CARTESIAN_POINT('Ctrl Pts',(0.835849241,3.784676613,-7.453278208));
#124442=CARTESIAN_POINT('Ctrl Pts',(0.831755981529315,3.78402137462933,
-7.453737247326));
#124443=CARTESIAN_POINT('Ctrl Pts',(0.82766272205863,3.78336613625867,-7.45419628665201));
#124444=CARTESIAN_POINT('',(1.35207303378698,3.91326598496294,-7.12280833054815));
#124445=CARTESIAN_POINT('Ctrl Pts',(1.35207303380376,3.91326598533785,-7.12280833096319));
#124446=CARTESIAN_POINT('Ctrl Pts',(1.22330513007813,3.8919692459027,-7.14725144316222));
#124447=CARTESIAN_POINT('Ctrl Pts',(1.09393752589995,3.87079709988476,-7.16819340483977));
#124448=CARTESIAN_POINT('Ctrl Pts',(0.898788929512348,3.83867884132354,
-7.19437302890363));
#124449=CARTESIAN_POINT('Ctrl Pts',(0.833497623644794,3.82792484808616,
-7.20222919913091));
#124450=CARTESIAN_POINT('Ctrl Pts',(0.735362384832814,3.81174904529717,
-7.21268513953307));
#124451=CARTESIAN_POINT('Ctrl Pts',(0.702589622489829,3.80634502484376,
-7.21595125144429));
#124452=CARTESIAN_POINT('Ctrl Pts',(0.653387038160116,3.7982287896232,-7.22051639285995));
#124453=CARTESIAN_POINT('Ctrl Pts',(0.63697249111092,3.79552061309923,-7.22198294333527));
#124454=CARTESIAN_POINT('Ctrl Pts',(0.612340585893026,3.79145592377342,
-7.22409904167042));
#124455=CARTESIAN_POINT('Ctrl Pts',(0.604126726459193,3.79010036842672,
-7.22479057511699));
#124456=CARTESIAN_POINT('Ctrl Pts',(0.588071960564506,3.78745055934405,
-7.22611467263649));
#124457=CARTESIAN_POINT('Ctrl Pts',(0.584120650273446,3.78679841930492,
-7.22644236935304));
#124458=CARTESIAN_POINT('Ctrl Pts',(0.571267371024303,3.78467661302323,
-7.227458308743));
#124459=CARTESIAN_POINT('Ctrl Pts',(1.39650135047031,3.8743504132196,-7.36883871285757));
#124460=CARTESIAN_POINT('Ctrl Pts',(1.39135174990272,3.87860220112565,-7.34059990434166));
#124461=CARTESIAN_POINT('Ctrl Pts',(1.3862285232922,3.8829215912896,-7.31236636061691));
#124462=CARTESIAN_POINT('Ctrl Pts',(1.38113356873396,3.88731207463253,-7.28413886241582));
#124463=CARTESIAN_POINT('Ctrl Pts',(1.37627678961713,3.89149731467127,-7.2572309239414));
#124464=CARTESIAN_POINT('Ctrl Pts',(1.37145162997354,3.89574618496625,-7.23032707475948));
#124465=CARTESIAN_POINT('Ctrl Pts',(1.36661140419777,3.90006996195997,-7.20343806747132));
#124466=CARTESIAN_POINT('Ctrl Pts',(1.36177104430707,3.90439385875865,-7.17654831513167));
#124467=CARTESIAN_POINT('Ctrl Pts',(1.35692498200478,3.9087911806267,-7.14967128594964));
#124468=CARTESIAN_POINT('Ctrl Pts',(1.35207303748469,3.91326598396996,-7.12280833022491));
#124469=CARTESIAN_POINT('Ctrl Pts',(2.11910088016766,3.78339966801642,-6.93339548231832));
#124470=CARTESIAN_POINT('Ctrl Pts',(2.11535111508383,3.78403814050821,-6.93453711665916));
#124471=CARTESIAN_POINT('Ctrl Pts',(2.11160135,3.784676613,-6.935678751));
#124472=CARTESIAN_POINT('Ctrl Pts',(1.734631949,3.848863192,-7.05044893100001));
#124473=CARTESIAN_POINT('Ctrl Pts',(1.347443968,3.914045302,-7.123685476));
#124474=CARTESIAN_POINT('Ctrl Pts',(1.95576969930549,3.78339966801642,-7.24051314774188));
#124475=CARTESIAN_POINT('Ctrl Pts',(1.95185398715275,3.78403814050821,-7.24156629787095));
#124476=CARTESIAN_POINT('Ctrl Pts',(1.947938275,3.784676613,-7.242619448));
#124477=CARTESIAN_POINT('Ctrl Pts',(1.554285971,3.848863192,-7.34849418));
#124478=CARTESIAN_POINT('Ctrl Pts',(1.151477492,3.914045302,-7.41107951600001));
#124479=CARTESIAN_POINT('Origin',(-0.0189470914091824,4.01777118429656,
0.192897026293775));
#124480=CARTESIAN_POINT('Ctrl Pts',(2.855994272,3.914032935,-6.663767457));
#124481=CARTESIAN_POINT('Ctrl Pts',(2.795991928,3.90342418,-6.689483593));
#124482=CARTESIAN_POINT('Ctrl Pts',(2.735536241,3.892857143,-6.714115092));
#124483=CARTESIAN_POINT('Ctrl Pts',(2.428632656,3.839213527,-6.839157018));
#124484=CARTESIAN_POINT('Ctrl Pts',(2.11160135,3.784676613,-6.935678751));
#124485=CARTESIAN_POINT('Ctrl Pts',(2.10779235053235,3.78402137462933,-6.93683841953322));
#124486=CARTESIAN_POINT('Ctrl Pts',(2.10398335106471,3.78336613625867,-6.93799808806644));
#124487=CARTESIAN_POINT('Ctrl Pts',(3.178964521,3.914032935,-6.792951095));
#124488=CARTESIAN_POINT('Ctrl Pts',(3.117798973,3.90342418,-6.821575341));
#124489=CARTESIAN_POINT('Ctrl Pts',(3.056127904,3.892857143,-6.849093534));
#124490=CARTESIAN_POINT('Ctrl Pts',(2.743054426,3.839213527,-6.98878977));
#124491=CARTESIAN_POINT('Ctrl Pts',(2.418542048,3.784676613,-7.099341826));
#124492=CARTESIAN_POINT('Ctrl Pts',(2.41464316655942,3.78402137462933,-7.10067006303679));
#124493=CARTESIAN_POINT('Ctrl Pts',(2.41074428511883,3.78336613625867,-7.10199830007358));
#124494=CARTESIAN_POINT('',(2.85165556048068,3.91326598476041,-6.66562529465688));
#124495=CARTESIAN_POINT('Ctrl Pts',(2.85165556055619,3.9132659853381,-6.66562529507203));
#124496=CARTESIAN_POINT('Ctrl Pts',(2.73115277808001,3.89196925540924,-6.71717821224725));
#124497=CARTESIAN_POINT('Ctrl Pts',(2.60931161017231,3.87079710731511,-6.7654407793461));
#124498=CARTESIAN_POINT('Ctrl Pts',(2.4243532403872,3.83867883409976,-6.8329595489516));
#124499=CARTESIAN_POINT('Ctrl Pts',(2.36227721360391,3.82792483428054,-6.85466775799881));
#124500=CARTESIAN_POINT('Ctrl Pts',(2.26868411913098,3.81174904513295,-6.88597539349721));
#124501=CARTESIAN_POINT('Ctrl Pts',(2.23737968355868,3.80634502473174,-6.89621032060966));
#124502=CARTESIAN_POINT('Ctrl Pts',(2.19030879911846,3.79822878957728,-6.91124583270203));
#124503=CARTESIAN_POINT('Ctrl Pts',(2.174593280194,3.79552061307862,-6.91620673842056));
#124504=CARTESIAN_POINT('Ctrl Pts',(2.15099215400452,3.79145592378738,-6.92356849502875));
#124505=CARTESIAN_POINT('Ctrl Pts',(2.14311898935416,3.79010036845298,-6.92600959777435));
#124506=CARTESIAN_POINT('Ctrl Pts',(2.12772421691881,3.78745055939456,-6.93075403869919));
#124507=CARTESIAN_POINT('Ctrl Pts',(2.12393573115497,3.78679841935278,-6.93192348897099));
#124508=CARTESIAN_POINT('Ctrl Pts',(2.11160135139247,3.78467661307689,-6.93567875136807));
#124509=CARTESIAN_POINT('Ctrl Pts',(2.94793442687894,3.8743504132592,-6.89635284857505));
#124510=CARTESIAN_POINT('Ctrl Pts',(2.93683471205565,3.87860220112973,-6.86988125968828));
#124511=CARTESIAN_POINT('Ctrl Pts',(2.92576188631293,3.88292159126709,-6.84340914287658));
#124512=CARTESIAN_POINT('Ctrl Pts',(2.91471797125888,3.88731207458112,-6.8169368525907));
#124513=CARTESIAN_POINT('Ctrl Pts',(2.90419032953263,3.89149731460779,-6.79170207068235));
#124514=CARTESIAN_POINT('Ctrl Pts',(2.89369444699761,3.8957461849108,-6.76646448526374));
#124515=CARTESIAN_POINT('Ctrl Pts',(2.8831870411466,3.90006996191208,-6.74124463351251));
#124516=CARTESIAN_POINT('Ctrl Pts',(2.87267934415219,3.9043938587183,-6.71602408295953));
#124517=CARTESIAN_POINT('Ctrl Pts',(2.86216881324473,3.90879118058129,-6.6908171839199));
#124518=CARTESIAN_POINT('Ctrl Pts',(2.85165556371442,3.9132659838416,-6.66562529299552));
#124519=CARTESIAN_POINT('Ctrl Pts',(3.56003255805081,3.78339966801642,-6.31575249957073));
#124520=CARTESIAN_POINT('Ctrl Pts',(3.5566158780254,3.78403814050821,-6.31767353178537));
#124521=CARTESIAN_POINT('Ctrl Pts',(3.553199198,3.784676613,-6.319594564));
#124522=CARTESIAN_POINT('Ctrl Pts',(3.209715328,3.848863192,-6.512718759));
#124523=CARTESIAN_POINT('Ctrl Pts',(2.847323279,3.914045302,-6.667477045));
#124524=CARTESIAN_POINT('Ctrl Pts',(3.46654118966067,3.78339966801642,-6.65080130115457));
#124525=CARTESIAN_POINT('Ctrl Pts',(3.46294342083033,3.78403814050821,-6.65267159157729));
#124526=CARTESIAN_POINT('Ctrl Pts',(3.459345652,3.784676613,-6.654541882));
#124527=CARTESIAN_POINT('Ctrl Pts',(3.097656658,3.848863192,-6.84256493));
#124528=CARTESIAN_POINT('Ctrl Pts',(2.717719614,3.914045302,-6.990278972));
#124529=CARTESIAN_POINT('Origin',(-0.0599712116260304,4.0177709640612,0.184313895487016));
#124530=CARTESIAN_POINT('Ctrl Pts',(4.221735737,3.914032935,-5.894017931));
#124531=CARTESIAN_POINT('Ctrl Pts',(4.168664423,3.90342418,-5.93203156800001));
#124532=CARTESIAN_POINT('Ctrl Pts',(4.114917201,3.892857143,-5.969083383));
#124533=CARTESIAN_POINT('Ctrl Pts',(3.842069169,3.839213527,-6.157177096));
#124534=CARTESIAN_POINT('Ctrl Pts',(3.553199198,3.784676613,-6.319594564));
#124535=CARTESIAN_POINT('Ctrl Pts',(3.54972854527601,3.78402137462933,-6.32154594242049));
#124536=CARTESIAN_POINT('Ctrl Pts',(3.54625789255202,3.78336613625867,-6.32349732084099));
#124537=CARTESIAN_POINT('Ctrl Pts',(4.564925784,3.914032935,-5.950752271));
#124538=CARTESIAN_POINT('Ctrl Pts',(4.51134362,3.90342418,-5.991856083));
#124539=CARTESIAN_POINT('Ctrl Pts',(4.457029984,3.892857143,-6.031988372));
#124540=CARTESIAN_POINT('Ctrl Pts',(4.181306552,3.839213527,-6.235720132));
#124541=CARTESIAN_POINT('Ctrl Pts',(3.888146516,3.784676613,-6.41344811100001));
#124542=CARTESIAN_POINT('Ctrl Pts',(3.88462431992685,3.78402137462933,-6.41558343885118));
#124543=CARTESIAN_POINT('Ctrl Pts',(3.88110212385369,3.78336613625867,-6.41771876670236));
#124544=CARTESIAN_POINT('',(4.21789784165354,3.91326598485098,-5.89676502733377));
#124545=CARTESIAN_POINT('Ctrl Pts',(4.21789784484407,3.9132659850464,-5.89676502406029));
#124546=CARTESIAN_POINT('Ctrl Pts',(4.166721337,3.903042157,-5.93337107700001));
#124547=CARTESIAN_POINT('Ctrl Pts',(4.114917201,3.892857143,-5.969083383));
#124548=CARTESIAN_POINT('Ctrl Pts',(3.8420691693967,3.83921352754342,-6.15717709595602));
#124549=CARTESIAN_POINT('Ctrl Pts',(3.55319919982665,3.78467661280563,-6.3195945646125));
#124550=CARTESIAN_POINT('Ctrl Pts',(4.36152536588842,3.87435041321657,-6.10140118971835));
#124551=CARTESIAN_POINT('Ctrl Pts',(4.34499454697019,3.87860220111063,-6.07793460252609));
#124552=CARTESIAN_POINT('Ctrl Pts',(4.32848987505951,3.88292159125983,-6.05446171928498));
#124553=CARTESIAN_POINT('Ctrl Pts',(4.31201340060561,3.88731207458989,-6.03098245170927));
#124554=CARTESIAN_POINT('Ctrl Pts',(4.29630715704654,3.89149731462512,-6.00860077678455));
#124555=CARTESIAN_POINT('Ctrl Pts',(4.28063132748528,3.8957461849378,-5.98620953662333));
#124556=CARTESIAN_POINT('Ctrl Pts',(4.26494805633297,3.90006996192755,-5.963838092623));
#124557=CARTESIAN_POINT('Ctrl Pts',(4.24926435062234,3.90439385872224,-5.94146602874582));
#124558=CARTESIAN_POINT('Ctrl Pts',(4.23358081196648,3.90879118056435,-5.91910790639487));
#124559=CARTESIAN_POINT('Ctrl Pts',(4.21789784426514,3.91326598386267,-5.89676502585713));
#124560=CARTESIAN_POINT('Ctrl Pts',(4.83450107061284,3.78339966801642,-5.40279194947145));
#124561=CARTESIAN_POINT('Ctrl Pts',(4.83157723580641,3.78403814050821,-5.40540255423573));
#124562=CARTESIAN_POINT('Ctrl Pts',(4.828653401,3.784676613,-5.40801315900001));
#124563=CARTESIAN_POINT('Ctrl Pts',(4.534715986,3.848863192,-5.670461097));
#124564=CARTESIAN_POINT('Ctrl Pts',(4.214064918,3.914045302,-5.899504798));
#124565=CARTESIAN_POINT('Ctrl Pts',(4.81522106667948,3.78339966801642,-5.75010537695528));
#124566=CARTESIAN_POINT('Ctrl Pts',(4.81210946883974,3.78403814050821,-5.75270535497764));
#124567=CARTESIAN_POINT('Ctrl Pts',(4.808997871,3.784676613,-5.755305333));
#124568=CARTESIAN_POINT('Ctrl Pts',(4.496184362,3.848863192,-6.016684949));
#124569=CARTESIAN_POINT('Ctrl Pts',(4.156884187,3.914045302,-6.242620752));
#124570=CARTESIAN_POINT('Origin',(-0.0981910086943499,4.0177709938306,0.167112529190243));
#124571=CARTESIAN_POINT('Ctrl Pts',(5.39007353,3.914032935,-4.848670677));
#124572=CARTESIAN_POINT('Ctrl Pts',(5.346414803,3.90342418,-4.89720434));
#124573=CARTESIAN_POINT('Ctrl Pts',(5.301889206,3.892857143,-4.944943968));
#124574=CARTESIAN_POINT('Ctrl Pts',(5.075854798,3.839213527,-5.187294417));
#124575=CARTESIAN_POINT('Ctrl Pts',(4.828653401,3.784676613,-5.408013159));
#124576=CARTESIAN_POINT('Ctrl Pts',(4.82568337888624,3.78402137462933,-5.41066500301309));
#124577=CARTESIAN_POINT('Ctrl Pts',(4.82271335677248,3.78336613625867,-5.41331684702618));
#124578=CARTESIAN_POINT('Ctrl Pts',(5.737436191,3.914032935,-4.830302884));
#124579=CARTESIAN_POINT('Ctrl Pts',(5.693942853,3.90342418,-4.881964294));
#124580=CARTESIAN_POINT('Ctrl Pts',(5.649526295,3.892857143,-4.932834139));
#124581=CARTESIAN_POINT('Ctrl Pts',(5.42404543,3.839213527,-5.19107515));
#124582=CARTESIAN_POINT('Ctrl Pts',(5.175945575,3.784676613,-5.42766869));
#124583=CARTESIAN_POINT('Ctrl Pts',(5.17296475828653,3.78402137462933,-5.43051126311771));
#124584=CARTESIAN_POINT('Ctrl Pts',(5.16998394157306,3.78336613625867,-5.43335383623542));
#124585=CARTESIAN_POINT('',(5.38691590799243,3.9132659848901,-4.85217858241229));
#124586=CARTESIAN_POINT('Ctrl Pts',(5.38691591059486,3.91326598504639,-4.85217857849253));
#124587=CARTESIAN_POINT('Ctrl Pts',(5.3448051,3.903042157,-4.898930239));
#124588=CARTESIAN_POINT('Ctrl Pts',(5.301889206,3.892857143,-4.944943968));
#124589=CARTESIAN_POINT('Ctrl Pts',(5.07585479797788,3.83921352754011,-5.18729441661446));
#124590=CARTESIAN_POINT('Ctrl Pts',(4.82865340218875,3.78467661181152,-5.40801315812267));
#124591=CARTESIAN_POINT('Ctrl Pts',(5.57117622601867,3.87435041325356,-5.02115479276776));
#124592=CARTESIAN_POINT('Ctrl Pts',(5.54998726589277,3.87860220115474,-5.00179047883341));
#124593=CARTESIAN_POINT('Ctrl Pts',(5.52882248806047,3.88292159129895,-4.98241439514008));
#124594=CARTESIAN_POINT('Ctrl Pts',(5.50768387603071,3.88731207461873,-4.96302601472333));
#124595=CARTESIAN_POINT('Ctrl Pts',(5.48753343726377,3.89149731465094,-4.94454398894852));
#124596=CARTESIAN_POINT('Ctrl Pts',(5.46741064524587,3.89574618494883,-4.92604608339457));
#124597=CARTESIAN_POINT('Ctrl Pts',(5.44728484119411,3.90006996193012,-4.90756911091528));
#124598=CARTESIAN_POINT('Ctrl Pts',(5.42715847948854,3.90439385871635,-4.88909162646865));
#124599=CARTESIAN_POINT('Ctrl Pts',(5.40703527793493,3.90879118055703,-4.87062772170752));
#124600=CARTESIAN_POINT('Ctrl Pts',(5.3869159104284,3.91326598389117,-4.85217858048639));
#124601=CARTESIAN_POINT('Ctrl Pts',(5.88291368665964,3.78339966801642,-4.23720285334885));
#124602=CARTESIAN_POINT('Ctrl Pts',(5.88061941232982,3.78403814050821,-4.24038096167442));
#124603=CARTESIAN_POINT('Ctrl Pts',(5.878325138,3.784676613,-4.24355907));
#124604=CARTESIAN_POINT('Ctrl Pts',(5.64767836400001,3.848863192,-4.563058976));
#124605=CARTESIAN_POINT('Ctrl Pts',(5.383761566,3.914045302,-4.855678264));
#124606=CARTESIAN_POINT('Ctrl Pts',(5.93874655798517,3.78339966801642,-4.58054091591451));
#124607=CARTESIAN_POINT('Ctrl Pts',(5.93626662599258,3.78403814050821,-4.58374900945725));
#124608=CARTESIAN_POINT('Ctrl Pts',(5.933786694,3.784676613,-4.586957103));
#124609=CARTESIAN_POINT('Ctrl Pts',(5.684475482,3.848863192,-4.909471467));
#124610=CARTESIAN_POINT('Ctrl Pts',(5.401677476,3.914045302,-5.203064524));
#124611=CARTESIAN_POINT('Origin',(-0.131819659600271,4.01777116439499,0.142097461283107));
#124612=CARTESIAN_POINT('Ctrl Pts',(6.306377476,3.914032935,-3.576604972));
#124613=CARTESIAN_POINT('Ctrl Pts',(6.274172769,3.90342418,-3.633389281));
#124614=CARTESIAN_POINT('Ctrl Pts',(6.240950764,3.892857143,-3.68958447));
#124615=CARTESIAN_POINT('Ctrl Pts',(6.072299097,3.839213527,-3.974859616));
#124616=CARTESIAN_POINT('Ctrl Pts',(5.878325138,3.784676613,-4.24355907));
#124617=CARTESIAN_POINT('Ctrl Pts',(5.87599462144663,3.78402137462933,-4.24678738233974));
#124618=CARTESIAN_POINT('Ctrl Pts',(5.87366410489327,3.78336613625867,-4.25001569467947));
#124619=CARTESIAN_POINT('Ctrl Pts',(6.641670459,3.914032935,-3.483993903));
#124620=CARTESIAN_POINT('Ctrl Pts',(6.610299646,3.90342418,-3.54379728));
#124621=CARTESIAN_POINT('Ctrl Pts',(6.577857036,3.892857143,-3.603026063));
#124622=CARTESIAN_POINT('Ctrl Pts',(6.41316197200001,3.839213527,-3.903701264));
#124623=CARTESIAN_POINT('Ctrl Pts',(6.221723171,3.784676613,-4.188097513));
#124624=CARTESIAN_POINT('Ctrl Pts',(6.21942311331706,3.78402137462933,-4.19151441581224));
#124625=CARTESIAN_POINT('Ctrl Pts',(6.21712305563413,3.78336613625867,-4.1949313186245));
#124626=CARTESIAN_POINT('',(6.30404777322913,3.91326598495116,-3.58070966019294));
#124627=CARTESIAN_POINT('Ctrl Pts',(6.30404777308629,3.91326598539557,-3.58070966019485));
#124628=CARTESIAN_POINT('Ctrl Pts',(6.28331170433608,3.90644394844782,-3.61721671670234));
#124629=CARTESIAN_POINT('Ctrl Pts',(6.26227721073114,3.89964051892997,-3.65351067815672));
#124630=CARTESIAN_POINT('Ctrl Pts',(6.24095076432879,3.89285714298821,-3.68958446996868));
#124631=CARTESIAN_POINT('Ctrl Pts',(6.16580889148348,3.86895650882096,-3.81668732776632));
#124632=CARTESIAN_POINT('Ctrl Pts',(6.08652135128144,3.84480661539908,-3.94193107106089));
#124633=CARTESIAN_POINT('Ctrl Pts',(6.00324074906257,3.82047220032148,-4.06492318798607));
#124634=CARTESIAN_POINT('Ctrl Pts',(5.96254746592548,3.8085817094227,-4.12502065251343));
#124635=CARTESIAN_POINT('Ctrl Pts',(5.92090156723483,3.79664722485402,-4.18458072582146));
#124636=CARTESIAN_POINT('Ctrl Pts',(5.87832513995717,3.78467661302156,-4.24355906959005));
#124637=CARTESIAN_POINT('Ctrl Pts',(6.52032507810972,3.87435041328379,-3.70612477820758));
#124638=CARTESIAN_POINT('Ctrl Pts',(6.49546874906344,3.87860220115049,-3.69176819098134));
#124639=CARTESIAN_POINT('Ctrl Pts',(6.47063350665611,3.88292159130609,-3.67739491099258));
#124640=CARTESIAN_POINT('Ctrl Pts',(6.44582117486303,3.88731207464001,-3.6630039969133));
#124641=CARTESIAN_POINT('Ctrl Pts',(6.42216875293301,3.89149731467131,-3.64928581941188));
#124642=CARTESIAN_POINT('Ctrl Pts',(6.39853991765918,3.89574618498043,-3.63554619022822));
#124643=CARTESIAN_POINT('Ctrl Pts',(6.37491264077159,3.9000699619687,-3.6218276521987));
#124644=CARTESIAN_POINT('Ctrl Pts',(6.35128470921004,3.9043938587619,-3.60810873405048));
#124645=CARTESIAN_POINT('Ctrl Pts',(6.32766278316446,3.90879118060183,-3.59440239872993));
#124646=CARTESIAN_POINT('Ctrl Pts',(6.30404777520749,3.91326598385711,-3.58070965616348));
#124647=CARTESIAN_POINT('Ctrl Pts',(6.6562477962472,3.78339966801642,-2.87348685982246));
#124648=CARTESIAN_POINT('Ctrl Pts',(6.6546903601236,3.78403814050821,-2.87708386691123));
#124649=CARTESIAN_POINT('Ctrl Pts',(6.653132924,3.784676613,-2.880680874));
#124650=CARTESIAN_POINT('Ctrl Pts',(6.496561579,3.848863192,-3.242293289));
#124651=CARTESIAN_POINT('Ctrl Pts',(6.301719506,3.914045302,-3.58480561));
#124652=CARTESIAN_POINT('Ctrl Pts',(6.78458286054716,3.78339966801642,-3.19679545366646));
#124653=CARTESIAN_POINT('Ctrl Pts',(6.78285055327358,3.78403814050821,-3.20046165583323));
#124654=CARTESIAN_POINT('Ctrl Pts',(6.781118246,3.784676613,-3.204127858));
#124655=CARTESIAN_POINT('Ctrl Pts',(6.606966847,3.848863192,-3.572696556));
#124656=CARTESIAN_POINT('Ctrl Pts',(6.39389433,3.914045302,-3.920218782));
#124657=CARTESIAN_POINT('Origin',(-0.1592844565639,4.0177710357927,0.110437880897422));
#124658=CARTESIAN_POINT('Ctrl Pts',(6.927802221,3.914032935,-2.137301193));
#124659=CARTESIAN_POINT('Ctrl Pts',(6.90855739,3.90342418,-2.199680976));
#124660=CARTESIAN_POINT('Ctrl Pts',(6.888192401,3.892857143,-2.261704102));
#124661=CARTESIAN_POINT('Ctrl Pts',(6.78480944,3.839213527,-2.576564797));
#124662=CARTESIAN_POINT('Ctrl Pts',(6.653132924,3.784676613,-2.880680874));
#124663=CARTESIAN_POINT('Ctrl Pts',(6.65155088535002,3.78402137462933,-2.88433470235535));
#124664=CARTESIAN_POINT('Ctrl Pts',(6.64996884670004,3.78336613625867,-2.8879885307107));
#124665=CARTESIAN_POINT('Ctrl Pts',(7.235347597,3.914032935,-1.97477724));
#124666=CARTESIAN_POINT('Ctrl Pts',(7.217566175,3.90342418,-2.039926244));
#124667=CARTESIAN_POINT('Ctrl Pts',(7.198614493,3.892857143,-2.104744493));
#124668=CARTESIAN_POINT('Ctrl Pts',(7.102406188,3.839213527,-2.433794646));
#124669=CARTESIAN_POINT('Ctrl Pts',(6.976579907,3.784676613,-2.752695552));
#124670=CARTESIAN_POINT('Ctrl Pts',(6.97506815649374,3.78402137462933,-2.75652701393514));
#124671=CARTESIAN_POINT('Ctrl Pts',(6.97355640598748,3.78336613625867,-2.76035847587028));
#124672=CARTESIAN_POINT('',(6.92640937136214,3.91326598485584,-2.14181073245289));
#124673=CARTESIAN_POINT('Ctrl Pts',(6.92640937187168,3.9132659850464,-2.14181072785087));
#124674=CARTESIAN_POINT('Ctrl Pts',(6.907821148,3.903042157,-2.201923256));
#124675=CARTESIAN_POINT('Ctrl Pts',(6.888192401,3.892857143,-2.261704102));
#124676=CARTESIAN_POINT('Ctrl Pts',(6.78480944057515,3.83921352756187,-2.57656479577017));
#124677=CARTESIAN_POINT('Ctrl Pts',(6.65313292409509,3.78467661195603,-2.88068087233164));
#124678=CARTESIAN_POINT('Ctrl Pts',(7.16459077630807,3.87435041327016,-2.21780048805586));
#124679=CARTESIAN_POINT('Ctrl Pts',(7.1372293325444,3.87860220113624,-2.20912292591441));
#124680=CARTESIAN_POINT('Ctrl Pts',(7.10988489401252,3.88292159127784,-2.20042452820071));
#124681=CARTESIAN_POINT('Ctrl Pts',(7.08255903964796,3.88731207459879,-2.19170398356326));
#124682=CARTESIAN_POINT('Ctrl Pts',(7.05651059551731,3.89149731462703,-2.18339110094494));
#124683=CARTESIAN_POINT('Ctrl Pts',(7.03048057511907,3.89574618493553,-2.17505219774218));
#124684=CARTESIAN_POINT('Ctrl Pts',(7.00445661063303,3.90006996193304,-2.16673355763766));
#124685=CARTESIAN_POINT('Ctrl Pts',(6.97843192506453,3.90439385873549,-2.15841468703692));
#124686=CARTESIAN_POINT('Ctrl Pts',(6.95241580953439,3.9087911805915,-2.15010681410914));
#124687=CARTESIAN_POINT('Ctrl Pts',(6.92640937246644,3.9132659839127,-2.1418107295464));
#124688=CARTESIAN_POINT('Ctrl Pts',(7.11834315687191,3.78339966801642,-1.37540981543085));
#124689=CARTESIAN_POINT('Ctrl Pts',(7.11759538293595,3.78403814050821,-1.37925752921543));
#124690=CARTESIAN_POINT('Ctrl Pts',(7.116847609,3.784676613,-1.383105243));
#124691=CARTESIAN_POINT('Ctrl Pts',(7.041672795,3.848863192,-1.769921571));
#124692=CARTESIAN_POINT('Ctrl Pts',(6.925016046,3.914045302,-2.146311431));
#124693=CARTESIAN_POINT('Ctrl Pts',(7.31317960960073,3.78339966801642,-1.66357138748205));
#124694=CARTESIAN_POINT('Ctrl Pts',(7.31227592780037,3.78403814050821,-1.66752427074103));
#124695=CARTESIAN_POINT('Ctrl Pts',(7.311372246,3.784676613,-1.671477154));
#124696=CARTESIAN_POINT('Ctrl Pts',(7.220523785,3.848863192,-2.068866324));
#124697=CARTESIAN_POINT('Ctrl Pts',(7.087139791,3.914045302,-2.454067967));
#124698=CARTESIAN_POINT('Origin',(-0.179301663651004,4.01777114362114,0.073614573874817));
#124699=CARTESIAN_POINT('Ctrl Pts',(7.225290633,3.914032935,-0.598059586000001));
#124700=CARTESIAN_POINT('Ctrl Pts',(7.219905545,3.90342418,-0.663118034));
#124701=CARTESIAN_POINT('Ctrl Pts',(7.213349817,3.892857143,-0.728068964));
#124702=CARTESIAN_POINT('Ctrl Pts',(7.180069635,3.839213527,-1.057792671));
#124703=CARTESIAN_POINT('Ctrl Pts',(7.116847609,3.784676613,-1.383105243));
#124704=CARTESIAN_POINT('Ctrl Pts',(7.11608802261588,3.78402137462933,-1.38701373843915));
#124705=CARTESIAN_POINT('Ctrl Pts',(7.11532843623176,3.78336613625867,-1.39092223387829));
#124706=CARTESIAN_POINT('Ctrl Pts',(7.490707924,3.914032935,-0.373222187));
#124707=CARTESIAN_POINT('Ctrl Pts',(7.487347331,3.90342418,-0.440670524));
#124708=CARTESIAN_POINT('Ctrl Pts',(7.482772737,3.892857143,-0.50804741));
#124709=CARTESIAN_POINT('Ctrl Pts',(7.459549785,3.839213527,-0.850086495));
#124710=CARTESIAN_POINT('Ctrl Pts',(7.40521952,3.784676613,-1.188580606));
#124711=CARTESIAN_POINT('Ctrl Pts',(7.40456676443124,3.78402137462933,-1.19264747215549));
#124712=CARTESIAN_POINT('Ctrl Pts',(7.40391400886248,3.78336613625867,-1.19671433831097));
#124713=CARTESIAN_POINT('',(7.22489976603046,3.91326598469533,-0.602763115539841));
#124714=CARTESIAN_POINT('Ctrl Pts',(7.22489976555627,3.91326598504641,-0.60276311152549));
#124715=CARTESIAN_POINT('Ctrl Pts',(7.21966854000001,3.903042157,-0.665466161));
#124716=CARTESIAN_POINT('Ctrl Pts',(7.213349817,3.892857143,-0.728068964));
#124717=CARTESIAN_POINT('Ctrl Pts',(7.18006963483772,3.83921352756005,-1.0577926705533));
#124718=CARTESIAN_POINT('Ctrl Pts',(7.11684761074545,3.78467661272573,-1.38310524181887));
#124719=CARTESIAN_POINT('Ctrl Pts',(7.47384817275591,3.87435041323356,-0.625774312184501));
#124720=CARTESIAN_POINT('Ctrl Pts',(7.44526100500474,3.87860220111994,-0.623181528288914));
#124721=CARTESIAN_POINT('Ctrl Pts',(7.41668596593887,3.88292159125359,-0.620564740192355));
#124722=CARTESIAN_POINT('Ctrl Pts',(7.38812431561052,3.88731207456684,-0.617922327910737));
#124723=CARTESIAN_POINT('Ctrl Pts',(7.36089784559792,3.89149731459655,-0.615403441294617));
#124724=CARTESIAN_POINT('Ctrl Pts',(7.33368377491932,3.89574618490019,-0.612855181841101));
#124725=CARTESIAN_POINT('Ctrl Pts',(7.30647997453019,3.900069961904,-0.610325409987334));
#124726=CARTESIAN_POINT('Ctrl Pts',(7.27927542036719,3.90439385871277,-0.607795568037624));
#124727=CARTESIAN_POINT('Ctrl Pts',(7.25208160005011,3.90879118058398,-0.60527462440069));
#124728=CARTESIAN_POINT('Ctrl Pts',(7.22489976652122,3.91326598385759,-0.602763113096661));
#124729=CARTESIAN_POINT('Ctrl Pts',(7.24759270333537,3.78339966801643,0.18697986331215));
#124730=CARTESIAN_POINT('Ctrl Pts',(7.24768955666769,3.78403814050821,0.183061357656075));
#124731=CARTESIAN_POINT('Ctrl Pts',(7.24778641,3.784676613,0.179142852));
#124732=CARTESIAN_POINT('Ctrl Pts',(7.257523218,3.848863192,-0.214790287));
#124733=CARTESIAN_POINT('Ctrl Pts',(7.224506533,3.914045302,-0.607458115));
#124734=CARTESIAN_POINT('Ctrl Pts',(7.49982020834237,3.78339966801643,-0.0525605731549361));
#124735=CARTESIAN_POINT('Ctrl Pts',(7.49978740717118,3.78403814050821,-0.056615305077468));
#124736=CARTESIAN_POINT('Ctrl Pts',(7.499754606,3.784676613,-0.060670037));
#124737=CARTESIAN_POINT('Ctrl Pts',(7.496457056,3.848863192,-0.468298203));
#124738=CARTESIAN_POINT('Ctrl Pts',(7.448998472,3.914045302,-0.873167661));
#124739=CARTESIAN_POINT('Origin',(-0.190934635113679,4.01777094613612,0.0333488982646781));
#124740=CARTESIAN_POINT('Ctrl Pts',(7.184932486,3.914032935,0.969146623));
#124741=CARTESIAN_POINT('Ctrl Pts',(7.193658941,3.90342418,0.90445157));
#124742=CARTESIAN_POINT('Ctrl Pts',(7.201219013,3.892857143,0.839609869));
#124743=CARTESIAN_POINT('Ctrl Pts',(7.239597753,3.839213527,0.510440663));
#124744=CARTESIAN_POINT('Ctrl Pts',(7.24778641,3.784676613,0.179142852));
#124745=CARTESIAN_POINT('Ctrl Pts',(7.24788479331283,3.78402137462933,0.175162446400145));
#124746=CARTESIAN_POINT('Ctrl Pts',(7.24798317662565,3.78336613625867,0.17118204080029));
#124747=CARTESIAN_POINT('Ctrl Pts',(7.395811073,3.914032935,1.24578432));
#124748=CARTESIAN_POINT('Ctrl Pts',(7.407028448,3.90342418,1.17919046));
#124749=CARTESIAN_POINT('Ctrl Pts',(7.417044844,3.892857143,1.112405405));
#124750=CARTESIAN_POINT('Ctrl Pts',(7.46789312400001,3.839213527,0.773370756));
#124751=CARTESIAN_POINT('Ctrl Pts',(7.487599299,3.784676613,0.431111049));
#124752=CARTESIAN_POINT('Ctrl Pts',(7.48783606050798,3.78402137462933,0.426998940772556));
#124753=CARTESIAN_POINT('Ctrl Pts',(7.48807282201595,3.78336613625867,0.422886832545111));
#124754=CARTESIAN_POINT('',(7.1855618765768,3.91326598494572,0.964469033495719));
#124755=CARTESIAN_POINT('Ctrl Pts',(7.18556187701648,3.91326598546387,0.964469033469786));
#124756=CARTESIAN_POINT('Ctrl Pts',(7.19114716531835,3.90644394851566,0.922857084753342));
#124757=CARTESIAN_POINT('Ctrl Pts',(7.19636592023783,3.89964051897578,0.881234180225402));
#124758=CARTESIAN_POINT('Ctrl Pts',(7.20121901293983,3.89285714308741,0.839609869539318));
#124759=CARTESIAN_POINT('Ctrl Pts',(7.21831844637703,3.8689565293465,0.692950366790978));
#124760=CARTESIAN_POINT('Ctrl Pts',(7.23099246243938,3.84480665659152,0.545262042106412));
#124761=CARTESIAN_POINT('Ctrl Pts',(7.23912501119572,3.82047226237412,0.396949723893768));
#124762=CARTESIAN_POINT('Ctrl Pts',(7.24309881727761,3.808581750969,0.324479898038566));
#124763=CARTESIAN_POINT('Ctrl Pts',(7.24598903370267,3.79664724571288,0.251861386589163));
#124764=CARTESIAN_POINT('Ctrl Pts',(7.2477864112848,3.78467661306747,0.179142853770467));
#124765=CARTESIAN_POINT('Ctrl Pts',(7.43363673495892,3.87435041323103,0.99551237504792));
#124766=CARTESIAN_POINT('Ctrl Pts',(7.40516054742332,3.87860220113494,0.991899144976729));
#124767=CARTESIAN_POINT('Ctrl Pts',(7.37669104475964,3.88292159128888,0.988311965239462));
#124768=CARTESIAN_POINT('Ctrl Pts',(7.3482291093774,3.88731207462033,0.984752688798702));
#124769=CARTESIAN_POINT('Ctrl Pts',(7.32109769297024,3.89149731465741,0.981359798964424));
#124770=CARTESIAN_POINT('Ctrl Pts',(7.2939720717114,3.89574618495298,0.977998260824981));
#124771=CARTESIAN_POINT('Ctrl Pts',(7.26686045491279,3.90006996194473,0.97462087514303));
#124772=CARTESIAN_POINT('Ctrl Pts',(7.23974808689462,3.90439385874143,0.97124339587912));
#124773=CARTESIAN_POINT('Ctrl Pts',(7.21264811464817,3.90879118060208,0.967859533782324));
#124774=CARTESIAN_POINT('Ctrl Pts',(7.18556187633381,3.91326598387345,0.964469036847748));
#124775=CARTESIAN_POINT('Ctrl Pts',(7.03795286930082,3.78339966801642,1.74062657215132));
#124776=CARTESIAN_POINT('Ctrl Pts',(7.03888982115041,3.78403814050821,1.73682049957566));
#124777=CARTESIAN_POINT('Ctrl Pts',(7.039826773,3.784676613,1.733014427));
#124778=CARTESIAN_POINT('Ctrl Pts',(7.134019921,3.848863192,1.350384351));
#124779=CARTESIAN_POINT('Ctrl Pts',(7.186187123,3.914045302,0.959799268000001));
#124780=CARTESIAN_POINT('Ctrl Pts',(7.33577754858687,3.78339966801642,1.56090791565573));
#124781=CARTESIAN_POINT('Ctrl Pts',(7.33661716179344,3.78403814050821,1.55694092982786));
#124782=CARTESIAN_POINT('Ctrl Pts',(7.337456775,3.784676613,1.552973944));
#124783=CARTESIAN_POINT('Ctrl Pts',(7.421864326,3.848863192,1.154167022));
#124784=CARTESIAN_POINT('Ctrl Pts',(7.462550264,3.914045302,0.748560994));
#124785=CARTESIAN_POINT('Origin',(-0.19363957425676,4.01777115777898,-0.00847600782555386));
#124786=CARTESIAN_POINT('Ctrl Pts',(6.808614881,3.914032935,2.491036613));
#124787=CARTESIAN_POINT('Ctrl Pts',(6.83104484,3.90342418,2.429730024));
#124788=CARTESIAN_POINT('Ctrl Pts',(6.852367211,3.892857143,2.368029478));
#124789=CARTESIAN_POINT('Ctrl Pts',(6.96061032600001,3.839213527,2.05480636));
#124790=CARTESIAN_POINT('Ctrl Pts',(7.039826773,3.784676613,1.733014427));
#124791=CARTESIAN_POINT('Ctrl Pts',(7.04077852570941,3.78402137462933,1.7291482305762));
#124792=CARTESIAN_POINT('Ctrl Pts',(7.04173027841881,3.78336613625867,1.7252820341524));
#124793=CARTESIAN_POINT('Ctrl Pts',(6.955094316,3.914032935,2.806539337));
#124794=CARTESIAN_POINT('Ctrl Pts',(6.980365147,3.90342418,2.743913808));
#124795=CARTESIAN_POINT('Ctrl Pts',(7.004504177,3.892857143,2.68084338));
#124796=CARTESIAN_POINT('Ctrl Pts',(7.127046081,3.839213527,2.36066605));
#124797=CARTESIAN_POINT('Ctrl Pts',(7.219867256,3.784676613,2.030644429));
#124798=CARTESIAN_POINT('Ctrl Pts',(7.22098246386582,3.78402137462933,2.02667935629295));
#124799=CARTESIAN_POINT('Ctrl Pts',(7.22209767173163,3.78336613625867,2.0227142835859));
#124800=CARTESIAN_POINT('',(6.81023510037854,3.9132659847791,2.48660368285477));
#124801=CARTESIAN_POINT('Ctrl Pts',(6.81023510083825,3.91326598538396,2.486603682918));
#124802=CARTESIAN_POINT('Ctrl Pts',(6.85518854064161,3.89196924655433,2.36348655994546));
#124803=CARTESIAN_POINT('Ctrl Pts',(6.89678398055128,3.87079709579665,2.23921118101377));
#124804=CARTESIAN_POINT('Ctrl Pts',(6.95419025090827,3.83867884087599,2.0508687836617));
#124805=CARTESIAN_POINT('Ctrl Pts',(6.97250588636221,3.82792484728307,1.9877085761306));
#124806=CARTESIAN_POINT('Ctrl Pts',(6.99870059935963,3.81174904528243,1.89255770731536));
#124807=CARTESIAN_POINT('Ctrl Pts',(7.00722572817433,3.80634502483808,1.86074507440694));
#124808=CARTESIAN_POINT('Ctrl Pts',(7.01969082320505,3.79822878962379,1.81292921698448));
#124809=CARTESIAN_POINT('Ctrl Pts',(7.02379363232968,3.79552061310379,1.79696816810188));
#124810=CARTESIAN_POINT('Ctrl Pts',(7.0298668531405,3.791455923782,1.77300309738959));
#124811=CARTESIAN_POINT('Ctrl Pts',(7.03187813128029,3.79010036843707,1.76500932072657));
#124812=CARTESIAN_POINT('Ctrl Pts',(7.03578215795174,3.78745055935128,1.74938026706327));
#124813=CARTESIAN_POINT('Ctrl Pts',(7.03674478870647,3.78679841926599,1.7455340244289));
#124814=CARTESIAN_POINT('Ctrl Pts',(7.03982677379995,3.78467661301969,1.73301442848594));
#124815=CARTESIAN_POINT('Ctrl Pts',(7.04583670530855,3.87435041328414,2.57025001046774));
#124816=CARTESIAN_POINT('Ctrl Pts',(7.01880301281211,3.87860220114356,2.56059971734375));
#124817=CARTESIAN_POINT('Ctrl Pts',(6.99177024888423,3.88292159129812,2.55097630231711));
#124818=CARTESIAN_POINT('Ctrl Pts',(6.96473887695021,3.88731207463272,2.54138176494956));
#124819=CARTESIAN_POINT('Ctrl Pts',(6.93897114900317,3.89149731467151,2.53223574641716));
#124820=CARTESIAN_POINT('Ctrl Pts',(6.91320234107663,3.89574618498536,2.52312159228064));
#124821=CARTESIAN_POINT('Ctrl Pts',(6.88745061690712,3.90006996197851,2.51399497175813));
#124822=CARTESIAN_POINT('Ctrl Pts',(6.86169817919848,3.90439385877662,2.50486809835155));
#124823=CARTESIAN_POINT('Ctrl Pts',(6.83595921954747,3.90879118062751,2.49573765613441));
#124824=CARTESIAN_POINT('Ctrl Pts',(6.81023509907772,3.91326598391623,2.48660368644794));
#124825=CARTESIAN_POINT('Ctrl Pts',(6.49922618194218,3.78339966801642,3.21288351652541));
#124826=CARTESIAN_POINT('Ctrl Pts',(6.50095942147108,3.78403814050821,3.20936784476271));
#124827=CARTESIAN_POINT('Ctrl Pts',(6.502692661,3.784676613,3.205852173));
#124828=CARTESIAN_POINT('Ctrl Pts',(6.676937781,3.848863192,2.852416518));
#124829=CARTESIAN_POINT('Ctrl Pts',(6.81184959,3.914045302,2.482177504));
#124830=CARTESIAN_POINT('Ctrl Pts',(6.8287220845867,3.78339966801642,3.10139008475842));
#124831=CARTESIAN_POINT('Ctrl Pts',(6.83039485279335,3.78403814050821,3.09769633687921));
#124832=CARTESIAN_POINT('Ctrl Pts',(6.832067621,3.784676613,3.094002589));
#124833=CARTESIAN_POINT('Ctrl Pts',(7.00023347,3.848863192,2.72266468));
#124834=CARTESIAN_POINT('Ctrl Pts',(7.127161499,3.914045302,2.33528777));
#124835=CARTESIAN_POINT('Origin',(-0.187290317839145,4.01777099682798,-0.0499046783036339));
#124836=CARTESIAN_POINT('Ctrl Pts',(6.113934011,3.914032935,3.896448499));
#124837=CARTESIAN_POINT('Ctrl Pts',(6.149018675,3.90342418,3.841397003));
#124838=CARTESIAN_POINT('Ctrl Pts',(6.183106334,3.892857143,3.785722661));
#124839=CARTESIAN_POINT('Ctrl Pts',(6.356152497,3.839213527,3.503091595));
#124840=CARTESIAN_POINT('Ctrl Pts',(6.502692661,3.784676613,3.205852173));
#124841=CARTESIAN_POINT('Ctrl Pts',(6.50445328020732,3.78402137462933,3.20228096479837));
#124842=CARTESIAN_POINT('Ctrl Pts',(6.50621389941464,3.78336613625867,3.19870975659674));
#124843=CARTESIAN_POINT('Ctrl Pts',(6.18916508000001,3.914032935,4.236063694));
#124844=CARTESIAN_POINT('Ctrl Pts',(6.22730773,3.90342418,4.180334797));
#124845=CARTESIAN_POINT('Ctrl Pts',(6.264440681,3.892857143,4.123928098));
#124846=CARTESIAN_POINT('Ctrl Pts',(6.452946284,3.839213527,3.837579223));
#124847=CARTESIAN_POINT('Ctrl Pts',(6.614542245,3.784676613,3.535227133));
#124848=CARTESIAN_POINT('Ctrl Pts',(6.61648375335509,3.78402137462933,3.53159449821582));
#124849=CARTESIAN_POINT('Ctrl Pts',(6.61842526171017,3.78336613625867,3.52796186343163));
#124850=CARTESIAN_POINT('',(6.11646929938807,3.91326598466575,3.89246750905316));
#124851=CARTESIAN_POINT('Ctrl Pts',(6.11646929645235,3.91326598504639,3.8924675123496));
#124852=CARTESIAN_POINT('Ctrl Pts',(6.150251023,3.903042157,3.839384247));
#124853=CARTESIAN_POINT('Ctrl Pts',(6.183106334,3.892857143,3.785722661));
#124854=CARTESIAN_POINT('Ctrl Pts',(6.35615249632147,3.83921352755049,3.50309159634728));
#124855=CARTESIAN_POINT('Ctrl Pts',(6.50269266136571,3.78467661279065,3.20585217521131));
#124856=CARTESIAN_POINT('Ctrl Pts',(6.32858118267264,3.87435041327332,4.02480561173716));
#124857=CARTESIAN_POINT('Ctrl Pts',(6.30425405066542,3.87860220115422,4.0095694921564));
#124858=CARTESIAN_POINT('Ctrl Pts',(6.2799220475138,3.88292159129824,3.99435982204413));
#124859=CARTESIAN_POINT('Ctrl Pts',(6.25558519594437,3.88731207462102,3.97917865369964));
#124860=CARTESIAN_POINT('Ctrl Pts',(6.23238602679852,3.89149731464463,3.96470716418707));
#124861=CARTESIAN_POINT('Ctrl Pts',(6.20917895297857,3.89574618493737,3.95026656197386));
#124862=CARTESIAN_POINT('Ctrl Pts',(6.18599124343745,3.90006996191926,3.93581745729566));
#124863=CARTESIAN_POINT('Ctrl Pts',(6.162802891402,3.90439385870609,3.92136795225589));
#124864=CARTESIAN_POINT('Ctrl Pts',(6.13962846950894,3.90879118055024,3.90691785921443));
#124865=CARTESIAN_POINT('Ctrl Pts',(6.1164692969636,3.91326598372466,3.89246751191928));
#124866=CARTESIAN_POINT('Ctrl Pts',(5.65660290128854,3.78339966801643,4.53490959909924));
#124867=CARTESIAN_POINT('Ctrl Pts',(5.65905138414427,3.78403814050821,4.53184871704962));
#124868=CARTESIAN_POINT('Ctrl Pts',(5.661499867,3.784676613,4.528787835));
#124869=CARTESIAN_POINT('Ctrl Pts',(5.907649451,3.848863192,4.221072859));
#124870=CARTESIAN_POINT('Ctrl Pts',(6.118997541,3.914045302,3.888491878));
#124871=CARTESIAN_POINT('Ctrl Pts',(6.00236316514701,3.78339966801643,4.49685470076832));
#124872=CARTESIAN_POINT('Ctrl Pts',(6.00479087157351,3.78403814050821,4.49360690638416));
#124873=CARTESIAN_POINT('Ctrl Pts',(6.007218578,3.784676613,4.490359112));
#124874=CARTESIAN_POINT('Ctrl Pts',(6.251279477,3.848863192,4.163853564));
#124875=CARTESIAN_POINT('Ctrl Pts',(6.458514584,3.914045302,3.812819084));
#124876=CARTESIAN_POINT('Origin',(-0.172183610538041,4.01777098821472,-0.0889998762653649));
#124877=CARTESIAN_POINT('Ctrl Pts',(5.133372382,3.914032935,5.119666785));
#124878=CARTESIAN_POINT('Ctrl Pts',(5.179471231,3.90342418,5.073444527));
#124879=CARTESIAN_POINT('Ctrl Pts',(5.224730277,3.892857143,5.026399659));
#124880=CARTESIAN_POINT('Ctrl Pts',(5.454488042,3.839213527,4.787576161));
#124881=CARTESIAN_POINT('Ctrl Pts',(5.661499867,3.784676613,4.528787835));
#124882=CARTESIAN_POINT('Ctrl Pts',(5.66398702809829,3.78402137462934,4.52567860074675));
#124883=CARTESIAN_POINT('Ctrl Pts',(5.66647418919657,3.78336613625867,4.5225693664935));
#124884=CARTESIAN_POINT('Ctrl Pts',(5.13383736200001,3.914032935,5.46751442));
#124885=CARTESIAN_POINT('Ctrl Pts',(5.18306832399999,3.90342418,5.421287976));
#124886=CARTESIAN_POINT('Ctrl Pts',(5.2314589,3.892857143,5.374182522));
#124887=CARTESIAN_POINT('Ctrl Pts',(5.477113891,3.839213527,5.135051457));
#124888=CARTESIAN_POINT('Ctrl Pts',(5.69992859,3.784676613,4.874506546));
#124889=CARTESIAN_POINT('Ctrl Pts',(5.70260561606593,3.78402137462934,4.87137620710754));
#124890=CARTESIAN_POINT('Ctrl Pts',(5.70528264213184,3.78336613625867,4.86824586821509));
#124891=CARTESIAN_POINT('',(5.13670419225033,3.91326598486893,5.11632387946452));
#124892=CARTESIAN_POINT('Ctrl Pts',(5.13670418872993,3.91326598504639,5.11632388223311));
#124893=CARTESIAN_POINT('Ctrl Pts',(5.18110745,3.903042157,5.071743746));
#124894=CARTESIAN_POINT('Ctrl Pts',(5.224730277,3.892857143,5.026399659));
#124895=CARTESIAN_POINT('Ctrl Pts',(5.45448804055648,3.83921352755582,4.78757616143772));
#124896=CARTESIAN_POINT('Ctrl Pts',(5.66149986570685,3.7846766119556,4.52878783597895));
#124897=CARTESIAN_POINT('Ctrl Pts',(5.31540823715458,3.87435041321081,5.2911657759504));
#124898=CARTESIAN_POINT('Ctrl Pts',(5.29492517538631,3.87860220111821,5.27105625408227));
#124899=CARTESIAN_POINT('Ctrl Pts',(5.2744316704039,3.88292159127204,5.25097151622122));
#124900=CARTESIAN_POINT('Ctrl Pts',(5.2539273033291,3.88731207460207,5.23091357150108));
#124901=CARTESIAN_POINT('Ctrl Pts',(5.23438146031949,3.89149731463373,5.21179328180058));
#124902=CARTESIAN_POINT('Ctrl Pts',(5.2148212576476,3.89574618494381,5.19270145794553));
#124903=CARTESIAN_POINT('Ctrl Pts',(5.19528179427941,3.90006996193226,5.17360549318181));
#124904=CARTESIAN_POINT('Ctrl Pts',(5.17574178950408,3.90439385872563,5.15450899929958));
#124905=CARTESIAN_POINT('Ctrl Pts',(5.15621551555658,3.90879118056291,5.13541492577162));
#124906=CARTESIAN_POINT('Ctrl Pts',(5.13670419026838,3.91326598375979,5.11632388192909));
#124907=CARTESIAN_POINT('Ctrl Pts',(4.54948315630955,3.78339966801642,5.64488834877326));
#124908=CARTESIAN_POINT('Ctrl Pts',(4.55253239415478,3.78403814050821,5.64242537988663));
#124909=CARTESIAN_POINT('Ctrl Pts',(4.555581632,3.784676613,5.639962411));
#124910=CARTESIAN_POINT('Ctrl Pts',(4.862125999,3.848863192,5.392356525));
#124911=CARTESIAN_POINT('Ctrl Pts',(5.140027969,3.914045302,5.112984694));
#124912=CARTESIAN_POINT('Ctrl Pts',(4.89534041542821,3.78339966801642,5.68205138827747));
#124913=CARTESIAN_POINT('Ctrl Pts',(4.8984095432141,3.78403814050821,5.67940141063874));
#124914=CARTESIAN_POINT('Ctrl Pts',(4.901478671,3.784676613,5.676751433));
#124915=CARTESIAN_POINT('Ctrl Pts',(5.210022603,3.848863192,5.410345282));
#124916=CARTESIAN_POINT('Ctrl Pts',(5.487874705,3.914045302,5.11206721600001));
#124917=CARTESIAN_POINT('Origin',(-0.149025773014475,4.01777117436562,-0.123933495488204));
#124918=CARTESIAN_POINT('Ctrl Pts',(3.912779966,3.914032935,6.103495141));
#124919=CARTESIAN_POINT('Ctrl Pts',(3.967737468,3.90342418,6.068263424));
#124920=CARTESIAN_POINT('Ctrl Pts',(4.022051639,3.892857143,6.032047796));
#124921=CARTESIAN_POINT('Ctrl Pts',(4.297777787,3.839213527,5.848198986));
#124922=CARTESIAN_POINT('Ctrl Pts',(4.555581632,3.784676613,5.639962411));
#124923=CARTESIAN_POINT('Ctrl Pts',(4.55867903812293,3.78402137462933,5.63746053503914));
#124924=CARTESIAN_POINT('Ctrl Pts',(4.56177644424584,3.78336613625867,5.63495865907829));
#124925=CARTESIAN_POINT('Ctrl Pts',(3.838457116,3.914032935,6.44331024900001));
#124926=CARTESIAN_POINT('Ctrl Pts',(3.896474404,3.90342418,6.408747755));
#124927=CARTESIAN_POINT('Ctrl Pts',(3.953859916,3.892857143,6.373146144));
#124928=CARTESIAN_POINT('Ctrl Pts',(4.24517774,3.839213527,6.192414392));
#124929=CARTESIAN_POINT('Ctrl Pts',(4.518792609,3.784676613,5.98585945));
#124930=CARTESIAN_POINT('Ctrl Pts',(4.52207997800942,3.78402137462933,5.9833777781612));
#124931=CARTESIAN_POINT('Ctrl Pts',(4.52536734701884,3.78336613625867,5.9808961063224));
#124932=CARTESIAN_POINT('',(3.91675250608448,3.91326598469296,6.10094663184978));
#124933=CARTESIAN_POINT('Ctrl Pts',(3.91675250213917,3.91326598504639,6.10094663341301));
#124934=CARTESIAN_POINT('Ctrl Pts',(3.969701051,3.903042157,6.06695414500001));
#124935=CARTESIAN_POINT('Ctrl Pts',(4.022051639,3.892857143,6.032047796));
#124936=CARTESIAN_POINT('Ctrl Pts',(4.29777778699874,3.83921352751727,5.84819898632377));
#124937=CARTESIAN_POINT('Ctrl Pts',(4.55558163184143,3.78467661273374,5.63996241260665));
#124938=CARTESIAN_POINT('Ctrl Pts',(4.05369271047263,3.87435041321389,6.31011690926935));
#124939=CARTESIAN_POINT('Ctrl Pts',(4.03801148411031,3.87860220114895,6.28607428389986));
#124940=CARTESIAN_POINT('Ctrl Pts',(4.02231473078001,3.88292159129884,6.2620536182469));
#124941=CARTESIAN_POINT('Ctrl Pts',(4.0066016095796,3.88731207462764,6.23805678428031));
#124942=CARTESIAN_POINT('Ctrl Pts',(3.99162303459158,3.89149731465319,6.21518173784877));
#124943=CARTESIAN_POINT('Ctrl Pts',(3.97662431624531,3.89574618493986,6.19233140489362));
#124944=CARTESIAN_POINT('Ctrl Pts',(3.96164674257626,3.90006996191702,6.16948148613298));
#124945=CARTESIAN_POINT('Ctrl Pts',(3.94666875390264,3.90439385869913,6.14663093423767));
#124946=CARTESIAN_POINT('Ctrl Pts',(3.93170365482692,3.90879118054072,6.12378569777082));
#124947=CARTESIAN_POINT('Ctrl Pts',(3.91675250287682,3.91326598379626,6.10094663327454));
#124948=CARTESIAN_POINT('Ctrl Pts',(3.22963463525794,3.78339966801642,6.49091839309238));
#124949=CARTESIAN_POINT('Ctrl Pts',(3.23314204912897,3.78403814050821,6.48916850304618));
#124950=CARTESIAN_POINT('Ctrl Pts',(3.236649463,3.784676613,6.487418613));
#124951=CARTESIAN_POINT('Ctrl Pts',(3.58925494,3.848863192,6.311499592));
#124952=CARTESIAN_POINT('Ctrl Pts',(3.9207164,3.914045302,6.098400028));
#124953=CARTESIAN_POINT('Ctrl Pts',(3.55941698871103,3.78339966801642,6.6015616687789));
#124954=CARTESIAN_POINT('Ctrl Pts',(3.56298402885552,3.78403814050821,6.59963341788945));
#124955=CARTESIAN_POINT('Ctrl Pts',(3.566551069,3.784676613,6.59770516700001));
#124956=CARTESIAN_POINT('Ctrl Pts',(3.925150863,3.848863192,6.403855268));
#124957=CARTESIAN_POINT('Ctrl Pts',(4.260627904,3.914045302,6.172280767));
#124958=CARTESIAN_POINT('Origin',(-0.118899507874863,4.0177710088603,-0.153072028990134));
#124959=CARTESIAN_POINT('Ctrl Pts',(2.509230308,3.914032935,6.801930848));
#124960=CARTESIAN_POINT('Ctrl Pts',(2.570476711,3.90342418,6.779337068));
#124961=CARTESIAN_POINT('Ctrl Pts',(2.631306337,3.892857143,6.755644082));
#124962=CARTESIAN_POINT('Ctrl Pts',(2.940108221,3.839213527,6.635366527));
#124963=CARTESIAN_POINT('Ctrl Pts',(3.236649463,3.784676613,6.487418613));
#124964=CARTESIAN_POINT('Ctrl Pts',(3.24021228285891,3.78402137462934,6.48564108026112));
#124965=CARTESIAN_POINT('Ctrl Pts',(3.24377510271782,3.78336613625867,6.48386354752224));
#124966=CARTESIAN_POINT('Ctrl Pts',(2.363594881,3.914032935,7.117824052));
#124967=CARTESIAN_POINT('Ctrl Pts',(2.427685672,3.90342418,7.096541612));
#124968=CARTESIAN_POINT('Ctrl Pts',(2.491382836,3.892857143,7.074108535));
#124969=CARTESIAN_POINT('Ctrl Pts',(2.814741796,3.839213527,6.960226912));
#124970=CARTESIAN_POINT('Ctrl Pts',(3.126362908,3.784676613,6.81732021899999));
#124971=CARTESIAN_POINT('Ctrl Pts',(3.13010690623377,3.78402137462934,6.81560325443765));
#124972=CARTESIAN_POINT('Ctrl Pts',(3.13385090446755,3.78336613625867,6.81388628987528));
#124973=CARTESIAN_POINT('',(2.51365782730426,3.91326598478301,6.80029589995261));
#124974=CARTESIAN_POINT('Ctrl Pts',(2.51365782739205,3.91326598534454,6.80029589992694));
#124975=CARTESIAN_POINT('Ctrl Pts',(2.55303868075648,3.90644394844332,6.78573918197759));
#124976=CARTESIAN_POINT('Ctrl Pts',(2.59225752687014,3.89964051893982,6.77085349511628));
#124977=CARTESIAN_POINT('Ctrl Pts',(2.63130633659125,3.89285714306086,6.75564408226938));
#124978=CARTESIAN_POINT('Ctrl Pts',(2.76889106306463,3.86895656917362,6.70205517870409));
#124979=CARTESIAN_POINT('Ctrl Pts',(2.90531186822816,3.84480673693962,6.64407447046975));
#124980=CARTESIAN_POINT('Ctrl Pts',(3.0401567232433,3.82047238378624,6.58178905128594));
#124981=CARTESIAN_POINT('Ctrl Pts',(3.10604627856664,3.80858183217285,6.55135438195659));
#124982=CARTESIAN_POINT('Ctrl Pts',(3.17155963440329,3.79664728639182,6.51989269544317));
#124983=CARTESIAN_POINT('Ctrl Pts',(3.23664946230039,3.78467661300963,6.48741861496226));
#124984=CARTESIAN_POINT('Ctrl Pts',(2.60243101783683,3.87435041322623,7.03401398873241));
#124985=CARTESIAN_POINT('Ctrl Pts',(2.59228486354879,3.87860220112027,7.00716246659475));
#124986=CARTESIAN_POINT('Ctrl Pts',(2.58211882471485,3.8829215912644,6.98032905281386));
#124987=CARTESIAN_POINT('Ctrl Pts',(2.57193167755894,3.88731207458757,6.95351539495929));
#124988=CARTESIAN_POINT('Ctrl Pts',(2.56222075215247,3.89149731461572,6.92795520354208));
#124989=CARTESIAN_POINT('Ctrl Pts',(2.55248484170893,3.89574618491529,6.90241481758498));
#124990=CARTESIAN_POINT('Ctrl Pts',(2.54276949248602,3.90006996190096,6.87687938164382));
#124991=CARTESIAN_POINT('Ctrl Pts',(2.5330538740663,3.90439385869159,6.85134323815647));
#124992=CARTESIAN_POINT('Ctrl Pts',(2.52334970118558,3.90879118054061,6.82581505672652));
#124993=CARTESIAN_POINT('Ctrl Pts',(2.5136578228534,3.91326598381907,6.80029590129335));
#124994=CARTESIAN_POINT('Ctrl Pts',(1.75877198777081,3.78339966801642,7.03344030656226));
#124995=CARTESIAN_POINT('Ctrl Pts',(1.76257357488541,3.78403814050821,7.03248531828113));
#124996=CARTESIAN_POINT('Ctrl Pts',(1.766375162,3.784676613,7.03153033));
#124997=CARTESIAN_POINT('Ctrl Pts',(2.148554308,3.848863192,6.93552395300001));
#124998=CARTESIAN_POINT('Ctrl Pts',(2.518076491,3.914045302,6.798660955));
#124999=CARTESIAN_POINT('Ctrl Pts',(2.05705917966293,3.78339966801642,7.21239026252005));
#125000=CARTESIAN_POINT('Ctrl Pts',(2.06095734133146,3.78403814050821,7.21127390126003));
#125001=CARTESIAN_POINT('Ctrl Pts',(2.064855503,3.784676613,7.21015754));
#125002=CARTESIAN_POINT('Ctrl Pts',(2.456743431,3.848863192,7.0979281));
#125003=CARTESIAN_POINT('Ctrl Pts',(2.834158878,3.914045302,6.94388532800001));
#125004=CARTESIAN_POINT('Origin',(-0.0832137526056376,4.017770990989,-0.175053254770167));
#125005=CARTESIAN_POINT('Ctrl Pts',(0.988351829,3.914032935,7.182315829));
#125006=CARTESIAN_POINT('Ctrl Pts',(1.053023321,3.90342418,7.173416445));
#125007=CARTESIAN_POINT('Ctrl Pts',(1.117524075,3.892857143,7.163353959));
#125008=CARTESIAN_POINT('Ctrl Pts',(1.444962461,3.839213527,7.112271703));
#125009=CARTESIAN_POINT('Ctrl Pts',(1.766375162,3.784676613,7.03153033));
#125010=CARTESIAN_POINT('Ctrl Pts',(1.77023680210883,3.78402137462933,7.03056025593805));
#125011=CARTESIAN_POINT('Ctrl Pts',(1.77409844221766,3.78336613625867,7.02959018187611));
#125012=CARTESIAN_POINT('Ctrl Pts',(0.778213576,3.914032935,7.45951631300001));
#125013=CARTESIAN_POINT('Ctrl Pts',(0.845381055,3.90342418,7.45250907));
#125014=CARTESIAN_POINT('Ctrl Pts',(0.912411464,3.892857143,7.444293474));
#125015=CARTESIAN_POINT('Ctrl Pts',(1.252691653,3.839213527,7.402586957));
#125016=CARTESIAN_POINT('Ctrl Pts',(1.587747952,3.784676613,7.330010671));
#125017=CARTESIAN_POINT('Ctrl Pts',(1.59177351427215,3.78402137462933,7.32913869706712));
#125018=CARTESIAN_POINT('Ctrl Pts',(1.59579907654429,3.78336613625867,7.32826672313425));
#125019=CARTESIAN_POINT('',(0.993027300813708,3.91326598477827,7.18167089038567));
#125020=CARTESIAN_POINT('Ctrl Pts',(0.993027300977299,3.91326598535293,
7.18167089088704));
#125021=CARTESIAN_POINT('Ctrl Pts',(1.03461671607111,3.9064439485324,7.17592022021272));
#125022=CARTESIAN_POINT('Ctrl Pts',(1.07611863008281,3.89964051902724,7.16981344487701));
#125023=CARTESIAN_POINT('Ctrl Pts',(1.11752407430451,3.89285714307317,7.16335395941058));
#125024=CARTESIAN_POINT('Ctrl Pts',(1.26341255565324,3.86895650694317,7.14059452521847));
#125025=CARTESIAN_POINT('Ctrl Pts',(1.40910843260399,3.84480661167109,7.1132957314019));
#125026=CARTESIAN_POINT('Ctrl Pts',(1.5541905854932,3.82047219473368,7.0814540622888));
#125027=CARTESIAN_POINT('Ctrl Pts',(1.62508185668359,3.80858170568305,7.06589531605229));
#125028=CARTESIAN_POINT('Ctrl Pts',(1.69582650333231,3.79664722298046,7.04925270345853));
#125029=CARTESIAN_POINT('Ctrl Pts',(1.76637516097775,3.78467661301146,7.03153033161224));
#125030=CARTESIAN_POINT('Ctrl Pts',(1.02948254308918,3.87435041323043,7.42900839219754));
#125031=CARTESIAN_POINT('Ctrl Pts',(1.02534588378698,3.87860220113284,7.40060352041932));
#125032=CARTESIAN_POINT('Ctrl Pts',(1.0211859121115,3.88292159128409,7.3722120590852));
#125033=CARTESIAN_POINT('Ctrl Pts',(1.01700107867272,3.88731207461403,7.34383535412217));
#125034=CARTESIAN_POINT('Ctrl Pts',(1.01301187494508,3.89149731465338,7.31678518381723));
#125035=CARTESIAN_POINT('Ctrl Pts',(1.00899401265604,3.89574618495283,7.28974898488849));
#125036=CARTESIAN_POINT('Ctrl Pts',(1.00499516686957,3.90006996195267,7.26272204028935));
#125037=CARTESIAN_POINT('Ctrl Pts',(1.00099621028148,3.90439385875746,7.23569434681681));
#125038=CARTESIAN_POINT('Ctrl Pts',(0.99700672008525,3.90879118062775,7.208676889702));
#125039=CARTESIAN_POINT('Ctrl Pts',(0.993027296840861,3.91326598383751,
7.18167089110787));
#125040=CARTESIAN_POINT('Ctrl Pts',(0.205671117258216,3.78339966801642,
7.24708636966053));
#125041=CARTESIAN_POINT('Ctrl Pts',(0.209589119629108,3.78403814050821,
7.24697093733027));
#125042=CARTESIAN_POINT('Ctrl Pts',(0.213507122,3.784676613,7.246855505));
#125043=CARTESIAN_POINT('Ctrl Pts',(0.607389665,3.848863192,7.235250923));
#125044=CARTESIAN_POINT('Ctrl Pts',(0.997694124,3.914045302,7.181024052));
#125045=CARTESIAN_POINT('Ctrl Pts',(0.458515569029854,3.78339966801642,
7.48597550365515));
#125046=CARTESIAN_POINT('Ctrl Pts',(0.462562578514927,3.78403814050821,
7.48572323182757));
#125047=CARTESIAN_POINT('Ctrl Pts',(0.466609588,3.784676613,7.48547096));
#125048=CARTESIAN_POINT('Ctrl Pts',(0.873461406,3.848863192,7.460109702));
#125049=CARTESIAN_POINT('Ctrl Pts',(1.275167733,3.914045302,7.39080153));
#125050=CARTESIAN_POINT('Origin',(-0.0436369827697361,4.01777097706205,
-0.18884908381595));
#125051=CARTESIAN_POINT('Ctrl Pts',(-0.578740883,3.914032935,7.226863704));
#125052=CARTESIAN_POINT('Ctrl Pts',(-0.51366827,3.90342418,7.232074841));
#125053=CARTESIAN_POINT('Ctrl Pts',(-0.448512371,3.892857143,7.236113367));
#125054=CARTESIAN_POINT('Ctrl Pts',(-0.117748137,3.839213527,7.25661495900001));
#125055=CARTESIAN_POINT('Ctrl Pts',(0.213507122,3.784676613,7.246855505));
#125056=CARTESIAN_POINT('Ctrl Pts',(0.217487016355248,3.78402137462933,
7.24673824921362));
#125057=CARTESIAN_POINT('Ctrl Pts',(0.221466910710496,3.78336613625867,
7.24662099342725));
#125058=CARTESIAN_POINT('Ctrl Pts',(-0.84355613,3.914032935,7.452409882));
#125059=CARTESIAN_POINT('Ctrl Pts',(-0.776452639,3.90342418,7.460005487));
#125060=CARTESIAN_POINT('Ctrl Pts',(-0.709223254,3.892857143,7.466391523));
#125061=CARTESIAN_POINT('Ctrl Pts',(-0.367932958,3.839213527,7.498810264));
#125062=CARTESIAN_POINT('Ctrl Pts',(-0.025108333,3.784676613,7.499957971));
#125063=CARTESIAN_POINT('Ctrl Pts',(-0.0209894375174155,3.78402137462933,
7.49997176022292));
#125064=CARTESIAN_POINT('Ctrl Pts',(-0.016870542034831,3.78336613625867,
7.49998554944585));
#125065=CARTESIAN_POINT('Ctrl Pts',(-0.574036075078507,3.91326598479031,
7.22723893284684));
#125066=CARTESIAN_POINT('Ctrl Pts',(-0.443380136338622,3.89196922700598,
7.23761650894715));
#125067=CARTESIAN_POINT('Ctrl Pts',(-0.312506527981107,3.87079705839004,
7.24444860561573));
#125068=CARTESIAN_POINT('Ctrl Pts',(-0.115671644510548,3.8386788420296,
7.24937548238318));
#125069=CARTESIAN_POINT('Ctrl Pts',(-0.0499136823355695,3.82792484954096,
7.2501263677632));
#125070=CARTESIAN_POINT('Ctrl Pts',(0.0487767784342727,3.81174904529917,
7.24991072932808));
#125071=CARTESIAN_POINT('Ctrl Pts',(0.0817105542309791,3.80634502485406,
7.24961433627786));
#125072=CARTESIAN_POINT('Ctrl Pts',(0.131118289538351,3.79822878963818,
7.24883298155762));
#125073=CARTESIAN_POINT('Ctrl Pts',(0.147595175806614,3.7955206131177,7.2485162103515));
#125074=CARTESIAN_POINT('Ctrl Pts',(0.172311478230664,3.79145592379503,
7.24795672663783));
#125075=CARTESIAN_POINT('Ctrl Pts',(0.180551955589269,3.79010036844976,
7.24775613187476));
#125076=CARTESIAN_POINT('Ctrl Pts',(0.196655767919899,3.78745055936495,
7.24733664196481));
#125077=CARTESIAN_POINT('Ctrl Pts',(0.200619346131265,3.78679841925717,
7.24723520591059));
#125078=CARTESIAN_POINT('Ctrl Pts',(0.213507120912194,3.78467661303892,
7.24685550591003));
#125079=CARTESIAN_POINT('Ctrl Pts',(0.178767433842035,1.96978752941321,
7.24784744327216));
#125080=CARTESIAN_POINT('Ctrl Pts',(0.192458160921018,1.97205380720657,
7.24745799913609));
#125081=CARTESIAN_POINT('Ctrl Pts',(0.206148888,1.974320085,7.247068555));
#125082=CARTESIAN_POINT('Ctrl Pts',(0.603261147,2.040055578,7.23577236600001));
#125083=CARTESIAN_POINT('Ctrl Pts',(0.99676151,2.104802836,7.181153563));
#125084=CARTESIAN_POINT('Ctrl Pts',(0.431246454094205,1.96978752941321,
7.48817152332989));
#125085=CARTESIAN_POINT('Ctrl Pts',(0.445389378432169,1.97205380720657,
7.48730340247219));
#125086=CARTESIAN_POINT('Ctrl Pts',(0.459532302770134,1.974320085,7.48643528161457));
#125087=CARTESIAN_POINT('Ctrl Pts',(0.869760963404042,2.040055578,7.46125462956701));
#125088=CARTESIAN_POINT('Ctrl Pts',(1.27478211834185,2.104802836,7.39140133707004));
#125089=CARTESIAN_POINT('',(0.459008938997241,1.97432008542257,7.48594087559712));
#125090=CARTESIAN_POINT('',(1.02461500783359,2.06488542555259,7.42968127597571));
#125091=CARTESIAN_POINT('Origin',(0.0043556889311553,1.87505116433469,-0.188905834260398));
#125092=CARTESIAN_POINT('Ctrl Pts',(0.992091959997776,2.10403448596886,
7.18180016033055));
#125093=CARTESIAN_POINT('Ctrl Pts',(0.997458679234665,2.09719849231725,
7.22306246022236));
#125094=CARTESIAN_POINT('Ctrl Pts',(1.00285674280479,2.09052285934313,7.26437149725571));
#125095=CARTESIAN_POINT('Ctrl Pts',(1.01369768214475,2.07748305174204,7.34698583760116));
#125096=CARTESIAN_POINT('Ctrl Pts',(1.01914634417815,2.07111192519156,7.38833520691057));
#125097=CARTESIAN_POINT('Ctrl Pts',(1.02461500444344,2.06488542585939,7.42968127647032));
#125098=CARTESIAN_POINT('',(0.332578908769879,1.97432008626233,7.366504715349));
#125099=CARTESIAN_POINT('Origin',(-2.01526078810743E-13,2.06597317200011,
-1.06425285251177E-12));
#125100=CARTESIAN_POINT('',(1.02305817476535,1.88359401259106,7.42989582457252));
#125101=CARTESIAN_POINT('Origin',(-0.00472924854615489,2.01784565612039,
-0.191489621333766));
#125102=CARTESIAN_POINT('',(1.5803045683921,1.97432008362733,7.33161902003294));
#125103=CARTESIAN_POINT('Origin',(-0.024888475172779,1.87500215864661,-0.190931453900025));
#125104=CARTESIAN_POINT('Origin',(-0.0338263713808067,2.01785750447293,
-0.190074353583174));
#125105=CARTESIAN_POINT('Ctrl Pts',(0.987449852,2.104810499,7.182439891));
#125106=CARTESIAN_POINT('Ctrl Pts',(1.377390219,2.039629277,7.128830454));
#125107=CARTESIAN_POINT('Ctrl Pts',(1.759234759,1.974320085,7.033320202));
#125108=CARTESIAN_POINT('Ctrl Pts',(0.77727679,2.104810499,7.459613984));
#125109=CARTESIAN_POINT('Ctrl Pts',(1.182265159,2.039629277,7.41741501));
#125110=CARTESIAN_POINT('Ctrl Pts',(1.580304579,1.974320085,7.331619019));
#125111=CARTESIAN_POINT('',(1.66976965661296,1.97432008293108,7.18246961337972));
#125112=CARTESIAN_POINT('Ctrl Pts',(1.73266090573731,1.96978752936799,7.03996708358226));
#125113=CARTESIAN_POINT('Ctrl Pts',(1.74594783236865,1.97205380718396,7.0366436427912));
#125114=CARTESIAN_POINT('Ctrl Pts',(1.759234759,1.974320085,7.033320202));
#125115=CARTESIAN_POINT('Ctrl Pts',(2.144634407,2.040055578,6.936920715));
#125116=CARTESIAN_POINT('Ctrl Pts',(2.517193523,2.104802836,6.798987922));
#125117=CARTESIAN_POINT('Ctrl Pts',(2.03089967991489,1.96978752936799,7.22039699500751));
#125118=CARTESIAN_POINT('Ctrl Pts',(2.04452533034233,1.97205380718396,7.21650885961273));
#125119=CARTESIAN_POINT('Ctrl Pts',(2.05815098076969,1.974320085,7.21262072421792));
#125120=CARTESIAN_POINT('Ctrl Pts',(2.45337562708394,2.040055578,7.09984174574467));
#125121=CARTESIAN_POINT('Ctrl Pts',(2.83391121931717,2.104802836,6.94455400749346));
#125122=CARTESIAN_POINT('',(2.05753356652339,1.97432008541403,7.21225038508608));
#125123=CARTESIAN_POINT('',(2.59782193263601,2.06488542558443,7.03571751704224));
#125124=CARTESIAN_POINT('Origin',(-0.0363552949333781,1.87505115563869,
-0.185425571201403));
#125125=CARTESIAN_POINT('Ctrl Pts',(2.51277214423581,2.10403448587199,6.80062321814657));
#125126=CARTESIAN_POINT('Ctrl Pts',(2.52688364672442,2.09719845370066,6.83976736318672));
#125127=CARTESIAN_POINT('Ctrl Pts',(2.54103581863248,2.09052278112002,6.87895044282818));
#125128=CARTESIAN_POINT('Ctrl Pts',(2.56938277355433,2.07748305176976,6.95730235436121));
#125129=CARTESIAN_POINT('Ctrl Pts',(2.58359294085558,2.07111192522839,6.99651369714983));
#125130=CARTESIAN_POINT('Ctrl Pts',(2.59782192948137,2.06488542591375,7.03571751823952));
#125131=CARTESIAN_POINT('',(1.90838416002563,1.97432008626233,7.12278529450258));
#125132=CARTESIAN_POINT('Origin',(4.74446870679657E-13,2.06597317200044,
1.06858966120171E-12));
#125133=CARTESIAN_POINT('',(2.59634761954241,1.88359401255043,7.03626172285193));
#125134=CARTESIAN_POINT('Origin',(-0.045783351768986,2.01784567000082,-0.185996229389547));
#125135=CARTESIAN_POINT('',(3.11943929387699,1.97432008362731,6.82049107327776));
#125136=CARTESIAN_POINT('Origin',(-0.0653511309221899,1.87500216096182,
-0.18111710065302));
#125137=CARTESIAN_POINT('Origin',(-0.0738959797718136,2.017857509494,-0.178359071339537));
#125138=CARTESIAN_POINT('Ctrl Pts',(2.508376089,2.104810499,6.802245908));
#125139=CARTESIAN_POINT('Ctrl Pts',(2.877675422,2.039629277,6.66606417800001));
#125140=CARTESIAN_POINT('Ctrl Pts',(3.230060768,1.974320085,6.490701613));
#125141=CARTESIAN_POINT('Ctrl Pts',(2.362700993,2.104810499,7.118120821));
#125142=CARTESIAN_POINT('Ctrl Pts',(2.749149426,2.039629277,6.989847907));
#125143=CARTESIAN_POINT('Ctrl Pts',(3.119439304,1.974320085,6.82049107000001));
#125144=CARTESIAN_POINT('',(3.17475002452162,1.97432008293108,6.65559634697524));
#125145=CARTESIAN_POINT('Ctrl Pts',(3.20553707944452,1.9697875293269,6.50290568719135));
#125146=CARTESIAN_POINT('Ctrl Pts',(3.21779892372226,1.97205380716342,6.49680365009561));
#125147=CARTESIAN_POINT('Ctrl Pts',(3.230060768,1.974320085,6.49070161300001));
#125148=CARTESIAN_POINT('Ctrl Pts',(3.585726947,2.040055578,6.313706361));
#125149=CARTESIAN_POINT('Ctrl Pts',(3.919924364,2.104802836,6.098909163));
#125150=CARTESIAN_POINT('Ctrl Pts',(3.5355902941514,1.9697875293269,6.61500472717748));
#125151=CARTESIAN_POINT('Ctrl Pts',(3.54806155038054,1.97205380716342,6.6082783821254));
#125152=CARTESIAN_POINT('Ctrl Pts',(3.56053280660969,1.974320085,6.60155203707342));
#125153=CARTESIAN_POINT('Ctrl Pts',(3.92227317370945,2.040055578,6.4064481530988));
#125154=CARTESIAN_POINT('Ctrl Pts',(4.26052978288015,2.104802836,6.17298705222455));
#125155=CARTESIAN_POINT('',(3.55985021522416,1.97432008541403,6.60132308208483));
#125156=CARTESIAN_POINT('',(4.04955759140998,2.06488542558083,6.31277142726971));
#125157=CARTESIAN_POINT('Origin',(-0.0753663103962776,1.87505112929091,
-0.17327508517603));
#125158=CARTESIAN_POINT('Ctrl Pts',(3.91595789455973,2.10403448589348,6.10145669238763));
#125159=CARTESIAN_POINT('Ctrl Pts',(3.93815431207447,2.09719845373132,6.13665211315745));
#125160=CARTESIAN_POINT('Ctrl Pts',(3.96039881815478,2.09052278109977,6.17187681586637));
#125161=CARTESIAN_POINT('Ctrl Pts',(4.00492638198642,2.07748305174562,6.24230314600544));
#125162=CARTESIAN_POINT('Ctrl Pts',(4.02723360302552,2.07111192522287,6.27754298342747));
#125163=CARTESIAN_POINT('Ctrl Pts',(4.04955758851027,2.06488542589252,6.31277142916232));
#125164=CARTESIAN_POINT('',(3.39495548913088,1.97432008626233,6.54601234906254));
#125165=CARTESIAN_POINT('Origin',(-5.68772459685896E-13,2.06597317199978,
-8.68229099726392E-13));
#125166=CARTESIAN_POINT('',(4.04823473517134,1.88359401261641,6.31361984319499));
#125167=CARTESIAN_POINT('Origin',(-0.0846965919862108,2.01784564054595,
-0.171805572819673));
#125168=CARTESIAN_POINT('',(4.51271250479587,1.97432008362732,5.99044454341028));
#125169=CARTESIAN_POINT('Origin',(-0.102758079614512,1.87500221011058,-0.162834088004034));
#125170=CARTESIAN_POINT('Origin',(-0.110510209683147,2.0178575028769,-0.158303586201035));
#125171=CARTESIAN_POINT('Ctrl Pts',(3.912013447,2.104810499,6.103986467));
#125172=CARTESIAN_POINT('Ctrl Pts',(4.243403721,2.039629277,5.89160015));
#125173=CARTESIAN_POINT('Ctrl Pts',(4.549852726,1.974320085,5.644585031));
#125174=CARTESIAN_POINT('Ctrl Pts',(3.837647923,2.104810499,6.443792239));
#125175=CARTESIAN_POINT('Ctrl Pts',(4.187486522,2.039629277,6.235443285));
#125176=CARTESIAN_POINT('Ctrl Pts',(4.512712514,1.974320085,5.990444538));
#125177=CARTESIAN_POINT('',(4.53128260996699,1.97432008293108,5.81751479231475));
#125178=CARTESIAN_POINT('Ctrl Pts',(4.52852590254689,1.9697875292444,5.66177564912586));
#125179=CARTESIAN_POINT('Ctrl Pts',(4.53918931427345,1.97205380712217,5.653180340063));
#125180=CARTESIAN_POINT('Ctrl Pts',(4.549852726,1.974320085,5.644585031));
#125181=CARTESIAN_POINT('Ctrl Pts',(4.859154879,2.040055578,5.395270115));
#125182=CARTESIAN_POINT('Ctrl Pts',(5.139363898,2.104802836,5.11365219));
#125183=CARTESIAN_POINT('Ctrl Pts',(4.87496063661739,1.9697875292444,5.70030219096034));
#125184=CARTESIAN_POINT('Ctrl Pts',(4.8856943566356,1.97205380712217,5.69105215250749));
#125185=CARTESIAN_POINT('Ctrl Pts',(4.89642807665381,1.974320085,5.68180211405464));
#125186=CARTESIAN_POINT('Ctrl Pts',(5.2077695869007,2.040055578,5.41349616449857));
#125187=CARTESIAN_POINT('Ctrl Pts',(5.48793070796859,2.104802836,5.1127780815485));
#125188=CARTESIAN_POINT('',(4.8957122252653,1.97432008541403,5.68172524887134));
#125189=CARTESIAN_POINT('',(5.3119404380159,2.06488542554777,5.29464716104061));
#125190=CARTESIAN_POINT('Origin',(-0.110853200776553,1.87505113429841,-0.153022349890662));
#125191=CARTESIAN_POINT('Ctrl Pts',(5.13603780673366,2.10403448590885,5.11699283318292));
#125192=CARTESIAN_POINT('Ctrl Pts',(5.16528125943058,2.09719845369597,5.14659383102125));
#125193=CARTESIAN_POINT('Ctrl Pts',(5.19457797081671,2.09052278110507,5.17621308819953));
#125194=CARTESIAN_POINT('Ctrl Pts',(5.25320408410194,2.07748305170339,5.23542077989614));
#125195=CARTESIAN_POINT('Ctrl Pts',(5.28256529802559,2.07111192517364,5.26504133632377));
#125196=CARTESIAN_POINT('Ctrl Pts',(5.31194043558567,2.06488542584355,5.2946471635141));
#125197=CARTESIAN_POINT('',(4.72278247355731,1.97432008626233,5.6631551419559));
#125198=CARTESIAN_POINT('Origin',(5.09575021068187E-13,2.06597317199967,
3.72965547335014E-13));
#125199=CARTESIAN_POINT('',(5.31083089400445,1.88359401261276,5.29576011612746));
#125200=CARTESIAN_POINT('Origin',(-0.119649861527216,2.01784567590668,-0.149581916488767));
#125201=CARTESIAN_POINT('',(5.69497629518068,1.97432008362732,4.88029148524348));
#125202=CARTESIAN_POINT('Origin',(-0.135360135114847,1.8750021533394,-0.136937159342184));
#125203=CARTESIAN_POINT('Origin',(-0.141957160544719,2.01785751579753,-0.130846144117192));
#125204=CARTESIAN_POINT('Ctrl Pts',(5.132729405,2.104810499,5.120311403));
#125205=CARTESIAN_POINT('Ctrl Pts',(5.410715178,2.039629277,4.841651446));
#125206=CARTESIAN_POINT('Ctrl Pts',(5.656898626,1.974320085,4.534533927));
#125207=CARTESIAN_POINT('Ctrl Pts',(5.133150701,2.104810499,5.468159094));
#125208=CARTESIAN_POINT('Ctrl Pts',(5.430021402,2.039629277,5.189476265));
#125209=CARTESIAN_POINT('Ctrl Pts',(5.69497630300001,1.974320085,4.880291478));
#125210=CARTESIAN_POINT('',(5.6759374563815,1.97432008293108,4.70741271228884));
#125211=CARTESIAN_POINT('Ctrl Pts',(5.63976588660991,1.96978752926671,4.55590727463079));
#125212=CARTESIAN_POINT('Ctrl Pts',(5.64833225630496,1.97205380713332,4.5452206008154));
#125213=CARTESIAN_POINT('Ctrl Pts',(5.656898626,1.974320085,4.534533927));
#125214=CARTESIAN_POINT('Ctrl Pts',(5.90537413,2.040055578,4.224557034));
#125215=CARTESIAN_POINT('Ctrl Pts',(6.118492488,2.104802836,3.889286524));
#125216=CARTESIAN_POINT('Ctrl Pts',(5.98638323718693,1.96978752926671,4.51905985893111));
#125217=CARTESIAN_POINT('Ctrl Pts',(5.99487752390771,1.97205380713332,4.50771864877803));
#125218=CARTESIAN_POINT('Ctrl Pts',(6.00337181062865,1.974320085,4.49637743862502));
#125219=CARTESIAN_POINT('Ctrl Pts',(6.24975648105858,2.040055578,4.16741511163491));
#125220=CARTESIAN_POINT('Ctrl Pts',(6.45872209265358,2.104802836,3.81350129129357));
#125221=CARTESIAN_POINT('',(6.00265617455652,1.97432008542257,4.49645625496983));
#125222=CARTESIAN_POINT('',(6.32594285336114,2.06488542554472,4.02895107831226));
#125223=CARTESIAN_POINT('Origin',(-0.141156925378861,1.87505112236032,-0.125614706819361));
#125224=CARTESIAN_POINT('Ctrl Pts',(6.1159622987499,2.10403448590706,3.89326407603806));
#125225=CARTESIAN_POINT('Ctrl Pts',(6.15088539536528,2.09719845368304,3.91588654113296));
#125226=CARTESIAN_POINT('Ctrl Pts',(6.1858644305456,2.09052278111875,3.9385153895049));
#125227=CARTESIAN_POINT('Ctrl Pts',(6.25584780147992,2.07748305171283,3.98373595689417));
#125228=CARTESIAN_POINT('Ctrl Pts',(6.29089011066474,2.07111192517319,4.00635220811398));
#125229=CARTESIAN_POINT('Ctrl Pts',(6.32594285153372,2.06488542584587,4.02895108122973));
#125230=CARTESIAN_POINT('',(5.82977739726162,1.97432008626233,4.51549509461754));
#125231=CARTESIAN_POINT('Origin',(1.48318857196017E-13,2.06597317199933,
4.31512464649231E-14));
#125232=CARTESIAN_POINT('',(6.32509850206447,1.8835940125713,4.03027653313335));
#125233=CARTESIAN_POINT('Origin',(-0.149007952235226,2.01784564257634,-0.120363418775087));
#125234=CARTESIAN_POINT('',(6.61094932292352,1.97432008362731,3.54194142174975));
#125235=CARTESIAN_POINT('Origin',(-0.161633041338647,1.87500220953601,-0.104637270587731));
#125236=CARTESIAN_POINT('Origin',(-0.166766339652466,2.01785753493042,-0.0972704506244883));
#125237=CARTESIAN_POINT('Ctrl Pts',(6.11344464,2.104810499,3.897216268));
#125238=CARTESIAN_POINT('Ctrl Pts',(6.325027606,2.039629277,3.565312503));
#125239=CARTESIAN_POINT('Ctrl Pts',(6.499434234,1.974320085,3.212453056));
#125240=CARTESIAN_POINT('Ctrl Pts',(6.188633058,2.104810499,4.236840907));
#125241=CARTESIAN_POINT('Ctrl Pts',(6.41865451600001,2.039629277,3.900855103));
#125242=CARTESIAN_POINT('Ctrl Pts',(6.610949329,1.974320085,3.541941413));
#125243=CARTESIAN_POINT('',(6.55519177567562,1.97432008293108,3.37719724580523));
#125244=CARTESIAN_POINT('Ctrl Pts',(6.48729668650738,1.969787529284,3.23700973907726));
#125245=CARTESIAN_POINT('Ctrl Pts',(6.49336546025369,1.97205380714197,3.22473139753864));
#125246=CARTESIAN_POINT('Ctrl Pts',(6.499434234,1.974320085,3.212453056));
#125247=CARTESIAN_POINT('Ctrl Pts',(6.67546465,2.040055578,2.856308362));
#125248=CARTESIAN_POINT('Ctrl Pts',(6.81152717,2.104802836,2.483062143));
#125249=CARTESIAN_POINT('Ctrl Pts',(6.81788921130267,1.969787529284,3.12651131127987));
#125250=CARTESIAN_POINT('Ctrl Pts',(6.82374688136015,1.97205380714197,3.11360923180562));
#125251=CARTESIAN_POINT('Ctrl Pts',(6.82960455141775,1.974320085,3.10070715233132));
#125252=CARTESIAN_POINT('Ctrl Pts',(6.99951170896415,2.040055578,2.72647036050727));
#125253=CARTESIAN_POINT('Ctrl Pts',(7.12751081015265,2.104802836,2.33590941933527));
#125254=CARTESIAN_POINT('',(6.82892258744442,1.97432008541403,3.10093796957677));
#125255=CARTESIAN_POINT('',(7.04415121165797,2.06488542558693,2.57486572117495));
#125256=CARTESIAN_POINT('Origin',(-0.164860089069191,1.87505114807512,-0.0923332809654503));
#125257=CARTESIAN_POINT('Ctrl Pts',(6.80991119064009,2.10403448596401,2.48749061800447));
#125258=CARTESIAN_POINT('Ctrl Pts',(6.84888096585377,2.09719845377735,2.50207674884828));
#125259=CARTESIAN_POINT('Ctrl Pts',(6.88790674456954,2.09052278115302,2.51665708882608));
#125260=CARTESIAN_POINT('Ctrl Pts',(6.96597502846516,2.07748305177085,2.54577606833292));
#125261=CARTESIAN_POINT('Ctrl Pts',(7.00505989342596,2.07111192523824,2.56033050351797));
#125262=CARTESIAN_POINT('Ctrl Pts',(7.0441512104955,2.06488542590153,2.57486572443612));
#125263=CARTESIAN_POINT('',(6.66417840968749,1.97432008626233,3.15669551549313));
#125264=CARTESIAN_POINT('Origin',(-4.06358974247567E-13,2.06597317199956,
-5.05238212378245E-14));
#125265=CARTESIAN_POINT('',(7.04361153473072,1.88359401255142,2.57634169805879));
#125266=CARTESIAN_POINT('Origin',(-0.171398987472374,2.01784567825094,-0.0855171611339606));
#125267=CARTESIAN_POINT('',(7.21780170794699,1.97432008362733,2.03797411287211));
#125268=CARTESIAN_POINT('Origin',(-0.180347906282772,1.87500217343594,-0.0674445279812566));
#125269=CARTESIAN_POINT('Origin',(-0.183777732123206,2.01785750426266,-0.0591464868456302));
#125270=CARTESIAN_POINT('Ctrl Pts',(6.808301998,2.104810499,2.491891632));
#125271=CARTESIAN_POINT('Ctrl Pts',(6.943588774,2.039629277,2.122263509));
#125272=CARTESIAN_POINT('Ctrl Pts',(7.038063521,1.974320085,1.74016145));
#125273=CARTESIAN_POINT('Ctrl Pts',(6.954741811,2.104810499,2.807412748));
#125274=CARTESIAN_POINT('Ctrl Pts',(7.10715847900001,2.039629277,2.429834291));
#125275=CARTESIAN_POINT('Ctrl Pts',(7.21780171200001,1.974320085,2.037974103));
#125276=CARTESIAN_POINT('',(7.12793261324207,1.97432008293108,1.88906778879299));
#125277=CARTESIAN_POINT('Ctrl Pts',(7.03148870360976,1.96978752929256,1.76675322528271));
#125278=CARTESIAN_POINT('Ctrl Pts',(7.03477611230488,1.97205380714625,1.75345733764136));
#125279=CARTESIAN_POINT('Ctrl Pts',(7.038063521,1.974320085,1.74016145));
#125280=CARTESIAN_POINT('Ctrl Pts',(7.133417862,2.040055578,1.354501886));
#125281=CARTESIAN_POINT('Ctrl Pts',(7.18606241200001,2.104802836,0.960732536));
#125282=CARTESIAN_POINT('Ctrl Pts',(7.33059826296775,1.96978752929256,1.58777056923608));
#125283=CARTESIAN_POINT('Ctrl Pts',(7.33354541825529,1.97205380714625,1.57391090731557));
#125284=CARTESIAN_POINT('Ctrl Pts',(7.33649257354279,1.974320085,1.56005124539505));
#125285=CARTESIAN_POINT('Ctrl Pts',(7.42197754858784,2.040055578,1.15803888505944));
#125286=CARTESIAN_POINT('Ctrl Pts',(7.46302504513293,2.104802836,0.749093018303043));
#125287=CARTESIAN_POINT('',(7.335876173956,1.97432008542257,1.56042326496528));
#125288=CARTESIAN_POINT('',(7.43298288878896,2.06488542554557,1.00038250462391));
#125289=CARTESIAN_POINT('Origin',(-0.180854772319673,1.87505114218545,-0.0547345597610988));
#125290=CARTESIAN_POINT('Ctrl Pts',(7.1854362047806,2.10403448594993,0.965404863426473));
#125291=CARTESIAN_POINT('Ctrl Pts',(7.22663047536372,2.09719845374919,0.971272628909129));
#125292=CARTESIAN_POINT('Ctrl Pts',(7.26787819505574,2.09052278113993,0.977122699762518));
#125293=CARTESIAN_POINT('Ctrl Pts',(7.35038100578259,2.07748305173631,0.988778520285952));
#125294=CARTESIAN_POINT('Ctrl Pts',(7.39168086172629,2.07111192518725,0.994590590199989));
#125295=CARTESIAN_POINT('Ctrl Pts',(7.43298288835397,2.06488542584543,1.00038250804817));
#125296=CARTESIAN_POINT('',(7.18696984626825,1.97432008626233,1.65029236204173));
#125297=CARTESIAN_POINT('Origin',(3.46077333457373E-13,2.06597317199922,
1.03731042852551E-13));
#125298=CARTESIAN_POINT('',(7.43277311984019,1.88359401261866,1.00193998853181));
#125299=CARTESIAN_POINT('Origin',(-0.18577510321681,2.01784564018602,-0.0466720355230915));
#125300=CARTESIAN_POINT('',(7.48715770716292,1.97432008362733,0.438713400513213));
#125301=CARTESIAN_POINT('Origin',(-0.19063011925592,1.87500216022345,-0.0270982572346022));
#125302=CARTESIAN_POINT('Origin',(-0.192195711059792,2.01785751467762,-0.0182568766687107));
#125303=CARTESIAN_POINT('Ctrl Pts',(7.184810722,2.104810499,0.970048913));
#125304=CARTESIAN_POINT('Ctrl Pts',(7.23747544800001,2.039629277,0.579979832));
#125305=CARTESIAN_POINT('Ctrl Pts',(7.24760078,1.974320085,0.186501829));
#125306=CARTESIAN_POINT('Ctrl Pts',(7.395654567,2.104810499,1.24671309));
#125307=CARTESIAN_POINT('Ctrl Pts',(7.463339611,2.039629277,0.845197129));
#125308=CARTESIAN_POINT('Ctrl Pts',(7.487157709,1.974320085,0.43871339));
#125309=CARTESIAN_POINT('',(7.36737924396087,1.97432008293108,0.312607622205938));
#125310=CARTESIAN_POINT('Ctrl Pts',(7.24689612384429,1.96978752930384,0.213885294717906));
#125311=CARTESIAN_POINT('Ctrl Pts',(7.24724845192216,1.97205380715189,0.200193561858956));
#125312=CARTESIAN_POINT('Ctrl Pts',(7.24760078,1.974320085,0.186501829));
#125313=CARTESIAN_POINT('Ctrl Pts',(7.257820383,2.040055578,-0.210639594));
#125314=CARTESIAN_POINT('Ctrl Pts',(7.224585363,2.104802836,-0.606519857));
#125315=CARTESIAN_POINT('Ctrl Pts',(7.50053668693796,1.96978752930384,-0.0252125596737303));
#125316=CARTESIAN_POINT('Ctrl Pts',(7.50043552174716,1.97205380715189,-0.0393817416357748));
#125317=CARTESIAN_POINT('Ctrl Pts',(7.50033435655642,1.974320085,-0.0535509235978196));
#125318=CARTESIAN_POINT('Ctrl Pts',(7.49739996627716,2.040055578,-0.464541201097412));
#125319=CARTESIAN_POINT('Ctrl Pts',(7.44957652221315,2.104802836,-0.872750138699384));
#125320=CARTESIAN_POINT('',(7.49981234051242,1.97432008541403,-0.0530550903464663));
#125321=CARTESIAN_POINT('',(7.47425654638148,2.06488542557781,-0.620877486031077));
#125322=CARTESIAN_POINT('Origin',(-0.188392808761042,1.87505115454289,-0.0145764631325766));
#125323=CARTESIAN_POINT('Ctrl Pts',(7.22497820783533,2.10403448606495,-0.601822150024921));
#125324=CARTESIAN_POINT('Ctrl Pts',(7.26647055856495,2.09719848953937,-0.604947103725027));
#125325=CARTESIAN_POINT('Ctrl Pts',(7.30801127704622,2.09052285362558,-0.608100825741811));
#125326=CARTESIAN_POINT('Ctrl Pts',(7.39109133589379,2.07748305180721,-0.614453212590015));
#125327=CARTESIAN_POINT('Ctrl Pts',(7.43267504747039,2.07111192523526,-0.617655273859918));
#125328=CARTESIAN_POINT('Ctrl Pts',(7.47425654669052,2.0648854259041,-0.620877482673569));
#125329=CARTESIAN_POINT('',(7.37370656042999,1.97432008626233,0.0667233722376788));
#125330=CARTESIAN_POINT('Origin',(-3.56919355182228E-13,2.06597317199989,
-5.50571415715295E-14));
#125331=CARTESIAN_POINT('',(7.47438649539287,1.88359401260575,-0.619311321310287));
#125332=CARTESIAN_POINT('Origin',(-0.191465076505951,2.01784564451317,-0.00564471672548951));
#125333=CARTESIAN_POINT('',(7.40642253346448,1.97432008362734,-1.1810610633371));
#125334=CARTESIAN_POINT('Origin',(-0.191998518223641,1.87500217719841,0.0145151198199273));
#125335=CARTESIAN_POINT('Origin',(-0.191626963176276,2.01785748769558,0.0234863549441309));
#125336=CARTESIAN_POINT('Ctrl Pts',(7.225365682,2.104810499,-0.597152216));
#125337=CARTESIAN_POINT('Ctrl Pts',(7.192945813,2.039629277,-0.989423057));
#125338=CARTESIAN_POINT('Ctrl Pts',(7.118248282,1.974320085,-1.375878411));
#125339=CARTESIAN_POINT('Ctrl Pts',(7.490754735,2.104810499,-0.372281487));
#125340=CARTESIAN_POINT('Ctrl Pts',(7.470543277,2.039629277,-0.778960512000001));
#125341=CARTESIAN_POINT('Ctrl Pts',(7.406422533,1.974320085,-1.181061074));
#125342=CARTESIAN_POINT('',(7.26233540970488,1.97432008293108,-1.27846972997522));
#125343=CARTESIAN_POINT('Ctrl Pts',(7.12344673600873,1.96978752934063,-1.34898367552147));
#125344=CARTESIAN_POINT('Ctrl Pts',(7.12084750900437,1.97205380717028,-1.36243104326073));
#125345=CARTESIAN_POINT('Ctrl Pts',(7.118248282,1.974320085,-1.375878411));
#125346=CARTESIAN_POINT('Ctrl Pts',(7.04285528900001,2.040055578,-1.7659318));
#125347=CARTESIAN_POINT('Ctrl Pts',(6.925294731,2.104802836,-2.145412056));
#125348=CARTESIAN_POINT('Ctrl Pts',(7.31975835219021,1.96978752934063,-1.63701677796964));
#125349=CARTESIAN_POINT('Ctrl Pts',(7.31661359694591,1.97205380717028,-1.65083294469777));
#125350=CARTESIAN_POINT('Ctrl Pts',(7.31346884170166,1.974320085,-1.66464911142589));
#125351=CARTESIAN_POINT('Ctrl Pts',(7.22225229550629,2.040055578,-2.06539985757794));
#125352=CARTESIAN_POINT('Ctrl Pts',(7.08779408177615,2.104802836,-2.45378447032773));
#125353=CARTESIAN_POINT('',(7.31306561959532,1.97432008541404,-1.66405265246183));
#125354=CARTESIAN_POINT('',(7.16604227551646,2.06488542558446,-2.21310593549342));
#125355=CARTESIAN_POINT('Origin',(-0.187121611163891,1.87505116918617,0.0262631604130306));
#125356=CARTESIAN_POINT('Ctrl Pts',(6.92668825952681,2.10403448598584,-2.14090862818555));
#125357=CARTESIAN_POINT('Ctrl Pts',(6.9665387449173,2.09719849370837,-2.15288014382144));
#125358=CARTESIAN_POINT('Ctrl Pts',(7.00643027970097,2.09052286216309,-2.16489015172776));
#125359=CARTESIAN_POINT('Ctrl Pts',(7.08620245038645,2.07748305175337,-2.18895379605831));
#125360=CARTESIAN_POINT('Ctrl Pts',(7.12612560916814,2.07111192523224,-2.20102026360126));
#125361=CARTESIAN_POINT('Ctrl Pts',(7.16604227657075,2.06488542588779,-2.21310593216758));
#125362=CARTESIAN_POINT('',(7.21565695159499,1.97432008626233,-1.51996552892817));
#125363=CARTESIAN_POINT('Origin',(-6.78276879106932E-13,2.06597317200044,
1.95915332568131E-13));
#125364=CARTESIAN_POINT('',(7.16650586494505,1.8835940125881,-2.21160432283929));
#125365=CARTESIAN_POINT('Origin',(-0.188202231489694,2.01784568714537,0.0356465962586838));
#125366=CARTESIAN_POINT('',(6.979371273744,1.97432008362733,-2.74561042469069));
#125367=CARTESIAN_POINT('Origin',(-0.184389231669062,1.87500215963995,0.0554497128324294));
#125368=CARTESIAN_POINT('Origin',(-0.182098181484285,2.01785749936806,0.0641314642319986));
#125369=CARTESIAN_POINT('Ctrl Pts',(6.928070572,2.104810499,-2.13643117));
#125370=CARTESIAN_POINT('Ctrl Pts',(6.812082027,2.039629277,-2.512561624));
#125371=CARTESIAN_POINT('Ctrl Pts',(6.656054405,1.974320085,-2.873924105));
#125372=CARTESIAN_POINT('Ctrl Pts',(7.235595536,2.104810499,-1.973868596));
#125373=CARTESIAN_POINT('Ctrl Pts',(7.128432642,2.039629277,-2.366694825));
#125374=CARTESIAN_POINT('Ctrl Pts',(6.979371271,1.974320085,-2.745610435));
#125375=CARTESIAN_POINT('',(6.81771284284578,1.97432008293108,-2.80976725824203));
#125376=CARTESIAN_POINT('Ctrl Pts',(6.66691289521506,1.96978752930778,-2.84877566723));
#125377=CARTESIAN_POINT('Ctrl Pts',(6.66148365010753,1.97205380715386,-2.86134988611501));
#125378=CARTESIAN_POINT('Ctrl Pts',(6.656054405,1.974320085,-2.873924105));
#125379=CARTESIAN_POINT('Ctrl Pts',(6.49857411,2.040055578,-3.238650998));
#125380=CARTESIAN_POINT('Ctrl Pts',(6.302185015,2.104802836,-3.583987171));
#125381=CARTESIAN_POINT('Ctrl Pts',(6.79671625280338,1.96978752930778,-3.1722759107947));
#125382=CARTESIAN_POINT('Ctrl Pts',(6.79067495268329,1.97205380715386,-3.18509303387333));
#125383=CARTESIAN_POINT('Ctrl Pts',(6.78463365256321,1.974320085,-3.19791015695202));
#125384=CARTESIAN_POINT('Ctrl Pts',(6.60940013367591,2.040055578,-3.56968271160877));
#125385=CARTESIAN_POINT('Ctrl Pts',(6.39459426724597,2.104802836,-3.92008256653065));
#125386=CARTESIAN_POINT('',(6.78436807859121,1.97432008541403,-3.19724096198437));
#125387=CARTESIAN_POINT('',(6.52275183234442,2.06488542557874,-3.70185201111922));
#125388=CARTESIAN_POINT('Origin',(-0.177101200238827,1.8750511420646,0.0658748586744901));
#125389=CARTESIAN_POINT('Ctrl Pts',(6.304514067401,2.10403448599765,-3.57988859824468));
#125390=CARTESIAN_POINT('Ctrl Pts',(6.3408593461888,2.09719849416704,-3.60014690175533));
#125391=CARTESIAN_POINT('Ctrl Pts',(6.37723643971121,2.09052286306901,-3.62045162178728));
#125392=CARTESIAN_POINT('Ctrl Pts',(6.44997061394838,2.07748305178323,-3.66110133296034));
#125393=CARTESIAN_POINT('Ctrl Pts',(6.48636645772073,2.07111192523635,-3.6814679922869));
#125394=CARTESIAN_POINT('Ctrl Pts',(6.52275183406528,2.06488542589603,-3.70185200814441));
#125395=CARTESIAN_POINT('',(6.72021124318542,1.97432008626233,-3.03558253094808));
#125396=CARTESIAN_POINT('Origin',(4.77482636762616E-13,2.06597317200011,
-2.85795692667179E-13));
#125397=CARTESIAN_POINT('',(6.52352738588618,1.88359401261646,-3.70048516261239));
#125398=CARTESIAN_POINT('Origin',(-0.176139373126123,2.01784567505773,0.075271214052744));
#125399=CARTESIAN_POINT('',(6.22597237088156,1.97432008362661,-4.18177809352906));
#125400=CARTESIAN_POINT('Origin',(-0.168158374947894,1.87500219531754,0.093791632467935));
#125401=CARTESIAN_POINT('Origin',(-0.164054535610359,2.01785749475703,0.101777878198789));
#125402=CARTESIAN_POINT('Ctrl Pts',(6.306826583,2.104810499,-3.575812977));
#125403=CARTESIAN_POINT('Ctrl Pts',(6.112692857,2.039629277,-3.918215602));
#125404=CARTESIAN_POINT('Ctrl Pts',(5.882630822,1.974320085,-4.237588302));
#125405=CARTESIAN_POINT('Ctrl Pts',(6.64210793300001,2.104810499,-3.483159803));
#125406=CARTESIAN_POINT('Ctrl Pts',(6.45300442,2.039629277,-3.843765118));
#125407=CARTESIAN_POINT('Ctrl Pts',(6.225972366,1.974320085,-4.181778103));
#125408=CARTESIAN_POINT('',(6.05430160126387,1.97432008293001,-4.2096831920532));
#125409=CARTESIAN_POINT('Ctrl Pts',(5.89864161766491,1.96978752925783,-4.21536207494712));
#125410=CARTESIAN_POINT('Ctrl Pts',(5.89063621983239,1.97205380712895,-4.22647518847359));
#125411=CARTESIAN_POINT('Ctrl Pts',(5.882630822,1.974320085,-4.237588302));
#125412=CARTESIAN_POINT('Ctrl Pts',(5.650426828,2.040055578,-4.559934474));
#125413=CARTESIAN_POINT('Ctrl Pts',(5.384392131,2.104802836,-4.85497903));
#125414=CARTESIAN_POINT('Ctrl Pts',(5.95586725441693,1.96978752925783,-4.55920294697488));
#125415=CARTESIAN_POINT('Ctrl Pts',(5.94721189386265,1.97205380712895,-4.57042171203193));
#125416=CARTESIAN_POINT('Ctrl Pts',(5.93855653330852,1.974320085,-4.58164047708885));
#125417=CARTESIAN_POINT('Ctrl Pts',(5.68749976732876,2.040055578,-4.90705116978796));
#125418=CARTESIAN_POINT('Ctrl Pts',(5.40239033188223,2.104802836,-5.2030819588303));
#125419=CARTESIAN_POINT('',(5.93844102545487,1.97432008541404,-4.58092983702517));
#125420=CARTESIAN_POINT('',(5.57446476273787,2.06488542557757,-5.01750360090843));
#125421=CARTESIAN_POINT('Origin',(-0.158799451568832,1.87505116138121,0.102406197804297));
#125422=CARTESIAN_POINT('Ctrl Pts',(5.38754780344266,2.10403448599945,-4.85147695703863));
#125423=CARTESIAN_POINT('Ctrl Pts',(5.41868842775781,2.09719849105826,-4.87907480555496));
#125424=CARTESIAN_POINT('Ctrl Pts',(5.44985014665898,2.09052285673973,-4.9067248264811));
#125425=CARTESIAN_POINT('Ctrl Pts',(5.51214531992537,2.07748305178984,-4.9620598403968));
#125426=CARTESIAN_POINT('Ctrl Pts',(5.54331201945759,2.07111192523415,-4.98977436912689));
#125427=CARTESIAN_POINT('Ctrl Pts',(5.57446476503845,2.06488542589882,-5.01750359839596));
#125428=CARTESIAN_POINT('',(5.91053592562699,1.97432008626236,-4.40925906729761));
#125429=CARTESIAN_POINT('Origin',(-1.21430643318376E-14,2.06597317200067,
5.03069808033274E-14));
#125430=CARTESIAN_POINT('',(5.57551601667315,1.88359401262239,-5.01633542971868));
#125431=CARTESIAN_POINT('Origin',(-0.155839863892731,2.01784566950499,0.11137583991492));
#125432=CARTESIAN_POINT('',(5.18145391881594,1.97432008362662,-5.42241046679518));
#125433=CARTESIAN_POINT('Origin',(-0.14406458720886,1.87500217976684,0.127748007483152));
#125434=CARTESIAN_POINT('Origin',(-0.138339389893165,2.01785750358587,0.134664849330288));
#125435=CARTESIAN_POINT('Ctrl Pts',(5.390682393,2.104810499,-4.847993744));
#125436=CARTESIAN_POINT('Ctrl Pts',(5.127480962,2.039629277,-5.140658173));
#125437=CARTESIAN_POINT('Ctrl Pts',(4.83414196,1.974320085,-5.403107579));
#125438=CARTESIAN_POINT('Ctrl Pts',(5.738042744,2.104810499,-4.829582328));
#125439=CARTESIAN_POINT('Ctrl Pts',(5.475840884,2.039629277,-5.141105227));
#125440=CARTESIAN_POINT('Ctrl Pts',(5.181453912,1.974320085,-5.422410475));
#125441=CARTESIAN_POINT('',(5.0077979453398,1.97432008293002,-5.41275901835897));
#125442=CARTESIAN_POINT('Ctrl Pts',(4.85455641397875,1.96978752925425,-5.38484283648086));
#125443=CARTESIAN_POINT('Ctrl Pts',(4.84434918698943,1.97205380712716,-5.39397520774036));
#125444=CARTESIAN_POINT('Ctrl Pts',(4.83414196,1.974320085,-5.403107579));
#125445=CARTESIAN_POINT('Ctrl Pts',(4.538071868,2.040055578,-5.668000483));
#125446=CARTESIAN_POINT('Ctrl Pts',(4.214831056,2.104802836,-5.898957465));
#125447=CARTESIAN_POINT('Ctrl Pts',(4.83652852359848,1.96978752925425,-5.73294672106691));
#125448=CARTESIAN_POINT('Ctrl Pts',(4.82566381768852,1.97205380712716,-5.74204255096055));
#125449=CARTESIAN_POINT('Ctrl Pts',(4.81479911177867,1.974320085,-5.75113838085421));
#125450=CARTESIAN_POINT('Ctrl Pts',(4.49965823349521,2.040055578,-6.01497136862089));
#125451=CARTESIAN_POINT('Ctrl Pts',(4.15757662825725,2.104802836,-6.24279102253975));
#125452=CARTESIAN_POINT('',(4.81483906876701,1.97432008542257,-5.75041952730824));
#125453=CARTESIAN_POINT('',(4.36552191631196,2.06488542557993,-6.09854229912174));
#125454=CARTESIAN_POINT('Origin',(-0.133072574609535,1.87505111885393,0.134149269772198));
#125455=CARTESIAN_POINT('Ctrl Pts',(4.21866579300695,2.10403448594715,-5.89621564465873));
#125456=CARTESIAN_POINT('Ctrl Pts',(4.24314564015502,2.09719849237975,-5.92986257791126));
#125457=CARTESIAN_POINT('Ctrl Pts',(4.26763487253668,2.09052285948726,-5.96356499754119));
#125458=CARTESIAN_POINT('Ctrl Pts',(4.31657823718754,2.0774830517774,-6.03099794484554));
#125459=CARTESIAN_POINT('Ctrl Pts',(4.34105847207769,2.07111192523094,-6.0647644424249));
#125460=CARTESIAN_POINT('Ctrl Pts',(4.3655219191016,2.06488542590188,-6.0985422971607));
#125461=CARTESIAN_POINT('',(4.82449051785214,1.97432008626236,-5.57676354993728));
#125462=CARTESIAN_POINT('Origin',(6.03250088770935E-13,2.06597317199933,
-7.52869988573934E-13));
#125463=CARTESIAN_POINT('',(4.36679971533024,1.88359401259344,-6.0976274274486));
#125464=CARTESIAN_POINT('Origin',(-0.128253981616274,2.01784565151063,0.142273006942648));
#125465=CARTESIAN_POINT('',(3.89465644041332,1.97432008362662,-6.40949695345443));
#125466=CARTESIAN_POINT('Origin',(-0.113234348416686,1.87500219878722,0.155730897896531));
#125467=CARTESIAN_POINT('Origin',(-0.106156210910903,2.01785750866169,0.161255456921047));
#125468=CARTESIAN_POINT('Ctrl Pts',(4.222475885,2.104810499,-5.893487711));
#125469=CARTESIAN_POINT('Ctrl Pts',(3.902513756,2.039629277,-6.122729281));
#125470=CARTESIAN_POINT('Ctrl Pts',(3.559613992,1.974320085,-6.315983552));
#125471=CARTESIAN_POINT('Ctrl Pts',(4.565673054,2.104810499,-5.950178952));
#125472=CARTESIAN_POINT('Ctrl Pts',(4.242633113,2.039629277,-6.198052969));
#125473=CARTESIAN_POINT('Ctrl Pts',(3.894656432,1.974320085,-6.40949696));
#125474=CARTESIAN_POINT('',(3.72713522297897,1.97432008293002,-6.3627402495688));
#125475=CARTESIAN_POINT('Ctrl Pts',(3.58347754718451,1.96978752924432,-6.30253433321539));
#125476=CARTESIAN_POINT('Ctrl Pts',(3.57154576959229,1.97205380712213,-6.30925894260769));
#125477=CARTESIAN_POINT('Ctrl Pts',(3.559613992,1.974320085,-6.315983552));
#125478=CARTESIAN_POINT('Ctrl Pts',(3.21352171,2.040055578,-6.511037088));
#125479=CARTESIAN_POINT('Ctrl Pts',(2.848189165,2.104802836,-6.667107205));
#125480=CARTESIAN_POINT('Ctrl Pts',(3.49103909375301,1.96978752924423,-6.63862427934538));
#125481=CARTESIAN_POINT('Ctrl Pts',(3.47847306406143,1.97205380712215,-6.64517186317271));
#125482=CARTESIAN_POINT('Ctrl Pts',(3.46590703436985,1.974320085,-6.65171944700002));
#125483=CARTESIAN_POINT('Ctrl Pts',(3.10141768163073,2.040055578,-6.84163819220421));
#125484=CARTESIAN_POINT('Ctrl Pts',(2.71835926323473,2.104802836,-6.9905941149948));
#125485=CARTESIAN_POINT('',(3.46610058947509,1.97432008542257,-6.65102598939106));
#125486=CARTESIAN_POINT('',(2.95245211747942,2.06488542557422,-6.89441993709166));
#125487=CARTESIAN_POINT('Origin',(-0.10112323409008,1.87505112184823,0.159619520245724));
#125488=CARTESIAN_POINT('Ctrl Pts',(2.85252365852959,2.10403448588764,-6.66525384212721));
#125489=CARTESIAN_POINT('Ctrl Pts',(2.8691981784706,2.097198453736,-6.70337678752731));
#125490=CARTESIAN_POINT('Ctrl Pts',(2.88586994821712,2.09052278108633,-6.74155596809501));
#125491=CARTESIAN_POINT('Ctrl Pts',(2.91917275381454,2.07748305174459,-6.81793328817871));
#125492=CARTESIAN_POINT('Ctrl Pts',(2.93582185562442,2.07111192521568,-6.85617287054979));
#125493=CARTESIAN_POINT('Ctrl Pts',(2.9524521206652,2.06488542588622,-6.89441993575723));
#125494=CARTESIAN_POINT('',(3.51285729480354,1.97432008626233,-6.48350476831375));
#125495=CARTESIAN_POINT('Origin',(2.97071395261028E-13,2.06597317199944,
-7.02996688639601E-13));
#125496=CARTESIAN_POINT('',(2.95389671194769,1.88359401259013,-6.8938011436048));
#125497=CARTESIAN_POINT('Origin',(-0.0946710014919422,2.01784568231715,
0.166517615899912));
#125498=CARTESIAN_POINT('',(2.42574915565128,1.97432008362663,-7.09688248541461));
#125499=CARTESIAN_POINT('Origin',(-0.0771095214129697,1.87500220161273,
0.176432218877178));
#125500=CARTESIAN_POINT('Origin',(-0.0690092930180509,2.01785749278518,
0.180306152982286));
#125501=CARTESIAN_POINT('Ctrl Pts',(2.856831098,2.104810499,-6.663408743));
#125502=CARTESIAN_POINT('Ctrl Pts',(2.495069344,2.039629277,-6.81850837300001));
#125503=CARTESIAN_POINT('Ctrl Pts',(2.118642431,1.974320085,-6.933531153));
#125504=CARTESIAN_POINT('Ctrl Pts',(3.179817567,2.104810499,-6.79255182100001));
#125505=CARTESIAN_POINT('Ctrl Pts',(2.811044533,2.039629277,-6.965186642));
#125506=CARTESIAN_POINT('Ctrl Pts',(2.425749146,1.974320085,-7.09688249));
#125507=CARTESIAN_POINT('',(2.27219580060485,1.97432008293002,-7.01520681757929));
#125508=CARTESIAN_POINT('Ctrl Pts',(2.14483925400811,1.96978752925302,-6.92552632842096));
#125509=CARTESIAN_POINT('Ctrl Pts',(2.13174084250406,1.97205380712647,-6.92952874071054));
#125510=CARTESIAN_POINT('Ctrl Pts',(2.118642431,1.974320085,-6.93353115299999));
#125511=CARTESIAN_POINT('Ctrl Pts',(1.738710849,2.040055578,-7.049624836));
#125512=CARTESIAN_POINT('Ctrl Pts',(1.348369115,2.104802836,-7.123510422));
#125513=CARTESIAN_POINT('Ctrl Pts',(1.9823125558243,1.96978752925301,-7.23388714288003));
#125514=CARTESIAN_POINT('Ctrl Pts',(1.9686327759748,1.97205380712648,-7.23758032291807));
#125515=CARTESIAN_POINT('Ctrl Pts',(1.95495299612523,1.974320085,-7.24127350295612));
#125516=CARTESIAN_POINT('Ctrl Pts',(1.55815828570982,2.040055578,-7.34839761751268));
#125517=CARTESIAN_POINT('Ctrl Pts',(1.1520344401105,2.104802836,-7.41152479726465));
#125518=CARTESIAN_POINT('',(1.9552910988738,1.97432008542256,-7.24063786665295));
#125519=CARTESIAN_POINT('',(1.40132893891287,2.06488542556653,-7.36792216172689));
#125520=CARTESIAN_POINT('Origin',(-0.0644455498001614,1.8750511310427,0.177626164917501));
#125521=CARTESIAN_POINT('Ctrl Pts',(1.35300068819368,2.10403448599822,-7.12263217760191));
#125522=CARTESIAN_POINT('Ctrl Pts',(1.36109001434623,2.09719849307877,-7.1634481242099));
#125523=CARTESIAN_POINT('Ctrl Pts',(1.36916456012967,2.09052286086466,-7.20431836909688));
#125524=CARTESIAN_POINT('Ctrl Pts',(1.38526999696438,2.07748305175325,-7.2860696486221));
#125525=CARTESIAN_POINT('Ctrl Pts',(1.39330947212822,2.07111192521438,-7.32699427557641));
#125526=CARTESIAN_POINT('Ctrl Pts',(1.40132894232119,2.06488542587175,-7.3679221611055));
#125527=CARTESIAN_POINT('',(2.03696676943691,1.97432008626233,-7.08708450836249));
#125528=CARTESIAN_POINT('Origin',(-3.10894972960218E-13,2.06597317200011,
1.45413195373756E-12));
#125529=CARTESIAN_POINT('',(1.40287278194287,1.88359401260661,-7.36762838021725));
#125530=CARTESIAN_POINT('Origin',(-0.056661288712726,2.01784569359405,0.182975980514766));
#125531=CARTESIAN_POINT('',(0.843416536409591,1.97432008362659,-7.45242568060032));
#125532=CARTESIAN_POINT('Origin',(-0.0373790373345705,1.87500222213718,
0.18888364590116));
#125533=CARTESIAN_POINT('Origin',(-0.0286353804236349,2.01785753439472,
0.190925474714267));
#125534=CARTESIAN_POINT('Ctrl Pts',(1.357604063,2.104810499,-7.121756188));
#125535=CARTESIAN_POINT('Ctrl Pts',(0.970958263,2.039629277,-7.19546159100001));
#125536=CARTESIAN_POINT('Ctrl Pts',(0.578605504,1.974320085,-7.22687454400001));
#125537=CARTESIAN_POINT('Ctrl Pts',(1.645277344,2.104810499,-7.317312516));
#125538=CARTESIAN_POINT('Ctrl Pts',(1.248014636,2.039629277,-7.40663593));
#125539=CARTESIAN_POINT('Ctrl Pts',(0.843416526,1.974320085,-7.452425683));
#125540=CARTESIAN_POINT('',(0.71101102766468,1.97432008293001,-7.33965011227314));
#125541=CARTESIAN_POINT('Ctrl Pts',(0.589148911429185,1.97256991806615,
-7.22603040681208));
#125542=CARTESIAN_POINT('Ctrl Pts',(0.583877207714593,1.97344500153307,
-7.22645247540605));
#125543=CARTESIAN_POINT('Ctrl Pts',(0.578605504,1.974320085,-7.226874544));
#125544=CARTESIAN_POINT('Ctrl Pts',(0.182599802,2.040055578,-7.258579962));
#125545=CARTESIAN_POINT('Ctrl Pts',(-0.214499177,2.104802836,-7.246826209));
#125546=CARTESIAN_POINT('Ctrl Pts',(0.363804157315899,1.97256991806615,
-7.4913823886135));
#125547=CARTESIAN_POINT('Ctrl Pts',(0.35833913061739,1.97344500153307,-7.49163979556223));
#125548=CARTESIAN_POINT('Ctrl Pts',(0.35287410391888,1.974320085,-7.49189720251094));
#125549=CARTESIAN_POINT('Ctrl Pts',(-0.0576538489707087,2.040055578,-7.51123338393259));
#125550=CARTESIAN_POINT('Ctrl Pts',(-0.467836611157437,2.104802836,-7.48559768636607));
#125551=CARTESIAN_POINT('Ctrl Pts',(-0.209787090640295,2.10403448593187,
-7.2469641490316));
#125552=CARTESIAN_POINT('Ctrl Pts',(-0.210661115512503,2.09719845377858,
-7.28856504641087));
#125553=CARTESIAN_POINT('Ctrl Pts',(-0.211561248998728,2.09052278112551,
-7.33021582666021));
#125554=CARTESIAN_POINT('Ctrl Pts',(-0.213406445786063,2.07748305177212,
-7.41351749012979));
#125555=CARTESIAN_POINT('Ctrl Pts',(-0.214352514273131,2.0711119252164,
-7.45521357168871));
#125556=CARTESIAN_POINT('Ctrl Pts',(-0.215318820520802,2.06488542588042,
-7.49690853500171));
#125557=CARTESIAN_POINT('',(0.465829941722541,1.97432008626233,-7.35928005451118));
#125558=CARTESIAN_POINT('Ctrl Pts',(-0.205103028,2.104810499,-7.247098229));
#125559=CARTESIAN_POINT('Ctrl Pts',(-0.598553747,2.039629277,-7.235963023));
#125560=CARTESIAN_POINT('Ctrl Pts',(-0.988486373,1.974320085,-7.18229731300001));
#125561=CARTESIAN_POINT('Ctrl Pts',(0.033805781,2.104810499,-7.49992381100001));
#125562=CARTESIAN_POINT('Ctrl Pts',(-0.373371039,2.039629277,-7.501759154));
#125563=CARTESIAN_POINT('Ctrl Pts',(-0.778353314,1.974320085,-7.459501734));
#125564=CARTESIAN_POINT('',(-0.883419830867674,1.97432008293002,-7.32089952502436));
#125565=CARTESIAN_POINT('Ctrl Pts',(-0.961349641748257,1.96978752924776,
-7.18603209141629));
#125566=CARTESIAN_POINT('Ctrl Pts',(-0.974918007374125,1.97205380712385,
-7.18416470220819));
#125567=CARTESIAN_POINT('Ctrl Pts',(-0.988486373000001,1.974320085,-7.182297313));
#125568=CARTESIAN_POINT('Ctrl Pts',(-1.38204941,2.040055578,-7.128131956));
#125569=CARTESIAN_POINT('Ctrl Pts',(-1.767337726,2.104802836,-7.031288457));
#125570=CARTESIAN_POINT('Ctrl Pts',(-1.23833222251996,1.96978752924775,
-7.3976495986289));
#125571=CARTESIAN_POINT('Ctrl Pts',(-1.25229838056131,1.97205380712385,
-7.39525744755006));
#125572=CARTESIAN_POINT('Ctrl Pts',(-1.2662645386027,1.974320085,-7.39286529647123));
#125573=CARTESIAN_POINT('Ctrl Pts',(-1.67136591378274,2.040055578,-7.32347873441183));
#125574=CARTESIAN_POINT('Ctrl Pts',(-2.06646034810132,2.104802836,-7.21024443357639));
#125575=CARTESIAN_POINT('',(-1.26569078805863,1.97432008542257,-7.39243037423573));
#125576=CARTESIAN_POINT('',(-1.82189851740587,2.0648854255639,-7.27534779711598));
#125577=CARTESIAN_POINT('Origin',(0.0160941115438731,1.87505115732695,0.188269130444804));
#125578=CARTESIAN_POINT('Ctrl Pts',(-1.76276545876383,2.10403448595781,
-7.0324361312964));
#125579=CARTESIAN_POINT('Ctrl Pts',(-1.77256201257561,2.09719845378385,
-7.07287653328555));
#125580=CARTESIAN_POINT('Ctrl Pts',(-1.78239478794987,2.09052278111519,
-7.11336003937026));
#125581=CARTESIAN_POINT('Ctrl Pts',(-1.80210424018197,2.07748305175972,
-7.19431749343474));
#125582=CARTESIAN_POINT('Ctrl Pts',(-1.81199161504939,2.07111192520572,
-7.23483536702823));
#125583=CARTESIAN_POINT('Ctrl Pts',(-1.82189851412105,2.06488542588051,
-7.27534779796791));
#125584=CARTESIAN_POINT('',(-1.12708857585293,1.97432008626233,-7.28736384418272));
#125585=CARTESIAN_POINT('Origin',(-1.65991352607531E-13,2.06597317199956,
-9.19403442267708E-14));
#125586=CARTESIAN_POINT('',(-1.82037400765965,1.88359401257266,-7.27572941129029));
#125587=CARTESIAN_POINT('Origin',(0.0254052287321954,2.01784566722006,0.189855907214538));
#125588=CARTESIAN_POINT('',(-2.36372820653794,1.97432008362663,-7.11777977619209));
#125589=CARTESIAN_POINT('Origin',(0.0453858973819207,1.87500220797284,0.18712122657347));
#125590=CARTESIAN_POINT('Origin',(0.0541787152175737,2.01785749269258,0.185302764171555));
#125591=CARTESIAN_POINT('Ctrl Pts',(-1.75821973,2.104810499,-7.033574012));
#125592=CARTESIAN_POINT('Ctrl Pts',(-2.14007805,2.039629277,-6.938118866));
#125593=CARTESIAN_POINT('Ctrl Pts',(-2.509357726,1.974320085,-6.801883842));
#125594=CARTESIAN_POINT('Ctrl Pts',(-1.579246502,2.104810499,-7.331847004));
#125595=CARTESIAN_POINT('Ctrl Pts',(-1.9772983,2.039629277,-7.246108457));
#125596=CARTESIAN_POINT('Ctrl Pts',(-2.363728217,1.974320085,-7.117779774));
#125597=CARTESIAN_POINT('',(-2.4365429594907,1.97432008293001,-6.95983181220429));
#125598=CARTESIAN_POINT('Ctrl Pts',(-2.48365830353901,1.96978752926819,
-6.81136489836744));
#125599=CARTESIAN_POINT('Ctrl Pts',(-2.49650801476954,1.97205380713406,
-6.80662437018367));
#125600=CARTESIAN_POINT('Ctrl Pts',(-2.509357726,1.974320085,-6.801883842));
#125601=CARTESIAN_POINT('Ctrl Pts',(-2.882075527,2.040055578,-6.664380422));
#125602=CARTESIAN_POINT('Ctrl Pts',(-3.237537527,2.104802836,-6.486975471));
#125603=CARTESIAN_POINT('Ctrl Pts',(-2.79965669405202,1.96978752926819,
-6.95849183810364));
#125604=CARTESIAN_POINT('Ctrl Pts',(-2.81278208925584,1.97205380713406,
-6.95315330308681));
#125605=CARTESIAN_POINT('Ctrl Pts',(-2.82590748445965,1.974320085,-6.94781476807013));
#125606=CARTESIAN_POINT('Ctrl Pts',(-3.20662175498896,2.040055578,-6.79296560482468));
#125607=CARTESIAN_POINT('Ctrl Pts',(-3.56813707398421,2.104802836,-6.59744503541926));
#125608=CARTESIAN_POINT('',(-2.8252536488491,1.97432008541403,-6.94751335411902));
#125609=CARTESIAN_POINT('',(-3.34328826125575,2.06488542556126,-6.71359988234816));
#125610=CARTESIAN_POINT('Origin',(0.0561901580705221,1.87505115267705,0.180407822666179));
#125611=CARTESIAN_POINT('Ctrl Pts',(-3.23331887272832,2.1040344859088,-6.48907921578793));
#125612=CARTESIAN_POINT('Ctrl Pts',(-3.25157987960098,2.09719845374874,
-6.52646817427314));
#125613=CARTESIAN_POINT('Ctrl Pts',(-3.26988552728305,2.09052278109752,
-6.56389144244372));
#125614=CARTESIAN_POINT('Ctrl Pts',(-3.30653764310171,2.07748305174118,
-6.63871920671912));
#125615=CARTESIAN_POINT('Ctrl Pts',(-3.32490400174457,2.07111192520323,
-6.67616430152468));
#125616=CARTESIAN_POINT('Ctrl Pts',(-3.34328825817631,2.06488542586829,
-6.71359988391151));
#125617=CARTESIAN_POINT('',(-2.66730568478596,1.97432008626233,-6.87469859929897));
#125618=CARTESIAN_POINT('Origin',(2.41126563160776E-13,2.06597317199933,
3.90312782094782E-13));
#125619=CARTESIAN_POINT('',(-3.34188142941272,1.88359401257845,-6.71430029892486));
#125620=CARTESIAN_POINT('Origin',(0.0656246953443929,2.01784563381219,0.179955857994889));
#125621=CARTESIAN_POINT('',(-3.83857780625906,1.97432008362732,-6.44323834739318));
#125622=CARTESIAN_POINT('Origin',(0.0845502529405523,1.87500220753361,0.172989665325833));
#125623=CARTESIAN_POINT('Origin',(0.0927466982508323,2.01785752670413,0.169323740462473));
#125624=CARTESIAN_POINT('Ctrl Pts',(-3.229124031,2.104810499,-6.491167691));
#125625=CARTESIAN_POINT('Ctrl Pts',(-3.581534681,2.039629277,-6.315855982));
#125626=CARTESIAN_POINT('Ctrl Pts',(-3.912894301,1.974320085,-6.103421843));
#125627=CARTESIAN_POINT('Ctrl Pts',(-3.118454975,2.104810499,-6.820941179));
#125628=CARTESIAN_POINT('Ctrl Pts',(-3.488769289,2.039629277,-6.651637782));
#125629=CARTESIAN_POINT('Ctrl Pts',(-3.838577816,1.974320085,-6.443238343));
#125630=CARTESIAN_POINT('',(-3.87573604768088,1.97432008293108,-6.27333009968417));
#125631=CARTESIAN_POINT('Ctrl Pts',(-3.88983386359933,1.96978752926216,
-6.11820585377211));
#125632=CARTESIAN_POINT('Ctrl Pts',(-3.90136408229967,1.97205380713105,
-6.11081384838606));
#125633=CARTESIAN_POINT('Ctrl Pts',(-3.912894301,1.974320085,-6.103421843));
#125634=CARTESIAN_POINT('Ctrl Pts',(-4.247338996,2.040055578,-5.889009866));
#125635=CARTESIAN_POINT('Ctrl Pts',(-4.556353671,2.104802836,-5.639338722));
#125636=CARTESIAN_POINT('Ctrl Pts',(-4.23007233002474,1.96978752926216,
-6.19396273380434));
#125637=CARTESIAN_POINT('Ctrl Pts',(-4.24174323357281,1.97205380713104,
-6.1859274387742));
#125638=CARTESIAN_POINT('Ctrl Pts',(-4.25341413712091,1.974320085,-6.17789214374396));
#125639=CARTESIAN_POINT('Ctrl Pts',(-4.59193952670449,2.040055578,-5.94482095355561));
#125640=CARTESIAN_POINT('Ctrl Pts',(-4.90297167475003,2.104802836,-5.67615643917303));
#125641=CARTESIAN_POINT('',(-4.25271079273639,1.97432008541403,-6.1777383320139));
#125642=CARTESIAN_POINT('',(-4.70834956143689,2.0648854255707,-5.83793149851878));
#125643=CARTESIAN_POINT('Origin',(0.093658769871397,1.87505117108866,0.164110696979646));
#125644=CARTESIAN_POINT('Ctrl Pts',(-4.55268589017149,2.10403448591427,
-5.64230016841548));
#125645=CARTESIAN_POINT('Ctrl Pts',(-4.57855748566152,2.09719845371626,
-5.67488941724997));
#125646=CARTESIAN_POINT('Ctrl Pts',(-4.60448005358777,2.0905227811132,-5.70750257679646));
#125647=CARTESIAN_POINT('Ctrl Pts',(-4.6563610206253,2.07748305174171,-5.77270178809585));
#125648=CARTESIAN_POINT('Ctrl Pts',(-4.68234757248036,2.07111192520591,
-5.80532321318402));
#125649=CARTESIAN_POINT('Ctrl Pts',(-4.70834955878,2.06488542588462,-5.83793150069733));
#125650=CARTESIAN_POINT('',(-4.08280254455632,1.97432008626233,-6.14058008928434));
#125651=CARTESIAN_POINT('Origin',(-2.09034178855205E-13,2.06597317199922,
-3.12250225675825E-13));
#125652=CARTESIAN_POINT('',(-4.70712619026902,1.88359401258214,-5.83891796682442));
#125653=CARTESIAN_POINT('Origin',(0.102775484829765,2.01784565942823,0.161641054547004));
#125654=CARTESIAN_POINT('',(-5.13393977442981,1.97432008362732,-5.46741825438345));
#125655=CARTESIAN_POINT('Origin',(0.119761026372398,1.87500217170092,0.150769287710907));
#125656=CARTESIAN_POINT('Origin',(0.126977900188805,2.01785750701945,0.14542721135377));
#125657=CARTESIAN_POINT('Ctrl Pts',(-4.549038082,2.104810499,-5.645241583));
#125658=CARTESIAN_POINT('Ctrl Pts',(-4.855522731,2.039629277,-5.398270692));
#125659=CARTESIAN_POINT('Ctrl Pts',(-5.133468287,1.974320085,-5.119570621));
#125660=CARTESIAN_POINT('Ctrl Pts',(-4.511847958,2.104810499,-5.991095726));
#125661=CARTESIAN_POINT('Ctrl Pts',(-4.83710930400001,2.039629277,-5.746143917));
#125662=CARTESIAN_POINT('Ctrl Pts',(-5.133939783,1.974320085,-5.467418248));
#125663=CARTESIAN_POINT('',(-5.13370402587073,1.97432008293108,-5.29349444335369));
#125664=CARTESIAN_POINT('Ctrl Pts',(-5.11412511472685,1.96978752917448,
-5.13896630254029));
#125665=CARTESIAN_POINT('Ctrl Pts',(-5.12379670086343,1.97205380708721,
-5.12926846177013));
#125666=CARTESIAN_POINT('Ctrl Pts',(-5.133468287,1.974320085,-5.119570621));
#125667=CARTESIAN_POINT('Ctrl Pts',(-5.41400161399999,2.040055578,-4.83827575400001));
#125668=CARTESIAN_POINT('Ctrl Pts',(-5.66211978200001,2.104802836,-4.528012762));
#125669=CARTESIAN_POINT('Ctrl Pts',(-5.46269448542457,1.96978752917448,
-5.1398108166444));
#125670=CARTESIAN_POINT('Ctrl Pts',(-5.47236517900318,1.97205380708721,
-5.12945448288212));
#125671=CARTESIAN_POINT('Ctrl Pts',(-5.48203587258168,1.974320085,-5.11909814911986));
#125672=CARTESIAN_POINT('Ctrl Pts',(-5.76254331010755,2.040055578,-4.81870308208225));
#125673=CARTESIAN_POINT('Ctrl Pts',(-6.00854877035677,2.104802836,-4.4894570760898));
#125674=CARTESIAN_POINT('',(-5.48131591003525,1.97432008542256,-5.1190991295705));
#125675=CARTESIAN_POINT('',(-5.85325366966401,2.06488542555512,-4.68928792635981));
#125676=CARTESIAN_POINT('Origin',(0.12674794337641,1.87505114974812,0.140139938977898));
#125677=CARTESIAN_POINT('Ctrl Pts',(-5.65917437480889,2.10403448600368,
-4.53169343556461));
#125678=CARTESIAN_POINT('Ctrl Pts',(-5.69144666801797,2.09719848852933,
-4.55795900408713));
#125679=CARTESIAN_POINT('Ctrl Pts',(-5.72377386052729,2.09052285163215,
-4.5842369499391));
#125680=CARTESIAN_POINT('Ctrl Pts',(-5.78845813227907,2.07748305175775,
-4.63675924955608));
#125681=CARTESIAN_POINT('Ctrl Pts',(-5.82084977523512,2.07111192519836,
-4.6630316634958));
#125682=CARTESIAN_POINT('Ctrl Pts',(-5.85325366755331,2.06488542586541,
-4.68928792903829));
#125683=CARTESIAN_POINT('',(-5.30739209512797,1.97432008626233,-5.11933487856937));
#125684=CARTESIAN_POINT('Origin',(-3.62557206479153E-13,2.06597317200011,
-2.83193607453214E-13));
#125685=CARTESIAN_POINT('',(-5.85227096105508,1.88359401263917,-4.69051432075498));
#125686=CARTESIAN_POINT('Origin',(0.135120953411509,2.01784566648913,0.135768498711389));
#125687=CARTESIAN_POINT('',(-6.18924442501226,1.97432008362733,-4.23594776103393));
#125688=CARTESIAN_POINT('Origin',(0.149372346640306,1.87500214029896,0.121499565369763));
#125689=CARTESIAN_POINT('Origin',(0.15527189438599,2.01785750689169,0.114730801693088));
#125690=CARTESIAN_POINT('Ctrl Pts',(-5.656244168,2.104810499,-4.535350253));
#125691=CARTESIAN_POINT('Ctrl Pts',(-5.902471935,2.039629277,-4.228268264));
#125692=CARTESIAN_POINT('Ctrl Pts',(-6.114007001,1.974320085,-3.896333968));
#125693=CARTESIAN_POINT('Ctrl Pts',(-5.694271946,2.104810499,-4.881113296));
#125694=CARTESIAN_POINT('Ctrl Pts',(-5.959271464,2.039629277,-4.571966749));
#125695=CARTESIAN_POINT('Ctrl Pts',(-6.189244432,1.974320085,-4.235947753));
#125696=CARTESIAN_POINT('',(-6.15162570948745,1.97432008293108,-4.06614087110922));
#125697=CARTESIAN_POINT('Ctrl Pts',(-6.0992855593784,1.96978752911656,-3.91943439982929));
#125698=CARTESIAN_POINT('Ctrl Pts',(-6.10664628018919,1.97205380705825,
-3.90788418391467));
#125699=CARTESIAN_POINT('Ctrl Pts',(-6.114007001,1.974320085,-3.896333968));
#125700=CARTESIAN_POINT('Ctrl Pts',(-6.327511533,2.040055578,-3.561309246));
#125701=CARTESIAN_POINT('Ctrl Pts',(-6.503131465,2.104802836,-3.204961958));
#125702=CARTESIAN_POINT('Ctrl Pts',(-6.43988711735395,1.96978752911656,
-3.84532705777992));
#125703=CARTESIAN_POINT('Ctrl Pts',(-6.44710540996376,1.97205380705825,
-3.83313393594917));
#125704=CARTESIAN_POINT('Ctrl Pts',(-6.45432370257357,1.974320085,-3.82094081411849));
#125705=CARTESIAN_POINT('Ctrl Pts',(-6.66369697254378,2.040055578,-3.4672680099197));
#125706=CARTESIAN_POINT('Ctrl Pts',(-6.83317280303885,2.104802836,-3.09283569069017));
#125707=CARTESIAN_POINT('',(-6.45362078060153,1.97432008541403,-3.82109654502115));
#125708=CARTESIAN_POINT('',(-6.72446614117549,2.06488542555435,-3.32137846279023));
#125709=CARTESIAN_POINT('Origin',(0.153910537074243,1.875051149797,0.10961646125067));
#125710=CARTESIAN_POINT('Ctrl Pts',(-6.5010461556297,2.10403448604283,-3.20918975482682));
#125711=CARTESIAN_POINT('Ctrl Pts',(-6.53821023998976,2.09719849249568,
-3.22790364918131));
#125712=CARTESIAN_POINT('Ctrl Pts',(-6.5754305981183,2.09052285962829,-3.24661782843558));
#125713=CARTESIAN_POINT('Ctrl Pts',(-6.64989337486342,2.07748305175858,
-3.28400700247734));
#125714=CARTESIAN_POINT('Ctrl Pts',(-6.68717551143973,2.07111192520455,
-3.30270193622378));
#125715=CARTESIAN_POINT('Ctrl Pts',(-6.72446613966908,2.06488542585766,
-3.32137846589913));
#125716=CARTESIAN_POINT('',(-6.28381388945082,1.97432008626233,-3.85871525909399));
#125717=CARTESIAN_POINT('Origin',(-7.48099499014998E-13,2.06597317199967,
-4.36282954208167E-13));
#125718=CARTESIAN_POINT('',(-6.7237700463037,1.88359401261698,-3.32278743789529));
#125719=CARTESIAN_POINT('Origin',(0.161148139917844,2.01784564836717,0.103547310673459));
#125720=CARTESIAN_POINT('',(-6.95514688390034,1.97432008362734,-2.80640905739787));
#125721=CARTESIAN_POINT('Origin',(0.171998886078484,1.87500216690848,0.0865483033650638));
#125722=CARTESIAN_POINT('Origin',(0.176305524741013,2.01785750020066,0.0786696112267905));
#125723=CARTESIAN_POINT('Ctrl Pts',(-6.498970563,2.104810499,-3.213390985));
#125724=CARTESIAN_POINT('Ctrl Pts',(-6.673428112,2.039629277,-2.860556712));
#125725=CARTESIAN_POINT('Ctrl Pts',(-6.808661543,1.974320085,-2.490909068));
#125726=CARTESIAN_POINT('Ctrl Pts',(-6.61043810600001,2.104810499,-3.542895433));
#125727=CARTESIAN_POINT('Ctrl Pts',(-6.802784713,2.039629277,-3.184009497));
#125728=CARTESIAN_POINT('Ctrl Pts',(-6.955146889,1.974320085,-2.806409048));
#125729=CARTESIAN_POINT('',(-6.88190421143207,1.97432008293108,-2.64865906986868));
#125730=CARTESIAN_POINT('Ctrl Pts',(-6.79925019074248,1.96978752924164,
-2.51663409861818));
#125731=CARTESIAN_POINT('Ctrl Pts',(-6.80395586687118,1.97205380712079,
-2.50377158330912));
#125732=CARTESIAN_POINT('Ctrl Pts',(-6.80866154300001,1.974320085,-2.490909068));
#125733=CARTESIAN_POINT('Ctrl Pts',(-6.945154046,2.040055578,-2.117819875));
#125734=CARTESIAN_POINT('Ctrl Pts',(-7.040063948,2.104802836,-1.732050695));
#125735=CARTESIAN_POINT('Ctrl Pts',(-7.11595778587165,1.96978752924164,
-2.37104007871296));
#125736=CARTESIAN_POINT('Ctrl Pts',(-7.12038615790618,1.97205380712079,
-2.35758030613505));
#125737=CARTESIAN_POINT('Ctrl Pts',(-7.12481452994075,1.974320085,-2.34412053355715));
#125738=CARTESIAN_POINT('Ctrl Pts',(-7.25326357034823,2.040055578,-1.9537073392189));
#125739=CARTESIAN_POINT('Ctrl Pts',(-7.3382852704879,2.104802836,-1.55159674539325));
#125740=CARTESIAN_POINT('',(-7.12416152133647,1.97432008542256,-2.34442372779283));
#125741=CARTESIAN_POINT('',(-7.28125004982754,2.06488542555286,-1.79816503360501));
#125742=CARTESIAN_POINT('Origin',(0.173876656861732,1.87505112352018,0.0739675246104965));
#125743=CARTESIAN_POINT('Ctrl Pts',(-7.03893624352271,2.10403448598341,
-1.73662792835122));
#125744=CARTESIAN_POINT('Ctrl Pts',(-7.07925461425185,2.09719845379898,
-1.74691518076445));
#125745=CARTESIAN_POINT('Ctrl Pts',(-7.11962803445628,2.09052278112076,
-1.75719062130498));
#125746=CARTESIAN_POINT('Ctrl Pts',(-7.20038699405701,2.07748305173764,
-1.77769823778878));
#125747=CARTESIAN_POINT('Ctrl Pts',(-7.24081635312325,2.07111192519368,
-1.78794153699519));
#125748=CARTESIAN_POINT('Ctrl Pts',(-7.2812500490213,2.06488542585132,-1.79816503697546));
#125749=CARTESIAN_POINT('',(-6.966411530463,1.97432008626233,-2.41766640231028));
#125750=CARTESIAN_POINT('Origin',(8.06646416329215E-14,2.06597317199956,
8.67361737988404E-15));
#125751=CARTESIAN_POINT('',(-7.2808731171701,1.88359401257591,-1.79969070725037));
#125752=CARTESIAN_POINT('Origin',(0.179640001142697,2.01784567761325,0.0664842918032968));
#125753=CARTESIAN_POINT('',(-7.39583440602958,1.97432008362734,-1.24564578622645));
#125754=CARTESIAN_POINT('Origin',(0.186582973207047,1.87500218005872,0.0475501875908102));
#125755=CARTESIAN_POINT('Origin',(0.189095318358905,2.0178574927992,0.0389299101556073));
#125756=CARTESIAN_POINT('Ctrl Pts',(-7.037812317,2.104810499,-1.741177127));
#125757=CARTESIAN_POINT('Ctrl Pts',(-7.132342206,2.039629277,-1.359088706));
#125758=CARTESIAN_POINT('Ctrl Pts',(-7.184950639,1.974320085,-0.969012029));
#125759=CARTESIAN_POINT('Ctrl Pts',(-7.217507527,2.104810499,-2.039015717));
#125760=CARTESIAN_POINT('Ctrl Pts',(-7.32820731,2.039629277,-1.6471715));
#125761=CARTESIAN_POINT('Ctrl Pts',(-7.39583440900001,1.974320085,-1.245645776));
#125762=CARTESIAN_POINT('',(-7.29039252209028,1.97432008293108,-1.10732891507316));
#125763=CARTESIAN_POINT('Ctrl Pts',(-7.18128944022013,1.96978752940308,
-0.996158784306705));
#125764=CARTESIAN_POINT('Ctrl Pts',(-7.18312003961001,1.97205380720151,
-0.982585406653354));
#125765=CARTESIAN_POINT('Ctrl Pts',(-7.18495063900001,1.974320085,-0.969012029));
#125766=CARTESIAN_POINT('Ctrl Pts',(-7.238048875,2.040055578,-0.5753036));
#125767=CARTESIAN_POINT('Ctrl Pts',(-7.247810865,2.104802836,-0.178150666));
#125768=CARTESIAN_POINT('Ctrl Pts',(-7.45929417670702,1.96978752940307,
-0.785885901131069));
#125769=CARTESIAN_POINT('Ctrl Pts',(-7.46072556256693,1.97205380720151,
-0.771788841946397));
#125770=CARTESIAN_POINT('Ctrl Pts',(-7.46215694842695,1.974320085,-0.757691782761731));
#125771=CARTESIAN_POINT('Ctrl Pts',(-7.50367562510637,2.040055578,-0.348793484426639));
#125772=CARTESIAN_POINT('Ctrl Pts',(-7.50026767388759,2.104802836,0.0621931387486895));
#125773=CARTESIAN_POINT('',(-7.4615843846223,1.97432008542257,-0.75812826601158));
#125774=CARTESIAN_POINT('',(-7.4975707984158,2.06488542435384,-0.190871407260673));
#125775=CARTESIAN_POINT('Origin',(0.185712462960369,1.8750511548578,0.0348598629889121));
#125776=CARTESIAN_POINT('Ctrl Pts',(-7.24769349606498,2.10403448591232,
-0.182863309195361));
#125777=CARTESIAN_POINT('Ctrl Pts',(-7.28928070105476,2.09719845372094,
-0.184242793533437));
#125778=CARTESIAN_POINT('Ctrl Pts',(-7.33091912871676,2.09052278112048,
-0.185598908102442));
#125779=CARTESIAN_POINT('Ctrl Pts',(-7.41419852012812,2.07748305174943,
-0.18826627887279));
#125780=CARTESIAN_POINT('Ctrl Pts',(-7.45588466985395,2.0711119252019,-0.189578978335218));
#125781=CARTESIAN_POINT('Ctrl Pts',(-7.49757079858528,2.06488542588253,
-0.190871409159069));
#125782=CARTESIAN_POINT('',(-7.32326751109381,1.97432008626233,-0.86357015218475));
#125783=CARTESIAN_POINT('Ctrl Pts',(-7.24757379,2.104810499,-0.187547762));
#125784=CARTESIAN_POINT('Ctrl Pts',(-7.25775590700001,2.039629277,0.205928776));
#125785=CARTESIAN_POINT('Ctrl Pts',(-7.225279428,1.974320085,0.598194935));
#125786=CARTESIAN_POINT('Ctrl Pts',(-7.487094318,2.104810499,-0.439793892));
#125787=CARTESIAN_POINT('Ctrl Pts',(-7.510971078,2.039629277,-0.033313594));
#125788=CARTESIAN_POINT('Ctrl Pts',(-7.490700931,1.974320085,0.373362509));
#125789=CARTESIAN_POINT('',(-7.4907009161437,1.97432008293385,0.373362508483209));
#125790=CARTESIAN_POINT('Origin',(0.193037880697701,2.01785620729277,-0.00263048357573647));
#125791=CARTESIAN_POINT('',(-7.35799018033779,1.97432008293106,0.485778709310116));
#125792=CARTESIAN_POINT('Origin',(1.67097238823466E-12,2.06597317199989,
6.95515693649451E-14));
#125793=CARTESIAN_POINT('',(-7.49753065369832,1.88359401161432,-0.19244243844303));
#125794=CARTESIAN_POINT('Origin',(0.189732461945215,2.01784566286124,0.0263126490594483));
#125795=CARTESIAN_POINT('Origin',(0.19243733327029,1.87500051292121,0.00632878849069943));
#125796=CARTESIAN_POINT('Ctrl Pts',(-7.22753957590222,1.96978752942611,
0.570895806364564));
#125797=CARTESIAN_POINT('Ctrl Pts',(-7.22640950195114,1.97205380721309,
0.584545370682287));
#125798=CARTESIAN_POINT('Ctrl Pts',(-7.225279428,1.974320085,0.598194935));
#125799=CARTESIAN_POINT('Ctrl Pts',(-7.192500583,2.040055578,0.994113231));
#125800=CARTESIAN_POINT('Ctrl Pts',(-7.116658202,2.104802836,1.38407949));
#125801=CARTESIAN_POINT('Ctrl Pts',(-7.45384226286143,1.96978752942612,
0.836015428168855));
#125802=CARTESIAN_POINT('Ctrl Pts',(-7.4522097326846,1.97205380721309,0.850090611511704));
#125803=CARTESIAN_POINT('Ctrl Pts',(-7.45057720250766,1.974320085,0.864165794854558));
#125804=CARTESIAN_POINT('Ctrl Pts',(-7.40322414780391,2.040055578,1.27242956615732));
#125805=CARTESIAN_POINT('Ctrl Pts',(-7.31154589716983,2.104802836,1.67307494163324));
#125806=CARTESIAN_POINT('',(-7.45011185591378,1.97432008542257,0.863616432006661));
#125807=CARTESIAN_POINT('',(-7.337695642267,1.97432008626236,0.730905678799971));
#125808=CARTESIAN_POINT('',(-7.36331346990707,2.06488542554735,1.4253471567595));
#125809=CARTESIAN_POINT('Origin',(0.188864511309988,1.87505115067447,-0.00587784889222384));
#125810=CARTESIAN_POINT('Ctrl Pts',(-7.11755665585574,2.10403448593754,
1.37945179480568));
#125811=CARTESIAN_POINT('Ctrl Pts',(-7.15846812337888,2.09719845374601,
1.38704458172499));
#125812=CARTESIAN_POINT('Ctrl Pts',(-7.19942459243104,2.09052278110782,
1.39467120347564));
#125813=CARTESIAN_POINT('Ctrl Pts',(-7.28133036377528,2.07748305171712,
1.40996880174503));
#125814=CARTESIAN_POINT('Ctrl Pts',(-7.3223241059206,2.07111192517997,1.41764808240219));
#125815=CARTESIAN_POINT('Ctrl Pts',(-7.36331347059013,2.06488542584423,
1.42534715336305));
#125816=CARTESIAN_POINT('Origin',(7.27282817303276E-13,2.06597317200033,
-1.77321265310004E-13));
#125817=CARTESIAN_POINT('',(-7.23531060460637,1.97432008362732,1.97491276746511));
#125818=CARTESIAN_POINT('Origin',(0.18796447481838,2.01785751978077,-0.0440672207483484));
#125819=CARTESIAN_POINT('',(-7.36361198950017,1.88359401260101,1.423804222735));
#125820=CARTESIAN_POINT('Origin',(0.190953218088885,2.01784568550177,-0.0150894238754196));
#125821=CARTESIAN_POINT('Origin',(0.189303689485433,1.87500217028609,-0.035188726902253));
#125822=CARTESIAN_POINT('Ctrl Pts',(-7.118446767,2.104810499,1.374851129));
#125823=CARTESIAN_POINT('Ctrl Pts',(-7.043805007,2.039629277,1.761317258));
#125824=CARTESIAN_POINT('Ctrl Pts',(-6.927762182,1.974320085,2.137430969));
#125825=CARTESIAN_POINT('Ctrl Pts',(-7.4065929,2.104810499,1.179992206));
#125826=CARTESIAN_POINT('Ctrl Pts',(-7.342530186,2.039629277,1.582102018));
#125827=CARTESIAN_POINT('Ctrl Pts',(-7.235310603,1.974320085,1.974912778));
#125828=CARTESIAN_POINT('',(-7.08153639604613,1.97432008293108,2.05617186128699));
#125829=CARTESIAN_POINT('Ctrl Pts',(-6.93583799508597,1.96978752918469,
2.11125594238362));
#125830=CARTESIAN_POINT('Ctrl Pts',(-6.93180008854293,1.97205380709238,
2.12434345569181));
#125831=CARTESIAN_POINT('Ctrl Pts',(-6.927762182,1.974320085,2.137430969));
#125832=CARTESIAN_POINT('Ctrl Pts',(-6.810638957,2.040055578,2.517046433));
#125833=CARTESIAN_POINT('Ctrl Pts',(-6.652738511,2.104802836,2.881591627));
#125834=CARTESIAN_POINT('Ctrl Pts',(-7.09985696869169,1.96978752918469,
2.41882560241395));
#125835=CARTESIAN_POINT('Ctrl Pts',(-7.09523685758261,1.97205380709238,
2.43222077080092));
#125836=CARTESIAN_POINT('Ctrl Pts',(-7.09061674647364,1.974320085,2.44561593918789));
#125837=CARTESIAN_POINT('Ctrl Pts',(-6.95660613795933,2.040055578,2.8341552241412));
#125838=CARTESIAN_POINT('Ctrl Pts',(-6.78094436032466,2.104802836,3.20572561953813));
#125839=CARTESIAN_POINT('',(-7.09028037660616,1.97432008541402,2.44497938066934));
#125840=CARTESIAN_POINT('',(-6.88475578729827,2.06488542555484,2.97491807055449));
#125841=CARTESIAN_POINT('Origin',(0.183185163030007,1.87505116189093,-0.0463406174919131));
#125842=CARTESIAN_POINT('Ctrl Pts',(-6.65461077690117,2.10403448600761,
2.87726526592325));
#125843=CARTESIAN_POINT('Ctrl Pts',(-6.69293353219664,2.0971984538097,2.89347529398928));
#125844=CARTESIAN_POINT('Ctrl Pts',(-6.73129296363881,2.09052278114379,
2.90972803985757));
#125845=CARTESIAN_POINT('Ctrl Pts',(-6.80799529212629,2.07748305175425,
2.94227530853572));
#125846=CARTESIAN_POINT('Ctrl Pts',(-6.84637980517642,2.0711119251996,2.95858749470928));
#125847=CARTESIAN_POINT('Ctrl Pts',(-6.88475578868484,2.06488542586237,
2.97491806741338));
#125848=CARTESIAN_POINT('',(-7.00902128040429,1.97432008626232,2.29120517214505));
#125849=CARTESIAN_POINT('Origin',(6.34475111338517E-13,2.06597317200078,
-3.15285991758785E-13));
#125850=CARTESIAN_POINT('',(-6.88537901244729,1.88359401260015,2.97347538228458));
#125851=CARTESIAN_POINT('Origin',(0.18324471553533,2.01784562527804,-0.0557858145456952));
#125852=CARTESIAN_POINT('',(-6.6416051968254,1.97432008362727,3.48411831007128));
#125853=CARTESIAN_POINT('Origin',(0.177313480385554,1.87500217804533,-0.0750607933144437));
#125854=CARTESIAN_POINT('Origin',(0.174096740851528,2.01785756261903,-0.0834437133487326));
#125855=CARTESIAN_POINT('Ctrl Pts',(-6.656469085,2.104810499,2.872963509));
#125856=CARTESIAN_POINT('Ctrl Pts',(-6.50049361399999,2.039629277,3.234348502));
#125857=CARTESIAN_POINT('Ctrl Pts',(-6.306310476,1.974320085,3.576723107));
#125858=CARTESIAN_POINT('Ctrl Pts',(-6.97976743,2.104810499,2.744603181));
#125859=CARTESIAN_POINT('Ctrl Pts',(-6.830760744,2.039629277,3.123540298));
#125860=CARTESIAN_POINT('Ctrl Pts',(-6.641605193,1.974320085,3.48411832));
#125861=CARTESIAN_POINT('',(-6.47395784058873,1.97432008293106,3.53042070233472));
#125862=CARTESIAN_POINT('Ctrl Pts',(-6.31982433767558,1.96978752932471,
3.55289609980211));
#125863=CARTESIAN_POINT('Ctrl Pts',(-6.31306740683774,1.97205380716239,
3.56480960340106));
#125864=CARTESIAN_POINT('Ctrl Pts',(-6.306310476,1.974320085,3.576723107));
#125865=CARTESIAN_POINT('Ctrl Pts',(-6.110319423,2.040055578,3.922285341));
#125866=CARTESIAN_POINT('Ctrl Pts',(-5.877744161,2.104802836,4.244363742));
#125867=CARTESIAN_POINT('Ctrl Pts',(-6.41389025301481,1.96978752932471,
3.88853418294504));
#125868=CARTESIAN_POINT('Ctrl Pts',(-6.40649859251036,1.97205380716239,
3.90062299204184));
#125869=CARTESIAN_POINT('Ctrl Pts',(-6.39910693200597,1.974320085,3.9127118011387));
#125870=CARTESIAN_POINT('Ctrl Pts',(-6.18470495565525,2.040055578,4.26335893388342));
#125871=CARTESIAN_POINT('Ctrl Pts',(-5.9332734024071,2.104802836,4.58848012970813));
#125872=CARTESIAN_POINT('',(-6.39891526755264,1.97432008541402,3.91201781545349));
#125873=CARTESIAN_POINT('',(-6.08427457567457,2.0648854255748,4.38538512164169));
#125874=CARTESIAN_POINT('Origin',(0.168940651985443,1.87505118558091,-0.0846366779811158));
#125875=CARTESIAN_POINT('Ctrl Pts',(-5.88050269401229,2.10403448603753,
4.24054101089173));
#125876=CARTESIAN_POINT('Ctrl Pts',(-5.91444480773726,2.09719845385691,
4.26461031715442));
#125877=CARTESIAN_POINT('Ctrl Pts',(-5.94841355701859,2.09052278120813,
4.28872922672933));
#125878=CARTESIAN_POINT('Ctrl Pts',(-6.01632592706529,2.07748305181364,
4.33700429176202));
#125879=CARTESIAN_POINT('Ctrl Pts',(-6.050306393732,2.07111192524561,4.36118664380401));
#125880=CARTESIAN_POINT('Ctrl Pts',(-6.08427457769155,2.06488542589445,
4.38538511889264));
#125881=CARTESIAN_POINT('',(-6.35261287342917,1.97432008626232,3.74437045883386));
#125882=CARTESIAN_POINT('Origin',(3.33934269125535E-14,2.06597317200022,
-1.17093834628434E-13));
#125883=CARTESIAN_POINT('',(-6.08519336544764,1.88359401258516,4.38411013764511));
#125884=CARTESIAN_POINT('Origin',(0.16696819574831,2.01784563268764,-0.0938737286868618));
#125885=CARTESIAN_POINT('',(-5.73734571087834,1.97432008362714,4.83041035311533));
#125886=CARTESIAN_POINT('Origin',(0.157031971549915,1.87500216085911,-0.111422941102539));
#125887=CARTESIAN_POINT('Origin',(0.152088705016516,2.01785751253689,-0.118918655078524));
#125888=CARTESIAN_POINT('Ctrl Pts',(-5.88324230700001,2.104810499,4.236739308));
#125889=CARTESIAN_POINT('Ctrl Pts',(-5.653226364,2.039629277,4.556145206));
#125890=CARTESIAN_POINT('Ctrl Pts',(-5.3899827,1.974320085,4.848771648));
#125891=CARTESIAN_POINT('Ctrl Pts',(-6.22657579300001,2.104810499,4.180879561));
#125892=CARTESIAN_POINT('Ctrl Pts',(-5.99959252,2.039629277,4.518925306));
#125893=CARTESIAN_POINT('Ctrl Pts',(-5.737345705,1.974320085,4.830410362));
#125894=CARTESIAN_POINT('',(-5.5636642108475,1.97432008293083,4.8395909954036));
#125895=CARTESIAN_POINT('Ctrl Pts',(-5.40830271781122,1.96978752917624,
4.82840678318885));
#125896=CARTESIAN_POINT('Ctrl Pts',(-5.39914270890567,1.97205380708815,
4.83858921559444));
#125897=CARTESIAN_POINT('Ctrl Pts',(-5.3899827,1.974320085,4.848771648));
#125898=CARTESIAN_POINT('Ctrl Pts',(-5.12428814500001,2.040055578,5.144122545));
#125899=CARTESIAN_POINT('Ctrl Pts',(-4.827913027,2.104802836,5.408674126));
#125900=CARTESIAN_POINT('Ctrl Pts',(-5.42801715832236,1.96978752917623,
5.17641922496828));
#125901=CARTESIAN_POINT('Ctrl Pts',(-5.41819957382225,1.97205380708815,
5.18663641624999));
#125902=CARTESIAN_POINT('Ctrl Pts',(-5.40838198932213,1.974320085,5.1968536075316));
#125903=CARTESIAN_POINT('Ctrl Pts',(-5.12361384424682,2.040055578,5.493212717974));
#125904=CARTESIAN_POINT('Ctrl Pts',(-4.80816917351054,2.104802836,5.7566824093551));
#125905=CARTESIAN_POINT('',(-5.40834399228508,1.97432008541403,5.19613464466293));
#125906=CARTESIAN_POINT('',(-4.99929944699896,2.0648854255675,5.59079643827862));
#125907=CARTESIAN_POINT('Origin',(0.146796408726788,1.87505116076644,-0.1189750306459));
#125908=CARTESIAN_POINT('Ctrl Pts',(-4.83142884124745,2.10403448603426,
5.40553377141309));
#125909=CARTESIAN_POINT('Ctrl Pts',(-4.85940321785624,2.09719845384183,
5.43633690176658));
#125910=CARTESIAN_POINT('Ctrl Pts',(-4.88739294396725,2.09052278119847,
5.46719420155808));
#125911=CARTESIAN_POINT('Ctrl Pts',(-4.94333984845768,2.07748305180029,
5.52893977444882));
#125912=CARTESIAN_POINT('Ctrl Pts',(-4.97132737977632,2.0711119252313,5.55986155241276));
#125913=CARTESIAN_POINT('Ctrl Pts',(-4.99929944955791,2.06488542588397,
5.59079643602845));
#125914=CARTESIAN_POINT('',(-5.39916334827033,1.97432008626232,5.02245314433436));
#125915=CARTESIAN_POINT('Origin',(-5.5424415057459E-13,2.065973171999,6.82180006927879E-13));
#125916=CARTESIAN_POINT('',(-5.00047084026875,1.88359401262509,5.58974877539356));
#125917=CARTESIAN_POINT('Origin',(0.14288452164617,2.01784567409964,-0.127572246574718));
#125918=CARTESIAN_POINT('',(-4.56481431668053,1.97432008362732,5.95083777557622));
#125919=CARTESIAN_POINT('Origin',(0.129407994727996,1.87500218148817,-0.142575166280723));
#125920=CARTESIAN_POINT('Origin',(0.12296869673353,2.01785750439565,-0.148832672745743));
#125921=CARTESIAN_POINT('Ctrl Pts',(-4.834921657,2.104810499,5.402409886));
#125922=CARTESIAN_POINT('Ctrl Pts',(-4.541620533,2.039629277,5.664901623));
#125923=CARTESIAN_POINT('Ctrl Pts',(-4.221625324,1.974320085,5.894097015));
#125924=CARTESIAN_POINT('Ctrl Pts',(-5.182236391,2.104810499,5.421662659));
#125925=CARTESIAN_POINT('Ctrl Pts',(-4.887890019,2.039629277,5.70301038900001));
#125926=CARTESIAN_POINT('Ctrl Pts',(-4.564814309,1.974320085,5.950837783));
#125927=CARTESIAN_POINT('',(-4.39321982671405,1.97432008293108,5.92246739142333));
#125928=CARTESIAN_POINT('Ctrl Pts',(-4.24389487418159,1.96978752913463,
5.87814653153815));
#125929=CARTESIAN_POINT('Ctrl Pts',(-4.23276009909078,1.97205380706735,
5.88612177326912));
#125930=CARTESIAN_POINT('Ctrl Pts',(-4.221625324,1.974320085,5.894097015));
#125931=CARTESIAN_POINT('Ctrl Pts',(-3.898650847,2.040055578,6.125426297));
#125932=CARTESIAN_POINT('Ctrl Pts',(-3.552334045,2.104802836,6.32008092));
#125933=CARTESIAN_POINT('Ctrl Pts',(-4.18833601474106,1.96978752913463,
6.22226065806384));
#125934=CARTESIAN_POINT('Ctrl Pts',(-4.17655156568981,1.97205380706735,
6.23012848670628));
#125935=CARTESIAN_POINT('Ctrl Pts',(-4.1647671166385,1.974320085,6.23799631534876));
#125936=CARTESIAN_POINT('Ctrl Pts',(-3.82294824395876,2.040055578,6.46620998111279));
#125937=CARTESIAN_POINT('Ctrl Pts',(-3.4582402984613,2.104802836,6.6557086175373));
#125938=CARTESIAN_POINT('',(-4.16488456114592,1.97432008542257,6.23728599583473));
#125939=CARTESIAN_POINT('',(-3.6805626329654,2.06488542554733,6.5347883272354));
#125940=CARTESIAN_POINT('Origin',(0.117788238628589,1.87505116461688,-0.147750294515482));
#125941=CARTESIAN_POINT('Ctrl Pts',(-3.55644274524795,2.10403448598181,
6.31776978077794));
#125942=CARTESIAN_POINT('Ctrl Pts',(-3.57714133401449,2.09719845378938,
6.35386641504643));
#125943=CARTESIAN_POINT('Ctrl Pts',(-3.59784326874741,2.09052278111202,
6.39001925219844));
#125944=CARTESIAN_POINT('Ctrl Pts',(-3.63920869287107,2.07748305173078,
6.46234817845479));
#125945=CARTESIAN_POINT('Ctrl Pts',(-3.65989462309973,2.07111192518344,
6.49856351423839));
#125946=CARTESIAN_POINT('Ctrl Pts',(-3.68056263598081,2.06488542584907,
6.53478832556683));
#125947=CARTESIAN_POINT('',(-4.19325494636506,1.97432008626232,6.06569150259979));
#125948=CARTESIAN_POINT('Origin',(-2.54787510534094E-13,2.06597317199889,
4.4799233767101E-13));
#125949=CARTESIAN_POINT('',(-3.68193185568052,1.88359401262617,6.53401697296669));
#125950=CARTESIAN_POINT('Origin',(0.112119777202641,2.01784565321898,-0.155305776233697));
#125951=CARTESIAN_POINT('',(-3.17883727810966,1.97432008362732,6.79301063840171));
#125952=CARTESIAN_POINT('Origin',(0.0957330760861524,1.87500219779642,-0.167060764696217));
#125953=CARTESIAN_POINT('Origin',(0.0880991938531066,2.01785752956562,-0.171787801691451));
#125954=CARTESIAN_POINT('Ctrl Pts',(-3.560525444,2.104810499,6.315469782));
#125955=CARTESIAN_POINT('Ctrl Pts',(-3.217653573,2.039629277,6.508773536));
#125956=CARTESIAN_POINT('Ctrl Pts',(-2.85586944,1.974320085,6.663820956));
#125957=CARTESIAN_POINT('Ctrl Pts',(-3.895581376,2.104810499,6.408934837));
#125958=CARTESIAN_POINT('Ctrl Pts',(-3.547635213,2.039629277,6.62042904400001));
#125959=CARTESIAN_POINT('Ctrl Pts',(-3.178837269,1.974320085,6.793010644));
#125960=CARTESIAN_POINT('',(-3.01735336610401,1.97432008293108,6.72841579479619));
#125961=CARTESIAN_POINT('Ctrl Pts',(-2.88104722229099,1.96978752923893,
6.65303068119339));
#125962=CARTESIAN_POINT('Ctrl Pts',(-2.86845833114553,1.9720538071195,6.65842581859663));
#125963=CARTESIAN_POINT('Ctrl Pts',(-2.85586944,1.974320085,6.663820956));
#125964=CARTESIAN_POINT('Ctrl Pts',(-2.49071697,2.040055578,6.82031192300001));
#125965=CARTESIAN_POINT('Ctrl Pts',(-2.110651872,2.104802836,6.935967753));
#125966=CARTESIAN_POINT('Ctrl Pts',(-2.7528129322015,1.96978752923893,6.97715609885582));
#125967=CARTESIAN_POINT('Ctrl Pts',(-2.73961264674685,1.9720538071195,6.98230667369879));
#125968=CARTESIAN_POINT('Ctrl Pts',(-2.72641236129213,1.974320085,6.9874572485419));
#125969=CARTESIAN_POINT('Ctrl Pts',(-2.34352583198828,2.040055578,7.13685445153059));
#125970=CARTESIAN_POINT('Ctrl Pts',(-1.94660795094088,2.104802836,7.24352128796493));
#125971=CARTESIAN_POINT('',(-2.72667975770036,1.97432008542256,6.98678878301995));
#125972=CARTESIAN_POINT('',(-2.18972680033077,2.06488542555802,7.17322077696606));
#125973=CARTESIAN_POINT('Origin',(0.0832725217709313,1.87505115884544,-0.169617116136719));
#125974=CARTESIAN_POINT('Ctrl Pts',(-2.11516133959159,2.10403448594589,
6.93459389664791));
#125975=CARTESIAN_POINT('Ctrl Pts',(-2.12761629754393,2.09719845375242,
6.97429619653596));
#125976=CARTESIAN_POINT('Ctrl Pts',(-2.14006244105225,2.09052278115065,
7.0140541040936));
#125977=CARTESIAN_POINT('Ctrl Pts',(-2.16491218327615,2.07748305176128,
7.09358436382901));
#125978=CARTESIAN_POINT('Ctrl Pts',(-2.17732926116173,2.07111192520406,
7.13339986879836));
#125979=CARTESIAN_POINT('Ctrl Pts',(-2.18972680358998,2.06488542587125,
7.17322077600033));
#125980=CARTESIAN_POINT('',(-2.79127460316217,1.97432008626232,6.82530486757097));
#125981=CARTESIAN_POINT('Origin',(-4.86481514794246E-13,2.06597317199956,
1.71217207078911E-12));
#125982=CARTESIAN_POINT('',(-2.19122982986192,1.88359401259214,7.17276179905091));
#125983=CARTESIAN_POINT('Origin',(0.0761123067457722,2.01784568248533,-0.17577716954979));
#125984=CARTESIAN_POINT('',(-1.6442213420479,1.97432008362732,7.31754987448154));
#125985=CARTESIAN_POINT('Origin',(0.0575818226720837,1.87500221280571,-0.183734943946949));
#125986=CARTESIAN_POINT('Origin',(0.0491101563790857,2.01785750222948,-0.186710084026774));
#125987=CARTESIAN_POINT('Ctrl Pts',(-2.119643019,2.104810499,6.93322533));
#125988=CARTESIAN_POINT('Ctrl Pts',(-1.743232708,2.039629277,7.048302433));
#125989=CARTESIAN_POINT('Ctrl Pts',(-1.356576276,1.974320085,7.121952036));
#125990=CARTESIAN_POINT('Ctrl Pts',(-2.426773305,2.104810499,7.096532345));
#125991=CARTESIAN_POINT('Ctrl Pts',(-2.041496927,2.039629277,7.228283796));
#125992=CARTESIAN_POINT('Ctrl Pts',(-1.644221332,1.974320085,7.317549878));
#125993=CARTESIAN_POINT('',(-1.50039881645138,1.97432008293108,7.21975095441237));
#125994=CARTESIAN_POINT('Ctrl Pts',(-1.38348500528046,1.96978752935668,
7.11682651089333));
#125995=CARTESIAN_POINT('Ctrl Pts',(-1.37003064064024,1.97205380717837,
7.11938927344667));
#125996=CARTESIAN_POINT('Ctrl Pts',(-1.356576276,1.974320085,7.121952036));
#125997=CARTESIAN_POINT('Ctrl Pts',(-0.966319934,2.040055578,7.196287344));
#125998=CARTESIAN_POINT('Ctrl Pts',(-0.570277963,2.104802836,7.227536444));
#125999=CARTESIAN_POINT('Ctrl Pts',(-1.18857137701003,1.96978752935668,
7.40580747507847));
#126000=CARTESIAN_POINT('Ctrl Pts',(-1.17457248592774,1.97205380717837,
7.40799996110077));
#126001=CARTESIAN_POINT('Ctrl Pts',(-1.1605735948454,1.974320085,7.41019244712308));
#126002=CARTESIAN_POINT('Ctrl Pts',(-0.75452275766884,2.040055578,7.47378754044986));
#126003=CARTESIAN_POINT('Ctrl Pts',(-0.343954378698039,2.104802836,7.49263495404393));
#126004=CARTESIAN_POINT('',(-1.16097844002199,1.97432008542257,7.40959709227556));
#126005=CARTESIAN_POINT('',(-0.59650177670354,2.0648854255752,7.47624139567281));
#126006=CARTESIAN_POINT('Origin',(0.0448629872232868,1.87505114104151,-0.183552688534319));
#126007=CARTESIAN_POINT('Ctrl Pts',(-0.574977340857676,2.10403448596467,
7.22716410902309));
#126008=CARTESIAN_POINT('Ctrl Pts',(-0.578606266727296,2.09719849327752,
7.26861539947383));
#126009=CARTESIAN_POINT('Ctrl Pts',(-0.582214628220441,2.09052286129755,
7.31011907167483));
#126010=CARTESIAN_POINT('Ctrl Pts',(-0.589386786364929,2.07748305174417,
7.39313242856107));
#126011=CARTESIAN_POINT('Ctrl Pts',(-0.592954403264341,2.07111192522242,
7.43468637364651));
#126012=CARTESIAN_POINT('Ctrl Pts',(-0.596501780179169,2.06488542587664,
7.47624139542128));
#126013=CARTESIAN_POINT('',(-1.25877736262437,1.97432008626232,7.2657745631791));
#126014=CARTESIAN_POINT('Origin',(4.55364912443912E-14,2.06597317199933,
-1.16486681411843E-12));
#126015=CARTESIAN_POINT('',(-0.598068333136003,1.8835940126128,7.47611625540618));
#126016=CARTESIAN_POINT('Origin',(0.0365459521448464,2.01784563964012,-0.188029636822713));
#126017=CARTESIAN_POINT('',(-0.0327234426157351,1.97432008362731,7.49992860974549));
#126018=CARTESIAN_POINT('Origin',(0.016738008922914,1.87500216842685,-0.191817838129081));
#126019=CARTESIAN_POINT('Origin',(0.00782484507779792,2.01785753732395,
-0.192902388630886));
#126020=CARTESIAN_POINT('Ctrl Pts',(-0.579648442,2.104810499,7.226790967));
#126021=CARTESIAN_POINT('Ctrl Pts',(-0.18730022,2.039629277,7.258260542));
#126022=CARTESIAN_POINT('Ctrl Pts',(0.206148888,1.974320085,7.247068555));
#126023=CARTESIAN_POINT('Ctrl Pts',(-0.844492011,2.104810499,7.452303888));
#126024=CARTESIAN_POINT('Ctrl Pts',(-0.439900514,2.039629277,7.49815203));
#126025=CARTESIAN_POINT('Ctrl Pts',(-0.032723432,1.974320085,7.499928611));
#126026=CARTESIAN_POINT('',(0.0867127152835091,1.97432008293108,7.37349858314955));
#126027=CARTESIAN_POINT('Ctrl Pts',(-1.641510318,3.783915088,7.318158503));
#126028=CARTESIAN_POINT('Ctrl Pts',(-1.24377052,3.848090541,7.407374114));
#126029=CARTESIAN_POINT('Ctrl Pts',(-0.838704438,3.913265985,7.452957458));
#126030=CARTESIAN_POINT('Ctrl Pts',(-0.834644171981073,3.91391928492389,
7.45341437234286));
#126031=CARTESIAN_POINT('Ctrl Pts',(-0.830583905962144,3.91457258484778,
7.45387128668572));
#126032=CARTESIAN_POINT('Ctrl Pts',(-1.353937744,3.783915088,7.122454113));
#126033=CARTESIAN_POINT('Ctrl Pts',(-0.966834423,3.848090541,7.196040237));
#126034=CARTESIAN_POINT('Ctrl Pts',(-0.574036077,3.913265985,7.227238932));
#126035=CARTESIAN_POINT('Ctrl Pts',(-0.570098779241866,3.91391928492389,
7.2275516587544));
#126036=CARTESIAN_POINT('Ctrl Pts',(-0.56616148148373,3.91457258484778,
7.22786438550881));
#126037=CARTESIAN_POINT('',(-0.838704432778282,3.9132659845887,7.45295745868655));
#126038=CARTESIAN_POINT('',(-0.706370249897001,3.91326598377978,7.34009819573167));
#126039=CARTESIAN_POINT('',(-1.39529141150652,3.82362522065936,7.36906791091339));
#126040=CARTESIAN_POINT('Origin',(0.00437564016434397,4.01780065316102,
-0.188625706529489));
#126041=CARTESIAN_POINT('Ctrl Pts',(-1.34934427444366,3.78467661296189,
7.12332577189278));
#126042=CARTESIAN_POINT('Ctrl Pts',(-1.35687852219608,3.79148857314734,
7.16424520945549));
#126043=CARTESIAN_POINT('Ctrl Pts',(-1.36448261962806,3.79813536725102,
7.20520610145691));
#126044=CARTESIAN_POINT('Ctrl Pts',(-1.37979916234012,3.81110763474039,
7.28710522003744));
#126045=CARTESIAN_POINT('Ctrl Pts',(-1.38752070317403,3.81744080403857,
7.32809204393903));
#126046=CARTESIAN_POINT('Ctrl Pts',(-1.39529141290873,3.82362522065907,
7.36906791064074));
#126047=CARTESIAN_POINT('Ctrl Pts',(-1.95071269,3.913265985,7.241872686));
#126048=CARTESIAN_POINT('Ctrl Pts',(-1.887862343,3.903042157,7.258802419));
#126049=CARTESIAN_POINT('Ctrl Pts',(-1.824727629,3.892857143,7.274638759));
#126050=CARTESIAN_POINT('Ctrl Pts',(-1.48981453,3.838828313,7.358646393));
#126051=CARTESIAN_POINT('Ctrl Pts',(-1.148599349,3.783894965,7.411526127));
#126052=CARTESIAN_POINT('Ctrl Pts',(-2.114258167,3.913265985,6.934869314));
#126053=CARTESIAN_POINT('Ctrl Pts',(-2.054072224,3.903042157,6.95321841600001));
#126054=CARTESIAN_POINT('Ctrl Pts',(-1.993576877,3.892857143,6.970520155));
#126055=CARTESIAN_POINT('Ctrl Pts',(-1.672664928,3.838828313,7.06230134600001));
#126056=CARTESIAN_POINT('Ctrl Pts',(-1.344677418,3.783894965,7.124208212));
#126057=CARTESIAN_POINT('',(-1.95071268475464,3.91326598587933,7.24187268671574));
#126058=CARTESIAN_POINT('Ctrl Pts',(-1.39529140955773,3.82362522012815,
7.36906791137212));
#126059=CARTESIAN_POINT('Ctrl Pts',(-1.53971171293186,3.8468929357324,7.34172274220185));
#126060=CARTESIAN_POINT('Ctrl Pts',(-1.68297367235439,3.86998912007469,
7.31019548872055));
#126061=CARTESIAN_POINT('Ctrl Pts',(-1.82472762875061,3.89285714276327,
7.27463875947624));
#126062=CARTESIAN_POINT('Ctrl Pts',(-1.86677632062748,3.89964051914521,
7.26409151275274));
#126063=CARTESIAN_POINT('Ctrl Pts',(-1.90877464357573,3.90644394874722,
7.25316936065063));
#126064=CARTESIAN_POINT('Ctrl Pts',(-1.95071268604322,3.91326598565651,
7.24187268712382));
#126065=CARTESIAN_POINT('',(-2.03248542073876,3.91326598631302,7.08837100222542));
#126066=CARTESIAN_POINT('Origin',(2.18954628733448E-13,4.00453392000067,
-1.05080874557295E-12));
#126067=CARTESIAN_POINT('',(-1.40235121259848,4.0034549417923,7.36772767361413));
#126068=CARTESIAN_POINT('Origin',(0.058873471497646,4.16057200915549,-0.175368207921701));
#126069=CARTESIAN_POINT('Origin',(0.0336955573596309,4.01785438784316,-0.189448533857115));
#126070=CARTESIAN_POINT('Ctrl Pts',(-3.17697582940556,3.783915088,6.79445025702659));
#126071=CARTESIAN_POINT('Ctrl Pts',(-2.80769942346504,3.848090541,6.96711797440197));
#126072=CARTESIAN_POINT('Ctrl Pts',(-2.42188459324435,3.913265985,7.09874670216657));
#126073=CARTESIAN_POINT('Ctrl Pts',(-2.40874325520729,3.91548594253982,
7.10323014207464));
#126074=CARTESIAN_POINT('Ctrl Pts',(-2.39560191717029,3.91770590007956,
7.10771358198274));
#126075=CARTESIAN_POINT('Ctrl Pts',(-2.853400528,3.783915088,6.6648785));
#126076=CARTESIAN_POINT('Ctrl Pts',(-2.491166309,3.848090541,6.819959994));
#126077=CARTESIAN_POINT('Ctrl Pts',(-2.114258167,3.913265985,6.934869314));
#126078=CARTESIAN_POINT('Ctrl Pts',(-2.10142020195832,3.91548594253982,
6.93878326986547));
#126079=CARTESIAN_POINT('Ctrl Pts',(-2.08858223691657,3.91770590007957,
6.94269722573092));
#126080=CARTESIAN_POINT('',(-2.42126153214055,3.91326598502339,7.09841479422943));
#126081=CARTESIAN_POINT('',(-2.26775984623204,3.91326598377978,7.01664205534898));
#126082=CARTESIAN_POINT('',(-2.94680204673062,3.82362522067675,6.89683678909558));
#126083=CARTESIAN_POINT('Origin',(0.0448223164287281,4.0178006398365,-0.183275168909287));
#126084=CARTESIAN_POINT('Ctrl Pts',(-2.84910183290045,3.78467661312367,
6.6667172412568));
#126085=CARTESIAN_POINT('Ctrl Pts',(-2.86525640352458,3.79148857330945,
6.7050603647789));
#126086=CARTESIAN_POINT('Ctrl Pts',(-2.88148810208281,3.7981353673104,6.74342895726899));
#126087=CARTESIAN_POINT('Ctrl Pts',(-2.9140524396325,3.81110763381503,6.8201207104001));
#126088=CARTESIAN_POINT('Ctrl Pts',(-2.93040440790468,3.8174408020963,6.85848937555338));
#126089=CARTESIAN_POINT('Ctrl Pts',(-2.94680204808744,3.82362522067661,
6.89683678851494));
#126090=CARTESIAN_POINT('Ctrl Pts',(-3.46189467,3.913265985,6.653216162));
#126091=CARTESIAN_POINT('Ctrl Pts',(-3.404153122,3.903042157,6.683261053));
#126092=CARTESIAN_POINT('Ctrl Pts',(-3.345898807,3.892857143,6.712299246));
#126093=CARTESIAN_POINT('Ctrl Pts',(-3.036874949,3.838828313,6.866339244));
#126094=CARTESIAN_POINT('Ctrl Pts',(-2.715004769,3.783894965,6.991333857));
#126095=CARTESIAN_POINT('Ctrl Pts',(-3.555619896,3.913265985,6.318232914));
#126096=CARTESIAN_POINT('Ctrl Pts',(-3.500785581,3.903042157,6.34909122300001));
#126097=CARTESIAN_POINT('Ctrl Pts',(-3.445423944,3.892857143,6.378993169));
#126098=CARTESIAN_POINT('Ctrl Pts',(-3.15174498,3.838828313,6.53761515));
#126099=CARTESIAN_POINT('Ctrl Pts',(-2.844733783,3.783894965,6.668582286));
#126100=CARTESIAN_POINT('',(-3.46189466553809,3.9132659854451,6.65321616350949));
#126101=CARTESIAN_POINT('Ctrl Pts',(-2.946802044864,3.82362522012809,6.89683678997819));
#126102=CARTESIAN_POINT('Ctrl Pts',(-3.0819674786481,3.84689293573234,6.83908483956707));
#126103=CARTESIAN_POINT('Ctrl Pts',(-3.2151026252374,3.86998912007487,6.77749758928962));
#126104=CARTESIAN_POINT('Ctrl Pts',(-3.34589880719272,3.89285714303369,
6.71229924590394));
#126105=CARTESIAN_POINT('Ctrl Pts',(-3.38469707799573,3.89964051918897,
6.69295936222793));
#126106=CARTESIAN_POINT('Ctrl Pts',(-3.42336556352837,3.90644394833732,
6.67326416630459));
#126107=CARTESIAN_POINT('Ctrl Pts',(-3.46189466668291,3.91326598441267,
6.653216163726));
#126108=CARTESIAN_POINT('',(-3.50875727589861,3.91326598631302,6.48572454184184));
#126109=CARTESIAN_POINT('Origin',(4.07009495551058E-13,4.00453392000044,
-9.09428782280841E-13));
#126110=CARTESIAN_POINT('',(-2.95340868202953,4.00345494158478,6.89401023776217));
#126111=CARTESIAN_POINT('Origin',(0.0951960599535917,4.16057204517788,-0.158612234165763));
#126112=CARTESIAN_POINT('Origin',(0.0736336047404013,4.0178542574278,-0.177775727115013));
#126113=CARTESIAN_POINT('Ctrl Pts',(-4.56330586299524,3.783915088,5.95264389353416));
#126114=CARTESIAN_POINT('Ctrl Pts',(-4.23978138941415,3.848090541,6.2006582472807));
#126115=CARTESIAN_POINT('Ctrl Pts',(-3.89128298043124,3.913265985,6.41214835224929));
#126116=CARTESIAN_POINT('Ctrl Pts',(-3.8794126874205,3.91548594238702,6.41935197054465));
#126117=CARTESIAN_POINT('Ctrl Pts',(-3.86754239440971,3.91770589977398,
6.42655558883999));
#126118=CARTESIAN_POINT('Ctrl Pts',(-4.219441475,3.783915088,5.895660577));
#126119=CARTESIAN_POINT('Ctrl Pts',(-3.899014027,3.848090541,6.124986001));
#126120=CARTESIAN_POINT('Ctrl Pts',(-3.555619896,3.913265985,6.318232914));
#126121=CARTESIAN_POINT('Ctrl Pts',(-3.54392346110081,3.91548594238702,
6.32481514629033));
#126122=CARTESIAN_POINT('Ctrl Pts',(-3.53222702620162,3.91770589977399,
6.33139737858057));
#126123=CARTESIAN_POINT('',(-3.89060313579128,3.91326598502339,6.41195814384659));
#126124=CARTESIAN_POINT('',(-3.72311151290693,3.91326598377978,6.36509553085646));
#126125=CARTESIAN_POINT('',(-4.36052349282626,3.82362522064783,6.10211724455119));
#126126=CARTESIAN_POINT('Origin',(0.0831729945559451,4.01780058964706,-0.169354587059151));
#126127=CARTESIAN_POINT('Ctrl Pts',(-4.21563855520111,3.78467661323922,
5.89838042225523));
#126128=CARTESIAN_POINT('Ctrl Pts',(-4.23965807938136,3.79148857344083,
5.9323543498312));
#126129=CARTESIAN_POINT('Ctrl Pts',(-4.2637584026862,3.79813536730393,5.96633656991507));
#126130=CARTESIAN_POINT('Ctrl Pts',(-4.31204787018211,3.81110763542439,
6.03423495106847));
#126131=CARTESIAN_POINT('Ctrl Pts',(-4.33626567407951,3.81744080533757,
6.06819139775185));
#126132=CARTESIAN_POINT('Ctrl Pts',(-4.36052349394067,3.82362522064755,
6.10211724370674));
#126133=CARTESIAN_POINT('Ctrl Pts',(-4.811202304,3.913265985,5.753462644));
#126134=CARTESIAN_POINT('Ctrl Pts',(-4.761269485,3.903042157,5.795217828));
#126135=CARTESIAN_POINT('Ctrl Pts',(-4.710619476,3.892857143,5.83610008));
#126136=CARTESIAN_POINT('Ctrl Pts',(-4.44193447,3.838828313,6.052969703));
#126137=CARTESIAN_POINT('Ctrl Pts',(-4.154459583,3.783894965,6.244234587));
#126138=CARTESIAN_POINT('Ctrl Pts',(-4.830724789,3.913265985,5.406162966));
#126139=CARTESIAN_POINT('Ctrl Pts',(-4.783806095,3.903042157,5.448087581));
#126140=CARTESIAN_POINT('Ctrl Pts',(-4.736166816,3.892857143,5.489191552));
#126141=CARTESIAN_POINT('Ctrl Pts',(-4.483452941,3.838828313,5.707237335));
#126142=CARTESIAN_POINT('Ctrl Pts',(-4.211773557,3.783894965,5.901140864));
#126143=CARTESIAN_POINT('',(-4.81120229945886,3.9132659858793,5.75346264667725));
#126144=CARTESIAN_POINT('Ctrl Pts',(-4.36052349132177,3.82362522012809,
6.1021172458116));
#126145=CARTESIAN_POINT('Ctrl Pts',(-4.48011387030856,3.84689293573233,
6.01665893095114));
#126146=CARTESIAN_POINT('Ctrl Pts',(-4.59689695300997,3.86998912007465,
5.92789143529639));
#126147=CARTESIAN_POINT('Ctrl Pts',(-4.71061947665133,3.89285714276327,
5.8361000802071));
#126148=CARTESIAN_POINT('Ctrl Pts',(-4.74435316195801,3.89964051914521,
5.80887187081367));
#126149=CARTESIAN_POINT('Ctrl Pts',(-4.7778837148795,3.90644394874722,5.78132455595175));
#126150=CARTESIAN_POINT('Ctrl Pts',(-4.81120230059236,3.91326598565651,
5.75346264633524));
#126151=CARTESIAN_POINT('',(-4.82096354039051,3.91326598631302,5.5798128102786));
#126152=CARTESIAN_POINT('Origin',(-7.63712010298789E-13,4.00453391999933,
1.09677891768634E-12));
#126153=CARTESIAN_POINT('',(-4.36636804460132,4.00345494180093,6.09793654434491));
#126154=CARTESIAN_POINT('Origin',(0.12706732881094,4.16057201538049,-0.134439565904996));
#126155=CARTESIAN_POINT('Origin',(0.110128494847791,4.01785439830898,-0.157790259172783));
#126156=CARTESIAN_POINT('Ctrl Pts',(-5.73626078558308,3.783915088,4.83249851653824));
#126157=CARTESIAN_POINT('Ctrl Pts',(-5.47361588965722,3.848090541,5.14426263175883));
#126158=CARTESIAN_POINT('Ctrl Pts',(-5.17872930030728,3.913265985,5.4257250712431));
#126159=CARTESIAN_POINT('Ctrl Pts',(-5.16868509190111,3.91548594265879,
5.43531203620788));
#126160=CARTESIAN_POINT('Ctrl Pts',(-5.15864088349497,3.91770590031752,
5.44489900117279));
#126161=CARTESIAN_POINT('Ctrl Pts',(-5.38818602700001,3.783915088,4.850768118));
#126162=CARTESIAN_POINT('Ctrl Pts',(-5.124548183,3.848090541,5.14361447));
#126163=CARTESIAN_POINT('Ctrl Pts',(-4.830724789,3.913265985,5.406162966));
#126164=CARTESIAN_POINT('Ctrl Pts',(-4.82071679436569,3.91548594265879,
5.41510569824279));
#126165=CARTESIAN_POINT('Ctrl Pts',(-4.81070879973142,3.91770590031752,
5.4240484304857));
#126166=CARTESIAN_POINT('',(-5.17802446096145,3.91326598502339,5.42568545648943));
#126167=CARTESIAN_POINT('',(-5.00437462239009,3.91326598377978,5.41592421368362));
#126168=CARTESIAN_POINT('',(-5.57035170717127,3.82362522068455,5.02206947957131));
#126169=CARTESIAN_POINT('Origin',(0.117634589582996,4.01780062259429,-0.14751536631502));
#126170=CARTESIAN_POINT('Ctrl Pts',(-5.38505670344997,3.78467661305223,
4.85424188932103));
#126171=CARTESIAN_POINT('Ctrl Pts',(-5.41581805460382,3.7914885732252,4.8822580373369));
#126172=CARTESIAN_POINT('Ctrl Pts',(-5.44666009944762,3.79813536727438,
4.91026491555166));
#126173=CARTESIAN_POINT('Ctrl Pts',(-5.50841686742267,3.81110766406195,
4.96619518564335));
#126174=CARTESIAN_POINT('Ctrl Pts',(-5.53936826028539,3.81744086358108,
4.99415177693172));
#126175=CARTESIAN_POINT('Ctrl Pts',(-5.57035170819594,3.8236252206782,5.02206947843552));
#126176=CARTESIAN_POINT('Ctrl Pts',(-5.935543465,3.913265985,4.584683607));
#126177=CARTESIAN_POINT('Ctrl Pts',(-5.895754178,3.903042157,4.636196659));
#126178=CARTESIAN_POINT('Ctrl Pts',(-5.855076814,3.892857143,4.687011361));
#126179=CARTESIAN_POINT('Ctrl Pts',(-5.639294072,3.838828313,4.956570027));
#126180=CARTESIAN_POINT('Ctrl Pts',(-5.399656485,3.783894965,5.205161847));
#126181=CARTESIAN_POINT('Ctrl Pts',(-5.879950361,3.913265985,4.241306845));
#126182=CARTESIAN_POINT('Ctrl Pts',(-5.843141152,3.903042157,4.292337419));
#126183=CARTESIAN_POINT('Ctrl Pts',(-5.805451792,3.892857143,4.342721438));
#126184=CARTESIAN_POINT('Ctrl Pts',(-5.605519625,3.838828313,4.609995445));
#126185=CARTESIAN_POINT('Ctrl Pts',(-5.381875481,3.783894965,4.85776865500001));
#126186=CARTESIAN_POINT('',(-5.93554346122029,3.91326598587964,4.58468361069559));
#126187=CARTESIAN_POINT('Ctrl Pts',(-5.57035170579324,3.82362522012809,
5.02206948117668));
#126188=CARTESIAN_POINT('Ctrl Pts',(-5.66877511654743,3.84689293573234,
4.91290073788479));
#126189=CARTESIAN_POINT('Ctrl Pts',(-5.76374548809422,3.86998912007465,
4.80110366621072));
#126190=CARTESIAN_POINT('Ctrl Pts',(-5.85507681427008,3.89285714276327,
4.68701136109109));
#126191=CARTESIAN_POINT('Ctrl Pts',(-5.88216856458662,3.89964051914521,
4.65316798694159));
#126192=CARTESIAN_POINT('Ctrl Pts',(-5.90899333344674,3.90644394874722,
4.61905663523193));
#126193=CARTESIAN_POINT('Ctrl Pts',(-5.93554346242304,3.91326598565651,
4.58468361020552));
#126194=CARTESIAN_POINT('',(-5.90774690816809,3.91326598631302,4.41299523246855));
#126195=CARTESIAN_POINT('Origin',(4.70543742858709E-13,4.00453392000044,
-5.54677831443584E-13));
#126196=CARTESIAN_POINT('',(-5.57516088947638,4.0034549415791,5.01673011568443));
#126197=CARTESIAN_POINT('Origin',(0.152997134137387,4.16057204596886,-0.10398076501913));
#126198=CARTESIAN_POINT('Origin',(0.14147395430415,4.01785425857555,-0.130426777184716));
#126199=CARTESIAN_POINT('Ctrl Pts',(-6.64099453019887,3.783915088,3.48639088072739));
#126200=CARTESIAN_POINT('Ctrl Pts',(-6.45151019389346,3.848090541,3.84732701283557));
#126201=CARTESIAN_POINT('Ctrl Pts',(-6.22402399486561,3.913265985,4.18560091662053));
#126202=CARTESIAN_POINT('Ctrl Pts',(-6.21627552944004,3.91548594241539,
4.19712295030455));
#126203=CARTESIAN_POINT('Ctrl Pts',(-6.20852706401435,3.91770589983073,
4.20864498398861));
#126204=CARTESIAN_POINT('Ctrl Pts',(-6.30498499000001,3.783915088,3.579059133));
#126205=CARTESIAN_POINT('Ctrl Pts',(-6.110464161,3.848090541,3.921733244));
#126206=CARTESIAN_POINT('Ctrl Pts',(-5.87995036100001,3.913265985,4.241306845));
#126207=CARTESIAN_POINT('Ctrl Pts',(-5.87209877168578,3.91548594241539,
4.25219192290301));
#126208=CARTESIAN_POINT('Ctrl Pts',(-5.86424718237167,3.91770589983073,
4.26307700080593));
#126209=CARTESIAN_POINT('',(-6.22332711995899,3.91326598459135,4.18571374571257));
#126210=CARTESIAN_POINT('',(-6.05163873763557,3.91326598377978,4.2135102992684));
#126211=CARTESIAN_POINT('',(-6.51971646641597,3.82362522066975,3.70719532745384));
#126212=CARTESIAN_POINT('Origin',(0.146596010521638,4.01780065125232,-0.118778704970577));
#126213=CARTESIAN_POINT('Ctrl Pts',(-6.30267558681799,3.78467661304239,
3.58312440139765));
#126214=CARTESIAN_POINT('Ctrl Pts',(-6.33874039805141,3.79148857322278,
3.60387276644293));
#126215=CARTESIAN_POINT('Ctrl Pts',(-6.3748820238234,3.79813536728634,3.6245947315682));
#126216=CARTESIAN_POINT('Ctrl Pts',(-6.44721814073559,3.81110763418867,
3.66594140820452));
#126217=CARTESIAN_POINT('Ctrl Pts',(-6.48345555858731,3.81744080288131,
3.68659064831504));
#126218=CARTESIAN_POINT('Ctrl Pts',(-6.51971646712109,3.82362522066945,
3.707195326179));
#126219=CARTESIAN_POINT('Ctrl Pts',(-6.78234521,3.913265985,3.201529861));
#126220=CARTESIAN_POINT('Ctrl Pts',(-6.754559958,3.903042157,3.260392086));
#126221=CARTESIAN_POINT('Ctrl Pts',(-6.725757268,3.892857143,3.3187632));
#126222=CARTESIAN_POINT('Ctrl Pts',(-6.572966551,3.838828313,3.628406645));
#126223=CARTESIAN_POINT('Ctrl Pts',(-6.39237145,3.783894965,3.922701524));
#126224=CARTESIAN_POINT('Ctrl Pts',(-6.654235988,3.913265985,2.878131931));
#126225=CARTESIAN_POINT('Ctrl Pts',(-6.629257423,3.903042157,2.935882329));
#126226=CARTESIAN_POINT('Ctrl Pts',(-6.603280295,3.892857143,2.993190497));
#126227=CARTESIAN_POINT('Ctrl Pts',(-6.465478441,3.838828313,3.297195292));
#126228=CARTESIAN_POINT('Ctrl Pts',(-6.30032689000001,3.783894965,3.587252582));
#126229=CARTESIAN_POINT('',(-6.78234520716211,3.91326598587963,3.20152986547135));
#126230=CARTESIAN_POINT('Ctrl Pts',(-6.51971646550344,3.82362522012805,
3.70719532928111));
#126231=CARTESIAN_POINT('Ctrl Pts',(-6.59237073886474,3.8468929357323,3.57942076650544));
#126232=CARTESIAN_POINT('Ctrl Pts',(-6.66108769022292,3.86998912007463,
3.44982162559431));
#126233=CARTESIAN_POINT('Ctrl Pts',(-6.72575726773051,3.89285714276327,
3.31876319968304));
#126234=CARTESIAN_POINT('Ctrl Pts',(-6.74494030295258,3.89964051914521,
3.27988713929576));
#126235=CARTESIAN_POINT('Ctrl Pts',(-6.76380499121347,3.90644394874722,
3.24080675989453));
#126236=CARTESIAN_POINT('Ctrl Pts',(-6.78234520833622,3.91326598565651,
3.20152986476135));
#126237=CARTESIAN_POINT('',(-6.71829059567161,3.91326598631302,3.03983090335604));
#126238=CARTESIAN_POINT('Origin',(3.38271077815477E-14,4.00453391999933,
3.20923843055709E-14));
#126239=CARTESIAN_POINT('',(-6.523265407003,4.00345494158755,3.70094696342879));
#126240=CARTESIAN_POINT('Origin',(0.171773019413894,4.16057204387436,-0.0686599350762412));
#126241=CARTESIAN_POINT('Origin',(0.166204606815189,4.01785424021442,-0.0969649222269142));
#126242=CARTESIAN_POINT('Ctrl Pts',(-7.234578469,3.783915088,1.977593076));
#126243=CARTESIAN_POINT('Ctrl Pts',(-7.127096857,3.848090541,2.370790323));
#126244=CARTESIAN_POINT('Ctrl Pts',(-6.977633919,3.913265985,2.750022709));
#126245=CARTESIAN_POINT('Ctrl Pts',(-6.97613574545446,3.91391928492389,
2.75382402547298));
#126246=CARTESIAN_POINT('Ctrl Pts',(-6.97463757190891,3.91457258484778,
2.75762534194596));
#126247=CARTESIAN_POINT('Ctrl Pts',(-6.926969862,3.783915088,2.13999732));
#126248=CARTESIAN_POINT('Ctrl Pts',(-6.810661627,3.848090541,2.516476129));
#126249=CARTESIAN_POINT('Ctrl Pts',(-6.654235988,3.913265985,2.878131931));
#126250=CARTESIAN_POINT('Ctrl Pts',(-6.65266802234021,3.91391928492389,
2.88175706484522));
#126251=CARTESIAN_POINT('Ctrl Pts',(-6.65110005668042,3.91457258484778,
2.88538219869044));
#126252=CARTESIAN_POINT('',(-6.9776339183878,3.91326598458878,2.75002271233773));
#126253=CARTESIAN_POINT('',(-6.81593495058514,3.91326598377978,2.81407732706006));
#126254=CARTESIAN_POINT('',(-7.16422653006704,3.82362522066782,2.21897684172014));
#126255=CARTESIAN_POINT('Origin',(0.168702890671167,4.01780065157927,-0.0844880162775102));
#126256=CARTESIAN_POINT('Ctrl Pts',(-6.92558836378585,3.78467661306916,
2.14446399830583));
#126257=CARTESIAN_POINT('Ctrl Pts',(-6.96527028494623,3.79148857322583,
2.15697440977198));
#126258=CARTESIAN_POINT('Ctrl Pts',(-7.00502154967839,3.798135367293,2.16944252569916));
#126259=CARTESIAN_POINT('Ctrl Pts',(-7.08455480235546,3.81110763428842,
2.19427241333284));
#126260=CARTESIAN_POINT('Ctrl Pts',(-7.12438398655221,3.81744080309546,
2.20664891226419));
#126261=CARTESIAN_POINT('Ctrl Pts',(-7.16422653047534,3.82362522066753,
2.21897684032714));
#126262=CARTESIAN_POINT('Ctrl Pts',(-7.312012032,3.913265985,1.668676136));
#126263=CARTESIAN_POINT('Ctrl Pts',(-7.297530022,3.903042157,1.732135204));
#126264=CARTESIAN_POINT('Ctrl Pts',(-7.281948786,3.892857143,1.79533336));
#126265=CARTESIAN_POINT('Ctrl Pts',(-7.19929442,3.838828313,2.130583001));
#126266=CARTESIAN_POINT('Ctrl Pts',(-7.086186231,3.783894965,2.456820037));
#126267=CARTESIAN_POINT('Ctrl Pts',(-7.117376937,3.913265985,1.380378766));
#126268=CARTESIAN_POINT('Ctrl Pts',(-7.105396986,3.903042157,1.442148645));
#126269=CARTESIAN_POINT('Ctrl Pts',(-7.09234675,3.892857143,1.503701295));
#126270=CARTESIAN_POINT('Ctrl Pts',(-7.023118672,3.838828313,1.830221952));
#126271=CARTESIAN_POINT('Ctrl Pts',(-6.924182015,3.783894965,2.149000565));
#126272=CARTESIAN_POINT('',(-7.31201203007925,3.91326598587931,1.66867614091864));
#126273=CARTESIAN_POINT('Ctrl Pts',(-7.16422652957999,3.82362522012809,
2.21897684369667));
#126274=CARTESIAN_POINT('Ctrl Pts',(-7.20771443234409,3.84689293573233,
2.07857105821795));
#126275=CARTESIAN_POINT('Ctrl Pts',(-7.24696483514426,3.86998912007465,
1.93722976007989));
#126276=CARTESIAN_POINT('Ctrl Pts',(-7.2819487862808,3.89285714276327,1.79533336012661));
#126277=CARTESIAN_POINT('Ctrl Pts',(-7.29232612896224,3.89964051914521,
1.75324241500064));
#126278=CARTESIAN_POINT('Ctrl Pts',(-7.30234864499589,3.90644394874722,
1.71102036257375));
#126279=CARTESIAN_POINT('Ctrl Pts',(-7.31201203089214,3.91326598565651,
1.66867613996504));
#126280=CARTESIAN_POINT('',(-7.21469448283075,3.91326598631302,1.52452745889956));
#126281=CARTESIAN_POINT('Origin',(1.29236898960272E-13,4.00453392000067,
-1.20888542232134E-13));
#126282=CARTESIAN_POINT('',(-7.16634928489015,4.00345494175446,2.21211164336112));
#126283=CARTESIAN_POINT('Origin',(0.182516852497029,4.16057202103997,-0.0301285563182022));
#126284=CARTESIAN_POINT('Origin',(0.183163364923503,4.0178544102177,-0.058968874271389));
#126285=CARTESIAN_POINT('Ctrl Pts',(-7.49110093225904,3.783915088,0.375681439532661));
#126286=CARTESIAN_POINT('Ctrl Pts',(-7.47068275464331,3.848090541,0.782820608964772));
#126287=CARTESIAN_POINT('Ctrl Pts',(-7.40625939708089,3.913265985,1.1853486654421));
#126288=CARTESIAN_POINT('Ctrl Pts',(-7.4040650565511,3.91548594253913,1.19905927696758));
#126289=CARTESIAN_POINT('Ctrl Pts',(-7.40187071602134,3.9177059000782,1.21276988849307));
#126290=CARTESIAN_POINT('Ctrl Pts',(-7.225057322,3.783915088,0.600871612));
#126291=CARTESIAN_POINT('Ctrl Pts',(-7.192400124,3.848090541,0.993551388));
#126292=CARTESIAN_POINT('Ctrl Pts',(-7.117376937,3.913265985,1.380378766));
#126293=CARTESIAN_POINT('Ctrl Pts',(-7.11482155295706,3.91548594253913,
1.39355459268297));
#126294=CARTESIAN_POINT('Ctrl Pts',(-7.11226616891413,3.91770590007819,
1.4067304193659));
#126295=CARTESIAN_POINT('',(-7.40567430623151,3.91326598459133,1.18574367653095));
#126296=CARTESIAN_POINT('',(-7.26152562067098,3.91326598377978,1.28306122602161));
#126297=CARTESIAN_POINT('',(-7.4737453237154,3.8236252207137,0.627001465451102));
#126298=CARTESIAN_POINT('Origin',(0.182920815903383,4.01780065137544,-0.0462465742457208));
#126299=CARTESIAN_POINT('Ctrl Pts',(-7.22466832584242,3.78467661301739,
0.605530843173444));
#126300=CARTESIAN_POINT('Ctrl Pts',(-7.26611187466958,3.79148857323157,
0.609218327966945));
#126301=CARTESIAN_POINT('Ctrl Pts',(-7.30761405303173,3.79813536726189,
0.612849599230928));
#126302=CARTESIAN_POINT('Ctrl Pts',(-7.39062574518316,3.81110766408171,
0.620001695735266));
#126303=CARTESIAN_POINT('Ctrl Pts',(-7.43218454272656,3.81744086362057,
0.623526759203508));
#126304=CARTESIAN_POINT('Ctrl Pts',(-7.4737453238487,3.82362522071367,0.627001463856704));
#126305=CARTESIAN_POINT('Ctrl Pts',(-7.499777297,3.913265985,0.05779697));
#126306=CARTESIAN_POINT('Ctrl Pts',(-7.499275692,3.903042157,0.122885604));
#126307=CARTESIAN_POINT('Ctrl Pts',(-7.497644473,3.892857143,0.187955727));
#126308=CARTESIAN_POINT('Ctrl Pts',(-7.488991283,3.838828313,0.533135664000001));
#126309=CARTESIAN_POINT('Ctrl Pts',(-7.44865882,3.783894965,0.876060377));
#126310=CARTESIAN_POINT('Ctrl Pts',(-7.24771725,3.913265985,-0.181919376));
#126311=CARTESIAN_POINT('Ctrl Pts',(-7.249296082,3.903042157,-0.119018306));
#126312=CARTESIAN_POINT('Ctrl Pts',(-7.249782953,3.892857143,-0.056099309));
#126313=CARTESIAN_POINT('Ctrl Pts',(-7.25236567800001,3.838828313,0.277669467));
#126314=CARTESIAN_POINT('Ctrl Pts',(-7.224270084,3.783894965,0.610263670000001));
#126315=CARTESIAN_POINT('',(-7.49977729625428,3.91326598544903,0.0577969751222766));
#126316=CARTESIAN_POINT('Ctrl Pts',(-7.47374532365293,3.82362522012805,
0.627001467668876));
#126317=CARTESIAN_POINT('Ctrl Pts',(-7.48603340995214,3.84689293573231,
0.48052967758556));
#126318=CARTESIAN_POINT('Ctrl Pts',(-7.49398195897382,3.86998912007412,
0.334055183764473));
#126319=CARTESIAN_POINT('Ctrl Pts',(-7.49764447287357,3.89285714292383,
0.187955727374184));
#126320=CARTESIAN_POINT('Ctrl Pts',(-7.49873088980851,3.89964051904629,
0.144618023667244));
#126321=CARTESIAN_POINT('Ctrl Pts',(-7.49944259184632,3.90644394833731,
0.101228554286914));
#126322=CARTESIAN_POINT('Ctrl Pts',(-7.49977729697119,3.91326598441267,
0.0577969737391663));
#126323=CARTESIAN_POINT('',(-7.37374727356795,3.91326598631302,-0.0620611949262858));
#126324=CARTESIAN_POINT('Origin',(-2.30067701001424E-12,4.00453392,1.76098149734169E-13));
#126325=CARTESIAN_POINT('',(-7.47434263494074,4.00345494159181,0.619840442693622));
#126326=CARTESIAN_POINT('Origin',(0.18472655890323,4.16057205720237,0.00981153923062972));
#126327=CARTESIAN_POINT('Origin',(0.191557339022314,4.01785420958081,-0.0182154483150819));
#126328=CARTESIAN_POINT('Ctrl Pts',(-7.39629537,3.783915088,-1.242905788));
#126329=CARTESIAN_POINT('Ctrl Pts',(-7.46384694,3.848090541,-0.840919274));
#126330=CARTESIAN_POINT('Ctrl Pts',(-7.487433596,3.913265985,-0.433979423));
#126331=CARTESIAN_POINT('Ctrl Pts',(-7.48767002186263,3.91391928492389,
-0.429900374859003));
#126332=CARTESIAN_POINT('Ctrl Pts',(-7.48790644772526,3.91457258484778,
-0.425821326718006));
#126333=CARTESIAN_POINT('Ctrl Pts',(-7.185309132,3.783915088,-0.966350186));
#126334=CARTESIAN_POINT('Ctrl Pts',(-7.237829985,3.848090541,-0.575830712));
#126335=CARTESIAN_POINT('Ctrl Pts',(-7.24771725000001,3.913265985,-0.181919376));
#126336=CARTESIAN_POINT('Ctrl Pts',(-7.24781635710346,3.91391928492389,
-0.177970921949899));
#126337=CARTESIAN_POINT('Ctrl Pts',(-7.24791546420693,3.91457258484778,
-0.174022467899798));
#126338=CARTESIAN_POINT('',(-7.48743359644336,3.9132659845887,-0.433979417791379));
#126339=CARTESIAN_POINT('',(-7.36757542331898,3.91326598377978,-0.307949391868539));
#126340=CARTESIAN_POINT('',(-7.43380009195768,3.82362522069477,-0.994291802622036));
#126341=CARTESIAN_POINT('Origin',(0.188585881119456,4.01780062346965,-0.00584277760883337));
#126342=CARTESIAN_POINT('Ctrl Pts',(-7.18593082774993,3.78467661310377,
-0.961716262313775));
#126343=CARTESIAN_POINT('Ctrl Pts',(-7.22719814967869,3.79148857331076,
-0.967024126778678));
#126344=CARTESIAN_POINT('Ctrl Pts',(-7.26851064564091,3.79813536726239,
-0.972399494037209));
#126345=CARTESIAN_POINT('Ctrl Pts',(-7.35111886069136,3.81110763282126,
-0.983259643223968));
#126346=CARTESIAN_POINT('Ctrl Pts',(-7.39246359533456,3.81744080007791,
-0.988750875908959));
#126347=CARTESIAN_POINT('Ctrl Pts',(-7.43380009175475,3.82362522069464,
-0.994291804132863));
#126348=CARTESIAN_POINT('Ctrl Pts',(-7.336861312,3.913265985,-1.555784718));
#126349=CARTESIAN_POINT('Ctrl Pts',(-7.350363566,3.903042157,-1.49210999));
#126350=CARTESIAN_POINT('Ctrl Pts',(-7.362758637,3.892857143,-1.428210506));
#126351=CARTESIAN_POINT('Ctrl Pts',(-7.428511236,3.838828313,-1.089240504));
#126352=CARTESIAN_POINT('Ctrl Pts',(-7.462840401,3.783894965,-0.745662894));
#126353=CARTESIAN_POINT('Ctrl Pts',(-7.03916236,3.913265985,-1.73571117));
#126354=CARTESIAN_POINT('Ctrl Pts',(-7.05422615,3.903042157,-1.674620094));
#126355=CARTESIAN_POINT('Ctrl Pts',(-7.068227363,3.892857143,-1.613276771));
#126356=CARTESIAN_POINT('Ctrl Pts',(-7.14250012700001,3.838828313,-1.287866533));
#126357=CARTESIAN_POINT('Ctrl Pts',(-7.186559314,3.783894965,-0.957008476));
#126358=CARTESIAN_POINT('',(-7.33686131228228,3.91326598544478,-1.55578471328563));
#126359=CARTESIAN_POINT('Ctrl Pts',(-7.43380009232047,3.82362522012808,
-0.994291800520328));
#126360=CARTESIAN_POINT('Ctrl Pts',(-7.41431378467035,3.84689293573234,
-1.13998073657581));
#126361=CARTESIAN_POINT('Ctrl Pts',(-7.39058881472474,3.86998912007434,
-1.28473944107708));
#126362=CARTESIAN_POINT('Ctrl Pts',(-7.36275863686772,3.89285714295372,
-1.42821050582817));
#126363=CARTESIAN_POINT('Ctrl Pts',(-7.3545033286935,3.89964051908512,-1.4707685459966));
#126364=CARTESIAN_POINT('Ctrl Pts',(-7.34587093849312,3.90644394833732,
-1.51329658840766));
#126365=CARTESIAN_POINT('Ctrl Pts',(-7.33686131277566,3.91326598441268,
-1.55578471434209));
#126366=CARTESIAN_POINT('',(-7.18801183780196,3.91326598631302,-1.6457479361297));
#126367=CARTESIAN_POINT('Origin',(7.64145691167784E-13,4.00453392000044,
-2.8162151430311E-14));
#126368=CARTESIAN_POINT('',(-7.43284403006748,4.00345494177907,-1.00141380955596));
#126369=CARTESIAN_POINT('Origin',(0.178298505928733,4.16057201474277,0.0492928937590242));
#126370=CARTESIAN_POINT('Origin',(0.190994943113921,4.01785441543893,0.0233895974095227));
#126371=CARTESIAN_POINT('Ctrl Pts',(-6.95648361438047,3.783915088,-2.80447239965452));
#126372=CARTESIAN_POINT('Ctrl Pts',(-7.10890587833995,3.848090541,-2.42638952729282));
#126373=CARTESIAN_POINT('Ctrl Pts',(-7.2194539668175,3.913265985,-2.03401429123132));
#126374=CARTESIAN_POINT('Ctrl Pts',(-7.22321937368872,3.91548594255921,
-2.020649497409));
#126375=CARTESIAN_POINT('Ctrl Pts',(-7.22698478055991,3.91770590011835,
-2.00728470358669));
#126376=CARTESIAN_POINT('Ctrl Pts',(-6.809583872,3.783915088,-2.488386523));
#126377=CARTESIAN_POINT('Ctrl Pts',(-6.94482696000001,3.848090541,-2.118287608));
#126378=CARTESIAN_POINT('Ctrl Pts',(-7.03916236,3.913265985,-1.73571117));
#126379=CARTESIAN_POINT('Ctrl Pts',(-7.04237554231957,3.91548594255921,
-1.7226801355584));
#126380=CARTESIAN_POINT('Ctrl Pts',(-7.04558872463913,3.91770590011835,
-1.70964910111681));
#126381=CARTESIAN_POINT('',(-7.21908881398541,3.91326598502339,-2.03341011308339));
#126382=CARTESIAN_POINT('',(-7.12912558795207,3.91326598377977,-1.88456063811549));
#126383=CARTESIAN_POINT('',(-7.04625863050199,3.82362522070109,-2.56909309101298));
#126384=CARTESIAN_POINT('Origin',(0.185432846277829,4.01780061998897,0.0348342047164549));
#126385=CARTESIAN_POINT('Ctrl Pts',(-6.81118718964651,3.78467661311381,
-2.4839945843682));
#126386=CARTESIAN_POINT('Ctrl Pts',(-6.85034867044299,3.79148857328906,
-2.49804960808278));
#126387=CARTESIAN_POINT('Ctrl Pts',(-6.88953975868089,3.79813536731663,
-2.51218026776745));
#126388=CARTESIAN_POINT('Ctrl Pts',(-6.96788202635751,3.81110763248485,
-2.54054483607025));
#126389=CARTESIAN_POINT('Ctrl Pts',(-7.00707968910712,3.81744079938323,
-2.55479558166922));
#126390=CARTESIAN_POINT('Ctrl Pts',(-7.04625862997314,3.82362522070093,
-2.56909309246075));
#126391=CARTESIAN_POINT('Ctrl Pts',(-6.830881846,3.913265985,-3.096619642));
#126392=CARTESIAN_POINT('Ctrl Pts',(-6.85775661,3.903042157,-3.037336179));
#126393=CARTESIAN_POINT('Ctrl Pts',(-6.883598391,3.892857143,-2.977595203));
#126394=CARTESIAN_POINT('Ctrl Pts',(-7.02068226100001,3.838828313,-2.660684997));
#126395=CARTESIAN_POINT('Ctrl Pts',(-7.128067859,3.783894965,-2.332519796));
#126396=CARTESIAN_POINT('Ctrl Pts',(-6.501464062,3.913265985,-3.208343039));
#126397=CARTESIAN_POINT('Ctrl Pts',(-6.52930844400001,3.903042157,-3.151918508));
#126398=CARTESIAN_POINT('Ctrl Pts',(-6.556169318,3.892857143,-3.095019205));
#126399=CARTESIAN_POINT('Ctrl Pts',(-6.698659207,3.838828313,-2.793183326));
#126400=CARTESIAN_POINT('Ctrl Pts',(-6.812813018,3.783894965,-2.479531969));
#126401=CARTESIAN_POINT('',(-6.83088184728228,3.9132659854451,-3.09661963745733));
#126402=CARTESIAN_POINT('Ctrl Pts',(-7.04625863131703,3.82362522012808,
-2.56909308901641));
#126403=CARTESIAN_POINT('Ctrl Pts',(-6.99590908811595,3.84689293573234,
-2.70718691856856));
#126404=CARTESIAN_POINT('Ctrl Pts',(-6.94161995248627,3.86998912007467,
-2.84346107764366));
#126405=CARTESIAN_POINT('Ctrl Pts',(-6.88359839099153,3.89285714300334,
-2.97759520301957));
#126406=CARTESIAN_POINT('Ctrl Pts',(-6.86638736695053,3.89964051914954,
-3.01738361288811));
#126407=CARTESIAN_POINT('Ctrl Pts',(-6.84881452494633,3.90644394833732,
-3.05706166447821));
#126408=CARTESIAN_POINT('Ctrl Pts',(-6.83088184754387,3.91326598441267,
-3.09661963859435));
#126409=CARTESIAN_POINT('',(-6.66617295745172,3.91326598631302,-3.15248133320107));
#126410=CARTESIAN_POINT('Origin',(1.23772520010945E-12,4.00453392000089,
3.67544536472586E-13));
#126411=CARTESIAN_POINT('',(-7.04379390009593,4.00345494159456,-2.57584306385732));
#126412=CARTESIAN_POINT('Origin',(0.163533465628372,4.16057204973995,0.0864693627536012));
#126413=CARTESIAN_POINT('Origin',(0.181501620989318,4.01785426451466,0.0639010988808864));
#126414=CARTESIAN_POINT('Ctrl Pts',(-6.19096622720938,3.783915088,-4.23434373834982));
#126415=CARTESIAN_POINT('Ctrl Pts',(-6.42110158485165,3.848090541,-3.89786651471394));
#126416=CARTESIAN_POINT('Ctrl Pts',(-6.6134141979455,3.913265985,-3.53842936551643));
#126417=CARTESIAN_POINT('Ctrl Pts',(-6.61996460689183,3.91548594241512,
-3.52618648513606));
#126418=CARTESIAN_POINT('Ctrl Pts',(-6.62651501583818,3.91770589983019,
-3.51394360475565));
#126419=CARTESIAN_POINT('Ctrl Pts',(-6.115450039,3.783915088,-3.894068671));
#126420=CARTESIAN_POINT('Ctrl Pts',(-6.327091546,3.848090541,-3.56169573));
#126421=CARTESIAN_POINT('Ctrl Pts',(-6.501464062,3.913265985,-3.208343039));
#126422=CARTESIAN_POINT('Ctrl Pts',(-6.50740340872524,3.91548594241512,
-3.19630740290158));
#126423=CARTESIAN_POINT('Ctrl Pts',(-6.51334275545048,3.91770589983019,
-3.18427176680309));
#126424=CARTESIAN_POINT('',(-6.61318746238803,3.91326598502339,-3.53776081555977));
#126425=CARTESIAN_POINT('',(-6.55732576399389,3.91326598377977,-3.37305192420777));
#126426=CARTESIAN_POINT('',(-6.32924194658555,3.82362522064777,-4.02376644191561));
#126427=CARTESIAN_POINT('Origin',(0.173609143530363,4.01780060722512,0.0738823615602285));
#126428=CARTESIAN_POINT('Ctrl Pts',(-6.11796000902615,3.78467661310375,
-3.89012407986765));
#126429=CARTESIAN_POINT('Ctrl Pts',(-6.15318450146292,3.79148857325392,
-3.91226906565243));
#126430=CARTESIAN_POINT('Ctrl Pts',(-6.18842164977781,3.79813536728931,
-3.9344942839077));
#126431=CARTESIAN_POINT('Ctrl Pts',(-6.25883479088989,3.81110763537301,
-3.97903698618127));
#126432=CARTESIAN_POINT('Ctrl Pts',(-6.29405256303366,3.81744080530427,
-4.00138090761849));
#126433=CARTESIAN_POINT('Ctrl Pts',(-6.32924194583481,3.82362522064763,
-4.02376644309495));
#126434=CARTESIAN_POINT('Ctrl Pts',(-6.005497937,3.913265985,-4.492660073));
#126435=CARTESIAN_POINT('Ctrl Pts',(-6.044488575,3.903042157,-4.440539904));
#126436=CARTESIAN_POINT('Ctrl Pts',(-6.082568734,3.892857143,-4.387750858));
#126437=CARTESIAN_POINT('Ctrl Pts',(-6.284573986,3.838828313,-4.107718817));
#126438=CARTESIAN_POINT('Ctrl Pts',(-6.459994786,3.783894965,-3.810310665));
#126439=CARTESIAN_POINT('Ctrl Pts',(-5.65976453,3.913265985,-4.530956353));
#126440=CARTESIAN_POINT('Ctrl Pts',(-5.69908753200001,3.903042157,-4.481836715));
#126441=CARTESIAN_POINT('Ctrl Pts',(-5.737552082,3.892857143,-4.43204198));
#126442=CARTESIAN_POINT('Ctrl Pts',(-5.941596428,3.838828313,-4.167893971));
#126443=CARTESIAN_POINT('Ctrl Pts',(-6.12050715700001,3.783894965,-3.886115303));
#126444=CARTESIAN_POINT('',(-6.00549793922011,3.9132659854451,-4.49266006884022));
#126445=CARTESIAN_POINT('Ctrl Pts',(-6.32924194769678,3.82362522012804,
-4.02376644030595));
#126446=CARTESIAN_POINT('Ctrl Pts',(-6.25038345750539,3.8468929357323,-4.14780804938589));
#126447=CARTESIAN_POINT('Ctrl Pts',(-6.16806865568598,3.86998912007458,
-4.2692256348332));
#126448=CARTESIAN_POINT('Ctrl Pts',(-6.08256873377003,3.89285714299345,
-4.38775085799873));
#126449=CARTESIAN_POINT('Ctrl Pts',(-6.05720676147809,3.89964051913671,
-4.42290917543916));
#126450=CARTESIAN_POINT('Ctrl Pts',(-6.03151515499193,3.90644394833732,
-4.45788193471822));
#126451=CARTESIAN_POINT('Ctrl Pts',(-6.00549793923989,3.91326598441267,
-4.49266007000586));
#126452=CARTESIAN_POINT('',(-5.83263123844007,3.91326598631302,-4.51180820661373));
#126453=CARTESIAN_POINT('Origin',(3.25260651745651E-14,4.00453392000067,
8.13151629364128E-14));
#126454=CARTESIAN_POINT('',(-6.32538379609172,4.00345494159109,-4.02982876001983));
#126455=CARTESIAN_POINT('Origin',(0.141121856785884,4.16057201893952,0.119602660310776));
#126456=CARTESIAN_POINT('Origin',(0.163521298014353,4.01785421895581,0.101424576841471));
#126457=CARTESIAN_POINT('Ctrl Pts',(-5.13596613941495,3.783915088,-5.46622186992519));
#126458=CARTESIAN_POINT('Ctrl Pts',(-5.43305371731725,3.848090541,-5.18708359570571));
#126459=CARTESIAN_POINT('Ctrl Pts',(-5.69813853003985,3.913265985,-4.87739141458904));
#126460=CARTESIAN_POINT('Ctrl Pts',(-5.70716765213171,3.91548594258725,
-4.86684290943145));
#126461=CARTESIAN_POINT('Ctrl Pts',(-5.71619677422368,3.91770590017445,
-4.85629440427387));
#126462=CARTESIAN_POINT('Ctrl Pts',(-5.135364559,3.783915088,-5.11766849700001));
#126463=CARTESIAN_POINT('Ctrl Pts',(-5.413508362,3.848090541,-4.838562918));
#126464=CARTESIAN_POINT('Ctrl Pts',(-5.65976453,3.913265985,-4.530956353));
#126465=CARTESIAN_POINT('Ctrl Pts',(-5.66815232477374,3.91548594258725,
-4.52047888655021));
#126466=CARTESIAN_POINT('Ctrl Pts',(-5.67654011954747,3.91770590017445,
-4.51000142010045));
#126467=CARTESIAN_POINT('',(-5.69806081408175,3.91326598502339,-4.87668975361084));
#126468=CARTESIAN_POINT('',(-5.67891267437233,3.91326598377977,-4.70382305061765));
#126469=CARTESIAN_POINT('',(-5.31627694370513,3.82362522068245,-5.29029294613879));
#126470=CARTESIAN_POINT('Origin',(0.153667820396709,4.01780065382243,0.10947592326954));
#126471=CARTESIAN_POINT('Ctrl Pts',(-5.13866381815813,3.78467661318519,
-5.11435569671692));
#126472=CARTESIAN_POINT('Ctrl Pts',(-5.16830426428969,3.79148857338208,
-5.14355516998409));
#126473=CARTESIAN_POINT('Ctrl Pts',(-5.19793982225928,3.79813536732747,
-5.1728357199823));
#126474=CARTESIAN_POINT('Ctrl Pts',(-5.25713137033582,3.81110763353346,
-5.23147377430861));
#126475=CARTESIAN_POINT('Ctrl Pts',(-5.28672247804631,3.81744080148512,
-5.26086607751029));
#126476=CARTESIAN_POINT('Ctrl Pts',(-5.31627694263694,3.82362522068214,
-5.290292947179));
#126477=CARTESIAN_POINT('Ctrl Pts',(-4.899303619,3.913265985,-5.678628712));
#126478=CARTESIAN_POINT('Ctrl Pts',(-4.948586973,3.903042157,-5.636108919));
#126479=CARTESIAN_POINT('Ctrl Pts',(-4.997124924,3.892857143,-5.59274016));
#126480=CARTESIAN_POINT('Ctrl Pts',(-5.254606016,3.838828313,-5.36268027));
#126481=CARTESIAN_POINT('Ctrl Pts',(-5.489859537,3.783894965,-5.109935642));
#126482=CARTESIAN_POINT('Ctrl Pts',(-4.553420698,3.913265985,-5.64170718300001));
#126483=CARTESIAN_POINT('Ctrl Pts',(-4.602383621,3.903042157,-5.602189219));
#126484=CARTESIAN_POINT('Ctrl Pts',(-4.650653287,3.892857143,-5.561827398));
#126485=CARTESIAN_POINT('Ctrl Pts',(-4.906711204,3.838828313,-5.347718525));
#126486=CARTESIAN_POINT('Ctrl Pts',(-5.142013183,3.783894965,-5.110988204));
#126487=CARTESIAN_POINT('',(-4.89930362251608,3.91326598587964,-5.67862870804665));
#126488=CARTESIAN_POINT('Ctrl Pts',(-5.31627694526545,3.82362522012808,
-5.29029294474692));
#126489=CARTESIAN_POINT('Ctrl Pts',(-5.21259684342557,3.84689293573233,
-5.39448228564937));
#126490=CARTESIAN_POINT('Ctrl Pts',(-5.10610532417885,3.86998912007464,
-5.49536594628879));
#126491=CARTESIAN_POINT('Ctrl Pts',(-4.9971249235474,3.89285714276326,-5.59274016010589));
#126492=CARTESIAN_POINT('Ctrl Pts',(-4.96479790140804,3.89964051914521,
-5.6216244213825));
#126493=CARTESIAN_POINT('Ctrl Pts',(-4.93218884071494,3.90644394874722,
-5.65025660069319));
#126494=CARTESIAN_POINT('Ctrl Pts',(-4.8993036221179,3.91326598565651,-5.67862870931902));
#126495=CARTESIAN_POINT('',(-4.72636216469744,3.91326598631302,-5.66016794232501));
#126496=CARTESIAN_POINT('Origin',(-3.02709246557953E-13,4.00453392,-1.45716771982052E-13));
#126497=CARTESIAN_POINT('',(-5.31120577464656,4.00345494159129,-5.29538414253212));
#126498=CARTESIAN_POINT('Origin',(0.112111455877779,4.16057203305905,0.147143430146888));
#126499=CARTESIAN_POINT('Origin',(0.137894918506129,4.01785427167017,0.134205497386245));
#126500=CARTESIAN_POINT('Ctrl Pts',(-3.84081398363233,3.783915088,-6.44250554227282));
#126501=CARTESIAN_POINT('Ctrl Pts',(-4.19096229675016,3.848090541,-6.23375841256356));
#126502=CARTESIAN_POINT('Ctrl Pts',(-4.51642423896958,3.913265985,-5.9882920620467));
#126503=CARTESIAN_POINT('Ctrl Pts',(-4.52750988138672,3.91548594245996,
-5.97993116992911));
#126504=CARTESIAN_POINT('Ctrl Pts',(-4.53859552380381,3.91770589991986,
-5.97157027781169));
#126505=CARTESIAN_POINT('Ctrl Pts',(-3.91515514,3.783915088,-6.101971831));
#126506=CARTESIAN_POINT('Ctrl Pts',(-4.246795545,3.848090541,-5.889184282));
#126507=CARTESIAN_POINT('Ctrl Pts',(-4.553420698,3.913265985,-5.641707183));
#126508=CARTESIAN_POINT('Ctrl Pts',(-4.56386473572397,3.91548594245996,
-5.63327780226433));
#126509=CARTESIAN_POINT('Ctrl Pts',(-4.57430877344792,3.91770589991986,
-5.62484842152856));
#126510=CARTESIAN_POINT('',(-4.51649917455088,3.91326598459136,-5.98759010069319));
#126511=CARTESIAN_POINT('',(-4.53495994002295,3.91326598377977,-5.81464863880259));
#126512=CARTESIAN_POINT('',(-4.05472873979337,3.82362522068753,-6.30945123164814));
#126513=CARTESIAN_POINT('Origin',(0.126541207839908,4.01780067271071,0.13995068839164));
#126514=CARTESIAN_POINT('Ctrl Pts',(-3.91908941737862,3.78467661291985,
-6.09944572486574));
#126515=CARTESIAN_POINT('Ctrl Pts',(-3.94175982073275,3.79148856047556,
-6.13433428550706));
#126516=CARTESIAN_POINT('Ctrl Pts',(-3.96440801632649,3.79813534156362,
-6.16930096846007));
#126517=CARTESIAN_POINT('Ctrl Pts',(-4.00961033894422,3.81110763314013,
-6.23929266744067));
#126518=CARTESIAN_POINT('Ctrl Pts',(-4.03219114569097,3.81744080085026,
-6.27435900682164));
#126519=CARTESIAN_POINT('Ctrl Pts',(-4.05472873852679,3.82362522068738,
-6.30945123246102));
#126520=CARTESIAN_POINT('Ctrl Pts',(-3.564023309,3.913265985,-6.599070984));
#126521=CARTESIAN_POINT('Ctrl Pts',(-3.621294945,3.903042157,-6.568139745));
#126522=CARTESIAN_POINT('Ctrl Pts',(-3.678021106,3.892857143,-6.536219148));
#126523=CARTESIAN_POINT('Ctrl Pts',(-3.978938509,3.838828313,-6.366888754));
#126524=CARTESIAN_POINT('Ctrl Pts',(-4.263024558,3.783894965,-6.170625707));
#126525=CARTESIAN_POINT('Ctrl Pts',(-3.234163976,3.913265985,-6.488658057));
#126526=CARTESIAN_POINT('Ctrl Pts',(-3.290477367,3.903042157,-6.460589581));
#126527=CARTESIAN_POINT('Ctrl Pts',(-3.346295113,3.892857143,-6.431547949));
#126528=CARTESIAN_POINT('Ctrl Pts',(-3.642393617,3.838828313,-6.277489706));
#126529=CARTESIAN_POINT('Ctrl Pts',(-3.923084388,3.783894965,-6.09687697800001));
#126530=CARTESIAN_POINT('',(-3.56402331315857,3.91326598544902,-6.59907098094449));
#126531=CARTESIAN_POINT('Ctrl Pts',(-4.05472874160685,3.82362522012805,
-6.30945123057785));
#126532=CARTESIAN_POINT('Ctrl Pts',(-3.93107499426224,3.8468929357323,-6.38891652569893));
#126533=CARTESIAN_POINT('Ctrl Pts',(-3.80538618257823,3.86998912007455,
-6.46454905386878));
#126534=CARTESIAN_POINT('Ctrl Pts',(-3.67802110594336,3.89285714298927,
-6.53621914792962));
#126535=CARTESIAN_POINT('Ctrl Pts',(-3.6402406092741,3.89964051913127,-6.55747875699982));
#126536=CARTESIAN_POINT('Ctrl Pts',(-3.60223885805458,3.90644394833732,
-6.578431547705));
#126537=CARTESIAN_POINT('Ctrl Pts',(-3.56402331229007,3.91326598441268,
-6.5990709822231));
#126538=CARTESIAN_POINT('',(-3.39909364966501,3.91326598631302,-6.54386451677826));
#126539=CARTESIAN_POINT('Origin',(-2.91216703529606E-13,4.00453391999933,
-5.03069808033274E-13));
#126540=CARTESIAN_POINT('',(-4.04868167575611,4.00345494161998,-6.313333246779));
#126541=CARTESIAN_POINT('Origin',(0.0778588908243844,4.16057202404688,0.167803995367347));
#126542=CARTESIAN_POINT('Origin',(0.105820797950587,4.01785426712178,0.160711179465115));
#126543=CARTESIAN_POINT('Ctrl Pts',(-2.36606963524325,3.783915088,-7.11754481581828));
#126544=CARTESIAN_POINT('Ctrl Pts',(-2.75290613681028,3.848090541,-6.98894961498189));
#126545=CARTESIAN_POINT('Ctrl Pts',(-3.12352696960768,3.913265985,-6.81918682763074));
#126546=CARTESIAN_POINT('Ctrl Pts',(-3.13615078042259,3.91548594243905,
-6.813404493986));
#126547=CARTESIAN_POINT('Ctrl Pts',(-3.14877459123754,3.91770589987804,
-6.80762216034113));
#126548=CARTESIAN_POINT('Ctrl Pts',(-2.511877418,3.783915088,-6.800953745));
#126549=CARTESIAN_POINT('Ctrl Pts',(-2.881507287,3.848090541,-6.664433933));
#126550=CARTESIAN_POINT('Ctrl Pts',(-3.234163976,3.913265985,-6.488658057));
#126551=CARTESIAN_POINT('Ctrl Pts',(-3.24617590552632,3.91548594243905,
-6.48267091000746));
#126552=CARTESIAN_POINT('Ctrl Pts',(-3.25818783505264,3.91770589987804,
-6.47668376301503));
#126553=CARTESIAN_POINT('',(-3.12375105627747,3.91326598502339,-6.81851738529729));
#126554=CARTESIAN_POINT('',(-3.17895751939195,3.91326598377977,-6.65358771970716));
#126555=CARTESIAN_POINT('',(-2.60358592652387,3.823625220675,-7.03358659017151));
#126556=CARTESIAN_POINT('Origin',(0.0934974573071612,4.01780061747444,0.163881283245135));
#126557=CARTESIAN_POINT('Ctrl Pts',(-2.51626275246637,3.78467661289495,
-6.79933245052332));
#126558=CARTESIAN_POINT('Ctrl Pts',(-2.53090315221161,3.79148857308155,
-6.8382788747793));
#126559=CARTESIAN_POINT('Ctrl Pts',(-2.54550507273525,3.7981353672037,-6.87729683093022));
#126560=CARTESIAN_POINT('Ctrl Pts',(-2.57460438787571,3.81110763385064,
-6.95536917604575));
#126561=CARTESIAN_POINT('Ctrl Pts',(-2.58911904323647,3.81744080227308,
-6.99446989459292));
#126562=CARTESIAN_POINT('Ctrl Pts',(-2.60358592513734,3.82362522067471,
-7.03358659066263));
#126563=CARTESIAN_POINT('Ctrl Pts',(-2.06209323,3.913265985,-7.210948031));
#126564=CARTESIAN_POINT('Ctrl Pts',(-2.124675189,3.903042157,-7.193051656));
#126565=CARTESIAN_POINT('Ctrl Pts',(-2.186937109,3.892857143,-7.174071792));
#126566=CARTESIAN_POINT('Ctrl Pts',(-2.51722026,3.838828313,-7.07338859600001));
#126567=CARTESIAN_POINT('Ctrl Pts',(-2.836855288,3.783894965,-6.942784173));
#126568=CARTESIAN_POINT('Ctrl Pts',(-1.763681341,3.913265985,-7.032206491));
#126569=CARTESIAN_POINT('Ctrl Pts',(-1.824712048,3.903042157,-7.016899955));
#126570=CARTESIAN_POINT('Ctrl Pts',(-1.885467899,3.892857143,-7.000536465));
#126571=CARTESIAN_POINT('Ctrl Pts',(-2.207761753,3.838828313,-6.913732444));
#126572=CARTESIAN_POINT('Ctrl Pts',(-2.520716527,3.783894965,-6.79768256));
#126573=CARTESIAN_POINT('',(-2.06209323492269,3.91326598587965,-7.21094802900807));
#126574=CARTESIAN_POINT('Ctrl Pts',(-2.6035859284959,3.82362522012808,-7.03358658956712));
#126575=CARTESIAN_POINT('Ctrl Pts',(-2.46574044770231,3.84689293573232,
-7.08461212960003));
#126576=CARTESIAN_POINT('Ctrl Pts',(-2.32673141273862,3.86998912007464,
-7.13145703192533));
#126577=CARTESIAN_POINT('Ctrl Pts',(-2.1869371088004,3.89285714276326,-7.17407179237508));
#126578=CARTESIAN_POINT('Ctrl Pts',(-2.14546971161537,3.89964051914521,
-7.18671267363943));
#126579=CARTESIAN_POINT('Ctrl Pts',(-2.10385218957373,3.90644394874722,
-7.19900634661474));
#126580=CARTESIAN_POINT('Ctrl Pts',(-2.0620932340453,3.91326598565651,-7.21094803019025));
#126581=CARTESIAN_POINT('',(-1.91288729329756,3.91326598631302,-7.12157725890554));
#126582=CARTESIAN_POINT('Origin',(-2.96637714392034E-13,4.00453391999933,
-4.55798593312906E-13));
#126583=CARTESIAN_POINT('',(-2.59684572075897,4.00345494161613,-7.03607790633473));
#126584=CARTESIAN_POINT('Origin',(0.0399656944168258,4.16057204697022,0.180618175150855));
#126585=CARTESIAN_POINT('Origin',(0.0687986019714082,4.01785423229436,0.179702194074176));
#126586=CARTESIAN_POINT('Ctrl Pts',(-0.781116749,3.783915088,-7.45921286900001));
#126587=CARTESIAN_POINT('Ctrl Pts',(-1.186522811,3.848090541,-7.41675940000001));
#126588=CARTESIAN_POINT('Ctrl Pts',(-1.5849398,3.913265985,-7.33061838));
#126589=CARTESIAN_POINT('Ctrl Pts',(-1.58893341742117,3.91391928492389,
-7.32975492716629));
#126590=CARTESIAN_POINT('Ctrl Pts',(-1.59292703484234,3.91457258484778,
-7.32889147433258));
#126591=CARTESIAN_POINT('Ctrl Pts',(-0.9911471,3.783915088,-7.18193062000001));
#126592=CARTESIAN_POINT('Ctrl Pts',(-1.381482952,3.848090541,-7.128062062));
#126593=CARTESIAN_POINT('Ctrl Pts',(-1.763681341,3.913265985,-7.032206491));
#126594=CARTESIAN_POINT('Ctrl Pts',(-1.76751238783483,3.91391928492389,
-7.03124566229834));
#126595=CARTESIAN_POINT('Ctrl Pts',(-1.77134343466967,3.91457258484778,
-7.03028483359667));
#126596=CARTESIAN_POINT('',(-1.58493980516177,3.91326598458871,-7.33061837899305));
#126597=CARTESIAN_POINT('',(-1.67431057793867,3.91326598377977,-7.18141243376571));
#126598=CARTESIAN_POINT('',(-1.03070232883522,3.82362522068708,-7.42883925714906));
#126599=CARTESIAN_POINT('Origin',(0.0560818424519852,4.01780061746597,0.180148661364434));
#126600=CARTESIAN_POINT('Ctrl Pts',(-0.995778437857862,3.78467661298457,
-7.18128994883607));
#126601=CARTESIAN_POINT('Ctrl Pts',(-1.00170422328431,3.79148857321378,
-7.22247308061018));
#126602=CARTESIAN_POINT('Ctrl Pts',(-1.00757705172603,3.79813536725245,
-7.26371779929363));
#126603=CARTESIAN_POINT('Ctrl Pts',(-1.01921279396379,3.81110763322192,
-7.34622034452923));
#126604=CARTESIAN_POINT('Ctrl Pts',(-1.02498260530706,3.81744080091515,
-7.3875271267582));
#126605=CARTESIAN_POINT('Ctrl Pts',(-1.03070232734514,3.82362522068701,
-7.42883925735537));
#126606=CARTESIAN_POINT('Ctrl Pts',(-0.463741963,3.913265985,-7.48564916299999));
#126607=CARTESIAN_POINT('Ctrl Pts',(-0.528707983,3.903042157,-7.481624466));
#126608=CARTESIAN_POINT('Ctrl Pts',(-0.593594363,3.892857143,-7.476472814));
#126609=CARTESIAN_POINT('Ctrl Pts',(-0.937799589,3.838828313,-7.449144649));
#126610=CARTESIAN_POINT('Ctrl Pts',(-1.278037818,3.783894965,-7.390305767));
#126611=CARTESIAN_POINT('Ctrl Pts',(-0.210730926,3.913265985,-7.246936765));
#126612=CARTESIAN_POINT('Ctrl Pts',(-0.273625222,3.903042157,-7.245107886));
#126613=CARTESIAN_POINT('Ctrl Pts',(-0.336478302,3.892857143,-7.242187677));
#126614=CARTESIAN_POINT('Ctrl Pts',(-0.669897403,3.838828313,-7.226696737));
#126615=CARTESIAN_POINT('Ctrl Pts',(-1.000482763,3.783894965,-7.18063606100001));
#126616=CARTESIAN_POINT('',(-0.463741967619782,3.9132659854451,-7.48564916201049));
#126617=CARTESIAN_POINT('Ctrl Pts',(-1.0307023309297,3.82362522012805,-7.42883925694053));
#126618=CARTESIAN_POINT('Ctrl Pts',(-0.885110617978232,3.8468929357323,
-7.44903914474112));
#126619=CARTESIAN_POINT('Ctrl Pts',(-0.739281267546468,3.86998912007422,
-7.46490600598539));
#126620=CARTESIAN_POINT('Ctrl Pts',(-0.593594363125153,3.89285714293964,
-7.47647281373311));
#126621=CARTESIAN_POINT('Ctrl Pts',(-0.550379035012223,3.89964051906683,
-7.47990389320791));
#126622=CARTESIAN_POINT('Ctrl Pts',(-0.507091730846385,3.90644394833732,
-7.48296361012156));
#126623=CARTESIAN_POINT('Ctrl Pts',(-0.463741966732096,3.91326598441267,
-7.48564916276879));
#126624=CARTESIAN_POINT('',(-0.337236452565506,3.91326598631302,-7.36629296363075));
#126625=CARTESIAN_POINT('Origin',(-1.8564251698383E-13,4.00453391999933,
-1.12800394025392E-12));
#126626=CARTESIAN_POINT('',(-1.02358414613794,4.00345494160212,-7.4298233824669));
#126627=CARTESIAN_POINT('Origin',(0.000203746966547652,4.16057200674162,
0.184986838640377));
#126628=CARTESIAN_POINT('Origin',(0.0285594814776714,4.01785425606131,0.190290541207166));
#126629=CARTESIAN_POINT('Ctrl Pts',(0.840655601,3.783915088,-7.452737629));
#126630=CARTESIAN_POINT('Ctrl Pts',(0.435601466,3.848090541,-7.498427017));
#126631=CARTESIAN_POINT('Ctrl Pts',(0.027981472,3.913265985,-7.499947802));
#126632=CARTESIAN_POINT('Ctrl Pts',(0.0238956063009955,3.91391928492389,
-7.49996304591187));
#126633=CARTESIAN_POINT('Ctrl Pts',(0.0198097406019911,3.91457258484778,
-7.49997828982376));
#126634=CARTESIAN_POINT('Ctrl Pts',(0.575928156,3.783915088,-7.227088401));
#126635=CARTESIAN_POINT('Ctrl Pts',(0.183137991,3.848090541,-7.25838993));
#126636=CARTESIAN_POINT('Ctrl Pts',(-0.210730926,3.913265985,-7.246936765));
#126637=CARTESIAN_POINT('Ctrl Pts',(-0.214678954854233,3.91391928492389,
-7.24682196176486));
#126638=CARTESIAN_POINT('Ctrl Pts',(-0.218626983708466,3.91457258484778,
-7.24670715852972));
#126639=CARTESIAN_POINT('',(0.0279814687166059,3.91326598458875,-7.49994780268229));
#126640=CARTESIAN_POINT('',(-0.091374734637584,3.91326598377977,-7.37344228340535));
#126641=CARTESIAN_POINT('',(0.590375764720165,3.82362522068314,-7.4767276570203));
#126642=CARTESIAN_POINT('Origin',(0.0160440437016413,4.01780066691501,0.187993198170781));
#126643=CARTESIAN_POINT('Ctrl Pts',(0.57126737071102,3.78467661311086,-7.22745830969002));
#126644=CARTESIAN_POINT('Ctrl Pts',(0.574333282887148,3.79148857330225,
-7.26895247153846));
#126645=CARTESIAN_POINT('Ctrl Pts',(0.577464153266443,3.79813536727869,
-7.31049539597131));
#126646=CARTESIAN_POINT('Ctrl Pts',(0.583836056796043,3.81110763340525,
-7.39357041946398));
#126647=CARTESIAN_POINT('Ctrl Pts',(0.587080877680916,3.81744080128018,
-7.43515181229454));
#126648=CARTESIAN_POINT('Ctrl Pts',(0.590375766210829,3.8236252206831,-7.47672765690217));
#126649=CARTESIAN_POINT('Ctrl Pts',(1.156293362,3.913265985,-7.410329659));
#126650=CARTESIAN_POINT('Ctrl Pts',(1.091981021,3.903042157,-7.42036483100001));
#126651=CARTESIAN_POINT('Ctrl Pts',(1.027504195,3.892857143,-7.429282275));
#126652=CARTESIAN_POINT('Ctrl Pts',(0.685471549,3.838828313,-7.476586977));
#126653=CARTESIAN_POINT('Ctrl Pts',(0.340539281,3.783894965,-7.492264878));
#126654=CARTESIAN_POINT('Ctrl Pts',(1.352073032,3.913265985,-7.122808331));
#126655=CARTESIAN_POINT('Ctrl Pts',(1.290256015,3.903042157,-7.134542624));
#126656=CARTESIAN_POINT('Ctrl Pts',(1.228244647,3.892857143,-7.145202243));
#126657=CARTESIAN_POINT('Ctrl Pts',(0.899290605,3.838828313,-7.201748723));
#126658=CARTESIAN_POINT('Ctrl Pts',(0.566532463,3.783894965,-7.227831));
#126659=CARTESIAN_POINT('',(1.15629335682361,3.91326598544904,-7.41032965909334));
#126660=CARTESIAN_POINT('Ctrl Pts',(0.590375762642652,3.82362522012806,
-7.47672765726934));
#126661=CARTESIAN_POINT('Ctrl Pts',(0.736906000733055,3.84689293573232,
-7.46515736797145));
#126662=CARTESIAN_POINT('Ctrl Pts',(0.882736847828371,3.86998912007489,
-7.44930427085053));
#126663=CARTESIAN_POINT('Ctrl Pts',(1.02750419524605,3.89285714303887,-7.42928227496597));
#126664=CARTESIAN_POINT('Ctrl Pts',(1.07044675420083,3.89964051919568,-7.42334311994632));
#126665=CARTESIAN_POINT('Ctrl Pts',(1.11337977344539,3.90644394833732,-7.41702581146743));
#126666=CARTESIAN_POINT('Ctrl Pts',(1.15629335830546,3.91326598441268,-7.41032965957648));
#126667=CARTESIAN_POINT('',(1.25418318904368,3.91326598631302,-7.26656899637323));
#126668=CARTESIAN_POINT('Origin',(-5.45048760899197E-14,4.00453391999978,
-4.81385764583564E-14));
#126669=CARTESIAN_POINT('',(0.597539085963977,4.00345494159452,-7.47615857508329));
#126670=CARTESIAN_POINT('Origin',(-0.039567714929107,4.1605720347916,0.180705713604262));
#126671=CARTESIAN_POINT('Origin',(-0.0130150327720951,4.01785424798534,
0.191980769929868));
#126672=CARTESIAN_POINT('Ctrl Pts',(2.42374296910668,3.783915088,-7.09811240703523));
#126673=CARTESIAN_POINT('Ctrl Pts',(2.03796261175096,3.848090541,-7.22984213651986));
#126674=CARTESIAN_POINT('Ctrl Pts',(1.64017787606862,3.913265985,-7.3189853293929));
#126675=CARTESIAN_POINT('Ctrl Pts',(1.6266288282028,3.91548594250772,-7.32202165853979));
#126676=CARTESIAN_POINT('Ctrl Pts',(1.61307978033704,3.91770590001538,-7.3250579876868));
#126677=CARTESIAN_POINT('Ctrl Pts',(2.116073651,3.783915088,-6.93431556100001));
#126678=CARTESIAN_POINT('Ctrl Pts',(1.739195605,3.848090541,-7.049323552));
#126679=CARTESIAN_POINT('Ctrl Pts',(1.352073032,3.913265985,-7.122808331));
#126680=CARTESIAN_POINT('Ctrl Pts',(1.33888715079087,3.91548594250772,-7.1253113148975));
#126681=CARTESIAN_POINT('Ctrl Pts',(1.32570126958175,3.91770590001538,-7.12781429879499));
#126682=CARTESIAN_POINT('',(1.6395943529807,3.91326598502339,-7.318588002526));
#126683=CARTESIAN_POINT('',(1.49583368902063,3.91326598377977,-7.22069816754942));
#126684=CARTESIAN_POINT('',(2.18384854246494,3.82362522068674,-7.1750125812294));
#126685=CARTESIAN_POINT('Origin',(-0.024743966257188,4.01780066281652,0.187046725071964));
#126686=CARTESIAN_POINT('Ctrl Pts',(2.11160135128517,3.7846766132022,-6.93567875271368));
#126687=CARTESIAN_POINT('Ctrl Pts',(2.1235156023276,3.791488573401,-6.97554372364169));
#126688=CARTESIAN_POINT('Ctrl Pts',(2.13550377534536,3.79813536735995,-7.01544235294169));
#126689=CARTESIAN_POINT('Ctrl Pts',(2.1595853812163,3.81110763330458,-7.09520535668598));
#126690=CARTESIAN_POINT('Ctrl Pts',(2.17169310987897,3.81744080099409,-7.13511705796493));
#126691=CARTESIAN_POINT('Ctrl Pts',(2.18384854390247,3.82362522068656,-7.17501258079074));
#126692=CARTESIAN_POINT('Ctrl Pts',(2.722261695,3.913265985,-6.988511377));
#126693=CARTESIAN_POINT('Ctrl Pts',(2.661610206,3.903042157,-7.012137184));
#126694=CARTESIAN_POINT('Ctrl Pts',(2.600557799,3.892857143,-7.034706755));
#126695=CARTESIAN_POINT('Ctrl Pts',(2.276690798,3.838828313,-7.154432408));
#126696=CARTESIAN_POINT('Ctrl Pts',(1.94319314,3.783894965,-7.243894009));
#126697=CARTESIAN_POINT('Ctrl Pts',(2.851655559,3.913265985,-6.665625295));
#126698=CARTESIAN_POINT('Ctrl Pts',(2.793806315,3.903042157,-6.690374079));
#126699=CARTESIAN_POINT('Ctrl Pts',(2.735536241,3.892857143,-6.714115092));
#126700=CARTESIAN_POINT('Ctrl Pts',(2.426428783,3.838828313,-6.840054943));
#126701=CARTESIAN_POINT('Ctrl Pts',(2.10705726,3.783894965,-6.937060595));
#126702=CARTESIAN_POINT('',(2.72226169039741,3.9132659854451,-6.98851137802784));
#126703=CARTESIAN_POINT('Ctrl Pts',(2.18384854047772,3.823625220128,-7.17501258191799));
#126704=CARTESIAN_POINT('Ctrl Pts',(2.32446571297695,3.84689293573225,-7.13221312998114));
#126705=CARTESIAN_POINT('Ctrl Pts',(2.46347916887734,3.86998912007484,-7.08538134813477));
#126706=CARTESIAN_POINT('Ctrl Pts',(2.60055779923158,3.89285714303828,-7.03470675491019));
#126707=CARTESIAN_POINT('Ctrl Pts',(2.6412196424011,3.89964051919493,-7.01967507308682));
#126708=CARTESIAN_POINT('Ctrl Pts',(2.68179087705118,3.90644394833732,-7.00427612982547));
#126709=CARTESIAN_POINT('Ctrl Pts',(2.72226169151576,3.91326598441267,-6.98851137835724));
#126710=CARTESIAN_POINT('',(2.7869586195249,3.91326598631302,-6.8270683390515));
#126711=CARTESIAN_POINT('Origin',(3.67436116255337E-13,4.00453392,-1.32055824608734E-12));
#126712=CARTESIAN_POINT('',(2.19072205418073,4.00345494162733,-7.17291690205873));
#126713=CARTESIAN_POINT('Origin',(-0.0774889773561682,4.16057201301482,
0.167974844056662));
#126714=CARTESIAN_POINT('Origin',(-0.0539810493423482,4.01785423855514,
0.184694845267614));
#126715=CARTESIAN_POINT('Ctrl Pts',(3.89296155423979,3.783915088,-6.41112939026784));
#126716=CARTESIAN_POINT('Ctrl Pts',(3.54451852593086,3.848090541,-6.62271072494345));
#126717=CARTESIAN_POINT('Ctrl Pts',(3.17519692666322,3.913265985,-6.79528175958383));
#126718=CARTESIAN_POINT('Ctrl Pts',(3.16261736907935,3.91548594249093,-6.80115974579389));
#126719=CARTESIAN_POINT('Ctrl Pts',(3.15003781149546,3.91770589998178,-6.80703773200397));
#126720=CARTESIAN_POINT('Ctrl Pts',(3.557273893,3.783915088,-6.317301833));
#126721=CARTESIAN_POINT('Ctrl Pts',(3.213930366,3.848090541,-6.51063864));
#126722=CARTESIAN_POINT('Ctrl Pts',(2.851655559,3.913265985,-6.665625295));
#126723=CARTESIAN_POINT('Ctrl Pts',(2.83931602401239,3.91548594249093,-6.67090433515139));
#126724=CARTESIAN_POINT('Ctrl Pts',(2.82697648902474,3.91770589998178,-6.67618337530266));
#126725=CARTESIAN_POINT('',(3.17454163251317,3.91326598502339,-6.79501916224925));
#126726=CARTESIAN_POINT('',(3.01309859252858,3.91326598377977,-6.73032223012104));
#126727=CARTESIAN_POINT('',(3.67520699077175,3.82362522066602,-6.53780189151137));
#126728=CARTESIAN_POINT('Origin',(-0.0643749718556375,4.01780061212694,
0.17735441925624));
#126729=CARTESIAN_POINT('Ctrl Pts',(3.55319919914492,3.78467661303912,-6.31959456555699));
#126730=CARTESIAN_POINT('Ctrl Pts',(3.57340469212595,3.7914885732178,-6.35596630351304));
#126731=CARTESIAN_POINT('Ctrl Pts',(3.59368961467049,3.79813536727529,-6.39235502254762));
#126732=CARTESIAN_POINT('Ctrl Pts',(3.63435489786552,3.81110763438811,-6.4650763843928));
#126733=CARTESIAN_POINT('Ctrl Pts',(3.65475939482177,3.81744080329316,-6.50145217583232));
#126734=CARTESIAN_POINT('Ctrl Pts',(3.67520699201307,3.82362522066573,-6.53780189076739));
#126735=CARTESIAN_POINT('Ctrl Pts',(4.160940096,3.913265985,-6.23991807));
#126736=CARTESIAN_POINT('Ctrl Pts',(4.106785456,3.903042157,-6.27602979600001));
#126737=CARTESIAN_POINT('Ctrl Pts',(4.052012211,3.892857143,-6.311196166));
#126738=CARTESIAN_POINT('Ctrl Pts',(3.761454517,3.838828313,-6.49774453));
#126739=CARTESIAN_POINT('Ctrl Pts',(3.454985449,3.783894965,-6.656806708));
#126740=CARTESIAN_POINT('Ctrl Pts',(4.21789784,3.913265985,-5.89676502900001));
#126741=CARTESIAN_POINT('Ctrl Pts',(4.166721337,3.903042157,-5.93337107700001));
#126742=CARTESIAN_POINT('Ctrl Pts',(4.114917201,3.892857143,-5.969083383));
#126743=CARTESIAN_POINT('Ctrl Pts',(3.840109849,3.838828313,-6.15852779600001));
#126744=CARTESIAN_POINT('Ctrl Pts',(3.549058402,3.783894965,-6.32192094700001));
#126745=CARTESIAN_POINT('',(4.16094009122337,3.91326598587964,-6.23991807225179));
#126746=CARTESIAN_POINT('Ctrl Pts',(3.67520698908242,3.82362522012807,-6.53780189263945));
#126747=CARTESIAN_POINT('Ctrl Pts',(3.80333599309538,3.84689293573232,-6.46577453255949));
#126748=CARTESIAN_POINT('Ctrl Pts',(3.92903194273447,3.86998912007464,-6.39015386811644));
#126749=CARTESIAN_POINT('Ctrl Pts',(4.05201221122165,3.89285714276326,-6.31119616555459));
#126750=CARTESIAN_POINT('Ctrl Pts',(4.08849203547497,3.89964051914521,-6.28777482204693));
#126751=CARTESIAN_POINT('Ctrl Pts',(4.12480441948583,3.90644394874722,-6.26401428120537));
#126752=CARTESIAN_POINT('Ctrl Pts',(4.16094009247477,3.91326598565652,-6.23991807212533));
#126753=CARTESIAN_POINT('',(4.18941896135557,3.91326598631303,-6.06834155408714));
#126754=CARTESIAN_POINT('Origin',(5.49039980146659E-13,4.00453391999933,
-7.86263415486488E-13));
#126755=CARTESIAN_POINT('',(3.68146929365972,4.00345494161081,-6.53427760673526));
#126756=CARTESIAN_POINT('Origin',(-0.111786908240756,4.1605720525608,0.147389746905117));
#126757=CARTESIAN_POINT('Origin',(-0.0924228179123909,4.01785422783766,
0.168772261566034));
#126758=CARTESIAN_POINT('Ctrl Pts',(5.18014958364216,3.783915088,-5.42436908871496));
#126759=CARTESIAN_POINT('Ctrl Pts',(4.88533669232189,3.848090541,-5.7059087207646));
#126760=CARTESIAN_POINT('Ctrl Pts',(4.56174729882825,3.913265985,-5.95383836687107));
#126761=CARTESIAN_POINT('Ctrl Pts',(4.5507254370256,3.91548594261029,-5.9622831625013));
#126762=CARTESIAN_POINT('Ctrl Pts',(4.53970357522298,3.91770590022054,-5.97072795813157));
#126763=CARTESIAN_POINT('Ctrl Pts',(4.832139962,3.783915088,-5.404898092));
#126764=CARTESIAN_POINT('Ctrl Pts',(4.538385314,3.848090541,-5.667523501));
#126765=CARTESIAN_POINT('Ctrl Pts',(4.21789784,3.913265985,-5.896765029));
#126766=CARTESIAN_POINT('Ctrl Pts',(4.20698163347736,3.91548594261029,-5.90457328381877));
#126767=CARTESIAN_POINT('Ctrl Pts',(4.1960654269548,3.91770590022053,-5.91238153863744));
#126768=CARTESIAN_POINT('',(4.56105087436595,3.91326598502339,-5.95372277775558));
#126769=CARTESIAN_POINT('',(4.38947435436249,3.91326598377977,-5.92524390554672));
#126770=CARTESIAN_POINT('',(4.99471684429243,3.82362522071687,-5.59489085202631));
#126771=CARTESIAN_POINT('Origin',(-0.100995931843701,4.017800660735,0.159369335230573));
#126772=CARTESIAN_POINT('Ctrl Pts',(4.82865340169588,3.78467661288032,-5.40801315977069));
#126773=CARTESIAN_POINT('Ctrl Pts',(4.8562052884917,3.79148855789405,-5.43919089353966));
#126774=CARTESIAN_POINT('Ctrl Pts',(4.88383838974289,3.79813533635186,-5.47036812749705));
#126775=CARTESIAN_POINT('Ctrl Pts',(4.93918600393071,3.81110763150659,-5.53264760509342));
#126776=CARTESIAN_POINT('Ctrl Pts',(4.96693316125902,3.81744079750135,-5.5637865717557));
#126777=CARTESIAN_POINT('Ctrl Pts',(4.99471684547528,3.82362522071682,-5.59489085096975));
#126778=CARTESIAN_POINT('Ctrl Pts',(5.405057563,3.913265985,-5.199553129));
#126779=CARTESIAN_POINT('Ctrl Pts',(5.359931982,3.903042157,-5.24646223));
#126780=CARTESIAN_POINT('Ctrl Pts',(5.313999035,3.892857143,-5.292581058));
#126781=CARTESIAN_POINT('Ctrl Pts',(5.070336803,3.838828313,-5.537229341));
#126782=CARTESIAN_POINT('Ctrl Pts',(4.805226477,3.783894965,-5.758454524));
#126783=CARTESIAN_POINT('Ctrl Pts',(5.386915907,3.913265985,-4.852178584));
#126784=CARTESIAN_POINT('Ctrl Pts',(5.3448051,3.903042157,-4.898930239));
#126785=CARTESIAN_POINT('Ctrl Pts',(5.301889206,3.892857143,-4.944943968));
#126786=CARTESIAN_POINT('Ctrl Pts',(5.074231646,3.838828313,-5.189034734));
#126787=CARTESIAN_POINT('Ctrl Pts',(4.825109518,3.783894965,-5.411175301));
#126788=CARTESIAN_POINT('',(5.40505755925474,3.9132659854451,-5.19955313187586));
#126789=CARTESIAN_POINT('Ctrl Pts',(4.9947168426979,3.82362522012808,-5.59489085356987));
#126790=CARTESIAN_POINT('Ctrl Pts',(5.10436650864171,3.84689293573234,-5.49700350466743));
#126791=CARTESIAN_POINT('Ctrl Pts',(5.21086754932514,3.86998912007495,-5.39612989562032));
#126792=CARTESIAN_POINT('Ctrl Pts',(5.31399903520763,3.89285714304604,-5.29258105779153));
#126793=CARTESIAN_POINT('Ctrl Pts',(5.34459108521124,3.899640519205,-5.26186520817721));
#126794=CARTESIAN_POINT('Ctrl Pts',(5.37494669178829,3.90644394833732,-5.23085408659784));
#126795=CARTESIAN_POINT('Ctrl Pts',(5.40505756040768,3.91326598441267,-5.19955313169478));
#126796=CARTESIAN_POINT('',(5.39598672949708,3.91326598631302,-5.02586586240818));
#126797=CARTESIAN_POINT('Origin',(1.03562991515815E-12,4.00453391999933,
-1.23989360445442E-12));
#126798=CARTESIAN_POINT('',(5.00007512100252,4.00345494156695,-5.59010275254307));
#126799=CARTESIAN_POINT('Origin',(-0.14085793492312,4.16057199345265,0.119913108511505));
#126800=CARTESIAN_POINT('Origin',(-0.126543208492973,4.01785425210612,0.144958433320892));
#126801=CARTESIAN_POINT('Ctrl Pts',(6.224422733,3.783915088,-4.184084325));
#126802=CARTESIAN_POINT('Ctrl Pts',(5.99701896,3.848090541,-4.5223799));
#126803=CARTESIAN_POINT('Ctrl Pts',(5.734290451,3.913265985,-4.834036928));
#126804=CARTESIAN_POINT('Ctrl Pts',(5.73165693591518,3.91391928492389,-4.83716088850072));
#126805=CARTESIAN_POINT('Ctrl Pts',(5.72902342083036,3.91457258484779,-4.84028484900144));
#126806=CARTESIAN_POINT('Ctrl Pts',(5.88106053800001,3.783915088,-4.239767323));
#126807=CARTESIAN_POINT('Ctrl Pts',(5.65063041,3.848090541,-4.559401263));
#126808=CARTESIAN_POINT('Ctrl Pts',(5.386915907,3.913265985,-4.852178584));
#126809=CARTESIAN_POINT('Ctrl Pts',(5.38427250859463,3.91391928492389,-4.85511329974243));
#126810=CARTESIAN_POINT('Ctrl Pts',(5.38162911018926,3.91457258484779,-4.85804801548486));
#126811=CARTESIAN_POINT('',(5.73429044772017,3.9132659845887,-4.83403693208736));
#126812=CARTESIAN_POINT('',(5.56060317398342,3.91326598377978,-4.84310776175977));
#126813=CARTESIAN_POINT('',(6.08067928922541,3.82362522067835,-4.39036893445263));
#126814=CARTESIAN_POINT('Origin',(-0.132894517210351,4.01780063623296,0.133932311186329));
#126815=CARTESIAN_POINT('Ctrl Pts',(5.87832513986311,3.78467661310213,-4.24355907047409));
#126816=CARTESIAN_POINT('Ctrl Pts',(5.91193524479655,3.79148857330863,-4.26808509992057));
#126817=CARTESIAN_POINT('Ctrl Pts',(5.94562456780292,3.79813536728978,-4.2925931888642));
#126818=CARTESIAN_POINT('Ctrl Pts',(6.01306644055515,3.81110766408669,-4.34151851229078));
#126819=CARTESIAN_POINT('Ctrl Pts',(6.04685903415429,3.81744086360286,-4.36596478657745));
#126820=CARTESIAN_POINT('Ctrl Pts',(6.08067929013269,3.82362522067827,-4.3903689331953));
#126821=CARTESIAN_POINT('Ctrl Pts',(6.396440546,3.913265985,-3.916062862));
#126822=CARTESIAN_POINT('Ctrl Pts',(6.362454046,3.903042157,-3.971575921));
#126823=CARTESIAN_POINT('Ctrl Pts',(6.327509171,3.892857143,-4.026490742));
#126824=CARTESIAN_POINT('Ctrl Pts',(6.142135775,3.838828313,-4.317799462));
#126825=CARTESIAN_POINT('Ctrl Pts',(5.930780456,3.783894965,-4.590843406));
#126826=CARTESIAN_POINT('Ctrl Pts',(6.304047773,3.913265985,-3.580709661));
#126827=CARTESIAN_POINT('Ctrl Pts',(6.272971717,3.903042157,-3.635420867));
#126828=CARTESIAN_POINT('Ctrl Pts',(6.240950764,3.892857143,-3.68958447));
#126829=CARTESIAN_POINT('Ctrl Pts',(6.07108801100001,3.838828313,-3.976908175));
#126830=CARTESIAN_POINT('Ctrl Pts',(5.875543876,3.783894965,-4.247409112));
#126831=CARTESIAN_POINT('',(6.39644054272282,3.91326598544903,-3.91606286599203));
#126832=CARTESIAN_POINT('Ctrl Pts',(6.08067928814615,3.82362522012804,-4.3903689362603));
#126833=CARTESIAN_POINT('Ctrl Pts',(6.16672251947261,3.8468929357323,-4.27119870229895));
#126834=CARTESIAN_POINT('Ctrl Pts',(6.24904878106583,3.86998912007446,-4.14978888647607));
#126835=CARTESIAN_POINT('Ctrl Pts',(6.3275091708798,3.89285714297538,-4.02649074199364));
#126836=CARTESIAN_POINT('Ctrl Pts',(6.35078299564904,3.89964051911324,-3.98991662566928));
#126837=CARTESIAN_POINT('Ctrl Pts',(6.37376243079214,3.90644394833732,-3.95310496831084));
#126838=CARTESIAN_POINT('Ctrl Pts',(6.39644054404758,3.91326598441267,-3.91606286518905));
#126839=CARTESIAN_POINT('',(6.35024415539581,3.91326598631302,-3.74838626845302));
#126840=CARTESIAN_POINT('Origin',(-1.17093834628434E-13,4.00453392000044,
1.46150452851046E-13));
#126841=CARTESIAN_POINT('',(6.08488299311143,4.00345494165009,-4.38454090602215));
#126842=CARTESIAN_POINT('Origin',(-0.163342471740709,4.16057201846061,0.0868292585406771));
#126843=CARTESIAN_POINT('Origin',(-0.154746379352955,4.01785422327006,0.114366264473377));
#126844=CARTESIAN_POINT('Ctrl Pts',(6.97900989537378,3.783915088,-2.74793569772871));
#126845=CARTESIAN_POINT('Ctrl Pts',(6.829660385282,3.848090541,-3.12724286712813));
#126846=CARTESIAN_POINT('Ctrl Pts',(6.64008156229168,3.913265985,-3.48812937990599));
#126847=CARTESIAN_POINT('Ctrl Pts',(6.63362426926477,3.91548594255344,-3.50042162819467));
#126848=CARTESIAN_POINT('Ctrl Pts',(6.62716697623774,3.91770590010688,-3.51271387648341));
#126849=CARTESIAN_POINT('Ctrl Pts',(6.654989258,3.783915088,-2.876389747));
#126850=CARTESIAN_POINT('Ctrl Pts',(6.498658307,3.848090541,-3.238086488));
#126851=CARTESIAN_POINT('Ctrl Pts',(6.304047773,3.913265985,-3.580709661));
#126852=CARTESIAN_POINT('Ctrl Pts',(6.29741909357082,3.91548594255344,-3.59237983697737));
#126853=CARTESIAN_POINT('Ctrl Pts',(6.2907904141416,3.91770590010688,-3.60405001295468));
#126854=CARTESIAN_POINT('',(6.63940096982187,3.91326598502339,-3.48831689502031));
#126855=CARTESIAN_POINT('',(6.47172436983887,3.91326598377977,-3.53451328120357));
#126856=CARTESIAN_POINT('',(6.88231592933023,3.82362522069825,-2.98055824466829));
#126857=CARTESIAN_POINT('Origin',(-0.15857890756012,4.01780063905968,0.102232605658803));
#126858=CARTESIAN_POINT('Ctrl Pts',(6.65313292416621,3.78467661285622,-2.88068087466204));
#126859=CARTESIAN_POINT('Ctrl Pts',(6.69122961500491,3.79148857305671,-2.89740831972643));
#126860=CARTESIAN_POINT('Ctrl Pts',(6.72939981611138,3.79813536720143,-2.91410121473867));
#126861=CARTESIAN_POINT('Ctrl Pts',(6.80578224859457,3.81110763252607,-2.94738460114917));
#126862=CARTESIAN_POINT('Ctrl Pts',(6.84403980611034,3.81744079956995,-2.96399483581662));
#126863=CARTESIAN_POINT('Ctrl Pts',(6.88231592994026,3.82362522069821,-2.9805582432586));
#126864=CARTESIAN_POINT('Ctrl Pts',(7.088733078,3.913265985,-2.449461849));
#126865=CARTESIAN_POINT('Ctrl Pts',(7.06747483,3.903042157,-2.510983136));
#126866=CARTESIAN_POINT('Ctrl Pts',(7.04515201,3.892857143,-2.572126194));
#126867=CARTESIAN_POINT('Ctrl Pts',(6.926735305,3.838828313,-2.896474078));
#126868=CARTESIAN_POINT('Ctrl Pts',(6.779017733,3.783894965,-3.208569553));
#126869=CARTESIAN_POINT('Ctrl Pts',(6.926409371,3.913265985,-2.141810735));
#126870=CARTESIAN_POINT('Ctrl Pts',(6.907821148,3.903042157,-2.201923256));
#126871=CARTESIAN_POINT('Ctrl Pts',(6.888192401,3.892857143,-2.261704102));
#126872=CARTESIAN_POINT('Ctrl Pts',(6.784067048,3.838828313,-2.578825809));
#126873=CARTESIAN_POINT('Ctrl Pts',(6.65124433100001,3.783894965,-2.885038794));
#126874=CARTESIAN_POINT('',(7.08873307580789,3.9132659854451,-2.44946185318189));
#126875=CARTESIAN_POINT('Ctrl Pts',(6.88231592855685,3.82362522012813,-2.9805582466734));
#126876=CARTESIAN_POINT('Ctrl Pts',(6.94072943918886,3.84689293573239,-2.84567739513467));
#126877=CARTESIAN_POINT('Ctrl Pts',(6.99503143687744,3.86998912007453,-2.70940836070635));
#126878=CARTESIAN_POINT('Ctrl Pts',(7.04515200990613,3.89285714297705,-2.57212619405164));
#126879=CARTESIAN_POINT('Ctrl Pts',(7.0600193517086,3.8996405191154,-2.53140397600461));
#126880=CARTESIAN_POINT('Ctrl Pts',(7.0745481222804,3.90644394833732,-2.49051305559514));
#126881=CARTESIAN_POINT('Ctrl Pts',(7.08873307677877,3.91326598441267,-2.44946185253423));
#126882=CARTESIAN_POINT('',(7.00757122198645,3.91326598631302,-2.29563629967278));
#126883=CARTESIAN_POINT('Origin',(-1.25247034965525E-12,4.00453392000044,
6.18862600054726E-13));
#126884=CARTESIAN_POINT('',(6.88516849880378,4.00345494158127,-2.9739628013933));
#126885=CARTESIAN_POINT('Origin',(-0.178189687407482,4.16057206045661,0.0496855948308278));
#126886=CARTESIAN_POINT('Origin',(-0.175713817176157,4.01785418818641,0.0784265254962754));
#126887=CARTESIAN_POINT('Ctrl Pts',(7.405984482,3.783915088,-1.183804818));
#126888=CARTESIAN_POINT('Ctrl Pts',(7.341645033,3.848090541,-1.586317932));
#126889=CARTESIAN_POINT('Ctrl Pts',(7.234060485,3.913265985,-1.979487028));
#126890=CARTESIAN_POINT('Ctrl Pts',(7.23298208840295,3.91391928492389,-1.98342804204961));
#126891=CARTESIAN_POINT('Ctrl Pts',(7.23190369180592,3.91457258484779,-1.98736905609922));
#126892=CARTESIAN_POINT('Ctrl Pts',(7.117738078,3.783915088,-1.378515382));
#126893=CARTESIAN_POINT('Ctrl Pts',(7.042816165,3.848090541,-1.765362388));
#126894=CARTESIAN_POINT('Ctrl Pts',(6.92640937100001,3.913265985,-2.141810735));
#126895=CARTESIAN_POINT('Ctrl Pts',(6.92524254274394,3.91391928492389,-2.14558414506598));
#126896=CARTESIAN_POINT('Ctrl Pts',(6.92407571448788,3.91457258484779,-2.14935755513196));
#126897=CARTESIAN_POINT('',(7.23406048375419,3.9132659845887,-1.97948703307904));
#126898=CARTESIAN_POINT('',(7.08023492586553,3.91326598377977,-2.06064888883387));
#126899=CARTESIAN_POINT('',(7.36214312522358,3.82362522066215,-1.43137996415906));
#126900=CARTESIAN_POINT('Origin',(-0.176848370913549,4.01780060574887,0.0657526788448023));
#126901=CARTESIAN_POINT('Ctrl Pts',(7.11684761097684,3.78467661312194,-1.38310524299807));
#126902=CARTESIAN_POINT('Ctrl Pts',(7.15764952855394,3.79148857330044,-1.39125194736918));
#126903=CARTESIAN_POINT('Ctrl Pts',(7.19851580975261,3.79813536730619,-1.39934910677069));
#126904=CARTESIAN_POINT('Ctrl Pts',(7.2802674200159,3.81110763459257,-1.41543438358567));
#126905=CARTESIAN_POINT('Ctrl Pts',(7.32120126067541,3.81744080367663,-1.42343203901384));
#126906=CARTESIAN_POINT('Ctrl Pts',(7.36214312549663,3.82362522066195,-1.43137996274802));
#126907=CARTESIAN_POINT('Ctrl Pts',(7.44956433,3.913265985,-0.868326722));
#126908=CARTESIAN_POINT('Ctrl Pts',(7.442028346,3.903042157,-0.93297957));
#126909=CARTESIAN_POINT('Ctrl Pts',(7.433371371,3.892857143,-0.997491884));
#126910=CARTESIAN_POINT('Ctrl Pts',(7.38744839000001,3.838828313,-1.339712786));
#126911=CARTESIAN_POINT('Ctrl Pts',(7.310275675,3.783894965,-1.676266553));
#126912=CARTESIAN_POINT('Ctrl Pts',(7.224899766,3.913265985,-0.602763118));
#126913=CARTESIAN_POINT('Ctrl Pts',(7.21966854,3.903042157,-0.665466161));
#126914=CARTESIAN_POINT('Ctrl Pts',(7.213349817,3.892857143,-0.728068964));
#126915=CARTESIAN_POINT('Ctrl Pts',(7.17983065,3.838828313,-1.060160415));
#126916=CARTESIAN_POINT('Ctrl Pts',(7.115939995,3.783894965,-1.387767269));
#126917=CARTESIAN_POINT('',(7.44956432875072,3.91326598544511,-0.868326726546466));
#126918=CARTESIAN_POINT('Ctrl Pts',(7.36214312491588,3.82362522012806,-1.43137996614573));
#126919=CARTESIAN_POINT('Ctrl Pts',(7.39019556395953,3.84689293573232,-1.28709537604623));
#126920=CARTESIAN_POINT('Ctrl Pts',(7.41393419676835,3.8699891200747,-1.14233891164205));
#126921=CARTESIAN_POINT('Ctrl Pts',(7.4333713710084,3.89285714300989,-0.997491883937365));
#126922=CARTESIAN_POINT('Ctrl Pts',(7.43913704965416,3.89964051915805,-0.954525689482439));
#126923=CARTESIAN_POINT('Ctrl Pts',(7.44453580649954,3.90644394833731,-0.911467520086951));
#126924=CARTESIAN_POINT('Ctrl Pts',(7.44956432956707,3.91326598441266,-0.868326725714184));
#126925=CARTESIAN_POINT('',(7.33723204719462,3.91326598631305,-0.735544928033871));
#126926=CARTESIAN_POINT('Origin',(-1.03649727689614E-13,4.00453392000044,
4.01154803819637E-14));
#126927=CARTESIAN_POINT('',(7.36351117796384,4.0034549415695,-1.42432549981701));
#126928=CARTESIAN_POINT('Origin',(-0.184704478685992,4.16057204671496,0.010218425212104));
#126929=CARTESIAN_POINT('Origin',(-0.188465182015064,4.01785424450927,0.0388197041150465));
#126930=CARTESIAN_POINT('Ctrl Pts',(7.48753937344939,3.783915088,0.436170706963458));
#126931=CARTESIAN_POINT('Ctrl Pts',(7.51124512463192,3.848090541,0.0292251070786374));
#126932=CARTESIAN_POINT('Ctrl Pts',(7.49070676901765,3.913265985,-0.37789263964191));
#126933=CARTESIAN_POINT('Ctrl Pts',(7.49039083490264,3.91426855534244,-0.384155185068383));
#126934=CARTESIAN_POINT('Ctrl Pts',(7.49007490078761,3.91527112568487,-0.390417730494854));
#126935=CARTESIAN_POINT('Ctrl Pts',(7.247669375,3.783915088,0.183816829));
#126936=CARTESIAN_POINT('Ctrl Pts',(7.257659767,3.848090541,-0.210091905));
#126937=CARTESIAN_POINT('Ctrl Pts',(7.224899766,3.913265985,-0.602763118));
#126938=CARTESIAN_POINT('Ctrl Pts',(7.22439583072308,3.91426855534243,-0.608803437609964));
#126939=CARTESIAN_POINT('Ctrl Pts',(7.22389189544616,3.91527112568487,-0.614843757219925));
#126940=CARTESIAN_POINT('',(7.35768156699201,3.91326598377978,-0.490430843621213));
#126941=CARTESIAN_POINT('Ctrl Pts',(7.24778641174106,3.7846766131314,0.179142852983126));
#126942=CARTESIAN_POINT('Ctrl Pts',(7.28938570379294,3.7914885733155,0.179957820111429));
#126943=CARTESIAN_POINT('Ctrl Pts',(7.3310372038869,3.79813536731177,0.180835010192609));
#126944=CARTESIAN_POINT('Ctrl Pts',(7.41433536513795,3.811107634472,0.182699977771355));
#126945=CARTESIAN_POINT('Ctrl Pts',(7.45603145391974,3.81744080342295,0.18368886879813));
#126946=CARTESIAN_POINT('Ctrl Pts',(7.49772469110044,3.82362522066469,0.184728053864386));
#126947=CARTESIAN_POINT('Ctrl Pts',(7.46206223300001,3.913265985,0.753410398));
#126948=CARTESIAN_POINT('Ctrl Pts',(7.468600888,3.903042157,0.688649083));
#126949=CARTESIAN_POINT('Ctrl Pts',(7.474014549,3.892857143,0.623784038));
#126950=CARTESIAN_POINT('Ctrl Pts',(7.502732599,3.838828313,0.279691987));
#126951=CARTESIAN_POINT('Ctrl Pts',(7.499713251,3.783894965,-0.065583193));
#126952=CARTESIAN_POINT('Ctrl Pts',(7.185561877,3.913265985,0.964469032));
#126953=CARTESIAN_POINT('Ctrl Pts',(7.19393225500001,3.903042157,0.902107393));
#126954=CARTESIAN_POINT('Ctrl Pts',(7.201219013,3.892857143,0.839609869));
#126955=CARTESIAN_POINT('Ctrl Pts',(7.23987335,3.838828313,0.508076902));
#126956=CARTESIAN_POINT('Ctrl Pts',(7.247902213,3.783894965,0.174394712));
#126957=CARTESIAN_POINT('',(7.32381205594047,3.91326598631302,0.858939706981007));
#126958=CARTESIAN_POINT('Ctrl Pts',(7.21892121262391,3.783915088,2.03590428179448));
#126959=CARTESIAN_POINT('Ctrl Pts',(7.32957202129409,3.848090541,1.64355800233434));
#126960=CARTESIAN_POINT('Ctrl Pts',(7.39704884754676,3.913265985,1.24153053636633));
#126961=CARTESIAN_POINT('Ctrl Pts',(7.3993471930232,3.91548594250557,1.22783697578976));
#126962=CARTESIAN_POINT('Ctrl Pts',(7.4016455384996,3.91770590001114,1.21414341521315));
#126963=CARTESIAN_POINT('Ctrl Pts',(7.038707708,3.783915088,1.73755397));
#126964=CARTESIAN_POINT('Ctrl Pts',(7.133143264,3.848090541,1.355002242));
#126965=CARTESIAN_POINT('Ctrl Pts',(7.185561877,3.913265985,0.964469032));
#126966=CARTESIAN_POINT('Ctrl Pts',(7.18734732081472,3.91548594250557,0.951166980222463));
#126967=CARTESIAN_POINT('Ctrl Pts',(7.18913276462937,3.91770590001114,0.937864928444939));
#126968=CARTESIAN_POINT('',(7.39662051189907,3.91326598502339,1.24096937987799));
#126969=CARTESIAN_POINT('',(7.29109119514221,3.91326598377978,1.10271920244776));
#126970=CARTESIAN_POINT('',(7.282720983891,3.82362522068904,1.79219839063914));
#126971=CARTESIAN_POINT('Origin',(-0.188112269141258,4.01780062535348,-0.0145812353583524));
#126972=CARTESIAN_POINT('Ctrl Pts',(7.03982677471336,3.78467661306702,1.73301442817107));
#126973=CARTESIAN_POINT('Ctrl Pts',(7.08027830455524,3.79148857324013,1.74275295989348));
#126974=CARTESIAN_POINT('Ctrl Pts',(7.12076744619297,3.79813536730068,1.75256348314844));
#126975=CARTESIAN_POINT('Ctrl Pts',(7.20171741464376,3.81110766407564,1.77229153622958));
#126976=CARTESIAN_POINT('Ctrl Pts',(7.24222629903117,3.81744086360407,1.78222078615965));
#126977=CARTESIAN_POINT('Ctrl Pts',(7.28272098352246,3.82362522068899,1.7921983921349));
#126978=CARTESIAN_POINT('Ctrl Pts',(7.1256424,3.913265985,2.339918885));
#126979=CARTESIAN_POINT('Ctrl Pts',(7.145949953,3.903042157,2.278077271));
#126980=CARTESIAN_POINT('Ctrl Pts',(7.165181113,3.892857143,2.215892511));
#126981=CARTESIAN_POINT('Ctrl Pts',(7.267197371,3.838828313,1.886018673));
#126982=CARTESIAN_POINT('Ctrl Pts',(7.338472571,3.783894965,1.548166765));
#126983=CARTESIAN_POINT('Ctrl Pts',(6.810235101,3.913265985,2.486603681));
#126984=CARTESIAN_POINT('Ctrl Pts',(6.831815693,3.903042157,2.427499407));
#126985=CARTESIAN_POINT('Ctrl Pts',(6.852367211,3.892857143,2.368029478));
#126986=CARTESIAN_POINT('Ctrl Pts',(6.96138761900001,3.838828313,2.052557107));
#126987=CARTESIAN_POINT('Ctrl Pts',(7.040960579,3.783894965,1.72840219));
#126988=CARTESIAN_POINT('',(7.12564240078609,3.91326598544483,2.33991888034567));
#126989=CARTESIAN_POINT('Ctrl Pts',(7.28272098452153,3.82362522012728,1.79219838860444));
#126990=CARTESIAN_POINT('Ctrl Pts',(7.24759716170778,3.84689293573178,1.93492644936675));
#126991=CARTESIAN_POINT('Ctrl Pts',(7.20836009960477,3.86998912007441,2.07627145146909));
#126992=CARTESIAN_POINT('Ctrl Pts',(7.16518111287426,3.89285714300848,2.21589251110512));
#126993=CARTESIAN_POINT('Ctrl Pts',(7.15237286416935,3.89964051915622,2.25730851876993));
#126994=CARTESIAN_POINT('Ctrl Pts',(7.139192987011,3.90644394833732,2.29865393432783));
#126995=CARTESIAN_POINT('Ctrl Pts',(7.1256424011666,3.91326598441267,2.33991888144739));
#126996=CARTESIAN_POINT('',(6.96793875314233,3.91326598631302,2.41326127537066));
#126997=CARTESIAN_POINT('Origin',(6.26235174827627E-13,4.00453392000022,
1.57751416096641E-13));
#126998=CARTESIAN_POINT('',(7.28100050215491,4.00345494179838,1.79917527897799));
#126999=CARTESIAN_POINT('Origin',(-0.171923644953278,4.16057201721044,-0.0682813678646113));
#127000=CARTESIAN_POINT('Origin',(-0.187346446645758,4.01785439732041,-0.0439026729701864));
#127001=CARTESIAN_POINT('Ctrl Pts',(6.61248760692043,3.783915088,3.54016064187857));
#127002=CARTESIAN_POINT('Ctrl Pts',(6.80489431323841,3.848090541,3.18077385319475));
#127003=CARTESIAN_POINT('Ctrl Pts',(6.95721758996345,3.913265985,2.80265108972526));
#127004=CARTESIAN_POINT('Ctrl Pts',(6.96240591211869,3.91548594249667,2.78977175339997));
#127005=CARTESIAN_POINT('Ctrl Pts',(6.967594234274,3.91770589999335,2.77689241707473));
#127006=CARTESIAN_POINT('Ctrl Pts',(6.50062389200001,3.783915088,3.210045018));
#127007=CARTESIAN_POINT('Ctrl Pts',(6.67508891,3.848090541,2.85673799));
#127008=CARTESIAN_POINT('Ctrl Pts',(6.81023510100001,3.913265985,2.486603681));
#127009=CARTESIAN_POINT('Ctrl Pts',(6.8148383500374,3.91548594249667,2.47399644146913));
#127010=CARTESIAN_POINT('Ctrl Pts',(6.81944159907491,3.91770589999335,2.46138920193821));
#127011=CARTESIAN_POINT('',(6.95691990064213,3.91326598502339,2.8020109732692));
#127012=CARTESIAN_POINT('',(6.88357750223904,3.91326598377977,2.64430732386983));
#127013=CARTESIAN_POINT('',(6.72718533731447,3.82362522065873,3.31586752406077));
#127014=CARTESIAN_POINT('Origin',(-0.180579847175079,4.01780064981072,-0.054678938592192));
#127015=CARTESIAN_POINT('Ctrl Pts',(6.50269266259973,3.78467661305534,3.20585217381019));
#127016=CARTESIAN_POINT('Ctrl Pts',(6.54010496184601,3.79148857326335,3.22405890755018));
#127017=CARTESIAN_POINT('Ctrl Pts',(6.57753851684415,3.79813536723926,3.24234403476636));
#127018=CARTESIAN_POINT('Ctrl Pts',(6.65235497190099,3.81110766404678,3.27901270766542));
#127019=CARTESIAN_POINT('Ctrl Pts',(6.68978228575723,3.81744086356219,3.29741803003803));
#127020=CARTESIAN_POINT('Ctrl Pts',(6.72718533666519,3.82362522064911,3.31586752538029));
#127021=CARTESIAN_POINT('Ctrl Pts',(6.456035448,3.913265985,3.817015365));
#127022=CARTESIAN_POINT('Ctrl Pts',(6.48916234,3.903042157,3.760985098));
#127023=CARTESIAN_POINT('Ctrl Pts',(6.521311771,3.892857143,3.704388314));
#127024=CARTESIAN_POINT('Ctrl Pts',(6.691856071,3.838828313,3.404157223));
#127025=CARTESIAN_POINT('Ctrl Pts',(6.83409306900001,3.783894965,3.089526165));
#127026=CARTESIAN_POINT('Ctrl Pts',(6.116469301,3.913265985,3.892467507));
#127027=CARTESIAN_POINT('Ctrl Pts',(6.15025102300001,3.903042157,3.839384247));
#127028=CARTESIAN_POINT('Ctrl Pts',(6.183106334,3.892857143,3.785722661));
#127029=CARTESIAN_POINT('Ctrl Pts',(6.35739514,3.838828313,3.501062024));
#127030=CARTESIAN_POINT('Ctrl Pts',(6.504791453,3.783894965,3.201591502));
#127031=CARTESIAN_POINT('',(6.45603544999917,3.91326598587966,3.81701536011091));
#127032=CARTESIAN_POINT('Ctrl Pts',(6.72718533822867,3.82362522012764,3.31586752225138));
#127033=CARTESIAN_POINT('Ctrl Pts',(6.66220037684142,3.84689293573204,3.44770809685697));
#127034=CARTESIAN_POINT('Ctrl Pts',(6.59349565802203,3.86998912007451,3.57731372301597));
#127035=CARTESIAN_POINT('Ctrl Pts',(6.52131177123793,3.89285714276323,3.70438831419086));
#127036=CARTESIAN_POINT('Ctrl Pts',(6.49989975501614,3.89964051914521,3.74208264361581));
#127037=CARTESIAN_POINT('Ctrl Pts',(6.47813997398258,3.90644394874722,3.77962814197985));
#127038=CARTESIAN_POINT('Ctrl Pts',(6.45603544995081,3.91326598565651,3.81701536137577));
#127039=CARTESIAN_POINT('',(6.28625237872063,3.91326598631302,3.85474142911706));
#127040=CARTESIAN_POINT('Origin',(6.58761240002192E-13,4.00453391999933,
3.91613824701764E-13));
#127041=CARTESIAN_POINT('',(6.72400525501397,4.00345494160178,3.32231144352664));
#127042=CARTESIAN_POINT('Origin',(-0.153225813809006,4.16057200299011,-0.103643539873452));
#127043=CARTESIAN_POINT('Origin',(-0.173528731529875,4.01785423819475,-0.0831502913203769));
#127044=CARTESIAN_POINT('Ctrl Pts',(5.69686142934184,3.783915088,4.87888302588861));
#127045=CARTESIAN_POINT('Ctrl Pts',(5.96202731116912,3.848090541,4.56926025475706));
#127046=CARTESIAN_POINT('Ctrl Pts',(6.19207457063733,3.913265985,4.23272279231243));
#127047=CARTESIAN_POINT('Ctrl Pts',(6.19991026931688,3.91548594250644,4.2212599035295));
#127048=CARTESIAN_POINT('Ctrl Pts',(6.20774596799649,3.91770590001281,4.20979701474663));
#127049=CARTESIAN_POINT('Ctrl Pts',(5.658578127,3.783915088,4.53243792899999));
#127050=CARTESIAN_POINT('Ctrl Pts',(5.904914818,3.848090541,4.224895844));
#127051=CARTESIAN_POINT('Ctrl Pts',(6.116469301,3.913265985,3.892467507));
#127052=CARTESIAN_POINT('Ctrl Pts',(6.12367511247948,3.91548594250644,3.88114458019227));
#127053=CARTESIAN_POINT('Ctrl Pts',(6.13088092395888,3.91770590001281,3.86982165338449));
#127054=CARTESIAN_POINT('',(6.19192144724153,3.91326598502339,4.23203364701685));
#127055=CARTESIAN_POINT('',(6.15419537620777,3.91326598377977,4.06225057412534));
#127056=CARTESIAN_POINT('',(5.8570939813402,3.82362522065945,4.68449037745577));
#127057=CARTESIAN_POINT('Origin',(-0.164603298449912,4.01780062929309,-0.0922196567071654));
#127058=CARTESIAN_POINT('Ctrl Pts',(5.66149986785939,3.78467661292693,4.52878783530389));
#127059=CARTESIAN_POINT('Ctrl Pts',(5.69412357866396,3.79148857310069,4.55461144403524));
#127060=CARTESIAN_POINT('Ctrl Pts',(5.72675119669208,3.79813536718563,4.58051618334602));
#127061=CARTESIAN_POINT('Ctrl Pts',(5.79193565618604,3.81110763458452,4.63241077165652));
#127062=CARTESIAN_POINT('Ctrl Pts',(5.82453117336164,3.81744080378591,4.65843141993921));
#127063=CARTESIAN_POINT('Ctrl Pts',(5.85709398044422,3.82362522065944,4.68449037857536));
#127064=CARTESIAN_POINT('Ctrl Pts',(5.48455145300001,3.913265985,5.115632449));
#127065=CARTESIAN_POINT('Ctrl Pts',(5.528948709,3.903042157,5.068033441));
#127066=CARTESIAN_POINT('Ctrl Pts',(5.57251314,3.892857143,5.019671036));
#127067=CARTESIAN_POINT('Ctrl Pts',(5.803611018,3.838828313,4.763121164));
#127068=CARTESIAN_POINT('Ctrl Pts',(6.010158971,3.783894965,4.486422756));
#127069=CARTESIAN_POINT('Ctrl Pts',(5.136704194,3.913265985,5.116323878));
#127070=CARTESIAN_POINT('Ctrl Pts',(5.18110745,3.903042157,5.071743746));
#127071=CARTESIAN_POINT('Ctrl Pts',(5.224730277,3.892857143,5.026399659));
#127072=CARTESIAN_POINT('Ctrl Pts',(5.45613793,3.838828313,4.785861171));
#127073=CARTESIAN_POINT('Ctrl Pts',(5.664465509,3.783894965,4.525077954));
#127074=CARTESIAN_POINT('',(5.48455145598281,3.91326598544904,5.11563244476761));
#127075=CARTESIAN_POINT('Ctrl Pts',(5.85709398265966,3.82362522012791,4.68449037594388));
#127076=CARTESIAN_POINT('Ctrl Pts',(5.76528650735208,3.84689293573221,4.79927874531267));
#127077=CARTESIAN_POINT('Ctrl Pts',(5.67032668828692,3.86998912007453,4.91108478021124));
#127078=CARTESIAN_POINT('Ctrl Pts',(5.57251313993674,3.89285714299297,5.01967103596844));
#127079=CARTESIAN_POINT('Ctrl Pts',(5.54349855809972,3.89964051913609,5.05188114233675));
#127080=CARTESIAN_POINT('Ctrl Pts',(5.51417633597186,3.90644394833732,5.08387113827877));
#127081=CARTESIAN_POINT('Ctrl Pts',(5.48455145555049,3.91326598441267,5.11563244626558));
#127082=CARTESIAN_POINT('',(5.31062782910159,3.91326598631302,5.11597815768528));
#127083=CARTESIAN_POINT('Origin',(8.0708009719821E-13,4.00453392000044,
6.55725473919233E-13));
#127084=CARTESIAN_POINT('',(5.85260299487725,4.00345494155467,4.69010001812929));
#127085=CARTESIAN_POINT('Origin',(-0.127363302147928,4.16057203396705,-0.134159530637787));
#127086=CARTESIAN_POINT('Origin',(-0.151596600062219,4.01785425931465,-0.118509602027252));
#127087=CARTESIAN_POINT('Ctrl Pts',(4.51485634319997,3.783915088,5.98947426037819));
#127088=CARTESIAN_POINT('Ctrl Pts',(4.84038253734848,3.848090541,5.74409312384617));
#127089=CARTESIAN_POINT('Ctrl Pts',(5.13739702623243,3.913265985,5.46487708158082));
#127090=CARTESIAN_POINT('Ctrl Pts',(5.14751371322919,3.91548594258288,5.45536663205805));
#127091=CARTESIAN_POINT('Ctrl Pts',(5.15763040022591,3.9177059001657,5.44585618253516));
#127092=CARTESIAN_POINT('Ctrl Pts',(4.551943538,3.783915088,5.64289908));
#127093=CARTESIAN_POINT('Ctrl Pts',(4.858633471,3.848090541,5.395502265));
#127094=CARTESIAN_POINT('Ctrl Pts',(5.136704194,3.913265985,5.11632387800001));
#127095=CARTESIAN_POINT('Ctrl Pts',(5.14617563250833,3.91548594258288,5.1068147110629));
#127096=CARTESIAN_POINT('Ctrl Pts',(5.15564707101679,3.9177059001657,5.09730554412581));
#127097=CARTESIAN_POINT('',(5.13739562869265,3.91326598502339,5.46417113114432));
#127098=CARTESIAN_POINT('',(5.13704991397976,3.91326598377977,5.29024750217892));
#127099=CARTESIAN_POINT('',(4.71313142014474,3.82362522063888,5.83407166691751));
#127100=CARTESIAN_POINT('Origin',(-0.140930620901902,4.01780066783773,-0.125448627999198));
#127101=CARTESIAN_POINT('Ctrl Pts',(4.55558163274279,3.784676613028,5.6399624125463));
#127102=CARTESIAN_POINT('Ctrl Pts',(4.58189130678319,3.7914885732022,5.67219541290958));
#127103=CARTESIAN_POINT('Ctrl Pts',(4.60818735596335,3.79813536726801,5.70450848694832));
#127104=CARTESIAN_POINT('Ctrl Pts',(4.66069215544137,3.81110766403254,5.76920268671428));
#127105=CARTESIAN_POINT('Ctrl Pts',(4.68693207139744,3.81744086356028,5.80162222601506));
#127106=CARTESIAN_POINT('Ctrl Pts',(4.7131314190678,3.8236252206388,5.83407166778703));
#127107=CARTESIAN_POINT('Ctrl Pts',(4.256615929,3.913265985,6.175048246));
#127108=CARTESIAN_POINT('Ctrl Pts',(4.310207581,3.903042157,6.138106173));
#127109=CARTESIAN_POINT('Ctrl Pts',(4.363149987,3.892857143,6.100239519));
#127110=CARTESIAN_POINT('Ctrl Pts',(4.643995564,3.838828313,5.899366853));
#127111=CARTESIAN_POINT('Ctrl Pts',(4.905196519,3.783894965,5.673539205));
#127112=CARTESIAN_POINT('Ctrl Pts',(3.916752508,3.913265985,6.100946631));
#127113=CARTESIAN_POINT('Ctrl Pts',(3.969701051,3.903042157,6.06695414500001));
#127114=CARTESIAN_POINT('Ctrl Pts',(4.022051639,3.892857143,6.032047796));
#127115=CARTESIAN_POINT('Ctrl Pts',(4.299757775,3.838828313,5.846878769));
#127116=CARTESIAN_POINT('Ctrl Pts',(4.559275454,3.783894965,5.636976791));
#127117=CARTESIAN_POINT('',(4.25661593240909,3.91326598544479,6.17504824276322));
#127118=CARTESIAN_POINT('Ctrl Pts',(4.71313142169647,3.82362522012804,5.83407166577598));
#127119=CARTESIAN_POINT('Ctrl Pts',(4.59879424790011,3.8468929357323,5.92644045331317));
#127120=CARTESIAN_POINT('Ctrl Pts',(4.48201954411058,3.86998912007458,6.015218971059));
#127121=CARTESIAN_POINT('Ctrl Pts',(4.36314998703682,3.89285714299292,6.10023951897366));
#127122=CARTESIAN_POINT('Ctrl Pts',(4.32788952948444,3.89964051913601,6.1254592935724));
#127123=CARTESIAN_POINT('Ctrl Pts',(4.29237594126452,3.90644394833732,6.15039797052489));
#127124=CARTESIAN_POINT('Ctrl Pts',(4.25661593207867,3.91326598441268,6.17504824387779));
#127125=CARTESIAN_POINT('',(4.08668422522062,3.91326598631302,6.1379974340254));
#127126=CARTESIAN_POINT('Origin',(-6.90419943438769E-13,4.00453391999933,
-8.03176969377262E-13));
#127127=CARTESIAN_POINT('',(4.70753952324103,4.00345494176913,5.83858472873869));
#127128=CARTESIAN_POINT('Origin',(-0.0955451242393152,4.1605720476159,-0.158402113833271));
#127129=CARTESIAN_POINT('Origin',(-0.122576384829521,4.01785438464529,-0.148327773608642));
#127130=CARTESIAN_POINT('Ctrl Pts',(3.12174159235361,3.783915088,6.82000433694904));
#127131=CARTESIAN_POINT('Ctrl Pts',(3.49240685596093,3.848090541,6.65033858412427));
#127132=CARTESIAN_POINT('Ctrl Pts',(3.84250050621632,3.913265985,6.44149979260178));
#127133=CARTESIAN_POINT('Ctrl Pts',(3.85442513550379,3.91548594245362,6.43438648115518));
#127134=CARTESIAN_POINT('Ctrl Pts',(3.8663497647913,3.91770589990719,6.42727316970848));
#127135=CARTESIAN_POINT('Ctrl Pts',(3.232465128,3.783915088,6.489504542));
#127136=CARTESIAN_POINT('Ctrl Pts',(3.585167823,3.848090541,6.313820997));
#127137=CARTESIAN_POINT('Ctrl Pts',(3.916752508,3.913265985,6.100946631));
#127138=CARTESIAN_POINT('Ctrl Pts',(3.92804669869196,3.91548594245362,6.09369586281981));
#127139=CARTESIAN_POINT('Ctrl Pts',(3.93934088938394,3.91770589990718,6.08644509463963));
#127140=CARTESIAN_POINT('',(3.84265089985369,3.91326598502339,6.44081004656437));
#127141=CARTESIAN_POINT('',(3.87970170699552,3.91326598377977,6.27087833698131));
#127142=CARTESIAN_POINT('',(3.34878807226981,3.82362522063631,6.71085824953841));
#127143=CARTESIAN_POINT('Origin',(-0.110667850082253,4.01780063234556,-0.152811367961587));
#127144=CARTESIAN_POINT('Ctrl Pts',(3.23664946349505,3.78467661316556,6.48741861484588));
#127145=CARTESIAN_POINT('Ctrl Pts',(3.25541488977027,3.79148857336469,6.52455382809183));
#127146=CARTESIAN_POINT('Ctrl Pts',(3.2741497958025,3.79813536728641,6.56176431297438));
#127147=CARTESIAN_POINT('Ctrl Pts',(3.31151964099757,3.81110763603767,6.63623281746942));
#127148=CARTESIAN_POINT('Ctrl Pts',(3.33017674893767,3.81744080660581,6.67353502924518));
#127149=CARTESIAN_POINT('Ctrl Pts',(3.34878807103834,3.82362522063603,6.71085825013198));
#127150=CARTESIAN_POINT('Ctrl Pts',(2.829645774,3.913265985,6.945725649));
#127151=CARTESIAN_POINT('Ctrl Pts',(2.889925936,3.903042157,6.92116788300001));
#127152=CARTESIAN_POINT('Ctrl Pts',(2.94977079,3.892857143,6.895567583));
#127153=CARTESIAN_POINT('Ctrl Pts',(3.267232039,3.838828313,6.759764705));
#127154=CARTESIAN_POINT('Ctrl Pts',(3.57087253,3.783894965,6.59536726600001));
#127155=CARTESIAN_POINT('Ctrl Pts',(2.513657828,3.913265985,6.80029590000001));
#127156=CARTESIAN_POINT('Ctrl Pts',(2.572675843,3.903042157,6.77848051100001));
#127157=CARTESIAN_POINT('Ctrl Pts',(2.631306337,3.892857143,6.755644082));
#127158=CARTESIAN_POINT('Ctrl Pts',(2.942325725,3.838828313,6.634502815));
#127159=CARTESIAN_POINT('Ctrl Pts',(3.240898745,3.783894965,6.48529685700001));
#127160=CARTESIAN_POINT('',(2.82964577863558,3.91326598587967,6.9457256464307));
#127161=CARTESIAN_POINT('Ctrl Pts',(3.34878807403057,3.82362522012801,6.71085824878091));
#127162=CARTESIAN_POINT('Ctrl Pts',(3.21726748079077,3.84689293573226,6.77648839291499));
#127163=CARTESIAN_POINT('Ctrl Pts',(3.08413814752668,3.8699891200746,6.83808820886709));
#127164=CARTESIAN_POINT('Ctrl Pts',(2.94977078968296,3.89285714276324,6.89556758275439));
#127165=CARTESIAN_POINT('Ctrl Pts',(2.90991319577925,3.89964051914521,6.91261777693104));
#127166=CARTESIAN_POINT('Ctrl Pts',(2.86986881736904,3.90644394874724,6.92933902946402));
#127167=CARTESIAN_POINT('Ctrl Pts',(2.82964577787071,3.91326598565656,6.9457256476036));
#127168=CARTESIAN_POINT('',(2.67165180852597,3.91326598631311,6.87301077157454));
#127169=CARTESIAN_POINT('Origin',(7.4723213727701E-13,4.00453391999956,
1.41163122857613E-12));
#127170=CARTESIAN_POINT('',(3.34235673590872,4.00345494162035,6.71406370599629));
#127171=CARTESIAN_POINT('Origin',(-0.0592595316714378,4.16057203004573,
-0.175238072865184));
#127172=CARTESIAN_POINT('Origin',(-0.0878244445791232,4.01785425743471,
-0.171210135190435));
#127173=CARTESIAN_POINT('Ctrl Pts',(1.583020583,3.783915088,7.331033067));
#127174=CARTESIAN_POINT('Ctrl Pts',(1.98146011,3.848090541,7.244996356));
#127175=CARTESIAN_POINT('Ctrl Pts',(2.368228079,3.913265985,7.11628384500001));
#127176=CARTESIAN_POINT('Ctrl Pts',(2.37210492999178,3.91391928492389,7.11499366777252));
#127177=CARTESIAN_POINT('Ctrl Pts',(2.37598178098357,3.91457258484778,7.11370349054503));
#127178=CARTESIAN_POINT('Ctrl Pts',(1.761840242,3.783915088,7.032667983));
#127179=CARTESIAN_POINT('Ctrl Pts',(2.144063713,3.848090541,6.936912476));
#127180=CARTESIAN_POINT('Ctrl Pts',(2.513657828,3.913265985,6.8002959));
#127181=CARTESIAN_POINT('Ctrl Pts',(2.51736253321383,3.91391928492389,6.79892649469601));
#127182=CARTESIAN_POINT('Ctrl Pts',(2.52106723842766,3.91457258484778,6.79755708939203));
#127183=CARTESIAN_POINT('',(2.36822808400883,3.9132659845887,7.11628384347087));
#127184=CARTESIAN_POINT('',(2.44094296070756,3.91326598377977,6.95828986997161));
#127185=CARTESIAN_POINT('',(1.82785911574402,3.82362522063531,7.27385255908872));
#127186=CARTESIAN_POINT('Origin',(-0.0752306557181101,4.01780064760607,
-0.173029325392347));
#127187=CARTESIAN_POINT('Ctrl Pts',(1.76637516223459,3.78467661302819,7.03153033179064));
#127188=CARTESIAN_POINT('Ctrl Pts',(1.77671889009897,3.79148857321477,7.07183135625115));
#127189=CARTESIAN_POINT('Ctrl Pts',(1.78701663017569,3.79813536722453,7.1121993322267));
#127190=CARTESIAN_POINT('Ctrl Pts',(1.80750430603842,3.81110766402319,7.19296039122642));
#127191=CARTESIAN_POINT('Ctrl Pts',(1.81770639741428,3.8174408635424,7.23340142297894));
#127192=CARTESIAN_POINT('Ctrl Pts',(1.82785911431772,3.82362522063523,7.27385255944672));
#127193=CARTESIAN_POINT('Ctrl Pts',(1.270364528,3.913265985,7.391628641));
#127194=CARTESIAN_POINT('Ctrl Pts',(1.334514567,3.903042157,7.380603475));
#127195=CARTESIAN_POINT('Ctrl Pts',(1.398463589,3.892857143,7.36846657));
#127196=CARTESIAN_POINT('Ctrl Pts',(1.737696375,3.838828313,7.304083473));
#127197=CARTESIAN_POINT('Ctrl Pts',(2.06957851,3.783894965,7.208803284));
#127198=CARTESIAN_POINT('Ctrl Pts',(0.993027301999999,3.913265985,7.18167089));
#127199=CARTESIAN_POINT('Ctrl Pts',(1.055355172,3.903042157,7.173052662));
#127200=CARTESIAN_POINT('Ctrl Pts',(1.117524075,3.892857143,7.163353959));
#127201=CARTESIAN_POINT('Ctrl Pts',(1.447313794,3.838828313,7.111904882));
#127202=CARTESIAN_POINT('Ctrl Pts',(1.770981213,3.783894965,7.03037165));
#127203=CARTESIAN_POINT('',(1.27036453248304,3.9132659854451,7.39162863951458));
#127204=CARTESIAN_POINT('Ctrl Pts',(1.8278591176894,3.82362522012808,7.27385255883624));
#127205=CARTESIAN_POINT('Ctrl Pts',(1.6853048618196,3.84689293573234,7.30967526699593));
#127206=CARTESIAN_POINT('Ctrl Pts',(1.54204587881209,3.86998912007467,7.34121604212135));
#127207=CARTESIAN_POINT('Ctrl Pts',(1.3984635889666,3.89285714300268,7.36846656999108));
#127208=CARTESIAN_POINT('Ctrl Pts',(1.35587255566562,3.89964051914869,7.37654993559321));
#127209=CARTESIAN_POINT('Ctrl Pts',(1.31316981756267,3.90644394833732,7.38427189684407));
#127210=CARTESIAN_POINT('Ctrl Pts',(1.27036453168524,3.91326598441267,7.39162864036663));
#127211=CARTESIAN_POINT('',(1.13169592297835,3.91326598631302,7.28664976426088));
#127212=CARTESIAN_POINT('Origin',(-2.03938428644523E-13,4.00453392000067,
-6.67868538251071E-13));
#127213=CARTESIAN_POINT('',(1.82088906321882,4.00345494158282,7.27560052616864));
#127214=CARTESIAN_POINT('Origin',(-0.0202030731523872,4.16057201776935,
-0.18388014126873));
#127215=CARTESIAN_POINT('Origin',(-0.0489661124333862,4.01785421495085,
-0.186087345027113));
#127216=CARTESIAN_POINT('Ctrl Pts',(-0.029944964,3.783915088,7.49994022));
#127217=CARTESIAN_POINT('Ctrl Pts',(0.377674617,3.848090541,7.50156772));
#127218=CARTESIAN_POINT('Ctrl Pts',(0.783069551000001,3.913265985,7.459008116));
#127219=CARTESIAN_POINT('Ctrl Pts',(0.787133113336888,3.91391928492389,
7.45858151075809));
#127220=CARTESIAN_POINT('Ctrl Pts',(0.791196675673776,3.91457258484778,
7.45815490551618));
#127221=CARTESIAN_POINT('Ctrl Pts',(0.208833664,3.783915088,7.246991686));
#127222=CARTESIAN_POINT('Ctrl Pts',(0.602705566,3.848090541,7.235641637));
#127223=CARTESIAN_POINT('Ctrl Pts',(0.993027302,3.913265985,7.18167089));
#127224=CARTESIAN_POINT('Ctrl Pts',(0.996939774931096,3.91391928492389,
7.18112990273941));
#127225=CARTESIAN_POINT('Ctrl Pts',(1.00085224786219,3.91457258484778,7.18058891547881));
#127226=CARTESIAN_POINT('',(0.783069554340072,3.91326598458875,7.45900811632261));
#127227=CARTESIAN_POINT('',(0.888048434082487,3.91326598377978,7.32033950208015));
#127228=CARTESIAN_POINT('',(0.22146149895969,3.82362522067689,7.49672960729196));
#127229=CARTESIAN_POINT('Origin',(-0.0362756098282808,4.01780061753748,
-0.185156279461053));
#127230=CARTESIAN_POINT('Ctrl Pts',(0.213507121533661,3.78467661307173,
7.2468555066897));
#127231=CARTESIAN_POINT('Ctrl Pts',(0.214945489938668,3.79148857326155,
7.28843791132082));
#127232=CARTESIAN_POINT('Ctrl Pts',(0.216324553099686,3.79813536727868,
7.33007581620001));
#127233=CARTESIAN_POINT('Ctrl Pts',(0.218971991994922,3.811107633564,7.41335277529608));
#127234=CARTESIAN_POINT('Ctrl Pts',(0.220241931798139,3.8174408015945,7.45504124418656));
#127235=CARTESIAN_POINT('Ctrl Pts',(0.22146149747299,3.82362522066709,7.49672960733691));
#127236=CARTESIAN_POINT('Ctrl Pts',(-0.348317552,3.913265985,7.491907293));
#127237=CARTESIAN_POINT('Ctrl Pts',(-0.28329722,3.903042157,7.49493025100001));
#127238=CARTESIAN_POINT('Ctrl Pts',(-0.218234215,3.892857143,7.496824249));
#127239=CARTESIAN_POINT('Ctrl Pts',(0.12690796,3.838828313,7.506871415));
#127240=CARTESIAN_POINT('Ctrl Pts',(0.4715133,3.783894965,7.485163673));
#127241=CARTESIAN_POINT('Ctrl Pts',(-0.574036077000001,3.913265985,7.227238932));
#127242=CARTESIAN_POINT('Ctrl Pts',(-0.511312734,3.903042157,7.232220843));
#127243=CARTESIAN_POINT('Ctrl Pts',(-0.448512371,3.892857143,7.236113367));
#127244=CARTESIAN_POINT('Ctrl Pts',(-0.115372922,3.838828313,7.256762181));
#127245=CARTESIAN_POINT('Ctrl Pts',(0.218254568,3.783894965,7.246714079));
#127246=CARTESIAN_POINT('',(-0.348317546752673,3.91326598587967,7.49190729243567));
#127247=CARTESIAN_POINT('Ctrl Pts',(0.221461498925141,3.82362522046317,
7.49672960726836));
#127248=CARTESIAN_POINT('Ctrl Pts',(0.0745392594698745,3.8468929359541,
7.50106984909109));
#127249=CARTESIAN_POINT('Ctrl Pts',(-0.0721507419137992,3.86998912018444,
7.50107677173588));
#127250=CARTESIAN_POINT('Ctrl Pts',(-0.218234214930474,3.89285714276327,
7.49682424946948));
#127251=CARTESIAN_POINT('Ctrl Pts',(-0.261567177774771,3.89964051909098,
7.49556281732005));
#127252=CARTESIAN_POINT('Ctrl Pts',(-0.304931542627311,3.90644394863843,
7.49392441705024));
#127253=CARTESIAN_POINT('Ctrl Pts',(-0.348317546838671,3.91326598549287,
7.49190729297715));
#127254=CARTESIAN_POINT('',(-0.461176806441806,3.91326598631302,7.35957311300495));
#127255=CARTESIAN_POINT('Origin',(1.13136496698862E-13,4.00453391999956,
7.10369263412503E-13));
#127256=CARTESIAN_POINT('',(0.214278640529085,4.00345494161128,7.49693835249986));
#127257=CARTESIAN_POINT('Origin',(0.0197980510491458,4.16057202135974,-0.183924310788655));
#127258=CARTESIAN_POINT('Origin',(-0.0078180414431836,4.01785424473155,
-0.192262944664429));
#127259=CARTESIAN_POINT('Ctrl Pts',(0.431320676484365,1.97885290483257,
7.48816481493075));
#127260=CARTESIAN_POINT('Ctrl Pts',(0.44542542366215,1.97658649491626,7.48729904127472));
#127261=CARTESIAN_POINT('Ctrl Pts',(0.459530170839939,1.974320085,7.4864332676187));
#127262=CARTESIAN_POINT('Ctrl Pts',(0.868621014284314,1.908585653,7.46132256760333));
#127263=CARTESIAN_POINT('Ctrl Pts',(1.27253989903237,1.843501847,7.39178552536167));
#127264=CARTESIAN_POINT('Ctrl Pts',(0.17884133945574,1.97885290483257,7.24784534091357));
#127265=CARTESIAN_POINT('Ctrl Pts',(0.192495113727867,1.97658649491626,
7.24745694795684));
#127266=CARTESIAN_POINT('Ctrl Pts',(0.206148888,1.974320085,7.247068555));
#127267=CARTESIAN_POINT('Ctrl Pts',(0.602159817,1.908585653,7.23580369500001));
#127268=CARTESIAN_POINT('Ctrl Pts',(0.994585354,1.843501847,7.181455282));
#127269=CARTESIAN_POINT('',(0.989922562761728,1.84427517322922,7.1820995058139));
#127270=CARTESIAN_POINT('Origin',(0.00165684739715746,2.01783539001702,
-0.19726511916484));
#127271=CARTESIAN_POINT('Ctrl Pts',(1.02305817352955,1.88359401258998,7.42989582473918));
#127272=CARTESIAN_POINT('Ctrl Pts',(1.01748970331488,1.8773452349313,7.38856271124362));
#127273=CARTESIAN_POINT('Ctrl Pts',(1.01194012110602,1.87094900374799,7.34722645205979));
#127274=CARTESIAN_POINT('Ctrl Pts',(1.00089520291886,1.85785292454026,7.26464059629853));
#127275=CARTESIAN_POINT('Ctrl Pts',(0.995393852709155,1.8511459533259,7.22334605434188));
#127276=CARTESIAN_POINT('Ctrl Pts',(0.989922562684033,1.84427517325669,
7.18209950581963));
#127277=CARTESIAN_POINT('Ctrl Pts',(0.775003908,1.843494248,7.459850464));
#127278=CARTESIAN_POINT('Ctrl Pts',(1.181144933,1.909007671,7.41765647000001));
#127279=CARTESIAN_POINT('Ctrl Pts',(1.580304579,1.974320085,7.331619019));
#127280=CARTESIAN_POINT('Ctrl Pts',(0.985261412,1.843494248,7.182740421));
#127281=CARTESIAN_POINT('Ctrl Pts',(1.376315572,1.909007671,7.129099254));
#127282=CARTESIAN_POINT('Ctrl Pts',(1.759234759,1.974320085,7.033320202));
#127283=CARTESIAN_POINT('Origin',(-0.0322702647863354,1.87500004439775,
-0.196842784057325));
#127284=CARTESIAN_POINT('Ctrl Pts',(2.0309707252744,1.97885290481358,7.22037448773906));
#127285=CARTESIAN_POINT('Ctrl Pts',(2.04455959549943,1.97658649490676,7.21649685167196));
#127286=CARTESIAN_POINT('Ctrl Pts',(2.05814846572453,1.974320085,7.21261921560488));
#127287=CARTESIAN_POINT('Ctrl Pts',(2.45227693432097,1.908585653,7.10015315039258));
#127288=CARTESIAN_POINT('Ctrl Pts',(2.83180401172431,1.843501847,6.94541122513066));
#127289=CARTESIAN_POINT('Ctrl Pts',(1.73273263193011,1.97885290481358,7.03994914282426));
#127290=CARTESIAN_POINT('Ctrl Pts',(1.74598369546509,1.97658649490676,7.03663467241213));
#127291=CARTESIAN_POINT('Ctrl Pts',(1.759234759,1.974320085,7.033320202));
#127292=CARTESIAN_POINT('Ctrl Pts',(2.14356556,1.908585653,6.937188064));
#127293=CARTESIAN_POINT('Ctrl Pts',(2.515133105,1.843501847,6.79975039700001));
#127294=CARTESIAN_POINT('',(2.51071781581557,1.84427517322324,6.80138192165602));
#127295=CARTESIAN_POINT('Origin',(-0.0407880620217305,2.01783544827035,
-0.193009651875682));
#127296=CARTESIAN_POINT('Ctrl Pts',(2.59634761838852,1.88359401254937,7.03626172327405));
#127297=CARTESIAN_POINT('Ctrl Pts',(2.58202393835256,1.8773452349134,6.997092011555));
#127298=CARTESIAN_POINT('Ctrl Pts',(2.56771802844592,1.87094900373487,6.95791516722647));
#127299=CARTESIAN_POINT('Ctrl Pts',(2.53917783475688,1.85785293292152,6.87963450385735));
#127300=CARTESIAN_POINT('Ctrl Pts',(2.52492798746053,1.85114595747494,6.84048800649519));
#127301=CARTESIAN_POINT('Ctrl Pts',(2.51071781591354,1.84427517330664,6.80138192161454));
#127302=CARTESIAN_POINT('Ctrl Pts',(2.360532086,1.843494248,7.118840374));
#127303=CARTESIAN_POINT('Ctrl Pts',(2.748107298,1.909007671,6.99032453800001));
#127304=CARTESIAN_POINT('Ctrl Pts',(3.119439304,1.974320085,6.82049107000001));
#127305=CARTESIAN_POINT('Ctrl Pts',(2.506303418,1.843494248,6.803009862));
#127306=CARTESIAN_POINT('Ctrl Pts',(2.876683684,1.909007671,6.666557711));
#127307=CARTESIAN_POINT('Ctrl Pts',(3.230060768,1.974320085,6.490701613));
#127308=CARTESIAN_POINT('Origin',(-0.0738311105701356,1.87500004546059,
-0.185303373844017));
#127309=CARTESIAN_POINT('Ctrl Pts',(3.53565484055987,1.9788529047602,6.61496747322476));
#127310=CARTESIAN_POINT('Ctrl Pts',(3.54809243330167,1.97658649488008,6.60825928880557));
#127311=CARTESIAN_POINT('Ctrl Pts',(3.56053002604348,1.974320085,6.60155110438651));
#127312=CARTESIAN_POINT('Ctrl Pts',(3.92126711138468,1.908585653,6.40698846308583));
#127313=CARTESIAN_POINT('Ctrl Pts',(4.25865611684382,1.843501847,6.17427721524676));
#127314=CARTESIAN_POINT('Ctrl Pts',(3.20560327250901,1.97885290476021,6.50287274661561));
#127315=CARTESIAN_POINT('Ctrl Pts',(3.21783202025451,1.97658649488008,6.4967871798078));
#127316=CARTESIAN_POINT('Ctrl Pts',(3.230060768,1.974320085,6.490701613));
#127317=CARTESIAN_POINT('Ctrl Pts',(3.584740561,1.908585653,6.31419723));
#127318=CARTESIAN_POINT('Ctrl Pts',(3.918076027,1.843501847,6.100096741));
#127319=CARTESIAN_POINT('',(3.91411469490178,1.84427517306064,6.10263927730789));
#127320=CARTESIAN_POINT('Origin',(-0.0813257725786604,2.01783541886837,
-0.179728872211489));
#127321=CARTESIAN_POINT('Ctrl Pts',(4.04823473411854,1.88359401261533,6.3136198438659));
#127322=CARTESIAN_POINT('Ctrl Pts',(4.02582560354359,1.87734523497682,6.27844506607643));
#127323=CARTESIAN_POINT('Ctrl Pts',(4.00343229437791,1.87094900381564,6.24325950250469));
#127324=CARTESIAN_POINT('Ctrl Pts',(3.95873129615144,1.85785292434757,6.17294424923507));
#127325=CARTESIAN_POINT('Ctrl Pts',(3.93639927824253,1.85114595331107,6.13777629603404));
#127326=CARTESIAN_POINT('Ctrl Pts',(3.91411469398354,1.84427517339915,6.10263927840607));
#127327=CARTESIAN_POINT('Ctrl Pts',(3.835684406,1.843494248,6.44496122100001));
#127328=CARTESIAN_POINT('Ctrl Pts',(4.18657122,1.909007671,6.236132799));
#127329=CARTESIAN_POINT('Ctrl Pts',(4.512712514,1.974320085,5.990444538));
#127330=CARTESIAN_POINT('Ctrl Pts',(3.910153461,1.843494248,6.105178123));
#127331=CARTESIAN_POINT('Ctrl Pts',(4.242541264,1.909007671,5.89229533900001));
#127332=CARTESIAN_POINT('Ctrl Pts',(4.549852726,1.974320085,5.644585031));
#127333=CARTESIAN_POINT('Origin',(-0.111939653748659,1.87500003546859,-0.16509948825185));
#127334=CARTESIAN_POINT('Ctrl Pts',(4.87501566615518,1.9788529047133,5.70025193191983));
#127335=CARTESIAN_POINT('Ctrl Pts',(4.88572041336524,1.97658649485662,5.69102686641532));
#127336=CARTESIAN_POINT('Ctrl Pts',(4.89642516057517,1.974320085,5.68180180091079));
#127337=CARTESIAN_POINT('Ctrl Pts',(5.20690319502679,1.908585653,5.41424011548591));
#127338=CARTESIAN_POINT('Ctrl Pts',(5.48637819364505,1.843501847,5.11444086518299));
#127339=CARTESIAN_POINT('Ctrl Pts',(4.52858346737681,1.9788529047133,5.66172924861175));
#127340=CARTESIAN_POINT('Ctrl Pts',(4.5392180966884,1.97658649485662,5.65315713980588));
#127341=CARTESIAN_POINT('Ctrl Pts',(4.549852726,1.974320085,5.644585031));
#127342=CARTESIAN_POINT('Ctrl Pts',(4.858297077,1.908585653,5.395961552));
#127343=CARTESIAN_POINT('Ctrl Pts',(5.137814068,1.843501847,5.115209341));
#127344=CARTESIAN_POINT('',(5.13449191936986,1.84427517322394,5.11854400394933));
#127345=CARTESIAN_POINT('Origin',(-0.118060676876202,2.01783543967816,-0.158044115063364));
#127346=CARTESIAN_POINT('Ctrl Pts',(5.31083089269158,1.88359401260886,5.29576011741492));
#127347=CARTESIAN_POINT('Ctrl Pts',(5.28138452430791,1.87734531701701,5.26622539498652));
#127348=CARTESIAN_POINT('Ctrl Pts',(5.25195069654588,1.87094904413585,5.23667614406208));
#127349=CARTESIAN_POINT('Ctrl Pts',(5.19317884859687,1.85785291265372,5.17761398118619));
#127350=CARTESIAN_POINT('Ctrl Pts',(5.16380889825467,1.85114594749935,5.14806898668561));
#127351=CARTESIAN_POINT('Ctrl Pts',(5.13449191955354,1.84427517329317,5.11854400434702));
#127352=CARTESIAN_POINT('Ctrl Pts',(5.131484387,1.843494248,5.469722844));
#127353=CARTESIAN_POINT('Ctrl Pts',(5.429275724,1.909007671,5.19034642200001));
#127354=CARTESIAN_POINT('Ctrl Pts',(5.694976303,1.974320085,4.880291478));
#127355=CARTESIAN_POINT('Ctrl Pts',(5.131169075,1.843494248,5.12187504));
#127356=CARTESIAN_POINT('Ctrl Pts',(5.410022329,1.909007671,4.842515785));
#127357=CARTESIAN_POINT('Ctrl Pts',(5.656898626,1.974320085,4.534533927));
#127358=CARTESIAN_POINT('Origin',(-0.144814243662199,1.87500002627446,-0.137175988992163));
#127359=CARTESIAN_POINT('Ctrl Pts',(5.98642617657734,1.97885290449943,4.51899894419897));
#127360=CARTESIAN_POINT('Ctrl Pts',(5.99489753597836,1.97658649474969,4.50768835193765));
#127361=CARTESIAN_POINT('Ctrl Pts',(6.00336889537952,1.974320085,4.49637775967633));
#127362=CARTESIAN_POINT('Ctrl Pts',(6.24907027333074,1.908585653,4.16832791874103));
#127363=CARTESIAN_POINT('Ctrl Pts',(6.45756332514675,1.843501847,3.81545894504712));
#127364=CARTESIAN_POINT('Ctrl Pts',(5.63981213161998,1.97885290449943,4.55584958327403));
#127365=CARTESIAN_POINT('Ctrl Pts',(5.64835537881002,1.97658649474969,4.54519175513701));
#127366=CARTESIAN_POINT('Ctrl Pts',(5.656898626,1.974320085,4.534533927));
#127367=CARTESIAN_POINT('Ctrl Pts',(5.904685021,1.908585653,4.225416708));
#127368=CARTESIAN_POINT('Ctrl Pts',(6.117313634,1.843501847,3.891140437));
#127369=CARTESIAN_POINT('',(6.11478600923873,1.84427517321823,3.89511130174437));
#127370=CARTESIAN_POINT('Origin',(-0.149275386552622,2.01783542593181,-0.128969635675294));
#127371=CARTESIAN_POINT('Ctrl Pts',(6.32509850137208,1.88359401257019,4.03027653421333));
#127372=CARTESIAN_POINT('Ctrl Pts',(6.28999101930453,1.87734523490686,4.00776212019143));
#127373=CARTESIAN_POINT('Ctrl Pts',(6.25489336773249,1.87094900375861,3.98523127410483));
#127374=CARTESIAN_POINT('Ctrl Pts',(6.18479924655972,1.85785292702313,3.94018434990008));
#127375=CARTESIAN_POINT('Ctrl Pts',(6.14976460795124,1.85114595460251,3.9176437458544));
#127376=CARTESIAN_POINT('Ctrl Pts',(6.11478600941527,1.8442751733602,3.89511130181847));
#127377=CARTESIAN_POINT('Ctrl Pts',(6.187341861,1.843494248,4.238726305));
#127378=CARTESIAN_POINT('Ctrl Pts',(6.41811333,1.909007671,3.901865214));
#127379=CARTESIAN_POINT('Ctrl Pts',(6.610949329,1.974320085,3.541941413));
#127380=CARTESIAN_POINT('Ctrl Pts',(6.112256925,1.843494248,3.899078773));
#127381=CARTESIAN_POINT('Ctrl Pts',(6.324536764,1.909007671,3.566305575));
#127382=CARTESIAN_POINT('Ctrl Pts',(6.49943423400001,1.974320085,3.212453056));
#127383=CARTESIAN_POINT('Origin',(-0.170917169116834,1.87500007773979,-0.102838001282375));
#127384=CARTESIAN_POINT('Ctrl Pts',(6.81791805171561,1.97885290458604,3.12644259057752));
#127385=CARTESIAN_POINT('Ctrl Pts',(6.8237599125367,1.976586494793,3.11357534157059));
#127386=CARTESIAN_POINT('Ctrl Pts',(6.82960177335764,1.974320085,3.10070809256374));
#127387=CARTESIAN_POINT('Ctrl Pts',(6.99903777035848,1.908585653,2.72750934118146));
#127388=CARTESIAN_POINT('Ctrl Pts',(7.12679997215744,1.843501847,2.33807040446541));
#127389=CARTESIAN_POINT('Ctrl Pts',(6.48732944815439,1.97885290458604,3.23694345578894));
#127390=CARTESIAN_POINT('Ctrl Pts',(6.49338184107711,1.976586494793,3.2246982558945));
#127391=CARTESIAN_POINT('Ctrl Pts',(6.499434234,1.974320085,3.212453056));
#127392=CARTESIAN_POINT('Ctrl Pts',(6.674976456,1.908585653,2.857296075));
#127393=CARTESIAN_POINT('Ctrl Pts',(6.810774414,1.843501847,2.485126131));
#127394=CARTESIAN_POINT('',(6.80915950174646,1.84427517325685,2.48954752345402));
#127395=CARTESIAN_POINT('Origin',(-0.173510263844014,2.01783543082771,-0.0938646918006689));
#127396=CARTESIAN_POINT('Ctrl Pts',(7.04361153430039,1.88359401255035,2.57634169922522));
#127397=CARTESIAN_POINT('Ctrl Pts',(7.00448491229141,1.87734523491764,2.5619007306039));
#127398=CARTESIAN_POINT('Ctrl Pts',(6.96536435829275,1.87094900376008,2.54744160075242));
#127399=CARTESIAN_POINT('Ctrl Pts',(6.88722512871215,1.85785290811974,2.51851597096455));
#127400=CARTESIAN_POINT('Ctrl Pts',(6.84816407707341,1.85114594533474,2.50403378766267));
#127401=CARTESIAN_POINT('Ctrl Pts',(6.80915950224257,1.84427517341445,2.48954752411438));
#127402=CARTESIAN_POINT('Ctrl Pts',(6.953886107,1.843494248,2.809531636));
#127403=CARTESIAN_POINT('Ctrl Pts',(7.10684709,1.909007671,2.430937126));
#127404=CARTESIAN_POINT('Ctrl Pts',(7.217801712,1.974320085,2.037974103));
#127405=CARTESIAN_POINT('Ctrl Pts',(6.807542435,1.843494248,2.493965916));
#127406=CARTESIAN_POINT('Ctrl Pts',(6.943322888,1.909007671,2.12333888));
#127407=CARTESIAN_POINT('Ctrl Pts',(7.038063521,1.974320085,1.74016145));
#127408=CARTESIAN_POINT('Origin',(-0.189028489599921,1.87500006543182,-0.0636916109352054));
#127409=CARTESIAN_POINT('Ctrl Pts',(7.33061165607248,1.97885290465309,1.58769725582771));
#127410=CARTESIAN_POINT('Ctrl Pts',(7.33355085931847,1.97658649482652,1.57387500833381));
#127411=CARTESIAN_POINT('Ctrl Pts',(7.33649006256462,1.974320085,1.56005276083997));
#127412=CARTESIAN_POINT('Ctrl Pts',(7.42173804095537,1.908585653,1.15915545738787));
#127413=CARTESIAN_POINT('Ctrl Pts',(7.4627953726707,1.843501847,0.751356289701777));
#127414=CARTESIAN_POINT('Ctrl Pts',(7.03150645023676,1.97885290465309,1.76668144932446));
#127415=CARTESIAN_POINT('Ctrl Pts',(7.03478498561844,1.97658649482652,1.75342144966226));
#127416=CARTESIAN_POINT('Ctrl Pts',(7.038063521,1.974320085,1.74016145));
#127417=CARTESIAN_POINT('Ctrl Pts',(7.133153411,1.908585653,1.355571454));
#127418=CARTESIAN_POINT('Ctrl Pts',(7.185770951,1.843501847,0.962910089));
#127419=CARTESIAN_POINT('',(7.18514426358531,1.84427517325349,0.967575271040671));
#127420=CARTESIAN_POINT('Origin',(-0.18963165884277,2.0178354651733,-0.0543705811767188));
#127421=CARTESIAN_POINT('Ctrl Pts',(7.43277311966718,1.88359401261756,1.00193998978874));
#127422=CARTESIAN_POINT('Ctrl Pts',(7.39145687490835,1.87734523496621,0.996247710126135));
#127423=CARTESIAN_POINT('Ctrl Pts',(7.35014265232055,1.87094900381072,0.990536389400879));
#127424=CARTESIAN_POINT('Ctrl Pts',(7.26761217221817,1.8578529165569,0.979084656609812));
#127425=CARTESIAN_POINT('Ctrl Pts',(7.2263510766818,1.85114594946581,0.973338026201722));
#127426=CARTESIAN_POINT('Ctrl Pts',(7.18514426386498,1.84427517338048,0.967575270475462));
#127427=CARTESIAN_POINT('Ctrl Pts',(7.395274366,1.843494248,1.24896639));
#127428=CARTESIAN_POINT('Ctrl Pts',(7.463272578,1.909007671,0.84634112));
#127429=CARTESIAN_POINT('Ctrl Pts',(7.487157709,1.974320085,0.43871339));
#127430=CARTESIAN_POINT('Ctrl Pts',(7.184514827,1.843494248,0.972237985));
#127431=CARTESIAN_POINT('Ctrl Pts',(7.23744695100001,1.909007671,0.58108722));
#127432=CARTESIAN_POINT('Ctrl Pts',(7.24760078,1.974320085,0.186501829));
#127433=CARTESIAN_POINT('Origin',(-0.198300997752738,1.8750000238648,-0.0215670094842346));
#127434=CARTESIAN_POINT('Ctrl Pts',(7.50053400668084,1.97885290461155,-0.025287038347163));
#127435=CARTESIAN_POINT('Ctrl Pts',(7.50043311836844,1.97658649480575,-0.0394179710704729));
#127436=CARTESIAN_POINT('Ctrl Pts',(7.50033223005592,1.974320085,-0.0535489037937829));
#127437=CARTESIAN_POINT('Ctrl Pts',(7.49740608849883,1.908585653,-0.463399246762781));
#127438=CARTESIAN_POINT('Ctrl Pts',(7.44983875707374,1.843501847,-0.870490409364686));
#127439=CARTESIAN_POINT('Ctrl Pts',(7.24689802587571,1.97885290461155,0.213811381676077));
#127440=CARTESIAN_POINT('Ctrl Pts',(7.24724940293787,1.97658649480575,0.200156605338041));
#127441=CARTESIAN_POINT('Ctrl Pts',(7.24760078,1.974320085,0.186501829));
#127442=CARTESIAN_POINT('Ctrl Pts',(7.25779204,1.908585653,-0.209538183));
#127443=CARTESIAN_POINT('Ctrl Pts',(7.224768825,1.843501847,-0.604330558));
#127444=CARTESIAN_POINT('',(7.22515966553458,1.84427517322513,-0.59963972759421));
#127445=CARTESIAN_POINT('Origin',(-0.196886367451559,2.01783541028853,-0.0123342117785667));
#127446=CARTESIAN_POINT('Ctrl Pts',(7.4743864954929,1.88359401260467,-0.61931132006069));
#127447=CARTESIAN_POINT('Ctrl Pts',(7.43281252968542,1.87734523494865,-0.615988746101347));
#127448=CARTESIAN_POINT('Ctrl Pts',(7.39123644540397,1.87094900377294,-0.61268520272327));
#127449=CARTESIAN_POINT('Ctrl Pts',(7.30817373059725,1.85785292164987,-0.606127589323485));
#127450=CARTESIAN_POINT('Ctrl Pts',(7.26664192341387,1.85114595192226,-0.60286994943654));
#127451=CARTESIAN_POINT('Ctrl Pts',(7.22515966555154,1.84427517329407,-0.599639727229753));
#127452=CARTESIAN_POINT('Ctrl Pts',(7.490867816,1.843494248,-0.369999136));
#127453=CARTESIAN_POINT('Ctrl Pts',(7.470723736,1.909007671,-0.777828857000001));
#127454=CARTESIAN_POINT('Ctrl Pts',(7.406422533,1.974320085,-1.181061074));
#127455=CARTESIAN_POINT('Ctrl Pts',(7.225547291,1.843494248,-0.594950714));
#127456=CARTESIAN_POINT('Ctrl Pts',(7.193156039,1.909007671,-0.988335434000001));
#127457=CARTESIAN_POINT('Ctrl Pts',(7.118248282,1.974320085,-1.375878411));
#127458=CARTESIAN_POINT('Origin',(-0.198301150915829,1.87500003685011,0.0215660772445789));
#127459=CARTESIAN_POINT('Ctrl Pts',(7.31973972432723,1.9788529048441,-1.63708893764741));
#127460=CARTESIAN_POINT('Ctrl Pts',(7.31660346173343,1.97658649492202,-1.65086780969589));
#127461=CARTESIAN_POINT('Ctrl Pts',(7.3134671991396,1.974320085,-1.66464668174432));
#127462=CARTESIAN_POINT('Ctrl Pts',(7.22250376035314,1.908585653,-2.06428591686262));
#127463=CARTESIAN_POINT('Ctrl Pts',(7.08853595973428,1.843501847,-2.45163394439753));
#127464=CARTESIAN_POINT('Ctrl Pts',(7.12343270472288,1.9788529048441,-1.34905626783604));
#127465=CARTESIAN_POINT('Ctrl Pts',(7.12084049336147,1.97658649492202,-1.36246733941802));
#127466=CARTESIAN_POINT('Ctrl Pts',(7.118248282,1.974320085,-1.375878411));
#127467=CARTESIAN_POINT('Ctrl Pts',(7.04306438000001,1.908585653,-1.764850046));
#127468=CARTESIAN_POINT('Ctrl Pts',(6.925944539,1.843501847,-2.14331338));
#127469=CARTESIAN_POINT('',(6.92733463110791,1.84427517321638,-2.138816237699));
#127470=CARTESIAN_POINT('Origin',(-0.194934900054559,2.01783545594361,0.0302789327713401));
#127471=CARTESIAN_POINT('Ctrl Pts',(7.16650586548861,1.88359401258645,-2.21160432106037));
#127472=CARTESIAN_POINT('Ctrl Pts',(7.12661813124974,1.87734523495188,-2.19942225327674));
#127473=CARTESIAN_POINT('Ctrl Pts',(7.08672423681744,1.87094900375853,-2.1872583156522));
#127474=CARTESIAN_POINT('Ctrl Pts',(7.00701309419383,1.85785290831506,-2.16299796235914));
#127475=CARTESIAN_POINT('Ctrl Pts',(6.96715261721269,1.85114594538467,-2.15088838650028));
#127476=CARTESIAN_POINT('Ctrl Pts',(6.92733463187897,1.84427517331601,-2.13881623722281));
#127477=CARTESIAN_POINT('Ctrl Pts',(7.236196612,1.843494248,-1.971663914));
#127478=CARTESIAN_POINT('Ctrl Pts',(7.128852155,1.909007671,-2.365628421));
#127479=CARTESIAN_POINT('Ctrl Pts',(6.979371271,1.974320085,-2.745610435));
#127480=CARTESIAN_POINT('Ctrl Pts',(6.928721193,1.843494248,-2.134320179));
#127481=CARTESIAN_POINT('Ctrl Pts',(6.812521145,1.909007671,-2.511544621));
#127482=CARTESIAN_POINT('Ctrl Pts',(6.656054405,1.974320085,-2.873924105));
#127483=CARTESIAN_POINT('Origin',(-0.189028709532146,1.87500002431909,0.0636906784464586));
#127484=CARTESIAN_POINT('Ctrl Pts',(6.79668254745504,1.97885290457719,-3.17234238059632));
#127485=CARTESIAN_POINT('Ctrl Pts',(6.79065755907535,1.97658649478857,-3.18512490576253));
#127486=CARTESIAN_POINT('Ctrl Pts',(6.78463257069555,1.974320085,-3.19790743092867));
#127487=CARTESIAN_POINT('Ctrl Pts',(6.60988518346303,1.908585653,-3.56864887210941));
#127488=CARTESIAN_POINT('Ctrl Pts',(6.39578110021144,1.843501847,-3.91814180098456));
#127489=CARTESIAN_POINT('Ctrl Pts',(6.66688358603411,1.97885290457719,-2.84884354773725));
#127490=CARTESIAN_POINT('Ctrl Pts',(6.6614689955171,1.97658649478857,-2.86138382636864));
#127491=CARTESIAN_POINT('Ctrl Pts',(6.656054405,1.974320085,-2.873924105));
#127492=CARTESIAN_POINT('Ctrl Pts',(6.49901085800001,1.908585653,-3.237639483));
#127493=CARTESIAN_POINT('Ctrl Pts',(6.303270783,1.843501847,-3.582077251));
#127494=CARTESIAN_POINT('',(6.30559512912612,1.8442751732378,-3.57798407743432));
#127495=CARTESIAN_POINT('Origin',(-0.183868084562621,2.01783547332994,0.0714761343217757));
#127496=CARTESIAN_POINT('Ctrl Pts',(6.52352738649043,1.8835940126154,-3.7004851615402));
#127497=CARTESIAN_POINT('Ctrl Pts',(6.48719098969058,1.87734523496561,-3.68001321990517));
#127498=CARTESIAN_POINT('Ctrl Pts',(6.45084467936221,1.87094900377755,-3.65955766037718));
#127499=CARTESIAN_POINT('Ctrl Pts',(6.37821249536725,1.8578529259649,-3.61872901632466));
#127500=CARTESIAN_POINT('Ctrl Pts',(6.34188708286931,1.85114595406991,-3.59833370212756));
#127501=CARTESIAN_POINT('Ctrl Pts',(6.30559512917684,1.84427517334982,-3.57798407768235));
#127502=CARTESIAN_POINT('Ctrl Pts',(6.64316889699999,1.843494248,-3.481135878));
#127503=CARTESIAN_POINT('Ctrl Pts',(6.45364337,1.909007671,-3.842813829));
#127504=CARTESIAN_POINT('Ctrl Pts',(6.225972366,1.974320085,-4.181778103));
#127505=CARTESIAN_POINT('Ctrl Pts',(6.307915794,1.843494248,-3.573891204));
#127506=CARTESIAN_POINT('Ctrl Pts',(6.113340333,1.909007671,-3.917316773));
#127507=CARTESIAN_POINT('Ctrl Pts',(5.882630822,1.974320085,-4.237588302));
#127508=CARTESIAN_POINT('Origin',(-0.170917924837104,1.87500005981962,0.102837358194177));
#127509=CARTESIAN_POINT('Ctrl Pts',(5.95582004877323,1.97885290483854,-4.55926061605723));
#127510=CARTESIAN_POINT('Ctrl Pts',(5.94718805576368,1.97658649491924,-4.57044909915949));
#127511=CARTESIAN_POINT('Ctrl Pts',(5.93855606275414,1.974320085,-4.58163758226185));
#127512=CARTESIAN_POINT('Ctrl Pts',(5.68819572295363,1.908585653,-4.90614577269425));
#127513=CARTESIAN_POINT('Ctrl Pts',(5.40396662443388,1.843501847,-5.20144170167195));
#127514=CARTESIAN_POINT('Ctrl Pts',(5.8985984021513,1.97885290483854,-4.21542206677501));
#127515=CARTESIAN_POINT('Ctrl Pts',(5.89061461207569,1.97658649491924,-4.2265051843875));
#127516=CARTESIAN_POINT('Ctrl Pts',(5.882630822,1.974320085,-4.237588302));
#127517=CARTESIAN_POINT('Ctrl Pts',(5.651070811,1.908585653,-4.559040496));
#127518=CARTESIAN_POINT('Ctrl Pts',(5.385863092,1.843501847,-4.85334717));
#127519=CARTESIAN_POINT('',(5.3890130067386,1.84427517318824,-4.84984935889788));
#127520=CARTESIAN_POINT('Origin',(-0.164204111051632,2.01783546428834,0.10933127938741));
#127521=CARTESIAN_POINT('Ctrl Pts',(5.57551601750762,1.88359401262131,-5.01633542878597));
#127522=CARTESIAN_POINT('Ctrl Pts',(5.54443000772672,1.87734523496005,-4.98853085853225));
#127523=CARTESIAN_POINT('Ctrl Pts',(5.51333079461951,1.87094900377837,-4.96074015636165));
#127524=CARTESIAN_POINT('Ctrl Pts',(5.45117360658552,1.85785291420127,-4.90525224101142));
#127525=CARTESIAN_POINT('Ctrl Pts',(5.42008188133855,1.85114594825435,-4.87752489447751));
#127526=CARTESIAN_POINT('Ctrl Pts',(5.38901300719691,1.84427517327111,-4.84984935883641));
#127527=CARTESIAN_POINT('Ctrl Pts',(5.739513988,1.843494248,-4.82783379800001));
#127528=CARTESIAN_POINT('Ctrl Pts',(5.476669394,1.909007671,-5.14031353300001));
#127529=CARTESIAN_POINT('Ctrl Pts',(5.181453912,1.974320085,-5.422410475));
#127530=CARTESIAN_POINT('Ctrl Pts',(5.392159262,1.843494248,-4.846351049));
#127531=CARTESIAN_POINT('Ctrl Pts',(5.12830652300001,1.909007671,-5.139919546));
#127532=CARTESIAN_POINT('Ctrl Pts',(4.83414196,1.974320085,-5.403107579));
#127533=CARTESIAN_POINT('Origin',(-0.144814768045344,1.87500001817188,0.137175170863457));
#127534=CARTESIAN_POINT('Ctrl Pts',(4.83647002372375,1.97885290468778,-5.73299289464033));
#127535=CARTESIAN_POINT('Ctrl Pts',(4.82563464912652,1.97658649484386,-5.74206417358371));
#127536=CARTESIAN_POINT('Ctrl Pts',(4.81479927452918,1.974320085,-5.75113545252697));
#127537=CARTESIAN_POINT('Ctrl Pts',(4.5005325515057,1.908585653,-6.01423674925969));
#127538=CARTESIAN_POINT('Ctrl Pts',(4.15946867633154,1.843501847,-6.24152796918688));
#127539=CARTESIAN_POINT('Ctrl Pts',(4.85450131171783,1.97885290468778,-5.38489213629658));
#127540=CARTESIAN_POINT('Ctrl Pts',(4.84432163585891,1.97658649484386,-5.39399985764828));
#127541=CARTESIAN_POINT('Ctrl Pts',(4.83414196,1.974320085,-5.403107579));
#127542=CARTESIAN_POINT('Ctrl Pts',(4.538892973,1.908585653,-5.667265843));
#127543=CARTESIAN_POINT('Ctrl Pts',(4.216618428,1.843501847,-5.89767997));
#127544=CARTESIAN_POINT('',(4.22044662604908,1.84427517322959,-5.8949410741957));
#127545=CARTESIAN_POINT('Origin',(-0.136862052139167,2.01783541418011,0.14207413403895));
#127546=CARTESIAN_POINT('Ctrl Pts',(4.36679971634735,1.88359401259236,-6.0976274267159));
#127547=CARTESIAN_POINT('Ctrl Pts',(4.34241764086487,1.87734523493682,-6.06379033863203));
#127548=CARTESIAN_POINT('Ctrl Pts',(4.31801968949418,1.87094900376049,-6.02996395608223));
#127549=CARTESIAN_POINT('Ctrl Pts',(4.26924399912386,1.85785292379131,-5.96241140879724));
#127550=CARTESIAN_POINT('Ctrl Pts',(4.24483972189638,1.85114595296674,-5.92864848400608));
#127551=CARTESIAN_POINT('Ctrl Pts',(4.22044662594175,1.84427517327394,-5.89494107440453));
#127552=CARTESIAN_POINT('Ctrl Pts',(4.567485784,1.843494248,-5.948787575));
#127553=CARTESIAN_POINT('Ctrl Pts',(4.243612444,1.909007671,-6.19745789));
#127554=CARTESIAN_POINT('Ctrl Pts',(3.894656432,1.974320085,-6.40949696000001));
#127555=CARTESIAN_POINT('Ctrl Pts',(4.224271357,1.843494248,-5.892200905));
#127556=CARTESIAN_POINT('Ctrl Pts',(3.903478799,1.909007671,-6.122185394));
#127557=CARTESIAN_POINT('Ctrl Pts',(3.559613992,1.974320085,-6.315983552));
#127558=CARTESIAN_POINT('Origin',(-0.111940529213434,1.87499999749396,0.165099073720274));
#127559=CARTESIAN_POINT('Ctrl Pts',(3.49097203493613,1.97885290457087,-6.63865679804626));
#127560=CARTESIAN_POINT('Ctrl Pts',(3.47843992888034,1.97658649478541,-6.64518671007442));
#127561=CARTESIAN_POINT('Ctrl Pts',(3.46590782282453,1.974320085,-6.65171662210265));
#127562=CARTESIAN_POINT('Ctrl Pts',(3.10242947983344,1.908585653,-6.84110869980463));
#127563=CARTESIAN_POINT('Ctrl Pts',(2.72047859428653,1.843501847,-6.98976732606163));
#127564=CARTESIAN_POINT('Ctrl Pts',(3.58341313450755,1.97885290457087,-6.30257063543203));
#127565=CARTESIAN_POINT('Ctrl Pts',(3.57151356325381,1.97658649478541,-6.30927709371597));
#127566=CARTESIAN_POINT('Ctrl Pts',(3.559613992,1.974320085,-6.315983552));
#127567=CARTESIAN_POINT('Ctrl Pts',(3.214481544,1.908585653,-6.510496137));
#127568=CARTESIAN_POINT('Ctrl Pts',(2.850209373,1.843501847,-6.66624381));
#127569=CARTESIAN_POINT('',(2.8545368520132,1.84427517323806,-6.66439189667409));
#127570=CARTESIAN_POINT('Origin',(-0.103120705606142,2.0178354347729,0.168174104005968));
#127571=CARTESIAN_POINT('Ctrl Pts',(2.95389671312413,1.88359401258902,-6.89380114309682));
#127572=CARTESIAN_POINT('Ctrl Pts',(2.93735865075846,1.87734523494571,-6.85551372191643));
#127573=CARTESIAN_POINT('Ctrl Pts',(2.92080278241338,1.87094900380797,-6.81723334327731));
#127574=CARTESIAN_POINT('Ctrl Pts',(2.88768920088988,1.85785290772959,-6.74077471128772));
#127575=CARTESIAN_POINT('Ctrl Pts',(2.87111353481052,1.85114594513236,-6.70255499693849));
#127576=CARTESIAN_POINT('Ctrl Pts',(2.854536852026,1.84427517338418,-6.66439189732531));
#127577=CARTESIAN_POINT('Ctrl Pts',(3.18188702,1.843494248,-6.791582657));
#127578=CARTESIAN_POINT('Ctrl Pts',(2.812128892,1.909007671,-6.964816003));
#127579=CARTESIAN_POINT('Ctrl Pts',(2.425749146,1.974320085,-7.09688249000001));
#127580=CARTESIAN_POINT('Ctrl Pts',(2.858861218,1.843494248,-6.662537995));
#127581=CARTESIAN_POINT('Ctrl Pts',(2.496128744,1.909007671,-6.818184657));
#127582=CARTESIAN_POINT('Ctrl Pts',(2.118642431,1.974320085,-6.933531153));
#127583=CARTESIAN_POINT('Origin',(-0.0738320489149108,1.87500005047324,
0.18530320439424));
#127584=CARTESIAN_POINT('Ctrl Pts',(1.98224007482369,1.97885290466213,-7.23390448551782));
#127585=CARTESIAN_POINT('Ctrl Pts',(1.96859722411596,1.97658649483104,-7.23758769956478));
#127586=CARTESIAN_POINT('Ctrl Pts',(1.95495437340829,1.974320085,-7.2412709136117));
#127587=CARTESIAN_POINT('Ctrl Pts',(1.55926025408112,1.908585653,-7.34809801080844));
#127588=CARTESIAN_POINT('Ctrl Pts',(1.1542819576241,1.843501847,-7.4111729312694));
#127589=CARTESIAN_POINT('Ctrl Pts',(2.14476854387364,1.97885290466213,-6.92554793491932));
#127590=CARTESIAN_POINT('Ctrl Pts',(2.13170548743684,1.97658649483104,-6.92953954395966));
#127591=CARTESIAN_POINT('Ctrl Pts',(2.118642431,1.974320085,-6.933531153));
#127592=CARTESIAN_POINT('Ctrl Pts',(1.739764532,1.908585653,-7.049302868));
#127593=CARTESIAN_POINT('Ctrl Pts',(1.350527695,1.843501847,-7.123101498));
#127594=CARTESIAN_POINT('',(1.35515210699593,1.84427517325148,-7.12222316151573));
#127595=CARTESIAN_POINT('Origin',(-0.0645573202645811,2.01783546286368,
0.186410085552468));
#127596=CARTESIAN_POINT('Ctrl Pts',(1.40287278318668,1.88359401260551,-7.36762837997682));
#127597=CARTESIAN_POINT('Ctrl Pts',(1.39495203533525,1.8773452349598,-7.32668090293733));
#127598=CARTESIAN_POINT('Ctrl Pts',(1.38701238381451,1.87094900380986,-7.28573647595215));
#127599=CARTESIAN_POINT('Ctrl Pts',(1.37110933005997,1.85785291182603,-7.20394698873801));
#127600=CARTESIAN_POINT('Ctrl Pts',(1.36313729993217,1.8511459471543,-7.16305753829043));
#127601=CARTESIAN_POINT('Ctrl Pts',(1.35515210661453,1.84427517341028,-7.12222316206877));
#127602=CARTESIAN_POINT('Ctrl Pts',(1.647506757,1.843494248,-7.316810882));
#127603=CARTESIAN_POINT('Ctrl Pts',(1.249153319,1.909007671,-7.40650706100001));
#127604=CARTESIAN_POINT('Ctrl Pts',(0.843416526000001,1.974320085,-7.452425683));
#127605=CARTESIAN_POINT('Ctrl Pts',(1.359773906,1.843494248,-7.121342214));
#127606=CARTESIAN_POINT('Ctrl Pts',(0.972062484,1.909007671,-7.195373184));
#127607=CARTESIAN_POINT('Ctrl Pts',(0.578605504,1.974320085,-7.226874544));
#127608=CARTESIAN_POINT('Origin',(-0.0322711797376609,1.87500005190778,
0.196842596558592));
#127609=CARTESIAN_POINT('Ctrl Pts',(0.363832912865866,1.97607974481604,
-7.49138129256546));
#127610=CARTESIAN_POINT('Ctrl Pts',(0.358353393929661,1.97519991490802,
-7.49163938192452));
#127611=CARTESIAN_POINT('Ctrl Pts',(0.352873874993457,1.974320085,-7.49189747128358));
#127612=CARTESIAN_POINT('Ctrl Pts',(-0.0565155554200859,1.908585653,-7.51118001358909));
#127613=CARTESIAN_POINT('Ctrl Pts',(-0.465568481217692,1.843501847,-7.48573935389003));
#127614=CARTESIAN_POINT('Ctrl Pts',(0.589176870235917,1.97607974481604,
-7.22602816834229));
#127615=CARTESIAN_POINT('Ctrl Pts',(0.583891187117959,1.97519991490802,
-7.22645135617115));
#127616=CARTESIAN_POINT('Ctrl Pts',(0.578605504000001,1.974320085,-7.226874544));
#127617=CARTESIAN_POINT('Ctrl Pts',(0.183698063,1.908585653,-7.258492032));
#127618=CARTESIAN_POINT('Ctrl Pts',(-0.212303156,1.843501847,-7.246890876));
#127619=CARTESIAN_POINT('',(-0.207598044914298,1.84427517323019,-7.24702718644853));
#127620=CARTESIAN_POINT('Origin',(-0.0229753300834366,2.01783542455855,
0.195929666395933));
#127621=CARTESIAN_POINT('Ctrl Pts',(-0.21374791896889,1.8835940087603,-7.49695347696991));
#127622=CARTESIAN_POINT('Ctrl Pts',(-0.212680986910686,1.87734523105937,
-7.45526060255581));
#127623=CARTESIAN_POINT('Ctrl Pts',(-0.211633172836878,1.87094900376037,
-7.41356666842629));
#127624=CARTESIAN_POINT('Ctrl Pts',(-0.209582099320414,1.85785290956532,
-7.33027067337607));
#127625=CARTESIAN_POINT('Ctrl Pts',(-0.208577724648135,1.85114594601346,
-7.28862345213287));
#127626=CARTESIAN_POINT('Ctrl Pts',(-0.207598044645778,1.84427517335404,
-7.24702718686974));
#127627=CARTESIAN_POINT('Ctrl Pts',(0.036090908,1.843494248,-7.499913163));
#127628=CARTESIAN_POINT('Ctrl Pts',(-0.372231275,1.909007671,-7.501878081));
#127629=CARTESIAN_POINT('Ctrl Pts',(-0.778353314,1.974320085,-7.459501734));
#127630=CARTESIAN_POINT('Ctrl Pts',(-0.202894923,1.843494248,-7.247160385));
#127631=CARTESIAN_POINT('Ctrl Pts',(-0.597456338,1.909007671,-7.236114058));
#127632=CARTESIAN_POINT('Ctrl Pts',(-0.988486373,1.974320085,-7.18229731300001));
#127633=CARTESIAN_POINT('Origin',(0.0107986194233051,1.87500008133751,0.199177593578839));
#127634=CARTESIAN_POINT('Ctrl Pts',(-1.23840528663667,1.97885290464283,
-7.3976349043454));
#127635=CARTESIAN_POINT('Ctrl Pts',(-1.25233374400524,1.97658649482139,
-7.39524921454754));
#127636=CARTESIAN_POINT('Ctrl Pts',(-1.26626220137385,1.974320085,-7.39286352474967));
#127637=CARTESIAN_POINT('Ctrl Pts',(-1.67023999264394,1.908585653,-7.32366952359896));
#127638=CARTESIAN_POINT('Ctrl Pts',(-2.06427281170063,1.843501847,-7.21086879728102));
#127639=CARTESIAN_POINT('Ctrl Pts',(-0.961422888963519,1.97885290464283,
-7.18602201056086));
#127640=CARTESIAN_POINT('Ctrl Pts',(-0.974954630981765,1.97658649482139,
-7.18415966178044));
#127641=CARTESIAN_POINT('Ctrl Pts',(-0.988486373,1.974320085,-7.182297313));
#127642=CARTESIAN_POINT('Ctrl Pts',(-1.380957923,1.908585653,-7.128282175));
#127643=CARTESIAN_POINT('Ctrl Pts',(-1.765206948,1.843501847,-7.031823692));
#127644=CARTESIAN_POINT('',(-1.76064114303171,1.84427517321804,-7.03296827513242));
#127645=CARTESIAN_POINT('Origin',(0.0196809364373435,2.01783541913575,0.196288130969764));
#127646=CARTESIAN_POINT('Ctrl Pts',(-1.82037400642531,1.88359401257156,
-7.27572941159547));
#127647=CARTESIAN_POINT('Ctrl Pts',(-1.81036928315231,1.8773452349258,-7.23524065217637));
#127648=CARTESIAN_POINT('Ctrl Pts',(-1.80038299703606,1.87094900377655,
-7.19474672350987));
#127649=CARTESIAN_POINT('Ctrl Pts',(-1.78047370253419,1.85785291130399,
-7.11383907339911));
#127650=CARTESIAN_POINT('Ctrl Pts',(-1.77053988675437,1.85114594686103,
-7.07338144623067));
#127651=CARTESIAN_POINT('Ctrl Pts',(-1.76064114249265,1.8442751733294,-7.03296827581398));
#127652=CARTESIAN_POINT('Ctrl Pts',(-1.577012512,1.843494248,-7.332327839));
#127653=CARTESIAN_POINT('Ctrl Pts',(-1.976210748,1.909007671,-7.246469619));
#127654=CARTESIAN_POINT('Ctrl Pts',(-2.363728217,1.974320085,-7.117779774));
#127655=CARTESIAN_POINT('Ctrl Pts',(-1.756076611,1.843494248,-7.034109392));
#127656=CARTESIAN_POINT('Ctrl Pts',(-2.139038765,1.909007671,-6.93850228));
#127657=CARTESIAN_POINT('Ctrl Pts',(-2.509357726,1.974320085,-6.801883842));
#127658=CARTESIAN_POINT('Origin',(0.0533635186575132,1.87500006335565,0.192199759904844));
#127659=CARTESIAN_POINT('Ctrl Pts',(-2.7997248903699,1.97885290475382,-6.95846178108168));
#127660=CARTESIAN_POINT('Ctrl Pts',(-2.81281485569747,1.97658649487688,
-6.95313766064793));
#127661=CARTESIAN_POINT('Ctrl Pts',(-2.82590482102504,1.974320085,-6.94781354021427));
#127662=CARTESIAN_POINT('Ctrl Pts',(-3.20556317165334,1.908585653,-6.79339397287292));
#127663=CARTESIAN_POINT('Ctrl Pts',(-3.56613489944187,1.843501847,-6.59852505700183));
#127664=CARTESIAN_POINT('Ctrl Pts',(-2.48372767044605,1.97885290475382,
-6.81133930751265));
#127665=CARTESIAN_POINT('Ctrl Pts',(-2.49654269822303,1.97658649487688,
-6.80661157475634));
#127666=CARTESIAN_POINT('Ctrl Pts',(-2.509357726,1.974320085,-6.801883842));
#127667=CARTESIAN_POINT('Ctrl Pts',(-2.881041851,1.908585653,-6.664761766));
#127668=CARTESIAN_POINT('Ctrl Pts',(-3.235571625,1.843501847,-6.487956247));
#127669=CARTESIAN_POINT('',(-3.23135861738484,1.84427517325405,-6.49005558348848));
#127670=CARTESIAN_POINT('Origin',(0.061416984041453,2.01783542994364,0.187468286320502));
#127671=CARTESIAN_POINT('Ctrl Pts',(-3.34188142830792,1.88359401257738,
-6.71430029947091));
#127672=CARTESIAN_POINT('Ctrl Pts',(-3.32340672345605,1.87734523493612,
-6.67690886461151));
#127673=CARTESIAN_POINT('Ctrl Pts',(-3.30494891336787,1.87094900375898,
-6.63950841770348));
#127674=CARTESIAN_POINT('Ctrl Pts',(-3.2681123138241,1.85785290416819,-6.5647722127061));
#127675=CARTESIAN_POINT('Ctrl Pts',(-3.24971356186856,1.85114594335815,
-6.52739596080021));
#127676=CARTESIAN_POINT('Ctrl Pts',(-3.2313586170509,1.84427517334694,-6.49005558433552));
#127677=CARTESIAN_POINT('Ctrl Pts',(-3.116376579,1.843494248,-6.821891015));
#127678=CARTESIAN_POINT('Ctrl Pts',(-3.487784803,1.909007671,-6.652224292));
#127679=CARTESIAN_POINT('Ctrl Pts',(-3.838577816,1.974320085,-6.443238343));
#127680=CARTESIAN_POINT('Ctrl Pts',(-3.227146108,1.843494248,-6.492151261));
#127681=CARTESIAN_POINT('Ctrl Pts',(-3.580602117,1.909007671,-6.316453848));
#127682=CARTESIAN_POINT('Ctrl Pts',(-3.912894301,1.974320085,-6.103421843));
#127683=CARTESIAN_POINT('Origin',(0.0934331116373954,1.8750000554617,0.176234561179568));
#127684=CARTESIAN_POINT('Ctrl Pts',(-4.23013246931658,1.97885290501278,
-6.19391872016159));
#127685=CARTESIAN_POINT('Ctrl Pts',(-4.2417718706794,1.97658649500636,-6.18590511866234));
#127686=CARTESIAN_POINT('Ctrl Pts',(-4.25341127204229,1.974320085,-6.17789151716295));
#127687=CARTESIAN_POINT('Ctrl Pts',(-4.590997779011,1.908585653,-5.94546687142094));
#127688=CARTESIAN_POINT('Ctrl Pts',(-4.90124848337868,1.843501847,-5.67764161845627));
#127689=CARTESIAN_POINT('Ctrl Pts',(-3.88989610614884,1.97885290501277,
-6.11816595014865));
#127690=CARTESIAN_POINT('Ctrl Pts',(-3.90139520357438,1.97658649500636,
-6.11079389657425));
#127691=CARTESIAN_POINT('Ctrl Pts',(-3.912894301,1.974320085,-6.103421843));
#127692=CARTESIAN_POINT('Ctrl Pts',(-4.246411465,1.908585653,-5.889604505));
#127693=CARTESIAN_POINT('Ctrl Pts',(-4.55464456900001,1.843501847,-5.640719178));
#127694=CARTESIAN_POINT('',(-4.55098135447045,1.84427517323348,-5.64367510627636));
#127695=CARTESIAN_POINT('Origin',(0.100281084782381,2.0178354216955,0.169882325749594));
#127696=CARTESIAN_POINT('Ctrl Pts',(-4.70712618881639,1.8835940125805,-5.83891796798881));
#127697=CARTESIAN_POINT('Ctrl Pts',(-4.68104535907145,1.87734523494553,
-5.80637223946444));
#127698=CARTESIAN_POINT('Ctrl Pts',(-4.65497909171563,1.87094900375453,
-5.77381407758736));
#127699=CARTESIAN_POINT('Ctrl Pts',(-4.60293773645489,1.85785292930389,
-5.70874406817867));
#127700=CARTESIAN_POINT('Ctrl Pts',(-4.57693429465633,1.85114595572434,
-5.67619677356006));
#127701=CARTESIAN_POINT('Ctrl Pts',(-4.55098135450667,1.84427517335135,
-5.64367510622254));
#127702=CARTESIAN_POINT('Ctrl Pts',(-4.510022341,1.843494248,-5.992470149));
#127703=CARTESIAN_POINT('Ctrl Pts',(-4.836273917,1.909007671,-5.746928351));
#127704=CARTESIAN_POINT('Ctrl Pts',(-5.133939783,1.974320085,-5.467418248));
#127705=CARTESIAN_POINT('Ctrl Pts',(-4.54731784,1.843494248,-5.646627353));
#127706=CARTESIAN_POINT('Ctrl Pts',(-4.854740493,1.909007671,-5.399055054));
#127707=CARTESIAN_POINT('Ctrl Pts',(-5.133468287,1.974320085,-5.119570621));
#127708=CARTESIAN_POINT('Origin',(0.129133949454096,1.87500001391295,0.152028971897913));
#127709=CARTESIAN_POINT('Ctrl Pts',(-5.46274375875203,1.97885290469671,
-5.13975490206963));
#127710=CARTESIAN_POINT('Ctrl Pts',(-5.4723883492393,1.97658649484833,-5.12942652758237));
#127711=CARTESIAN_POINT('Ctrl Pts',(-5.48203293972668,1.974320085,-5.11909815309525));
#127712=CARTESIAN_POINT('Ctrl Pts',(-5.7617624326188,1.908585653,-4.81953634573062));
#127713=CARTESIAN_POINT('Ctrl Pts',(-6.00718513649799,1.843501847,-4.49127796844836));
#127714=CARTESIAN_POINT('Ctrl Pts',(-5.11417732576643,1.97885290469671,
-5.13891394976885));
#127715=CARTESIAN_POINT('Ctrl Pts',(-5.12382280638329,1.97658649484833,
-5.12924228538445));
#127716=CARTESIAN_POINT('Ctrl Pts',(-5.133468287,1.974320085,-5.119570621));
#127717=CARTESIAN_POINT('Ctrl Pts',(-5.413223597,1.908585653,-4.839055883));
#127718=CARTESIAN_POINT('Ctrl Pts',(-5.660747395,1.843501847,-4.529728351));
#127719=CARTESIAN_POINT('',(-5.65780526120229,1.84427517321323,-4.53340265363974));
#127720=CARTESIAN_POINT('Origin',(0.134456337787581,2.01783546924622,0.144353208218378));
#127721=CARTESIAN_POINT('Ctrl Pts',(-5.85227096027949,1.8835940126381,-4.69051432171716));
#127722=CARTESIAN_POINT('Ctrl Pts',(-5.8198035162661,1.87734523498062,-4.66433610172389));
#127723=CARTESIAN_POINT('Ctrl Pts',(-5.78734762151557,1.87094900379007,
-4.6381426087021));
#127724=CARTESIAN_POINT('Ctrl Pts',(-5.72253480594809,1.85785292328267,
-4.58578122911845));
#127725=CARTESIAN_POINT('Ctrl Pts',(-5.69014261976781,1.85114595273634,
-4.55958485635383));
#127726=CARTESIAN_POINT('Ctrl Pts',(-5.65780526166866,1.84427517329743,
-4.5334026538501));
#127727=CARTESIAN_POINT('Ctrl Pts',(-5.692784471,1.843494248,-4.882848039));
#127728=CARTESIAN_POINT('Ctrl Pts',(-5.958624237,1.909007671,-4.572912427));
#127729=CARTESIAN_POINT('Ctrl Pts',(-6.189244432,1.974320085,-4.235947753));
#127730=CARTESIAN_POINT('Ctrl Pts',(-5.65486204400001,1.843494248,-4.537073425));
#127731=CARTESIAN_POINT('Ctrl Pts',(-5.9018766,1.909007671,-4.229202446));
#127732=CARTESIAN_POINT('Ctrl Pts',(-6.114007001,1.974320085,-3.896333968));
#127733=CARTESIAN_POINT('Origin',(0.158796591899705,1.87500003312575,0.120714626166288));
#127734=CARTESIAN_POINT('Ctrl Pts',(-6.43992321904848,1.97885290464865,
-3.845261857605));
#127735=CARTESIAN_POINT('Ctrl Pts',(-6.44712202908693,1.9765864948243,-3.83310165304336));
#127736=CARTESIAN_POINT('Ctrl Pts',(-6.45432083912527,1.974320085,-3.8209414484817));
#127737=CARTESIAN_POINT('Ctrl Pts',(-6.6631134784233,1.908585653,-3.46824965757397));
#127738=CARTESIAN_POINT('Ctrl Pts',(-6.83223248791254,1.843501847,-3.09490715287089));
#127739=CARTESIAN_POINT('Ctrl Pts',(-6.09932529574889,1.97885290464865,
-3.9193720467135));
#127740=CARTESIAN_POINT('Ctrl Pts',(-6.10666614837438,1.9765864948243,-3.90785300735674));
#127741=CARTESIAN_POINT('Ctrl Pts',(-6.114007001,1.974320085,-3.896333968));
#127742=CARTESIAN_POINT('Ctrl Pts',(-6.326919411,1.908585653,-3.562238386));
#127743=CARTESIAN_POINT('Ctrl Pts',(-6.502159964,1.843501847,-3.20693246));
#127744=CARTESIAN_POINT('',(-6.50007648227949,1.84427517319966,-3.21115333101409));
#127745=CARTESIAN_POINT('Origin',(0.162344440832116,2.0178354426907,0.112074132583747));
#127746=CARTESIAN_POINT('Ctrl Pts',(-6.72377004575471,1.88359401261591,
-3.32278743899844));
#127747=CARTESIAN_POINT('Ctrl Pts',(-6.68643412903717,1.87734523495608,
-3.30420079201031));
#127748=CARTESIAN_POINT('Ctrl Pts',(-6.64910620829137,1.87094900376282,
-3.28559674629494));
#127749=CARTESIAN_POINT('Ctrl Pts',(-6.57455251052133,1.85785291958716,
-3.24839237571781));
#127750=CARTESIAN_POINT('Ctrl Pts',(-6.5372862009905,1.8511459509194,-3.22977182764321));
#127751=CARTESIAN_POINT('Ctrl Pts',(-6.50007648257382,1.84427517330869,
-3.21115333145443));
#127752=CARTESIAN_POINT('Ctrl Pts',(-6.609358326,1.843494248,-3.544909382));
#127753=CARTESIAN_POINT('Ctrl Pts',(-6.80235591100001,1.909007671,-3.1850722));
#127754=CARTESIAN_POINT('Ctrl Pts',(-6.955146889,1.974320085,-2.806409048));
#127755=CARTESIAN_POINT('Ctrl Pts',(-6.497991183,1.843494248,-3.215370987));
#127756=CARTESIAN_POINT('Ctrl Pts',(-6.673047516,1.909007671,-2.861597032));
#127757=CARTESIAN_POINT('Ctrl Pts',(-6.808661543,1.974320085,-2.490909068));
#127758=CARTESIAN_POINT('Origin',(0.181034151572665,1.8750000352612,0.0837558341553082));
#127759=CARTESIAN_POINT('Ctrl Pts',(-7.11597902687631,1.97885290480238,
-2.37096864369072));
#127760=CARTESIAN_POINT('Ctrl Pts',(-7.12039544836194,1.97658649490116,
-2.35754520615908));
#127761=CARTESIAN_POINT('Ctrl Pts',(-7.1248118698477,1.974320085,-2.34412176862744));
#127762=CARTESIAN_POINT('Ctrl Pts',(-7.25290474381949,1.908585653,-1.95479147088445));
#127763=CARTESIAN_POINT('Ctrl Pts',(-7.3378122417283,1.843501847,-1.55382191763709));
#127764=CARTESIAN_POINT('Ctrl Pts',(-6.79927559345178,1.97885290480238,
-2.51656466271515));
#127765=CARTESIAN_POINT('Ctrl Pts',(-6.80396856822594,1.97658649490116,
-2.50373686535758));
#127766=CARTESIAN_POINT('Ctrl Pts',(-6.808661543,1.974320085,-2.490909068));
#127767=CARTESIAN_POINT('Ctrl Pts',(-6.944775505,1.908585653,-2.118854581));
#127768=CARTESIAN_POINT('Ctrl Pts',(-7.03953876,1.843501847,-1.734183971));
#127769=CARTESIAN_POINT('',(-7.03841135126299,1.84427517321604,-1.73875404815287));
#127770=CARTESIAN_POINT('Origin',(0.18264148930203,2.01783545948557,0.0745546352118537));
#127771=CARTESIAN_POINT('Ctrl Pts',(-7.2808731168689,1.88359401257483,-1.79969070845451));
#127772=CARTESIAN_POINT('Ctrl Pts',(-7.24041451346207,1.87734523492967,
-1.78956472535042));
#127773=CARTESIAN_POINT('Ctrl Pts',(-7.19995997890268,1.87094900375224,
-1.77942003139443));
#127774=CARTESIAN_POINT('Ctrl Pts',(-7.11915142346661,1.85785291281086,
-1.75911230892196));
#127775=CARTESIAN_POINT('Ctrl Pts',(-7.07875353435036,1.85114594757699,
-1.74893825936029));
#127776=CARTESIAN_POINT('Ctrl Pts',(-7.0384113518051,1.84427517329423,-1.73875404767566));
#127777=CARTESIAN_POINT('Ctrl Pts',(-7.216885931,1.843494248,-2.041214701));
#127778=CARTESIAN_POINT('Ctrl Pts',(-7.328016983,1.909007671,-1.648301537));
#127779=CARTESIAN_POINT('Ctrl Pts',(-7.395834409,1.974320085,-1.245645776));
#127780=CARTESIAN_POINT('Ctrl Pts',(-7.037281477,1.843494248,-1.743321375));
#127781=CARTESIAN_POINT('Ctrl Pts',(-7.132194147,1.909007671,-1.360186522));
#127782=CARTESIAN_POINT('Ctrl Pts',(-7.184950639,1.974320085,-0.969012029));
#127783=CARTESIAN_POINT('Origin',(0.194806796921273,1.87500000247012,0.0428807018730129));
#127784=CARTESIAN_POINT('Ctrl Pts',(-7.45929956467652,1.97885290464129,
-0.78581157002746));
#127785=CARTESIAN_POINT('Ctrl Pts',(-7.46072709035288,1.97658649482061,
-0.771752565412755));
#127786=CARTESIAN_POINT('Ctrl Pts',(-7.46215461602913,1.974320085,-0.757693560798031));
#127787=CARTESIAN_POINT('Ctrl Pts',(-7.50355824419952,1.908585653,-0.349929406925505));
#127788=CARTESIAN_POINT('Ctrl Pts',(-7.50028405152686,1.843501847,0.0599183031176641));
#127789=CARTESIAN_POINT('Ctrl Pts',(-7.18129932238051,1.97885290464129,
-0.996085510899448));
#127790=CARTESIAN_POINT('Ctrl Pts',(-7.18312498069023,1.97658649482062,
-0.982548769949733));
#127791=CARTESIAN_POINT('Ctrl Pts',(-7.184950639,1.974320085,-0.969012029));
#127792=CARTESIAN_POINT('Ctrl Pts',(-7.237901615,1.908585653,-0.576395491));
#127793=CARTESIAN_POINT('Ctrl Pts',(-7.24775654700001,1.843501847,-0.180346967));
#127794=CARTESIAN_POINT('',(-7.24763792831109,1.84427517320559,-0.185052557572839));
#127795=CARTESIAN_POINT('Origin',(0.194398464462716,2.01783547761427,0.033549063015667));
#127796=CARTESIAN_POINT('Ctrl Pts',(-7.49753065349355,1.88359401255793,
-0.192442440658495));
#127797=CARTESIAN_POINT('Ctrl Pts',(-7.45584116260488,1.87734523490727,
-0.191250601215969));
#127798=CARTESIAN_POINT('Ctrl Pts',(-7.41415162318411,1.8709490037309,-0.190039613672411));
#127799=CARTESIAN_POINT('Ctrl Pts',(-7.33086684937498,1.85785292580537,
-0.187578127585151));
#127800=CARTESIAN_POINT('Ctrl Pts',(-7.28922627644197,1.85114595396848,
-0.186326292333262));
#127801=CARTESIAN_POINT('Ctrl Pts',(-7.24763792841524,1.84427517330524,
-0.185052557297351));
#127802=CARTESIAN_POINT('Ctrl Pts',(-7.486959971,1.843494248,-0.44207509));
#127803=CARTESIAN_POINT('Ctrl Pts',(-7.511028126,1.909007671,-0.034458126));
#127804=CARTESIAN_POINT('Ctrl Pts',(-7.490700931,1.974320085,0.373362509));
#127805=CARTESIAN_POINT('Ctrl Pts',(-7.24751631,1.843494248,-0.189755993));
#127806=CARTESIAN_POINT('Ctrl Pts',(-7.25784730700001,1.909007671,0.204824799));
#127807=CARTESIAN_POINT('Ctrl Pts',(-7.225279428,1.974320085,0.598194935));
#127808=CARTESIAN_POINT('Origin',(0.199470203545421,1.8750000464348,4.69240410416738E-7));
#127809=CARTESIAN_POINT('Ctrl Pts',(-7.45383154587489,1.97885290461806,
0.836089179740119));
#127810=CARTESIAN_POINT('Ctrl Pts',(-7.45220342637013,1.97658649480901,
0.850126368365636));
#127811=CARTESIAN_POINT('Ctrl Pts',(-7.45057530686525,1.974320085,0.864163556991164));
#127812=CARTESIAN_POINT('Ctrl Pts',(-7.40335370093351,1.908585653,1.27129496698858));
#127813=CARTESIAN_POINT('Ctrl Pts',(-7.31205091452462,1.843501847,1.6708568105315));
#127814=CARTESIAN_POINT('Ctrl Pts',(-7.2275334754168,1.97885290461807,0.570969491001635));
#127815=CARTESIAN_POINT('Ctrl Pts',(-7.22640645170834,1.97658649480901,
0.584582213000813));
#127816=CARTESIAN_POINT('Ctrl Pts',(-7.225279428,1.974320085,0.598194935));
#127817=CARTESIAN_POINT('Ctrl Pts',(-7.19259149,1.908585653,0.993015212));
#127818=CARTESIAN_POINT('Ctrl Pts',(-7.117077294,1.843501847,1.38192286));
#127819=CARTESIAN_POINT('',(-7.11797301108935,1.84427517323171,1.37730178478774));
#127820=CARTESIAN_POINT('Origin',(0.197065557394361,2.01783543356719,-0.00902521413189389));
#127821=CARTESIAN_POINT('Ctrl Pts',(-7.36361198972978,1.88359401259995,
1.42380422152944));
#127822=CARTESIAN_POINT('Ctrl Pts',(-7.32264096579086,1.87734523495685,
1.41600618821186));
#127823=CARTESIAN_POINT('Ctrl Pts',(-7.28166577807059,1.87094900376748,
1.40822684487038));
#127824=CARTESIAN_POINT('Ctrl Pts',(-7.19979893011702,1.85785291315852,
1.39272700326356));
#127825=CARTESIAN_POINT('Ctrl Pts',(-7.15886282522385,1.85114594774797,
1.38499808700488));
#127826=CARTESIAN_POINT('Ctrl Pts',(-7.11797301143247,1.84427517330014,
1.37730178429855));
#127827=CARTESIAN_POINT('Ctrl Pts',(-7.406952085,1.843494248,1.17773546));
#127828=CARTESIAN_POINT('Ctrl Pts',(-7.34283194100001,1.909007671,1.580996508));
#127829=CARTESIAN_POINT('Ctrl Pts',(-7.235310603,1.974320085,1.974912778));
#127830=CARTESIAN_POINT('Ctrl Pts',(-7.118865336,1.843494248,1.372682168));
#127831=CARTESIAN_POINT('Ctrl Pts',(-7.044131593,1.909007671,1.760258739));
#127832=CARTESIAN_POINT('Ctrl Pts',(-6.927762182,1.974320085,2.137430969));
#127833=CARTESIAN_POINT('Origin',(0.194806978520468,1.87500002902488,-0.0428797811532663));
#127834=CARTESIAN_POINT('Ctrl Pts',(-7.0998306478305,1.97885290483717,2.41889532596028));
#127835=CARTESIAN_POINT('Ctrl Pts',(-7.09522301202677,1.97658649491861,
2.43225433604723));
#127836=CARTESIAN_POINT('Ctrl Pts',(-7.09061537622306,1.974320085,2.44561334613417));
#127837=CARTESIAN_POINT('Ctrl Pts',(-6.95697656713838,1.908585653,2.83307500209442));
#127838=CARTESIAN_POINT('Ctrl Pts',(-6.78191440264508,1.843501847,3.20366791034174));
#127839=CARTESIAN_POINT('Ctrl Pts',(-6.9358161971165,1.97885290483725,2.1113265930496));
#127840=CARTESIAN_POINT('Ctrl Pts',(-6.9317891895583,1.9765864949186,2.12437878102484));
#127841=CARTESIAN_POINT('Ctrl Pts',(-6.927762182,1.974320085,2.137430969));
#127842=CARTESIAN_POINT('Ctrl Pts',(-6.810963781,1.908585653,2.515993627));
#127843=CARTESIAN_POINT('Ctrl Pts',(-6.653611416,1.843501847,2.87957551));
#127844=CARTESIAN_POINT('',(-6.65547958671787,1.84427517323839,2.87525502574098));
#127845=CARTESIAN_POINT('Origin',(0.19051800560499,2.01783542516648,-0.0511774464633824));
#127846=CARTESIAN_POINT('Ctrl Pts',(-6.88537901292717,1.8835940125991,2.9734753811648));
#127847=CARTESIAN_POINT('Ctrl Pts',(-6.84704221537492,1.87734523494283,
2.95705210249745));
#127848=CARTESIAN_POINT('Ctrl Pts',(-6.8086973335707,1.87094900373705,2.94064618172785));
#127849=CARTESIAN_POINT('Ctrl Pts',(-6.73207659066844,1.85785292950792,
2.90790980639309));
#127850=CARTESIAN_POINT('Ctrl Pts',(-6.69375898680419,1.85114595578537,
2.8915615135695));
#127851=CARTESIAN_POINT('Ctrl Pts',(-6.65547958676117,1.8442751732726,2.87525502562493));
#127852=CARTESIAN_POINT('Ctrl Pts',(-6.98060335100001,1.843494248,2.74247641));
#127853=CARTESIAN_POINT('Ctrl Pts',(-6.831293095,1.909007671,3.122525503));
#127854=CARTESIAN_POINT('Ctrl Pts',(-6.641605193,1.974320085,3.48411832));
#127855=CARTESIAN_POINT('Ctrl Pts',(-6.65734413,1.843494248,2.870935237));
#127856=CARTESIAN_POINT('Ctrl Pts',(-6.501040115,1.909007671,3.233384938));
#127857=CARTESIAN_POINT('Ctrl Pts',(-6.30631047600001,1.974320085,3.576723107));
#127858=CARTESIAN_POINT('Origin',(0.181034478711073,1.8750000457319,-0.0837549443066887));
#127859=CARTESIAN_POINT('Ctrl Pts',(-6.41384955941865,1.9788529048304,3.88859661749972));
#127860=CARTESIAN_POINT('Ctrl Pts',(-6.40647785532257,1.97658649491523,
3.90065279583295));
#127861=CARTESIAN_POINT('Ctrl Pts',(-6.39910615122662,1.974320085,3.91270897416618));
#127862=CARTESIAN_POINT('Ctrl Pts',(-6.185298940816,1.908585653,4.26238359811813));
#127863=CARTESIAN_POINT('Ctrl Pts',(-5.93466311168911,1.843501847,4.58667905970337));
#127864=CARTESIAN_POINT('Ctrl Pts',(-6.31978786192062,1.97885290483039,
3.5529604120461));
#127865=CARTESIAN_POINT('Ctrl Pts',(-6.31304916896038,1.97658649491523,
3.56484175952307));
#127866=CARTESIAN_POINT('Ctrl Pts',(-6.306310476,1.974320085,3.576723107));
#127867=CARTESIAN_POINT('Ctrl Pts',(-6.110862975,1.908585653,3.921326977));
#127868=CARTESIAN_POINT('Ctrl Pts',(-5.879030064,1.843501847,4.24258241));
#127869=CARTESIAN_POINT('',(-5.88178333417953,1.84427517320727,4.2387645372747));
#127870=CARTESIAN_POINT('Origin',(0.175062231257839,2.01783539552014,-0.0909367358907742));
#127871=CARTESIAN_POINT('Ctrl Pts',(-6.08519336616643,1.8835940125841,4.38411013664153));
#127872=CARTESIAN_POINT('Ctrl Pts',(-6.05128338114171,1.87734523493651,
4.35982954685315));
#127873=CARTESIAN_POINT('Ctrl Pts',(-6.01736176949405,1.87094900374865,
4.33556417130605));
#127874=CARTESIAN_POINT('Ctrl Pts',(-5.94956971260758,1.85785292613734,
4.28712194686461));
#127875=CARTESIAN_POINT('Ctrl Pts',(-5.91566236205193,1.85114595411764,
4.26291872248372));
#127876=CARTESIAN_POINT('Ctrl Pts',(-5.88178333430147,1.84427517325654,
4.23876453754314));
#127877=CARTESIAN_POINT('Ctrl Pts',(-6.227849362,1.843494248,4.178982211));
#127878=CARTESIAN_POINT('Ctrl Pts',(-6.000330577,1.909007671,4.518048676));
#127879=CARTESIAN_POINT('Ctrl Pts',(-5.737345705,1.974320085,4.83041036200001));
#127880=CARTESIAN_POINT('Ctrl Pts',(-5.884532912,1.843494248,4.234946565));
#127881=CARTESIAN_POINT('Ctrl Pts',(-5.653967226,1.909007671,4.55532165));
#127882=CARTESIAN_POINT('Ctrl Pts',(-5.3899827,1.974320085,4.848771648));
#127883=CARTESIAN_POINT('Origin',(0.158797259040808,1.87500001238811,-0.120713940850057));
#127884=CARTESIAN_POINT('Ctrl Pts',(-5.42796399395947,1.97885290484628,
5.17647145251215));
#127885=CARTESIAN_POINT('Ctrl Pts',(-5.41817291423544,1.97658649492317,
5.18666106564932));
#127886=CARTESIAN_POINT('Ctrl Pts',(-5.40838183451139,1.974320085,5.1968506787866));
#127887=CARTESIAN_POINT('Ctrl Pts',(-5.12440361073545,1.908585653,5.4923878739928));
#127888=CARTESIAN_POINT('Ctrl Pts',(-4.80991356956785,1.843501847,5.75522219450518));
#127889=CARTESIAN_POINT('Ctrl Pts',(-5.40825326913996,1.97885290484627,
4.82846175120978));
#127890=CARTESIAN_POINT('Ctrl Pts',(-5.39911798456999,1.97658649492317,
4.83861669960489));
#127891=CARTESIAN_POINT('Ctrl Pts',(-5.3899827,1.974320085,4.848771648));
#127892=CARTESIAN_POINT('Ctrl Pts',(-5.125025008,1.908585653,5.143303435));
#127893=CARTESIAN_POINT('Ctrl Pts',(-4.8295518,1.843501847,5.407210872));
#127894=CARTESIAN_POINT('',(-4.83306143001308,1.84427517321803,5.40407413043285));
#127895=CARTESIAN_POINT('Origin',(0.151420717533058,2.01783542771218,-0.12644393058023));
#127896=CARTESIAN_POINT('Ctrl Pts',(-5.00047084119181,1.88359401262403,
5.58974877456317));
#127897=CARTESIAN_POINT('Ctrl Pts',(-4.9725732618044,1.87734523497229,5.55874620709685));
#127898=CARTESIAN_POINT('Ctrl Pts',(-4.94466105705933,1.87094900379013,
5.52775599881469));
#127899=CARTESIAN_POINT('Ctrl Pts',(-4.88886753539191,1.85785291404029,
5.46587298098978));
#127900=CARTESIAN_POINT('Ctrl Pts',(-4.86095592515359,1.85114594819124,
5.43494656698241));
#127901=CARTESIAN_POINT('Ctrl Pts',(-4.8330614303298,1.84427517330843,5.40407413074732));
#127902=CARTESIAN_POINT('Ctrl Pts',(-5.18388806,1.843494248,5.420083448));
#127903=CARTESIAN_POINT('Ctrl Pts',(-4.88879927000001,1.909007671,5.702312914));
#127904=CARTESIAN_POINT('Ctrl Pts',(-4.564814309,1.974320085,5.950837783));
#127905=CARTESIAN_POINT('Ctrl Pts',(-4.836567476,1.843494248,5.400936498));
#127906=CARTESIAN_POINT('Ctrl Pts',(-4.542521114,1.909007671,5.66425658500001));
#127907=CARTESIAN_POINT('Ctrl Pts',(-4.221625324,1.974320085,5.894097015));
#127908=CARTESIAN_POINT('Origin',(0.129134690010521,1.87500003313059,-0.152028384945208));
#127909=CARTESIAN_POINT('Ctrl Pts',(-4.18827286488025,1.97885290466945,
6.22230023654242));
#127910=CARTESIAN_POINT('Ctrl Pts',(-4.17652022996333,1.9765864948347,6.23014682915233));
#127911=CARTESIAN_POINT('Ctrl Pts',(-4.16476759504639,1.974320085,6.23799342176233));
#127912=CARTESIAN_POINT('Ctrl Pts',(-3.82389686242845,1.908585653,6.46557419751403));
#127913=CARTESIAN_POINT('Ctrl Pts',(-3.46025781439298,1.843501847,6.65465753517254));
#127914=CARTESIAN_POINT('Ctrl Pts',(-4.24383476395218,1.97885290466945,
5.87818958520869));
#127915=CARTESIAN_POINT('Ctrl Pts',(-4.23273004397611,1.9765864948347,5.88614330010443));
#127916=CARTESIAN_POINT('Ctrl Pts',(-4.221625324,1.974320085,5.894097015));
#127917=CARTESIAN_POINT('Ctrl Pts',(-3.899546568,1.908585653,6.124784741));
#127918=CARTESIAN_POINT('Ctrl Pts',(-3.554249061,1.843501847,6.319004163));
#127919=CARTESIAN_POINT('',(-3.55835094425643,1.84427517323502,6.3166952236111));
#127920=CARTESIAN_POINT('Origin',(0.120698810536738,2.01783543734752,-0.156038612833972));
#127921=CARTESIAN_POINT('Ctrl Pts',(-3.68193185676623,1.88359401262509,
6.5340169723509));
#127922=CARTESIAN_POINT('Ctrl Pts',(-3.66135114289436,1.87734523497312,
6.49774207272003));
#127923=CARTESIAN_POINT('Ctrl Pts',(-3.64075348875807,1.87094900379698,
6.4614760993466));
#127924=CARTESIAN_POINT('Ctrl Pts',(-3.59956739575161,1.85785291007888,
6.38904589216518));
#127925=CARTESIAN_POINT('Ctrl Pts',(-3.57895661493645,1.85114594625855,
6.35284236110538));
#127926=CARTESIAN_POINT('Ctrl Pts',(-3.55835094491587,1.84427517333389,
6.31669522370333));
#127927=CARTESIAN_POINT('Ctrl Pts',(-3.897533913,1.843494248,6.407747607));
#127928=CARTESIAN_POINT('Ctrl Pts',(-3.548673142,1.909007671,6.619943338));
#127929=CARTESIAN_POINT('Ctrl Pts',(-3.178837269,1.974320085,6.793010644));
#127930=CARTESIAN_POINT('Ctrl Pts',(-3.562449519,1.843494248,6.314384643));
#127931=CARTESIAN_POINT('Ctrl Pts',(-3.218671763,1.909007671,6.508337177));
#127932=CARTESIAN_POINT('Ctrl Pts',(-2.85586944,1.974320085,6.663820956));
#127933=CARTESIAN_POINT('Origin',(0.0934339420673402,1.87500003180126,-0.176234096547346));
#127934=CARTESIAN_POINT('Ctrl Pts',(-2.7527427519229,1.97885290481218,6.97718117610168));
#127935=CARTESIAN_POINT('Ctrl Pts',(-2.73957810122948,1.97658649490612,
6.98231785079368));
#127936=CARTESIAN_POINT('Ctrl Pts',(-2.72641345053611,1.974320085,6.98745452548581));
#127937=CARTESIAN_POINT('Ctrl Pts',(-2.34458894761934,1.908585653,7.13643745763093));
#127938=CARTESIAN_POINT('Ctrl Pts',(-1.94880424992615,1.843501847,7.2429284854553));
#127939=CARTESIAN_POINT('Ctrl Pts',(-2.88097926358645,1.97885290481218,
6.6530598058356));
#127940=CARTESIAN_POINT('Ctrl Pts',(-2.86842435179319,1.97658649490612,
6.65844038091781));
#127941=CARTESIAN_POINT('Ctrl Pts',(-2.85586944,1.974320085,6.66382095600001));
#127942=CARTESIAN_POINT('Ctrl Pts',(-2.491729664,1.908585653,6.819877919));
#127943=CARTESIAN_POINT('Ctrl Pts',(-2.112753586,1.843501847,6.935327843));
#127944=CARTESIAN_POINT('',(-2.11725592452661,1.84427517324134,6.93395466841877));
#127945=CARTESIAN_POINT('Origin',(0.08433334788541,2.0178354534903,-0.178337430490919));
#127946=CARTESIAN_POINT('Ctrl Pts',(-2.19122983104428,1.88359401259107,
7.1727617986861));
#127947=CARTESIAN_POINT('Ctrl Pts',(-2.178928313942,1.8773452349571,7.13291074102052));
#127948=CARTESIAN_POINT('Ctrl Pts',(-2.16660833371645,1.87094900378916,
7.09306475921236));
#127949=CARTESIAN_POINT('Ctrl Pts',(-2.14195551515702,1.85785291701669,
7.01347417968665));
#127950=CARTESIAN_POINT('Ctrl Pts',(-2.12960928501872,1.85114594968925,
6.97368633612843));
#127951=CARTESIAN_POINT('Ctrl Pts',(-2.11725592405781,1.84427517337193,
6.93395466915275));
#127952=CARTESIAN_POINT('Ctrl Pts',(-2.428935412,1.843494248,7.09579261));
#127953=CARTESIAN_POINT('Ctrl Pts',(-2.042615002,1.909007671,7.228032569));
#127954=CARTESIAN_POINT('Ctrl Pts',(-1.644221332,1.974320085,7.317549878));
#127955=CARTESIAN_POINT('Ctrl Pts',(-2.121755383,1.843494248,6.932579181));
#127956=CARTESIAN_POINT('Ctrl Pts',(-1.744320898,1.909007671,7.048095157));
#127957=CARTESIAN_POINT('Ctrl Pts',(-1.356576276,1.974320085,7.121952036));
#127958=CARTESIAN_POINT('Origin',(0.0533643618955854,1.87500006267099,-0.19219931587071));
#127959=CARTESIAN_POINT('Ctrl Pts',(-1.18849744514977,1.97885290443969,
7.40581687957402));
#127960=CARTESIAN_POINT('Ctrl Pts',(-1.17453634458622,1.97658649471982,
7.40800345071329));
#127961=CARTESIAN_POINT('Ctrl Pts',(-1.16057524402267,1.974320085,7.41019002185252));
#127962=CARTESIAN_POINT('Ctrl Pts',(-0.755650658846319,1.908585653,7.47360883382083));
#127963=CARTESIAN_POINT('Ctrl Pts',(-0.346226765269648,1.843501847,7.4925281505468));
#127964=CARTESIAN_POINT('Ctrl Pts',(-1.38341237288645,1.97885290443961,
7.11684034579532));
#127965=CARTESIAN_POINT('Ctrl Pts',(-1.36999432444322,1.97658649471983,
7.11939619089766));
#127966=CARTESIAN_POINT('Ctrl Pts',(-1.356576276,1.974320085,7.121952036));
#127967=CARTESIAN_POINT('Ctrl Pts',(-0.967402251,1.908585653,7.19608118600001));
#127968=CARTESIAN_POINT('Ctrl Pts',(-0.572468102,1.843501847,7.2273633));
#127969=CARTESIAN_POINT('',(-0.577160369379612,1.84427517324856,7.22699009949689));
#127970=CARTESIAN_POINT('Origin',(0.0440243840339853,2.01783543703188,-0.192297093393963));
#127971=CARTESIAN_POINT('Ctrl Pts',(-0.598068334408665,1.8835940126117,
7.4761162553008));
#127972=CARTESIAN_POINT('Ctrl Pts',(-0.5946212192703,1.8773452349364,7.43455243048903));
#127973=CARTESIAN_POINT('Ctrl Pts',(-0.591154981516255,1.87094900377116,
7.3929895940939));
#127974=CARTESIAN_POINT('Ctrl Pts',(-0.584188154548803,1.85785291826439,
7.30996017883959));
#127975=CARTESIAN_POINT('Ctrl Pts',(-0.580683782159009,1.85114595026308,
7.26844847389072));
#127976=CARTESIAN_POINT('Ctrl Pts',(-0.577160369361556,1.84427517331935,
7.22699009982512));
#127977=CARTESIAN_POINT('Ctrl Pts',(-0.846762591,1.843494248,7.452046237));
#127978=CARTESIAN_POINT('Ctrl Pts',(-0.441046456,1.909007671,7.49814703));
#127979=CARTESIAN_POINT('Ctrl Pts',(-0.032723432,1.974320085,7.499928611));
#127980=CARTESIAN_POINT('Ctrl Pts',(-0.581850323,1.843494248,7.226614021));
#127981=CARTESIAN_POINT('Ctrl Pts',(-0.188407526,1.909007671,7.25829204));
#127982=CARTESIAN_POINT('Ctrl Pts',(0.206148888,1.974320085,7.247068555));
#127983=CARTESIAN_POINT('Origin',(0.0107996477400095,1.87500005687486,-0.199177772428364));
#127984=CARTESIAN_POINT('Ctrl Pts',(-1.361045197,4.043593265,7.121099351));
#127985=CARTESIAN_POINT('Ctrl Pts',(-0.970451525,3.977881214,7.195752943));
#127986=CARTESIAN_POINT('Ctrl Pts',(-0.574036077000001,3.913265985,7.227238932));
#127987=CARTESIAN_POINT('Ctrl Pts',(-0.560316581672474,3.91102972418618,
7.2283286268672));
#127988=CARTESIAN_POINT('Ctrl Pts',(-0.546597086344946,3.90879346337243,
7.22941832173442));
#127989=CARTESIAN_POINT('Ctrl Pts',(-1.64941712647202,4.043593265,7.31692694226861));
#127990=CARTESIAN_POINT('Ctrl Pts',(-1.24808227386308,3.977881214,7.40739779012264));
#127991=CARTESIAN_POINT('Ctrl Pts',(-0.839260127710279,3.913265985,7.45343136981116));
#127992=CARTESIAN_POINT('Ctrl Pts',(-0.825111250434607,3.91102972418618,
7.45502454052292));
#127993=CARTESIAN_POINT('Ctrl Pts',(-0.810962373158929,3.90879346337243,
7.45661771123472));
#127994=CARTESIAN_POINT('',(-1.35637331166053,4.04280735947538,7.12199069250356));
#127995=CARTESIAN_POINT('Origin',(0.0550901651735161,4.16060449436388,-0.184791223054491));
#127996=CARTESIAN_POINT('Ctrl Pts',(-1.4023512112938,4.00345494164046,7.36772767377926));
#127997=CARTESIAN_POINT('Ctrl Pts',(-1.39471645654411,4.00969641606142,
7.32672440067642));
#127998=CARTESIAN_POINT('Ctrl Pts',(-1.38706468140527,4.01609134931217,
7.28572337574004));
#127999=CARTESIAN_POINT('Ctrl Pts',(-1.37174236273169,4.02919780697387,
7.20382449064816));
#128000=CARTESIAN_POINT('Ctrl Pts',(-1.36406293274999,4.03591692798231,
7.1628791187943));
#128001=CARTESIAN_POINT('Ctrl Pts',(-1.35637331617947,4.04280735924498,
7.1219906928173));
#128002=CARTESIAN_POINT('Ctrl Pts',(-2.114258167,3.913265985,6.934869314));
#128003=CARTESIAN_POINT('Ctrl Pts',(-1.738111442,3.978309763,7.049546498));
#128004=CARTESIAN_POINT('Ctrl Pts',(-1.351767779,4.043585554,7.122866268));
#128005=CARTESIAN_POINT('Ctrl Pts',(-1.95071269,3.913265985,7.241872686));
#128006=CARTESIAN_POINT('Ctrl Pts',(-1.557914128,3.978309763,7.347679177));
#128007=CARTESIAN_POINT('Ctrl Pts',(-1.155975786,4.043585554,7.410379206));
#128008=CARTESIAN_POINT('Origin',(0.0413517804109204,4.01785698658068,-0.195051286303896));
#128009=CARTESIAN_POINT('Ctrl Pts',(-2.860050579,4.043593265,6.662027521));
#128010=CARTESIAN_POINT('Ctrl Pts',(-2.494637086,3.977881214,6.818901846));
#128011=CARTESIAN_POINT('Ctrl Pts',(-2.114258167,3.913265985,6.934869314));
#128012=CARTESIAN_POINT('Ctrl Pts',(-2.10109367821903,3.91102972422222,
6.93888281831157));
#128013=CARTESIAN_POINT('Ctrl Pts',(-2.08792918943805,3.90879346344451,
6.9428963226233));
#128014=CARTESIAN_POINT('Ctrl Pts',(-3.18377767658012,4.043593265,6.79128533119683));
#128015=CARTESIAN_POINT('Ctrl Pts',(-2.81127436820558,3.977881214,6.96591615008532));
#128016=CARTESIAN_POINT('Ctrl Pts',(-2.42190611501457,3.913265985,7.09875816714873));
#128017=CARTESIAN_POINT('Ctrl Pts',(-2.40843051543541,3.91102972422222,
7.1033556807225));
#128018=CARTESIAN_POINT('Ctrl Pts',(-2.39495491585624,3.90879346344451,
7.10795319429614));
#128019=CARTESIAN_POINT('',(-2.85567953173816,4.04280735940842,6.66390234035358));
#128020=CARTESIAN_POINT('Origin',(0.093526238274001,4.1606042522063,-0.168626831068563));
#128021=CARTESIAN_POINT('Ctrl Pts',(-2.95340868090112,4.00345494158623,
6.89401023824049));
#128022=CARTESIAN_POINT('Ctrl Pts',(-2.93713793079008,4.00969641602971,
6.85560684540525));
#128023=CARTESIAN_POINT('Ctrl Pts',(-2.92085104149721,4.01609134928399,
6.81720930716438));
#128024=CARTESIAN_POINT('Ctrl Pts',(-2.88828110970197,4.02919780727587,
6.74051901626863));
#128025=CARTESIAN_POINT('Ctrl Pts',(-2.87197917614151,4.03591692811964,
6.70218177595648));
#128026=CARTESIAN_POINT('Ctrl Pts',(-2.85567953565621,4.04280735921878,
6.66390233986534));
#128027=CARTESIAN_POINT('Ctrl Pts',(-3.555619896,3.913265985,6.318232914));
#128028=CARTESIAN_POINT('Ctrl Pts',(-3.212919477,3.978309763,6.511089437));
#128029=CARTESIAN_POINT('Ctrl Pts',(-2.851369896,4.043585554,6.665747499));
#128030=CARTESIAN_POINT('Ctrl Pts',(-3.46189467,3.913265985,6.653216162));
#128031=CARTESIAN_POINT('Ctrl Pts',(-3.101024788,3.978309763,6.840989036));
#128032=CARTESIAN_POINT('Ctrl Pts',(-2.721962195,4.043585554,6.988628035));
#128033=CARTESIAN_POINT('Origin',(0.08231519453825,4.01785696096065,-0.18160153963801));
#128034=CARTESIAN_POINT('Ctrl Pts',(-4.225323174,4.043593265,5.891446688));
#128035=CARTESIAN_POINT('Ctrl Pts',(-3.902176188,3.977881214,6.123206478));
#128036=CARTESIAN_POINT('Ctrl Pts',(-3.555619896,3.913265985,6.318232914));
#128037=CARTESIAN_POINT('Ctrl Pts',(-3.54362597031878,3.9110297241893,6.32498256083445));
#128038=CARTESIAN_POINT('Ctrl Pts',(-3.53163204463758,3.90879346337866,
6.3317322076689));
#128039=CARTESIAN_POINT('Ctrl Pts',(-4.56926832085833,4.043593265,5.94809076502108));
#128040=CARTESIAN_POINT('Ctrl Pts',(-4.24301439629109,3.977881214,6.1987160133802));
#128041=CARTESIAN_POINT('Ctrl Pts',(-3.89130646372376,3.913265985,6.41215492265816));
#128042=CARTESIAN_POINT('Ctrl Pts',(-3.87913424552404,3.9110297241893,6.41954180460044));
#128043=CARTESIAN_POINT('Ctrl Pts',(-3.86696202732437,3.90879346337866,
6.42692868654285));
#128044=CARTESIAN_POINT('',(-4.22145735075434,4.04280735946812,5.89421732096231));
#128045=CARTESIAN_POINT('Origin',(0.127589615055383,4.16060422397286,-0.144579345889145));
#128046=CARTESIAN_POINT('Ctrl Pts',(-4.36636804309703,4.00345494166535,
6.0979365453881));
#128047=CARTESIAN_POINT('Ctrl Pts',(-4.34222209965502,4.00969641612163,
6.06392873275961));
#128048=CARTESIAN_POINT('Ctrl Pts',(-4.31806165314822,4.01609134933484,
6.02993010761872));
#128049=CARTESIAN_POINT('Ctrl Pts',(-4.26976703323223,4.02919780985992,
5.96203435267121));
#128050=CARTESIAN_POINT('Ctrl Pts',(-4.24560486129794,4.03591692942932,
5.9280978565823));
#128051=CARTESIAN_POINT('Ctrl Pts',(-4.22145735427668,4.04280735935845,
5.89421731921874));
#128052=CARTESIAN_POINT('Ctrl Pts',(-4.830724789,3.913265985,5.406162966));
#128053=CARTESIAN_POINT('Ctrl Pts',(-4.537494967,3.978309763,5.66818106999999));
#128054=CARTESIAN_POINT('Ctrl Pts',(-4.217645127,4.043585554,5.89694578400001));
#128055=CARTESIAN_POINT('Ctrl Pts',(-4.811202304,3.913265985,5.753462644));
#128056=CARTESIAN_POINT('Ctrl Pts',(-4.499134977,3.978309763,6.01442185));
#128057=CARTESIAN_POINT('Ctrl Pts',(-4.160672677,4.043585554,6.240096384));
#128058=CARTESIAN_POINT('Origin',(0.119429677617298,4.01785699117882,-0.159660485123626));
#128059=CARTESIAN_POINT('Ctrl Pts',(-5.393024354,4.043593265,4.845388355));
#128060=CARTESIAN_POINT('Ctrl Pts',(-5.12725387,3.977881214,5.14119678));
#128061=CARTESIAN_POINT('Ctrl Pts',(-4.830724789,3.913265985,5.406162966));
#128062=CARTESIAN_POINT('Ctrl Pts',(-4.82046224918153,3.911029724198,5.41533314932637));
#128063=CARTESIAN_POINT('Ctrl Pts',(-4.81019970936308,3.90879346339606,
5.42450333265286));
#128064=CARTESIAN_POINT('Ctrl Pts',(-5.74110505755348,4.043593265,4.82677008554403));
#128065=CARTESIAN_POINT('Ctrl Pts',(-5.47635578817261,3.977881214,5.14167080416162));
#128066=CARTESIAN_POINT('Ctrl Pts',(-5.17875364692804,3.913265985,5.42572643982063));
#128067=CARTESIAN_POINT('Ctrl Pts',(-5.16845396969476,3.911029724198,5.4355572876477));
#128068=CARTESIAN_POINT('Ctrl Pts',(-5.15815429246146,3.90879346339607,
5.44538813547477));
#128069=CARTESIAN_POINT('',(-5.38984451562663,4.04280735947174,4.84892525021678));
#128070=CARTESIAN_POINT('Origin',(0.155686880665156,4.16060425506628,-0.11377110263744));
#128071=CARTESIAN_POINT('Ctrl Pts',(-5.57516088824713,4.00345494158135,
5.01673011704008));
#128072=CARTESIAN_POINT('Ctrl Pts',(-5.54426878915666,4.00969641603625,
4.98870805233074));
#128073=CARTESIAN_POINT('Ctrl Pts',(-5.51336450100241,4.01609134927232,
4.96069807790655));
#128074=CARTESIAN_POINT('Ctrl Pts',(-5.45160341771255,4.02919780652563,
4.90477161763664));
#128075=CARTESIAN_POINT('Ctrl Pts',(-5.42071079214696,4.0359169277958,4.87682268306445));
#128076=CARTESIAN_POINT('Ctrl Pts',(-5.38984451945149,4.04280735930418,
4.8489252475705));
#128077=CARTESIAN_POINT('Ctrl Pts',(-5.87995036100001,3.913265985,4.241306845));
#128078=CARTESIAN_POINT('Ctrl Pts',(-5.649902236,3.978309763,4.560234855));
#128079=CARTESIAN_POINT('Ctrl Pts',(-5.386707959,4.043585554,4.852409439));
#128080=CARTESIAN_POINT('Ctrl Pts',(-5.935543465,3.913265985,4.584683607));
#128081=CARTESIAN_POINT('Ctrl Pts',(-5.686870614,3.978309763,4.906626983));
#128082=CARTESIAN_POINT('Ctrl Pts',(-5.404834728,4.043585554,5.199784761));
#128083=CARTESIAN_POINT('Origin',(0.150959951003408,4.01785697866393,-0.130254007742173));
#128084=CARTESIAN_POINT('Ctrl Pts',(-6.30855371000001,4.043593265,3.572765048));
#128085=CARTESIAN_POINT('Ctrl Pts',(-6.112586858,3.977881214,3.918790435));
#128086=CARTESIAN_POINT('Ctrl Pts',(-5.879950361,3.913265985,4.241306845));
#128087=CARTESIAN_POINT('Ctrl Pts',(-5.87189907219411,3.91102972423848,
4.25246877700563));
#128088=CARTESIAN_POINT('Ctrl Pts',(-5.86384778338835,3.90879346347703,
4.2636307090113));
#128089=CARTESIAN_POINT('Ctrl Pts',(-6.64449410151252,4.043593265,3.47975500206386));
#128090=CARTESIAN_POINT('Ctrl Pts',(-6.45362886927749,3.977881214,3.8442067835082));
#128091=CARTESIAN_POINT('Ctrl Pts',(-6.22404806647888,3.913265985,4.18559701939786));
#128092=CARTESIAN_POINT('Ctrl Pts',(-6.21610253182957,3.91102972423849,
4.19741215339487));
#128093=CARTESIAN_POINT('Ctrl Pts',(-6.20815699718011,3.90879346347704,
4.20922728739196));
#128094=CARTESIAN_POINT('',(-6.30620854175752,4.04280735942323,3.57690282405529));
#128095=CARTESIAN_POINT('Origin',(0.176504357918572,4.16060427540505,-0.0776430649302001));
#128096=CARTESIAN_POINT('Ctrl Pts',(-6.52326540639354,4.00345494158901,
3.70094696449352));
#128097=CARTESIAN_POINT('Ctrl Pts',(-6.48707163187172,4.00969641603995,
3.68022092820222));
#128098=CARTESIAN_POINT('Ctrl Pts',(-6.45086855211453,4.01609134930151,
3.65950931972563));
#128099=CARTESIAN_POINT('Ctrl Pts',(-6.37852886526694,4.02919780789907,
3.61816719197021));
#128100=CARTESIAN_POINT('Ctrl Pts',(-6.34235030148427,4.03591692842555,
3.59751269169148));
#128101=CARTESIAN_POINT('Ctrl Pts',(-6.30620854453905,4.04280735922747,
3.57690282104795));
#128102=CARTESIAN_POINT('Ctrl Pts',(-6.654235988,3.913265985,2.878131931));
#128103=CARTESIAN_POINT('Ctrl Pts',(-6.498126356,3.978309763,3.239057128));
#128104=CARTESIAN_POINT('Ctrl Pts',(-6.303894313,4.043585554,3.580979822));
#128105=CARTESIAN_POINT('Ctrl Pts',(-6.78234521,3.913265985,3.201529861));
#128106=CARTESIAN_POINT('Ctrl Pts',(-6.608694501,3.978309763,3.569403691));
#128107=CARTESIAN_POINT('Ctrl Pts',(-6.396272715,4.043585554,3.916336982));
#128108=CARTESIAN_POINT('Origin',(0.17543108332065,4.01785695518326,-0.0947566751364476));
#128109=CARTESIAN_POINT('Ctrl Pts',(-6.929102105,4.043593265,2.133083219));
#128110=CARTESIAN_POINT('Ctrl Pts',(-6.812102079,3.977881214,2.513145805));
#128111=CARTESIAN_POINT('Ctrl Pts',(-6.654235988,3.913265985,2.878131931));
#128112=CARTESIAN_POINT('Ctrl Pts',(-6.64877241920947,3.91102972421517,
2.89076369247807));
#128113=CARTESIAN_POINT('Ctrl Pts',(-6.64330885041899,3.9087934634304,2.90339545395617));
#128114=CARTESIAN_POINT('Ctrl Pts',(-7.23719398613233,4.043593265,1.97003044157168));
#128115=CARTESIAN_POINT('Ctrl Pts',(-7.12913743724499,3.977881214,2.36699192665264));
#128116=CARTESIAN_POINT('Ctrl Pts',(-6.9783129155358,3.913265985,2.74975373474382));
#128117=CARTESIAN_POINT('Ctrl Pts',(-6.97309304758036,3.91102972421517,
2.76300069269182));
#128118=CARTESIAN_POINT('Ctrl Pts',(-6.96787317962509,3.9087934634304,2.7762476506398));
#128119=CARTESIAN_POINT('',(-6.92770126536622,4.04280735945235,2.13762839710923));
#128120=CARTESIAN_POINT('Origin',(0.189068793117305,4.16060424051219,-0.0378846249697654));
#128121=CARTESIAN_POINT('Ctrl Pts',(-7.16634928428786,4.00345494158682,
2.21211164520099));
#128122=CARTESIAN_POINT('Ctrl Pts',(-7.12654621497235,4.00969641602803,
2.19965076379814));
#128123=CARTESIAN_POINT('Ctrl Pts',(-7.0867371595319,4.01609134928607,2.18720597323838));
#128124=CARTESIAN_POINT('Ctrl Pts',(-7.00720139359496,4.02919780879388,
2.16238129410652));
#128125=CARTESIAN_POINT('Ctrl Pts',(-6.96742856043411,4.03591692888643,
2.14998700724193));
#128126=CARTESIAN_POINT('Ctrl Pts',(-6.92770126721526,4.04280735930234,
2.13762839403927));
#128127=CARTESIAN_POINT('Ctrl Pts',(-7.117376937,3.913265985,1.380378766));
#128128=CARTESIAN_POINT('Ctrl Pts',(-7.042505309,3.978309763,1.766424689));
#128129=CARTESIAN_POINT('Ctrl Pts',(-6.926317576,4.043585554,2.142107568));
#128130=CARTESIAN_POINT('Ctrl Pts',(-7.312012032,3.913265985,1.668676136));
#128131=CARTESIAN_POINT('Ctrl Pts',(-7.221503179,3.978309763,2.06527905));
#128132=CARTESIAN_POINT('Ctrl Pts',(-7.088628098,4.043585554,2.449765639));
#128133=CARTESIAN_POINT('Origin',(0.191699739144654,4.01785698088617,-0.0548288895525728));
#128134=CARTESIAN_POINT('Ctrl Pts',(-7.225653387,4.043593265,0.593660789));
#128135=CARTESIAN_POINT('Ctrl Pts',(-7.193090978,3.977881214,0.989989269000001));
#128136=CARTESIAN_POINT('Ctrl Pts',(-7.117376937,3.913265985,1.380378766));
#128137=CARTESIAN_POINT('Ctrl Pts',(-7.11475655877205,3.91102972423475,
1.39388970960905));
#128138=CARTESIAN_POINT('Ctrl Pts',(-7.11213618054409,3.90879346346956,
1.40740065321813));
#128139=CARTESIAN_POINT('Ctrl Pts',(-7.49149072463913,4.043593265,0.368189448020171));
#128140=CARTESIAN_POINT('Ctrl Pts',(-7.47129546192345,3.977881214,0.779099157186393));
#128141=CARTESIAN_POINT('Ctrl Pts',(-7.40627960745195,3.913265985,1.18533502103219));
#128142=CARTESIAN_POINT('Ctrl Pts',(-7.40402948148748,3.91102972423475,
1.19939438966423));
#128143=CARTESIAN_POINT('Ctrl Pts',(-7.40177935552301,3.90879346346956,
1.21345375829623));
#128144=CARTESIAN_POINT('',(-7.22526237695295,4.04280735944336,0.598400842538234));
#128145=CARTESIAN_POINT('Origin',(0.19279253096347,4.16060420866803,0.00364529811502957));
#128146=CARTESIAN_POINT('Ctrl Pts',(-7.4743426348343,4.00345494159327,0.619840443920183));
#128147=CARTESIAN_POINT('Ctrl Pts',(-7.43279141797487,4.00969641603819,
0.616227374350984));
#128148=CARTESIAN_POINT('Ctrl Pts',(-7.39123781394975,4.01609134930466,
0.612631306257523));
#128149=CARTESIAN_POINT('Ctrl Pts',(-7.30822498460285,4.02919780773243,
0.605484853522622));
#128150=CARTESIAN_POINT('Ctrl Pts',(-7.26671760915875,4.03591692837949,
0.601930321309054));
#128151=CARTESIAN_POINT('Ctrl Pts',(-7.22526237832533,4.04280735930948,
0.598400839016713));
#128152=CARTESIAN_POINT('Ctrl Pts',(-7.24771725000001,3.913265985,-0.181919376));
#128153=CARTESIAN_POINT('Ctrl Pts',(-7.257584542,3.978309763,0.211196195));
#128154=CARTESIAN_POINT('Ctrl Pts',(-7.224873927,4.043585554,0.603072745000001));
#128155=CARTESIAN_POINT('Ctrl Pts',(-7.499777297,3.913265985,0.05779697));
#128156=CARTESIAN_POINT('Ctrl Pts',(-7.496642395,3.978309763,0.464584256));
#128157=CARTESIAN_POINT('Ctrl Pts',(-7.44952710999999,4.043585554,0.868645977));
#128158=CARTESIAN_POINT('Origin',(0.199004244133321,4.0178569914715,-0.0123372337777652));
#128159=CARTESIAN_POINT('Ctrl Pts',(-7.184341147,4.043593265,-0.97352056));
#128160=CARTESIAN_POINT('Ctrl Pts',(-7.237738938,3.977881214,-0.579458064));
#128161=CARTESIAN_POINT('Ctrl Pts',(-7.24771725,3.913265985,-0.181919376));
#128162=CARTESIAN_POINT('Ctrl Pts',(-7.24806258821313,3.91102972422533,
-0.168161006833082));
#128163=CARTESIAN_POINT('Ctrl Pts',(-7.24840792642623,3.90879346345072,
-0.154402637666171));
#128164=CARTESIAN_POINT('Ctrl Pts',(-7.39549368163611,4.043593265,-1.25086767559276));
#128165=CARTESIAN_POINT('Ctrl Pts',(-7.46410401451045,3.977881214,-0.845223421831474));
#128166=CARTESIAN_POINT('Ctrl Pts',(-7.48793689720315,3.913265985,-0.434508640665116));
#128167=CARTESIAN_POINT('Ctrl Pts',(-7.48876172660541,3.91102972422533,
-0.420294261657062));
#128168=CARTESIAN_POINT('Ctrl Pts',(-7.48958655600768,3.90879346345073,
-0.406079882649009));
#128169=CARTESIAN_POINT('',(-7.18497825053082,4.04280735945212,-0.968807270126785));
#128170=CARTESIAN_POINT('Origin',(0.18750158142266,4.16060424972495,0.0450047815784264));
#128171=CARTESIAN_POINT('Ctrl Pts',(-7.43284403029268,4.00345494162532,
-1.00141380765489));
#128172=CARTESIAN_POINT('Ctrl Pts',(-7.39148755465654,4.00969641607202,
-0.996010122351671));
#128173=CARTESIAN_POINT('Ctrl Pts',(-7.35013240261112,4.0160913493177,-0.990589319895412));
#128174=CARTESIAN_POINT('Ctrl Pts',(-7.26752408918023,4.02919780802441,
-0.979723387895262));
#128175=CARTESIAN_POINT('Ctrl Pts',(-7.22622301479033,4.03591692850297,
-0.974271958496376));
#128176=CARTESIAN_POINT('Ctrl Pts',(-7.18497825071308,4.04280735926566,
-0.968807274322354));
#128177=CARTESIAN_POINT('Ctrl Pts',(-7.03916236,3.913265985,-1.73571117));
#128178=CARTESIAN_POINT('Ctrl Pts',(-7.133307187,3.978309763,-1.353907599));
#128179=CARTESIAN_POINT('Ctrl Pts',(-7.185603203,4.043585554,-0.964161089));
#128180=CARTESIAN_POINT('Ctrl Pts',(-7.336861312,3.913265985,-1.555784718));
#128181=CARTESIAN_POINT('Ctrl Pts',(-7.421246943,3.978309763,-1.157833981));
#128182=CARTESIAN_POINT('Ctrl Pts',(-7.462094514,4.043585554,-0.753090606));
#128183=CARTESIAN_POINT('Origin',(0.197003933960296,4.01785696054259,0.0307312683205818));
#128184=CARTESIAN_POINT('Ctrl Pts',(-6.8070971,4.043593265,-2.495181169));
#128185=CARTESIAN_POINT('Ctrl Pts',(-6.943958268,3.977881214,-2.121810582));
#128186=CARTESIAN_POINT('Ctrl Pts',(-7.03916236,3.913265985,-1.73571117));
#128187=CARTESIAN_POINT('Ctrl Pts',(-7.04245726710452,3.91102972421939,
-1.72234870134003));
#128188=CARTESIAN_POINT('Ctrl Pts',(-7.04575217420907,3.9087934634388,-1.70898623267999));
#128189=CARTESIAN_POINT('Ctrl Pts',(-6.95369157447094,4.043593265,-2.81143561710356));
#128190=CARTESIAN_POINT('Ctrl Pts',(-7.10789935959764,3.977881214,-2.43002429438841));
#128191=CARTESIAN_POINT('Ctrl Pts',(-7.21946658014773,3.913265985,-2.0340351607318));
#128192=CARTESIAN_POINT('Ctrl Pts',(-7.22332779682342,3.91102972421939,
-2.02033041987044));
#128193=CARTESIAN_POINT('Ctrl Pts',(-7.22718901349899,3.9087934634388,-2.00662567900909));
#128194=CARTESIAN_POINT('',(-6.80873252631852,4.0428073594254,-2.49071503209414));
#128195=CARTESIAN_POINT('Origin',(0.173442981650553,4.16060425035759,0.0842598250759541));
#128196=CARTESIAN_POINT('Ctrl Pts',(-7.04379390051592,4.00345494159632,
-2.57584306268899));
#128197=CARTESIAN_POINT('Ctrl Pts',(-7.00456594895749,4.00969641603317,
-2.56167529283629));
#128198=CARTESIAN_POINT('Ctrl Pts',(-6.9653429695701,4.0160913492954,-2.5474910904707));
#128199=CARTESIAN_POINT('Ctrl Pts',(-6.88700185498726,4.02919780663038,
-2.51912085535247));
#128200=CARTESIAN_POINT('Ctrl Pts',(-6.84783826859157,4.0359169278048,-2.50491836557248));
#128201=CARTESIAN_POINT('Ctrl Pts',(-6.80873252610599,4.04280735920979,
-2.49071503615566));
#128202=CARTESIAN_POINT('Ctrl Pts',(-6.501464062,3.913265985,-3.208343039));
#128203=CARTESIAN_POINT('Ctrl Pts',(-6.675484317,3.978309763,-2.855704178));
#128204=CARTESIAN_POINT('Ctrl Pts',(-6.81034166,4.043585554,-2.486311822));
#128205=CARTESIAN_POINT('Ctrl Pts',(-6.830881846,3.913265985,-3.096619642));
#128206=CARTESIAN_POINT('Ctrl Pts',(-6.998842233,3.978309763,-2.726113188));
#128207=CARTESIAN_POINT('Ctrl Pts',(-7.125742672,4.043585554,-2.339613509));
#128208=CARTESIAN_POINT('Origin',(0.185791769945699,4.01785695583774,0.0723628059211712));
#128209=CARTESIAN_POINT('Ctrl Pts',(-6.111560759,4.043593265,-3.90016988));
#128210=CARTESIAN_POINT('Ctrl Pts',(-6.325485828,3.977881214,-3.564949595));
#128211=CARTESIAN_POINT('Ctrl Pts',(-6.501464062,3.913265985,-3.208343039));
#128212=CARTESIAN_POINT('Ctrl Pts',(-6.50755447170544,3.91102972424845,
-3.19600128524829));
#128213=CARTESIAN_POINT('Ctrl Pts',(-6.51364488141098,3.90879346349691,
-3.18365953149656));
#128214=CARTESIAN_POINT('Ctrl Pts',(-6.18674257775371,4.043593265,-4.24054395383126));
#128215=CARTESIAN_POINT('Ctrl Pts',(-6.41933723072147,3.977881214,-3.90119993089582));
#128216=CARTESIAN_POINT('Ctrl Pts',(-6.61342203006904,3.913265985,-3.53845245862718));
#128217=CARTESIAN_POINT('Ctrl Pts',(-6.62013908773441,3.91102972424845,
-3.52589817463696));
#128218=CARTESIAN_POINT('Ctrl Pts',(-6.62685614539979,3.90879346349691,
-3.51334389064676));
#128219=CARTESIAN_POINT('',(-6.11411803676986,4.04280735945579,-3.89615972702897));
#128220=CARTESIAN_POINT('Origin',(0.15127470020613,4.16060424379175,0.119575041319216));
#128221=CARTESIAN_POINT('Ctrl Pts',(-6.3253837967532,4.00345494159254,-4.02982875897273));
#128222=CARTESIAN_POINT('Ctrl Pts',(-6.29011862453826,4.00969641604317,
-4.00755937353869));
#128223=CARTESIAN_POINT('Ctrl Pts',(-6.2548618407542,4.01609134932245,-3.98527500864474));
#128224=CARTESIAN_POINT('Ctrl Pts',(-6.18445104407342,4.02919780960704,
-3.94072701982691));
#128225=CARTESIAN_POINT('Ctrl Pts',(-6.149256204571,4.03591692928036,-3.91843756826656));
#128226=CARTESIAN_POINT('Ctrl Pts',(-6.11411803576209,4.04280735930486,
-3.89615973061763));
#128227=CARTESIAN_POINT('Ctrl Pts',(-5.65976453,3.913265985,-4.530956353));
#128228=CARTESIAN_POINT('Ctrl Pts',(-5.905523219,3.978309763,-4.223971203));
#128229=CARTESIAN_POINT('Ctrl Pts',(-6.116636109,4.043585554,-3.892205378));
#128230=CARTESIAN_POINT('Ctrl Pts',(-6.005497937,3.913265985,-4.492660073));
#128231=CARTESIAN_POINT('Ctrl Pts',(-6.249179439,3.978309763,-4.166922373));
#128232=CARTESIAN_POINT('Ctrl Pts',(-6.456199023,4.043585554,-3.816738684));
#128233=CARTESIAN_POINT('Origin',(0.165892242201615,4.01785698412803,0.110610760434389));
#128234=CARTESIAN_POINT('Ctrl Pts',(-5.130254628,4.043593265,-5.122790982));
#128235=CARTESIAN_POINT('Ctrl Pts',(-5.411240701,3.977881214,-4.841395528));
#128236=CARTESIAN_POINT('Ctrl Pts',(-5.65976453,3.913265985,-4.530956353));
#128237=CARTESIAN_POINT('Ctrl Pts',(-5.66836566160238,3.91102972423425,
-4.52021240056111));
#128238=CARTESIAN_POINT('Ctrl Pts',(-5.67696679320477,3.90879346346851,
-4.50946844812222));
#128239=CARTESIAN_POINT('Ctrl Pts',(-5.13050837364047,4.043593265,-5.4713691678521));
#128240=CARTESIAN_POINT('Ctrl Pts',(-5.4306140264266,3.977881214,-5.18995979468907));
#128241=CARTESIAN_POINT('Ctrl Pts',(-5.69814121471092,3.913265985,-4.87741565142092));
#128242=CARTESIAN_POINT('Ctrl Pts',(-5.70740003131173,3.91102972423425,
-4.8665988483859));
#128243=CARTESIAN_POINT('Ctrl Pts',(-5.71665884791265,3.90879346346851,
-4.85578204535089));
#128244=CARTESIAN_POINT('',(-5.13361418334659,4.04280735946019,-5.11942432351775));
#128245=CARTESIAN_POINT('Origin',(0.122032764432595,4.16060423114288,0.149298916294309));
#128246=CARTESIAN_POINT('Ctrl Pts',(-5.31120577594162,4.00345494159354,
-5.29538414122324));
#128247=CARTESIAN_POINT('Ctrl Pts',(-5.2815523434773,4.00969641605275,-5.26605443207314));
#128248=CARTESIAN_POINT('Ctrl Pts',(-5.25191032365656,4.01609134929042,
-5.23671189715124));
#128249=CARTESIAN_POINT('Ctrl Pts',(-5.19272219896807,4.02919780824411,
-5.17806918153805));
#128250=CARTESIAN_POINT('Ctrl Pts',(-5.16314176519752,4.03591692858593,
-5.14873499164139));
#128251=CARTESIAN_POINT('Ctrl Pts',(-5.13361418103969,4.04280735921221,
-5.1194243271406));
#128252=CARTESIAN_POINT('Ctrl Pts',(-4.553420698,3.913265985,-5.641707183));
#128253=CARTESIAN_POINT('Ctrl Pts',(-4.85942641899999,3.978309763,-5.39473003));
#128254=CARTESIAN_POINT('Ctrl Pts',(-5.136923453,4.043585554,-5.116103736));
#128255=CARTESIAN_POINT('Ctrl Pts',(-4.899303619,3.913265985,-5.678628712));
#128256=CARTESIAN_POINT('Ctrl Pts',(-5.20731196000001,3.978309763,-5.412890898));
#128257=CARTESIAN_POINT('Ctrl Pts',(-5.484770682,4.043585554,-5.115397401));
#128258=CARTESIAN_POINT('Origin',(0.138235559680123,4.01785695374291,0.143686509914068));
#128259=CARTESIAN_POINT('Ctrl Pts',(-3.909063493,4.043593265,-6.105876072));
#128260=CARTESIAN_POINT('Ctrl Pts',(-4.243971972,3.977881214,-5.891463186));
#128261=CARTESIAN_POINT('Ctrl Pts',(-4.553420698,3.913265985,-5.64170718300001));
#128262=CARTESIAN_POINT('Ctrl Pts',(-4.56413037193816,3.91102972426959,
-5.63306340737098));
#128263=CARTESIAN_POINT('Ctrl Pts',(-4.57484004587628,3.90879346353919,
-5.62441963174208));
#128264=CARTESIAN_POINT('Ctrl Pts',(-3.8343773006698,4.043593265,-6.44635924039629));
#128265=CARTESIAN_POINT('Ctrl Pts',(-4.18796134717372,3.977881214,-6.23604290637241));
#128266=CARTESIAN_POINT('Ctrl Pts',(-4.51642165067599,3.913265985,-5.98831630932453));
#128267=CARTESIAN_POINT('Ctrl Pts',(-4.52778929402551,3.91102972426959,
-5.97974276916334));
#128268=CARTESIAN_POINT('Ctrl Pts',(-4.539156937375,3.9087934635392,-5.97116922900215));
#128269=CARTESIAN_POINT('',(-3.91306823576687,4.04280735944647,-6.10331032894653));
#128270=CARTESIAN_POINT('Origin',(0.0870848940551211,4.16060424395647,0.172041892549754));
#128271=CARTESIAN_POINT('Ctrl Pts',(-4.04868167678957,4.00345494162143,
-6.31333324611067));
#128272=CARTESIAN_POINT('Ctrl Pts',(-4.02602654552544,4.00969641605222,
-6.27831463799619));
#128273=CARTESIAN_POINT('Ctrl Pts',(-4.00338531713494,4.01609134929976,
-6.24328595714909));
#128274=CARTESIAN_POINT('Ctrl Pts',(-3.95818743098564,4.02919780741784,
-6.17329058298552));
#128275=CARTESIAN_POINT('Ctrl Pts',(-3.93560455346319,4.03591692817666,
-6.13828328903173));
#128276=CARTESIAN_POINT('Ctrl Pts',(-3.91306823295186,4.04280735919888,
-6.10331033194858));
#128277=CARTESIAN_POINT('Ctrl Pts',(-3.234163976,3.913265985,-6.488658057));
#128278=CARTESIAN_POINT('Ctrl Pts',(-3.58610824,3.978309763,-6.31323727599999));
#128279=CARTESIAN_POINT('Ctrl Pts',(-3.917013965,4.043585554,-6.10077877));
#128280=CARTESIAN_POINT('Ctrl Pts',(-3.564023309,3.913265985,-6.599070984));
#128281=CARTESIAN_POINT('Ctrl Pts',(-3.921956361,3.978309763,-6.40575866100001));
#128282=CARTESIAN_POINT('Ctrl Pts',(-4.25688056,4.043585554,-6.17486582));
#128283=CARTESIAN_POINT('Origin',(0.104115509673351,4.01785695580956,0.170044049114778));
#128284=CARTESIAN_POINT('Ctrl Pts',(-2.505088894,4.043593265,-6.803457182));
#128285=CARTESIAN_POINT('Ctrl Pts',(-2.878259831,3.977881214,-6.666052574));
#128286=CARTESIAN_POINT('Ctrl Pts',(-3.234163976,3.913265985,-6.488658057));
#128287=CARTESIAN_POINT('Ctrl Pts',(-3.24648142007391,3.91102972425195,
-6.4825186313348));
#128288=CARTESIAN_POINT('Ctrl Pts',(-3.25879886414786,3.90879346350392,
-6.47637920566949));
#128289=CARTESIAN_POINT('Ctrl Pts',(-2.35895500654199,4.043593265,-7.11992472055484));
#128290=CARTESIAN_POINT('Ctrl Pts',(-2.74948424915754,3.977881214,-6.99053558333539));
#128291=CARTESIAN_POINT('Ctrl Pts',(-3.12351922935454,3.913265985,-6.81920995168694));
#128292=CARTESIAN_POINT('Ctrl Pts',(-3.1364641613397,3.91102972425195,-6.8132805633505));
#128293=CARTESIAN_POINT('Ctrl Pts',(-3.14940909332493,3.90879346350392,
-6.80735117501388));
#128294=CARTESIAN_POINT('',(-2.50955156673443,4.04280735945939,-6.80181232628126));
#128295=CARTESIAN_POINT('Origin',(0.0480650262536675,4.16060428568896,0.186740464814262));
#128296=CARTESIAN_POINT('Ctrl Pts',(-2.59684572190937,4.00345494161758,
-7.03607790590514));
#128297=CARTESIAN_POINT('Ctrl Pts',(-2.58224822063566,4.00969641605882,
-6.99700782975648));
#128298=CARTESIAN_POINT('Ctrl Pts',(-2.56766646253128,4.01609134931304,
-6.95793090509845));
#128299=CARTESIAN_POINT('Ctrl Pts',(-2.53857221501533,4.02919780708633,
-6.87985577640105));
#128300=CARTESIAN_POINT('Ctrl Pts',(-2.52404284554597,4.03591692804071,
-6.84081228116046));
#128301=CARTESIAN_POINT('Ctrl Pts',(-2.50955156324783,4.04280735924479,
-6.80181232858497));
#128302=CARTESIAN_POINT('Ctrl Pts',(-1.763681341,3.913265985,-7.032206491));
#128303=CARTESIAN_POINT('Ctrl Pts',(-2.145107626,3.978309763,-6.936544564));
#128304=CARTESIAN_POINT('Ctrl Pts',(-2.513949257,4.043585554,-6.800188169));
#128305=CARTESIAN_POINT('Ctrl Pts',(-2.06209323,3.913265985,-7.21094803100001));
#128306=CARTESIAN_POINT('Ctrl Pts',(-2.453214441,3.978309763,-7.099100269));
#128307=CARTESIAN_POINT('Ctrl Pts',(-2.829943435,4.043585554,-6.945604377));
#128308=CARTESIAN_POINT('Origin',(0.0651268731426771,4.01785696157778,0.18845016650496));
#128309=CARTESIAN_POINT('Ctrl Pts',(-0.983979122,4.043593265,-7.182916197));
#128310=CARTESIAN_POINT('Ctrl Pts',(-1.37796346,3.977881214,-7.128944752));
#128311=CARTESIAN_POINT('Ctrl Pts',(-1.763681341,3.913265985,-7.032206491));
#128312=CARTESIAN_POINT('Ctrl Pts',(-1.77703060513271,3.91102972424724,
-7.0288584880646));
#128313=CARTESIAN_POINT('Ctrl Pts',(-1.79037986926543,3.90879346349449,
-7.02551048512909));
#128314=CARTESIAN_POINT('Ctrl Pts',(-0.773230597839176,4.043593265,-7.46057043305692));
#128315=CARTESIAN_POINT('Ctrl Pts',(-1.18244432400907,3.977881214,-7.41815858538808));
#128316=CARTESIAN_POINT('Ctrl Pts',(-1.58456451966031,3.913265985,-7.3312449165871));
#128317=CARTESIAN_POINT('Ctrl Pts',(-1.59848144954423,3.91102972424724,
-7.32823693179117));
#128318=CARTESIAN_POINT('Ctrl Pts',(-1.61239837942815,3.90879346349449,
-7.32522894699524));
#128319=CARTESIAN_POINT('',(-0.988691055522213,4.04280735945093,-7.18226913894742));
#128320=CARTESIAN_POINT('Origin',(0.00679763605742609,4.16060425918084,
0.19270726971797));
#128321=CARTESIAN_POINT('Ctrl Pts',(-1.02358414735161,4.00345494160357,
-7.42982338229497));
#128322=CARTESIAN_POINT('Ctrl Pts',(-1.01772683905242,4.00969641604632,
-7.38852871155796));
#128323=CARTESIAN_POINT('Ctrl Pts',(-1.01188637805703,4.01609134930418,
-7.3472307367515));
#128324=CARTESIAN_POINT('Ctrl Pts',(-1.00025618222515,4.02919780756502,
-7.26472655507422));
#128325=CARTESIAN_POINT('Ctrl Pts',(-0.994459698903276,4.03591692827595,
-7.22347249182076));
#128326=CARTESIAN_POINT('Ctrl Pts',(-0.988691051854008,4.04280735925939,
-7.18226914059731));
#128327=CARTESIAN_POINT('Ctrl Pts',(-0.210730926,3.913265985,-7.246936765));
#128328=CARTESIAN_POINT('Ctrl Pts',(-0.603804163,3.978309763,-7.235506737));
#128329=CARTESIAN_POINT('Ctrl Pts',(-0.993335076,4.043585554,-7.181628327));
#128330=CARTESIAN_POINT('Ctrl Pts',(-0.463741963,3.913265985,-7.485649163));
#128331=CARTESIAN_POINT('Ctrl Pts',(-0.869762941,3.978309763,-7.460495838));
#128332=CARTESIAN_POINT('Ctrl Pts',(-1.2706813,4.043585554,-7.391574192));
#128333=CARTESIAN_POINT('Origin',(0.0230930328050315,4.01785696223938,0.198044760085584));
#128334=CARTESIAN_POINT('Ctrl Pts',(0.583140419,4.043593265,-7.226510033));
#128335=CARTESIAN_POINT('Ctrl Pts',(0.186764952,3.977881214,-7.258495397));
#128336=CARTESIAN_POINT('Ctrl Pts',(-0.210730926,3.913265985,-7.246936765));
#128337=CARTESIAN_POINT('Ctrl Pts',(-0.224487813524214,3.91102972423126,
-7.24653673368102));
#128338=CARTESIAN_POINT('Ctrl Pts',(-0.238244701048428,3.90879346346254,
-7.24613670236216));
#128339=CARTESIAN_POINT('Ctrl Pts',(0.848649214287638,4.043593265,-7.45236816437252));
#128340=CARTESIAN_POINT('Ctrl Pts',(0.439885384551184,3.977881214,-7.49891673678223));
#128341=CARTESIAN_POINT('Ctrl Pts',(0.0284826653429041,3.913265985,-7.5004790163336));
#128342=CARTESIAN_POINT('Ctrl Pts',(0.0142444776067684,3.91102972423126,
-7.50053308508062));
#128343=CARTESIAN_POINT('Ctrl Pts',(6.28987063271302E-6,3.90879346346255,
-7.50058715382766));
#128344=CARTESIAN_POINT('',(0.578399550099043,4.04280735946618,-7.22689102929937));
#128345=CARTESIAN_POINT('Origin',(-0.034787638241215,4.16060423561476,0.189663017005176));
#128346=CARTESIAN_POINT('Ctrl Pts',(0.597539084743176,4.00345494159598,
-7.47615857517617));
#128347=CARTESIAN_POINT('Ctrl Pts',(0.594382318797106,4.00969641605215,
-7.43457020272798));
#128348=CARTESIAN_POINT('Ctrl Pts',(0.591208389122248,4.01609134932308,
-7.39298222514298));
#128349=CARTESIAN_POINT('Ctrl Pts',(0.584830715843343,4.02919780977328,
-7.30990678336319));
#128350=CARTESIAN_POINT('Ctrl Pts',(0.581623276858757,4.03591692937593,
-7.26837115206616));
#128351=CARTESIAN_POINT('Ctrl Pts',(0.578399553874348,4.04280735933351,
-7.22689102998411));
#128352=CARTESIAN_POINT('Ctrl Pts',(1.352073032,3.913265985,-7.122808331));
#128353=CARTESIAN_POINT('Ctrl Pts',(0.965732511,3.978309763,-7.19614465799999));
#128354=CARTESIAN_POINT('Ctrl Pts',(0.573726349,4.043585554,-7.227263526));
#128355=CARTESIAN_POINT('Ctrl Pts',(1.156293362,3.913265985,-7.410329659));
#128356=CARTESIAN_POINT('Ctrl Pts',(0.754357708,3.978309763,-7.473046914));
#128357=CARTESIAN_POINT('Ctrl Pts',(0.347996481,4.043585554,-7.491922213));
#128358=CARTESIAN_POINT('Origin',(-0.0200205943985987,4.01785696253182,
0.198378610296422));
#128359=CARTESIAN_POINT('Ctrl Pts',(2.122992963,4.043593265,-6.932200291));
#128360=CARTESIAN_POINT('Ctrl Pts',(1.742760442,3.977881214,-7.048646864));
#128361=CARTESIAN_POINT('Ctrl Pts',(1.352073032,3.913265985,-7.122808331));
#128362=CARTESIAN_POINT('Ctrl Pts',(1.33855177753404,3.91102972416506,-7.12537497645928));
#128363=CARTESIAN_POINT('Ctrl Pts',(1.32503052306806,3.90879346333014,-7.12794162191861));
#128364=CARTESIAN_POINT('Ctrl Pts',(2.43084713209943,4.043593265,-7.09570144285702));
#128365=CARTESIAN_POINT('Ctrl Pts',(2.04164654045871,3.977881214,-7.22903387662127));
#128366=CARTESIAN_POINT('Ctrl Pts',(1.64019803211851,3.913265985,-7.31899905409572));
#128367=CARTESIAN_POINT('Ctrl Pts',(1.62630434807006,3.91102972416506,-7.32211264830573));
#128368=CARTESIAN_POINT('Ctrl Pts',(1.6124106640216,3.90879346333014,-7.32522624251587));
#128369=CARTESIAN_POINT('',(2.11844483583129,4.04280735942594,-6.93359152700834));
#128370=CARTESIAN_POINT('Origin',(-0.0747462306194105,4.16060422367809,
0.177750342392968));
#128371=CARTESIAN_POINT('Ctrl Pts',(2.19072205301252,4.00345494162878,-7.17291690241065));
#128372=CARTESIAN_POINT('Ctrl Pts',(2.17869881975252,4.00969641607101,-7.13297945426373));
#128373=CARTESIAN_POINT('Ctrl Pts',(2.16665890893221,4.01609134932407,-7.09304608144558));
#128374=CARTESIAN_POINT('Ctrl Pts',(2.14257158065363,4.02919780818236,-7.01328391782595));
#128375=CARTESIAN_POINT('Ctrl Pts',(2.13051019526031,4.03591692859592,-6.97340886569841));
#128376=CARTESIAN_POINT('Ctrl Pts',(2.11844483965137,4.04280735930388,-6.93359152644189));
#128377=CARTESIAN_POINT('Ctrl Pts',(2.851655559,3.913265985,-6.665625295));
#128378=CARTESIAN_POINT('Ctrl Pts',(2.490112606,3.978309763,-6.820298851));
#128379=CARTESIAN_POINT('Ctrl Pts',(2.113960967,4.043585554,-6.934959915));
#128380=CARTESIAN_POINT('Ctrl Pts',(2.722261695,3.913265985,-6.988511377));
#128381=CARTESIAN_POINT('Ctrl Pts',(2.343205429,3.978309763,-7.136166621));
#128382=CARTESIAN_POINT('Ctrl Pts',(1.950402333,4.043585554,-7.241956279));
#128383=CARTESIAN_POINT('Origin',(-0.0621981411914818,4.01785698790786,
0.18943702702451));
#128384=CARTESIAN_POINT('Ctrl Pts',(3.563576716,4.043593265,-6.313748569));
#128385=CARTESIAN_POINT('Ctrl Pts',(3.21726639,3.977881214,-6.509211438));
#128386=CARTESIAN_POINT('Ctrl Pts',(2.851655559,3.913265985,-6.665625295));
#128387=CARTESIAN_POINT('Ctrl Pts',(2.83900217674919,3.91102972413889,-6.67103860378116));
#128388=CARTESIAN_POINT('Ctrl Pts',(2.82634879449839,3.90879346327781,-6.67645191256244));
#128389=CARTESIAN_POINT('Ctrl Pts',(3.89938133908574,4.043593265,-6.40724760846984));
#128390=CARTESIAN_POINT('Ctrl Pts',(3.5479425741295,3.977881214,-6.6211294263161));
#128391=CARTESIAN_POINT('Ctrl Pts',(3.1752195618941,3.913265985,-6.79529083046101));
#128392=CARTESIAN_POINT('Ctrl Pts',(3.16232003499938,3.91102972413889,-6.80131836201407));
#128393=CARTESIAN_POINT('Ctrl Pts',(3.14942050810468,3.9087934632778,-6.80734589356702));
#128394=CARTESIAN_POINT('',(3.55943399567121,4.04280735940916,-6.31608499157434));
#128395=CARTESIAN_POINT('Origin',(-0.111209903497371,4.16060421018104,0.1575266722846));
#128396=CARTESIAN_POINT('Ctrl Pts',(3.68146929256206,4.00345494161536,-6.53427760732435));
#128397=CARTESIAN_POINT('Ctrl Pts',(3.66114178509397,4.00969641604704,-6.4978585143677));
#128398=CARTESIAN_POINT('Ctrl Pts',(3.64079886599986,4.01609134930843,-6.46144698653662));
#128399=CARTESIAN_POINT('Ctrl Pts',(3.60012817905465,4.02919780807987,-6.3887276820716));
#128400=CARTESIAN_POINT('Ctrl Pts',(3.57977682462897,4.03591692852018,-6.35237772768086));
#128401=CARTESIAN_POINT('Ctrl Pts',(3.55943399940581,4.04280735924911,-6.31608499035852));
#128402=CARTESIAN_POINT('Ctrl Pts',(4.21789784,3.913265985,-5.896765029));
#128403=CARTESIAN_POINT('Ctrl Pts',(3.898057804,3.978309763,-6.125543451));
#128404=CARTESIAN_POINT('Ctrl Pts',(3.55534912,4.043585554,-6.318385287));
#128405=CARTESIAN_POINT('Ctrl Pts',(4.160940096,3.913265985,-6.23991807));
#128406=CARTESIAN_POINT('Ctrl Pts',(3.822487468,3.978309763,-6.465607109));
#128407=CARTESIAN_POINT('Ctrl Pts',(3.461609539,4.043585554,-6.653364517));
#128408=CARTESIAN_POINT('Origin',(-0.101467299579598,4.01785693399817,0.17163723126743));
#128409=CARTESIAN_POINT('Ctrl Pts',(4.837531582,4.043593265,-5.400072981));
#128410=CARTESIAN_POINT('Ctrl Pts',(4.541336538,3.977881214,-5.66541252));
#128411=CARTESIAN_POINT('Ctrl Pts',(4.21789784,3.913265985,-5.896765029));
#128412=CARTESIAN_POINT('Ctrl Pts',(4.20670398840656,3.91102972419208,-5.90477188058432));
#128413=CARTESIAN_POINT('Ctrl Pts',(4.19551013681311,3.90879346338417,-5.91277873216877));
#128414=CARTESIAN_POINT('Ctrl Pts',(5.18558480998941,4.043593265,-5.41919799617495));
#128415=CARTESIAN_POINT('Ctrl Pts',(4.8883407551324,3.977881214,-5.703628322637));
#128416=CARTESIAN_POINT('Ctrl Pts',(4.56177135477598,3.913265985,-5.95384235976156));
#128417=CARTESIAN_POINT('Ctrl Pts',(4.55046915307545,3.91102972419208,-5.96250198773891));
#128418=CARTESIAN_POINT('Ctrl Pts',(4.53916695137504,3.90879346338417,-5.9711616157164));
#128419=CARTESIAN_POINT('',(4.83398797799277,4.04280735943435,-5.40324534134335));
#128420=CARTESIAN_POINT('Origin',(-0.142473359438421,4.16060420788965,0.129936838326903));
#128421=CARTESIAN_POINT('Ctrl Pts',(5.00007512009465,4.0034549415684,-5.5901027533489));
#128422=CARTESIAN_POINT('Ctrl Pts',(4.97239382994866,4.00969641603501,-5.55890493168669));
#128423=CARTESIAN_POINT('Ctrl Pts',(4.9446991148708,4.01609134930492,-5.52771781147437));
#128424=CARTESIAN_POINT('Ctrl Pts',(4.88934677262722,4.02919781104827,-5.46544162554518));
#128425=CARTESIAN_POINT('Ctrl Pts',(4.8616570626464,4.03591692995295,-5.43431646029451));
#128426=CARTESIAN_POINT('Ctrl Pts',(4.83398798131907,4.0428073592582,-5.40324533969528));
#128427=CARTESIAN_POINT('Ctrl Pts',(5.386915907,3.913265985,-4.852178584));
#128428=CARTESIAN_POINT('Ctrl Pts',(5.123734151,3.978309763,-5.14436444699999));
#128429=CARTESIAN_POINT('Ctrl Pts',(4.8304931,4.043585554,-5.406369984));
#128430=CARTESIAN_POINT('Ctrl Pts',(5.405057563,3.913265985,-5.199553129));
#128431=CARTESIAN_POINT('Ctrl Pts',(5.123034241,3.978309763,-5.492722994));
#128432=CARTESIAN_POINT('Ctrl Pts',(4.810955731,4.043585554,-5.753668826));
#128433=CARTESIAN_POINT('Origin',(-0.135991943969817,4.01785695574899,0.145811955776194));
#128434=CARTESIAN_POINT('Ctrl Pts',(5.885288847,4.043593265,-4.233895981));
#128435=CARTESIAN_POINT('Ctrl Pts',(5.65305883699999,3.977881214,-4.556705209));
#128436=CARTESIAN_POINT('Ctrl Pts',(5.386915907,3.913265985,-4.852178584));
#128437=CARTESIAN_POINT('Ctrl Pts',(5.37770499780094,3.91102972417881,-4.8624045871024));
#128438=CARTESIAN_POINT('Ctrl Pts',(5.36849408860187,3.90879346335763,-4.87263059020483));
#128439=CARTESIAN_POINT('Ctrl Pts',(6.22931609688157,4.043593265,-4.177752709251));
#128440=CARTESIAN_POINT('Ctrl Pts',(6.00016555589542,3.977881214,-4.51943189804367));
#128441=CARTESIAN_POINT('Ctrl Pts',(5.73501978812069,3.913265985,-4.83399883832596));
#128442=CARTESIAN_POINT('Ctrl Pts',(5.72584338959121,3.91102972417881,-4.84488564837186));
#128443=CARTESIAN_POINT('Ctrl Pts',(5.71666699106165,3.90879346335762,-4.8557724584176));
#128444=CARTESIAN_POINT('',(5.88251005481746,4.04280735943236,-4.23775594359663));
#128445=CARTESIAN_POINT('Origin',(-0.1670748624342,4.16060423972647,0.0962713050176661));
#128446=CARTESIAN_POINT('Ctrl Pts',(6.08488299206126,4.00345494165232,-4.38454090746794));
#128447=CARTESIAN_POINT('Ctrl Pts',(6.05114226559023,4.00969641611188,-4.36002313261344));
#128448=CARTESIAN_POINT('Ctrl Pts',(6.0173907288278,4.01609134931989,-4.33551869516663));
#128449=CARTESIAN_POINT('Ctrl Pts',(5.94994497316006,4.02919780739118,-4.28659762264593));
#128450=CARTESIAN_POINT('Ctrl Pts',(5.91621163238369,4.03591692819812,-4.26215260797922));
#128451=CARTESIAN_POINT('Ctrl Pts',(5.88251005761056,4.04280735926177,-4.2377559410218));
#128452=CARTESIAN_POINT('Ctrl Pts',(6.304047773,3.913265985,-3.580709661));
#128453=CARTESIAN_POINT('Ctrl Pts',(6.109830384,3.978309763,-3.922640679));
#128454=CARTESIAN_POINT('Ctrl Pts',(5.879768591,4.043585554,-4.24155883));
#128455=CARTESIAN_POINT('Ctrl Pts',(6.396440546,3.913265985,-3.916062862));
#128456=CARTESIAN_POINT('Ctrl Pts',(6.184033628,3.978309763,-4.263005256));
#128457=CARTESIAN_POINT('Ctrl Pts',(5.93534698,4.043585554,-4.584937975));
#128458=CARTESIAN_POINT('Origin',(-0.164157702665602,4.01785694770381,0.113168649877501));
#128459=CARTESIAN_POINT('Ctrl Pts',(6.657856548,4.043593265,-2.869746712));
#128460=CARTESIAN_POINT('Ctrl Pts',(6.500450388,3.977881214,-3.234931426));
#128461=CARTESIAN_POINT('Ctrl Pts',(6.304047773,3.913265985,-3.580709661));
#128462=CARTESIAN_POINT('Ctrl Pts',(6.297250498457,3.91102972429048,-3.59267665845715));
#128463=CARTESIAN_POINT('Ctrl Pts',(6.29045322391415,3.90879346358098,-3.60464365591426));
#128464=CARTESIAN_POINT('Ctrl Pts',(6.98177148812167,4.043593265,-2.74096034957502));
#128465=CARTESIAN_POINT('Ctrl Pts',(6.83142928431638,3.977881214,-3.12391186004807));
#128466=CARTESIAN_POINT('Ctrl Pts',(6.64010507143617,3.913265985,-3.48812290292875));
#128467=CARTESIAN_POINT('Ctrl Pts',(6.63348355470297,3.91102972429048,-3.50072783922272));
#128468=CARTESIAN_POINT('Ctrl Pts',(6.62686203796978,3.90879346358098,-3.5133327755167));
#128469=CARTESIAN_POINT('',(6.65597249944044,4.04280735944133,-2.87411378903347));
#128470=CARTESIAN_POINT('Origin',(-0.18386436534236,4.16060427247911,0.0581044355760535));
#128471=CARTESIAN_POINT('Ctrl Pts',(6.88516849829515,4.0034549415845,-2.97396280252883));
#128472=CARTESIAN_POINT('Ctrl Pts',(6.84694601453568,4.00969641602047,-2.95727149861208));
#128473=CARTESIAN_POINT('Ctrl Pts',(6.80871583992959,4.01609134928458,-2.94059554396096));
#128474=CARTESIAN_POINT('Ctrl Pts',(6.73233034632253,4.02919780699493,-2.90731706378765));
#128475=CARTESIAN_POINT('Ctrl Pts',(6.69413071574023,4.03591692798957,-2.89069523065496));
#128476=CARTESIAN_POINT('Ctrl Pts',(6.65597250201484,4.042807359239,-2.87411378614891));
#128477=CARTESIAN_POINT('Ctrl Pts',(6.92640937100001,3.913265985,-2.141810735));
#128478=CARTESIAN_POINT('Ctrl Pts',(6.810237738,3.978309763,-2.517498593));
#128479=CARTESIAN_POINT('Ctrl Pts',(6.654112638,4.043585554,-2.8784171));
#128480=CARTESIAN_POINT('Ctrl Pts',(7.088733078,3.913265985,-2.449461849));
#128481=CARTESIAN_POINT('Ctrl Pts',(6.955874475,3.978309763,-2.833954131));
#128482=CARTESIAN_POINT('Ctrl Pts',(6.782208,4.043585554,-3.20182052));
#128483=CARTESIAN_POINT('Origin',(-0.184647872090897,4.01785694219713,0.0752338312692788));
#128484=CARTESIAN_POINT('Ctrl Pts',(7.119110275,4.043593265,-1.371411276));
#128485=CARTESIAN_POINT('Ctrl Pts',(7.043888103,3.977881214,-1.761895846));
#128486=CARTESIAN_POINT('Ctrl Pts',(6.926409371,3.913265985,-2.141810735));
#128487=CARTESIAN_POINT('Ctrl Pts',(6.92234356355036,3.91102972423215,-2.15495916416351));
#128488=CARTESIAN_POINT('Ctrl Pts',(6.91827775610086,3.90879346346433,-2.16810759332702));
#128489=CARTESIAN_POINT('Ctrl Pts',(7.40776700316154,4.043593265,-1.1760037288039));
#128490=CARTESIAN_POINT('Ctrl Pts',(7.3432629714967,3.977881214,-1.58232117638743));
#128491=CARTESIAN_POINT('Ctrl Pts',(7.23470641998915,3.913265985,-1.9791462180463));
#128492=CARTESIAN_POINT('Ctrl Pts',(7.23094939922197,3.91102972423215,-1.99287988866998));
#128493=CARTESIAN_POINT('Ctrl Pts',(7.22719237845479,3.90879346346432,-2.00661355929366));
#128494=CARTESIAN_POINT('',(7.11820906756662,4.0428073594531,-1.37608126740113));
#128495=CARTESIAN_POINT('Origin',(-0.192056303862034,4.16060420929109,0.0172205636934611));
#128496=CARTESIAN_POINT('Ctrl Pts',(7.36351117761108,4.00345494157173,-1.42432550160411));
#128497=CARTESIAN_POINT('Ctrl Pts',(7.32259417719401,4.00969641604598,-1.4162411351845));
#128498=CARTESIAN_POINT('Ctrl Pts',(7.28167296572909,4.01609134929106,-1.40817341256506));
#128499=CARTESIAN_POINT('Ctrl Pts',(7.19991942750863,4.02919780789818,-1.39209358688646));
#128500=CARTESIAN_POINT('Ctrl Pts',(7.15903968301819,4.03591692847851,-1.384072154959));
#128501=CARTESIAN_POINT('Ctrl Pts',(7.11820906898563,4.04280735933872,-1.37608126395451));
#128502=CARTESIAN_POINT('Ctrl Pts',(7.224899766,3.913265985,-0.602763118));
#128503=CARTESIAN_POINT('Ctrl Pts',(7.192205945,3.978309763,-0.99464107));
#128504=CARTESIAN_POINT('Ctrl Pts',(7.117317773,4.043585554,-1.380683784));
#128505=CARTESIAN_POINT('Ctrl Pts',(7.44956433,3.913265985,-0.868326722));
#128506=CARTESIAN_POINT('Ctrl Pts',(7.402466362,3.978309763,-1.272390461));
#128507=CARTESIAN_POINT('Ctrl Pts',(7.311940513,4.043585554,-1.668989496));
#128508=CARTESIAN_POINT('Origin',(-0.196503946990214,4.0178569579,0.0337810818113829));
#128509=CARTESIAN_POINT('Ctrl Pts',(7.247482319,4.043593265,0.191049828));
#128510=CARTESIAN_POINT('Ctrl Pts',(7.257961439,3.977881214,-0.206475974));
#128511=CARTESIAN_POINT('Ctrl Pts',(7.224899766,3.913265985,-0.602763118));
#128512=CARTESIAN_POINT('Ctrl Pts',(7.22439618107746,3.91228178631499,-0.608799238153792));
#128513=CARTESIAN_POINT('Ctrl Pts',(7.22389259615494,3.91129758763,-0.614835358307581));
#128514=CARTESIAN_POINT('Ctrl Pts',(7.4871021457591,4.043593265,0.443644859291128));
#128515=CARTESIAN_POINT('Ctrl Pts',(7.51143615240166,3.977881214,0.0329758636738649));
#128516=CARTESIAN_POINT('Ctrl Pts',(7.49070876024168,3.913265985,-0.377890955083214));
#128517=CARTESIAN_POINT('Ctrl Pts',(7.49039304717491,3.91228178631499,-0.384149148221127));
#128518=CARTESIAN_POINT('Ctrl Pts',(7.49007733410815,3.91129758763,-0.390407341359038));
#128519=CARTESIAN_POINT('',(7.24760609127573,4.04280735946006,0.186295284467327));
#128520=CARTESIAN_POINT('Origin',(-0.191268234115439,4.1606042421385,-0.0244684761355934));
#128521=CARTESIAN_POINT('Ctrl Pts',(7.49754425842133,4.00345494160375,0.191911676403569));
#128522=CARTESIAN_POINT('Ctrl Pts',(7.45584597507905,4.00969641604305,0.191011089299511));
#128523=CARTESIAN_POINT('Ctrl Pts',(7.41414715678095,4.01609134929557,0.190093342264412));
#128524=CARTESIAN_POINT('Ctrl Pts',(7.33084828706427,4.0291978073406,0.188222636638881));
#128525=CARTESIAN_POINT('Ctrl Pts',(7.28919991587735,4.03591692815706,0.187268595286477));
#128526=CARTESIAN_POINT('Ctrl Pts',(7.247606092197,4.0428073592334,0.186295288614052));
#128527=CARTESIAN_POINT('Ctrl Pts',(7.185561877,3.913265985,0.964469032));
#128528=CARTESIAN_POINT('Ctrl Pts',(7.237874596,3.978309763,0.574724763));
#128529=CARTESIAN_POINT('Ctrl Pts',(7.24772504,4.043585554,0.18160877));
#128530=CARTESIAN_POINT('Ctrl Pts',(7.462062233,3.913265985,0.753410398));
#128531=CARTESIAN_POINT('Ctrl Pts',(7.50292714899999,3.978309763,0.348668774));
#128532=CARTESIAN_POINT('Ctrl Pts',(7.49977481399999,4.043585554,-0.058118378));
#128533=CARTESIAN_POINT('Origin',(-0.199171610314072,4.01785698284914,-0.00925123469850048));
#128534=CARTESIAN_POINT('Ctrl Pts',(7.036970144,4.043593265,1.744577653));
#128535=CARTESIAN_POINT('Ctrl Pts',(7.132660565,3.977881214,1.358598485));
#128536=CARTESIAN_POINT('Ctrl Pts',(7.185561877,3.913265985,0.964469032));
#128537=CARTESIAN_POINT('Ctrl Pts',(7.18739273225864,3.91102972417149,0.950828652313265));
#128538=CARTESIAN_POINT('Ctrl Pts',(7.18922358751719,3.90879346334299,0.937188272626531));
#128539=CARTESIAN_POINT('Ctrl Pts',(7.2168983954371,4.043593265,2.04312855315919));
#128540=CARTESIAN_POINT('Ctrl Pts',(7.32896439106459,3.977881214,1.64728028570918));
#128541=CARTESIAN_POINT('Ctrl Pts',(7.39706364334686,3.913265985,1.24154991981403));
#128542=CARTESIAN_POINT('Ctrl Pts',(7.39942048232563,3.91102972417149,1.22750804550314));
#128543=CARTESIAN_POINT('Ctrl Pts',(7.40177732130451,3.90879346334299,1.21346617119224));
#128544=CARTESIAN_POINT('',(7.03811310896934,4.04280735943817,1.73996087631982));
#128545=CARTESIAN_POINT('Origin',(-0.181536210942169,4.16060424174822,-0.065013380066494));
#128546=CARTESIAN_POINT('Ctrl Pts',(7.28100050240532,4.00345494164967,1.79917527769442));
#128547=CARTESIAN_POINT('Ctrl Pts',(7.24047070142337,4.00969641607446,1.78933184746784));
#128548=CARTESIAN_POINT('Ctrl Pts',(7.19994406678762,4.0160913493275,1.77947154348191));
#128549=CARTESIAN_POINT('Ctrl Pts',(7.11899482593457,4.02919780717941,1.75973777943903));
#128550=CARTESIAN_POINT('Ctrl Pts',(7.07852526065663,4.03591692808004,1.74985287418798));
#128551=CARTESIAN_POINT('Ctrl Pts',(7.03811310915023,4.04280735923492,1.73996088015336));
#128552=CARTESIAN_POINT('Ctrl Pts',(6.81023510100001,3.913265985,2.486603681));
#128553=CARTESIAN_POINT('Ctrl Pts',(6.945108274,3.978309763,2.117217106));
#128554=CARTESIAN_POINT('Ctrl Pts',(7.039236739,4.043585554,1.7354095));
#128555=CARTESIAN_POINT('Ctrl Pts',(7.12564240000001,3.913265985,2.339918885));
#128556=CARTESIAN_POINT('Ctrl Pts',(7.252559402,3.978309763,1.953424644));
#128557=CARTESIAN_POINT('Ctrl Pts',(7.336927979,4.043585554,1.555470291));
#128558=CARTESIAN_POINT('Origin',(-0.192526489986816,4.01785691537832,-0.0518510129485522));
#128559=CARTESIAN_POINT('Ctrl Pts',(6.497417067,4.043593265,3.216530967));
#128560=CARTESIAN_POINT('Ctrl Pts',(6.67384440999999,3.977881214,2.860146389));
#128561=CARTESIAN_POINT('Ctrl Pts',(6.810235101,3.913265985,2.486603681));
#128562=CARTESIAN_POINT('Ctrl Pts',(6.81495543020653,3.91102972422297,2.47367578583701));
#128563=CARTESIAN_POINT('Ctrl Pts',(6.81967575941306,3.90879346344597,2.46074789067403));
#128564=CARTESIAN_POINT('Ctrl Pts',(6.60895907756968,4.043593265,3.54678116859732));
#128565=CARTESIAN_POINT('Ctrl Pts',(6.80350070809697,3.977881214,3.18427848912944));
#128566=CARTESIAN_POINT('Ctrl Pts',(6.95722787297176,3.913265985,2.80267320064579));
#128567=CARTESIAN_POINT('Ctrl Pts',(6.96254819814112,3.91102972422297,2.78946626859357));
#128568=CARTESIAN_POINT('Ctrl Pts',(6.96786852331048,3.90879346344595,2.77625933654135));
#128569=CARTESIAN_POINT('',(6.49952578032111,4.04280735945842,3.21226783088978));
#128570=CARTESIAN_POINT('Origin',(-0.163316158576928,4.16060424653016,-0.102518366934566));
#128571=CARTESIAN_POINT('Ctrl Pts',(6.72400525554583,4.0034549416088,3.32231144235511));
#128572=CARTESIAN_POINT('Ctrl Pts',(6.68653913777703,4.00969640396818,3.30398547236695));
#128573=CARTESIAN_POINT('Ctrl Pts',(6.64907962791028,4.01609134349056,3.28564364915466));
#128574=CARTESIAN_POINT('Ctrl Pts',(6.57426505880515,4.02919781055076,3.24896952995097));
#128575=CARTESIAN_POINT('Ctrl Pts',(6.53686662234059,4.03591692971601,3.23061597316373));
#128576=CARTESIAN_POINT('Ctrl Pts',(6.49952577957866,4.04280735926632,3.21226783479966));
#128577=CARTESIAN_POINT('Ctrl Pts',(6.116469301,3.913265985,3.892467507));
#128578=CARTESIAN_POINT('Ctrl Pts',(6.32759640899999,3.978309763,3.560710729));
#128579=CARTESIAN_POINT('Ctrl Pts',(6.501601551,4.043585554,3.208064411));
#128580=CARTESIAN_POINT('Ctrl Pts',(6.456035448,3.913265985,3.817015365));
#128581=CARTESIAN_POINT('Ctrl Pts',(6.663070038,3.978309763,3.466840548));
#128582=CARTESIAN_POINT('Ctrl Pts',(6.831014547,4.043585554,3.096326897));
#128583=CARTESIAN_POINT('Origin',(-0.176878902022397,4.01785697920935,-0.0920262527008903));
#128584=CARTESIAN_POINT('Ctrl Pts',(5.654051988,4.043593265,4.538082868));
#128585=CARTESIAN_POINT('Ctrl Pts',(5.902966708,3.977881214,4.227957027));
#128586=CARTESIAN_POINT('Ctrl Pts',(6.116469301,3.913265985,3.892467507));
#128587=CARTESIAN_POINT('Ctrl Pts',(6.12385838672874,3.9110297242607,3.88085659029149));
#128588=CARTESIAN_POINT('Ctrl Pts',(6.13124747245758,3.90879346352142,3.86924567358297));
#128589=CARTESIAN_POINT('Ctrl Pts',(5.69199217717727,4.043593265,4.88459023813079));
#128590=CARTESIAN_POINT('Ctrl Pts',(5.95991289298509,3.977881214,4.57238337002353));
#128591=CARTESIAN_POINT('Ctrl Pts',(6.19207986003697,3.913265985,4.23274659681963));
#128592=CARTESIAN_POINT('Ctrl Pts',(6.20011489885699,3.9110297242607,4.22099214832055));
#128593=CARTESIAN_POINT('Ctrl Pts',(6.20814993767701,3.90879346352142,4.20923769982152));
#128594=CARTESIAN_POINT('',(5.65702784913764,4.04280735944397,4.53437271253314));
#128595=CARTESIAN_POINT('Origin',(-0.137459569024259,4.16060421429331,-0.135229751280873));
#128596=CARTESIAN_POINT('Ctrl Pts',(5.85260299563805,4.00345494155613,4.69010001717245));
#128597=CARTESIAN_POINT('Ctrl Pts',(5.81995229347557,4.00969641600747,4.66414834014744));
#128598=CARTESIAN_POINT('Ctrl Pts',(5.7873115502117,4.01609134926909,4.63818267851389));
#128599=CARTESIAN_POINT('Ctrl Pts',(5.72213000906131,4.02919780559788,4.58628310167405));
#128600=CARTESIAN_POINT('Ctrl Pts',(5.68955138599866,4.03591692734122,4.5603190719445));
#128601=CARTESIAN_POINT('Ctrl Pts',(5.65702784741048,4.04280735928509,4.53437271658464));
#128602=CARTESIAN_POINT('Ctrl Pts',(5.136704194,3.913265985,5.11632387800001));
#128603=CARTESIAN_POINT('Ctrl Pts',(5.414213168,3.978309763,4.837709477));
#128604=CARTESIAN_POINT('Ctrl Pts',(5.659958701,4.043585554,4.530713796));
#128605=CARTESIAN_POINT('Ctrl Pts',(5.484551453,3.913265985,5.115632449));
#128606=CARTESIAN_POINT('Ctrl Pts',(5.762022925,3.978309763,4.818150842));
#128607=CARTESIAN_POINT('Ctrl Pts',(6.005690467,4.043585554,4.492402699));
#128608=CARTESIAN_POINT('Origin',(-0.152960641359825,4.0178569617403,-0.127898470072109));
#128609=CARTESIAN_POINT('Ctrl Pts',(4.546309723,4.043593265,5.647439057));
#128610=CARTESIAN_POINT('Ctrl Pts',(4.856072844,3.977881214,5.39807309299999));
#128611=CARTESIAN_POINT('Ctrl Pts',(5.136704194,3.913265985,5.116323878));
#128612=CARTESIAN_POINT('Ctrl Pts',(5.1464165311493,3.91102972419369,5.10657285279335));
#128613=CARTESIAN_POINT('Ctrl Pts',(5.15612886829848,3.9087934633874,5.0968218275867));
#128614=CARTESIAN_POINT('Ctrl Pts',(4.50887404986768,4.043593265,5.99400129611241));
#128615=CARTESIAN_POINT('Ctrl Pts',(4.83764617598171,3.977881214,5.74668868624019));
#128616=CARTESIAN_POINT('Ctrl Pts',(5.13739707470347,3.913265985,5.46490146661399));
#128617=CARTESIAN_POINT('Ctrl Pts',(5.14777111804963,3.91102972419369,5.45514912610975));
#128618=CARTESIAN_POINT('Ctrl Pts',(5.15814516139567,3.9087934633874,5.4453967856054));
#128619=CARTESIAN_POINT('',(4.5500135837177,4.0428073594318,5.64445536550249));
#128620=CARTESIAN_POINT('Origin',(-0.105175429544502,4.16060423354011,-0.161617879588788));
#128621=CARTESIAN_POINT('Ctrl Pts',(4.70753952467976,4.00345494161455,5.83858472753934));
#128622=CARTESIAN_POINT('Ctrl Pts',(4.68123102122189,4.0096964160736,5.80622085031341));
#128623=CARTESIAN_POINT('Ctrl Pts',(4.65493525026559,4.01609134930381,5.7738454564778));
#128624=CARTESIAN_POINT('Ctrl Pts',(4.60243447779962,4.02919780923709,5.70914714015498));
#128625=CARTESIAN_POINT('Ctrl Pts',(4.57619903173416,4.03591692907489,5.67678670369158));
#128626=CARTESIAN_POINT('Ctrl Pts',(4.55001358156977,4.04280735924305,5.64445536838016));
#128627=CARTESIAN_POINT('Ctrl Pts',(3.916752508,3.913265985,6.100946631));
#128628=CARTESIAN_POINT('Ctrl Pts',(4.247667337,3.978309763,5.88850230599999));
#128629=CARTESIAN_POINT('Ctrl Pts',(4.553662473,4.043585554,5.641512038));
#128630=CARTESIAN_POINT('Ctrl Pts',(4.256615929,3.913265985,6.175048246));
#128631=CARTESIAN_POINT('Ctrl Pts',(4.591550023,3.978309763,5.944169758));
#128632=CARTESIAN_POINT('Ctrl Pts',(4.899546976,4.043585554,5.678418744));
#128633=CARTESIAN_POINT('Origin',(-0.121890082464141,4.01785694597163,-0.15779024085729));
#128634=CARTESIAN_POINT('Ctrl Pts',(3.225987068,4.043593265,6.492727273));
#128635=CARTESIAN_POINT('Ctrl Pts',(3.58211441,3.977881214,6.31578126));
#128636=CARTESIAN_POINT('Ctrl Pts',(3.916752508,3.913265985,6.100946631));
#128637=CARTESIAN_POINT('Ctrl Pts',(3.92833395842363,3.91102972416853,6.09351144469005));
#128638=CARTESIAN_POINT('Ctrl Pts',(3.93991540884725,3.90879346333707,6.08607625837996));
#128639=CARTESIAN_POINT('Ctrl Pts',(3.114925983046,4.043593265,6.82313951611881));
#128640=CARTESIAN_POINT('Ctrl Pts',(3.4891765001953,3.977881214,6.65228522632004));
#128641=CARTESIAN_POINT('Ctrl Pts',(3.84249531148228,3.913265985,6.44152361799445));
#128642=CARTESIAN_POINT('Ctrl Pts',(3.85472328050648,3.91102972416852,6.43422939437612));
#128643=CARTESIAN_POINT('Ctrl Pts',(3.86695124953061,3.90879346333707,6.42693517075777));
#128644=CARTESIAN_POINT('',(3.23024573998459,4.04280735943644,6.49060955893343));
#128645=CARTESIAN_POINT('Origin',(-0.0679733892149625,4.16060421634694,
-0.180448891774344));
#128646=CARTESIAN_POINT('Ctrl Pts',(3.34235673751932,4.00345494162258,6.71406370518684));
#128647=CARTESIAN_POINT('Ctrl Pts',(3.32362058915715,4.00969641608109,6.67680092687676));
#128648=CARTESIAN_POINT('Ctrl Pts',(3.30489935139104,4.01609134929957,6.6395296383611));
#128649=CARTESIAN_POINT('Ctrl Pts',(3.26753424118094,4.02919781000407,6.56505781410496));
#128650=CARTESIAN_POINT('Ctrl Pts',(3.24886870383412,4.03591692942377,6.52781410369642));
#128651=CARTESIAN_POINT('Ctrl Pts',(3.23024573750669,4.04280735919962,6.49060956132151));
#128652=CARTESIAN_POINT('Ctrl Pts',(2.513657828,3.913265985,6.8002959));
#128653=CARTESIAN_POINT('Ctrl Pts',(2.882505303,3.978309763,6.663955312));
#128654=CARTESIAN_POINT('Ctrl Pts',(3.234442049,4.043585554,6.488519448));
#128655=CARTESIAN_POINT('Ctrl Pts',(2.829645774,3.913265985,6.945725649));
#128656=CARTESIAN_POINT('Ctrl Pts',(3.206381346,3.978309763,6.792245902));
#128657=CARTESIAN_POINT('Ctrl Pts',(3.564306113,4.043585554,6.59891824));
#128658=CARTESIAN_POINT('Origin',(-0.0851200586046991,4.0178569676344,-0.180303803708096));
#128659=CARTESIAN_POINT('Ctrl Pts',(1.754820843,4.043593265,7.034422777));
#128660=CARTESIAN_POINT('Ctrl Pts',(2.140660288,3.977881214,6.938170516));
#128661=CARTESIAN_POINT('Ctrl Pts',(2.513657828,3.913265985,6.8002959));
#128662=CARTESIAN_POINT('Ctrl Pts',(2.52656685588248,3.91102972415818,6.79552421367136));
#128663=CARTESIAN_POINT('Ctrl Pts',(2.53947588376501,3.90879346331638,6.79075252734283));
#128664=CARTESIAN_POINT('Ctrl Pts',(1.5753274386396,4.043593265,7.33323531634172));
#128665=CARTESIAN_POINT('Ctrl Pts',(1.97755680933523,3.977881214,7.24682830281787));
#128666=CARTESIAN_POINT('Ctrl Pts',(2.36792273908028,3.913265985,7.11694728376972));
#128667=CARTESIAN_POINT('Ctrl Pts',(2.38143286751558,3.91102972415818,7.1124522468955));
#128668=CARTESIAN_POINT('Ctrl Pts',(2.39494299595088,3.90879346331638,7.10795721002117));
#128669=CARTESIAN_POINT('',(1.75943519548214,4.04280735942786,7.03327006341456));
#128670=CARTESIAN_POINT('Origin',(-0.0275930671524408,4.16060426191353,
-0.190842484786877));
#128671=CARTESIAN_POINT('Ctrl Pts',(1.82088906445054,4.00345494158803,7.27560052582954));
#128672=CARTESIAN_POINT('Ctrl Pts',(1.81060137241643,4.00969640404014,7.23518129027532));
#128673=CARTESIAN_POINT('Ctrl Pts',(1.80033004124381,4.01609134347794,7.19475682903795));
#128674=CARTESIAN_POINT('Ctrl Pts',(1.77984774251408,4.02919780709716,7.11399370280583));
#128675=CARTESIAN_POINT('Ctrl Pts',(1.76962488919475,4.03591692801806,7.07360818143289));
#128676=CARTESIAN_POINT('Ctrl Pts',(1.75943519192525,4.04280735920122,7.03327006541419));
#128677=CARTESIAN_POINT('Ctrl Pts',(0.993027302,3.913265985,7.18167089));
#128678=CARTESIAN_POINT('Ctrl Pts',(1.382560524,3.978309763,7.127809173));
#128679=CARTESIAN_POINT('Ctrl Pts',(1.763982709,4.043585554,7.032130901));
#128680=CARTESIAN_POINT('Ctrl Pts',(1.270364528,3.913265985,7.391628641));
#128681=CARTESIAN_POINT('Ctrl Pts',(1.67128584,3.978309763,7.322724176));
#128682=CARTESIAN_POINT('Ctrl Pts',(2.062402258,4.043585554,7.210859652));
#128683=CARTESIAN_POINT('Origin',(-0.0443700637133654,4.01785698804151,
-0.194387020948577));
#128684=CARTESIAN_POINT('Ctrl Pts',(0.201601146,4.043593265,7.247196491));
#128685=CARTESIAN_POINT('Ctrl Pts',(0.59911127,3.977881214,7.236138629));
#128686=CARTESIAN_POINT('Ctrl Pts',(0.993027301999999,3.913265985,7.18167089));
#128687=CARTESIAN_POINT('Ctrl Pts',(1.0066602952472,3.91102972420058,7.17978582247885));
#128688=CARTESIAN_POINT('Ctrl Pts',(1.02029328849439,3.90879346340122,7.17790075495781));
#128689=CARTESIAN_POINT('Ctrl Pts',(-0.0379316651698515,4.043593265,7.50043718252154));
#128690=CARTESIAN_POINT('Ctrl Pts',(0.373468759383329,3.977881214,7.50251774175908));
#128691=CARTESIAN_POINT('Ctrl Pts',(0.78262873003964,3.913265985,7.45959040487349));
#128692=CARTESIAN_POINT('Ctrl Pts',(0.796789298952412,3.91102972420058,
7.45810473776085));
#128693=CARTESIAN_POINT('Ctrl Pts',(0.810949867865185,3.90879346340121,
7.45661907064821));
#128694=CARTESIAN_POINT('',(0.20635541671928,4.04280735947359,7.24706267597459));
#128695=CARTESIAN_POINT('Origin',(0.0140775383825686,4.16060426862506,-0.192312383134926));
#128696=CARTESIAN_POINT('Ctrl Pts',(0.214278641765392,4.00345494161275,
7.4969383524598));
#128697=CARTESIAN_POINT('Ctrl Pts',(0.21292040859655,4.00969641605623,7.45525246640273));
#128698=CARTESIAN_POINT('Ctrl Pts',(0.211579281215642,4.01609134932557,
7.41356511708819));
#128699=CARTESIAN_POINT('Ctrl Pts',(0.208937532970993,4.02919780991452,
7.3302871182516));
#128700=CARTESIAN_POINT('Ctrl Pts',(0.20763537809521,4.03591692941635,7.28864818600079));
#128701=CARTESIAN_POINT('Ctrl Pts',(0.206355413357484,4.04280735927498,
7.24706267686669));
#128702=CARTESIAN_POINT('Ctrl Pts',(-0.574036077,3.913265985,7.227238932));
#128703=CARTESIAN_POINT('Ctrl Pts',(-0.182031249,3.978309763,7.2583746));
#128704=CARTESIAN_POINT('Ctrl Pts',(0.211041498,4.043585554,7.246927727));
#128705=CARTESIAN_POINT('Ctrl Pts',(-0.348317552,3.913265985,7.491907293));
#128706=CARTESIAN_POINT('Ctrl Pts',(0.0580428659999999,3.978309763,7.510800007));
#128707=CARTESIAN_POINT('Ctrl Pts',(0.464062765,4.043585554,7.485629282));
#128708=CARTESIAN_POINT('Origin',(-0.00154526844133959,4.01785679159005,
-0.199381631082065));
#128709=CARTESIAN_POINT('Ctrl Pts',(0.201420355,1.975104983,7.247201518));
#128710=CARTESIAN_POINT('Ctrl Pts',(0.597450238,1.909367073,7.23619472));
#128711=CARTESIAN_POINT('Ctrl Pts',(0.989922563999999,1.844275173,7.182099506));
#128712=CARTESIAN_POINT('Ctrl Pts',(0.993831803810694,1.84362682194445,
7.18156068797354));
#128713=CARTESIAN_POINT('Ctrl Pts',(0.997741043621388,1.84297847088892,
7.18102186994708));
#128714=CARTESIAN_POINT('Ctrl Pts',(-0.037616899,1.975104983,7.49990566400001));
#128715=CARTESIAN_POINT('Ctrl Pts',(0.372222232,1.909367073,7.501961273));
#128716=CARTESIAN_POINT('Ctrl Pts',(0.77984494,1.844275173,7.459345941));
#128717=CARTESIAN_POINT('Ctrl Pts',(0.783905085932064,1.84362682194446,
7.45892146890002));
#128718=CARTESIAN_POINT('Ctrl Pts',(0.787965231864127,1.84297847088891,
7.45849699680004));
#128719=CARTESIAN_POINT('',(0.213157852172123,1.93490816642933,7.49697023463349));
#128720=CARTESIAN_POINT('',(0.779844939665357,1.84427517280771,7.459345940031));
#128721=CARTESIAN_POINT('Origin',(0.00791499441159103,2.01782137169043,
-0.189678174975023));
#128722=CARTESIAN_POINT('',(0.884883748724035,1.84427517246151,7.32072272389598));
#128723=CARTESIAN_POINT('Ctrl Pts',(0.213157850962533,1.9349081733935,7.49697023571379));
#128724=CARTESIAN_POINT('Ctrl Pts',(0.211950237202354,1.94116543724157,
7.45528053998422));
#128725=CARTESIAN_POINT('Ctrl Pts',(0.210760567417153,1.94757342722814,
7.41358973092107));
#128726=CARTESIAN_POINT('Ctrl Pts',(0.208423369809919,1.96070006887751,
7.33030278216503));
#128727=CARTESIAN_POINT('Ctrl Pts',(0.20727451674072,1.967426141464,7.28865951924096));
#128728=CARTESIAN_POINT('Ctrl Pts',(0.206148889166361,1.97432008375446,
7.24706856084113));
#128729=CARTESIAN_POINT('Ctrl Pts',(0.963002974177823,1.83976484773663,
7.1858098847225));
#128730=CARTESIAN_POINT('Ctrl Pts',(0.976462769088904,1.84202001036834,
7.18395469536125));
#128731=CARTESIAN_POINT('Ctrl Pts',(0.989922564,1.844275173,7.182099506));
#128732=CARTESIAN_POINT('Ctrl Pts',(1.380938204,1.909789088,7.12820507000001));
#128733=CARTESIAN_POINT('Ctrl Pts',(1.763791699,1.975097379,7.032178812));
#128734=CARTESIAN_POINT('Ctrl Pts',(1.24002876832294,1.83976484773663,7.39735947533262));
#128735=CARTESIAN_POINT('Ctrl Pts',(1.25388307164246,1.84202001036834,7.39498364010001));
#128736=CARTESIAN_POINT('Ctrl Pts',(1.26773737496199,1.844275173,7.39260780486741));
#128737=CARTESIAN_POINT('Ctrl Pts',(1.67021373623052,1.909789088,7.32358827372707));
#128738=CARTESIAN_POINT('Ctrl Pts',(2.06281816648083,1.975097379,7.21128209294712));
#128739=CARTESIAN_POINT('',(1.26716903471351,1.8442751723037,7.39217717123405));
#128740=CARTESIAN_POINT('',(1.81980133219834,1.93490816640524,7.2758725994878));
#128741=CARTESIAN_POINT('Origin',(-0.0374597101700138,1.87499929406416,
-0.18934890740966));
#128742=CARTESIAN_POINT('Ctrl Pts',(1.75923475895739,1.97432008480599,7.03332020162639));
#128743=CARTESIAN_POINT('Ctrl Pts',(1.76927489670746,1.9674261427311,7.07369680848882));
#128744=CARTESIAN_POINT('Ctrl Pts',(1.77934896230285,1.96070006933456,7.11411951036083));
#128745=CARTESIAN_POINT('Ctrl Pts',(1.79953573986834,1.94757343428078,7.19495678728885));
#128746=CARTESIAN_POINT('Ctrl Pts',(1.80965987568692,1.94116545127622,7.235417097252));
#128747=CARTESIAN_POINT('Ctrl Pts',(1.81980133128369,1.93490817334207,7.27587260079001));
#128748=CARTESIAN_POINT('',(1.12854578661553,1.84427517216382,7.28713831720777));
#128749=CARTESIAN_POINT('Origin',(4.32271406169971E-13,1.93599222700044,
1.56385321359309E-12));
#128750=CARTESIAN_POINT('',(1.82542260132892,1.75423095989052,7.27446440115187));
#128751=CARTESIAN_POINT('Origin',(-0.00348377670905842,2.01767780014573,
-0.183605604020702));
#128752=CARTESIAN_POINT('',(2.365151478457,1.84427517280771,7.1173069671318));
#128753=CARTESIAN_POINT('Origin',(-0.065213110636855,1.87499309172002,-0.180566992369885));
#128754=CARTESIAN_POINT('Origin',(-0.0330452119085806,2.01782140614763,
-0.186944947047757));
#128755=CARTESIAN_POINT('Ctrl Pts',(1.754645359,1.975104983,7.03446655100001));
#128756=CARTESIAN_POINT('Ctrl Pts',(2.139050148,1.909367073,6.938582368));
#128757=CARTESIAN_POINT('Ctrl Pts',(2.510717817,1.844275173,6.801381922));
#128758=CARTESIAN_POINT('Ctrl Pts',(2.51441983100647,1.84362682194445,6.80001533024304));
#128759=CARTESIAN_POINT('Ctrl Pts',(2.51812184501293,1.84297847088892,6.79864873848607));
#128760=CARTESIAN_POINT('Ctrl Pts',(1.575520586,1.975104983,7.332648559));
#128761=CARTESIAN_POINT('Ctrl Pts',(1.9762198,1.909367073,7.246552811));
#128762=CARTESIAN_POINT('Ctrl Pts',(2.365151479,1.844275173,7.11730696800001));
#128763=CARTESIAN_POINT('Ctrl Pts',(2.36902545202297,1.84362682194445,7.11601960845552));
#128764=CARTESIAN_POINT('Ctrl Pts',(2.37289942504594,1.84297847088892,7.11473224891103));
#128765=CARTESIAN_POINT('',(2.43793464488575,1.84427517246151,6.95934444609096));
#128766=CARTESIAN_POINT('Ctrl Pts',(2.48522521582265,1.83976484806346,6.81079246957085));
#128767=CARTESIAN_POINT('Ctrl Pts',(2.49797151641135,1.84202001053176,6.80608719578537));
#128768=CARTESIAN_POINT('Ctrl Pts',(2.510717817,1.844275173,6.801381922));
#128769=CARTESIAN_POINT('Ctrl Pts',(2.881006018,1.909789088,6.664690703));
#128770=CARTESIAN_POINT('Ctrl Pts',(3.234265804,1.975097379,6.488607301));
#128771=CARTESIAN_POINT('Ctrl Pts',(2.80125120977367,1.83976484806346,6.95784379157643));
#128772=CARTESIAN_POINT('Ctrl Pts',(2.81427087187049,1.84202001053176,6.95254523672656));
#128773=CARTESIAN_POINT('Ctrl Pts',(2.82729053396737,1.844275173,6.94724668187658));
#128774=CARTESIAN_POINT('Ctrl Pts',(3.20552006197391,1.909789088,6.79332026772587));
#128775=CARTESIAN_POINT('Ctrl Pts',(3.56480310984828,1.975097379,6.5992413961445));
#128776=CARTESIAN_POINT('',(2.8266429077416,1.8442751723037,6.94694829259179));
#128777=CARTESIAN_POINT('',(3.3413529234146,1.93490816639311,6.71456324812156));
#128778=CARTESIAN_POINT('Origin',(-0.0772883907455425,1.87499928331842,
-0.176869385909534));
#128779=CARTESIAN_POINT('Ctrl Pts',(3.23006076814399,1.9743200848156,6.49070161308116));
#128780=CARTESIAN_POINT('Ctrl Pts',(3.24854594976339,1.96742614274508,6.52797590452996));
#128781=CARTESIAN_POINT('Ctrl Pts',(3.26707417510478,1.96070006935587,6.5652879197994));
#128782=CARTESIAN_POINT('Ctrl Pts',(3.30416664053432,1.94757342764407,6.63989574361088));
#128783=CARTESIAN_POINT('Ctrl Pts',(3.32275187261112,1.9411654374316,6.6772337690076));
#128784=CARTESIAN_POINT('Ctrl Pts',(3.34135292276299,1.93490817334722,6.71456324961192));
#128785=CARTESIAN_POINT('',(2.66868034532562,1.84427517216382,6.87416508912661));
#128786=CARTESIAN_POINT('Origin',(5.60966204044E-13,1.93599222699961,1.18524981496115E-12));
#128787=CARTESIAN_POINT('',(3.34654004958858,1.75423095987511,6.71197956603296));
#128788=CARTESIAN_POINT('Origin',(-0.0428723253219038,2.01767774273086,
-0.178564540033815));
#128789=CARTESIAN_POINT('',(3.83986616329838,1.84427517280772,6.44247063125013));
#128790=CARTESIAN_POINT('Origin',(-0.102505000051829,1.87499306998262,-0.162326509816113));
#128791=CARTESIAN_POINT('Origin',(-0.0724602198121888,2.01782139366673,
-0.175470450256001));
#128792=CARTESIAN_POINT('Ctrl Pts',(3.225825097,1.975104983,6.492807747));
#128793=CARTESIAN_POINT('Ctrl Pts',(3.580630451,1.909367073,6.316529616));
#128794=CARTESIAN_POINT('Ctrl Pts',(3.914114695,1.844275173,6.102639278));
#128795=CARTESIAN_POINT('Ctrl Pts',(3.91743638113306,1.84362682194445,6.10050881282057));
#128796=CARTESIAN_POINT('Ctrl Pts',(3.92075806726612,1.84297847088892,6.09837834764114));
#128797=CARTESIAN_POINT('Ctrl Pts',(3.114988478,1.975104983,6.822524956));
#128798=CARTESIAN_POINT('Ctrl Pts',(3.487811527,1.909367073,6.652303593));
#128799=CARTESIAN_POINT('Ctrl Pts',(3.839866164,1.844275173,6.442470632));
#128800=CARTESIAN_POINT('Ctrl Pts',(3.84337282144137,1.84362682194445,6.44038058052275));
#128801=CARTESIAN_POINT('Ctrl Pts',(3.84687947888274,1.84297847088892,6.4382905290455));
#128802=CARTESIAN_POINT('',(3.87699042669309,1.84427517246151,6.27255495673493));
#128803=CARTESIAN_POINT('Ctrl Pts',(3.89124108478693,1.83976484779183,6.11730996879012));
#128804=CARTESIAN_POINT('Ctrl Pts',(3.90267788989351,1.84202001039595,6.10997462339513));
#128805=CARTESIAN_POINT('Ctrl Pts',(3.914114695,1.844275173,6.102639278));
#128806=CARTESIAN_POINT('Ctrl Pts',(4.246361193,1.909789088,5.889542806));
#128807=CARTESIAN_POINT('Ctrl Pts',(4.553509235,1.975097379,5.641635724));
#128808=CARTESIAN_POINT('Ctrl Pts',(4.23149025439034,1.83976484779184,6.19298706509833));
#128809=CARTESIAN_POINT('Ctrl Pts',(4.24306649205931,1.84202001039594,6.18501354457374));
#128810=CARTESIAN_POINT('Ctrl Pts',(4.25464272972824,1.844275173,6.17704002404914));
#128811=CARTESIAN_POINT('Ctrl Pts',(4.59093983278288,1.909789088,5.94540415665823));
#128812=CARTESIAN_POINT('Ctrl Pts',(4.90010182207874,1.975097379,5.67862750577175));
#128813=CARTESIAN_POINT('',(4.25394609972331,1.84427517230371,6.17688783142564));
#128814=CARTESIAN_POINT('',(4.70666656643382,1.9349081664224,5.83928838194006));
#128815=CARTESIAN_POINT('Origin',(-0.11350299420495,1.87499925757301,-0.156119410337943));
#128816=CARTESIAN_POINT('Ctrl Pts',(4.54985272534518,1.9743200847369,5.64458503093839));
#128817=CARTESIAN_POINT('Ctrl Pts',(4.57591860462525,1.96742614269182,5.67701410255906));
#128818=CARTESIAN_POINT('Ctrl Pts',(4.60203463076806,1.96070006932564,5.70947076292011));
#128819=CARTESIAN_POINT('Ctrl Pts',(4.65429837177693,1.94757342765889,5.77436051368685));
#128820=CARTESIAN_POINT('Ctrl Pts',(4.68047566329595,1.94116543745121,5.80683032136998));
#128821=CARTESIAN_POINT('Ctrl Pts',(4.7066665661253,1.93490817338302,5.83928838353088));
#128822=CARTESIAN_POINT('',(4.08403037681007,1.84427517216382,6.13976354063303));
#128823=CARTESIAN_POINT('Origin',(-4.96564594998361E-13,1.93599222700044,
-6.63098048692135E-13));
#128824=CARTESIAN_POINT('',(4.7111770048529,1.75423095988382,5.83565002604275));
#128825=CARTESIAN_POINT('Origin',(-0.0802558982021118,2.01767775762883,
-0.165173268931585));
#128826=CARTESIAN_POINT('',(5.1350329741554,1.84427517280772,5.46639152841487));
#128827=CARTESIAN_POINT('Origin',(-0.13500413187521,1.87499307142583,-0.13649613936879));
#128828=CARTESIAN_POINT('Origin',(-0.108487184789677,2.01782137235173,-0.155791332412841));
#128829=CARTESIAN_POINT('Ctrl Pts',(4.546168838,1.975104983,5.647552469));
#128830=CARTESIAN_POINT('Ctrl Pts',(4.854784453,1.909367073,5.39912296));
#128831=CARTESIAN_POINT('Ctrl Pts',(5.134491921,1.844275173,5.118544003));
#128832=CARTESIAN_POINT('Ctrl Pts',(5.13727796092389,1.84362682194446,5.11574928256729));
#128833=CARTESIAN_POINT('Ctrl Pts',(5.14006400084776,1.84297847088891,5.11295456213457));
#128834=CARTESIAN_POINT('Ctrl Pts',(4.508802972,1.975104983,5.99338767));
#128835=CARTESIAN_POINT('Ctrl Pts',(4.836317064,1.909367073,5.747000052));
#128836=CARTESIAN_POINT('Ctrl Pts',(5.135032975,1.844275173,5.466391529));
#128837=CARTESIAN_POINT('Ctrl Pts',(5.13800834945066,1.84362682194446,5.4635965140737));
#128838=CARTESIAN_POINT('Ctrl Pts',(5.1409837239013,1.84297847088891,5.46080149914739));
#128839=CARTESIAN_POINT('',(5.13476244563166,1.84427517246151,5.29246776829776));
#128840=CARTESIAN_POINT('Ctrl Pts',(5.11530684846201,1.83976484789648,5.13778885074469));
#128841=CARTESIAN_POINT('Ctrl Pts',(5.12489938473102,1.84202001044827,5.12816642687234));
#128842=CARTESIAN_POINT('Ctrl Pts',(5.134491921,1.844275173,5.118544003));
#128843=CARTESIAN_POINT('Ctrl Pts',(5.413161237,1.909789088,4.839006433));
#128844=CARTESIAN_POINT('Ctrl Pts',(5.659835635,1.975097379,4.530867531));
#128845=CARTESIAN_POINT('Ctrl Pts',(5.46386952005827,1.83976484789648,5.13855314624981));
#128846=CARTESIAN_POINT('Ctrl Pts',(5.47346104026047,1.84202001044827,5.12827749352533));
#128847=CARTESIAN_POINT('Ctrl Pts',(5.4830525604627,1.844275173,5.11800184080086));
#128848=CARTESIAN_POINT('Ctrl Pts',(5.76169235907365,1.909789088,4.81948755470486));
#128849=CARTESIAN_POINT('Ctrl Pts',(6.00627721912842,1.975097379,4.49248730463809));
#128850=CARTESIAN_POINT('',(5.48233950037921,1.84427517230372,5.11800296121163));
#128851=CARTESIAN_POINT('',(5.85190171137635,1.93490816642628,4.69097488087022));
#128852=CARTESIAN_POINT('Origin',(-0.144410508305228,1.87499923698847,-0.128069709885178));
#128853=CARTESIAN_POINT('Ctrl Pts',(5.65689862657596,1.97432008475222,4.5345339261759));
#128854=CARTESIAN_POINT('Ctrl Pts',(5.68932639172034,1.96742614271044,4.56060143059601));
#128855=CARTESIAN_POINT('Ctrl Pts',(5.72180906206406,1.96070006934937,4.58668509865171));
#128856=CARTESIAN_POINT('Ctrl Pts',(5.78680028388126,1.9475734276705,4.6388226038334));
#128857=CARTESIAN_POINT('Ctrl Pts',(5.81934561353501,1.94116543746918,4.66490594160808));
#128858=CARTESIAN_POINT('Ctrl Pts',(5.85190171140948,1.9349081733955,4.69097488250165));
#128859=CARTESIAN_POINT('',(5.308415687593,1.84427517216382,5.11827347277353));
#128860=CARTESIAN_POINT('Origin',(-1.30494573480355E-12,1.93599222700033,
-1.11239142897013E-12));
#128861=CARTESIAN_POINT('',(5.85552455985458,1.754230959877,4.68645197672461));
#128862=CARTESIAN_POINT('Origin',(-0.11388718633198,2.01767782005154,-0.144059198590631));
#128863=CARTESIAN_POINT('',(6.19009135031759,1.84427517280653,4.23471003320411));
#128864=CARTESIAN_POINT('Origin',(-0.161190268281893,1.874993126293,-0.104282894811087));
#128865=CARTESIAN_POINT('Origin',(-0.139441557183412,2.01782139164873,-0.128827646493924));
#128866=CARTESIAN_POINT('Ctrl Pts',(5.653938778,1.975104983,4.538223914));
#128867=CARTESIAN_POINT('Ctrl Pts',(5.90193413,1.909367073,4.229259314));
#128868=CARTESIAN_POINT('Ctrl Pts',(6.114786011,1.844275173,3.895111301));
#128869=CARTESIAN_POINT('Ctrl Pts',(6.11690613257765,1.84362682194445,3.89178300336333));
#128870=CARTESIAN_POINT('Ctrl Pts',(6.11902625415531,1.84297847088892,3.88845470572666));
#128871=CARTESIAN_POINT('Ctrl Pts',(5.69179085,1.975104983,4.884006237));
#128872=CARTESIAN_POINT('Ctrl Pts',(5.958681789,1.909367073,4.572973176));
#128873=CARTESIAN_POINT('Ctrl Pts',(6.190091351,1.844275173,4.234710034));
#128874=CARTESIAN_POINT('Ctrl Pts',(6.19239631726747,1.84362682194445,4.23134074741953));
#128875=CARTESIAN_POINT('Ctrl Pts',(6.19470128353494,1.84297847088892,4.22797146083906));
#128876=CARTESIAN_POINT('',(6.15243867918099,1.84427517246151,4.06491067025317));
#128877=CARTESIAN_POINT('Ctrl Pts',(6.10018654800587,1.83976484784501,3.91803043868467));
#128878=CARTESIAN_POINT('Ctrl Pts',(6.10748627950293,1.84202001042253,3.90657086984234));
#128879=CARTESIAN_POINT('Ctrl Pts',(6.114786011,1.844275173,3.895111301));
#128880=CARTESIAN_POINT('Ctrl Pts',(6.326847879,1.909789088,3.562203498));
#128881=CARTESIAN_POINT('Ctrl Pts',(6.501514411,1.975097379,3.208241008));
#128882=CARTESIAN_POINT('Ctrl Pts',(6.44076431822769,1.83976484784501,3.84384619369943));
#128883=CARTESIAN_POINT('Ctrl Pts',(6.44792263252751,1.84202001042254,3.83174888655724));
#128884=CARTESIAN_POINT('Ctrl Pts',(6.45508094682746,1.844275173,3.8196515794151));
#128885=CARTESIAN_POINT('Ctrl Pts',(6.66303455481777,1.909789088,3.46821707098679));
#128886=CARTESIAN_POINT('Ctrl Pts',(6.83160576852397,1.975097379,3.09628339007489));
#128887=CARTESIAN_POINT('',(6.45438479854498,1.84427517230371,3.81980596047474));
#128888=CARTESIAN_POINT('',(6.72350843623044,1.93490816641997,3.32331660799437));
#128889=CARTESIAN_POINT('Origin',(-0.168565380183781,1.87499926396933,-0.0940314670157107));
#128890=CARTESIAN_POINT('Ctrl Pts',(6.49943423469485,1.97432008473515,3.21245305500109));
#128891=CARTESIAN_POINT('Ctrl Pts',(6.53670759948147,1.9674261426851,3.23094010477837));
#128892=CARTESIAN_POINT('Ctrl Pts',(6.57403806058471,1.96070006931838,3.24943113724768));
#128893=CARTESIAN_POINT('Ctrl Pts',(6.64871784604601,1.94757342764741,3.28637850489496));
#128894=CARTESIAN_POINT('Ctrl Pts',(6.68610943057429,1.94116543744624,3.30485574482876));
#128895=CARTESIAN_POINT('Ctrl Pts',(6.7235084366159,1.93490817338319,3.32331660957366));
#128896=CARTESIAN_POINT('',(6.28458538020791,1.84427517216382,3.85745862658826));
#128897=CARTESIAN_POINT('Origin',(1.45499931547555E-12,1.93599222699967,
7.1427239123345E-13));
#128898=CARTESIAN_POINT('',(6.72607429391972,1.75423095987622,3.31812064156621));
#128899=CARTESIAN_POINT('Origin',(-0.14219294244321,2.01767772921235,-0.116208729104463));
#128900=CARTESIAN_POINT('',(6.95570793398766,1.84427517280772,2.80501820382695));
#128901=CARTESIAN_POINT('Origin',(-0.179839597763203,1.87499310911281,-0.0671937332859013));
#128902=CARTESIAN_POINT('Origin',(-0.163875474593108,2.01782135634014,-0.0958398398494609));
#128903=CARTESIAN_POINT('Ctrl Pts',(6.497336824,1.975104983,3.216693053));
#128904=CARTESIAN_POINT('Ctrl Pts',(6.673115926,1.909367073,2.861640204));
#128905=CARTESIAN_POINT('Ctrl Pts',(6.809159503,1.844275173,2.489547522));
#128906=CARTESIAN_POINT('Ctrl Pts',(6.81051457170667,1.84362682194445,2.48584127463075));
#128907=CARTESIAN_POINT('Ctrl Pts',(6.81186964041335,1.84297847088892,2.48213502726149));
#128908=CARTESIAN_POINT('Ctrl Pts',(6.608636913,1.975104983,3.546254101));
#128909=CARTESIAN_POINT('Ctrl Pts',(6.802425177,1.909367073,3.185119157));
#128910=CARTESIAN_POINT('Ctrl Pts',(6.955707935,1.844275173,2.805018204));
#128911=CARTESIAN_POINT('Ctrl Pts',(6.95723471541271,1.84362682194445,2.80123218985553));
#128912=CARTESIAN_POINT('Ctrl Pts',(6.95876149582542,1.84297847088892,2.79744617571105));
#128913=CARTESIAN_POINT('',(6.88243371781536,1.84427517246151,2.64728286607984));
#128914=CARTESIAN_POINT('Ctrl Pts',(6.79982830483685,1.83976484801591,2.51506927495473));
#128915=CARTESIAN_POINT('Ctrl Pts',(6.80449390391836,1.84202001050798,2.50230839847734));
#128916=CARTESIAN_POINT('Ctrl Pts',(6.809159503,1.844275173,2.489547522));
#128917=CARTESIAN_POINT('Ctrl Pts',(6.94469814500001,1.909789088,2.118835886));
#128918=CARTESIAN_POINT('Ctrl Pts',(7.039189599,1.975097379,1.735600702));
#128919=CARTESIAN_POINT('Ctrl Pts',(7.11649613591557,1.83976484801591,2.36940526333307));
#128920=CARTESIAN_POINT('Ctrl Pts',(7.12088652920278,1.84202001050798,2.3560519590436));
#128921=CARTESIAN_POINT('Ctrl Pts',(7.12527692248992,1.844275173,2.34269865475413));
#128922=CARTESIAN_POINT('Ctrl Pts',(7.25282065986981,1.909789088,1.95477661131576));
#128923=CARTESIAN_POINT('Ctrl Pts',(7.33749602632692,1.975097379,1.55530070573886));
#128924=CARTESIAN_POINT('',(7.12463023715776,1.84427517230371,2.34299907776131));
#128925=CARTESIAN_POINT('',(7.28073137975271,1.93490816642443,1.80026374393309));
#128926=CARTESIAN_POINT('Origin',(-0.184838558833566,1.87499926562464,-0.0555965455474414));
#128927=CARTESIAN_POINT('Ctrl Pts',(7.03806352124641,1.97432008478782,1.7401614500682));
#128928=CARTESIAN_POINT('Ctrl Pts',(7.07843962488715,1.96742614271635,1.75020361104315));
#128929=CARTESIAN_POINT('Ctrl Pts',(7.11887234612364,1.96070006932726,1.76023738760861));
#128930=CARTESIAN_POINT('Ctrl Pts',(7.19974875171057,1.94757342764899,1.78026699959939));
#128931=CARTESIAN_POINT('Ctrl Pts',(7.24023820215542,1.94116543745568,1.79027416636109));
#128932=CARTESIAN_POINT('Ctrl Pts',(7.28073138046778,1.93490817339319,1.80026374539963));
#128933=CARTESIAN_POINT('',(6.96689484519621,1.84427517216382,2.41627330110929));
#128934=CARTESIAN_POINT('Origin',(2.55958448880378E-12,1.93599222699967,
5.89263880745872E-13));
#128935=CARTESIAN_POINT('',(7.28212026979303,1.75423095986773,1.79463767307641));
#128936=CARTESIAN_POINT('Origin',(-0.163849812250907,2.01767778307472,-0.0829245243346644));
#128937=CARTESIAN_POINT('',(7.3960833459743,1.84427517280772,1.24416684004963));
#128938=CARTESIAN_POINT('Origin',(-0.190079571013307,1.87499311850125,-0.0269625512453872));
#128939=CARTESIAN_POINT('Origin',(-0.180646895981356,2.01782136270622,-0.0583707742404796));
#128940=CARTESIAN_POINT('Ctrl Pts',(7.036926621,1.975104983,1.7447532));
#128941=CARTESIAN_POINT('Ctrl Pts',(7.132270238,1.909367073,1.360213978));
#128942=CARTESIAN_POINT('Ctrl Pts',(7.18514426400001,1.844275173,0.967575269));
#128943=CARTESIAN_POINT('Ctrl Pts',(7.18567091832362,1.84362682194445,0.963664371923291));
#128944=CARTESIAN_POINT('Ctrl Pts',(7.18619757264725,1.84297847088892,0.959753474846583));
#128945=CARTESIAN_POINT('Ctrl Pts',(7.21647046,1.975104983,2.042683064));
#128946=CARTESIAN_POINT('Ctrl Pts',(7.328094724,1.909367073,1.648332506));
#128947=CARTESIAN_POINT('Ctrl Pts',(7.396083347,1.844275173,1.24416684));
#128948=CARTESIAN_POINT('Ctrl Pts',(7.39676055100675,1.84362682194445,1.24014112810397));
#128949=CARTESIAN_POINT('Ctrl Pts',(7.39743775501351,1.84297847088892,1.23611541620793));
#128950=CARTESIAN_POINT('',(7.29061380500513,1.84427517246151,1.10587105776249));
#128951=CARTESIAN_POINT('Ctrl Pts',(7.18151764643602,1.83976484795739,0.994506269714354));
#128952=CARTESIAN_POINT('Ctrl Pts',(7.18333095521794,1.84202001047872,0.981040769357178));
#128953=CARTESIAN_POINT('Ctrl Pts',(7.18514426400001,1.844275173,0.967575269));
#128954=CARTESIAN_POINT('Ctrl Pts',(7.237822045,1.909789088,0.576393863000001));
#128955=CARTESIAN_POINT('Ctrl Pts',(7.247720104,1.975097379,0.181805635));
#128956=CARTESIAN_POINT('Ctrl Pts',(7.4594685041631,1.83976484795739,0.784173577930784));
#128957=CARTESIAN_POINT('Ctrl Pts',(7.46088568678953,1.84202001047873,0.770188661514518));
#128958=CARTESIAN_POINT('Ctrl Pts',(7.46230286941607,1.844275173,0.756203745098238));
#128959=CARTESIAN_POINT('Ctrl Pts',(7.50347293199812,1.909789088,0.349932970050721));
#128960=CARTESIAN_POINT('Ctrl Pts',(7.50029312324209,1.975097379,-0.0584061115540076));
#128961=CARTESIAN_POINT('Ctrl Pts',(7.24760078043643,1.97432008472553,0.18650182808193));
#128962=CARTESIAN_POINT('Ctrl Pts',(7.28919168066759,1.96742614270402,0.187629540275795));
#128963=CARTESIAN_POINT('Ctrl Pts',(7.3308360723623,1.96070006936449,0.188736892956852));
#128964=CARTESIAN_POINT('Ctrl Pts',(7.41412740699392,1.94757342767362,0.190912187477736));
#128965=CARTESIAN_POINT('Ctrl Pts',(7.45582148176827,1.94116543744791,0.191981357371365));
#128966=CARTESIAN_POINT('Ctrl Pts',(7.49751541633979,1.93490817336454,0.193032549346399));
#128967=CARTESIAN_POINT('',(7.32344005060519,1.84427517216382,0.862105722358991));
#128968=CARTESIAN_POINT('Ctrl Pts',(7.24747755100001,1.975104983,0.191230626));
#128969=CARTESIAN_POINT('Ctrl Pts',(7.257927521,1.909367073,-0.204814342));
#128970=CARTESIAN_POINT('Ctrl Pts',(7.225159666,1.844275173,-0.599639729));
#128971=CARTESIAN_POINT('Ctrl Pts',(7.22483328017661,1.84362682194445,-0.603572406589943));
#128972=CARTESIAN_POINT('Ctrl Pts',(7.22450689435324,1.84297847088892,-0.607505084179886));
#128973=CARTESIAN_POINT('Ctrl Pts',(7.486869868,1.975104983,0.443598437));
#128974=CARTESIAN_POINT('Ctrl Pts',(7.511110706,1.909367073,0.03447166));
#128975=CARTESIAN_POINT('Ctrl Pts',(7.490626122,1.844275173,-0.374860382));
#128976=CARTESIAN_POINT('Ctrl Pts',(7.49042208429855,1.84362682194446,-0.378937553837025));
#128977=CARTESIAN_POINT('Ctrl Pts',(7.49021804659711,1.84297847088891,-0.383014725674051));
#128978=CARTESIAN_POINT('',(7.35789289421804,1.84427517246151,-0.487250052207402));
#128979=CARTESIAN_POINT('Ctrl Pts',(7.22740720595187,1.83976484778612,-0.572558743505817));
#128980=CARTESIAN_POINT('Ctrl Pts',(7.22628343597594,1.84202001039309,-0.586099236252907));
#128981=CARTESIAN_POINT('Ctrl Pts',(7.225159666,1.844275173,-0.599639729));
#128982=CARTESIAN_POINT('Ctrl Pts',(7.19251343,1.909789088,-0.992999697));
#128983=CARTESIAN_POINT('Ctrl Pts',(7.117355273,1.975097379,-1.380490461));
#128984=CARTESIAN_POINT('Ctrl Pts',(7.45364441441404,1.83976484778612,-0.837725190583261));
#128985=CARTESIAN_POINT('Ctrl Pts',(7.45202212045395,1.84202001039309,-0.85168780034889));
#128986=CARTESIAN_POINT('Ctrl Pts',(7.45039982649387,1.844275173,-0.865650410114524));
#128987=CARTESIAN_POINT('Ctrl Pts',(7.40327115014889,1.909789088,-1.2712731472771));
#128988=CARTESIAN_POINT('Ctrl Pts',(7.31238485124716,1.975097379,-1.66938192346314));
#128989=CARTESIAN_POINT('',(7.44993905510662,1.8442751723037,-0.865106217428465));
#128990=CARTESIAN_POINT('',(7.3637239637713,1.93490816643208,-1.42322463483128));
#128991=CARTESIAN_POINT('Origin',(-0.191098975792415,1.87499926932447,0.0271535804640089));
#128992=CARTESIAN_POINT('Ctrl Pts',(7.11824828163573,1.97432008472359,-1.37587841094358));
#128993=CARTESIAN_POINT('Ctrl Pts',(7.15910923470359,1.96742614268816,-1.38371787822969));
#128994=CARTESIAN_POINT('Ctrl Pts',(7.20001805197713,1.96070006933971,-1.39158872810979));
#128995=CARTESIAN_POINT('Ctrl Pts',(7.28182970572695,1.94757342767431,-1.40736946568964));
#128996=CARTESIAN_POINT('Ctrl Pts',(7.32277883618453,1.94116543747195,-1.41528828601095));
#128997=CARTESIAN_POINT('Ctrl Pts',(7.36372396503634,1.93490817340353,-1.42322463380124));
#128998=CARTESIAN_POINT('',(7.33754933848588,1.84427517216382,-0.732372961650914));
#128999=CARTESIAN_POINT('Origin',(3.17020715234761E-13,1.9359922270005,
-2.51534904016637E-14));
#129000=CARTESIAN_POINT('',(7.36262215996559,1.75423095990768,-1.42891389846464));
#129001=CARTESIAN_POINT('Origin',(-0.183524819945431,2.01767779273109,-0.0064615644315455));
#129002=CARTESIAN_POINT('',(7.23491554310284,1.84427517280771,-1.97635954850599));
#129003=CARTESIAN_POINT('Origin',(-0.18383269442569,1.87499310861105,0.0553417618074034));
#129004=CARTESIAN_POINT('Origin',(-0.188459740288789,2.01782134606628,0.0228757494982959));
#129005=CARTESIAN_POINT('Ctrl Pts',(7.119144485,1.975104983,-1.371233679));
#129006=CARTESIAN_POINT('Ctrl Pts',(7.04421218,1.909367073,-1.76026577));
#129007=CARTESIAN_POINT('Ctrl Pts',(6.927334631,1.844275173,-2.138816239));
#129008=CARTESIAN_POINT('Ctrl Pts',(6.9261704664532,1.84362682194445,-2.14258680947271));
#129009=CARTESIAN_POINT('Ctrl Pts',(6.92500630190641,1.84297847088892,-2.14635737994542));
#129010=CARTESIAN_POINT('Ctrl Pts',(7.407191563,1.975104983,-1.176228359));
#129011=CARTESIAN_POINT('Ctrl Pts',(7.3429155,1.909367073,-1.581001044));
#129012=CARTESIAN_POINT('Ctrl Pts',(7.23491554400001,1.844275173,-1.976359549));
#129013=CARTESIAN_POINT('Ctrl Pts',(7.23383980515275,1.84362682194445,-1.98029753673787));
#129014=CARTESIAN_POINT('Ctrl Pts',(7.2327640663055,1.84297847088892,-1.98423552447575));
#129015=CARTESIAN_POINT('',(7.08112508842076,1.84427517246151,-2.05758789083126));
#129016=CARTESIAN_POINT('Ctrl Pts',(6.93535123579539,1.83976484792752,-2.11285154735182));
#129017=CARTESIAN_POINT('Ctrl Pts',(6.93134293339768,1.84202001046379,-2.12583389317593));
#129018=CARTESIAN_POINT('Ctrl Pts',(6.927334631,1.844275173,-2.138816239));
#129019=CARTESIAN_POINT('Ctrl Pts',(6.810890881,1.909789088,-2.515961694));
#129020=CARTESIAN_POINT('Ctrl Pts',(6.65419082,1.975097379,-2.878236358));
#129021=CARTESIAN_POINT('Ctrl Pts',(7.09929619710389,1.83976484792752,-2.42045286383165));
#129022=CARTESIAN_POINT('Ctrl Pts',(7.09471028323739,1.84202001046379,-2.43374028985965));
#129023=CARTESIAN_POINT('Ctrl Pts',(7.09012436937103,1.844275173,-2.44702771588773));
#129024=CARTESIAN_POINT('Ctrl Pts',(6.95690063652932,1.909789088,-2.83303594606772));
#129025=CARTESIAN_POINT('Ctrl Pts',(6.7825575900873,1.975097379,-3.20229929207681));
#129026=CARTESIAN_POINT('',(7.08979135591328,1.8442751723037,-2.44639719391422));
#129027=CARTESIAN_POINT('',(6.88561296333098,1.93490816641965,-2.9729334158594));
#129028=CARTESIAN_POINT('Origin',(-0.180794007691721,1.87499927918276,0.0675994000123735));
#129029=CARTESIAN_POINT('Ctrl Pts',(6.65605440467582,1.97432008470038,-2.87392410442729));
#129030=CARTESIAN_POINT('Ctrl Pts',(6.69427479778625,1.967426142658,-2.89036418659408));
#129031=CARTESIAN_POINT('Ctrl Pts',(6.7325351897511,1.96070006929071,-2.90684520700082));
#129032=CARTESIAN_POINT('Ctrl Pts',(6.80904174041082,1.94757342763362,-2.93984408706496));
#129033=CARTESIAN_POINT('Ctrl Pts',(6.84733119051825,1.94116543745505,-2.95638062234516));
#129034=CARTESIAN_POINT('Ctrl Pts',(6.88561296479118,1.93490817339084,-2.97293341511763));
#129035=CARTESIAN_POINT('',(7.0085629743906,1.84427517216382,-2.29260670041997));
#129036=CARTESIAN_POINT('Origin',(8.08381139805192E-13,1.93599222699978,
-2.81892564846231E-13));
#129037=CARTESIAN_POINT('',(6.88331389561855,1.75423095987297,-2.9782528121271));
#129038=CARTESIAN_POINT('Origin',(-0.180623275883013,2.01767780073337,0.0331419700085889));
#129039=CARTESIAN_POINT('',(6.64090835621196,1.84427517280772,-3.48544634034117));
#129040=CARTESIAN_POINT('Origin',(-0.167638058107709,1.87499306230618,0.0935665359471533));
#129041=CARTESIAN_POINT('Origin',(-0.17913610751596,2.01782140902048,0.0628542123918951));
#129042=CARTESIAN_POINT('Ctrl Pts',(6.657928135,1.975104983,-2.869580621));
#129043=CARTESIAN_POINT('Ctrl Pts',(6.501117306,1.909367073,-3.233409128));
#129044=CARTESIAN_POINT('Ctrl Pts',(6.305595129,1.844275173,-3.577984079));
#129045=CARTESIAN_POINT('Ctrl Pts',(6.30364762078715,1.84362682194445,-3.58141623466291));
#129046=CARTESIAN_POINT('Ctrl Pts',(6.3017001125743,1.84297847088892,-3.58484839032582));
#129047=CARTESIAN_POINT('Ctrl Pts',(6.981161212,1.975104983,-2.741056025));
#129048=CARTESIAN_POINT('Ctrl Pts',(6.831373726,1.909367073,-3.122547895));
#129049=CARTESIAN_POINT('Ctrl Pts',(6.640908357,1.844275173,-3.485446341));
#129050=CARTESIAN_POINT('Ctrl Pts',(6.63901121737071,1.84362682194445,-3.48906100873161));
#129051=CARTESIAN_POINT('Ctrl Pts',(6.63711407774142,1.84297847088892,-3.49267567646322));
#129052=CARTESIAN_POINT('',(6.47325174458042,1.84427517246151,-3.53171520710327));
#129053=CARTESIAN_POINT('Ctrl Pts',(6.31900595189991,1.83976484771587,-3.55434975934237));
#129054=CARTESIAN_POINT('Ctrl Pts',(6.31230054044995,1.84202001035797,-3.56616691917117));
#129055=CARTESIAN_POINT('Ctrl Pts',(6.305595129,1.844275173,-3.577984079));
#129056=CARTESIAN_POINT('Ctrl Pts',(6.11079864400001,1.909789088,-3.921280119));
#129057=CARTESIAN_POINT('Ctrl Pts',(5.87988380000001,1.975097379,-4.241399121));
#129058=CARTESIAN_POINT('Ctrl Pts',(6.41299278012332,1.83976484771587,-3.8900028482065));
#129059=CARTESIAN_POINT('Ctrl Pts',(6.40565767820976,1.84202001035797,-3.90199378622383));
#129060=CARTESIAN_POINT('Ctrl Pts',(6.3983225762964,1.844275173,-3.91398472424112));
#129061=CARTESIAN_POINT('Ctrl Pts',(6.18523318118433,1.909789088,-4.26232913159854));
#129062=CARTESIAN_POINT('Ctrl Pts',(5.93558547398072,1.975097379,-4.58548070487765));
#129063=CARTESIAN_POINT('',(6.3981328920845,1.84427517230371,-3.91329735543593));
#129064=CARTESIAN_POINT('',(6.085538353362,1.93490816644465,-4.38363113444891));
#129065=CARTESIAN_POINT('Origin',(-0.162035375565994,1.87499924434966,0.104884392132654));
#129066=CARTESIAN_POINT('Ctrl Pts',(5.88263082197736,1.97432008474662,-4.23758830135794));
#129067=CARTESIAN_POINT('Ctrl Pts',(5.91642351171437,1.96742614268605,-4.26186027830983));
#129068=CARTESIAN_POINT('Ctrl Pts',(5.95024646467421,1.9607000693096,-4.28618083493031));
#129069=CARTESIAN_POINT('Ctrl Pts',(6.01787055070326,1.94757342765885,-4.33485486632169));
#129070=CARTESIAN_POINT('Ctrl Pts',(6.05170994853469,1.94116543746026,-4.35923588659744));
#129071=CARTESIAN_POINT('Ctrl Pts',(6.08553835493332,1.93490817341264,-4.38363113405725));
#129072=CARTESIAN_POINT('',(6.35186399537058,1.84427517216382,-3.74564069745897));
#129073=CARTESIAN_POINT('Origin',(-9.35015953551499E-13,1.9359922270005,
6.64832772168111E-13));
#129074=CARTESIAN_POINT('',(6.08214952384334,1.75423095986658,-4.38833193473268));
#129075=CARTESIAN_POINT('Origin',(-0.169275759552884,2.01767772774323,0.0711957342580904));
#129076=CARTESIAN_POINT('',(5.73637967537476,1.84427517280772,-4.83155753418558));
#129077=CARTESIAN_POINT('Origin',(-0.143604888526623,1.87499308571353,0.127416356990073));
#129078=CARTESIAN_POINT('Origin',(-0.161436088595061,2.01782137054624,0.0998935968133235));
#129079=CARTESIAN_POINT('Ctrl Pts',(5.885394466,1.975104983,-4.233749163));
#129080=CARTESIAN_POINT('Ctrl Pts',(5.654037413,1.909367073,-4.555361869));
#129081=CARTESIAN_POINT('Ctrl Pts',(5.389013006,1.844275173,-4.84984936));
#129082=CARTESIAN_POINT('Ctrl Pts',(5.3863732174238,1.84362682194446,-4.85278261706631));
#129083=CARTESIAN_POINT('Ctrl Pts',(5.3837334288476,1.84297847088891,-4.8557158741326));
#129084=CARTESIAN_POINT('Ctrl Pts',(6.228699522,1.975104983,-4.177714957));
#129085=CARTESIAN_POINT('Ctrl Pts',(6.00040450900001,1.909367073,-4.518087878));
#129086=CARTESIAN_POINT('Ctrl Pts',(5.736379676,1.844275173,-4.831557535));
#129087=CARTESIAN_POINT('Ctrl Pts',(5.73374984372954,1.84362682194446,-4.83467986485973));
#129088=CARTESIAN_POINT('Ctrl Pts',(5.73112001145909,1.84297847088891,-4.83780219471946));
#129089=CARTESIAN_POINT('',(5.56269634316618,1.84427517246151,-4.84070344501074));
#129090=CARTESIAN_POINT('Ctrl Pts',(5.40719096992761,1.83976484806293,-4.8296505296743));
#129091=CARTESIAN_POINT('Ctrl Pts',(5.39810198796378,1.8420200105315,-4.83974994483714));
#129092=CARTESIAN_POINT('Ctrl Pts',(5.389013006,1.844275173,-4.84984936));
#129093=CARTESIAN_POINT('Ctrl Pts',(5.124972255,1.909789088,-5.143243843));
#129094=CARTESIAN_POINT('Ctrl Pts',(4.830639948,1.975097379,-5.406238775));
#129095=CARTESIAN_POINT('Ctrl Pts',(5.42682494726768,1.83976484806292,-5.17766062628129));
#129096=CARTESIAN_POINT('Ctrl Pts',(5.41708363943925,1.8420200105315,-5.18779439196334));
#129097=CARTESIAN_POINT('Ctrl Pts',(5.40734233161094,1.844275173,-5.19792815764526));
#129098=CARTESIAN_POINT('Ctrl Pts',(5.12435109618326,1.909789088,-5.49232054523886));
#129099=CARTESIAN_POINT('Ctrl Pts',(4.81107197827115,1.975097379,-5.75425013667933));
#129100=CARTESIAN_POINT('',(5.40730484608771,1.8442751723037,-5.1972160827018));
#129101=CARTESIAN_POINT('',(5.00091073363334,1.93490816642164,-5.58935513343184));
#129102=CARTESIAN_POINT('Origin',(-0.135700172412214,1.87499929261683,0.137265238893015));
#129103=CARTESIAN_POINT('Ctrl Pts',(4.83414195973404,1.97432008473011,-5.40310757969719));
#129104=CARTESIAN_POINT('Ctrl Pts',(4.86192683762261,1.96742614269327,-5.4340765203924));
#129105=CARTESIAN_POINT('Ctrl Pts',(4.88973082789581,1.9607000693384,-5.46509941077988));
#129106=CARTESIAN_POINT('Ctrl Pts',(4.94531042243446,1.94757342766584,-5.5271726498645));
#129107=CARTESIAN_POINT('Ctrl Pts',(4.97311747527434,1.94116543745111,-5.5582581257389));
#129108=CARTESIAN_POINT('Ctrl Pts',(5.000910735254,1.93490817338302,-5.58935513338412));
#129109=CARTESIAN_POINT('',(5.39815891547351,1.84427517216382,-5.02353269878948));
#129110=CARTESIAN_POINT('Origin',(5.77229236631283E-13,1.93599222699989,
-5.20850723662036E-13));
#129111=CARTESIAN_POINT('',(4.9965905998539,1.75423095988625,-5.5932175331293));
#129112=CARTESIAN_POINT('Origin',(-0.150013602016426,2.01767780695757,0.105920921450683));
#129113=CARTESIAN_POINT('',(4.56362425617614,1.84427517280653,-5.95175046836297));
#129114=CARTESIAN_POINT('Origin',(-0.112856569995003,1.8749930938328,0.155308033179116));
#129115=CARTESIAN_POINT('Origin',(-0.136187621335671,2.01782136224198,0.132262112235459));
#129116=CARTESIAN_POINT('Ctrl Pts',(4.837666293,1.975104983,-5.3999523));
#129117=CARTESIAN_POINT('Ctrl Pts',(4.542581014,1.909367073,-5.664310951));
#129118=CARTESIAN_POINT('Ctrl Pts',(4.220446625,1.844275173,-5.894941076));
#129119=CARTESIAN_POINT('Ctrl Pts',(4.21723798965313,1.84362682194446,-5.89723827864708));
#129120=CARTESIAN_POINT('Ctrl Pts',(4.21402935430626,1.84297847088891,-5.89953548129417));
#129121=CARTESIAN_POINT('Ctrl Pts',(5.184990765,1.975104983,-5.419028581));
#129122=CARTESIAN_POINT('Ctrl Pts',(4.888863046,1.909367073,-5.702367093));
#129123=CARTESIAN_POINT('Ctrl Pts',(4.563624257,1.844275173,-5.951750469));
#129124=CARTESIAN_POINT('Ctrl Pts',(4.560384700125,1.84362682194446,-5.95423446432145));
#129125=CARTESIAN_POINT('Ctrl Pts',(4.55714514325,1.84297847088891,-5.95671845964291));
#129126=CARTESIAN_POINT('',(4.39203544365065,1.84427517246151,-5.9233457705346));
#129127=CARTESIAN_POINT('Ctrl Pts',(4.24254175093117,1.83976484781954,-5.87912220719468));
#129128=CARTESIAN_POINT('Ctrl Pts',(4.23149418796559,1.8420200104098,-5.88703164159738));
#129129=CARTESIAN_POINT('Ctrl Pts',(4.220446625,1.844275173,-5.894941076));
#129130=CARTESIAN_POINT('Ctrl Pts',(3.899507858,1.909789088,-6.124715202));
#129131=CARTESIAN_POINT('Ctrl Pts',(3.555520741,1.975097379,-6.318288713));
#129132=CARTESIAN_POINT('Ctrl Pts',(4.18690481276021,1.83976484781954,-6.22321674467366));
#129133=CARTESIAN_POINT('Ctrl Pts',(4.17521279062538,1.8420200104098,-6.23101949575683));
#129134=CARTESIAN_POINT('Ctrl Pts',(4.16352076849056,1.844275173,-6.23882224684012));
#129135=CARTESIAN_POINT('Ctrl Pts',(3.82386005061316,1.909789088,-6.46549715420862));
#129136=CARTESIAN_POINT('Ctrl Pts',(3.46159810449352,1.975097379,-6.65395722672367));
#129137=CARTESIAN_POINT('',(4.16363723442891,1.8442751723037,-6.23811876149708));
#129138=CARTESIAN_POINT('',(3.68244608643453,1.93490816646172,-6.53372709829258));
#129139=CARTESIAN_POINT('Origin',(-0.103019443528005,1.87499926512958,0.1632272891718));
#129140=CARTESIAN_POINT('Ctrl Pts',(3.55961399212249,1.97432008477344,-6.31598355143885));
#129141=CARTESIAN_POINT('Ctrl Pts',(3.58009186819303,1.96742614271751,-6.35220138327312));
#129142=CARTESIAN_POINT('Ctrl Pts',(3.60057681232157,1.96070006934248,-6.38847601203026));
#129143=CARTESIAN_POINT('Ctrl Pts',(3.64151307538492,1.94757342769032,-6.46104598332777));
#129144=CARTESIAN_POINT('Ctrl Pts',(3.66198755638972,1.94116543749851,-6.49738239239404));
#129145=CARTESIAN_POINT('Ctrl Pts',(3.68244608803867,1.93490817344443,-6.53372709859178));
#129146=CARTESIAN_POINT('',(4.19204192424133,1.84427517216382,-6.06652989444278));
#129147=CARTESIAN_POINT('Origin',(8.97719398817998E-14,1.93599222699945,
-2.86229373536173E-13));
#129148=CARTESIAN_POINT('',(3.67739665313504,1.7542309598772,-6.53657049652741));
#129149=CARTESIAN_POINT('Origin',(-0.123736379684608,2.01767771480689,0.135692840214087));
#129150=CARTESIAN_POINT('',(3.17747883877507,1.84427517280771,-6.79364616499826));
#129151=CARTESIAN_POINT('Origin',(-0.0768314298773742,1.87499312527885,
0.175937908447522));
#129152=CARTESIAN_POINT('Origin',(-0.104571309852137,2.01782136834141,0.158446457629746));
#129153=CARTESIAN_POINT('Ctrl Pts',(3.56373422,1.975104983,-6.313659668));
#129154=CARTESIAN_POINT('Ctrl Pts',(3.218718575,1.909367073,-6.508403149));
#129155=CARTESIAN_POINT('Ctrl Pts',(2.85453685,1.844275173,-6.664391898));
#129156=CARTESIAN_POINT('Ctrl Pts',(2.85090940010511,1.84362682194445,-6.66594563156849));
#129157=CARTESIAN_POINT('Ctrl Pts',(2.84728195021021,1.84297847088892,-6.66749936513699));
#129158=CARTESIAN_POINT('Ctrl Pts',(3.898837603,1.975104983,-6.40695445200001));
#129159=CARTESIAN_POINT('Ctrl Pts',(3.54872378,1.909367073,-6.62000996));
#129160=CARTESIAN_POINT('Ctrl Pts',(3.177478839,1.844275173,-6.793646166));
#129161=CARTESIAN_POINT('Ctrl Pts',(3.17378103559647,1.84362682194445,-6.7953756779276));
#129162=CARTESIAN_POINT('Ctrl Pts',(3.17008323219293,1.84297847088892,-6.79710518985521));
#129163=CARTESIAN_POINT('',(3.01600784751118,1.84427517246151,-6.72901903065036));
#129164=CARTESIAN_POINT('Ctrl Pts',(2.87951599392262,1.83976484771735,-6.65369266423465));
#129165=CARTESIAN_POINT('Ctrl Pts',(2.86702642196131,1.84202001035871,-6.65904228111732));
#129166=CARTESIAN_POINT('Ctrl Pts',(2.85453685,1.844275173,-6.664391898));
#129167=CARTESIAN_POINT('Ctrl Pts',(2.491706808,1.909789088,-6.819801685));
#129168=CARTESIAN_POINT('Ctrl Pts',(2.114149336,1.975097379,-6.934902493));
#129169=CARTESIAN_POINT('Ctrl Pts',(2.75120966161612,1.83976484771735,-6.97778216615797));
#129170=CARTESIAN_POINT('Ctrl Pts',(2.73811363134117,1.84202001035871,-6.98288905421602));
#129171=CARTESIAN_POINT('Ctrl Pts',(2.7250176010662,1.844275173,-6.98799594227393));
#129172=CARTESIAN_POINT('Ctrl Pts',(2.34456955773702,1.909789088,-7.13635430189462));
#129173=CARTESIAN_POINT('Ctrl Pts',(1.95026374963917,1.975097379,-7.24253267265233));
#129174=CARTESIAN_POINT('',(2.72528257265718,1.8442751723037,-6.98733394074222));
#129175=CARTESIAN_POINT('',(2.1917943525619,1.93490816642349,-7.17258924576138));
#129176=CARTESIAN_POINT('Origin',(-0.0655218890860726,1.87499927162194,
0.181557335832974));
#129177=CARTESIAN_POINT('Ctrl Pts',(2.1186424305649,1.97432008479257,-6.93353115305763));
#129178=CARTESIAN_POINT('Ctrl Pts',(2.13085578203134,1.96742614271259,-6.97330437001318));
#129179=CARTESIAN_POINT('Ctrl Pts',(2.14306382662412,1.96070006932251,-7.01313457545201));
#129180=CARTESIAN_POINT('Ctrl Pts',(2.16744262388015,1.94757342764595,-7.09280798748468));
#129181=CARTESIAN_POINT('Ctrl Pts',(2.17962716904188,1.94116543742711,-7.13269627976358));
#129182=CARTESIAN_POINT('Ctrl Pts',(2.19179435403524,1.93490817337569,-7.17258924640248));
#129183=CARTESIAN_POINT('',(2.78990971120828,1.84427517216382,-6.8258628944585));
#129184=CARTESIAN_POINT('Origin',(-1.52330405234213E-13,1.93599222700022,
4.20670442924376E-13));
#129185=CARTESIAN_POINT('',(2.18625172570706,1.75423095985805,-7.17428068787748));
#129186=CARTESIAN_POINT('Origin',(-0.0916735934150878,2.01767777303238,
0.159120217776577));
#129187=CARTESIAN_POINT('',(1.64275804250921,1.84427517280653,-7.31787851806874));
#129188=CARTESIAN_POINT('Origin',(-0.0372137556883542,1.87499310686471,
0.188341216210165));
#129189=CARTESIAN_POINT('Origin',(-0.0680652128771495,2.01782136026042,
0.17722188718693));
#129190=CARTESIAN_POINT('Ctrl Pts',(2.123165896,1.975104983,-6.932147328));
#129191=CARTESIAN_POINT('Ctrl Pts',(1.744352434,1.909367073,-7.048169649));
#129192=CARTESIAN_POINT('Ctrl Pts',(1.355152105,1.844275173,-7.122223162));
#129193=CARTESIAN_POINT('Ctrl Pts',(1.35127545607555,1.84362682194446,-7.12296077564041));
#129194=CARTESIAN_POINT('Ctrl Pts',(1.34739880715111,1.84297847088891,-7.12369838928083));
#129195=CARTESIAN_POINT('Ctrl Pts',(2.430379128,1.975104983,-7.095298253));
#129196=CARTESIAN_POINT('Ctrl Pts',(2.042650135,1.909367073,-7.228108519));
#129197=CARTESIAN_POINT('Ctrl Pts',(1.642758043,1.844275173,-7.317878519));
#129198=CARTESIAN_POINT('Ctrl Pts',(1.63877489824694,1.84362682194446,-7.31877267747834));
#129199=CARTESIAN_POINT('Ctrl Pts',(1.63479175349388,1.84297847088891,-7.31966683595668));
#129200=CARTESIAN_POINT('',(1.49895507723091,1.84427517246151,-7.22005083982923));
#129201=CARTESIAN_POINT('Ctrl Pts',(1.38184726753537,1.83976484802767,-7.11714384826785));
#129202=CARTESIAN_POINT('Ctrl Pts',(1.36849968626769,1.84202001051386,-7.11968350513391));
#129203=CARTESIAN_POINT('Ctrl Pts',(1.355152105,1.844275173,-7.122223162));
#129204=CARTESIAN_POINT('Ctrl Pts',(0.967396318,1.909789088,-7.196001821));
#129205=CARTESIAN_POINT('Ctrl Pts',(0.573922658000001,1.975097379,-7.22724794000001));
#129206=CARTESIAN_POINT('Ctrl Pts',(1.18687100372472,1.83976484802767,-7.4060742490486));
#129207=CARTESIAN_POINT('Ctrl Pts',(1.17298332230654,1.84202001051386,-7.4082464813648));
#129208=CARTESIAN_POINT('Ctrl Pts',(1.15909564088837,1.844275173,-7.41041871368114));
#129209=CARTESIAN_POINT('Ctrl Pts',(0.755649598499641,1.909789088,-7.47352345411848));
#129210=CARTESIAN_POINT('Ctrl Pts',(0.34773722962562,1.975097379,-7.49245534066952));
#129211=CARTESIAN_POINT('',(1.15949672832168,1.8442751723037,-7.4098291504801));
#129212=CARTESIAN_POINT('',(0.598656751323674,1.93490816637869,-7.47606909172004));
#129213=CARTESIAN_POINT('Origin',(-0.0249605442852397,1.87499930398572,
0.191397811646769));
#129214=CARTESIAN_POINT('Ctrl Pts',(0.578605504166122,1.97432008478999,
-7.22687454364312));
#129215=CARTESIAN_POINT('Ctrl Pts',(0.58198324830084,1.96742614270447,-7.26834339443569));
#129216=CARTESIAN_POINT('Ctrl Pts',(0.585343558780459,1.96070006930478,
-7.30986676053086));
#129217=CARTESIAN_POINT('Ctrl Pts',(0.592024964817653,1.94757342759785,
-7.39291817330326));
#129218=CARTESIAN_POINT('Ctrl Pts',(0.595349838294234,1.94116543741407,
-7.43449321620619));
#129219=CARTESIAN_POINT('Ctrl Pts',(0.598656752668666,1.93490817333718,
-7.47606909266033));
#129220=CARTESIAN_POINT('',(1.25732442189929,1.84427517216382,-7.26602613188263));
#129221=CARTESIAN_POINT('Origin',(3.98681467613654E-14,1.93599222699989,
-1.71087102818213E-12));
#129222=CARTESIAN_POINT('',(0.592880097740823,1.75423095986685,-7.47652948834918));
#129223=CARTESIAN_POINT('Origin',(-0.0553241390603929,2.0176777484641,0.175106894883671));
#129224=CARTESIAN_POINT('',(0.0312237062239616,1.84427517280772,-7.49993500399908));
#129225=CARTESIAN_POINT('Origin',(0.00414408988284653,1.87499310458502,
0.191937658090853));
#129226=CARTESIAN_POINT('Origin',(-0.0283764098568524,2.01782136553556,
0.187710425868436));
#129227=CARTESIAN_POINT('Ctrl Pts',(0.583320695,1.975104983,-7.226495483));
#129228=CARTESIAN_POINT('Ctrl Pts',(0.188422311,1.909367073,-7.25837157));
#129229=CARTESIAN_POINT('Ctrl Pts',(-0.207598047,1.844275173,-7.247027187));
#129230=CARTESIAN_POINT('Ctrl Pts',(-0.21154262715707,1.84362682194445,
-7.24691419071793));
#129231=CARTESIAN_POINT('Ctrl Pts',(-0.215487207314141,1.84297847088892,
-7.24680119443587));
#129232=CARTESIAN_POINT('Ctrl Pts',(0.848278826,1.975104983,-7.451873793));
#129233=CARTESIAN_POINT('Ctrl Pts',(0.44106444,1.909367073,-7.49822875700001));
#129234=CARTESIAN_POINT('Ctrl Pts',(0.031223706,1.844275173,-7.499935005));
#129235=CARTESIAN_POINT('Ctrl Pts',(0.027141467311413,1.84362682194445,
-7.49995200016671));
#129236=CARTESIAN_POINT('Ctrl Pts',(0.0230592286228261,1.84297847088892,
-7.49996899533341));
#129237=CARTESIAN_POINT('',(-0.0881871672004261,1.84427517246151,-7.37348109603946));
#129238=CARTESIAN_POINT('Ctrl Pts',(-0.180435098984076,1.83976484782248,
-7.24780529572746));
#129239=CARTESIAN_POINT('Ctrl Pts',(-0.194016572992038,1.84202001041127,
-7.24741624136368));
#129240=CARTESIAN_POINT('Ctrl Pts',(-0.207598047,1.844275173,-7.247027187));
#129241=CARTESIAN_POINT('Ctrl Pts',(-0.60214855,1.909789088,-7.23572490900001));
#129242=CARTESIAN_POINT('Ctrl Pts',(-0.993140006,1.975097379,-7.181655306));
#129243=CARTESIAN_POINT('Ctrl Pts',(-0.432964422026658,1.83976484782248,
-7.48806653106592));
#129244=CARTESIAN_POINT('Ctrl Pts',(-0.446994383495375,1.84202001041127,
-7.48720253677105));
#129245=CARTESIAN_POINT('Ctrl Pts',(-0.461024344964088,1.844275173,-7.4863385424761));
#129246=CARTESIAN_POINT('Ctrl Pts',(-0.868603695431265,1.909789088,-7.46123895582905));
#129247=CARTESIAN_POINT('Ctrl Pts',(-1.27104909583471,1.975097379,-7.39203912418675));
#129248=CARTESIAN_POINT('',(-0.460505896043215,1.84427517230371,-7.48584898484908));
#129249=CARTESIAN_POINT('',(-1.02247337458115,1.93490816642325,-7.42997625662627));
#129250=CARTESIAN_POINT('Origin',(0.0167678890584535,1.87499924426971,0.192288926901991));
#129251=CARTESIAN_POINT('Ctrl Pts',(-0.988486372994197,1.97432008480372,
-7.18229731285597));
#129252=CARTESIAN_POINT('Ctrl Pts',(-0.994102175903929,1.96742614273032,
-7.22352276015986));
#129253=CARTESIAN_POINT('Ctrl Pts',(-0.999746723954761,1.96070006934087,
-7.26479770050498));
#129254=CARTESIAN_POINT('Ctrl Pts',(-1.01107512422156,1.94757342765696,
-7.34734372224098));
#129255=CARTESIAN_POINT('Ctrl Pts',(-1.01676538966857,1.94116543745716,
-7.38866151343647));
#129256=CARTESIAN_POINT('Ctrl Pts',(-1.02247337348717,1.93490817338918,
-7.42997625783242));
#129257=CARTESIAN_POINT('',(-0.334051961171194,1.84427517216382,-7.3664380632655));
#129258=CARTESIAN_POINT('Origin',(-2.28224557308199E-14,1.93599222699978,
-2.59774840527527E-13));
#129259=CARTESIAN_POINT('',(-1.0282139448201,1.75423095989281,-7.42918407905391));
#129260=CARTESIAN_POINT('Origin',(-0.0163878639005517,2.01767778891665,
0.182906237919405));
#129261=CARTESIAN_POINT('',(-1.58177061555176,1.8442751728077,-7.33130286507962));
#129262=CARTESIAN_POINT('Origin',(0.0453081133266309,1.87499312495344,0.186559308706026));
#129263=CARTESIAN_POINT('Origin',(0.0126391854568975,2.01782138537541,0.189421789738689));
#129264=CARTESIAN_POINT('Ctrl Pts',(-0.983799934,1.975104983,-7.182940741));
#129265=CARTESIAN_POINT('Ctrl Pts',(-1.37631823,1.909367073,-7.129180104));
#129266=CARTESIAN_POINT('Ctrl Pts',(-1.760641144,1.844275173,-7.032968275));
#129267=CARTESIAN_POINT('Ctrl Pts',(-1.76446921119364,1.84362682194445,
-7.03200995236865));
#129268=CARTESIAN_POINT('Ctrl Pts',(-1.76829727838728,1.84297847088892,
-7.03105162973729));
#129269=CARTESIAN_POINT('Ctrl Pts',(-0.773486052000001,1.975104983,-7.460007998));
#129270=CARTESIAN_POINT('Ctrl Pts',(-1.181144938,1.909367073,-7.417740153));
#129271=CARTESIAN_POINT('Ctrl Pts',(-1.581770616,1.844275173,-7.33130286600001));
#129272=CARTESIAN_POINT('Ctrl Pts',(-1.58576106767231,1.84362682194445,
-7.3304419031726));
#129273=CARTESIAN_POINT('Ctrl Pts',(-1.58975151934463,1.84297847088892,
-7.3295809403452));
#129274=CARTESIAN_POINT('',(-1.67120587678606,1.84427517246151,-7.18213557124785));
#129275=CARTESIAN_POINT('Ctrl Pts',(-1.73428052152909,1.83976484791691,
-7.0395674227088));
#129276=CARTESIAN_POINT('Ctrl Pts',(-1.74746083276452,1.84202001045849,
-7.03626784885441));
#129277=CARTESIAN_POINT('Ctrl Pts',(-1.760641144,1.844275173,-7.032968275));
#129278=CARTESIAN_POINT('Ctrl Pts',(-2.14353762,1.909789088,-6.937113543));
#129279=CARTESIAN_POINT('Ctrl Pts',(-2.513764547,1.975097379,-6.800256451));
#129280=CARTESIAN_POINT('Ctrl Pts',(-2.0325549126968,1.83976484791691,-7.21992514398248));
#129281=CARTESIAN_POINT('Ctrl Pts',(-2.04607112796701,1.84202001045849,
-7.21606532247525));
#129282=CARTESIAN_POINT('Ctrl Pts',(-2.05958734323724,1.844275173,-7.21220550096806));
#129283=CARTESIAN_POINT('Ctrl Pts',(-2.45224204640514,1.909789088,-7.10007521612984));
#129284=CARTESIAN_POINT('Ctrl Pts',(-2.83040257861434,1.975097379,-6.94597937370433));
#129285=CARTESIAN_POINT('',(-2.0589757749614,1.8442751723037,-7.21183884013004));
#129286=CARTESIAN_POINT('',(-2.59579378182585,1.93490816644005,-7.0364659890224));
#129287=CARTESIAN_POINT('Origin',(0.0577123295222959,1.87499926002918,0.184188807617139));
#129288=CARTESIAN_POINT('Ctrl Pts',(-2.50935772659468,1.97432008481419,
-6.80188384193689));
#129289=CARTESIAN_POINT('Ctrl Pts',(-2.52370448738016,1.96742614276615,
-6.84093822952676));
#129290=CARTESIAN_POINT('Ctrl Pts',(-2.53808996090291,1.96070006940037,
-6.8800347736293));
#129291=CARTESIAN_POINT('Ctrl Pts',(-2.56689846390454,1.94757342770655,
-6.95821564414435));
#129292=CARTESIAN_POINT('Ctrl Pts',(-2.58133779786748,1.941165437491,-6.99734420955772));
#129293=CARTESIAN_POINT('Ctrl Pts',(-2.59579378101694,1.93490817341297,
-7.03646599043658));
#129294=CARTESIAN_POINT('',(-1.90980844449988,1.84427517216382,-7.12240353765932));
#129295=CARTESIAN_POINT('Origin',(2.32236105346395E-13,1.9359922269995,
5.42968447980741E-13));
#129296=CARTESIAN_POINT('',(-2.60122984629159,1.7542309598968,-7.03445827962168));
#129297=CARTESIAN_POINT('Origin',(0.0233147369726394,2.01767778271143,0.182153020485395));
#129298=CARTESIAN_POINT('',(-3.1208031028258,1.84427517280652,-6.81986715296561));
#129299=CARTESIAN_POINT('Origin',(0.0843535976500759,1.8749931240214,0.172457830983335));
#129300=CARTESIAN_POINT('Origin',(0.053063772342255,2.01782137990498,0.182276190606282));
#129301=CARTESIAN_POINT('Ctrl Pts',(-2.504919172,1.975104983,-6.803519673));
#129302=CARTESIAN_POINT('Ctrl Pts',(-2.87670366,1.909367073,-6.66663609900001));
#129303=CARTESIAN_POINT('Ctrl Pts',(-3.231358619,1.844275173,-6.490055583));
#129304=CARTESIAN_POINT('Ctrl Pts',(-3.23489117707591,1.84362682194445,
-6.48829674412855));
#129305=CARTESIAN_POINT('Ctrl Pts',(-3.23842373515182,1.84297847088892,
-6.48653790525708));
#129306=CARTESIAN_POINT('Ctrl Pts',(-2.359083581,1.975104983,-7.11932051900001));
#129307=CARTESIAN_POINT('Ctrl Pts',(-2.748125292,1.909367073,-6.99040626299999));
#129308=CARTESIAN_POINT('Ctrl Pts',(-3.120803103,1.844275173,-6.819867154));
#129309=CARTESIAN_POINT('Ctrl Pts',(-3.1245151785753,1.84362682194445,-6.81816849085864));
#129310=CARTESIAN_POINT('Ctrl Pts',(-3.12822725415059,1.84297847088892,
-6.81646982771727));
#129311=CARTESIAN_POINT('',(-3.17608085802196,1.84427517246151,-6.65496136992127));
#129312=CARTESIAN_POINT('Ctrl Pts',(-3.20703291362491,1.83976484767348,
-6.5021672015293));
#129313=CARTESIAN_POINT('Ctrl Pts',(-3.21919576631243,1.84202001033677,
-6.49611139226473));
#129314=CARTESIAN_POINT('Ctrl Pts',(-3.231358619,1.844275173,-6.490055583));
#129315=CARTESIAN_POINT('Ctrl Pts',(-3.584697254,1.909789088,-6.314130458));
#129316=CARTESIAN_POINT('Ctrl Pts',(-3.916848252,1.975097379,-6.100885163));
#129317=CARTESIAN_POINT('Ctrl Pts',(-3.53710539384575,1.83976484767348,
-6.61418808232894));
#129318=CARTESIAN_POINT('Ctrl Pts',(-3.54947586064107,1.84202001033677,
-6.60751291421119));
#129319=CARTESIAN_POINT('Ctrl Pts',(-3.56184632743642,1.844275173,-6.60083774609345));
#129320=CARTESIAN_POINT('Ctrl Pts',(-3.92121628480267,1.909789088,-6.40691985103178));
#129321=CARTESIAN_POINT('Ctrl Pts',(-4.2574095828665,1.975097379,-6.17513334692924));
#129322=CARTESIAN_POINT('',(-3.56117023600558,1.84427517230372,-6.60061112666912));
#129323=CARTESIAN_POINT('',(-4.04773775692025,1.93490816643309,-6.31393839224868));
#129324=CARTESIAN_POINT('Origin',(0.0959581384459198,1.8749992416038,0.167476038574007));
#129325=CARTESIAN_POINT('Ctrl Pts',(-3.91289430058519,1.97432008476561,
-6.10342184256812));
#129326=CARTESIAN_POINT('Ctrl Pts',(-3.93530118123749,1.96742614271418,
-6.13847903078324));
#129327=CARTESIAN_POINT('Ctrl Pts',(-3.95775493188805,1.96070006933818,
-6.17356906786166));
#129328=CARTESIAN_POINT('Ctrl Pts',(-4.00269648439312,1.94757342766985,
-6.24372913630939));
#129329=CARTESIAN_POINT('Ctrl Pts',(-4.02520971972781,1.94116543745747,
-6.27883886758349));
#129330=CARTESIAN_POINT('Ctrl Pts',(-4.0477377564473,1.93490817339409,-6.31393839379318));
#129331=CARTESIAN_POINT('',(-3.39626440859479,1.84427517216382,-6.54533333861584));
#129332=CARTESIAN_POINT('Origin',(-7.53737350311923E-13,1.9359922269995,
-1.12713657851593E-12));
#129333=CARTESIAN_POINT('',(-4.05261513072725,1.75423095989077,-6.31080902887057));
#129334=CARTESIAN_POINT('Origin',(0.0619271358873585,2.01767776407916,0.17288233858718));
#129335=CARTESIAN_POINT('',(-4.51391030460794,1.84427517280653,-5.98954203202318));
#129336=CARTESIAN_POINT('Origin',(0.119454723687895,1.87499306953623,0.150292257931243));
#129337=CARTESIAN_POINT('Origin',(0.0910073243481019,2.01782139378126,0.166607771974832));
#129338=CARTESIAN_POINT('Ctrl Pts',(-3.908911172,1.975104983,-6.105973587));
#129339=CARTESIAN_POINT('Ctrl Pts',(-4.242577624,1.909367073,-5.892367599));
#129340=CARTESIAN_POINT('Ctrl Pts',(-4.550981356,1.844275173,-5.643675106));
#129341=CARTESIAN_POINT('Ctrl Pts',(-4.55405322646585,1.84362682194445,
-5.64119799225248));
#129342=CARTESIAN_POINT('Ctrl Pts',(-4.5571250969317,1.84297847088892,-5.63872087850496));
#129343=CARTESIAN_POINT('Ctrl Pts',(-3.834372984,1.975104983,-6.445741526));
#129344=CARTESIAN_POINT('Ctrl Pts',(-4.186606361,1.909367073,-6.236208745));
#129345=CARTESIAN_POINT('Ctrl Pts',(-4.513910305,1.844275173,-5.989542033));
#129346=CARTESIAN_POINT('Ctrl Pts',(-4.51717043195245,1.84362682194445,
-5.98708509714327));
#129347=CARTESIAN_POINT('Ctrl Pts',(-4.52043055890489,1.84297847088892,
-5.98462816128654));
#129348=CARTESIAN_POINT('',(-4.53244582789712,1.84427517246151,-5.81660857152823));
#129349=CARTESIAN_POINT('Ctrl Pts',(-4.52982801346281,1.83976484797872,
-5.66073286810881));
#129350=CARTESIAN_POINT('Ctrl Pts',(-4.54040468473138,1.84202001048939,
-5.65220398705446));
#129351=CARTESIAN_POINT('Ctrl Pts',(-4.550981356,1.844275173,-5.643675106));
#129352=CARTESIAN_POINT('Ctrl Pts',(-4.858240429,1.909789088,-5.39590565));
#129353=CARTESIAN_POINT('Ctrl Pts',(-5.136784486,1.975097379,-5.116243265));
#129354=CARTESIAN_POINT('Ctrl Pts',(-4.87626476083307,1.83976484797873,
-5.69917893640965));
#129355=CARTESIAN_POINT('Ctrl Pts',(-4.88691104845316,1.84202001048939,
-5.6900005459186));
#129356=CARTESIAN_POINT('Ctrl Pts',(-4.89755733607325,1.844275173,-5.68082215542769));
#129357=CARTESIAN_POINT('Ctrl Pts',(-5.20683880866133,1.909789088,-5.41418403439199));
#129358=CARTESIAN_POINT('Ctrl Pts',(-5.48534484687944,1.975097379,-5.11554494932952));
#129359=CARTESIAN_POINT('',(-4.89684833486108,1.8442751723037,-5.68074617391997));
#129360=CARTESIAN_POINT('',(-5.31041401337923,1.93490816641524,-5.29617805429529));
#129361=CARTESIAN_POINT('Origin',(0.129717093787129,1.87499928879841,0.142932365974908));
#129362=CARTESIAN_POINT('Ctrl Pts',(-5.13346828674901,1.97432008473599,
-5.11957062121532));
#129363=CARTESIAN_POINT('Ctrl Pts',(-5.16288756611726,1.96742614269138,
-5.14899137500026));
#129364=CARTESIAN_POINT('Ctrl Pts',(-5.19235968126211,1.96070006931876,
-5.17843413396415));
#129365=CARTESIAN_POINT('Ctrl Pts',(-5.25133286608795,1.94757342764768,
-5.23729279388055));
#129366=CARTESIAN_POINT('Ctrl Pts',(-5.28086730880979,1.94116543745644,
-5.26674199900533));
#129367=CARTESIAN_POINT('Ctrl Pts',(-5.31041401323378,1.93490817338208,
-5.29617805592223));
#129368=CARTESIAN_POINT('',(-4.72391482347484,1.84427517216382,-5.66221062818384));
#129369=CARTESIAN_POINT('Origin',(1.17657619758127E-12,1.935992227,1.09547787507935E-12));
#129370=CARTESIAN_POINT('',(-5.31450463659943,1.75423095987771,-5.29207336206581));
#129371=CARTESIAN_POINT('Origin',(0.0976439592437239,2.01767779117054,0.155528002201123));
#129372=CARTESIAN_POINT('',(-5.69595207709764,1.84427517280772,-4.87915258250815));
#129373=CARTESIAN_POINT('Origin',(0.148970427177585,1.87499306971534,0.121099350130393));
#129374=CARTESIAN_POINT('Origin',(0.124695325715196,2.01782141253908,0.143148641268627));
#129375=CARTESIAN_POINT('Ctrl Pts',(-5.130126831,1.975104983,-5.122918962));
#129376=CARTESIAN_POINT('Ctrl Pts',(-5.410073373,1.909367073,-4.84257854));
#129377=CARTESIAN_POINT('Ctrl Pts',(-5.657805263,1.844275173,-4.533402653));
#129378=CARTESIAN_POINT('Ctrl Pts',(-5.66027280861433,1.84362682194445,
-4.53032309144649));
#129379=CARTESIAN_POINT('Ctrl Pts',(-5.66274035422866,1.84297847088892,
-4.52724352989297));
#129380=CARTESIAN_POINT('Ctrl Pts',(-5.130371368,1.975104983,-5.470766823));
#129381=CARTESIAN_POINT('Ctrl Pts',(-5.42932637000001,1.909367073,-5.190413038));
#129382=CARTESIAN_POINT('Ctrl Pts',(-5.695952078,1.844275173,-4.879152583));
#129383=CARTESIAN_POINT('Ctrl Pts',(-5.69860781641318,1.84362682194445,
-4.8760522580049));
#129384=CARTESIAN_POINT('Ctrl Pts',(-5.70126355482636,1.84297847088892,
-4.87295193300981));
#129385=CARTESIAN_POINT('',(-5.67687866839398,1.84427517246151,-4.70627762054036));
#129386=CARTESIAN_POINT('Ctrl Pts',(-5.64081338858096,1.83976484799314,
-4.55460895740009));
#129387=CARTESIAN_POINT('Ctrl Pts',(-5.64930932579043,1.8420200104966,-4.54400580520006));
#129388=CARTESIAN_POINT('Ctrl Pts',(-5.657805263,1.844275173,-4.533402653));
#129389=CARTESIAN_POINT('Ctrl Pts',(-5.90461768,1.909789088,-4.225374291));
#129390=CARTESIAN_POINT('Ctrl Pts',(-6.11653038600001,1.975097379,-3.892371519));
#129391=CARTESIAN_POINT('Ctrl Pts',(-5.98741540489952,1.83976484799315,
-4.51768251699911));
#129392=CARTESIAN_POINT('Ctrl Pts',(-5.99583970555893,1.8420200104966,-4.50643007508651));
#129393=CARTESIAN_POINT('Ctrl Pts',(-6.00426400621848,1.844275173,-4.49517763317383));
#129394=CARTESIAN_POINT('Ctrl Pts',(-6.24899533556163,1.909789088,-4.16828698919722));
#129395=CARTESIAN_POINT('Ctrl Pts',(-6.45679148257349,1.975097379,-3.81675935454026));
#129396=CARTESIAN_POINT('',(-6.00355524728374,1.8442751723037,-4.49525584237545));
#129397=CARTESIAN_POINT('',(-6.32478121248456,1.93490816642691,-4.03077431595155));
#129398=CARTESIAN_POINT('Origin',(0.157410688850646,1.87499926823127,0.111705409770206));
#129399=CARTESIAN_POINT('Ctrl Pts',(-6.11400700101207,1.97432008478699,
-3.89633396802979));
#129400=CARTESIAN_POINT('Ctrl Pts',(-6.14906306633504,1.96742614273179,
-3.91874260539025));
#129401=CARTESIAN_POINT('Ctrl Pts',(-6.18417546265735,1.96070006935083,
-3.94116137532613));
#129402=CARTESIAN_POINT('Ctrl Pts',(-6.25442275922522,1.94757342766965,
-3.98596646072418));
#129403=CARTESIAN_POINT('Ctrl Pts',(-6.28959741168097,1.94116543747655,
-4.00837812750807));
#129404=CARTESIAN_POINT('Ctrl Pts',(-6.32478121269039,1.93490817340087,
-4.03077431757664));
#129405=CARTESIAN_POINT('',(-5.83068023116903,1.84427517216382,-4.5143292409069));
#129406=CARTESIAN_POINT('Origin',(-5.48172618408671E-13,1.93599222700028,
-3.3133218391157E-13));
#129407=CARTESIAN_POINT('',(-6.32789381150226,1.75423095987766,-4.02588622653618));
#129408=CARTESIAN_POINT('Origin',(0.128794683593468,2.01767775631336,0.130901045922478));
#129409=CARTESIAN_POINT('',(-6.61165746100905,1.84427517280771,-3.54061938074093));
#129410=CARTESIAN_POINT('Origin',(0.171520220308146,1.87499311130849,0.0862437827628504));
#129411=CARTESIAN_POINT('Origin',(0.152552479145713,2.01782135366553,0.112995927333402));
#129412=CARTESIAN_POINT('Ctrl Pts',(-6.111463461,1.975104983,-3.90032234));
#129413=CARTESIAN_POINT('Ctrl Pts',(-6.324600105,1.909367073,-3.56635589));
#129414=CARTESIAN_POINT('Ctrl Pts',(-6.500076484,1.844275173,-3.21115333));
#129415=CARTESIAN_POINT('Ctrl Pts',(-6.50182432506083,1.84362682194445,
-3.20761531751753));
#129416=CARTESIAN_POINT('Ctrl Pts',(-6.50357216612167,1.84297847088892,
-3.20407730503506));
#129417=CARTESIAN_POINT('Ctrl Pts',(-6.186479288,1.975104983,-4.239985143));
#129418=CARTESIAN_POINT('Ctrl Pts',(-6.418177113,1.909367073,-3.901919385));
#129419=CARTESIAN_POINT('Ctrl Pts',(-6.611657462,1.844275173,-3.540619381));
#129420=CARTESIAN_POINT('Ctrl Pts',(-6.61358463248514,1.84362682194445,
-3.53702063462816));
#129421=CARTESIAN_POINT('Ctrl Pts',(-6.61551180297026,1.84297847088892,
-3.53342188825632));
#129422=CARTESIAN_POINT('',(-6.55586697148932,1.84427517246151,-3.3758863584337));
#129423=CARTESIAN_POINT('Ctrl Pts',(-6.48804059799724,1.83976484770246,
-3.23551659508166));
#129424=CARTESIAN_POINT('Ctrl Pts',(-6.49405854099866,1.84202001035126,
-3.22333496254083));
#129425=CARTESIAN_POINT('Ctrl Pts',(-6.500076484,1.844275173,-3.21115333));
#129426=CARTESIAN_POINT('Ctrl Pts',(-6.674901571,1.909789088,-2.857269126));
#129427=CARTESIAN_POINT('Ctrl Pts',(-6.810274123,1.975097379,-2.486496806));
#129428=CARTESIAN_POINT('Ctrl Pts',(-6.81860115874642,1.83976484770246,
-3.12494428663886));
#129429=CARTESIAN_POINT('Ctrl Pts',(-6.82440956191935,1.84202001035126,
-3.11214394413541));
#129430=CARTESIAN_POINT('Ctrl Pts',(-6.83021796509225,1.844275173,-3.09934360163201));
#129431=CARTESIAN_POINT('Ctrl Pts',(-6.99895578627246,1.909789088,-2.72748547813659));
#129432=CARTESIAN_POINT('Ctrl Pts',(-7.12632572387792,1.975097379,-2.33950633402682));
#129433=CARTESIAN_POINT('',(-6.82954258916494,1.84427517230372,-3.09957234458067));
#129434=CARTESIAN_POINT('',(-7.04340867139713,1.93490816642142,-2.57689605099186));
#129435=CARTESIAN_POINT('Origin',(0.177743741960253,1.87499924246271,0.0752551014249897));
#129436=CARTESIAN_POINT('Ctrl Pts',(-6.80866154308647,1.97432008477238,
-2.49090906827571));
#129437=CARTESIAN_POINT('Ctrl Pts',(-6.84771521168073,1.96742614270981,
-2.50525778639195));
#129438=CARTESIAN_POINT('Ctrl Pts',(-6.88682607247638,1.96070006933242,
-2.51960429070294));
#129439=CARTESIAN_POINT('Ctrl Pts',(-6.96506279519489,1.94757342765555,
-2.54826076597791));
#129440=CARTESIAN_POINT('Ctrl Pts',(-7.00423292981718,1.94116543744924,
-2.56258695004634));
#129441=CARTESIAN_POINT('Ctrl Pts',(-7.04340867195185,1.93490817338345,
-2.57689605251758));
#129442=CARTESIAN_POINT('',(-6.66480951171505,1.84427517216382,-3.15536283582134));
#129443=CARTESIAN_POINT('Origin',(-9.29811783123569E-13,1.93599222699928,
-3.15069151324288E-13));
#129444=CARTESIAN_POINT('',(-7.04539770509782,1.75423095989962,-2.57145312556847));
#129445=CARTESIAN_POINT('Origin',(0.153923849122756,2.01767775774706,0.100153790920415));
#129446=CARTESIAN_POINT('',(-7.21820909110488,1.84427517280653,-2.03653075247311));
#129447=CARTESIAN_POINT('Origin',(0.186050156972235,1.87499306391399,0.047355726206694));
#129448=CARTESIAN_POINT('Origin',(0.173276963324477,2.01782136225575,0.0775599770843804));
#129449=CARTESIAN_POINT('Ctrl Pts',(-6.807034852,1.975104983,-2.495350981));
#129450=CARTESIAN_POINT('Ctrl Pts',(-6.943395564,1.909367073,-2.123374403));
#129451=CARTESIAN_POINT('Ctrl Pts',(-7.038411352,1.844275173,-1.738754046));
#129452=CARTESIAN_POINT('Ctrl Pts',(-7.03935776140644,1.84362682194445,
-1.7349230161108));
#129453=CARTESIAN_POINT('Ctrl Pts',(-7.04030417081289,1.84297847088892,
-1.73109198622161));
#129454=CARTESIAN_POINT('Ctrl Pts',(-6.953314313,1.975104983,-2.810946471));
#129455=CARTESIAN_POINT('Ctrl Pts',(-7.106921026,1.909367073,-2.430976319));
#129456=CARTESIAN_POINT('Ctrl Pts',(-7.21820909200001,1.844275173,-2.036530753));
#129457=CARTESIAN_POINT('Ctrl Pts',(-7.21931758222782,1.84362682194445,
-2.03260185863572));
#129458=CARTESIAN_POINT('Ctrl Pts',(-7.22042607245565,1.84297847088892,
-2.02867296427143));
#129459=CARTESIAN_POINT('',(-7.12831022115529,1.84427517246151,-1.88764240268987));
#129460=CARTESIAN_POINT('Ctrl Pts',(-7.03189424239342,1.83976484928362,
-1.76513506195534));
#129461=CARTESIAN_POINT('Ctrl Pts',(-7.0351527971967,1.84202001114184,-1.75194455397764));
#129462=CARTESIAN_POINT('Ctrl Pts',(-7.038411352,1.844275173,-1.738754046));
#129463=CARTESIAN_POINT('Ctrl Pts',(-7.13307448300001,1.909789088,-1.355561232));
#129464=CARTESIAN_POINT('Ctrl Pts',(-7.185577012,1.975097379,-0.964356266));
#129465=CARTESIAN_POINT('Ctrl Pts',(-7.33095670468933,1.83976484928362,
-1.58608712354138));
#129466=CARTESIAN_POINT('Ctrl Pts',(-7.33387761430758,1.84202001114184,
-1.57233741574218));
#129467=CARTESIAN_POINT('Ctrl Pts',(-7.33679852392583,1.844275173,-1.55858770794298));
#129468=CARTESIAN_POINT('Ctrl Pts',(-7.42165284325518,1.909789088,-1.15914977635031));
#129469=CARTESIAN_POINT('Ctrl Pts',(-7.46264089599617,1.975097379,-0.752860597832355));
#129470=CARTESIAN_POINT('',(-7.33618811052153,1.84427517230371,-1.55895628908607));
#129471=CARTESIAN_POINT('',(-7.43269416961486,1.9349081664758,-1.00252499180948));
#129472=CARTESIAN_POINT('Origin',(0.189766226780289,1.87499935596518,0.0352860788185521));
#129473=CARTESIAN_POINT('Ctrl Pts',(-7.18495063902355,1.97432008477277,
-0.969012029225634));
#129474=CARTESIAN_POINT('Ctrl Pts',(-7.22617580490572,1.96742614269331,
-0.97462989791423));
#129475=CARTESIAN_POINT('Ctrl Pts',(-7.26745634996787,1.96070006929825,
-0.980233309935613));
#129476=CARTESIAN_POINT('Ctrl Pts',(-7.35002423663735,1.94757342763221,
-0.991401229963115));
#129477=CARTESIAN_POINT('Ctrl Pts',(-7.39135830166391,1.94116543738299,
-0.996972054759698));
#129478=CARTESIAN_POINT('Ctrl Pts',(-7.43269417065052,1.93490817334005,
-1.002524991835));
#129479=CARTESIAN_POINT('',(-7.18729970665748,1.84427517216382,-1.64885517145456));
#129480=CARTESIAN_POINT('Ctrl Pts',(-7.184316859,1.975104983,-0.973699783));
#129481=CARTESIAN_POINT('Ctrl Pts',(-7.237525565,1.909367073,-0.581106288000001));
#129482=CARTESIAN_POINT('Ctrl Pts',(-7.24763792900001,1.844275173,-0.185052556));
#129483=CARTESIAN_POINT('Ctrl Pts',(-7.24773865369652,1.84362682194445,
-0.181107643419569));
#129484=CARTESIAN_POINT('Ctrl Pts',(-7.24783937839304,1.84297847088892,
-0.177162730839138));
#129485=CARTESIAN_POINT('Ctrl Pts',(-7.39502008900001,1.975104983,-1.250471066));
#129486=CARTESIAN_POINT('Ctrl Pts',(-7.463353212,1.909367073,-0.846363502));
#129487=CARTESIAN_POINT('Ctrl Pts',(-7.487245287,1.844275173,-0.437216209));
#129488=CARTESIAN_POINT('Ctrl Pts',(-7.48748326518231,1.84362682194445,
-0.433140877364431));
#129489=CARTESIAN_POINT('Ctrl Pts',(-7.48772124336463,1.84297847088892,
-0.429065545728861));
#129490=CARTESIAN_POINT('',(-7.48724528278758,1.84427517281017,-0.437216207964299));
#129491=CARTESIAN_POINT('Origin',(0.185898732641985,2.01782134991888,0.0384971496779662));
#129492=CARTESIAN_POINT('',(-7.36744160786082,1.8442751724617,-0.311134385795709));
#129493=CARTESIAN_POINT('Origin',(1.83447007584547E-13,1.93599222699972,
1.10859672136643E-13));
#129494=CARTESIAN_POINT('',(-7.43346663215192,1.75423095987132,-0.996781734801308));
#129495=CARTESIAN_POINT('Origin',(0.171855021166949,2.01767774414194,0.0647231140259243));
#129496=CARTESIAN_POINT('Origin',(0.19187885663823,1.87499240687786,0.00625317968707198));
#129497=CARTESIAN_POINT('Ctrl Pts',(-7.24694432414292,1.83976484770062,
-0.212217793924953));
#129498=CARTESIAN_POINT('Ctrl Pts',(-7.2472911265714,1.84202001035034,-0.198635174962476));
#129499=CARTESIAN_POINT('Ctrl Pts',(-7.24763792900001,1.844275173,-0.185052556));
#129500=CARTESIAN_POINT('Ctrl Pts',(-7.257712761,1.909789088,0.209531198));
#129501=CARTESIAN_POINT('Ctrl Pts',(-7.224890305,1.975097379,0.602876501));
#129502=CARTESIAN_POINT('Ctrl Pts',(-7.50052485709175,1.83976484770062,
0.0269336922108996));
#129503=CARTESIAN_POINT('Ctrl Pts',(-7.50042169673789,1.84202001035034,
0.0409898536246645));
#129504=CARTESIAN_POINT('Ctrl Pts',(-7.50031853638406,1.844275173,0.0550460150384293));
#129505=CARTESIAN_POINT('Ctrl Pts',(-7.49732166223242,1.909789088,0.463386479627454));
#129506=CARTESIAN_POINT('Ctrl Pts',(-7.45001127264835,1.975097379,0.868988062514227));
#129507=CARTESIAN_POINT('',(-7.49980162846453,1.84427517230371,0.0545548305699198));
#129508=CARTESIAN_POINT('',(-7.3737197555458,1.84427517216382,-0.0652488718236939));
#129509=CARTESIAN_POINT('',(-7.47443514884404,1.93490816642042,0.618723024003911));
#129510=CARTESIAN_POINT('Origin',(0.192914594014201,1.87499925147378,-0.00633297397302638));
#129511=CARTESIAN_POINT('Ctrl Pts',(-7.22527942811084,1.97432008477231,
0.59819493566734));
#129512=CARTESIAN_POINT('Ctrl Pts',(-7.26674844815987,1.96742614272921,
0.601570601553237));
#129513=CARTESIAN_POINT('Ctrl Pts',(-7.30826844486245,1.96070006936509,
0.604972290993));
#129514=CARTESIAN_POINT('Ctrl Pts',(-7.39130671311814,1.94757342767871,
0.611815125446106));
#129515=CARTESIAN_POINT('Ctrl Pts',(-7.43287197311172,1.94116543746252,
0.615260145461762));
#129516=CARTESIAN_POINT('Ctrl Pts',(-7.47443514998797,1.93490817338182,
0.618723022852726));
#129517=CARTESIAN_POINT('Origin',(1.31405303305243E-13,1.93599222699994,
-8.93856928578518E-14));
#129518=CARTESIAN_POINT('',(-7.40618621304167,1.84427517280771,1.18254207762937));
#129519=CARTESIAN_POINT('Origin',(0.189828273627123,2.01782140642892,-0.00236555032836309));
#129520=CARTESIAN_POINT('',(-7.47395492142815,1.75423095988376,0.62449806323406));
#129521=CARTESIAN_POINT('Origin',(0.181750375798407,2.01767778599679,0.0262662027630737));
#129522=CARTESIAN_POINT('Origin',(0.188738899843145,1.87499310194232,-0.0351415693773048));
#129523=CARTESIAN_POINT('Ctrl Pts',(-7.225668194,1.975104983,0.593480535));
#129524=CARTESIAN_POINT('Ctrl Pts',(-7.193236914,1.909367073,0.988333711));
#129525=CARTESIAN_POINT('Ctrl Pts',(-7.117973011,1.844275173,1.377301786));
#129526=CARTESIAN_POINT('Ctrl Pts',(-7.11722334121076,1.84362682194446,
1.38117612154711));
#129527=CARTESIAN_POINT('Ctrl Pts',(-7.11647367142152,1.84297847088891,
1.38505045709422));
#129528=CARTESIAN_POINT('Ctrl Pts',(-7.490942944,1.975104983,0.368474977));
#129529=CARTESIAN_POINT('Ctrl Pts',(-7.470807296,1.909367073,0.777824331));
#129530=CARTESIAN_POINT('Ctrl Pts',(-7.406186214,1.844275173,1.182542078));
#129531=CARTESIAN_POINT('Ctrl Pts',(-7.40554255255019,1.84362682194446,
1.18657328892585));
#129532=CARTESIAN_POINT('Ctrl Pts',(-7.40489889110037,1.84297847088891,
1.19060449985171));
#129533=CARTESIAN_POINT('',(-7.26207961307277,1.8442751724615,1.27992192875023));
#129534=CARTESIAN_POINT('Ctrl Pts',(-7.12313534524776,1.83976484781228,
1.35062255237286));
#129535=CARTESIAN_POINT('Ctrl Pts',(-7.12055417812381,1.84202001040617,
1.36396216918644));
#129536=CARTESIAN_POINT('Ctrl Pts',(-7.117973011,1.844275173,1.377301786));
#129537=CARTESIAN_POINT('Ctrl Pts',(-7.042988456,1.909789088,1.764826182));
#129538=CARTESIAN_POINT('Ctrl Pts',(-6.926375758,1.975097379,2.141919433));
#129539=CARTESIAN_POINT('Ctrl Pts',(-7.31937680634634,1.83976484781228,
1.63869512780091));
#129540=CARTESIAN_POINT('Ctrl Pts',(-7.31625439866584,1.84202001040617,
1.65240048722346));
#129541=CARTESIAN_POINT('Ctrl Pts',(-7.31313199098535,1.844275173,1.66610584664601));
#129542=CARTESIAN_POINT('Ctrl Pts',(-7.22242405181757,1.909789088,2.06425529924396));
#129543=CARTESIAN_POINT('Ctrl Pts',(-7.08902740285667,1.975097379,2.45020380704269));
#129544=CARTESIAN_POINT('',(-7.31273275824016,1.8442751723037,1.6655150258936));
#129545=CARTESIAN_POINT('',(-7.16667984767001,1.93490816644713,2.21104023792926));
#129546=CARTESIAN_POINT('Origin',(0.187043282828443,1.8749992713524,-0.0476559397633659));
#129547=CARTESIAN_POINT('Ctrl Pts',(-6.92776218226152,1.97432008467218,
2.13743097000644));
#129548=CARTESIAN_POINT('Ctrl Pts',(-6.96753601105857,1.96742614267118,
2.14964232808322));
#129549=CARTESIAN_POINT('Ctrl Pts',(-7.00735403038993,1.96070006934577,
2.16189005982757));
#129550=CARTESIAN_POINT('Ctrl Pts',(-7.08697986235771,1.94757343434173,
2.18642367327992));
#129551=CARTESIAN_POINT('Ctrl Pts',(-7.12683272412762,1.94116545135372,
2.19872343805099));
#129552=CARTESIAN_POINT('Ctrl Pts',(-7.16667984902619,1.93490817340589,
2.211040237077));
#129553=CARTESIAN_POINT('',(-7.21535286393197,1.84427517216381,1.52140839206518));
#129554=CARTESIAN_POINT('Origin',(3.06612374378901E-13,1.93599222699956,
-2.61617984220752E-13));
#129555=CARTESIAN_POINT('',(-7.16496938547227,1.75423095987033,2.216577024765));
#129556=CARTESIAN_POINT('Origin',(0.183147693307631,2.01767775526487,-0.0134188668528029));
#129557=CARTESIAN_POINT('',(-6.97882210397126,1.84427517280652,2.74700601187666));
#129558=CARTESIAN_POINT('Origin',(0.176771704887981,1.87499304877816,-0.0748931927939472));
#129559=CARTESIAN_POINT('Origin',(0.184881712020416,2.01782137571191,-0.0431177300554872));
#129560=CARTESIAN_POINT('Ctrl Pts',(-6.929155316,1.975104983,2.132910362));
#129561=CARTESIAN_POINT('Ctrl Pts',(-6.81260049900001,1.909367073,2.511560324));
#129562=CARTESIAN_POINT('Ctrl Pts',(-6.655479587,1.844275173,2.875255027));
#129563=CARTESIAN_POINT('Ctrl Pts',(-6.65391457646654,1.84362682194446,
2.87887762588843));
#129564=CARTESIAN_POINT('Ctrl Pts',(-6.65234956593308,1.84297847088891,
2.88250022477685));
#129565=CARTESIAN_POINT('Ctrl Pts',(-7.236597633,1.975104983,1.970191539));
#129566=CARTESIAN_POINT('Ctrl Pts',(-7.128934734,1.909367073,2.365641964));
#129567=CARTESIAN_POINT('Ctrl Pts',(-6.978822105,1.844275173,2.747006012));
#129568=CARTESIAN_POINT('Ctrl Pts',(-6.97732690081234,1.84362682194446,
2.75080460726404));
#129569=CARTESIAN_POINT('Ctrl Pts',(-6.97583169662468,1.84297847088891,
2.75460320252807));
#129570=CARTESIAN_POINT('',(-6.81715084725798,1.8442751724615,2.81113051644934));
#129571=CARTESIAN_POINT('Ctrl Pts',(-6.66625647519525,1.83976484790778,
2.85030928883513));
#129572=CARTESIAN_POINT('Ctrl Pts',(-6.66086803109762,1.84202001045392,
2.86278215791755));
#129573=CARTESIAN_POINT('Ctrl Pts',(-6.655479587,1.844275173,2.875255027));
#129574=CARTESIAN_POINT('Ctrl Pts',(-6.49894183800001,1.909789088,3.237599855));
#129575=CARTESIAN_POINT('Ctrl Pts',(-6.30399157900001,1.975097379,3.580808593));
#129576=CARTESIAN_POINT('Ctrl Pts',(-6.79598283116813,1.83976484790778,
3.17383300112513));
#129577=CARTESIAN_POINT('Ctrl Pts',(-6.78998717662345,1.84202001045392,
3.18654671124277));
#129578=CARTESIAN_POINT('Ctrl Pts',(-6.7839915220787,1.844275173,3.19926042136032));
#129579=CARTESIAN_POINT('Ctrl Pts',(-6.60981392104711,1.909789088,3.56860183554046));
#129580=CARTESIAN_POINT('Ctrl Pts',(-6.39656849030963,1.975097379,3.91685074512989));
#129581=CARTESIAN_POINT('',(-6.78372863217671,1.8442751723037,3.1985975904431));
#129582=CARTESIAN_POINT('',(-6.52381856217684,1.93490816641423,3.69997166723722));
#129583=CARTESIAN_POINT('Origin',(0.17242549256259,1.87499928258689,-0.0867504515316227));
#129584=CARTESIAN_POINT('Ctrl Pts',(-6.30631047561054,1.97432008478727,
3.57672310740659));
#129585=CARTESIAN_POINT('Ctrl Pts',(-6.34252933352834,1.96742614270498,
3.59719916832535));
#129586=CARTESIAN_POINT('Ctrl Pts',(-6.37878352963317,1.96070006931012,
3.61772025216601));
#129587=CARTESIAN_POINT('Ctrl Pts',(-6.4512737889157,1.94757342762861,3.65879750425718));
#129588=CARTESIAN_POINT('Ctrl Pts',(-6.48755087065177,1.94116543743315,
3.67937691934155));
#129589=CARTESIAN_POINT('Ctrl Pts',(-6.52381856370022,1.93490817337558,
3.69997166666959));
#129590=CARTESIAN_POINT('',(-6.71960409236808,1.84427517216381,3.03692629071717));
#129591=CARTESIAN_POINT('Origin',(1.40469233467222E-12,1.93599222700022,
-7.65013052905772E-13));
#129592=CARTESIAN_POINT('',(-6.52095784408861,1.75423095986924,3.70501130874087));
#129593=CARTESIAN_POINT('Origin',(0.175981522065984,2.01767778536792,-0.0524766778138985));
#129594=CARTESIAN_POINT('',(-6.22513603000557,1.84427517280653,4.18302299766104));
#129595=CARTESIAN_POINT('Origin',(0.156539136163832,1.87499309963404,-0.111142978868746));
#129596=CARTESIAN_POINT('Origin',(0.171290313807868,2.01782138396538,-0.0818538011439141));
#129597=CARTESIAN_POINT('Ctrl Pts',(-6.308642835,1.975104983,3.572607672));
#129598=CARTESIAN_POINT('Ctrl Pts',(-6.113414457,1.909367073,3.917349167));
#129599=CARTESIAN_POINT('Ctrl Pts',(-5.881783334,1.844275173,4.238764539));
#129600=CARTESIAN_POINT('Ctrl Pts',(-5.87947616086335,1.84362682194446,
4.24196601254285));
#129601=CARTESIAN_POINT('Ctrl Pts',(-5.87716898772669,1.84297847088891,
4.24516748608571));
#129602=CARTESIAN_POINT('Ctrl Pts',(-6.643877059,1.975104983,3.479784134));
#129603=CARTESIAN_POINT('Ctrl Pts',(-6.453721107,1.909367073,3.842844807));
#129604=CARTESIAN_POINT('Ctrl Pts',(-6.225136031,1.844275173,4.183022998));
#129605=CARTESIAN_POINT('Ctrl Pts',(-6.22285919816356,1.84362682194446,
4.18641135951976));
#129606=CARTESIAN_POINT('Ctrl Pts',(-6.22058236532713,1.84297847088891,
4.18979972103951));
#129607=CARTESIAN_POINT('',(-6.05345968438437,1.8442751724615,4.21089376579109));
#129608=CARTESIAN_POINT('Ctrl Pts',(-5.89767086073434,1.83976484792964,
4.21671873080049));
#129609=CARTESIAN_POINT('Ctrl Pts',(-5.88972709736717,1.84202001046485,
4.22774163490021));
#129610=CARTESIAN_POINT('Ctrl Pts',(-5.881783334,1.844275173,4.238764539));
#129611=CARTESIAN_POINT('Ctrl Pts',(-5.651011924,1.909789088,4.558986958));
#129612=CARTESIAN_POINT('Ctrl Pts',(-5.386839759,1.975097379,4.852263122));
#129613=CARTESIAN_POINT('Ctrl Pts',(-5.95481625195012,1.83976484792964,
4.56056597055263));
#129614=CARTESIAN_POINT('Ctrl Pts',(-5.94622770064011,1.84202001046485,
4.57169355263703));
#129615=CARTESIAN_POINT('Ctrl Pts',(-5.93763914933008,1.844275173,4.5828211347213));
#129616=CARTESIAN_POINT('Ctrl Pts',(-5.68813623691231,1.909789088,4.90608451616743));
#129617=CARTESIAN_POINT('Ctrl Pts',(-5.40501314457735,1.975097379,5.20035009539286));
#129618=CARTESIAN_POINT('',(-5.93752489475053,1.84427517230362,4.58211728676164));
#129619=CARTESIAN_POINT('',(-5.57591077120322,1.93490816643902,5.01589653422082));
#129620=CARTESIAN_POINT('Origin',(0.149745580527058,1.87499928425088,-0.12178873420025));
#129621=CARTESIAN_POINT('Ctrl Pts',(-5.38998270015481,1.97432008470267,
4.84877164788896));
#129622=CARTESIAN_POINT('Ctrl Pts',(-5.4209530333933,1.96742614267996,4.87655497353722));
#129623=CARTESIAN_POINT('Ctrl Pts',(-5.45194819995815,1.96070006933894,
4.90438986621784));
#129624=CARTESIAN_POINT('Ctrl Pts',(-5.5139132822696,1.94757342768204,4.96009001806846));
#129625=CARTESIAN_POINT('Ctrl Pts',(-5.54491826017082,1.94116543746585,
4.98798679832514));
#129626=CARTESIAN_POINT('Ctrl Pts',(-5.57591077280683,1.93490817340487,
5.01589653400181));
#129627=CARTESIAN_POINT('',(-5.90965410140387,1.84427517216381,4.41044089164858));
#129628=CARTESIAN_POINT('Origin',(-7.24247051220317E-13,1.93599222699922,
5.2432017061399E-13));
#129629=CARTESIAN_POINT('',(-5.57203356127325,1.75423095987769,5.02020338153605));
#129630=CARTESIAN_POINT('Origin',(0.160586504670851,2.01767779640965,-0.0890808571676227));
#129631=CARTESIAN_POINT('',(-5.18036951346625,1.84427517280771,5.42344647712285));
#129632=CARTESIAN_POINT('Origin',(0.12898694124733,1.87499308356648,-0.142195858114513));
#129633=CARTESIAN_POINT('Origin',(0.149689335412058,2.01782137334422,-0.116762313732693));
#129634=CARTESIAN_POINT('Ctrl Pts',(-5.393145228,1.975104983,4.845253817));
#129635=CARTESIAN_POINT('Ctrl Pts',(-5.128371949,1.909367073,5.139967117));
#129636=CARTESIAN_POINT('Ctrl Pts',(-4.833061429,1.844275173,5.404074132));
#129637=CARTESIAN_POINT('Ctrl Pts',(-4.83011997411306,1.84362682194446,
5.40670478284829));
#129638=CARTESIAN_POINT('Ctrl Pts',(-4.82717851922612,1.84297847088891,
5.40933543369657));
#129639=CARTESIAN_POINT('Ctrl Pts',(-5.740496178,1.975104983,4.826665891));
#129640=CARTESIAN_POINT('Ctrl Pts',(-5.476738654,1.909367073,5.14036049900001));
#129641=CARTESIAN_POINT('Ctrl Pts',(-5.180369514,1.844275173,5.423446478));
#129642=CARTESIAN_POINT('Ctrl Pts',(-5.17741751467674,1.84362682194446,
5.42626616974804));
#129643=CARTESIAN_POINT('Ctrl Pts',(-5.17446551535348,1.84297847088891,
5.42908586149607));
#129644=CARTESIAN_POINT('',(-5.00671547392265,1.8442751724615,5.4137603027595));
#129645=CARTESIAN_POINT('Ctrl Pts',(-4.85331671130139,1.83976484792442,
5.38595909115377));
#129646=CARTESIAN_POINT('Ctrl Pts',(-4.84318907015065,1.84202001046224,
5.39501661157687));
#129647=CARTESIAN_POINT('Ctrl Pts',(-4.83306142900001,1.844275173,5.404074132));
#129648=CARTESIAN_POINT('Ctrl Pts',(-4.538846972,1.909789088,5.667200897));
#129649=CARTESIAN_POINT('Ctrl Pts',(-4.2178053,1.975097379,5.896831221));
#129650=CARTESIAN_POINT('Ctrl Pts',(-4.83520908217589,1.83976484792441,
5.73405194302275));
#129651=CARTESIAN_POINT('Ctrl Pts',(-4.82442922520848,1.84202001046224,
5.74307308379315));
#129652=CARTESIAN_POINT('Ctrl Pts',(-4.81364936824105,1.844275173,5.75209422456359));
#129653=CARTESIAN_POINT('Ctrl Pts',(-4.50048762435396,1.909789088,6.01416413737017));
#129654=CARTESIAN_POINT('Ctrl Pts',(-4.1607253913209,1.975097379,6.2406868555797));
#129655=CARTESIAN_POINT('',(-4.81368909130657,1.8442751723037,5.75138227091392));
#129656=CARTESIAN_POINT('',(-4.36727958982717,1.93490816641456,6.09728365358735));
#129657=CARTESIAN_POINT('Origin',(0.120063566074309,1.87499928118574,-0.151132151585901));
#129658=CARTESIAN_POINT('Ctrl Pts',(-4.2216253242295,1.97432008482041,5.89409701454771));
#129659=CARTESIAN_POINT('Ctrl Pts',(-4.24589899453292,1.9674261427479,5.9278884878857));
#129660=CARTESIAN_POINT('Ctrl Pts',(-4.27018583224409,1.96070006935906,
5.96173566104478));
#129661=CARTESIAN_POINT('Ctrl Pts',(-4.31872831918151,1.94757342765911,
6.02945423542534));
#129662=CARTESIAN_POINT('Ctrl Pts',(-4.34301143469336,1.94116543745499,
6.06336395806756));
#129663=CARTESIAN_POINT('Ctrl Pts',(-4.367279591454,1.93490817337971,6.0972836537083));
#129664=CARTESIAN_POINT('',(-4.82337525208443,1.84427517216381,5.57772817788601));
#129665=CARTESIAN_POINT('Origin',(3.03576608295941E-15,1.9359922269995,
6.37510877421477E-14));
#129666=CARTESIAN_POINT('',(-4.36256718233698,1.75423095984561,6.10065632351581));
#129667=CARTESIAN_POINT('Origin',(0.137681771613398,2.01767770434297,-0.121518839677397));
#129668=CARTESIAN_POINT('',(-3.89337467666301,1.84427517280772,6.41027562702946));
#129669=CARTESIAN_POINT('Origin',(0.0954033633209667,1.87499309498197,-0.166599734341152));
#129670=CARTESIAN_POINT('Origin',(0.121089346307142,2.01782136500259,-0.146211421620384));
#129671=CARTESIAN_POINT('Ctrl Pts',(-4.225470143,1.975104983,5.891341279));
#129672=CARTESIAN_POINT('Ctrl Pts',(-3.903532469,1.909367073,6.122245918));
#129673=CARTESIAN_POINT('Ctrl Pts',(-3.558350943,1.844275173,6.316695225));
#129674=CARTESIAN_POINT('Ctrl Pts',(-3.55491274551712,1.84362682194446,
6.31863204683871));
#129675=CARTESIAN_POINT('Ctrl Pts',(-3.55147454803423,1.84297847088891,
6.32056886867742));
#129676=CARTESIAN_POINT('Ctrl Pts',(-4.568696076,1.975104983,5.947858115));
#129677=CARTESIAN_POINT('Ctrl Pts',(-4.243669988,1.909367073,6.197518646));
#129678=CARTESIAN_POINT('Ctrl Pts',(-3.893374677,1.844275173,6.410275628));
#129679=CARTESIAN_POINT('Ctrl Pts',(-3.88988554341135,1.84362682194446,
6.41239480433152));
#129680=CARTESIAN_POINT('Ctrl Pts',(-3.88639640982271,1.84297847088891,
6.41451398066305));
#129681=CARTESIAN_POINT('',(-3.72586281284765,1.8442751724615,6.36348542483268));
#129682=CARTESIAN_POINT('Ctrl Pts',(-3.58202686786243,1.8397648476387,6.30335798985825));
#129683=CARTESIAN_POINT('Ctrl Pts',(-3.57018890543119,1.84202001031938,
6.31002660742913));
#129684=CARTESIAN_POINT('Ctrl Pts',(-3.558350943,1.844275173,6.316695225));
#129685=CARTESIAN_POINT('Ctrl Pts',(-3.21445058,1.909789088,6.510422821));
#129686=CARTESIAN_POINT('Ctrl Pts',(-2.851550952,1.975097379,6.665670046));
#129687=CARTESIAN_POINT('Ctrl Pts',(-3.48951291167448,1.8397648476387,6.63942001909199));
#129688=CARTESIAN_POINT('Ctrl Pts',(-3.47704580241671,1.84202001031938,
6.64591290042925));
#129689=CARTESIAN_POINT('Ctrl Pts',(-3.46457869315892,1.844275173,6.65240578176653));
#129690=CARTESIAN_POINT('Ctrl Pts',(-3.10240121335745,1.909789088,6.84102812803436));
#129691=CARTESIAN_POINT('Ctrl Pts',(-2.72188674349151,1.975097379,6.98921603451046));
#129692=CARTESIAN_POINT('',(-3.46477053652249,1.84427517230371,6.65171901243283));
#129693=CARTESIAN_POINT('',(-2.95443926928893,1.93490816641705,6.89356856655105));
#129694=CARTESIAN_POINT('Origin',(0.0847675782078298,1.87499924514342,-0.173408794056555));
#129695=CARTESIAN_POINT('Ctrl Pts',(-2.85586943983058,1.97432008474088,
6.6638209567827));
#129696=CARTESIAN_POINT('Ctrl Pts',(-2.87231143740344,1.96742614270362,
6.70204052568845));
#129697=CARTESIAN_POINT('Ctrl Pts',(-2.88875432072029,1.96070006935415,
6.74031732275798));
#129698=CARTESIAN_POINT('Ctrl Pts',(-2.92160441985889,1.94757342767156,
6.81688787426888));
#129699=CARTESIAN_POINT('Ctrl Pts',(-2.93803022184158,1.94116543744954,
6.85522495862428));
#129700=CARTESIAN_POINT('Ctrl Pts',(-2.95443927083686,1.93490817337398,
6.89356856702391));
#129701=CARTESIAN_POINT('',(-3.51156073694809,1.84427517216381,6.48420709396512));
#129702=CARTESIAN_POINT('Origin',(5.48172618408671E-13,1.93599222700033,
-1.30581309654154E-12));
#129703=CARTESIAN_POINT('',(-2.94911201030461,1.75423095990399,6.89584935679358));
#129704=CARTESIAN_POINT('Origin',(0.108340146961858,2.01767777290915,-0.148275807789205));
#129705=CARTESIAN_POINT('',(-2.42432996691648,1.84427517280609,7.09736741297175));
#129706=CARTESIAN_POINT('Origin',(0.0573589000589378,1.87499309175534,-0.183213729321554));
#129707=CARTESIAN_POINT('Origin',(0.0868271630715356,2.0178213733533,-0.168823616204068));
#129708=CARTESIAN_POINT('Ctrl Pts',(-2.860216771,1.975104983,6.66195617100001));
#129709=CARTESIAN_POINT('Ctrl Pts',(-2.496168149,1.909367073,6.818255304));
#129710=CARTESIAN_POINT('Ctrl Pts',(-2.117255923,1.844275173,6.933954669));
#129711=CARTESIAN_POINT('Ctrl Pts',(-2.11348174922899,1.84362682194446,
6.9351070981874));
#129712=CARTESIAN_POINT('Ctrl Pts',(-2.10970757545798,1.84297847088891,
6.93625952737481));
#129713=CARTESIAN_POINT('Ctrl Pts',(-3.183268824,1.975104983,6.790935105));
#129714=CARTESIAN_POINT('Ctrl Pts',(-2.812172031,1.909367073,6.96488771));
#129715=CARTESIAN_POINT('Ctrl Pts',(-2.424329967,1.844275173,7.097367414));
#129716=CARTESIAN_POINT('Ctrl Pts',(-2.42046684714056,1.84362682194446,
7.09868698457524));
#129717=CARTESIAN_POINT('Ctrl Pts',(-2.41660372728113,1.84297847088891,
7.10000655515048));
#129718=CARTESIAN_POINT('',(-2.27079294816725,1.84427517245675,7.01566104047484));
#129719=CARTESIAN_POINT('Ctrl Pts',(-2.1432454269271,1.83976484804352,6.92601887564033));
#129720=CARTESIAN_POINT('Ctrl Pts',(-2.13025067496355,1.84202001052179,
6.92998677232021));
#129721=CARTESIAN_POINT('Ctrl Pts',(-2.117255923,1.844275173,6.933954669));
#129722=CARTESIAN_POINT('Ctrl Pts',(-1.739750052,1.909789088,7.04922461));
#129723=CARTESIAN_POINT('Ctrl Pts',(-1.351961251,1.975097379,7.122829548));
#129724=CARTESIAN_POINT('Ctrl Pts',(-1.98065099273836,1.83976484804352,
7.23433619666886));
#129725=CARTESIAN_POINT('Ctrl Pts',(-1.96707958119578,1.84202001052179,
7.23799721771154));
#129726=CARTESIAN_POINT('Ctrl Pts',(-1.95350816965328,1.844275173,7.24165823875426));
#129727=CARTESIAN_POINT('Ctrl Pts',(-1.5592499683863,1.909789088,7.34801324586424));
#129728=CARTESIAN_POINT('Ctrl Pts',(-1.15577569678679,1.975097379,7.41093723892653));
#129729=CARTESIAN_POINT('',(-1.95384316290116,1.8442751723037,7.24102876641797));
#129730=CARTESIAN_POINT('',(-1.40345265154337,1.93490816642678,7.36751787427784));
#129731=CARTESIAN_POINT('Origin',(0.0455080576337361,1.87499926986637,-0.187577469996594));
#129732=CARTESIAN_POINT('Ctrl Pts',(-1.35657627490455,1.9743200846916,7.12195203649257));
#129733=CARTESIAN_POINT('Ctrl Pts',(-1.36441779022587,1.9674261426747,7.16281259655497));
#129734=CARTESIAN_POINT('Ctrl Pts',(-1.37224786815185,1.96070006933634,
7.20372923723952));
#129735=CARTESIAN_POINT('Ctrl Pts',(-1.38786954499056,1.94757342767207,
7.28557141204423));
#129736=CARTESIAN_POINT('Ctrl Pts',(-1.39566998086786,1.94116543746633,
7.32654325846433));
#129737=CARTESIAN_POINT('Ctrl Pts',(-1.4034526529648,1.93490817339425,7.36751787507186));
#129738=CARTESIAN_POINT('',(-2.03554954552458,1.84427517216381,7.08749169292896));
#129739=CARTESIAN_POINT('Origin',(4.55364912443912E-15,1.93599222699994,
-1.80844922370582E-13));
#129740=CARTESIAN_POINT('',(-1.39775963854105,1.75423095988713,7.36860013786871));
#129741=CARTESIAN_POINT('Origin',(0.0739322772112747,2.01767774345327,-0.168099117039335));
#129742=CARTESIAN_POINT('',(-0.841926282128371,1.8442751728077,7.45259418698405));
#129743=CARTESIAN_POINT('Origin',(0.01663228595669,1.87499309352602,-0.191260385054375));
#129744=CARTESIAN_POINT('Origin',(0.0485051041280235,2.01782134416412,-0.183541901016625));
#129745=CARTESIAN_POINT('Ctrl Pts',(-1.361222842,1.975104983,7.121065396));
#129746=CARTESIAN_POINT('Ctrl Pts',(-0.972085781,1.909367073,7.19545065));
#129747=CARTESIAN_POINT('Ctrl Pts',(-0.577160368,1.844275173,7.2269901));
#129748=CARTESIAN_POINT('Ctrl Pts',(-0.573226694096189,1.84362682194446,
7.22730425023526));
#129749=CARTESIAN_POINT('Ctrl Pts',(-0.569293020192376,1.84297847088891,
7.22761840047053));
#129750=CARTESIAN_POINT('Ctrl Pts',(-1.648995459,1.975104983,7.316475516));
#129751=CARTESIAN_POINT('Ctrl Pts',(-1.249180034,1.909367073,7.406586365));
#129752=CARTESIAN_POINT('Ctrl Pts',(-0.841926282,1.844275173,7.452594188));
#129753=CARTESIAN_POINT('Ctrl Pts',(-0.837869811072231,1.84362682194446,
7.45305245117261));
#129754=CARTESIAN_POINT('Ctrl Pts',(-0.833813340144462,1.84297847088891,
7.45351071434522));
#129755=CARTESIAN_POINT('',(-0.709543328284545,1.8442751724615,7.33979214368248));
#129756=CARTESIAN_POINT('Origin',(-3.72694496791892E-14,1.93599222700011,
5.42101086242752E-14));
#129757=CARTESIAN_POINT('',(0.218950416952298,1.75423096007169,7.49680336637767));
#129758=CARTESIAN_POINT('',(-0.351556253986197,1.8442751723037,7.49175606294591));
#129759=CARTESIAN_POINT('Origin',(0.0360674549391415,2.01767783439293,-0.180062609324158));
#129760=CARTESIAN_POINT('Origin',(-0.0248718942039444,1.87499308268038,
-0.190364284420828));
#129761=CARTESIAN_POINT('Origin',(0.00412048493843249,1.87499926526327,
-0.192974814822687));
#129762=CARTESIAN_POINT('Ctrl Pts',(-0.604248213242546,1.83976484794618,
7.22482681617143));
#129763=CARTESIAN_POINT('Ctrl Pts',(-0.59070429062127,1.84202001047312,
7.22590845808572));
#129764=CARTESIAN_POINT('Ctrl Pts',(-0.577160368,1.844275173,7.2269901));
#129765=CARTESIAN_POINT('Ctrl Pts',(-0.183700746,1.909789088,7.25841249));
#129766=CARTESIAN_POINT('Ctrl Pts',(0.210844655,1.975097379,7.246933457));
#129767=CARTESIAN_POINT('Ctrl Pts',(-0.379176036910304,1.83976484794618,
7.49098285274321));
#129768=CARTESIAN_POINT('Ctrl Pts',(-0.365134905824976,1.84202001047312,
7.49164082883958));
#129769=CARTESIAN_POINT('Ctrl Pts',(-0.351093774739651,1.844275173,7.49229880493583));
#129770=CARTESIAN_POINT('Ctrl Pts',(0.0568100714185217,1.909789088,7.51141343172169));
#129771=CARTESIAN_POINT('Ctrl Pts',(0.464378137235999,1.975097379,7.48613125413578));
#129772=CARTESIAN_POINT('',(-0.464358318833719,1.84427517216381,7.35937305782598));
#129773=CARTESIAN_POINT('Ctrl Pts',(-1.160767276,4.042807359,7.409630175));
#129774=CARTESIAN_POINT('Ctrl Pts',(-0.754367972,3.977102825,7.473295298));
#129775=CARTESIAN_POINT('Ctrl Pts',(-0.343443638,3.912499672,7.49213230400001));
#129776=CARTESIAN_POINT('Ctrl Pts',(-1.356373314,4.042807359,7.121990693));
#129777=CARTESIAN_POINT('Ctrl Pts',(-0.965750302,3.977102825,7.196384307));
#129778=CARTESIAN_POINT('Ctrl Pts',(-0.569334295,3.912499672,7.22761084000001));
#129779=CARTESIAN_POINT('',(-0.595762404227082,3.95233946559532,7.47630027399342));
#129780=CARTESIAN_POINT('Ctrl Pts',(-0.595762404863384,3.95233945647622,
7.47630027530279));
#129781=CARTESIAN_POINT('Ctrl Pts',(-0.592182366064195,3.94612348982327,
7.43474870639099));
#129782=CARTESIAN_POINT('Ctrl Pts',(-0.588581597117314,3.93976379156922,
7.39319744671796));
#129783=CARTESIAN_POINT('Ctrl Pts',(-0.581342220634875,3.9267491041166,
7.31018955732445));
#129784=CARTESIAN_POINT('Ctrl Pts',(-0.577699717669751,3.92008711220508,
7.2686882076048));
#129785=CARTESIAN_POINT('Ctrl Pts',(-0.574036078608516,3.91326598549935,
7.22723893645966));
#129786=CARTESIAN_POINT('',(-1.16076727022619,4.04280736030966,7.40963015407995));
#129787=CARTESIAN_POINT('Origin',(0.0475501136360631,4.16063865198492,-0.181696116530682));
#129788=CARTESIAN_POINT('',(-1.25857027269469,4.04280736269456,7.26581043786369));
#129789=CARTESIAN_POINT('Ctrl Pts',(-2.42647005212533,3.912491975,7.09718410019861));
#129790=CARTESIAN_POINT('Ctrl Pts',(-2.04152351657078,3.97753138,7.22879421861146));
#129791=CARTESIAN_POINT('Ctrl Pts',(-1.64460027740355,4.042807359,7.31799624221166));
#129792=CARTESIAN_POINT('Ctrl Pts',(-1.63094216828536,4.0450535022237,7.3210656794521));
#129793=CARTESIAN_POINT('Ctrl Pts',(-1.61728405916712,4.04729964544735,
7.32413511669249));
#129794=CARTESIAN_POINT('Ctrl Pts',(-2.118733935,3.912491975,6.933503192));
#129795=CARTESIAN_POINT('Ctrl Pts',(-1.742665343,3.97753138,7.048421908));
#129796=CARTESIAN_POINT('Ctrl Pts',(-1.356373314,4.042807359,7.121990693));
#129797=CARTESIAN_POINT('Ctrl Pts',(-1.34308102430026,4.04505350222369,
7.12452219126988));
#129798=CARTESIAN_POINT('Ctrl Pts',(-1.32978873460052,4.04729964544735,
7.12705368953974));
#129799=CARTESIAN_POINT('',(-1.64401284267851,4.04280735814476,7.31759679238927));
#129800=CARTESIAN_POINT('',(-1.50019304561873,4.04280735744341,7.21979371444933));
#129801=CARTESIAN_POINT('',(-2.18901737117743,3.95233946528201,7.17343722208511));
#129802=CARTESIAN_POINT('Origin',(0.046198773551316,4.01785666264986,-0.187368441160566));
#129803=CARTESIAN_POINT('Ctrl Pts',(-2.11425816787987,3.91326598475539,
6.93486931359651));
#129804=CARTESIAN_POINT('Ctrl Pts',(-2.12674657908886,3.9200871429414,6.97456213285606));
#129805=CARTESIAN_POINT('Ctrl Pts',(-2.13922555207015,3.92674916804717,
7.01431038548526));
#129806=CARTESIAN_POINT('Ctrl Pts',(-2.1641397865704,3.93976378656247,7.09382092338471));
#129807=CARTESIAN_POINT('Ctrl Pts',(-2.17658865449891,3.94612348023444,
7.13362664806682));
#129808=CARTESIAN_POINT('Ctrl Pts',(-2.18901737207597,3.95233945645758,
7.17343722318243));
#129809=CARTESIAN_POINT('Ctrl Pts',(-2.726480643,4.042807359,6.986866487));
#129810=CARTESIAN_POINT('Ctrl Pts',(-2.343268848,3.977102825,7.136406991));
#129811=CARTESIAN_POINT('Ctrl Pts',(-1.946001096,3.912499672,7.243140185));
#129812=CARTESIAN_POINT('Ctrl Pts',(-2.855679535,4.042807359,6.66390234));
#129813=CARTESIAN_POINT('Ctrl Pts',(-2.4901815,3.977102825,6.820529074));
#129814=CARTESIAN_POINT('Ctrl Pts',(-2.109746259,3.912499672,6.936243271));
#129815=CARTESIAN_POINT('',(-2.72648063280564,4.04280736030989,6.98686646784853));
#129816=CARTESIAN_POINT('Origin',(0.0854978739401674,4.16063868872144,-0.167226751539388));
#129817=CARTESIAN_POINT('',(-2.79172606251171,4.04280736269456,6.82376960133532));
#129818=CARTESIAN_POINT('Origin',(-4.35849273339173E-14,4.13463032199956,
3.13984949151802E-13));
#129819=CARTESIAN_POINT('',(-2.19152447942122,4.13354310062559,7.17267177917869));
#129820=CARTESIAN_POINT('Origin',(0.0602927793603003,4.16070813241699,-0.182368014149964));
#129821=CARTESIAN_POINT('Origin',(0.0735723243195169,4.0178646340646,-0.177487496657471));
#129822=CARTESIAN_POINT('Ctrl Pts',(-3.89542532178459,3.912491975,6.40963654487194));
#129823=CARTESIAN_POINT('Ctrl Pts',(-3.54777090689269,3.97753138,6.62092181788924));
#129824=CARTESIAN_POINT('Ctrl Pts',(-3.17930331128518,4.042807359,6.79336511074186));
#129825=CARTESIAN_POINT('Ctrl Pts',(-3.16662435976257,4.04505350217026,
6.79929887581794));
#129826=CARTESIAN_POINT('Ctrl Pts',(-3.15394540823987,4.04729964534048,
6.80523264089403));
#129827=CARTESIAN_POINT('Ctrl Pts',(-3.559697347,3.912491975,6.315936573));
#129828=CARTESIAN_POINT('Ctrl Pts',(-3.217125156,3.97753138,6.509012185));
#129829=CARTESIAN_POINT('Ctrl Pts',(-2.855679535,4.042807359,6.66390234));
#129830=CARTESIAN_POINT('Ctrl Pts',(-2.84324220927218,4.04505350217026,
6.66923210248114));
#129831=CARTESIAN_POINT('Ctrl Pts',(-2.8308048835443,4.04729964534049,6.67456186496213));
#129832=CARTESIAN_POINT('',(-3.17864374056489,4.04280735814475,6.79310128093997));
#129833=CARTESIAN_POINT('',(-3.0171615997571,4.04280735744341,6.72850178992045));
#129834=CARTESIAN_POINT('',(-3.67991631910299,3.95233946528539,6.53515221828794));
#129835=CARTESIAN_POINT('Origin',(0.085397309970424,4.01785666792284,-0.173056431550604));
#129836=CARTESIAN_POINT('Ctrl Pts',(-3.555619897094,3.91326598481269,6.31823291346998));
#129837=CARTESIAN_POINT('Ctrl Pts',(-3.57634910582588,3.92008713877303,
6.35431307523612));
#129838=CARTESIAN_POINT('Ctrl Pts',(-3.59708101209336,3.92674915953913,
6.39044940039092));
#129839=CARTESIAN_POINT('Ctrl Pts',(-3.63850520916451,3.93976378698617,
6.46274525194019));
#129840=CARTESIAN_POINT('Ctrl Pts',(-3.65922008492869,3.94612348103791,
6.49894420465417));
#129841=CARTESIAN_POINT('Ctrl Pts',(-3.67991632022434,3.95233945646779,
6.53515221916074));
#129842=CARTESIAN_POINT('Ctrl Pts',(-4.164706805,4.042807359,6.237404687));
#129843=CARTESIAN_POINT('Ctrl Pts',(-3.822601077,3.977102825,6.465828226));
#129844=CARTESIAN_POINT('Ctrl Pts',(-3.457565706,3.912499672,6.65546688));
#129845=CARTESIAN_POINT('Ctrl Pts',(-4.221457354,4.042807359,5.89421732));
#129846=CARTESIAN_POINT('Ctrl Pts',(-3.898174577,3.977102825,6.125753481));
#129847=CARTESIAN_POINT('Ctrl Pts',(-3.551508834,3.912499672,6.320544676));
#129848=CARTESIAN_POINT('',(-4.16470679092074,4.0428073603099,6.23740467049541));
#129849=CARTESIAN_POINT('Origin',(0.119447674717098,4.16063866399011,-0.144937381015162));
#129850=CARTESIAN_POINT('',(-4.19336581362883,4.04280736269456,6.06409507953821));
#129851=CARTESIAN_POINT('Origin',(2.72568426162856E-13,4.13463032200044,
-2.20309881449055E-13));
#129852=CARTESIAN_POINT('',(-3.6822002655948,4.13354310057997,6.5338657166798));
#129853=CARTESIAN_POINT('Origin',(0.0980868956556286,4.16070812044129,-0.165143190232435));
#129854=CARTESIAN_POINT('Origin',(0.1100067681996,4.01786468285577,-0.157521998228017));
#129855=CARTESIAN_POINT('Ctrl Pts',(-5.18223483131303,3.912491975,5.42238150830926));
#129856=CARTESIAN_POINT('Ctrl Pts',(-4.88812847245207,3.97753138,5.70346247143213));
#129857=CARTESIAN_POINT('Ctrl Pts',(-4.56534565464645,4.042807359,5.95108377760583));
#129858=CARTESIAN_POINT('Ctrl Pts',(-4.55423871405474,4.04505350216756,
5.9596044143473));
#129859=CARTESIAN_POINT('Ctrl Pts',(-4.54313177346315,4.0472996453351,5.96812505108879));
#129860=CARTESIAN_POINT('Ctrl Pts',(-4.834213266,3.912491975,5.403043781));
#129861=CARTESIAN_POINT('Ctrl Pts',(-4.541155773,3.97753138,5.665248286));
#129862=CARTESIAN_POINT('Ctrl Pts',(-4.221457354,4.042807359,5.89421732));
#129863=CARTESIAN_POINT('Ctrl Pts',(-4.2104565474167,4.04505350216756,5.90209613299033));
#129864=CARTESIAN_POINT('Ctrl Pts',(-4.19945574083342,4.04729964533509,
5.90997494598055));
#129865=CARTESIAN_POINT('',(-4.56464478872052,4.04280735814476,5.95096790420922));
#129866=CARTESIAN_POINT('',(-4.39305102980428,4.04280735744341,5.92259260020826));
#129867=CARTESIAN_POINT('',(-4.99874646950625,3.95233946528412,5.59129076012302));
#129868=CARTESIAN_POINT('Origin',(0.120602791296842,4.0178566388305,-0.150652566420965));
#129869=CARTESIAN_POINT('Ctrl Pts',(-4.83072478992622,3.91326598477064,
5.406162965312));
#129870=CARTESIAN_POINT('Ctrl Pts',(-4.8587255272726,3.92008713815959,5.43694342298863));
#129871=CARTESIAN_POINT('Ctrl Pts',(-4.88674097220958,3.92674915833406,
5.46777815080322));
#129872=CARTESIAN_POINT('Ctrl Pts',(-4.94273817031434,3.93976378685885,
5.52947879248528));
#129873=CARTESIAN_POINT('Ctrl Pts',(-4.97075044803058,3.94612348078679,
5.5603783471148));
#129874=CARTESIAN_POINT('Ctrl Pts',(-4.99874647078695,3.95233945646387,
5.59129076073675));
#129875=CARTESIAN_POINT('Ctrl Pts',(-5.408195905,4.042807359,5.19628877700001));
#129876=CARTESIAN_POINT('Ctrl Pts',(-5.123192728,3.977102825,5.492914519));
#129877=CARTESIAN_POINT('Ctrl Pts',(-4.807458386,3.912499672,5.756591341));
#129878=CARTESIAN_POINT('Ctrl Pts',(-5.389844518,4.042807359,4.848925249));
#129879=CARTESIAN_POINT('Ctrl Pts',(-5.12389334400001,3.977102825,5.144544464));
#129880=CARTESIAN_POINT('Ctrl Pts',(-4.827206802,3.912499672,5.409304437));
#129881=CARTESIAN_POINT('',(-5.4081958877456,4.04280736030966,5.19628876383342));
#129882=CARTESIAN_POINT('Origin',(0.147812296518153,4.16063868253327,-0.115871092322576));
#129883=CARTESIAN_POINT('',(-5.39892843915143,4.04280736269456,5.02087021193417));
#129884=CARTESIAN_POINT('Origin',(9.61036805691151E-13,4.13463032200111,
-9.48026379621325E-13));
#129885=CARTESIAN_POINT('',(-5.00070045828517,4.13354310060792,5.58954335523504));
#129886=CARTESIAN_POINT('Origin',(0.131294733959384,4.16070811736415,-0.140196623117392));
#129887=CARTESIAN_POINT('Origin',(0.141297377257072,4.01786463695052,-0.13019094599066));
#129888=CARTESIAN_POINT('Ctrl Pts',(-6.22672880104064,3.912491975,4.18158193873128));
#129889=CARTESIAN_POINT('Ctrl Pts',(-5.99992258317702,3.97753138,4.51931555890433));
#129890=CARTESIAN_POINT('Ctrl Pts',(-5.73791750913712,4.042807359,4.83053638071154));
#129891=CARTESIAN_POINT('Ctrl Pts',(-5.72890192760565,4.04505350218207,
4.84124547366929));
#129892=CARTESIAN_POINT('Ctrl Pts',(-5.71988634607416,4.04729964536412,
4.85195456662708));
#129893=CARTESIAN_POINT('Ctrl Pts',(-5.882686747,3.912491975,4.237510666));
#129894=CARTESIAN_POINT('Ctrl Pts',(-5.652846992,3.97753138,4.556583674));
#129895=CARTESIAN_POINT('Ctrl Pts',(-5.389844518,4.042807359,4.848925249));
#129896=CARTESIAN_POINT('Ctrl Pts',(-5.38079461598564,4.04505350218207,
4.85898470801665));
#129897=CARTESIAN_POINT('Ctrl Pts',(-5.37174471397128,4.04729964536412,
4.86904416703315));
#129898=CARTESIAN_POINT('',(-5.73720811971194,4.04280735814475,4.83057388182148));
#129899=CARTESIAN_POINT('',(-5.56352627571132,4.04280735744341,4.83974956272915));
#129900=CARTESIAN_POINT('',(-6.08384079109198,3.95233946527227,4.38598675996371));
#129901=CARTESIAN_POINT('Origin',(0.150168970924535,4.01785667742024,-0.121204340528558));
#129902=CARTESIAN_POINT('Ctrl Pts',(-5.87995036175847,3.9132659847659,4.24130684477094));
#129903=CARTESIAN_POINT('Ctrl Pts',(-5.91391334079663,3.9200871371288,4.26534833799181));
#129904=CARTESIAN_POINT('Ctrl Pts',(-5.94790234940561,3.92674915624501,
4.2894396703587));
#129905=CARTESIAN_POINT('Ctrl Pts',(-6.01585418149866,3.93976378540211,
4.33766004531525));
#129906=CARTESIAN_POINT('Ctrl Pts',(-6.04985403012971,3.9461234778491,4.36181536781961));
#129907=CARTESIAN_POINT('Ctrl Pts',(-6.0838407924566,3.95233945642855,4.38598676031923));
#129908=CARTESIAN_POINT('Ctrl Pts',(-6.398803776,4.042807359,3.912200178));
#129909=CARTESIAN_POINT('Ctrl Pts',(-6.184229582,3.977102825,4.263158233));
#129910=CARTESIAN_POINT('Ctrl Pts',(-5.932559655,3.912499672,4.58854398900001));
#129911=CARTESIAN_POINT('Ctrl Pts',(-6.306208544,4.042807359,3.576902822));
#129912=CARTESIAN_POINT('Ctrl Pts',(-6.110024554,3.977102825,3.922782265));
#129913=CARTESIAN_POINT('Ctrl Pts',(-5.877189946,3.912499672,4.245131134));
#129914=CARTESIAN_POINT('',(-6.39880375628837,4.04280736030989,3.91220016894969));
#129915=CARTESIAN_POINT('Origin',(0.169265304818327,4.16063873557015,-0.0813867475649099));
#129916=CARTESIAN_POINT('',(-6.35204317234975,4.04280736269456,3.74287503272014));
#129917=CARTESIAN_POINT('Origin',(-1.25767452008319E-14,4.134630322,-9.84455572616838E-14));
#129918=CARTESIAN_POINT('',(-6.08537345602736,4.13354310061625,4.38386015920024));
#129919=CARTESIAN_POINT('Origin',(0.158363050465506,4.16070812830415,-0.108694257231567));
#129920=CARTESIAN_POINT('Origin',(0.165981115668196,4.01786465600101,-0.0967723840180312));
#129921=CARTESIAN_POINT('Ctrl Pts',(-6.98006785221684,3.912491975,2.7452562455473));
#129922=CARTESIAN_POINT('Ctrl Pts',(-6.83116698223101,3.97753138,3.12385047328293));
#129923=CARTESIAN_POINT('Ctrl Pts',(-6.64219071889822,4.042807359,3.48411847140535));
#129924=CARTESIAN_POINT('Ctrl Pts',(-6.63568805525163,4.04505350213012,
3.49651527496737));
#129925=CARTESIAN_POINT('Ctrl Pts',(-6.6291853916049,4.0472996452602,3.50891207852946));
#129926=CARTESIAN_POINT('Ctrl Pts',(-6.656092333,3.912491975,2.873836261));
#129927=CARTESIAN_POINT('Ctrl Pts',(-6.500217369,3.97753138,3.234858274));
#129928=CARTESIAN_POINT('Ctrl Pts',(-6.306208544,4.042807359,3.576902822));
#129929=CARTESIAN_POINT('Ctrl Pts',(-6.2995327101614,4.04505350213012,3.58867255756663));
#129930=CARTESIAN_POINT('Ctrl Pts',(-6.2928568763229,4.04729964526021,3.60044229313331));
#129931=CARTESIAN_POINT('',(-6.64150597624777,4.04280735814476,3.4843075935145));
#129932=CARTESIAN_POINT('',(-6.47385721741239,4.04280735744341,3.53060521441202));
#129933=CARTESIAN_POINT('',(-6.88446147873679,3.95233946528909,2.97559889404972));
#129934=CARTESIAN_POINT('Origin',(0.17271367438223,4.0178566438613,-0.0860888581960229));
#129935=CARTESIAN_POINT('Ctrl Pts',(-6.65423598875174,3.91326598480925,
2.8781319295331));
#129936=CARTESIAN_POINT('Ctrl Pts',(-6.69257316711119,3.9200871415113,2.89431032003077));
#129937=CARTESIAN_POINT('Ctrl Pts',(-6.73094648359607,3.9267491651031,2.91053179016838));
#129938=CARTESIAN_POINT('Ctrl Pts',(-6.80767555484976,3.93976378744888,
2.94301714747179));
#129939=CARTESIAN_POINT('Ctrl Pts',(-6.84607319970337,3.94612348197739,
2.95929877525651));
#129940=CARTESIAN_POINT('Ctrl Pts',(-6.88446148016122,3.95233945647872,
2.97559889405487));
#129941=CARTESIAN_POINT('Ctrl Pts',(-7.090210694,4.042807359,2.445181447));
#129942=CARTESIAN_POINT('Ctrl Pts',(-6.956098733,3.977102825,2.834061408));
#129943=CARTESIAN_POINT('Ctrl Pts',(-6.78026102800001,3.912499672,3.20594142));
#129944=CARTESIAN_POINT('Ctrl Pts',(-6.927701267,4.042807359,2.137628395));
#129945=CARTESIAN_POINT('Ctrl Pts',(-6.810457805,3.977102825,2.517595128));
#129946=CARTESIAN_POINT('Ctrl Pts',(-6.65236221900001,3.912499672,2.882460217));
#129947=CARTESIAN_POINT('',(-7.09021067281184,4.04280736030966,2.44518144232082));
#129948=CARTESIAN_POINT('Origin',(0.182803577580881,4.1606386766149,-0.043096885077048));
#129949=CARTESIAN_POINT('',(-7.00814342633534,4.04280736269456,2.2898671772543));
#129950=CARTESIAN_POINT('Origin',(2.70183181383388E-13,4.13463032199933,
-3.4477629085039E-14));
#129951=CARTESIAN_POINT('',(-6.88550115512097,4.13354310058775,2.97319253349686));
#129952=CARTESIAN_POINT('Origin',(0.178026526882995,4.16070809325089,-0.0721096142243627));
#129953=CARTESIAN_POINT('Origin',(0.182903650094188,4.01786467042396,-0.0588288152680649));
#129954=CARTESIAN_POINT('Ctrl Pts',(-7.4070266874212,3.912491975,1.18056542085387));
#129955=CARTESIAN_POINT('Ctrl Pts',(-7.34299360664207,3.97753138,1.58231761241509));
#129956=CARTESIAN_POINT('Ctrl Pts',(-7.23588247237805,4.042807359,1.97478705503451));
#129957=CARTESIAN_POINT('Ctrl Pts',(-7.2321967832453,4.04505350239193,1.98829191024431));
#129958=CARTESIAN_POINT('Ctrl Pts',(-7.22851109411266,4.04729964578383,
2.00179676545403));
#129959=CARTESIAN_POINT('Ctrl Pts',(-7.118266439,3.912491975,1.375784468));
#129960=CARTESIAN_POINT('Ctrl Pts',(-7.043644806,3.97753138,1.761874495));
#129961=CARTESIAN_POINT('Ctrl Pts',(-6.927701267,4.042807359,2.137628395));
#129962=CARTESIAN_POINT('Ctrl Pts',(-6.92371165523237,4.04505350239193,
2.15055806916811));
#129963=CARTESIAN_POINT('Ctrl Pts',(-6.91972204346475,4.04729964578383,
2.1634877433363));
#129964=CARTESIAN_POINT('',(-7.23525439422029,4.04280735814475,1.97511895503816));
#129965=CARTESIAN_POINT('',(-7.08147779032799,4.04280735744341,2.05637369070155));
#129966=CARTESIAN_POINT('',(-7.36317239935864,3.95233946528238,1.42607533064351));
#129967=CARTESIAN_POINT('Origin',(0.187181807889715,4.01785668190154,-0.0469477129738381));
#129968=CARTESIAN_POINT('Ctrl Pts',(-7.11737693710714,3.91326598474417,
1.38037876477042));
#129969=CARTESIAN_POINT('Ctrl Pts',(-7.15829567884329,3.92008713974062,
1.38793755120874));
#129970=CARTESIAN_POINT('Ctrl Pts',(-7.19925897335171,3.92674916156521,
1.39553064136023));
#129971=CARTESIAN_POINT('Ctrl Pts',(-7.28117757015847,3.93976378662875,
1.41076202997068));
#129972=CARTESIAN_POINT('Ctrl Pts',(-7.32217756234829,3.94612348031645,
1.41840864270744));
#129973=CARTESIAN_POINT('Ctrl Pts',(-7.36317240074903,3.95233945645877,
1.42607533036288));
#129974=CARTESIAN_POINT('Ctrl Pts',(-7.450087241,4.042807359,0.86382875));
#129975=CARTESIAN_POINT('Ctrl Pts',(-7.402708438,3.977102825,1.27244702));
#129976=CARTESIAN_POINT('Ctrl Pts',(-7.310924932,3.912499672,1.673432593));
#129977=CARTESIAN_POINT('Ctrl Pts',(-7.225262378,4.042807359,0.59840084));
#129978=CARTESIAN_POINT('Ctrl Pts',(-7.192441619,3.977102825,0.994688041));
#129979=CARTESIAN_POINT('Ctrl Pts',(-7.116477429,3.912499672,1.385008664));
#129980=CARTESIAN_POINT('',(-7.45008721928956,4.04280736030965,0.863828749933751));
#129981=CARTESIAN_POINT('Origin',(0.187794765762662,4.1606387163103,-0.00279201758977748));
#129982=CARTESIAN_POINT('',(-7.33655068294462,4.04280736269456,0.729787677972479));
#129983=CARTESIAN_POINT('Origin',(1.0698907038087E-12,4.13463032200044,
-2.8200098506348E-13));
#129984=CARTESIAN_POINT('',(-7.36367047205426,4.13354310059326,1.42350172983018));
#129985=CARTESIAN_POINT('Origin',(0.189366034920901,4.16070809352831,-0.0321533447766773));
#129986=CARTESIAN_POINT('Origin',(0.191273883476633,4.01786465346802,-0.0181345584468363));
#129987=CARTESIAN_POINT('Ctrl Pts',(-7.48764118870734,3.912491975,-0.439327330070044));
#129988=CARTESIAN_POINT('Ctrl Pts',(-7.5114700099638,3.97753138,-0.0332026624065126));
#129989=CARTESIAN_POINT('Ctrl Pts',(-7.49123240398283,4.042807359,0.373116790603217));
#129990=CARTESIAN_POINT('Ctrl Pts',(-7.49053602896029,4.04505350221427,
0.387098222918463));
#129991=CARTESIAN_POINT('Ctrl Pts',(-7.4898396539377,4.04729964542849,0.401079655233702));
#129992=CARTESIAN_POINT('Ctrl Pts',(-7.24759831800001,3.912491975,-0.186597478));
#129993=CARTESIAN_POINT('Ctrl Pts',(-7.257719241,3.97753138,0.206507424));
#129994=CARTESIAN_POINT('Ctrl Pts',(-7.225262378,4.042807359,0.59840084));
#129995=CARTESIAN_POINT('Ctrl Pts',(-7.22414553894681,4.04505350221427,
0.611885873094053));
#129996=CARTESIAN_POINT('Ctrl Pts',(-7.22302869989349,4.0472996454285,0.625370906188109));
#129997=CARTESIAN_POINT('',(-7.49069035867608,4.04280735814475,0.373575949174865));
#129998=CARTESIAN_POINT('',(-7.35797633236851,4.04280735744341,0.485988418560827));
#129999=CARTESIAN_POINT('',(-7.49758956224147,3.95233946528052,-0.190129930137772));
#130000=CARTESIAN_POINT('Origin',(0.192898267892459,4.01785666442251,-0.00561154578427628));
#130001=CARTESIAN_POINT('Ctrl Pts',(-7.24771725059274,3.91326598480197,
-0.181919376803831));
#130002=CARTESIAN_POINT('Ctrl Pts',(-7.28930422197603,3.92008713508906,
-0.183333629475567));
#130003=CARTESIAN_POINT('Ctrl Pts',(-7.33094207501763,3.92674915206884,
-0.18472395798091));
#130004=CARTESIAN_POINT('Ctrl Pts',(-7.4142198183722,3.93976378642255,-0.187458749621351));
#130005=CARTESIAN_POINT('Ctrl Pts',(-7.4559050477043,3.94612347989405,-0.188804696837706));
#130006=CARTESIAN_POINT('Ctrl Pts',(-7.49758956353974,3.95233945645325,
-0.190129930705654));
#130007=CARTESIAN_POINT('Ctrl Pts',(-7.461605988,4.042807359,-0.757915620000001));
#130008=CARTESIAN_POINT('Ctrl Pts',(-7.50317572500001,3.977102825,-0.348665576));
#130009=CARTESIAN_POINT('Ctrl Pts',(-7.499738111,3.912499672,0.062675918));
#130010=CARTESIAN_POINT('Ctrl Pts',(-7.18497825100001,4.042807359,-0.968807273));
#130011=CARTESIAN_POINT('Ctrl Pts',(-7.238114857,3.977102825,-0.574729554));
#130012=CARTESIAN_POINT('Ctrl Pts',(-7.24783406400001,3.912499672,-0.177204354));
#130013=CARTESIAN_POINT('',(-7.46160596678344,4.04280736030965,-0.757915615395764));
#130014=CARTESIAN_POINT('Origin',(0.184004250522272,4.16063871261539,0.0376435729130676));
#130015=CARTESIAN_POINT('',(-7.32190898346867,4.04280736269456,-0.864415882287469));
#130016=CARTESIAN_POINT('Origin',(1.65839564303383E-12,4.134630322,3.6239457615328E-14));
#130017=CARTESIAN_POINT('',(-7.49752274183165,4.13354310057391,-0.192750432608097));
#130018=CARTESIAN_POINT('Origin',(0.19185085619743,4.1607081097785,0.00930648937395421));
#130019=CARTESIAN_POINT('Origin',(0.190700775333477,4.01786464775998,0.0234076710092347));
#130020=CARTESIAN_POINT('Ctrl Pts',(-7.21814190835588,3.912491975,-2.03867762420809));
#130021=CARTESIAN_POINT('Ctrl Pts',(-7.32871842420211,3.97753138,-1.64717041730805));
#130022=CARTESIAN_POINT('Ctrl Pts',(-7.39630063392665,4.042807359,-1.24600000080534));
#130023=CARTESIAN_POINT('Ctrl Pts',(-7.39862613459791,4.04505350238006,
-1.23219574556317));
#130024=CARTESIAN_POINT('Ctrl Pts',(-7.40095163526915,4.04729964576008,
-1.21839149032102));
#130025=CARTESIAN_POINT('Ctrl Pts',(-7.038040555,3.912491975,-1.740254334));
#130026=CARTESIAN_POINT('Ctrl Pts',(-7.13243079,3.97753138,-1.358515705));
#130027=CARTESIAN_POINT('Ctrl Pts',(-7.184978251,4.042807359,-0.968807273));
#130028=CARTESIAN_POINT('Ctrl Pts',(-7.18678640667185,4.04505350238006,
-0.955397424107718));
#130029=CARTESIAN_POINT('Ctrl Pts',(-7.18859456234357,4.04729964576008,
-0.941987575215448));
#130030=CARTESIAN_POINT('',(-7.39586996682337,4.04280735814475,-1.24543505334257));
#130031=CARTESIAN_POINT('',(-7.29042407893858,4.04280735744341,-1.10712113202695));
#130032=CARTESIAN_POINT('',(-7.28142776983371,3.95233946530271,-1.79744492687227));
#130033=CARTESIAN_POINT('Origin',(0.189594772458952,4.01785666382256,0.0359870838592783));
#130034=CARTESIAN_POINT('Ctrl Pts',(-7.03916236014506,3.91326598479388,
-1.73571117070117));
#130035=CARTESIAN_POINT('Ctrl Pts',(-7.07947305393982,3.92008713936462,
-1.74603233504673));
#130036=CARTESIAN_POINT('Ctrl Pts',(-7.11983858613362,3.92674916075612,
-1.75634107334237));
#130037=CARTESIAN_POINT('Ctrl Pts',(-7.20058140535285,3.93976378909938,
-1.77691417074854));
#130038=CARTESIAN_POINT('Ctrl Pts',(-7.24100273676367,3.94612348529266,
-1.78718974722731));
#130039=CARTESIAN_POINT('Ctrl Pts',(-7.28142777095667,3.95233945651953,
-1.79744492776942));
#130040=CARTESIAN_POINT('Ctrl Pts',(-7.124228332,4.042807359,-2.344220698));
#130041=CARTESIAN_POINT('Ctrl Pts',(-7.252802854,3.977102825,-1.953474957));
#130042=CARTESIAN_POINT('Ctrl Pts',(-7.337871871,3.912499672,-1.551011413));
#130043=CARTESIAN_POINT('Ctrl Pts',(-6.808732526,4.042807359,-2.490715035));
#130044=CARTESIAN_POINT('Ctrl Pts',(-6.945341889,3.977102825,-2.117273434));
#130045=CARTESIAN_POINT('Ctrl Pts',(-7.04029003300001,3.912499672,-1.731131494));
#130046=CARTESIAN_POINT('',(-7.1242283122693,4.04280736030965,-2.34422068894288));
#130047=CARTESIAN_POINT('Origin',(0.17160996885161,4.1606386991441,0.0763189263862812));
#130048=CARTESIAN_POINT('',(-6.96490295739362,4.04280736269456,-2.41820031680348));
#130049=CARTESIAN_POINT('Origin',(-8.32667268468867E-13,4.13463032199911,
-3.12141805458577E-13));
#130050=CARTESIAN_POINT('',(-7.28079918139993,4.13354310058009,-1.79998979899541));
#130051=CARTESIAN_POINT('Origin',(0.185364917121934,4.16070811704502,0.0503311790112895));
#130052=CARTESIAN_POINT('Origin',(0.181210223905396,4.01786465413451,0.0638554106367939));
#130053=CARTESIAN_POINT('Ctrl Pts',(-6.61113033607533,3.912491975,-3.54270161749554));
#130054=CARTESIAN_POINT('Ctrl Pts',(-6.80328411084193,3.97753138,-3.18411831437587));
#130055=CARTESIAN_POINT('Ctrl Pts',(-6.95552606635459,4.042807359,-2.80685521578371));
#130056=CARTESIAN_POINT('Ctrl Pts',(-6.9607647044976,4.04505350220186,-2.79387361126094));
#130057=CARTESIAN_POINT('Ctrl Pts',(-6.9660033426406,4.0472996454037,-2.7808920067382));
#130058=CARTESIAN_POINT('Ctrl Pts',(-6.499391838,3.912491975,-3.212538831));
#130059=CARTESIAN_POINT('Ctrl Pts',(-6.673637803,3.97753138,-2.860016149));
#130060=CARTESIAN_POINT('Ctrl Pts',(-6.808732526,4.042807359,-2.490715035));
#130061=CARTESIAN_POINT('Ctrl Pts',(-6.81338112872218,4.04505350220186,
-2.47800740197241));
#130062=CARTESIAN_POINT('Ctrl Pts',(-6.81802973144437,4.04729964540369,
-2.46529976894482));
#130063=CARTESIAN_POINT('',(-6.95522691503914,4.04280735814474,-2.80621089584825));
#130064=CARTESIAN_POINT('',(-6.88197969794138,4.04280735744339,-2.64846292855763));
#130065=CARTESIAN_POINT('',(-6.7247945077253,3.95233946527634,-3.32071339609417));
#130066=CARTESIAN_POINT('Origin',(0.177425631813312,4.01785665619084,0.0759028331350597));
#130067=CARTESIAN_POINT('Ctrl Pts',(-6.50146406158771,3.91326598472177,
-3.20834303966903));
#130068=CARTESIAN_POINT('Ctrl Pts',(-6.53861356724024,3.92008713904787,
-3.22708850772555));
#130069=CARTESIAN_POINT('Ctrl Pts',(-6.5758193002426,3.92674916019177,-3.24583362881935));
#130070=CARTESIAN_POINT('Ctrl Pts',(-6.65025177415825,3.93976378587443,
-3.28328305016212));
#130071=CARTESIAN_POINT('Ctrl Pts',(-6.68751911182413,3.94612347883912,
-3.30200777054742));
#130072=CARTESIAN_POINT('Ctrl Pts',(-6.72479450867199,3.95233945644068,
-3.32071339714379));
#130073=CARTESIAN_POINT('Ctrl Pts',(-6.453729677,4.042807359,-3.820912621));
#130074=CARTESIAN_POINT('Ctrl Pts',(-6.663296982,3.977102825,-3.46694202));
#130075=CARTESIAN_POINT('Ctrl Pts',(-6.83289489800001,3.912499672,-3.092175175));
#130076=CARTESIAN_POINT('Ctrl Pts',(-6.114118036,4.042807359,-3.89615973));
#130077=CARTESIAN_POINT('Ctrl Pts',(-6.327812453,3.977102825,-3.560815961));
#130078=CARTESIAN_POINT('Ctrl Pts',(-6.503549865,3.912499672,-3.20411285));
#130079=CARTESIAN_POINT('',(-6.45372965975711,4.0428073603099,-3.82091260783521));
#130080=CARTESIAN_POINT('Origin',(0.151191584710254,4.16063868549269,0.111425745006766));
#130081=CARTESIAN_POINT('',(-6.28222581014146,4.04280736269456,-3.85891239175924));
#130082=CARTESIAN_POINT('Origin',(3.16153353496773E-13,4.13463032200067,
2.28766658394441E-13));
#130083=CARTESIAN_POINT('',(-6.72363354311164,4.13354310059453,-3.32306364287935));
#130084=CARTESIAN_POINT('Origin',(0.170211178350446,4.16070808827327,0.0890022978908028));
#130085=CARTESIAN_POINT('Origin',(0.163246422937403,4.01786466078058,0.101317255762698));
#130086=CARTESIAN_POINT('Ctrl Pts',(-5.69498965639203,3.912491975,-4.88107282109577));
#130087=CARTESIAN_POINT('Ctrl Pts',(-5.95973579334589,3.97753138,-4.57218037737035));
#130088=CARTESIAN_POINT('Ctrl Pts',(-6.189518831403,4.042807359,-4.23646500152237));
#130089=CARTESIAN_POINT('Ctrl Pts',(-6.19742565445324,4.04505350223037,
-4.22491305193323));
#130090=CARTESIAN_POINT('Ctrl Pts',(-6.20533247750354,4.04729964546071,
-4.21336110234407));
#130091=CARTESIAN_POINT('Ctrl Pts',(-5.65683878100001,3.912491975,-4.534608583));
#130092=CARTESIAN_POINT('Ctrl Pts',(-5.902792929,3.97753138,-4.227785417));
#130093=CARTESIAN_POINT('Ctrl Pts',(-6.11411803600001,4.042807359,-3.89615973));
#130094=CARTESIAN_POINT('Ctrl Pts',(-6.1213897225494,4.04505350223037,-3.88474850640318));
#130095=CARTESIAN_POINT('Ctrl Pts',(-6.12866140909881,4.04729964546071,
-3.87333728280642));
#130096=CARTESIAN_POINT('',(-6.18936518382027,4.04280735814474,-4.23577143670967));
#130097=CARTESIAN_POINT('',(-6.15174159578327,4.04280735744339,-4.0659655425065));
#130098=CARTESIAN_POINT('',(-5.85371732862051,3.95233946527141,-4.68870899803957));
#130099=CARTESIAN_POINT('Origin',(0.156960845813895,4.01785670332497,0.112269676904007));
#130100=CARTESIAN_POINT('Ctrl Pts',(-5.6597645288131,3.91326598485026,-4.53095635367109));
#130101=CARTESIAN_POINT('Ctrl Pts',(-5.69201580768911,3.92008714537315,
-4.55724963271236));
#130102=CARTESIAN_POINT('Ctrl Pts',(-5.72432207755014,3.9267491728499,-4.58355466295653));
#130103=CARTESIAN_POINT('Ctrl Pts',(-5.78896377745649,3.93976378526525,
-4.63612926594674));
#130104=CARTESIAN_POINT('Ctrl Pts',(-5.82133456077178,3.9461234775913,-4.66242758604197));
#130105=CARTESIAN_POINT('Ctrl Pts',(-5.85371732933022,3.95233945642611,
-4.68870899925716));
#130106=CARTESIAN_POINT('Ctrl Pts',(-5.481461795,4.042807359,-5.118942917));
#130107=CARTESIAN_POINT('Ctrl Pts',(-5.762222749,3.977102825,-4.818298728));
#130108=CARTESIAN_POINT('Ctrl Pts',(-6.008419354,3.912499672,-4.488752262));
#130109=CARTESIAN_POINT('Ctrl Pts',(-5.133614182,4.042807359,-5.119424326));
#130110=CARTESIAN_POINT('Ctrl Pts',(-5.41440154,3.977102825,-4.837858691));
#130111=CARTESIAN_POINT('Ctrl Pts',(-5.662710933,3.912499672,-4.527273449));
#130112=CARTESIAN_POINT('',(-5.48146178092909,4.04280736030966,-5.11894290047791));
#130113=CARTESIAN_POINT('Origin',(0.123703542979664,4.16063869601417,0.141322381082165));
#130114=CARTESIAN_POINT('',(-5.30579876615036,4.04280736269456,-5.11918601225676));
#130115=CARTESIAN_POINT('Origin',(-6.67001176513082E-13,4.13463032199978,
-5.13911829758129E-13));
#130116=CARTESIAN_POINT('',(-5.8520782731024,4.13354310059652,-4.69075472387006));
#130117=CARTESIAN_POINT('Origin',(0.147099097435169,4.16070813559084,0.123512037761863));
#130118=CARTESIAN_POINT('Origin',(0.137649683437396,4.01786468222999,0.134041740787689));
#130119=CARTESIAN_POINT('Ctrl Pts',(-4.51255758966453,3.912491975,-5.99121048432391));
#130120=CARTESIAN_POINT('Ctrl Pts',(-4.83751685380577,3.97753138,-5.74645236820935));
#130121=CARTESIAN_POINT('Ctrl Pts',(-5.13409657424069,4.042807359,-5.46798239187965));
#130122=CARTESIAN_POINT('Ctrl Pts',(-5.14430186812406,4.04505350229073,
-5.45840025341797));
#130123=CARTESIAN_POINT('Ctrl Pts',(-5.15450716200743,4.04729964558143,
-5.44881811495625));
#130124=CARTESIAN_POINT('Ctrl Pts',(-4.549778231,3.912491975,-5.64464507700001));
#130125=CARTESIAN_POINT('Ctrl Pts',(-4.855940018,3.97753138,-5.397868138));
#130126=CARTESIAN_POINT('Ctrl Pts',(-5.133614182,4.042807359,-5.119424326));
#130127=CARTESIAN_POINT('Ctrl Pts',(-5.14316893659779,4.04505350229073,
-5.10984308785164));
#130128=CARTESIAN_POINT('Ctrl Pts',(-5.15272369119556,4.04729964558143,
-5.10026184970315));
#130129=CARTESIAN_POINT('',(-5.13409561478568,4.04280735814474,-5.4672720125227));
#130130=CARTESIAN_POINT('',(-5.13385489337812,4.04280735744339,-5.29334812632912));
#130131=CARTESIAN_POINT('',(-4.7089268331995,3.95233946528876,-5.83746577823621));
#130132=CARTESIAN_POINT('Origin',(0.129156504148766,4.01785666691168,0.143386795471282));
#130133=CARTESIAN_POINT('Ctrl Pts',(-4.55342069737005,3.91326598475465,
-5.64170718417175));
#130134=CARTESIAN_POINT('Ctrl Pts',(-4.57926564397507,3.92008713542126,
-5.67431876535296));
#130135=CARTESIAN_POINT('Ctrl Pts',(-4.60516176501408,3.9267491527984,-5.7069536386321));
#130136=CARTESIAN_POINT('Ctrl Pts',(-4.65699028047525,3.93976378738226,
-5.77219524223799));
#130137=CARTESIAN_POINT('Ctrl Pts',(-4.68295090080554,3.94612348186694,
-5.80483749548642));
#130138=CARTESIAN_POINT('Ctrl Pts',(-4.70892683358658,3.95233945647787,
-5.83746577960661));
#130139=CARTESIAN_POINT('Ctrl Pts',(-4.252886852,4.042807359,-6.177617131));
#130140=CARTESIAN_POINT('Ctrl Pts',(-4.591713385,3.977102825,-5.944357142));
#130141=CARTESIAN_POINT('Ctrl Pts',(-4.902996799,3.912499672,-5.675440282));
#130142=CARTESIAN_POINT('Ctrl Pts',(-3.913068234,4.042807359,-6.103310331));
#130143=CARTESIAN_POINT('Ctrl Pts',(-4.247819228,3.977102825,-5.888688526));
#130144=CARTESIAN_POINT('Ctrl Pts',(-4.557089932,3.912499672,-5.638743774));
#130145=CARTESIAN_POINT('',(-4.25288684182705,4.04280736030967,-6.17761711183535));
#130146=CARTESIAN_POINT('Origin',(0.0904312725799133,4.16063868171559,0.164610930327612));
#130147=CARTESIAN_POINT('',(-4.08127846875943,4.04280736269456,-6.14009218447091));
#130148=CARTESIAN_POINT('Origin',(-5.33427468862868E-14,4.13463032200022,
-1.29236898960272E-13));
#130149=CARTESIAN_POINT('',(-4.70688632716557,4.13354310061502,-5.83911132777436));
#130150=CARTESIAN_POINT('Origin',(0.117108542261745,4.16070812578763,0.152246319600126));
#130151=CARTESIAN_POINT('Origin',(0.105616433177164,4.01786462505133,0.160498468657823));
#130152=CARTESIAN_POINT('Ctrl Pts',(-3.11912334532114,3.912491975,-6.82120580448832));
#130153=CARTESIAN_POINT('Ctrl Pts',(-3.48910100211822,3.97753138,-6.65202663257592));
#130154=CARTESIAN_POINT('Ctrl Pts',(-3.83860966710354,4.042807359,-6.44382300225625));
#130155=CARTESIAN_POINT('Ctrl Pts',(-3.85063624307732,4.04505350222721,
-6.43665872557614));
#130156=CARTESIAN_POINT('Ctrl Pts',(-3.86266281905113,4.0472996454544,-6.42949444889594));
#130157=CARTESIAN_POINT('Ctrl Pts',(-3.229975107,3.912491975,-6.490744241));
#130158=CARTESIAN_POINT('Ctrl Pts',(-3.582028749,3.97753138,-6.315552544));
#130159=CARTESIAN_POINT('Ctrl Pts',(-3.913068234,4.042807359,-6.103310331));
#130160=CARTESIAN_POINT('Ctrl Pts',(-3.92445928639878,4.04505350222722,
-6.09600708688845));
#130161=CARTESIAN_POINT('Ctrl Pts',(-3.93585033879756,4.04729964545439,
-6.08870384277701));
#130162=CARTESIAN_POINT('',(-3.83876144062878,4.04280735814475,-6.44312902495228));
#130163=CARTESIAN_POINT('',(-3.87591484165136,4.04280735744339,-6.27321963496368));
#130164=CARTESIAN_POINT('',(-3.34395215217457,3.95233946529221,-6.71326914644803));
#130165=CARTESIAN_POINT('Origin',(0.0953130054425495,4.01785664550041,0.167799374054779));
#130166=CARTESIAN_POINT('Ctrl Pts',(-3.23416397491899,3.91326598485202,
-6.4886580575758));
#130167=CARTESIAN_POINT('Ctrl Pts',(-3.25239416135484,3.92008713785229,
-6.52606311046376));
#130168=CARTESIAN_POINT('Ctrl Pts',(-3.27066931949185,3.92674915763536,
-6.56350191354768));
#130169=CARTESIAN_POINT('Ctrl Pts',(-3.30726108442044,3.9397637878327,-6.63835977825753));
#130170=CARTESIAN_POINT('Ctrl Pts',(-3.3255976415518,3.94612348273404,-6.67581964236287));
#130171=CARTESIAN_POINT('Ctrl Pts',(-3.34395215224815,3.95233945648807,
-6.71326914787331));
#130172=CARTESIAN_POINT('Ctrl Pts',(-2.825451647,4.042807359,-6.947432835));
#130173=CARTESIAN_POINT('Ctrl Pts',(-3.206500606,3.977102825,-6.792464023));
#130174=CARTESIAN_POINT('Ctrl Pts',(-3.568315562,3.912499672,-6.596751022));
#130175=CARTESIAN_POINT('Ctrl Pts',(-2.509551565,4.042807359,-6.801812328));
#130176=CARTESIAN_POINT('Ctrl Pts',(-2.88261361,3.977102825,-6.66416983));
#130177=CARTESIAN_POINT('Ctrl Pts',(-3.238384471,3.912499672,-6.486552707));
#130178=CARTESIAN_POINT('',(-2.82545164113304,4.04280736030965,-6.94743281409805));
#130179=CARTESIAN_POINT('Origin',(0.0529306025410337,4.16063867944897,0.180202534763928));
#130180=CARTESIAN_POINT('',(-2.66592212669213,4.04280736269456,-6.8738944707809));
#130181=CARTESIAN_POINT('Origin',(-5.57279916657549E-14,4.13463032200022,
-6.80878964320897E-14));
#130182=CARTESIAN_POINT('',(-3.34160560861239,4.13354310063453,-6.71443757508186));
#130183=CARTESIAN_POINT('Origin',(0.081642032993165,4.16070809414406,0.173861515886751));
#130184=CARTESIAN_POINT('Origin',(0.0686448621175723,4.01786462420063,0.179450723692286));
#130185=CARTESIAN_POINT('Ctrl Pts',(-1.57984236089796,3.912491975,-7.33224912145048));
#130186=CARTESIAN_POINT('Ctrl Pts',(-1.97753866607176,3.97753138,-7.24655952471014));
#130187=CARTESIAN_POINT('Ctrl Pts',(-2.36363363937118,4.042807359,-7.11835761149783));
#130188=CARTESIAN_POINT('Ctrl Pts',(-2.37691914846762,4.04505350223615,
-7.11394618995146));
#130189=CARTESIAN_POINT('Ctrl Pts',(-2.39020465756409,4.04729964547227,
-7.10953476840506));
#130190=CARTESIAN_POINT('Ctrl Pts',(-1.759141937,3.912491975,-7.033343419));
#130191=CARTESIAN_POINT('Ctrl Pts',(-2.140625797,3.97753138,-6.937928732));
#130192=CARTESIAN_POINT('Ctrl Pts',(-2.509551565,4.042807359,-6.801812328));
#130193=CARTESIAN_POINT('Ctrl Pts',(-2.52224628258409,4.04505350223615,
-6.79712856921376));
#130194=CARTESIAN_POINT('Ctrl Pts',(-2.5349410001682,4.04729964547226,-6.79244481042748));
#130195=CARTESIAN_POINT('',(-2.36393104912808,4.04280735814475,-7.1177124858181));
#130196=CARTESIAN_POINT('',(-2.43674132054344,4.04280735744339,-6.95976236583373));
#130197=CARTESIAN_POINT('',(-1.82261798542014,3.95233946528193,-7.27516751064553));
#130198=CARTESIAN_POINT('Origin',(0.0570127704426948,4.01785664805416,0.184365935620861));
#130199=CARTESIAN_POINT('Ctrl Pts',(-1.76368133957539,3.91326598486179,
-7.03220649175487));
#130200=CARTESIAN_POINT('Ctrl Pts',(-1.77344433390099,3.92008713797502,
-7.07265598703867));
#130201=CARTESIAN_POINT('Ctrl Pts',(-1.78324399318066,3.92674915786431,
-7.11314811114959));
#130202=CARTESIAN_POINT('Ctrl Pts',(-1.80288803263736,3.93976378662721,
-7.19412197946823));
#130203=CARTESIAN_POINT('Ctrl Pts',(-1.81274312564909,3.94612348027624,
-7.23464786204897));
#130204=CARTESIAN_POINT('Ctrl Pts',(-1.8226179852158,3.95233945645733,-7.27516751204908));
#130205=CARTESIAN_POINT('Ctrl Pts',(-1.265901463,4.042807359,-7.3923943));
#130206=CARTESIAN_POINT('Ctrl Pts',(-1.671355422,3.977102825,-7.322962836));
#130207=CARTESIAN_POINT('Ctrl Pts',(-2.066783856,3.912499672,-7.209605016));
#130208=CARTESIAN_POINT('Ctrl Pts',(-0.988691053000001,4.042807359,-7.18226914));
#130209=CARTESIAN_POINT('Ctrl Pts',(-1.382620184,3.977102825,-7.128041959));
#130210=CARTESIAN_POINT('Ctrl Pts',(-1.768255751,3.912499672,-7.031057645));
#130211=CARTESIAN_POINT('',(-1.26590146178554,4.04280736030965,-7.39239427832976));
#130212=CARTESIAN_POINT('Origin',(0.0129548444620933,4.1606387157555,0.187367821990734));
#130213=CARTESIAN_POINT('',(-1.12591022831811,4.04280736269456,-7.28628109074357));
#130214=CARTESIAN_POINT('Origin',(-4.87890977618477E-13,4.134630322,-1.20996962449382E-12));
#130215=CARTESIAN_POINT('',(-1.82007512463073,4.1335431006253,-7.27580418518327));
#130216=CARTESIAN_POINT('Origin',(0.0423581923295008,4.16070811576174,0.187347329555972));
#130217=CARTESIAN_POINT('Origin',(0.0284633256112127,4.01786458818801,0.190011699064334));
#130218=CARTESIAN_POINT('Ctrl Pts',(0.0333102964695516,3.912491975,-7.50044461904883));
#130219=CARTESIAN_POINT('Ctrl Pts',(-0.373508820894604,3.97753138,-7.50225134757834));
#130220=CARTESIAN_POINT('Ctrl Pts',(-0.778136729128367,4.042807359,-7.46004573014145));
#130221=CARTESIAN_POINT('Ctrl Pts',(-0.792059962488441,4.04505350334628,
-7.45859343619753));
#130222=CARTESIAN_POINT('Ctrl Pts',(-0.805983195848512,4.04729964769253,
-7.45714114225351));
#130223=CARTESIAN_POINT('Ctrl Pts',(-0.206053246,3.912491975,-7.247071275));
#130224=CARTESIAN_POINT('Ctrl Pts',(-0.599129562,3.97753138,-7.235895084));
#130225=CARTESIAN_POINT('Ctrl Pts',(-0.988691053,4.042807359,-7.18226914));
#130226=CARTESIAN_POINT('Ctrl Pts',(-1.00209585142571,4.04505350334628,
-7.18042387298486));
#130227=CARTESIAN_POINT('Ctrl Pts',(-1.01550064985142,4.04729964769254,
-7.17857860596984));
#130228=CARTESIAN_POINT('',(-0.883628482512665,4.04280735744339,-7.32087434385182));
#130229=CARTESIAN_POINT('Ctrl Pts',(-0.210730925519537,3.91326598472829,
-7.24693676511879));
#130230=CARTESIAN_POINT('Ctrl Pts',(-0.211570220743726,3.92008714020356,
-7.28853934331192));
#130231=CARTESIAN_POINT('Ctrl Pts',(-0.212436159929306,3.9267491625338,
-7.33019143747321));
#130232=CARTESIAN_POINT('Ctrl Pts',(-0.214213943682518,3.93976378611332,
-7.41349503639186));
#130233=CARTESIAN_POINT('Ctrl Pts',(-0.215126763178154,3.94612347931079,
-7.45519199686624));
#130234=CARTESIAN_POINT('Ctrl Pts',(-0.216060227165054,3.95233945644668,
-7.49688712928287));
#130235=CARTESIAN_POINT('Ctrl Pts',(0.352840867,4.042807359,-7.491695624));
#130236=CARTESIAN_POINT('Ctrl Pts',(-0.058059517,3.977102825,-7.511048045));
#130237=CARTESIAN_POINT('Ctrl Pts',(-0.468611634,3.912499672,-7.48534589300001));
#130238=CARTESIAN_POINT('Ctrl Pts',(0.578399553,4.042807359,-7.22689103));
#130239=CARTESIAN_POINT('Ctrl Pts',(0.182023025,3.977102825,-7.258614769));
#130240=CARTESIAN_POINT('Ctrl Pts',(-0.215445357,3.912499672,-7.246798141));
#130241=CARTESIAN_POINT('',(0.466747980841814,4.04280736269456,-7.35796930546287));
#130242=CARTESIAN_POINT('Ctrl Pts',(1.64490540305164,3.912491975,-7.31792766371014));
#130243=CARTESIAN_POINT('Ctrl Pts',(1.24798588321235,3.97753138,-7.40714623621052));
#130244=CARTESIAN_POINT('Ctrl Pts',(0.843744989901137,4.042807359,-7.45291040216964));
#130245=CARTESIAN_POINT('Ctrl Pts',(0.829835080901927,4.04505350218529,
-7.45448514484029));
#130246=CARTESIAN_POINT('Ctrl Pts',(0.815925171902729,4.04729964537055,
-7.45605988751085));
#130247=CARTESIAN_POINT('Ctrl Pts',(1.356670267,3.912491975,-7.121934132));
#130248=CARTESIAN_POINT('Ctrl Pts',(0.970381306,3.97753138,-7.195519024));
#130249=CARTESIAN_POINT('Ctrl Pts',(0.578399553,4.042807359,-7.22689103));
#130250=CARTESIAN_POINT('Ctrl Pts',(0.564911480408142,4.04505350218529,
-7.22797053916349));
#130251=CARTESIAN_POINT('Ctrl Pts',(0.551423407816283,4.04729964537055,
-7.22905004832698));
#130252=CARTESIAN_POINT('',(0.843204186876859,4.04280735814475,-7.45244978107983));
#130253=CARTESIAN_POINT('',(0.710801840462912,4.04280735744339,-7.33967037392361));
#130254=CARTESIAN_POINT('',(1.40060026653628,3.95233946528707,-7.36806063541257));
#130255=CARTESIAN_POINT('Origin',(-0.0256698380379148,4.01785665389522,
0.191264910989279));
#130256=CARTESIAN_POINT('Ctrl Pts',(1.35207303361503,3.91326598486611,-7.12280833059856));
#130257=CARTESIAN_POINT('Ctrl Pts',(1.36019668436733,3.92008713977612,-7.16361868414385));
#130258=CARTESIAN_POINT('Ctrl Pts',(1.36830495852077,3.92674916152212,-7.2044831231636));
#130259=CARTESIAN_POINT('Ctrl Pts',(1.3844765521872,3.93976378721589,-7.28622131472965));
#130260=CARTESIAN_POINT('Ctrl Pts',(1.39254868926144,3.9461234814825,-7.32713966009896));
#130261=CARTESIAN_POINT('Ctrl Pts',(1.40060026732549,3.95233945647285,-7.36806063659619));
#130262=CARTESIAN_POINT('Ctrl Pts',(1.95508475,4.042807359,-7.24069358700001));
#130263=CARTESIAN_POINT('Ctrl Pts',(1.557951187,3.977102825,-7.347924996));
#130264=CARTESIAN_POINT('Ctrl Pts',(1.151472347,3.912499672,-7.411080315));
#130265=CARTESIAN_POINT('Ctrl Pts',(2.118444839,4.042807359,-6.933591527));
#130266=CARTESIAN_POINT('Ctrl Pts',(1.73815504,3.977102825,-7.04978282));
#130267=CARTESIAN_POINT('Ctrl Pts',(1.347439022,3.912499672,-7.123686411));
#130268=CARTESIAN_POINT('',(1.95508474192627,4.04280736030989,-7.24069356686469));
#130269=CARTESIAN_POINT('Origin',(-0.0669162103268045,4.16063868480358,
0.175490039129509));
#130270=CARTESIAN_POINT('',(2.03758157319294,4.04280736269456,-7.08560705295516));
#130271=CARTESIAN_POINT('Origin',(-1.46475713502792E-13,4.134630322,4.87023615880489E-13));
#130272=CARTESIAN_POINT('',(1.40317543671779,4.13354310063947,-7.36757074555853));
#130273=CARTESIAN_POINT('Origin',(-0.0402218681886213,4.16070815660101,
0.187817616273244));
#130274=CARTESIAN_POINT('Origin',(-0.0539512478212259,4.01786461752988,
0.184401513983244));
#130275=CARTESIAN_POINT('Ctrl Pts',(3.17958655931402,3.912491975,-6.79323254224789));
#130276=CARTESIAN_POINT('Ctrl Pts',(2.81112615420095,3.97753138,-6.96569119870049));
#130277=CARTESIAN_POINT('Ctrl Pts',(2.42617413122656,4.042807359,-7.0972852663583));
#130278=CARTESIAN_POINT('Ctrl Pts',(2.41292795081507,4.04505350226662,-7.10181341183424));
#130279=CARTESIAN_POINT('Ctrl Pts',(2.39968177040358,4.0472996455332,-7.10634155731016));
#130280=CARTESIAN_POINT('Ctrl Pts',(2.855957386,3.912491975,-6.663783266));
#130281=CARTESIAN_POINT('Ctrl Pts',(2.494518222,3.97753138,-6.81868849100001));
#130282=CARTESIAN_POINT('Ctrl Pts',(2.118444839,4.042807359,-6.933591527));
#130283=CARTESIAN_POINT('Ctrl Pts',(2.10550417215875,4.04505350226662,-6.93754533488736));
#130284=CARTESIAN_POINT('Ctrl Pts',(2.09256350531744,4.0472996455332,-6.94149914277462));
#130285=CARTESIAN_POINT('',(2.42554695194231,4.04280735814475,-7.0969516709872));
#130286=CARTESIAN_POINT('',(2.27199585988443,4.04280735744339,-7.01527157445221));
#130287=CARTESIAN_POINT('',(2.95177024883494,3.95233946528638,-6.89471181604777));
#130288=CARTESIAN_POINT('Origin',(-0.0661859235379966,4.01785664201628,
0.181274795380851));
#130289=CARTESIAN_POINT('Ctrl Pts',(2.8516555602423,3.91326598479036,-6.6656252952509));
#130290=CARTESIAN_POINT('Ctrl Pts',(2.8683622922366,3.92008713489517,-6.70373515344066));
#130291=CARTESIAN_POINT('Ctrl Pts',(2.88506563246586,3.9267491516805,-6.74190113461209));
#130292=CARTESIAN_POINT('Ctrl Pts',(2.91843046311368,3.93976378714705,-6.81825197501983));
#130293=CARTESIAN_POINT('Ctrl Pts',(2.93511011255253,3.94612348134051,-6.8564784007494));
#130294=CARTESIAN_POINT('Ctrl Pts',(2.95177024985849,3.95233945647065,-6.89471181703501));
#130295=CARTESIAN_POINT('Ctrl Pts',(3.465911043,4.042807359,-6.651124765));
#130296=CARTESIAN_POINT('Ctrl Pts',(3.101113825,3.977102825,-6.84122114));
#130297=CARTESIAN_POINT('Ctrl Pts',(2.717714761,3.912499672,-6.99028085800001));
#130298=CARTESIAN_POINT('Ctrl Pts',(3.559433999,4.042807359,-6.316084991));
#130299=CARTESIAN_POINT('Ctrl Pts',(3.213012857,3.977102825,-6.51131086100001));
#130300=CARTESIAN_POINT('Ctrl Pts',(2.847318651,3.912499672,-6.667479022));
#130301=CARTESIAN_POINT('',(3.46591103084481,4.04280736030966,-6.6511247470209));
#130302=CARTESIAN_POINT('Origin',(-0.103076933933817,4.1606386869864,0.15700221155554));
#130303=CARTESIAN_POINT('',(3.51314011588116,4.04280736269456,-6.48192968991497));
#130304=CARTESIAN_POINT('Origin',(-4.38885039422132E-13,4.13463032199911,
7.97539118080337E-13));
#130305=CARTESIAN_POINT('',(2.95417990197285,4.13354310061305,-6.89367979403913));
#130306=CARTESIAN_POINT('Origin',(-0.079656774662682,4.16070809307365,0.174780159875999));
#130307=CARTESIAN_POINT('Origin',(-0.09233079221727,4.01786464488332,0.168492434329938));
#130308=CARTESIAN_POINT('Ctrl Pts',(4.56559378250116,3.912491975,-5.95089341838246));
#130309=CARTESIAN_POINT('Ctrl Pts',(4.2428212902823,3.97753138,-6.19852818282084));
#130310=CARTESIAN_POINT('Ctrl Pts',(3.89515806583989,4.042807359,-6.40979896040833));
#130311=CARTESIAN_POINT('Ctrl Pts',(3.88319499132248,4.04505350223884,-6.41706877751275));
#130312=CARTESIAN_POINT('Ctrl Pts',(3.87123191680507,4.04729964547766,-6.42433859461714));
#130313=CARTESIAN_POINT('Ctrl Pts',(4.221703111,3.912491975,-5.8940413));
#130314=CARTESIAN_POINT('Ctrl Pts',(3.902014239,3.97753138,-6.123023663));
#130315=CARTESIAN_POINT('Ctrl Pts',(3.559433999,4.042807359,-6.316084991));
#130316=CARTESIAN_POINT('Ctrl Pts',(3.54764582972819,4.04505350223885,-6.32272822183637));
#130317=CARTESIAN_POINT('Ctrl Pts',(3.53585766045637,4.04729964547766,-6.32937145267288));
#130318=CARTESIAN_POINT('',(3.89447383652341,4.04280735814476,-6.40960798932368));
#130319=CARTESIAN_POINT('',(3.72695387773219,4.04280735744339,-6.36284647384277));
#130320=CARTESIAN_POINT('',(4.36491873504013,3.95233946527757,-6.09897393563535));
#130321=CARTESIAN_POINT('Origin',(-0.103607243489299,4.01785664252565,0.162808653726628));
#130322=CARTESIAN_POINT('Ctrl Pts',(4.21789784076116,3.91326598469089,-5.89676502847127));
#130323=CARTESIAN_POINT('Ctrl Pts',(4.24240649246361,3.9200871405027,-5.93039247398505));
#130324=CARTESIAN_POINT('Ctrl Pts',(4.2669238990547,3.92674916318505,-5.9640754633098));
#130325=CARTESIAN_POINT('Ctrl Pts',(4.31592180509563,3.93976378604036,-6.03146874593862));
#130326=CARTESIAN_POINT('Ctrl Pts',(4.34042904091571,3.94612347918163,-6.06521582155868));
#130327=CARTESIAN_POINT('Ctrl Pts',(4.36491873623229,3.95233945644434,-6.09897393639698));
#130328=CARTESIAN_POINT('Ctrl Pts',(4.814675187,4.042807359,-5.750556742));
#130329=CARTESIAN_POINT('Ctrl Pts',(4.499271827,3.977102825,-6.014629387));
#130330=CARTESIAN_POINT('Ctrl Pts',(4.156879854,3.912499672,-6.242623638));
#130331=CARTESIAN_POINT('Ctrl Pts',(4.833987981,4.042807359,-5.40324534));
#130332=CARTESIAN_POINT('Ctrl Pts',(4.537633764,3.977102825,-5.668377243));
#130333=CARTESIAN_POINT('Ctrl Pts',(4.214060823,3.912499672,-5.899507723));
#130334=CARTESIAN_POINT('',(4.81467517126731,4.04280736030966,-5.75055672705016));
#130335=CARTESIAN_POINT('Origin',(-0.134418047111175,4.16063871796191,0.131173290137131));
#130336=CARTESIAN_POINT('',(4.82442813085483,4.04280736269456,-5.57516449880049));
#130337=CARTESIAN_POINT('Origin',(-8.08164299370695E-13,4.13463032200022,
9.68409380464053E-13));
#130338=CARTESIAN_POINT('',(4.36705019746166,4.13354310060638,-6.09744803724894));
#130339=CARTESIAN_POINT('Origin',(-0.115367111426155,4.16070813913995,0.15357017334568));
#130340=CARTESIAN_POINT('Origin',(-0.126392979154755,4.0178646284018,0.144704703487445));
#130341=CARTESIAN_POINT('Ctrl Pts',(5.7381189155374,3.912491975,-4.83029713213311));
#130342=CARTESIAN_POINT('Ctrl Pts',(5.4761268181007,3.97753138,-5.14152887785456));
#130343=CARTESIAN_POINT('Ctrl Pts',(5.18200873963653,4.042807359,-5.42259757788377));
#130344=CARTESIAN_POINT('Ctrl Pts',(5.171888151756,4.04505350206407,-5.43226913732674));
#130345=CARTESIAN_POINT('Ctrl Pts',(5.16176756387534,4.04729964512812,-5.44194069676973));
#130346=CARTESIAN_POINT('Ctrl Pts',(5.390046691,3.912491975,-4.848700513));
#130347=CARTESIAN_POINT('Ctrl Pts',(5.127056407,3.97753138,-5.141053053));
#130348=CARTESIAN_POINT('Ctrl Pts',(4.833987981,4.042807359,-5.40324534));
#130349=CARTESIAN_POINT('Ctrl Pts',(4.82390351160652,4.04505350206407,-5.41226736304614));
#130350=CARTESIAN_POINT('Ctrl Pts',(4.81381904221294,4.04729964512812,-5.42128938609216));
#130351=CARTESIAN_POINT('',(5.18129945413042,4.04280735814474,-5.42255816067613));
#130352=CARTESIAN_POINT('',(5.00764367496653,4.04280735744339,-5.41290174300688));
#130353=CARTESIAN_POINT('',(5.57396847208562,3.95233946527127,-5.01805481218518));
#130354=CARTESIAN_POINT('Origin',(-0.136184000983926,4.0178566698653,0.13672977369069));
#130355=CARTESIAN_POINT('Ctrl Pts',(5.38691590761031,3.91326598479672,-4.85217858324993));
#130356=CARTESIAN_POINT('Ctrl Pts',(5.4180804633958,3.92008713973162,-4.87975119871123));
#130357=CARTESIAN_POINT('Ctrl Pts',(5.44926550910729,3.92674916150384,-4.90737617685124));
#130358=CARTESIAN_POINT('Ctrl Pts',(5.51160543921952,3.9397637852627,-4.96266074458048));
#130359=CARTESIAN_POINT('Ctrl Pts',(5.54279432879826,3.94612347757219,-4.99035049725823));
#130360=CARTESIAN_POINT('Ctrl Pts',(5.57396847340179,3.95233945642564,-5.01805481268885));
#130361=CARTESIAN_POINT('Ctrl Pts',(5.938310471,4.042807359,-4.581099076));
#130362=CARTESIAN_POINT('Ctrl Pts',(5.687048879,3.977102825,-4.906800249));
#130363=CARTESIAN_POINT('Ctrl Pts',(5.401673864,3.912499672,-5.203068274));
#130364=CARTESIAN_POINT('Ctrl Pts',(5.882510057,4.042807359,-4.237755942));
#130365=CARTESIAN_POINT('Ctrl Pts',(5.65007996,3.977102825,-4.560396605));
#130366=CARTESIAN_POINT('Ctrl Pts',(5.383758195,3.912499672,-4.855682001));
#130367=CARTESIAN_POINT('',(5.93831045237977,4.0428073603099,-4.58109906488038));
#130368=CARTESIAN_POINT('Origin',(-0.159473693902303,4.16063870385668,0.0992105328740411));
#130369=CARTESIAN_POINT('',(5.9101312483988,4.04280736269456,-4.40771081147348));
#130370=CARTESIAN_POINT('Origin',(-7.66747776381749E-13,4.13463032199978,
7.53303669442928E-13));
#130371=CARTESIAN_POINT('',(5.57572207905876,4.13354310060491,-5.01610638780029));
#130372=CARTESIAN_POINT('Origin',(-0.145682930494174,4.16070809090573,0.12517927535747));
#130373=CARTESIAN_POINT('Origin',(-0.154545132451127,4.01786462453061,0.114150754036674));
#130374=CARTESIAN_POINT('Ctrl Pts',(6.64233598404738,3.912491975,-3.48384151984001));
#130375=CARTESIAN_POINT('Ctrl Pts',(6.45337474226534,3.97753138,-3.84411739653553));
#130376=CARTESIAN_POINT('Ctrl Pts',(6.22655444281494,4.042807359,-4.1818415599671));
#130377=CARTESIAN_POINT('Ctrl Pts',(6.21874956738325,4.04505350225091,-4.19346263194456));
#130378=CARTESIAN_POINT('Ctrl Pts',(6.21094469195147,4.04729964550179,-4.20508370392205));
#130379=CARTESIAN_POINT('Ctrl Pts',(6.306357679,3.912491975,-3.57663988));
#130380=CARTESIAN_POINT('Ctrl Pts',(6.112363115,3.97753138,-3.918692517));
#130381=CARTESIAN_POINT('Ctrl Pts',(5.882510057,4.042807359,-4.237755942));
#130382=CARTESIAN_POINT('Ctrl Pts',(5.87460082449465,4.04505350225091,-4.24873489887897));
#130383=CARTESIAN_POINT('Ctrl Pts',(5.8666915919893,4.04729964550179,-4.25971385575793));
#130384=CARTESIAN_POINT('',(6.22585326643108,4.04280735814475,-4.18195553973078));
#130385=CARTESIAN_POINT('',(6.05418161852976,4.04280735744339,-4.20985574286674));
#130386=CARTESIAN_POINT('',(6.52238563876683,3.95233946529696,-3.70249702295116));
#130387=CARTESIAN_POINT('Origin',(-0.162393127489747,4.01785661752674,0.104257678319604));
#130388=CARTESIAN_POINT('Ctrl Pts',(6.30404777361277,3.91326598474248,-3.58070966061121));
#130389=CARTESIAN_POINT('Ctrl Pts',(6.3404110065364,3.92008713781498,-3.6009381796591));
#130390=CARTESIAN_POINT('Ctrl Pts',(6.37680550547289,3.92674915766183,-3.62121343168818));
#130391=CARTESIAN_POINT('Ctrl Pts',(6.44957254934357,3.93976378842026,-3.66180425625756));
#130392=CARTESIAN_POINT('Ctrl Pts',(6.4859847578353,3.94612348394098,-3.68214195945266));
#130393=CARTESIAN_POINT('Ctrl Pts',(6.52238564019206,3.95233945650218,-3.70249702308815));
#130394=CARTESIAN_POINT('Ctrl Pts',(6.784276957,4.042807359,-3.19743431));
#130395=CARTESIAN_POINT('Ctrl Pts',(6.608905846,3.977102825,-3.569534585));
#130396=CARTESIAN_POINT('Ctrl Pts',(6.393891608,3.912499672,-3.920223221));
#130397=CARTESIAN_POINT('Ctrl Pts',(6.655972501,4.042807359,-2.874113787));
#130398=CARTESIAN_POINT('Ctrl Pts',(6.498334696,3.977102825,-3.23917689));
#130399=CARTESIAN_POINT('Ctrl Pts',(6.301717018,3.912499672,-3.584809985));
#130400=CARTESIAN_POINT('',(6.78427693644271,4.04280736030966,-3.19743430304974));
#130401=CARTESIAN_POINT('Origin',(-0.177072652585477,4.16063872579149,0.0626089307403355));
#130402=CARTESIAN_POINT('',(6.71948319740546,4.04280736269456,-3.0341574665131));
#130403=CARTESIAN_POINT('Origin',(-2.02528965820292E-13,4.13463032200022,
1.0321604682062E-13));
#130404=CARTESIAN_POINT('',(6.52367939390571,4.13354310057799,-3.70021717765555));
#130405=CARTESIAN_POINT('Origin',(-0.169186457818068,4.16070813326555,0.0909349252870628));
#130406=CARTESIAN_POINT('Origin',(-0.175471187222578,4.01786465903462,0.0782594480763255));
#130407=CARTESIAN_POINT('Ctrl Pts',(7.23596480548825,3.912491975,-1.97448535086908));
#130408=CARTESIAN_POINT('Ctrl Pts',(7.12887003564431,3.97753138,-2.36695925973825));
#130409=CARTESIAN_POINT('Ctrl Pts',(6.97995338116804,4.042807359,-2.74554727906954));
#130410=CARTESIAN_POINT('Ctrl Pts',(6.97482916644641,4.04505350221171,-2.75857447410635));
#130411=CARTESIAN_POINT('Ctrl Pts',(6.96970495172464,4.04729964542339,-2.77160166914315));
#130412=CARTESIAN_POINT('Ctrl Pts',(6.92779039,3.912491975,-2.137339541));
#130413=CARTESIAN_POINT('Ctrl Pts',(6.811862518,3.97753138,-2.513098274));
#130414=CARTESIAN_POINT('Ctrl Pts',(6.655972501,4.042807359,-2.874113787));
#130415=CARTESIAN_POINT('Ctrl Pts',(6.65060833321854,4.04505350221171,-2.88653631296233));
#130416=CARTESIAN_POINT('Ctrl Pts',(6.64524416543696,4.04729964542339,-2.89895883892467));
#130417=CARTESIAN_POINT('',(6.97929310018125,4.04280735814474,-2.74580932624543));
#130418=CARTESIAN_POINT('',(6.81763275884877,4.04280735744339,-2.80996156785876));
#130419=CARTESIAN_POINT('',(7.16582330193381,3.95233946527704,-2.21381458834179));
#130420=CARTESIAN_POINT('Origin',(-0.181008804869115,4.01785668701233,0.0669104859044277));
#130421=CARTESIAN_POINT('Ctrl Pts',(6.92640937123344,3.91326598469505,-2.14181073366623));
#130422=CARTESIAN_POINT('Ctrl Pts',(6.96627100041619,3.92008714027779,-2.15374930542941));
#130423=CARTESIAN_POINT('Ctrl Pts',(7.00617321276977,3.92674916271554,-2.16572679693359));
#130424=CARTESIAN_POINT('Ctrl Pts',(7.08596478508344,3.93976378594542,-2.18972585333134));
#130425=CARTESIAN_POINT('Ctrl Pts',(7.12589768481122,3.94612347897943,-2.20176051882883));
#130426=CARTESIAN_POINT('Ctrl Pts',(7.16582330334321,3.95233945644287,-2.21381458822912));
#130427=CARTESIAN_POINT('Ctrl Pts',(7.313018193,4.042807359,-1.664261068));
#130428=CARTESIAN_POINT('Ctrl Pts',(7.221737721,3.977102825,-2.065361451));
#130429=CARTESIAN_POINT('Ctrl Pts',(7.087138087,3.912499672,-2.454072887));
#130430=CARTESIAN_POINT('Ctrl Pts',(7.118209069,4.042807359,-1.376081265));
#130431=CARTESIAN_POINT('Ctrl Pts',(7.042734524,3.977102825,-1.766496865));
#130432=CARTESIAN_POINT('Ctrl Pts',(6.925014556,3.912499672,-2.146316238));
#130433=CARTESIAN_POINT('',(7.31301817143122,4.04280736030966,-1.66426106564211));
#130434=CARTESIAN_POINT('Origin',(-0.186391878506125,4.16063870704355,0.0230797878023903));
#130435=CARTESIAN_POINT('',(7.21463958071766,4.04280736269456,-1.51873028963318));
#130436=CARTESIAN_POINT('Origin',(7.93635990259389E-14,4.134630322,5.48606299277665E-14));
#130437=CARTESIAN_POINT('',(7.16659671034123,4.13354310061321,-2.21130992580493));
#130438=CARTESIAN_POINT('Origin',(-0.184779512955822,4.16070810473172,0.0524389094179195));
#130439=CARTESIAN_POINT('Origin',(-0.188191923671757,4.01786463325267,0.0387085766334819));
#130440=CARTESIAN_POINT('Ctrl Pts',(7.49124795482483,3.912491975,-0.372804441010172));
#130441=CARTESIAN_POINT('Ctrl Pts',(7.4710272900667,3.97753138,-0.779124736979639));
#130442=CARTESIAN_POINT('Ctrl Pts',(7.40697745695167,4.042807359,-1.18087425843626));
#130443=CARTESIAN_POINT('Ctrl Pts',(7.40477350540734,4.04505350216274,-1.19469843931525));
#130444=CARTESIAN_POINT('Ctrl Pts',(7.40256955386291,4.04729964532543,-1.20852262019425));
#130445=CARTESIAN_POINT('Ctrl Pts',(7.225287322,3.912491975,-0.59809958));
#130446=CARTESIAN_POINT('Ctrl Pts',(7.19284679999999,3.97753138,-0.989994349));
#130447=CARTESIAN_POINT('Ctrl Pts',(7.118209069,4.042807359,-1.376081265));
#130448=CARTESIAN_POINT('Ctrl Pts',(7.11564078842061,4.04505350216274,-1.38936649641096));
#130449=CARTESIAN_POINT('Ctrl Pts',(7.1130725078412,4.04729964532544,-1.40265172782197));
#130450=CARTESIAN_POINT('',(7.40638894538665,4.04280735814476,-1.18127211997347));
#130451=CARTESIAN_POINT('',(7.26229896883851,4.04280735744341,-1.27867671243651));
#130452=CARTESIAN_POINT('',(7.47419503215417,3.95233946528439,-0.621616643560051));
#130453=CARTESIAN_POINT('Origin',(-0.191160705533955,4.01785662612324,0.0264346106921929));
#130454=CARTESIAN_POINT('Ctrl Pts',(7.22489976603804,3.91326598485069,-0.602763116835091));
#130455=CARTESIAN_POINT('Ctrl Pts',(7.26639587926392,3.92008713822626,-0.605853498624219));
#130456=CARTESIAN_POINT('Ctrl Pts',(7.30793999166212,3.92674915839138,-0.608973165802315));
#130457=CARTESIAN_POINT('Ctrl Pts',(7.39102520304202,3.93976378691293,-0.61525831079887));
#130458=CARTESIAN_POINT('Ctrl Pts',(7.43261159764799,3.94612348087459,-0.618427219959677));
#130459=CARTESIAN_POINT('Ctrl Pts',(7.47419503350602,3.95233945646465,-0.621616643123829));
#130460=CARTESIAN_POINT('Ctrl Pts',(7.499810826,4.042807359,-0.0532688290000001));
#130461=CARTESIAN_POINT('Ctrl Pts',(7.496889167,3.977102825,-0.464614311));
#130462=CARTESIAN_POINT('Ctrl Pts',(7.448997866,3.912499672,-0.873172832));
#130463=CARTESIAN_POINT('Ctrl Pts',(7.247606092,4.042807359,0.186295287));
#130464=CARTESIAN_POINT('Ctrl Pts',(7.257823913,3.977102825,-0.211217409));
#130465=CARTESIAN_POINT('Ctrl Pts',(7.224506111,3.912499672,-0.60746313));
#130466=CARTESIAN_POINT('',(7.49981080442722,4.04280736030966,-0.0532688313318097));
#130467=CARTESIAN_POINT('Origin',(-0.18699551190703,4.16063870247584,-0.0175285563611807));
#130468=CARTESIAN_POINT('',(7.37244743553787,4.04280736269456,0.0677110269473681));
#130469=CARTESIAN_POINT('Origin',(-1.32706345912226E-13,4.13463032200111,
4.27649994409751E-14));
#130470=CARTESIAN_POINT('',(7.47441192976062,4.13354310062207,-0.619004279110432));
#130471=CARTESIAN_POINT('Origin',(-0.19173213084235,4.1607081265445,0.01149076061306));
#130472=CARTESIAN_POINT('Origin',(-0.192113445256573,4.01786460469813,-0.00265210371298302));
#130473=CARTESIAN_POINT('Ctrl Pts',(7.3962486753266,3.912491975,1.24630839070828));
#130474=CARTESIAN_POINT('Ctrl Pts',(7.46384761202233,3.97753138,0.845140791482356));
#130475=CARTESIAN_POINT('Ctrl Pts',(7.4876594991711,4.042807359,0.439015130657355));
#130476=CARTESIAN_POINT('Ctrl Pts',(7.48847886501099,4.04505350215634,0.425040367082017));
#130477=CARTESIAN_POINT('Ctrl Pts',(7.4892982308509,4.04729964531265,0.411065603506677));
#130478=CARTESIAN_POINT('Ctrl Pts',(7.18493785000001,3.912491975,0.969106852));
#130479=CARTESIAN_POINT('Ctrl Pts',(7.23750156,3.97753138,0.579400611999999));
#130480=CARTESIAN_POINT('Ctrl Pts',(7.247606092,4.042807359,0.186295287));
#130481=CARTESIAN_POINT('Ctrl Pts',(7.24795378843822,4.04505350215634,0.172768552525941));
#130482=CARTESIAN_POINT('Ctrl Pts',(7.24830148487646,4.04729964531265,0.159241818051882));
#130483=CARTESIAN_POINT('',(7.4871702751445,4.04280735814474,0.438500058308231));
#130484=CARTESIAN_POINT('',(7.36738815040593,4.04280735744339,0.312397644926896));
#130485=CARTESIAN_POINT('',(7.43308170904286,3.95233946527388,0.999647404285365));
#130486=CARTESIAN_POINT('Origin',(-0.192373731644399,4.01785666929138,-0.0152772730488699));
#130487=CARTESIAN_POINT('Ctrl Pts',(7.18556187680774,3.91326598473617,0.96446903296805));
#130488=CARTESIAN_POINT('Ctrl Pts',(7.22675217651942,3.92008713843996,0.970371340687591));
#130489=CARTESIAN_POINT('Ctrl Pts',(7.26799564899922,3.9267491589428,0.976255366041739));
#130490=CARTESIAN_POINT('Ctrl Pts',(7.35048948246961,3.93976378556259,0.987978026920435));
#130491=CARTESIAN_POINT('Ctrl Pts',(7.39178482283155,3.94612347820117,0.993823049286259));
#130492=CARTESIAN_POINT('Ctrl Pts',(7.43308171027695,3.95233945643343,0.999647404970062));
#130493=CARTESIAN_POINT('Ctrl Pts',(7.33592064100001,4.042807359,1.560214201));
#130494=CARTESIAN_POINT('Ctrl Pts',(7.421494407,3.977102825,1.157857678));
#130495=CARTESIAN_POINT('Ctrl Pts',(7.462550783,3.912499672,0.748555814));
#130496=CARTESIAN_POINT('Ctrl Pts',(7.038113109,4.042807359,1.739960879));
#130497=CARTESIAN_POINT('Ctrl Pts',(7.133545523,3.977102825,1.353938339));
#130498=CARTESIAN_POINT('Ctrl Pts',(7.18618778900001,3.912499672,0.95979428));
#130499=CARTESIAN_POINT('',(7.33592062045006,4.04280736030989,1.56021419403977));
#130500=CARTESIAN_POINT('Origin',(-0.178855668896493,4.16063873214872,-0.0573172701771181));
#130501=CARTESIAN_POINT('',(7.18552784240835,4.04280736269456,1.65098625133119));
#130502=CARTESIAN_POINT('Origin',(-8.49580822359641E-13,4.13463032200089,
-9.39732233001811E-14));
#130503=CARTESIAN_POINT('',(7.43273195498472,4.13354310059326,1.00224532016575));
#130504=CARTESIAN_POINT('Origin',(-0.189719945425788,4.16070812904751,-0.0299946459788324));
#130505=CARTESIAN_POINT('Origin',(-0.187051916916066,4.01786466354787,-0.0438888126460474));
#130506=CARTESIAN_POINT('Ctrl Pts',(6.95540902751334,3.912491975,2.80714522631661));
#130507=CARTESIAN_POINT('Ctrl Pts',(7.10766671470722,3.97753138,2.42988847618128));
#130508=CARTESIAN_POINT('Ctrl Pts',(7.21822690572252,4.042807359,2.03837665990852));
#130509=CARTESIAN_POINT('Ctrl Pts',(7.22203127675693,4.04505350240363,2.0249047565065));
#130510=CARTESIAN_POINT('Ctrl Pts',(7.22583564779146,4.04729964580723,2.01143285310446));
#130511=CARTESIAN_POINT('Ctrl Pts',(6.80862866900001,3.912491975,2.490998925));
#130512=CARTESIAN_POINT('Ctrl Pts',(6.943738791,3.97753138,2.121703444));
#130513=CARTESIAN_POINT('Ctrl Pts',(7.038113109,4.042807359,1.739960879));
#130514=CARTESIAN_POINT('Ctrl Pts',(7.04136052489626,4.04505350240363,1.72682513508024));
#130515=CARTESIAN_POINT('Ctrl Pts',(7.04460794079238,4.04729964580723,1.71368939116042));
#130516=CARTESIAN_POINT('',(7.21785984476897,4.04280735814474,2.03776846087977));
#130517=CARTESIAN_POINT('',(7.12798645045437,4.04280735744339,1.88886463573798));
#130518=CARTESIAN_POINT('',(7.04440574707233,3.95233946528394,2.5741690509787));
#130519=CARTESIAN_POINT('Origin',(-0.184592186119418,4.01785669121865,-0.0562748305058976));
#130520=CARTESIAN_POINT('Ctrl Pts',(6.81023510049717,3.91326598479217,2.48660368253256));
#130521=CARTESIAN_POINT('Ctrl Pts',(6.84919357950587,3.92008713976044,2.50122269724142));
#130522=CARTESIAN_POINT('Ctrl Pts',(6.88820791922027,3.92674916155891,2.51583528793693));
#130523=CARTESIAN_POINT('Ctrl Pts',(6.9662530591139,3.9397637868083,2.54501761238485));
#130524=CARTESIAN_POINT('Ctrl Pts',(7.00532643854862,3.94612348068096,2.55960326201085));
#130525=CARTESIAN_POINT('Ctrl Pts',(7.04440574811698,3.95233945646352,2.57416905194011));
#130526=CARTESIAN_POINT('Ctrl Pts',(6.829010959,4.042807359,3.10074335));
#130527=CARTESIAN_POINT('Ctrl Pts',(6.999078818,3.977102825,2.726189529));
#130528=CARTESIAN_POINT('Ctrl Pts',(7.12716312,3.912499672,2.335282822));
#130529=CARTESIAN_POINT('Ctrl Pts',(6.49952578000001,4.042807359,3.212267834));
#130530=CARTESIAN_POINT('Ctrl Pts',(6.675710472,3.977102825,2.855785434));
#130531=CARTESIAN_POINT('Ctrl Pts',(6.81185131300001,3.912499672,2.482172775));
#130532=CARTESIAN_POINT('',(6.82901094038103,4.04280736030966,3.10074333884465));
#130533=CARTESIAN_POINT('Origin',(-0.162352327731182,4.16063870640799,-0.0944257980160096));
#130534=CARTESIAN_POINT('',(6.66262095329685,4.04280736269456,3.15706319396646));
#130535=CARTESIAN_POINT('Origin',(-1.58727198051878E-13,4.13463032199933,
1.01915004213637E-14));
#130536=CARTESIAN_POINT('',(7.04350569485826,4.13354310058752,2.57663104168863));
#130537=CARTESIAN_POINT('Origin',(-0.178836261171845,4.16070812928274,-0.0700775177326174));
#130538=CARTESIAN_POINT('Origin',(-0.17324391522071,4.01786469226385,-0.0830733358114233));
#130539=CARTESIAN_POINT('Ctrl Pts',(6.18934218547474,3.912491975,4.23672307189534));
#130540=CARTESIAN_POINT('Ctrl Pts',(6.41913922087722,3.97753138,3.90101727661634));
#130541=CARTESIAN_POINT('Ctrl Pts',(6.61127804412574,4.042807359,3.54242596097349));
#130542=CARTESIAN_POINT('Ctrl Pts',(6.61788953126837,4.04505350211977,3.53008685202745));
#130543=CARTESIAN_POINT('Ctrl Pts',(6.62450101841088,4.04729964523953,3.51774774308143));
#130544=CARTESIAN_POINT('Ctrl Pts',(6.113955579,3.912491975,3.896414657));
#130545=CARTESIAN_POINT('Ctrl Pts',(6.325294513,3.97753138,3.564797781));
#130546=CARTESIAN_POINT('Ctrl Pts',(6.49952578,4.042807359,3.212267834));
#130547=CARTESIAN_POINT('Ctrl Pts',(6.50552106904223,4.04505350211977,3.20013729644091));
#130548=CARTESIAN_POINT('Ctrl Pts',(6.51151635808462,4.04729964523953,3.18800675888175));
#130549=CARTESIAN_POINT('',(6.61105030969852,4.04280735814475,3.54175307414439));
#130550=CARTESIAN_POINT('',(6.55528802638805,4.04280735744339,3.37701041498213));
#130551=CARTESIAN_POINT('',(6.32634120131164,3.95233946527627,4.02832541343909));
#130552=CARTESIAN_POINT('Origin',(-0.168179181945322,4.01785664306235,-0.094641074836807));
#130553=CARTESIAN_POINT('Ctrl Pts',(6.1164693003912,3.9132659848096,3.89246750855191));
#130554=CARTESIAN_POINT('Ctrl Pts',(6.15137427892296,3.92008713647702,3.91511964903297));
#130555=CARTESIAN_POINT('Ctrl Pts',(6.18633519089755,3.92674915487793,3.93777752275454));
#130556=CARTESIAN_POINT('Ctrl Pts',(6.25628237277549,3.93976378592067,3.98305499865668));
#130557=CARTESIAN_POINT('Ctrl Pts',(6.29130674935267,3.94612347887328,4.00569926190145));
#130558=CARTESIAN_POINT('Ctrl Pts',(6.32634120213922,3.9523394564405,4.02832541458508));
#130559=CARTESIAN_POINT('Ctrl Pts',(6.002784315,4.042807359,4.496285186));
#130560=CARTESIAN_POINT('Ctrl Pts',(6.249394081,3.977102825,4.167047787));
#130561=CARTESIAN_POINT('Ctrl Pts',(6.45851723100001,3.912499672,3.812814601));
#130562=CARTESIAN_POINT('Ctrl Pts',(5.657027848,4.042807359,4.534372715));
#130563=CARTESIAN_POINT('Ctrl Pts',(5.905726619,3.977102825,4.224099176));
#130564=CARTESIAN_POINT('Ctrl Pts',(6.119000241,3.912499672,3.888487631));
#130565=CARTESIAN_POINT('',(6.00278429926573,4.0428073603099,4.49628517105897));
#130566=CARTESIAN_POINT('Origin',(-0.138258169227965,4.16063871858951,-0.127119332806599));
#130567=CARTESIAN_POINT('',(5.82817731302716,4.04280736269456,4.51551937025311));
#130568=CARTESIAN_POINT('Origin',(-9.12030867494806E-13,4.13463032200044,
-4.96130914129367E-13));
#130569=CARTESIAN_POINT('',(6.32493293650023,4.13354310060994,4.0305363596011));
#130570=CARTESIAN_POINT('Origin',(-0.159590726451847,4.16070811817244,-0.106883739022645));
#130571=CARTESIAN_POINT('Origin',(-0.151335490861449,4.01786464595953,-0.118373611190034));
#130572=CARTESIAN_POINT('Ctrl Pts',(5.13386858061938,3.912491975,5.46819645487303));
#130573=CARTESIAN_POINT('Ctrl Pts',(5.43045991205592,3.97753138,5.18973884414867));
#130574=CARTESIAN_POINT('Ctrl Pts',(5.69519316883271,4.042807359,4.88083536282829));
#130575=CARTESIAN_POINT('Ctrl Pts',(5.70430262685269,4.04505350214671,4.87020600960848));
#130576=CARTESIAN_POINT('Ctrl Pts',(5.71341208487259,4.04729964529339,4.85957665638869));
#130577=CARTESIAN_POINT('Ctrl Pts',(5.133400721,3.912491975,5.11963837));
#130578=CARTESIAN_POINT('Ctrl Pts',(5.411086494,3.97753138,4.841206136));
#130579=CARTESIAN_POINT('Ctrl Pts',(5.657027848,4.042807359,4.534372715));
#130580=CARTESIAN_POINT('Ctrl Pts',(5.66549067759277,4.04505350214671,4.52381459245147));
#130581=CARTESIAN_POINT('Ctrl Pts',(5.6739535071854,4.04729964529339,4.51325646990289));
#130582=CARTESIAN_POINT('',(5.69511540948553,4.04280735814474,4.88012925152558));
#130583=CARTESIAN_POINT('',(5.67607161911655,4.04280735744339,4.70725094112458));
#130584=CARTESIAN_POINT('',(5.31246397217453,3.9523394652784,5.294121756425));
#130585=CARTESIAN_POINT('Origin',(-0.143902203581194,4.01785668194033,-0.128581964472328));
#130586=CARTESIAN_POINT('Ctrl Pts',(5.13670419329786,3.91326598482771,5.11632387889823));
#130587=CARTESIAN_POINT('Ctrl Pts',(5.16592358955759,3.92008714054823,5.14594998118222));
#130588=CARTESIAN_POINT('Ctrl Pts',(5.19519638141407,3.92674916312298,5.17559370893724));
#130589=CARTESIAN_POINT('Ctrl Pts',(5.25377488201198,3.93976378613899,5.23484916257931));
#130590=CARTESIAN_POINT('Ctrl Pts',(5.28311256198989,3.94612347931016,5.26449322226433));
#130591=CARTESIAN_POINT('Ctrl Pts',(5.31246397273214,3.95233945644694,5.29412175772542));
#130592=CARTESIAN_POINT('Ctrl Pts',(4.895874148,4.042807359,5.681585723));
#130593=CARTESIAN_POINT('Ctrl Pts',(5.207494623,3.977102825,5.413059522));
#130594=CARTESIAN_POINT('Ctrl Pts',(5.487878254,3.912499672,5.112063406));
#130595=CARTESIAN_POINT('Ctrl Pts',(4.550013582,4.042807359,5.644455368));
#130596=CARTESIAN_POINT('Ctrl Pts',(4.85959755300001,3.977102825,5.39489873600001));
#130597=CARTESIAN_POINT('Ctrl Pts',(5.14003151800001,3.912499672,5.112981126));
#130598=CARTESIAN_POINT('',(4.89587413578614,4.04280736030966,5.68158570505802));
#130599=CARTESIAN_POINT('Origin',(-0.107698786012628,4.16063874448231,-0.153868688590458));
#130600=CARTESIAN_POINT('',(4.72121457955431,4.04280736269456,5.66283487923137));
#130601=CARTESIAN_POINT('Origin',(-3.95516952522712E-13,4.13463032200044,
-2.42861286636753E-13));
#130602=CARTESIAN_POINT('',(5.31061334356406,4.13354310060541,5.29597827693931));
#130603=CARTESIAN_POINT('Origin',(-0.13288273199195,4.16070809434328,-0.138692140882561));
#130604=CARTESIAN_POINT('Origin',(-0.122350310308714,4.01786464218424,-0.148138533803406));
#130605=CARTESIAN_POINT('Ctrl Pts',(3.83834098716584,3.912491975,6.44398304893183));
#130606=CARTESIAN_POINT('Ctrl Pts',(4.18785833280819,3.97753138,6.23579399218282));
#130607=CARTESIAN_POINT('Ctrl Pts',(4.51280739112009,4.042807359,5.99102232646896));
#130608=CARTESIAN_POINT('Ctrl Pts',(4.52398887228891,4.04505350223783,5.98259974544947));
#130609=CARTESIAN_POINT('Ctrl Pts',(4.53517035345769,4.04729964547563,5.97417716442989));
#130610=CARTESIAN_POINT('Ctrl Pts',(3.912813751,3.912491975,6.10347348200001));
#130611=CARTESIAN_POINT('Ctrl Pts',(4.243862085,3.97753138,5.891245072));
#130612=CARTESIAN_POINT('Ctrl Pts',(4.550013582,4.042807359,5.644455368));
#130613=CARTESIAN_POINT('Ctrl Pts',(4.56054824000545,4.04505350223783,5.63596334638202));
#130614=CARTESIAN_POINT('Ctrl Pts',(4.57108289801093,4.04729964547563,5.62747132476391));
#130615=CARTESIAN_POINT('',(4.51288324280057,4.04280735814475,5.99031600768151));
#130616=CARTESIAN_POINT('',(4.53144841205905,4.04280735744339,5.81738564461189));
#130617=CARTESIAN_POINT('',(4.0501818321928,3.95233946528875,6.31237085081574));
#130618=CARTESIAN_POINT('Origin',(-0.112896553892237,4.01785663290102,-0.15651054669219));
#130619=CARTESIAN_POINT('Ctrl Pts',(3.91675250729274,3.91326598481149,6.10094663167513));
#130620=CARTESIAN_POINT('Ctrl Pts',(3.93892001924894,3.9200871359772,6.13616137514948));
#130621=CARTESIAN_POINT('Ctrl Pts',(3.96113588749605,3.9267491538669,6.17140480746271));
#130622=CARTESIAN_POINT('Ctrl Pts',(4.00560672030579,3.93976378742859,6.24186760464295));
#130623=CARTESIAN_POINT('Ctrl Pts',(4.02788591000546,3.94612348192951,6.27712534449124));
#130624=CARTESIAN_POINT('Ctrl Pts',(4.0501818324289,3.95233945647772,6.31237085222031));
#130625=CARTESIAN_POINT('Ctrl Pts',(3.560038347,4.042807359,6.601221627));
#130626=CARTESIAN_POINT('Ctrl Pts',(3.922098505,3.977102825,6.40596261));
#130627=CARTESIAN_POINT('Ctrl Pts',(4.26063218900001,3.912499672,6.172277809));
#130628=CARTESIAN_POINT('Ctrl Pts',(3.230245738,4.042807359,6.490609561));
#130629=CARTESIAN_POINT('Ctrl Pts',(3.586239107,3.977102825,6.313438827));
#130630=CARTESIAN_POINT('Ctrl Pts',(3.920720634,3.912499672,6.098397307));
#130631=CARTESIAN_POINT('',(3.56003833892888,4.04280736030966,6.60122160685206));
#130632=CARTESIAN_POINT('Origin',(-0.0721035891149052,4.16063868785459,
-0.173423303239003));
#130633=CARTESIAN_POINT('',(3.39349309954857,4.04280736269456,6.54536252325234));
#130634=CARTESIAN_POINT('Origin',(-5.67037736209919E-13,4.13463032199956,
-8.59989163215502E-13));
#130635=CARTESIAN_POINT('',(4.04797537267607,4.13354310057253,6.31378613641161));
#130636=CARTESIAN_POINT('Origin',(-0.0999613416876721,4.16070812441472,
-0.164015522838298));
#130637=CARTESIAN_POINT('Origin',(-0.0876443290261331,4.01786465820202,
-0.170976672463546));
#130638=CARTESIAN_POINT('Ctrl Pts',(2.3633368354835,3.912491975,7.11845615806791));
#130639=CARTESIAN_POINT('Ctrl Pts',(2.74943715310942,3.97753138,6.99027034331523));
#130640=CARTESIAN_POINT('Ctrl Pts',(3.11940775541563,4.042807359,6.82107574487869));
#130641=CARTESIAN_POINT('Ctrl Pts',(3.13213842513397,4.04505350213681,6.81525376730157));
#130642=CARTESIAN_POINT('Ctrl Pts',(3.14486909485237,4.0472996452736,6.80943178972441));
#130643=CARTESIAN_POINT('Ctrl Pts',(2.509267959,3.912491975,6.801916959));
#130644=CARTESIAN_POINT('Ctrl Pts',(2.878199401,3.97753138,6.665815937));
#130645=CARTESIAN_POINT('Ctrl Pts',(3.230245738,4.042807359,6.490609561));
#130646=CARTESIAN_POINT('Ctrl Pts',(3.24235963465547,4.04505350213681,6.4845807184609));
#130647=CARTESIAN_POINT('Ctrl Pts',(3.25447353131099,4.0472996452736,6.47855187592175));
#130648=CARTESIAN_POINT('',(3.11963367137329,4.04280735814475,6.82040224533391));
#130649=CARTESIAN_POINT('',(3.1749397136481,4.04280735744339,6.65550586087452));
#130650=CARTESIAN_POINT('',(2.59851769115575,3.95233946526203,7.03546049927267));
#130651=CARTESIAN_POINT('Origin',(-0.0766118672617057,4.01785667276765,
-0.177120613451401));
#130652=CARTESIAN_POINT('Ctrl Pts',(2.51365782782729,3.91326598475245,6.80029589983965));
#130653=CARTESIAN_POINT('Ctrl Pts',(2.52773696267312,3.92008714372177,6.8394527469043));
#130654=CARTESIAN_POINT('Ctrl Pts',(2.54185715832841,3.92674916966057,6.87864801310127));
#130655=CARTESIAN_POINT('Ctrl Pts',(2.5701408276257,3.93976378413994,6.95702322897541));
#130656=CARTESIAN_POINT('Ctrl Pts',(2.58431976246207,3.94612347533749,6.99624600796395));
#130657=CARTESIAN_POINT('Ctrl Pts',(2.59851769116312,3.95233945639798,7.03546050067506));
#130658=CARTESIAN_POINT('Ctrl Pts',(2.057739109,4.042807359,7.212191744));
#130659=CARTESIAN_POINT('Ctrl Pts',(2.453309419,3.977102825,7.099330006));
#130660=CARTESIAN_POINT('Ctrl Pts',(2.834163698,3.912499672,6.94388336100001));
#130661=CARTESIAN_POINT('Ctrl Pts',(1.759435193,4.042807359,7.033270065));
#130662=CARTESIAN_POINT('Ctrl Pts',(2.145192105,3.977102825,6.93676953500001));
#130663=CARTESIAN_POINT('Ctrl Pts',(2.518081211,3.912499672,6.798659207));
#130664=CARTESIAN_POINT('',(2.05773910548016,4.04280736030967,7.21219172259054));
#130665=CARTESIAN_POINT('Origin',(-0.0331369552820981,4.16063867128506,
-0.184868880908445));
#130666=CARTESIAN_POINT('',(1.90709565328332,4.04280736269456,7.12183629025041));
#130667=CARTESIAN_POINT('Origin',(9.0205620750794E-14,4.13463032200022,
4.76181594155634E-13));
#130668=CARTESIAN_POINT('',(2.59605857272175,4.1335431006069,7.03636837301566));
#130669=CARTESIAN_POINT('Origin',(-0.0623657656160265,4.16070813488204,
-0.181669549789484));
#130670=CARTESIAN_POINT('Origin',(-0.048840390273833,4.01786463811681,-0.185820511644359));
#130671=CARTESIAN_POINT('Ctrl Pts',(0.777825678986312,3.912491975,7.46007816895252));
#130672=CARTESIAN_POINT('Ctrl Pts',(1.18245534728826,3.97753138,7.41788942182325));
#130673=CARTESIAN_POINT('Ctrl Pts',(1.5801480792901,4.042807359,7.33218324370478));
#130674=CARTESIAN_POINT('Ctrl Pts',(1.59383266704732,4.04505350229402,7.32923409824292));
#130675=CARTESIAN_POINT('Ctrl Pts',(1.60751725480453,4.04729964558801,7.32628495278109));
#130676=CARTESIAN_POINT('Ctrl Pts',(0.988391585,3.912491975,7.182310358));
#130677=CARTESIAN_POINT('Ctrl Pts',(1.377955312,3.97753138,7.128700657));
#130678=CARTESIAN_POINT('Ctrl Pts',(1.759435193,4.042807359,7.033270065));
#130679=CARTESIAN_POINT('Ctrl Pts',(1.77256189733497,4.04505350229402,7.02998630292476));
#130680=CARTESIAN_POINT('Ctrl Pts',(1.78568860166998,4.04729964558801,7.02670254084949));
#130681=CARTESIAN_POINT('',(1.58051349599226,4.04280735814474,7.33157405540269));
#130682=CARTESIAN_POINT('',(1.66997436233271,4.04280735744341,7.18242202083006));
#130683=CARTESIAN_POINT('',(1.02534975047086,3.95233946528273,7.42957983493419));
#130684=CARTESIAN_POINT('Origin',(-0.036745124488227,4.01785670278804,-0.189449450308088));
#130685=CARTESIAN_POINT('Ctrl Pts',(0.993027301226501,3.91326598480419,
7.18167089032804));
#130686=CARTESIAN_POINT('Ctrl Pts',(0.998359708367689,3.92008714285065,
7.22293886440218));
#130687=CARTESIAN_POINT('Ctrl Pts',(1.003723957203,3.92674916782895,7.26425318546155));
#130688=CARTESIAN_POINT('Ctrl Pts',(1.01449801886883,3.93976378664668,7.34687621292028));
#130689=CARTESIAN_POINT('Ctrl Pts',(1.01991372227921,3.94612348037166,7.38823005464852));
#130690=CARTESIAN_POINT('Ctrl Pts',(1.02534975011445,3.95233945645996,7.42957983630734));
#130691=CARTESIAN_POINT('Ctrl Pts',(0.459222278,4.042807359,7.485927791));
#130692=CARTESIAN_POINT('Ctrl Pts',(0.869806311,3.977102825,7.460740622));
#130693=CARTESIAN_POINT('Ctrl Pts',(1.275172863,3.912499672,7.390800645));
#130694=CARTESIAN_POINT('Ctrl Pts',(0.206355414,4.042807359,7.247062677));
#130695=CARTESIAN_POINT('Ctrl Pts',(0.603838305,3.977102825,7.235744609));
#130696=CARTESIAN_POINT('Ctrl Pts',(0.997699109,3.912499672,7.181023359));
#130697=CARTESIAN_POINT('',(0.459222279251959,4.04280736030989,7.48592776935031));
#130698=CARTESIAN_POINT('Origin',(0.00737913518409336,4.16063869814088,
-0.187670095542209));
#130699=CARTESIAN_POINT('',(0.33152453429074,4.04280736269456,7.36530090741226));
#130700=CARTESIAN_POINT('Origin',(-9.78492460668168E-14,4.13463032200089,
-6.80011602582908E-13));
#130701=CARTESIAN_POINT('',(1.02275296005204,4.13354310061224,7.42993784484346));
#130702=CARTESIAN_POINT('Origin',(-0.0218540842582848,4.16070810453062,
-0.190828900716857));
#130703=CARTESIAN_POINT('Origin',(-0.00775259710145776,4.01786466043825,
-0.19197520892641));
#130704=CARTESIAN_POINT('Origin',(6.06492530893024E-14,4.13463032200089,
6.67868538251071E-14));
#130705=CARTESIAN_POINT('',(-0.0325097326105853,4.04280735814475,7.49992961001098));
#130706=CARTESIAN_POINT('Origin',(0.00483994282610858,4.01785698933134,
-0.192919282839389));
#130707=CARTESIAN_POINT('',(-0.59837544577304,4.13354310060964,7.47609168112341));
#130708=CARTESIAN_POINT('Origin',(0.0196794318998593,4.16070814981991,-0.191065540488097));
#130709=CARTESIAN_POINT('Origin',(0.0336976693805624,4.01786467675851,-0.189153730885039));
#130710=CARTESIAN_POINT('Ctrl Pts',(-0.844055740452712,3.912491975,7.45287521505932));
#130711=CARTESIAN_POINT('Ctrl Pts',(-0.439816755395279,3.97753138,7.49865623502238));
#130712=CARTESIAN_POINT('Ctrl Pts',(-0.0329975629266134,4.042807359,7.50044600138323));
#130713=CARTESIAN_POINT('Ctrl Pts',(-0.0189989277660423,4.04505350331101,
7.5005075871854));
#130714=CARTESIAN_POINT('Ctrl Pts',(-0.00500029260547111,4.04729964762199,
7.50056917298754));
#130715=CARTESIAN_POINT('Ctrl Pts',(-0.57870088,3.912491975,7.226866907));
#130716=CARTESIAN_POINT('Ctrl Pts',(-0.186720435,3.97753138,7.258255257));
#130717=CARTESIAN_POINT('Ctrl Pts',(0.206355414,4.042807359,7.247062677));
#130718=CARTESIAN_POINT('Ctrl Pts',(0.219881141159508,4.04505350331101,
7.24667754068681));
#130719=CARTESIAN_POINT('Ctrl Pts',(0.233406868319017,4.04729964762199,
7.24629240437362));
#130720=CARTESIAN_POINT('',(0.0869228665809933,4.04280735744341,7.37349610888705));
#130721=CARTESIAN_POINT('Ctrl Pts',(-0.029933757,1.714555786,7.499940264));
#130722=CARTESIAN_POINT('Ctrl Pts',(0.376054321,1.779135389,7.501560644));
#130723=CARTESIAN_POINT('Ctrl Pts',(0.77984494,1.844275173,7.459345941));
#130724=CARTESIAN_POINT('Ctrl Pts',(0.208844493,1.714555786,7.246991374));
#130725=CARTESIAN_POINT('Ctrl Pts',(0.601139897,1.779135389,7.235686168));
#130726=CARTESIAN_POINT('Ctrl Pts',(0.989922564,1.844275173,7.182099506));
#130727=CARTESIAN_POINT('',(0.213507114722386,1.71532338722497,7.24685550662799));
#130728=CARTESIAN_POINT('Origin',(-0.032091044012674,1.87498565506657,-0.195217911735541));
#130729=CARTESIAN_POINT('Ctrl Pts',(0.213507105706348,1.71532338483848,
7.24685550518316));
#130730=CARTESIAN_POINT('Ctrl Pts',(0.214203604296676,1.72001058631643,
7.27547631941166));
#130731=CARTESIAN_POINT('Ctrl Pts',(0.21487319422308,1.72461579686785,7.30411137271521));
#130732=CARTESIAN_POINT('Ctrl Pts',(0.215517557274855,1.72914335948484,
7.33275913756504));
#130733=CARTESIAN_POINT('Ctrl Pts',(0.216132017743193,1.73346081412226,
7.36007746216163));
#130734=CARTESIAN_POINT('Ctrl Pts',(0.216723540251772,1.73770768900512,
7.38740755584595));
#130735=CARTESIAN_POINT('Ctrl Pts',(0.217293427047396,1.74188747690247,
7.41474825875923));
#130736=CARTESIAN_POINT('Ctrl Pts',(0.217863328787458,1.74606737440856,
7.44208967864198));
#130737=CARTESIAN_POINT('Ctrl Pts',(0.218401490924672,1.75017861767189,
7.46944231625121));
#130738=CARTESIAN_POINT('Ctrl Pts',(0.218950417172741,1.75423096090297,
7.49680336627066));
#130739=CARTESIAN_POINT('Ctrl Pts',(1.267168999,1.844275173,7.39217713));
#130740=CARTESIAN_POINT('Ctrl Pts',(1.561876092,1.796786772,7.34165836100001));
#130741=CARTESIAN_POINT('Ctrl Pts',(1.851626136,1.75,7.267838788));
#130742=CARTESIAN_POINT('Ctrl Pts',(1.961045444,1.73233175,7.23996204900001));
#130743=CARTESIAN_POINT('Ctrl Pts',(2.069575967,1.714550109,7.208804014));
#130744=CARTESIAN_POINT('Ctrl Pts',(0.989922564,1.844275173,7.182099506));
#130745=CARTESIAN_POINT('Ctrl Pts',(1.276254403,1.796786772,7.142633839));
#130746=CARTESIAN_POINT('Ctrl Pts',(1.558535692,1.75,7.080499029));
#130747=CARTESIAN_POINT('Ctrl Pts',(1.665134548,1.73233175,7.057034846));
#130748=CARTESIAN_POINT('Ctrl Pts',(1.770978732,1.714550109,7.030372275));
#130749=CARTESIAN_POINT('',(1.76637515398525,1.71532338698357,7.03153033320607));
#130750=CARTESIAN_POINT('Ctrl Pts',(1.76637514766015,1.71532338940836,7.03153033360228));
#130751=CARTESIAN_POINT('Ctrl Pts',(1.6972361653671,1.72693520766404,7.04889858427259));
#130752=CARTESIAN_POINT('Ctrl Pts',(1.62794074337612,1.73849644464516,7.06522182174804));
#130753=CARTESIAN_POINT('Ctrl Pts',(1.55853569172686,1.75000000004527,7.08049902906013));
#130754=CARTESIAN_POINT('Ctrl Pts',(1.41430587426279,1.7739054021007,7.11224641273725));
#130755=CARTESIAN_POINT('Ctrl Pts',(1.26860743160117,1.79806016316673,7.1396923432409));
#130756=CARTESIAN_POINT('Ctrl Pts',(1.12183172733537,1.82239950660864,7.16268061375448));
#130757=CARTESIAN_POINT('Ctrl Pts',(1.07795450523445,1.82967552537028,7.16955274191823));
#130758=CARTESIAN_POINT('Ctrl Pts',(1.03398117244366,1.83696801257088,7.17602682336411));
#130759=CARTESIAN_POINT('Ctrl Pts',(0.989922562874548,1.84427517378427,
7.18209950596451));
#130760=CARTESIAN_POINT('Ctrl Pts',(1.82542260143802,1.75423096139436,7.27446440098633));
#130761=CARTESIAN_POINT('Ctrl Pts',(1.81869255493087,1.74998153251652,7.24656718951041));
#130762=CARTESIAN_POINT('Ctrl Pts',(1.81197503635218,1.74566717065959,7.21867673251375));
#130763=CARTESIAN_POINT('Ctrl Pts',(1.80522601115323,1.74127713117588,7.19080589214249));
#130764=CARTESIAN_POINT('Ctrl Pts',(1.79879017446392,1.73709081147133,7.16422839809913));
#130765=CARTESIAN_POINT('Ctrl Pts',(1.79233543785889,1.73283723876425,7.13766596825941));
#130766=CARTESIAN_POINT('Ctrl Pts',(1.78586077386494,1.72851290760487,7.11112002136436));
#130767=CARTESIAN_POINT('Ctrl Pts',(1.77938592092048,1.72418845024827,7.08457329977732));
#130768=CARTESIAN_POINT('Ctrl Pts',(1.77289109239293,1.71979319993659,7.05804286345013));
#130769=CARTESIAN_POINT('Ctrl Pts',(1.76637514608156,1.71532338474562,7.03153033395513));
#130770=CARTESIAN_POINT('Ctrl Pts',(1.583031538,1.714555786,7.331030702));
#130771=CARTESIAN_POINT('Ctrl Pts',(1.979876174,1.779135389,7.245337762));
#130772=CARTESIAN_POINT('Ctrl Pts',(2.365151479,1.844275173,7.117306968));
#130773=CARTESIAN_POINT('Ctrl Pts',(1.761850751,1.714555786,7.03266535000001));
#130774=CARTESIAN_POINT('Ctrl Pts',(2.142544221,1.779135389,6.937292538));
#130775=CARTESIAN_POINT('Ctrl Pts',(2.510717817,1.844275173,6.801381922));
#130776=CARTESIAN_POINT('Origin',(-0.0733067813757693,1.87498561224495,
-0.18375499371407));
#130777=CARTESIAN_POINT('Ctrl Pts',(2.826642864,1.844275173,6.94694826000001));
#130778=CARTESIAN_POINT('Ctrl Pts',(3.103599827,1.796786772,6.834257277));
#130779=CARTESIAN_POINT('Ctrl Pts',(3.370706649,1.75,6.699875871));
#130780=CARTESIAN_POINT('Ctrl Pts',(3.47157512,1.73233175,6.649128957));
#130781=CARTESIAN_POINT('Ctrl Pts',(3.570870203,1.714550109,6.59536852600001));
#130782=CARTESIAN_POINT('Ctrl Pts',(2.510717817,1.844275173,6.801381922));
#130783=CARTESIAN_POINT('Ctrl Pts',(2.781871425,1.796786772,6.70128605900001));
#130784=CARTESIAN_POINT('Ctrl Pts',(3.044195986,1.75,6.579921793));
#130785=CARTESIAN_POINT('Ctrl Pts',(3.143258515,1.73233175,6.534090586));
#130786=CARTESIAN_POINT('Ctrl Pts',(3.240896457,1.714550109,6.485298001));
#130787=CARTESIAN_POINT('',(3.23664945585214,1.71532338697944,6.48741861781993));
#130788=CARTESIAN_POINT('Ctrl Pts',(3.23664944972825,1.71532338941592,6.48741861962143));
#130789=CARTESIAN_POINT('Ctrl Pts',(3.1728605588578,1.72693520766624,6.51924364726614));
#130790=CARTESIAN_POINT('Ctrl Pts',(3.10869423851655,1.73849644464483,6.55008172375029));
#130791=CARTESIAN_POINT('Ctrl Pts',(3.04419598629713,1.74999999994701,6.57992179286254));
#130792=CARTESIAN_POINT('Ctrl Pts',(2.91016337108299,1.77390532353909,6.64193188382054));
#130793=CARTESIAN_POINT('Ctrl Pts',(2.77377179436078,1.79806000486797,6.70005682492887));
#130794=CARTESIAN_POINT('Ctrl Pts',(2.63536988905111,1.82239926748975,6.75405993082061));
#130795=CARTESIAN_POINT('Ctrl Pts',(2.59399534719788,1.82967536558803,6.77020388317389));
#130796=CARTESIAN_POINT('Ctrl Pts',(2.55244136939087,1.83696793249714,6.78597974788644));
#130797=CARTESIAN_POINT('Ctrl Pts',(2.51071781603781,1.84427517371954,6.80138192202261));
#130798=CARTESIAN_POINT('Ctrl Pts',(3.34654004953954,1.75423096141095,6.71197956579558));
#130799=CARTESIAN_POINT('Ctrl Pts',(3.33397027170787,1.74998153247943,6.68618133683395));
#130800=CARTESIAN_POINT('Ctrl Pts',(3.32141418136706,1.7456671706433,6.66038701106129));
#130801=CARTESIAN_POINT('Ctrl Pts',(3.30883153794968,1.74127713116734,6.63461861631227));
#130802=CARTESIAN_POINT('Ctrl Pts',(3.29683279212067,1.73709081148045,6.61004600396372));
#130803=CARTESIAN_POINT('Ctrl Pts',(3.28481882657189,1.73283723878304,6.58549216656776));
#130804=CARTESIAN_POINT('Ctrl Pts',(3.27278894282203,1.72851290761768,6.56095871051622));
#130805=CARTESIAN_POINT('Ctrl Pts',(3.2607587080534,1.72418845027309,6.53642453860544));
#130806=CARTESIAN_POINT('Ctrl Pts',(3.24871246551558,1.7197931999573,6.51191056533552));
#130807=CARTESIAN_POINT('Ctrl Pts',(3.23664944844862,1.71532338476526,6.48741861973777));
#130808=CARTESIAN_POINT('Ctrl Pts',(3.121976037,1.714555786,6.81933029100001));
#130809=CARTESIAN_POINT('Ctrl Pts',(3.491121217,1.779135389,6.650330939));
#130810=CARTESIAN_POINT('Ctrl Pts',(3.839866164,1.844275173,6.442470632));
#130811=CARTESIAN_POINT('Ctrl Pts',(3.232474826,1.714555786,6.489499711));
#130812=CARTESIAN_POINT('Ctrl Pts',(3.583765559,1.779135389,6.314518819));
#130813=CARTESIAN_POINT('Ctrl Pts',(3.914114695,1.844275173,6.102639278));
#130814=CARTESIAN_POINT('Origin',(-0.111095048004704,1.87498564516303,-0.163700524380229));
#130815=CARTESIAN_POINT('Ctrl Pts',(4.25394605,1.844275173,6.176887809));
#130816=CARTESIAN_POINT('Ctrl Pts',(4.500202683,1.796786772,6.007293919));
#130817=CARTESIAN_POINT('Ctrl Pts',(4.732176666,1.75,5.818634204));
#130818=CARTESIAN_POINT('Ctrl Pts',(4.819777801,1.73233175,5.747389985));
#130819=CARTESIAN_POINT('Ctrl Pts',(4.905194518,1.714550109,5.673540935));
#130820=CARTESIAN_POINT('Ctrl Pts',(3.914114695,1.844275173,6.102639278));
#130821=CARTESIAN_POINT('Ctrl Pts',(4.157411231,1.796786772,5.94659359));
#130822=CARTESIAN_POINT('Ctrl Pts',(4.38751306,1.75,5.771674726));
#130823=CARTESIAN_POINT('Ctrl Pts',(4.474407207,1.73233175,5.705619513));
#130824=CARTESIAN_POINT('Ctrl Pts',(4.559273465,1.714550109,5.636978399));
#130825=CARTESIAN_POINT('',(4.5555816269561,1.7153233868784,5.63996241661938));
#130826=CARTESIAN_POINT('Ctrl Pts',(4.55558162624592,1.71532338859363,5.63996241529551));
#130827=CARTESIAN_POINT('Ctrl Pts',(4.50012551473204,1.7269352089599,5.68475612547429));
#130828=CARTESIAN_POINT('Ctrl Pts',(4.44408864066811,1.73849644619173,5.72866708822583));
#130829=CARTESIAN_POINT('Ctrl Pts',(4.38751306021334,1.7500000000932,5.77167472643996));
#130830=CARTESIAN_POINT('Ctrl Pts',(4.26994398658319,1.77390540532321,5.86104841372417));
#130831=CARTESIAN_POINT('Ctrl Pts',(4.14923589214618,1.79806016925447,5.94713486426133));
#130832=CARTESIAN_POINT('Ctrl Pts',(4.02567838072189,1.82239951533986,6.02962798030087));
#130833=CARTESIAN_POINT('Ctrl Pts',(3.98874204125291,1.82967553068769,6.0542885104683));
#130834=CARTESIAN_POINT('Ctrl Pts',(3.95155133907772,1.83696801443579,6.07862813922019));
#130835=CARTESIAN_POINT('Ctrl Pts',(3.91411469928401,1.84427517216382,6.10263927525232));
#130836=CARTESIAN_POINT('Ctrl Pts',(4.71117700477546,1.75423096141368,5.83565002581548));
#130837=CARTESIAN_POINT('Ctrl Pts',(4.69335524483893,1.74998153250359,5.81315707568662));
#130838=CARTESIAN_POINT('Ctrl Pts',(4.67554769134855,1.7456671706691,5.79066499517674));
#130839=CARTESIAN_POINT('Ctrl Pts',(4.65771977994613,1.74127713119138,5.76820394759273));
#130840=CARTESIAN_POINT('Ctrl Pts',(4.64071917279701,1.73709081150169,5.74678520495294));
#130841=CARTESIAN_POINT('Ctrl Pts',(4.62370773780115,1.73283723880173,5.7253880701201));
#130842=CARTESIAN_POINT('Ctrl Pts',(4.60668513821075,1.72851290765366,5.70401426208977));
#130843=CARTESIAN_POINT('Ctrl Pts',(4.58966204185025,1.72418845030874,5.68263983030815));
#130844=CARTESIAN_POINT('Ctrl Pts',(4.57262765414895,1.71979320001295,5.66128856615154));
#130845=CARTESIAN_POINT('Ctrl Pts',(4.55558161933687,1.71532338483719,5.63996242078891));
#130846=CARTESIAN_POINT('Ctrl Pts',(4.514940407,1.714555786,5.988765576));
#130847=CARTESIAN_POINT('Ctrl Pts',(4.83912531200001,1.779135389,5.744362032));
#130848=CARTESIAN_POINT('Ctrl Pts',(5.135032975,1.844275173,5.466391529));
#130849=CARTESIAN_POINT('Ctrl Pts',(4.55195197,1.714555786,5.64289227800001));
#130850=CARTESIAN_POINT('Ctrl Pts',(4.85741400200001,1.779135389,5.396485218));
#130851=CARTESIAN_POINT('Ctrl Pts',(5.134491921,1.844275173,5.118544003));
#130852=CARTESIAN_POINT('Origin',(-0.143688351757486,1.87498561536551,-0.135991010582247));
#130853=CARTESIAN_POINT('Ctrl Pts',(5.482339447,1.844275173,5.11800295));
#130854=CARTESIAN_POINT('Ctrl Pts',(5.686381063,1.796786772,4.899436174));
#130855=CARTESIAN_POINT('Ctrl Pts',(5.872375362,1.75,4.665319669));
#130856=CARTESIAN_POINT('Ctrl Pts',(5.94261303,1.73233175,4.57690944600001));
#130857=CARTESIAN_POINT('Ctrl Pts',(6.010157388,1.714550109,4.486424876));
#130858=CARTESIAN_POINT('Ctrl Pts',(5.134491921,1.844275173,5.118544003));
#130859=CARTESIAN_POINT('Ctrl Pts',(5.338555108,1.796786772,4.913845014));
#130860=CARTESIAN_POINT('Ctrl Pts',(5.5256749,1.75,4.693550565));
#130861=CARTESIAN_POINT('Ctrl Pts',(5.596337592,1.73233175,4.610360012));
#130862=CARTESIAN_POINT('Ctrl Pts',(5.664463913,1.714550109,4.525079953));
#130863=CARTESIAN_POINT('',(5.66149986270782,1.71532338696423,4.52878784223245));
#130864=CARTESIAN_POINT('Ctrl Pts',(5.66149985801441,1.71532338934311,4.52878784623302));
#130865=CARTESIAN_POINT('Ctrl Pts',(5.61696961119619,1.7269352076431,4.58445571965647));
#130866=CARTESIAN_POINT('Ctrl Pts',(5.57168240855937,1.738496444645,4.63938633858587));
#130867=CARTESIAN_POINT('Ctrl Pts',(5.52567490000935,1.74999999999766,4.69355056498899));
#130868=CARTESIAN_POINT('Ctrl Pts',(5.4300673898056,1.77390536467005,4.80610842695748));
#130869=CARTESIAN_POINT('Ctrl Pts',(5.33068759992327,1.79806008776014,4.91613071518046));
#130870=CARTESIAN_POINT('Ctrl Pts',(5.22775255965428,1.82239939272323,5.02325623196279));
#130871=CARTESIAN_POINT('Ctrl Pts',(5.19698088489966,1.82967544929367,5.05528061891337));
#130872=CARTESIAN_POINT('Ctrl Pts',(5.16589180616078,1.83696797448142,5.08704628471413));
#130873=CARTESIAN_POINT('Ctrl Pts',(5.13449191974758,1.84427517382627,5.11854400418614));
#130874=CARTESIAN_POINT('Ctrl Pts',(5.85552455969772,1.75423096143509,4.68645197657854));
#130875=CARTESIAN_POINT('Ctrl Pts',(5.83328414297991,1.74998153247748,4.66831605084902));
#130876=CARTESIAN_POINT('Ctrl Pts',(5.81105778769197,1.74566717063503,4.65017792033718));
#130877=CARTESIAN_POINT('Ctrl Pts',(5.78881822167231,1.74127713116126,4.63207447348658));
#130878=CARTESIAN_POINT('Ctrl Pts',(5.76761068276119,1.73709081147863,4.61481111712567));
#130879=CARTESIAN_POINT('Ctrl Pts',(5.74639721422484,1.73283723879033,4.59757119101665));
#130880=CARTESIAN_POINT('Ctrl Pts',(5.7251778567166,1.72851290765275,4.58035644644634));
#130881=CARTESIAN_POINT('Ctrl Pts',(5.7039578798872,1.7241884503026,4.56314119943596));
#130882=CARTESIAN_POINT('Ctrl Pts',(5.68273185608999,1.71979320000101,4.5459510057534));
#130883=CARTESIAN_POINT('Ctrl Pts',(5.66149985709962,1.71532338474366,4.52878784834283));
#130884=CARTESIAN_POINT('Ctrl Pts',(5.696791181,1.714555786,4.878172838));
#130885=CARTESIAN_POINT('Ctrl Pts',(5.96085728700001,1.779135389,4.569793141));
#130886=CARTESIAN_POINT('Ctrl Pts',(6.19009135100001,1.844275173,4.234710034));
#130887=CARTESIAN_POINT('Ctrl Pts',(5.6585849,1.714555786,4.532429474));
#130888=CARTESIAN_POINT('Ctrl Pts',(5.903935165,1.779135389,4.226117966));
#130889=CARTESIAN_POINT('Ctrl Pts',(6.114786011,1.844275173,3.895111301));
#130890=CARTESIAN_POINT('Origin',(-0.169562945721984,1.8749856686932,-0.101922792765602));
#130891=CARTESIAN_POINT('Ctrl Pts',(6.454384744,1.844275173,3.819805961));
#130892=CARTESIAN_POINT('Ctrl Pts',(6.606670585,1.796786772,3.562486238));
#130893=CARTESIAN_POINT('Ctrl Pts',(6.737988312,1.75,3.293859971));
#130894=CARTESIAN_POINT('Ctrl Pts',(6.787578278,1.73233175,3.192417707));
#130895=CARTESIAN_POINT('Ctrl Pts',(6.834091979,1.714550109,3.089528577));
#130896=CARTESIAN_POINT('Ctrl Pts',(6.114786011,1.844275173,3.895111301));
#130897=CARTESIAN_POINT('Ctrl Pts',(6.270074082,1.796786772,3.651330506));
#130898=CARTESIAN_POINT('Ctrl Pts',(6.405462322,1.75,3.395961195));
#130899=CARTESIAN_POINT('Ctrl Pts',(6.45658945000001,1.73233175,3.299525202));
#130900=CARTESIAN_POINT('Ctrl Pts',(6.504790324,1.714550109,3.201593798));
#130901=CARTESIAN_POINT('',(6.502692658161,1.715323386995,3.20585218134069));
#130902=CARTESIAN_POINT('Ctrl Pts',(6.5026926542726,1.71532338947817,3.20585218664574));
#130903=CARTESIAN_POINT('Ctrl Pts',(6.47117044720264,1.72693520768658,3.26979126275422));
#130904=CARTESIAN_POINT('Ctrl Pts',(6.43875049337347,1.73849644464479,3.33317304402333));
#130905=CARTESIAN_POINT('Ctrl Pts',(6.40546232232299,1.7499999999346,3.39596119507856));
#130906=CARTESIAN_POINT('Ctrl Pts',(6.33628667717964,1.77390536429521,3.52644030471717));
#130907=CARTESIAN_POINT('Ctrl Pts',(6.26288187152611,1.79806008728388,3.65525404916549));
#130908=CARTESIAN_POINT('Ctrl Pts',(6.1853822153065,1.82239939206309,3.78200302082832));
#130909=CARTESIAN_POINT('Ctrl Pts',(6.1622142610839,1.82967544884116,3.81989369694854));
#130910=CARTESIAN_POINT('Ctrl Pts',(6.13868070620393,1.8369679742302,3.85759993313946));
#130911=CARTESIAN_POINT('Ctrl Pts',(6.11478600965671,1.84427517376166,3.89511130190476));
#130912=CARTESIAN_POINT('Ctrl Pts',(6.72607429382354,1.7542309613994,3.31812064141593));
#130913=CARTESIAN_POINT('Ctrl Pts',(6.70045515785928,1.74998153248024,3.30518975552672));
#130914=CARTESIAN_POINT('Ctrl Pts',(6.67484928050486,1.74566717064617,3.29225369376661));
#130915=CARTESIAN_POINT('Ctrl Pts',(6.64923795717485,1.74127713116247,3.27935434482503));
#130916=CARTESIAN_POINT('Ctrl Pts',(6.62481512732558,1.73709081146471,3.26705359018196));
#130917=CARTESIAN_POINT('Ctrl Pts',(6.60039154325329,1.73283723875166,3.25477699277116));
#130918=CARTESIAN_POINT('Ctrl Pts',(6.57596762111564,1.7285129075842,3.24252625409133));
#130919=CARTESIAN_POINT('Ctrl Pts',(6.55154298624939,1.72418845022592,3.2302751579156));
#130920=CARTESIAN_POINT('Ctrl Pts',(6.52711783144759,1.71979319991006,3.21804982922536));
#130921=CARTESIAN_POINT('Ctrl Pts',(6.50269265332106,1.71532338480411,3.20585218759416));
#130922=CARTESIAN_POINT('Ctrl Pts',(6.61226633200001,1.714555786,3.53948216));
#130923=CARTESIAN_POINT('Ctrl Pts',(6.803866199,1.779135389,3.181545802));
#130924=CARTESIAN_POINT('Ctrl Pts',(6.955707935,1.844275173,2.805018204));
#130925=CARTESIAN_POINT('Ctrl Pts',(6.500628688,1.714555786,3.210035304));
#130926=CARTESIAN_POINT('Ctrl Pts',(6.674394881,1.779135389,2.858142135));
#130927=CARTESIAN_POINT('Ctrl Pts',(6.809159503,1.844275173,2.489547522));
#130928=CARTESIAN_POINT('Origin',(-0.187509082124542,1.87498563387379,-0.0630888866187446));
#130929=CARTESIAN_POINT('Ctrl Pts',(7.124630184,1.844275173,2.34299909));
#130930=CARTESIAN_POINT('Ctrl Pts',(7.218039533,1.796786772,2.058958406));
#130931=CARTESIAN_POINT('Ctrl Pts',(7.288540418,1.75,1.768383042));
#130932=CARTESIAN_POINT('Ctrl Pts',(7.31516391,1.73233175,1.658652065));
#130933=CARTESIAN_POINT('Ctrl Pts',(7.338472024,1.714550109,1.548169354));
#130934=CARTESIAN_POINT('Ctrl Pts',(6.809159503,1.844275173,2.489547522));
#130935=CARTESIAN_POINT('Ctrl Pts',(6.908411361,1.796786772,2.218083843));
#130936=CARTESIAN_POINT('Ctrl Pts',(6.985737446,1.75,1.939580454));
#130937=CARTESIAN_POINT('Ctrl Pts',(7.014938362,1.73233175,1.83440826));
#130938=CARTESIAN_POINT('Ctrl Pts',(7.040959969,1.714550109,1.728404675));
#130939=CARTESIAN_POINT('',(7.03982677265495,1.71532338719604,1.73301443461817));
#130940=CARTESIAN_POINT('Ctrl Pts',(7.03982676947817,1.7153233893999,1.73301444130634));
#130941=CARTESIAN_POINT('Ctrl Pts',(7.02278654487449,1.72693520766041,1.80223500036135));
#130942=CARTESIAN_POINT('Ctrl Pts',(7.00474976112088,1.73849644464533,1.87110428255116));
#130943=CARTESIAN_POINT('Ctrl Pts',(6.98573744584127,1.75000000009604,1.93958045457169));
#130944=CARTESIAN_POINT('Ctrl Pts',(6.9462281097166,1.77390544324813,2.08188022262457));
#130945=CARTESIAN_POINT('Ctrl Pts',(6.90223045660141,1.79806024608469,2.22346269816108));
#130946=CARTESIAN_POINT('Ctrl Pts',(6.85378979382319,1.82239963186884,2.3639089373963));
#130947=CARTESIAN_POINT('Ctrl Pts',(6.83930901925183,1.82967560908574,2.40589371244103));
#130948=CARTESIAN_POINT('Ctrl Pts',(6.82443155112805,1.83696805454724,2.44777695512015));
#130949=CARTESIAN_POINT('Ctrl Pts',(6.80915950245155,1.8442751738645,2.48954752360552));
#130950=CARTESIAN_POINT('Ctrl Pts',(7.28212026958201,1.75423096143692,1.7946376730125));
#130951=CARTESIAN_POINT('Ctrl Pts',(7.25432033648641,1.7499815324715,1.78751646127468));
#130952=CARTESIAN_POINT('Ctrl Pts',(7.22653223945985,1.74566717064373,1.78038734412662));
#130953=CARTESIAN_POINT('Ctrl Pts',(7.19874671596365,1.74127713116593,1.77329525216261));
#130954=CARTESIAN_POINT('Ctrl Pts',(7.17225057973697,1.73709081147826,1.76653226873937));
#130955=CARTESIAN_POINT('Ctrl Pts',(7.14575890002104,1.73283723877416,1.75979303987636));
#130956=CARTESIAN_POINT('Ctrl Pts',(7.11927244903046,1.72851290761131,1.75307913787034));
#130957=CARTESIAN_POINT('Ctrl Pts',(7.09278522507288,1.72418845024939,1.74636503992924));
#130958=CARTESIAN_POINT('Ctrl Pts',(7.06630303261031,1.71979319992597,1.73967621882733));
#130959=CARTESIAN_POINT('Ctrl Pts',(7.03982676944971,1.71532338471622,1.73301444351913));
#130960=CARTESIAN_POINT('Ctrl Pts',(7.218559257,1.714555786,2.03528923));
#130961=CARTESIAN_POINT('Ctrl Pts',(7.32873389,1.779135389,1.644532917));
#130962=CARTESIAN_POINT('Ctrl Pts',(7.396083347,1.844275173,1.24416684));
#130963=CARTESIAN_POINT('Ctrl Pts',(7.038710305,1.714555786,1.737543452));
#130964=CARTESIAN_POINT('Ctrl Pts',(7.13276731100001,1.779135389,1.356522755));
#130965=CARTESIAN_POINT('Ctrl Pts',(7.185144264,1.844275173,0.967575269));
#130966=CARTESIAN_POINT('Origin',(-0.196687366030756,1.87498564470105,-0.0213049812195722));
#130967=CARTESIAN_POINT('Ctrl Pts',(7.461735836,1.844275173,0.756636186000001));
#130968=CARTESIAN_POINT('Ctrl Pts',(7.491900975,1.796786772,0.459155966));
#130969=CARTESIAN_POINT('Ctrl Pts',(7.498288474,1.75,0.160218487));
#130970=CARTESIAN_POINT('Ctrl Pts',(7.500700607,1.73233175,0.047329695));
#130971=CARTESIAN_POINT('Ctrl Pts',(7.499713274,1.714550109,-0.065580547));
#130972=CARTESIAN_POINT('Ctrl Pts',(7.185144264,1.844275173,0.967575269));
#130973=CARTESIAN_POINT('Ctrl Pts',(7.223719002,1.796786772,0.681122044));
#130974=CARTESIAN_POINT('Ctrl Pts',(7.23936725,1.75,0.392507087));
#130975=CARTESIAN_POINT('Ctrl Pts',(7.245276552,1.73233175,0.283516426));
#130976=CARTESIAN_POINT('Ctrl Pts',(7.247902151,1.714550109,0.17439727));
#130977=CARTESIAN_POINT('',(7.2477864108896,1.71532338699242,0.179142860916561));
#130978=CARTESIAN_POINT('Ctrl Pts',(7.24778640962524,1.7153233894705,0.179142867162212));
#130979=CARTESIAN_POINT('Ctrl Pts',(7.24602494966089,1.72693520768405,0.250408232466979));
#130980=CARTESIAN_POINT('Ctrl Pts',(7.24321471541452,1.7384964446451,0.321544764467899));
#130981=CARTESIAN_POINT('Ctrl Pts',(7.23936725011237,1.75000000002696,0.392507087301587));
#130982=CARTESIAN_POINT('Ctrl Pts',(7.23137187607232,1.77390540851427,0.539973091694986));
#130983=CARTESIAN_POINT('Ctrl Pts',(7.21883893532828,1.7980601762294,0.687703429362648));
#130984=CARTESIAN_POINT('Ctrl Pts',(7.20172261620258,1.822399526404,0.835279211927122));
#130985=CARTESIAN_POINT('Ctrl Pts',(7.19660585891261,1.82967553864264,0.87939555818794));
#130986=CARTESIAN_POINT('Ctrl Pts',(7.19107985214801,1.83696801928899,0.923498023146735));
#130987=CARTESIAN_POINT('Ctrl Pts',(7.18514426436052,1.84427517391947,0.967575271034647));
#130988=CARTESIAN_POINT('Ctrl Pts',(7.4976623948633,1.75423096140896,0.187239441348413));
#130989=CARTESIAN_POINT('Ctrl Pts',(7.46898155867245,1.74998153245423,0.186260883320029));
#130990=CARTESIAN_POINT('Ctrl Pts',(7.4403105823626,1.7456671706257,0.185272060355469));
#130991=CARTESIAN_POINT('Ctrl Pts',(7.41165007873351,1.74127713114288,0.184318843757033));
#130992=CARTESIAN_POINT('Ctrl Pts',(7.38431956598644,1.7370908114746,0.183409861181869));
#130993=CARTESIAN_POINT('Ctrl Pts',(7.35699851208546,1.73283723878819,0.182523119811445));
#130994=CARTESIAN_POINT('Ctrl Pts',(7.32968800914164,1.72851290763471,0.181659989172753));
#130995=CARTESIAN_POINT('Ctrl Pts',(7.30237670927953,1.72418845029759,0.180796833347977));
#130996=CARTESIAN_POINT('Ctrl Pts',(7.27507575700033,1.71979319999011,0.179957281808602));
#130997=CARTESIAN_POINT('Ctrl Pts',(7.24778640920089,1.7153233848652,0.179142868459304));
#130998=CARTESIAN_POINT('Ctrl Pts',(7.487320375,1.714555786,0.435928437));
#130999=CARTESIAN_POINT('Ctrl Pts',(7.510918129,1.779135389,0.030623501));
#131000=CARTESIAN_POINT('Ctrl Pts',(7.490626122,1.844275173,-0.374860382));
#131001=CARTESIAN_POINT('Ctrl Pts',(7.24766965,1.714555786,0.183805999));
#131002=CARTESIAN_POINT('Ctrl Pts',(7.257619468,1.779135389,-0.208526122));
#131003=CARTESIAN_POINT('Ctrl Pts',(7.225159666,1.844275173,-0.599639729));
#131004=CARTESIAN_POINT('Origin',(-0.196669206806751,1.87498565714627,0.0214751056292038));
#131005=CARTESIAN_POINT('Ctrl Pts',(7.449939012,1.844275173,-0.865106183999999));
#131006=CARTESIAN_POINT('Ctrl Pts',(7.41544945400001,1.796786772,-1.162116095));
#131007=CARTESIAN_POINT('Ctrl Pts',(7.357424895,1.75,-1.455437707));
#131008=CARTESIAN_POINT('Ctrl Pts',(7.335512881,1.73233175,-1.566205758));
#131009=CARTESIAN_POINT('Ctrl Pts',(7.310276266,1.714550109,-1.676263974));
#131010=CARTESIAN_POINT('Ctrl Pts',(7.225159666,1.844275173,-0.599639729));
#131011=CARTESIAN_POINT('Ctrl Pts',(7.201253572,1.796786772,-0.887688265));
#131012=CARTESIAN_POINT('Ctrl Pts',(7.154492288,1.75,-1.172919475));
#131013=CARTESIAN_POINT('Ctrl Pts',(7.136833664,1.73233175,-1.28063232));
#131014=CARTESIAN_POINT('Ctrl Pts',(7.11594048400001,1.714550109,-1.387764758));
#131015=CARTESIAN_POINT('',(7.11684761175525,1.71532338698871,-1.38310523484352));
#131016=CARTESIAN_POINT('Ctrl Pts',(7.11684761179474,1.71532338938623,-1.38310522861952));
#131017=CARTESIAN_POINT('Ctrl Pts',(7.13044728108712,1.72693520765624,-1.31312734623891));
#131018=CARTESIAN_POINT('Ctrl Pts',(7.14299500024421,1.7384964446449,-1.24304982945737));
#131019=CARTESIAN_POINT('Ctrl Pts',(7.15449228822887,1.74999999996677,-1.17291947501433));
#131020=CARTESIAN_POINT('Ctrl Pts',(7.17838464095599,1.77390537580904,-1.02718257393111));
#131021=CARTESIAN_POINT('Ctrl Pts',(7.19790234835856,1.79806011041741,-0.880212078894142));
#131022=CARTESIAN_POINT('Ctrl Pts',(7.21291062193433,1.822399427013,-0.732407236428844));
#131023=CARTESIAN_POINT('Ctrl Pts',(7.21739722597261,1.82967547216072,-0.688222154131791));
#131024=CARTESIAN_POINT('Ctrl Pts',(7.22148116085493,1.83696798586838,-0.643962651336697));
#131025=CARTESIAN_POINT('Ctrl Pts',(7.22515966590222,1.84427517368027,-0.599639727699752));
#131026=CARTESIAN_POINT('Ctrl Pts',(7.36262215969342,1.75423096149365,-1.42891389841392));
#131027=CARTESIAN_POINT('Ctrl Pts',(7.33440150456365,1.74998153254278,-1.42370404627898));
#131028=CARTESIAN_POINT('Ctrl Pts',(7.30618827216476,1.74566717068936,-1.41850633850759));
#131029=CARTESIAN_POINT('Ctrl Pts',(7.27799292189134,1.74127713120157,-1.4132761082767));
#131030=CARTESIAN_POINT('Ctrl Pts',(7.25110597695037,1.73709081151225,-1.40828858689877));
#131031=CARTESIAN_POINT('Ctrl Pts',(7.22423305089781,1.73283723881738,-1.40328137776424));
#131032=CARTESIAN_POINT('Ctrl Pts',(7.1973755047234,1.72851290767054,-1.39825337815015));
#131033=CARTESIAN_POINT('Ctrl Pts',(7.17051717483185,1.72418845033747,-1.39322523181642));
#131034=CARTESIAN_POINT('Ctrl Pts',(7.14367402481404,1.7197932000495,-1.38817625758044));
#131035=CARTESIAN_POINT('Ctrl Pts',(7.11684761220601,1.71532338486886,-1.38310522694114));
#131036=CARTESIAN_POINT('Ctrl Pts',(7.405982713,1.714555786,-1.183815884));
#131037=CARTESIAN_POINT('Ctrl Pts',(7.34190018500001,1.779135389,-1.584717836));
#131038=CARTESIAN_POINT('Ctrl Pts',(7.234915544,1.844275173,-1.976359549));
#131039=CARTESIAN_POINT('Ctrl Pts',(7.11773601800001,1.714555786,-1.378526018));
#131040=CARTESIAN_POINT('Ctrl Pts',(7.043113406,1.779135389,-1.763824549));
#131041=CARTESIAN_POINT('Ctrl Pts',(6.92733463100001,1.844275173,-2.138816239));
#131042=CARTESIAN_POINT('Origin',(-0.187454516868641,1.87498563159744,0.0632510508886766));
#131043=CARTESIAN_POINT('Ctrl Pts',(7.089791321,1.844275173,-2.446397152));
#131044=CARTESIAN_POINT('Ctrl Pts',(6.992259758,1.796786772,-2.7290489));
#131045=CARTESIAN_POINT('Ctrl Pts',(6.872536305,1.75,-3.00303925));
#131046=CARTESIAN_POINT('Ctrl Pts',(6.827324725,1.73233175,-3.106507171));
#131047=CARTESIAN_POINT('Ctrl Pts',(6.779018865,1.714550109,-3.208567161));
#131048=CARTESIAN_POINT('Ctrl Pts',(6.927334631,1.844275173,-2.138816239));
#131049=CARTESIAN_POINT('Ctrl Pts',(6.842065528,1.796786772,-2.414991257));
#131050=CARTESIAN_POINT('Ctrl Pts',(6.735081219,1.75,-2.683501626));
#131051=CARTESIAN_POINT('Ctrl Pts',(6.69468036500001,1.73233175,-2.784900123));
#131052=CARTESIAN_POINT('Ctrl Pts',(6.651245349,1.714550109,-2.885036447));
#131053=CARTESIAN_POINT('',(6.65313292778536,1.71532338722933,-2.88068086811694));
#131054=CARTESIAN_POINT('Ctrl Pts',(6.65313292980567,1.71532338938004,-2.88068086059141));
#131055=CARTESIAN_POINT('Ctrl Pts',(6.68145782268044,1.7269352076563,-2.81526254923147));
#131056=CARTESIAN_POINT('Ctrl Pts',(6.70877677796881,1.73849644464498,-2.74952079466792));
#131057=CARTESIAN_POINT('Ctrl Pts',(6.73508121897836,1.74999999999054,-2.68350162605432));
#131058=CARTESIAN_POINT('Ctrl Pts',(6.78974406744588,1.77390535875619,-2.54630822084171));
#131059=CARTESIAN_POINT('Ctrl Pts',(6.84039974034393,1.79806007584213,-2.40696964593335));
#131060=CARTESIAN_POINT('Ctrl Pts',(6.88683077358647,1.82239937471913,-2.26584683728512));
#131061=CARTESIAN_POINT('Ctrl Pts',(6.90071100498353,1.82967543723296,-2.22365916445846));
#131062=CARTESIAN_POINT('Ctrl Pts',(6.91421397780518,1.83696796839194,-2.18131224827326));
#131063=CARTESIAN_POINT('Ctrl Pts',(6.92733463124804,1.84427517373051,-2.13881623783067));
#131064=CARTESIAN_POINT('Ctrl Pts',(6.88331389536588,1.75423096141576,-2.97825281206678));
#131065=CARTESIAN_POINT('Ctrl Pts',(6.85687298763967,1.74998153248078,-2.96709815684415));
#131066=CARTESIAN_POINT('Ctrl Pts',(6.83043671842837,1.74566717062983,-2.95595695765252));
#131067=CARTESIAN_POINT('Ctrl Pts',(6.80402490463477,1.74127713115002,-2.94478784049848));
#131068=CARTESIAN_POINT('Ctrl Pts',(6.77883873113512,1.73709081146473,-2.93413702625764));
#131069=CARTESIAN_POINT('Ctrl Pts',(6.75367048106214,1.73283723877631,-2.92346999819169));
#131070=CARTESIAN_POINT('Ctrl Pts',(6.72852172072704,1.72851290764213,-2.91278597190329));
#131071=CARTESIAN_POINT('Ctrl Pts',(6.70337222640133,1.72418845029822,-2.90210163379136));
#131072=CARTESIAN_POINT('Ctrl Pts',(6.67824203453034,1.71979320000627,-2.89140021791908));
#131073=CARTESIAN_POINT('Ctrl Pts',(6.65313293024291,1.71532338480356,-2.88068085923549));
#131074=CARTESIAN_POINT('Ctrl Pts',(6.978349531,1.714555786,-2.748206291));
#131075=CARTESIAN_POINT('Ctrl Pts',(6.829583148,1.779135389,-3.125959528));
#131076=CARTESIAN_POINT('Ctrl Pts',(6.640908357,1.844275173,-3.485446341));
#131077=CARTESIAN_POINT('Ctrl Pts',(6.65498496,1.714555786,-2.876399691));
#131078=CARTESIAN_POINT('Ctrl Pts',(6.499279189,1.779135389,-3.236648501));
#131079=CARTESIAN_POINT('Ctrl Pts',(6.30559512900001,1.844275173,-3.577984079));
#131080=CARTESIAN_POINT('Origin',(-0.169474786281197,1.87498566159976,0.102069443457045));
#131081=CARTESIAN_POINT('Ctrl Pts',(6.398132867,1.844275173,-3.913297307));
#131082=CARTESIAN_POINT('Ctrl Pts',(6.242119767,1.796786772,-4.168374412));
#131083=CARTESIAN_POINT('Ctrl Pts',(6.066295556,1.75,-4.410222016));
#131084=CARTESIAN_POINT('Ctrl Pts',(5.999898453,1.73233175,-4.501551761));
#131085=CARTESIAN_POINT('Ctrl Pts',(5.930782076,1.714550109,-4.590841313));
#131086=CARTESIAN_POINT('Ctrl Pts',(6.305595129,1.844275173,-3.577984079));
#131087=CARTESIAN_POINT('Ctrl Pts',(6.162950104,1.796786772,-3.829371942));
#131088=CARTESIAN_POINT('Ctrl Pts',(6.000745237,1.75,-4.068606224));
#131089=CARTESIAN_POINT('Ctrl Pts',(5.939491253,1.73233175,-4.158949091));
#131090=CARTESIAN_POINT('Ctrl Pts',(5.875545374,1.714550109,-4.247407039));
#131091=CARTESIAN_POINT('',(5.87832514394337,1.7153233870063,-4.24355906365207));
#131092=CARTESIAN_POINT('Ctrl Pts',(5.87832514675913,1.71532338943757,-4.24355905786656));
#131093=CARTESIAN_POINT('Ctrl Pts',(5.92005082188062,1.72693520767362,-4.18575920521102));
#131094=CARTESIAN_POINT('Ctrl Pts',(5.96086360898721,1.73849644464494,-4.12742722417017));
#131095=CARTESIAN_POINT('Ctrl Pts',(6.00074523693298,1.74999999998067,-4.06860622409885));
#131096=CARTESIAN_POINT('Ctrl Pts',(6.08362259649407,1.77390535047736,-3.94637126312403));
#131097=CARTESIAN_POINT('Ctrl Pts',(6.16304761652092,1.7980600591429,-3.82117986309644));
#131098=CARTESIAN_POINT('Ctrl Pts',(6.23873032669115,1.82239934946658,-3.6933377730755));
#131099=CARTESIAN_POINT('Ctrl Pts',(6.26135517561757,1.8296754203857,-3.65512022025984));
#131100=CARTESIAN_POINT('Ctrl Pts',(6.28364581790097,1.83696795998772,-3.61666604713042));
#131101=CARTESIAN_POINT('Ctrl Pts',(6.30559512927184,1.84427517379952,-3.57798407762311));
#131102=CARTESIAN_POINT('Ctrl Pts',(6.08214952361998,1.75423096141961,-4.38833193459233));
#131103=CARTESIAN_POINT('Ctrl Pts',(6.05872471075126,1.74998153245681,-4.37175405532098));
#131104=CARTESIAN_POINT('Ctrl Pts',(6.03530153526694,1.74566717060285,-4.35519031474403));
#131105=CARTESIAN_POINT('Ctrl Pts',(6.01190824498387,1.74127713111933,-4.33860456609043));
#131106=CARTESIAN_POINT('Ctrl Pts',(5.98960052047753,1.73709081144454,-4.32278847920317));
#131107=CARTESIAN_POINT('Ctrl Pts',(5.96731378585211,1.73283723876601,-4.30696041055451));
#131108=CARTESIAN_POINT('Ctrl Pts',(5.94504973934713,1.72851290762539,-4.29111993073684));
#131109=CARTESIAN_POINT('Ctrl Pts',(5.92278504321281,1.72418845030769,-4.27527898871925));
#131110=CARTESIAN_POINT('Ctrl Pts',(5.9005428693928,1.71979320002457,-4.25942551758569));
#131111=CARTESIAN_POINT('Ctrl Pts',(5.87832514674664,1.71532338488821,-4.24355905666755));
#131112=CARTESIAN_POINT('Ctrl Pts',(6.224416481,1.714555786,-4.184093626));
#131113=CARTESIAN_POINT('Ctrl Pts',(5.997922393,1.779135389,-4.521034827));
#131114=CARTESIAN_POINT('Ctrl Pts',(5.736379676,1.844275173,-4.831557535));
#131115=CARTESIAN_POINT('Ctrl Pts',(5.881054202,1.714555786,-4.239776111));
#131116=CARTESIAN_POINT('Ctrl Pts',(5.6515459,1.779135389,-4.558130366));
#131117=CARTESIAN_POINT('Ctrl Pts',(5.389013006,1.844275173,-4.84984936));
#131118=CARTESIAN_POINT('Origin',(-0.143570649467616,1.87498566364901,0.136115196854825));
#131119=CARTESIAN_POINT('Ctrl Pts',(5.407304832,1.844275173,-5.19721603));
#131120=CARTESIAN_POINT('Ctrl Pts',(5.200105193,1.796786772,-5.412791368));
#131121=CARTESIAN_POINT('Ctrl Pts',(4.976401568,1.75,-5.611187702));
#131122=CARTESIAN_POINT('Ctrl Pts',(4.891923597,1.73233175,-5.686108794));
#131123=CARTESIAN_POINT('Ctrl Pts',(4.805228509,1.714550109,-5.75845282800001));
#131124=CARTESIAN_POINT('Ctrl Pts',(5.389013006,1.844275173,-4.84984936));
#131125=CARTESIAN_POINT('Ctrl Pts',(5.195661984,1.796786772,-5.06469545100001));
#131126=CARTESIAN_POINT('Ctrl Pts',(4.985821077,1.75,-5.263467316));
#131127=CARTESIAN_POINT('Ctrl Pts',(4.906578131,1.73233175,-5.338530221));
#131128=CARTESIAN_POINT('Ctrl Pts',(4.825111428,1.714550109,-5.411173598));
#131129=CARTESIAN_POINT('',(4.82865340810967,1.71532338695943,-5.40801315424955));
#131130=CARTESIAN_POINT('Ctrl Pts',(4.82865341177974,1.71532338935395,-5.40801314937509));
#131131=CARTESIAN_POINT('Ctrl Pts',(4.88182882469613,1.72693520764639,-5.36053441211114));
#131132=CARTESIAN_POINT('Ctrl Pts',(4.93422708346645,1.73849644464463,-5.31233974310289));
#131133=CARTESIAN_POINT('Ctrl Pts',(4.98582107697322,1.74999999988717,-5.26346731649234));
#131134=CARTESIAN_POINT('Ctrl Pts',(5.09303762256744,1.77390532985231,-5.16190641121414));
#131135=CARTESIAN_POINT('Ctrl Pts',(5.19751809382533,1.79806001794096,-5.05671604018305));
#131136=CARTESIAN_POINT('Ctrl Pts',(5.29891357386326,1.8223992873886,-4.94813247038953));
#131137=CARTESIAN_POINT('Ctrl Pts',(5.32922519817982,1.82967537890037,-4.91567200594574));
#131138=CARTESIAN_POINT('Ctrl Pts',(5.35926129425477,1.83696793918965,-4.88290860695238));
#131139=CARTESIAN_POINT('Ctrl Pts',(5.38901300743212,1.84427517375631,-4.84984935964758));
#131140=CARTESIAN_POINT('Ctrl Pts',(4.99659059962593,1.75423096137881,-5.59321753312504));
#131141=CARTESIAN_POINT('Ctrl Pts',(4.9772771996466,1.74998153250547,-5.57199159351297));
#131142=CARTESIAN_POINT('Ctrl Pts',(4.95796235969366,1.7456671706527,-5.5507798136574));
#131143=CARTESIAN_POINT('Ctrl Pts',(4.93868143733802,1.74127713116747,-5.52955296470416));
#131144=CARTESIAN_POINT('Ctrl Pts',(4.92029524621638,1.73709081147187,-5.50931114771194));
#131145=CARTESIAN_POINT('Ctrl Pts',(4.90193212997671,1.73283723877001,-5.4890621412984));
#131146=CARTESIAN_POINT('Ctrl Pts',(4.88359383955079,1.72851290761803,-5.46880589124527));
#131147=CARTESIAN_POINT('Ctrl Pts',(4.86525501387076,1.72418845024839,-5.44854904995705));
#131148=CARTESIAN_POINT('Ctrl Pts',(4.84694087742774,1.71979319992644,-5.42828481420679));
#131149=CARTESIAN_POINT('Ctrl Pts',(4.82865341408233,1.7153233846591,-5.40801314835518));
#131150=CARTESIAN_POINT('Ctrl Pts',(5.179436634,1.714555786,-5.424337393));
#131151=CARTESIAN_POINT('Ctrl Pts',(4.885805454,1.779135389,-5.704711563));
#131152=CARTESIAN_POINT('Ctrl Pts',(4.563624257,1.844275173,-5.951750469));
#131153=CARTESIAN_POINT('Ctrl Pts',(4.832131886,1.714555786,-5.404905313));
#131154=CARTESIAN_POINT('Ctrl Pts',(4.539552606,1.779135389,-5.666479121));
#131155=CARTESIAN_POINT('Ctrl Pts',(4.220446625,1.844275173,-5.894941076));
#131156=CARTESIAN_POINT('Origin',(-0.110953220978337,1.87498565391221,0.163796221188096));
#131157=CARTESIAN_POINT('Ctrl Pts',(4.163637232,1.844275173,-6.238118707));
#131158=CARTESIAN_POINT('Ctrl Pts',(3.91493948,1.796786772,-6.404112217));
#131159=CARTESIAN_POINT('Ctrl Pts',(3.653816575,1.75,-6.549780488));
#131160=CARTESIAN_POINT('Ctrl Pts',(3.555207832,1.73233175,-6.60478969900001));
#131161=CARTESIAN_POINT('Ctrl Pts',(3.454987798,1.714550109,-6.656805489));
#131162=CARTESIAN_POINT('Ctrl Pts',(4.220446625,1.844275173,-5.894941076));
#131163=CARTESIAN_POINT('Ctrl Pts',(3.985430483,1.796786772,-6.06319943));
#131164=CARTESIAN_POINT('Ctrl Pts',(3.737765465,1.75,-6.212214527));
#131165=CARTESIAN_POINT('Ctrl Pts',(3.64423887,1.73233175,-6.268487612));
#131166=CARTESIAN_POINT('Ctrl Pts',(3.549060633,1.714550109,-6.321919694));
#131167=CARTESIAN_POINT('',(3.5531992049754,1.71532338719967,-6.31959456164931));
#131168=CARTESIAN_POINT('Ctrl Pts',(3.55319921057251,1.71532338934942,-6.31959455693109));
#131169=CARTESIAN_POINT('Ctrl Pts',(3.61533793732367,1.72693520764435,-6.28465698753141));
#131170=CARTESIAN_POINT('Ctrl Pts',(3.67687158329099,1.73849644464494,-6.24885315985814));
#131171=CARTESIAN_POINT('Ctrl Pts',(3.73776546488684,1.74999999997862,-6.21221452706809));
#131172=CARTESIAN_POINT('Ctrl Pts',(3.86430804125286,1.77390534937231,-6.13607638508135));
#131173=CARTESIAN_POINT('Ctrl Pts',(3.98895873611091,1.79806005694259,-6.05580545205442));
#131174=CARTESIAN_POINT('Ctrl Pts',(4.11132599884036,1.82239934618419,-5.97155746290186));
#131175=CARTESIAN_POINT('Ctrl Pts',(4.14790689513797,1.8296754181976,-5.94637207519497));
#131176=CARTESIAN_POINT('Ctrl Pts',(4.18428382795472,1.83696795890152,-5.9208316068493));
#131177=CARTESIAN_POINT('Ctrl Pts',(4.22044662639856,1.84427517382187,-5.894941074851));
#131178=CARTESIAN_POINT('Ctrl Pts',(3.67739665300579,1.75423096143411,-6.53657049633415));
#131179=CARTESIAN_POINT('Ctrl Pts',(3.66309773951689,1.74998153247552,-6.51168899697367));
#131180=CARTESIAN_POINT('Ctrl Pts',(3.64879437539372,1.74566717062461,-6.48682101708093));
#131181=CARTESIAN_POINT('Ctrl Pts',(3.63452737529584,1.74127713113628,-6.46194561166913));
#131182=CARTESIAN_POINT('Ctrl Pts',(3.62092243537416,1.7370908114417,-6.4382245495094));
#131183=CARTESIAN_POINT('Ctrl Pts',(3.60734157634775,1.73283723873845,-6.4145014264286));
#131184=CARTESIAN_POINT('Ctrl Pts',(3.59378651978766,1.72851290758898,-6.39077656588435));
#131185=CARTESIAN_POINT('Ctrl Pts',(3.58023106762785,1.72418845023538,-6.36705101293812));
#131186=CARTESIAN_POINT('Ctrl Pts',(3.56670131697463,1.71979319993311,-6.34332354586962));
#131187=CARTESIAN_POINT('Ctrl Pts',(3.5531992128619,1.71532338470336,-6.31959455638273));
#131188=CARTESIAN_POINT('Ctrl Pts',(3.892272087,1.714555786,-6.410945172));
#131189=CARTESIAN_POINT('Ctrl Pts',(3.545233681,1.779135389,-6.621642326));
#131190=CARTESIAN_POINT('Ctrl Pts',(3.177478839,1.844275173,-6.793646166));
#131191=CARTESIAN_POINT('Ctrl Pts',(3.557264453,1.714555786,-6.317307149));
#131192=CARTESIAN_POINT('Ctrl Pts',(3.215294878,1.779135389,-6.50986961));
#131193=CARTESIAN_POINT('Ctrl Pts',(2.85453685,1.844275173,-6.664391898));
#131194=CARTESIAN_POINT('Origin',(-0.0731479700179943,1.87498564855422,
0.183818649927637));
#131195=CARTESIAN_POINT('Ctrl Pts',(2.725282582,1.844275173,-6.987333887));
#131196=CARTESIAN_POINT('Ctrl Pts',(2.446715548,1.796786772,-7.095983895));
#131197=CARTESIAN_POINT('Ctrl Pts',(2.160383179,1.75,-7.182112817));
#131198=CARTESIAN_POINT('Ctrl Pts',(2.052254499,1.73233175,-7.21463797899999));
#131199=CARTESIAN_POINT('Ctrl Pts',(1.943195696,1.714550109,-7.243893324));
#131200=CARTESIAN_POINT('Ctrl Pts',(2.85453685,1.844275173,-6.664391898));
#131201=CARTESIAN_POINT('Ctrl Pts',(2.588844683,1.796786772,-6.778194942));
#131202=CARTESIAN_POINT('Ctrl Pts',(2.314936093,1.75,-6.870485491));
#131203=CARTESIAN_POINT('Ctrl Pts',(2.211499049,1.73233175,-6.905337489));
#131204=CARTESIAN_POINT('Ctrl Pts',(2.107059708,1.714550109,-6.937059852));
#131205=CARTESIAN_POINT('',(2.11160135746148,1.71532338716952,-6.93567875019962));
#131206=CARTESIAN_POINT('Ctrl Pts',(2.11160136389839,1.71532338936648,-6.93567874676857));
#131207=CARTESIAN_POINT('Ctrl Pts',(2.17979786577418,1.72693520764907,-6.91491598770769));
#131208=CARTESIAN_POINT('Ctrl Pts',(2.24758965350799,1.73849644464509,-6.893177148517));
#131209=CARTESIAN_POINT('Ctrl Pts',(2.31493609321961,1.75000000002331,-6.87048549099526));
#131210=CARTESIAN_POINT('Ctrl Pts',(2.45488789203671,1.7739053949493,-6.82333023983162));
#131211=CARTESIAN_POINT('Ctrl Pts',(2.59388046275683,1.79806014881565,-6.77173210473685));
#131212=CARTESIAN_POINT('Ctrl Pts',(2.73149792979389,1.82239948494412,-6.71575900811587));
#131213=CARTESIAN_POINT('Ctrl Pts',(2.77263743592456,1.82967551094163,-6.69902635345241));
#131214=CARTESIAN_POINT('Ctrl Pts',(2.81365408042104,1.83696800541057,-6.68190307860387));
#131215=CARTESIAN_POINT('Ctrl Pts',(2.8545368519287,1.84427517391657,-6.66439189675992));
#131216=CARTESIAN_POINT('Ctrl Pts',(2.18625172552816,1.75423096135723,-7.17428068773433));
#131217=CARTESIAN_POINT('Ctrl Pts',(2.17763589926552,1.74998153246511,-7.14690706044567));
#131218=CARTESIAN_POINT('Ctrl Pts',(2.16901282041771,1.74566717062331,-7.11954567964696));
#131219=CARTESIAN_POINT('Ctrl Pts',(2.16042685174637,1.74127713113718,-7.09218486411791));
#131220=CARTESIAN_POINT('Ctrl Pts',(2.15223931497369,1.73709081144488,-7.06609372730505));
#131221=CARTESIAN_POINT('Ctrl Pts',(2.14407573916766,1.732837238741,-7.04000575443481));
#131222=CARTESIAN_POINT('Ctrl Pts',(2.1359377360913,1.72851290757632,-7.01392163141829));
#131223=CARTESIAN_POINT('Ctrl Pts',(2.12779949554998,1.72418845022869,-6.98783674727334));
#131224=CARTESIAN_POINT('Ctrl Pts',(2.11968676711798,1.71979319991724,-6.96175551874662));
#131225=CARTESIAN_POINT('Ctrl Pts',(2.11160136600415,1.71532338469401,-6.93567874658361));
#131226=CARTESIAN_POINT('Ctrl Pts',(2.423109222,1.714555786,-7.097784281));
#131227=CARTESIAN_POINT('Ctrl Pts',(2.038890722,1.779135389,-7.228952453));
#131228=CARTESIAN_POINT('Ctrl Pts',(1.642758043,1.844275173,-7.317878519));
#131229=CARTESIAN_POINT('Ctrl Pts',(2.116063288,1.714555786,-6.934318724));
#131230=CARTESIAN_POINT('Ctrl Pts',(1.740693535,1.779135389,-7.048865831));
#131231=CARTESIAN_POINT('Ctrl Pts',(1.355152105,1.844275173,-7.122223162));
#131232=CARTESIAN_POINT('Origin',(-0.031922228289937,1.87498560777645,0.195245673609244));
#131233=CARTESIAN_POINT('Ctrl Pts',(1.159496749,1.844275173,-7.4098291));
#131234=CARTESIAN_POINT('Ctrl Pts',(0.864085917,1.796786772,-7.456055254));
#131235=CARTESIAN_POINT('Ctrl Pts',(0.565932667,1.75,-7.478617534));
#131236=CARTESIAN_POINT('Ctrl Pts',(0.453340027,1.73233175,-7.487137805));
#131237=CARTESIAN_POINT('Ctrl Pts',(0.340541924,1.714550109,-7.492264758));
#131238=CARTESIAN_POINT('Ctrl Pts',(1.355152105,1.844275173,-7.122223162));
#131239=CARTESIAN_POINT('Ctrl Pts',(1.071207382,1.796786772,-7.176249592));
#131240=CARTESIAN_POINT('Ctrl Pts',(0.783862884,1.75,-7.207500189));
#131241=CARTESIAN_POINT('Ctrl Pts',(0.67535199,1.73233175,-7.21930146));
#131242=CARTESIAN_POINT('Ctrl Pts',(0.566535013,1.714550109,-7.22783080000001));
#131243=CARTESIAN_POINT('',(0.571267377317762,1.71532338719877,-7.22745830883115));
#131244=CARTESIAN_POINT('Ctrl Pts',(0.571267384531206,1.71532338937434,
-7.22745830685143));
#131245=CARTESIAN_POINT('Ctrl Pts',(0.642332869732959,1.72693520765293,
-7.22184120144342));
#131246=CARTESIAN_POINT('Ctrl Pts',(0.713212931112191,1.73849644464485,
-7.21518383454917));
#131247=CARTESIAN_POINT('Ctrl Pts',(0.783862883888383,1.74999999995389,
-7.20750018916874));
#131248=CARTESIAN_POINT('Ctrl Pts',(0.930679421736194,1.77390535412743,
-7.19153292890536));
#131249=CARTESIAN_POINT('Ctrl Pts',(1.07751424809532,1.79806006666806,-7.17102046623649));
#131250=CARTESIAN_POINT('Ctrl Pts',(1.22394660966233,1.82239936091677,-7.14593973521569));
#131251=CARTESIAN_POINT('Ctrl Pts',(1.26772157230118,1.82967542807154,-7.13844202055999));
#131252=CARTESIAN_POINT('Ctrl Pts',(1.31146051721306,1.83696796389124,-7.13053640196224));
#131253=CARTESIAN_POINT('Ctrl Pts',(1.35515210699587,1.84427517390224,-7.12222316208742));
#131254=CARTESIAN_POINT('Ctrl Pts',(0.592880097673218,1.75423096140348,
-7.47652948817272));
#131255=CARTESIAN_POINT('Ctrl Pts',(0.590350225508527,1.74998153246448,
-7.44794369301217));
#131256=CARTESIAN_POINT('Ctrl Pts',(0.587810637439113,1.74566717063106,
-7.41936829903185));
#131257=CARTESIAN_POINT('Ctrl Pts',(0.585307170438711,1.74127713115372,
-7.3908014346883));
#131258=CARTESIAN_POINT('Ctrl Pts',(0.582919876829699,1.7370908114675,-7.36356021574434));
#131259=CARTESIAN_POINT('Ctrl Pts',(0.580555303863958,1.73283723876916,
-7.33632723766341));
#131260=CARTESIAN_POINT('Ctrl Pts',(0.578214878173422,1.72851290761529,
-7.30910351682742));
#131261=CARTESIAN_POINT('Ctrl Pts',(0.575874384186324,1.724188450272,-7.28187900156907));
#131262=CARTESIAN_POINT('Ctrl Pts',(0.573558020025772,1.71979319997028,
-7.25466354083005));
#131263=CARTESIAN_POINT('Ctrl Pts',(0.571267386158136,1.7153233847658,-7.22745830671902));
#131264=CARTESIAN_POINT('Ctrl Pts',(0.840644464,1.714555786,-7.452738885));
#131265=CARTESIAN_POINT('Ctrl Pts',(0.437211499,1.779135389,-7.49824479800001));
#131266=CARTESIAN_POINT('Ctrl Pts',(0.031223706,1.844275173,-7.499935005));
#131267=CARTESIAN_POINT('Ctrl Pts',(0.575917356,1.714555786,-7.22708926200001));
#131268=CARTESIAN_POINT('Ctrl Pts',(0.184699296,1.779135389,-7.258264921));
#131269=CARTESIAN_POINT('Ctrl Pts',(-0.207598047,1.844275173,-7.247027187));
#131270=CARTESIAN_POINT('Origin',(0.0107961689541792,1.8749856554977,0.19754299577718));
#131271=CARTESIAN_POINT('Ctrl Pts',(-0.460505865,1.844275173,-7.48584894));
#131272=CARTESIAN_POINT('Ctrl Pts',(-0.758947412,1.796786772,-7.467489755));
#131273=CARTESIAN_POINT('Ctrl Pts',(-1.054980228,1.75,-7.425430406));
#131274=CARTESIAN_POINT('Ctrl Pts',(-1.166772121,1.73233175,-7.409547389));
#131275=CARTESIAN_POINT('Ctrl Pts',(-1.27803521,1.714550109,-7.390306218));
#131276=CARTESIAN_POINT('Ctrl Pts',(-0.207598047,1.844275173,-7.247027187));
#131277=CARTESIAN_POINT('Ctrl Pts',(-0.496518385,1.796786772,-7.238750787));
#131278=CARTESIAN_POINT('Ctrl Pts',(-0.783862884,1.75,-7.207500189));
#131279=CARTESIAN_POINT('Ctrl Pts',(-0.892373777000001,1.73233175,-7.19569891800001));
#131280=CARTESIAN_POINT('Ctrl Pts',(-1.00048023,1.714550109,-7.18063641400001));
#131281=CARTESIAN_POINT('',(-0.995778431050306,1.7153233872116,-7.18128994946387));
#131282=CARTESIAN_POINT('Ctrl Pts',(-0.995778423627768,1.71532338936346,
-7.1812899489929));
#131283=CARTESIAN_POINT('Ctrl Pts',(-0.925166898717766,1.72693520764936,
-7.19108114745931));
#131284=CARTESIAN_POINT('Ctrl Pts',(-0.854512836891311,1.7384964446448,
-7.19981654411594));
#131285=CARTESIAN_POINT('Ctrl Pts',(-0.783862883933284,1.74999999993805,
-7.20750018951493));
#131286=CARTESIAN_POINT('Ctrl Pts',(-0.637046086122069,1.77390539626308,
-7.22346747988324));
#131287=CARTESIAN_POINT('Ctrl Pts',(-0.489234340772536,1.79806015189128,
-7.23499974628836));
#131288=CARTESIAN_POINT('Ctrl Pts',(-0.340833606960876,1.82239948974368,
-7.24198401373006));
#131289=CARTESIAN_POINT('Ctrl Pts',(-0.296470552966318,1.82967551413793,
-7.24407189716345));
#131290=CARTESIAN_POINT('Ctrl Pts',(-0.252054988031275,1.8369680069904,
-7.24575367526172));
#131291=CARTESIAN_POINT('Ctrl Pts',(-0.207598045031906,1.84427517385712,
-7.24702718695691));
#131292=CARTESIAN_POINT('Ctrl Pts',(-1.02821394492889,1.75423096140346,
-7.42918407887295));
#131293=CARTESIAN_POINT('Ctrl Pts',(-1.02453956940233,1.7499815325155,-7.40072275602745));
#131294=CARTESIAN_POINT('Ctrl Pts',(-1.0208769182417,1.7456671706696,-7.37226950252867));
#131295=CARTESIAN_POINT('Ctrl Pts',(-1.01718082414328,1.74127713118194,
-7.34383234421274));
#131296=CARTESIAN_POINT('Ctrl Pts',(-1.0136562473036,1.73709081149108,-7.31671481232162));
#131297=CARTESIAN_POINT('Ctrl Pts',(-1.01011125257461,1.73283723879007,
-7.28961021289635));
#131298=CARTESIAN_POINT('Ctrl Pts',(-1.00654466515591,1.72851290763796,
-7.26251984527877));
#131299=CARTESIAN_POINT('Ctrl Pts',(-1.00297797364889,1.72418845028333,
-7.23542868704812));
#131300=CARTESIAN_POINT('Ctrl Pts',(-0.999389662915626,1.71979319997506,
-7.20835155888954));
#131301=CARTESIAN_POINT('Ctrl Pts',(-0.995778421714262,1.71532338474605,
-7.18128994961304));
#131302=CARTESIAN_POINT('Ctrl Pts',(-0.781127895000001,1.714555786,-7.459211702));
#131303=CARTESIAN_POINT('Ctrl Pts',(-1.184911248,1.779135389,-7.41692755));
#131304=CARTESIAN_POINT('Ctrl Pts',(-1.581770616,1.844275173,-7.331302866));
#131305=CARTESIAN_POINT('Ctrl Pts',(-0.991157831999999,1.714555786,-7.181929139));
#131306=CARTESIAN_POINT('Ctrl Pts',(-1.379931276,1.779135389,-7.12827561));
#131307=CARTESIAN_POINT('Ctrl Pts',(-1.760641144,1.844275173,-7.032968275));
#131308=CARTESIAN_POINT('Origin',(0.0530096988521347,1.87498560675979,0.190603958778421));
#131309=CARTESIAN_POINT('Ctrl Pts',(-2.058975735,1.844275173,-7.211838803));
#131310=CARTESIAN_POINT('Ctrl Pts',(-2.346493203,1.796786772,-7.129752735));
#131311=CARTESIAN_POINT('Ctrl Pts',(-2.62656342,1.75,-7.025038406));
#131312=CARTESIAN_POINT('Ctrl Pts',(-2.732327301,1.73233175,-6.98549477199999));
#131313=CARTESIAN_POINT('Ctrl Pts',(-2.836852838,1.714550109,-6.94278517400001));
#131314=CARTESIAN_POINT('Ctrl Pts',(-1.760641144,1.844275173,-7.032968275));
#131315=CARTESIAN_POINT('Ctrl Pts',(-2.041027504,1.796786772,-6.96277604));
#131316=CARTESIAN_POINT('Ctrl Pts',(-2.314936093,1.75,-6.870485491));
#131317=CARTESIAN_POINT('Ctrl Pts',(-2.418373138,1.73233175,-6.835633493));
#131318=CARTESIAN_POINT('Ctrl Pts',(-2.520714129,1.714550109,-6.79768345));
#131319=CARTESIAN_POINT('',(-2.51626274462168,1.71532338697785,-6.79933245394681));
#131320=CARTESIAN_POINT('Ctrl Pts',(-2.51626273833866,1.71532338937276,
-6.79933245505572));
#131321=CARTESIAN_POINT('Ctrl Pts',(-2.44940689025209,1.72693520765307,
-6.82407413079242));
#131322=CARTESIAN_POINT('Ctrl Pts',(-2.38228253315872,1.7384964446447,-6.84779383348064));
#131323=CARTESIAN_POINT('Ctrl Pts',(-2.31493609343453,1.74999999990727,
-6.87048549103555));
#131324=CARTESIAN_POINT('Ctrl Pts',(-2.17498473716275,1.7739053193183,-6.91764059378519));
#131325=CARTESIAN_POINT('Ctrl Pts',(-2.03310830652878,1.79805999654194,
-6.96067827377804));
#131326=CARTESIAN_POINT('Ctrl Pts',(-1.88967898132039,1.82239925498918,
-6.9994009276728));
#131327=CARTESIAN_POINT('Ctrl Pts',(-1.84680148610072,1.82967535725213,
-7.01097687565173));
#131328=CARTESIAN_POINT('Ctrl Pts',(-1.80378540390959,1.83696792834415,
-7.0221674928574));
#131329=CARTESIAN_POINT('Ctrl Pts',(-1.7606411431672,1.8442751737596,-7.03296827530728));
#131330=CARTESIAN_POINT('Ctrl Pts',(-2.60122984628299,1.75423096144644,
-7.03445827945573));
#131331=CARTESIAN_POINT('Ctrl Pts',(-2.5915230321622,1.74998153250533,-7.00745224865434));
#131332=CARTESIAN_POINT('Ctrl Pts',(-2.58182940328121,1.7456671706653,-6.98045157812462));
#131333=CARTESIAN_POINT('Ctrl Pts',(-2.57210657331054,1.74127713117846,
-6.95347381572797));
#131334=CARTESIAN_POINT('Ctrl Pts',(-2.56283493129394,1.73709081148723,
-6.92774795647658));
#131335=CARTESIAN_POINT('Ctrl Pts',(-2.55354612883298,1.73283723878164,
-6.90203911658116));
#131336=CARTESIAN_POINT('Ctrl Pts',(-2.54423929792918,1.72851290762179,
-6.87634881754053));
#131337=CARTESIAN_POINT('Ctrl Pts',(-2.53493219541867,1.72418845026245,
-6.85065776876484));
#131338=CARTESIAN_POINT('Ctrl Pts',(-2.52560699518005,1.71979319994618,
-6.82498506952868));
#131339=CARTESIAN_POINT('Ctrl Pts',(-2.51626273693115,1.71532338472195,
-6.79933245534817));
#131340=CARTESIAN_POINT('Ctrl Pts',(-2.366375582,1.714555786,-7.11690007));
#131341=CARTESIAN_POINT('Ctrl Pts',(-2.751628862,1.779135389,-6.988803013));
#131342=CARTESIAN_POINT('Ctrl Pts',(-3.120803103,1.844275173,-6.819867154));
#131343=CARTESIAN_POINT('Ctrl Pts',(-2.511887581,1.714555786,-6.800949991));
#131344=CARTESIAN_POINT('Ctrl Pts',(-2.880037795,1.779135389,-6.664976053));
#131345=CARTESIAN_POINT('Ctrl Pts',(-3.231358619,1.844275173,-6.49005558300001));
#131346=CARTESIAN_POINT('Origin',(0.0927445948128036,1.87498566366618,0.174752221623834));
#131347=CARTESIAN_POINT('Ctrl Pts',(-3.561170189,1.844275173,-6.600611099));
#131348=CARTESIAN_POINT('Ctrl Pts',(-3.82431958,1.796786772,-6.458636401));
#131349=CARTESIAN_POINT('Ctrl Pts',(-4.075331425,1.75,-6.296163417));
#131350=CARTESIAN_POINT('Ctrl Pts',(-4.170121894,1.73233175,-6.23480818400001));
#131351=CARTESIAN_POINT('Ctrl Pts',(-4.26302238,1.714550109,-6.170627212));
#131352=CARTESIAN_POINT('Ctrl Pts',(-3.231358619,1.844275173,-6.490055583));
#131353=CARTESIAN_POINT('Ctrl Pts',(-3.490100446,1.796786772,-6.361229625));
#131354=CARTESIAN_POINT('Ctrl Pts',(-3.737765465,1.75,-6.212214527));
#131355=CARTESIAN_POINT('Ctrl Pts',(-3.831292059,1.73233175,-6.155941442));
#131356=CARTESIAN_POINT('Ctrl Pts',(-3.923082237,1.714550109,-6.096878362));
#131357=CARTESIAN_POINT('',(-3.9190894118075,1.715323387189,-6.09944572887941));
#131358=CARTESIAN_POINT('Ctrl Pts',(-3.91908940514573,1.71532338929515,
-6.09944573161675));
#131359=CARTESIAN_POINT('Ctrl Pts',(-3.85911533782438,1.72693520762752,
-6.13798099222613));
#131360=CARTESIAN_POINT('Ctrl Pts',(-3.79865934604485,1.7384964446453,-6.17557589414559));
#131361=CARTESIAN_POINT('Ctrl Pts',(-3.73776546454411,1.75000000008612,
-6.2122145272743));
#131362=CARTESIAN_POINT('Ctrl Pts',(-3.6112224337199,1.77390543523616,-6.28835294289181));
#131363=CARTESIAN_POINT('Ctrl Pts',(-3.48191418812186,1.79806022994621,
-6.36088399665844));
#131364=CARTESIAN_POINT('Ctrl Pts',(-3.35016172797745,1.82239960750087,
-6.4295346952108));
#131365=CARTESIAN_POINT('Ctrl Pts',(-3.3107758002692,1.82967559281287,-6.45005705545622));
#131366=CARTESIAN_POINT('Ctrl Pts',(-3.27117169807065,1.83696804640807,
-6.47023289694387));
#131367=CARTESIAN_POINT('Ctrl Pts',(-3.23135861767661,1.8442751738904,-6.49005558383991));
#131368=CARTESIAN_POINT('Ctrl Pts',(-4.05261513068032,1.75423096141826,
-6.31080902862432));
#131369=CARTESIAN_POINT('Ctrl Pts',(-4.03732975837505,1.74998153251284,
-6.28652106195361));
#131370=CARTESIAN_POINT('Ctrl Pts',(-4.02205841514142,1.74566717066447,
-6.26223549580918));
#131371=CARTESIAN_POINT('Ctrl Pts',(-4.00676347813377,1.74127713117592,
-6.23797857957085));
#131372=CARTESIAN_POINT('Ctrl Pts',(-3.99217830271731,1.73709081148113,
-6.21484730559298));
#131373=CARTESIAN_POINT('Ctrl Pts',(-3.97758002674885,1.73283723877757,
-6.19173634204228));
#131374=CARTESIAN_POINT('Ctrl Pts',(-3.96296812961283,1.72851290762974,
-6.16864736146869));
#131375=CARTESIAN_POINT('Ctrl Pts',(-3.9483558060092,1.72418845027056,-6.14555770701255));
#131376=CARTESIAN_POINT('Ctrl Pts',(-3.93372975245047,1.71979319996508,
-6.12248986358579));
#131377=CARTESIAN_POINT('Ctrl Pts',(-3.91908940361339,1.71532338467323,
-6.09944573338996));
#131378=CARTESIAN_POINT('Ctrl Pts',(-3.840974177,1.714555786,-6.4418101));
#131379=CARTESIAN_POINT('Ctrl Pts',(-4.189683368,1.779135389,-6.233889815));
#131380=CARTESIAN_POINT('Ctrl Pts',(-4.513910305,1.844275173,-5.989542033));
#131381=CARTESIAN_POINT('Ctrl Pts',(-3.915164259,1.714555786,-6.101965981));
#131382=CARTESIAN_POINT('Ctrl Pts',(-4.245476948,1.779135389,-5.890029624));
#131383=CARTESIAN_POINT('Ctrl Pts',(-4.550981356,1.844275173,-5.643675106));
#131384=CARTESIAN_POINT('Origin',(0.128142651926348,1.87498565322314,0.150729012321198));
#131385=CARTESIAN_POINT('Ctrl Pts',(-4.896848283,1.844275173,-5.680746157));
#131386=CARTESIAN_POINT('Ctrl Pts',(-5.123325024,1.796786772,-5.485521408));
#131387=CARTESIAN_POINT('Ctrl Pts',(-5.333541463,1.75,-5.272886825));
#131388=CARTESIAN_POINT('Ctrl Pts',(-5.41292622100001,1.73233175,-5.192588894));
#131389=CARTESIAN_POINT('Ctrl Pts',(-5.489857734,1.714550109,-5.109937579));
#131390=CARTESIAN_POINT('Ctrl Pts',(-4.550981356,1.844275173,-5.643675106));
#131391=CARTESIAN_POINT('Ctrl Pts',(-4.77598017,1.796786772,-5.462239182));
#131392=CARTESIAN_POINT('Ctrl Pts',(-4.985821077,1.75,-5.263467316));
#131393=CARTESIAN_POINT('Ctrl Pts',(-5.065064022,1.73233175,-5.188404412));
#131394=CARTESIAN_POINT('Ctrl Pts',(-5.14201138,1.714550109,-5.110990019));
#131395=CARTESIAN_POINT('',(-5.13866381173065,1.71532338696204,-5.11435570193178));
#131396=CARTESIAN_POINT('Ctrl Pts',(-5.13866380664227,1.71532338939167,
-5.11435570540697));
#131397=CARTESIAN_POINT('Ctrl Pts',(-5.08837584222255,1.72693520765757,
-5.16488268446888));
#131398=CARTESIAN_POINT('Ctrl Pts',(-5.03741507052992,1.73849644464497,
-5.21459488956239));
#131399=CARTESIAN_POINT('Ctrl Pts',(-4.98582107705033,1.74999999998741,
-5.26346731617251));
#131400=CARTESIAN_POINT('Ctrl Pts',(-4.8786043022516,1.77390538127784,-5.36502844050722));
#131401=CARTESIAN_POINT('Ctrl Pts',(-4.76791149972737,1.79806012136271,
-5.46366099465171));
#131402=CARTESIAN_POINT('Ctrl Pts',(-4.65399747964481,1.82239944351147,
-5.55902936340484));
#131403=CARTESIAN_POINT('Ctrl Pts',(-4.61994382240916,1.82967548322283,
-5.58753895105952));
#131404=CARTESIAN_POINT('Ctrl Pts',(-4.58560259585709,1.83696799146888,
-5.61575701812922));
#131405=CARTESIAN_POINT('Ctrl Pts',(-4.55098135499805,1.84427517380053,
-5.64367510678222));
#131406=CARTESIAN_POINT('Ctrl Pts',(-5.31450463649893,1.75423096142994,
-5.29207336192635));
#131407=CARTESIAN_POINT('Ctrl Pts',(-5.29435543258047,1.74998153248503,
-5.27163913767342));
#131408=CARTESIAN_POINT('Ctrl Pts',(-5.27422044602439,1.74566717065283,
-5.25120424192191));
#131409=CARTESIAN_POINT('Ctrl Pts',(-5.25406857613305,1.74127713117215,
-5.23080239827337));
#131410=CARTESIAN_POINT('Ctrl Pts',(-5.23485185378547,1.73709081147825,
-5.21134730220106));
#131411=CARTESIAN_POINT('Ctrl Pts',(-5.21562670327365,1.73283723877023,
-5.19191485797558));
#131412=CARTESIAN_POINT('Ctrl Pts',(-5.19639297566802,1.72851290760489,
-5.17250681089194));
#131413=CARTESIAN_POINT('Ctrl Pts',(-5.17715868680678,1.72418845025209,
-5.15309819746591));
#131414=CARTESIAN_POINT('Ctrl Pts',(-5.15791567763788,1.71979319993897,
-5.13371383664131));
#131415=CARTESIAN_POINT('Ctrl Pts',(-5.13866380548064,1.71532338474424,
-5.11435570700624));
#131416=CARTESIAN_POINT('Ctrl Pts',(-5.135973089,1.714555786,-5.46550825));
#131417=CARTESIAN_POINT('Ctrl Pts',(-5.431832937,1.779135389,-5.187486857));
#131418=CARTESIAN_POINT('Ctrl Pts',(-5.695952078,1.844275173,-4.879152583));
#131419=CARTESIAN_POINT('Ctrl Pts',(-5.135372207,1.714555786,-5.117660823));
#131420=CARTESIAN_POINT('Ctrl Pts',(-5.412402317,1.779135389,-4.839671956));
#131421=CARTESIAN_POINT('Ctrl Pts',(-5.657805263,1.844275173,-4.533402653));
#131422=CARTESIAN_POINT('Origin',(0.15754918724798,1.87498566985664,0.119658311091085));
#131423=CARTESIAN_POINT('Ctrl Pts',(-6.003555193,1.844275173,-4.495255837));
#131424=CARTESIAN_POINT('Ctrl Pts',(-6.182769484,1.796786772,-4.25590953));
#131425=CARTESIAN_POINT('Ctrl Pts',(-6.342361029,1.75,-4.003055905));
#131426=CARTESIAN_POINT('Ctrl Pts',(-6.402628134,1.73233175,-3.907569919));
#131427=CARTESIAN_POINT('Ctrl Pts',(-6.45999344200001,1.714550109,-3.810312944));
#131428=CARTESIAN_POINT('Ctrl Pts',(-5.657805263,1.844275173,-4.533402653));
#131429=CARTESIAN_POINT('Ctrl Pts',(-5.838540369,1.796786772,-4.307840506));
#131430=CARTESIAN_POINT('Ctrl Pts',(-6.000745237,1.75,-4.068606224));
#131431=CARTESIAN_POINT('Ctrl Pts',(-6.06199922,1.73233175,-3.978263357));
#131432=CARTESIAN_POINT('Ctrl Pts',(-6.120505785,1.714550109,-3.886117463));
#131433=CARTESIAN_POINT('',(-6.11796000416365,1.71532338699328,-3.89012408614553));
#131434=CARTESIAN_POINT('Ctrl Pts',(-6.11795999984783,1.71532338947478,
-3.89012409082083));
#131435=CARTESIAN_POINT('Ctrl Pts',(-6.07970954685225,1.72693520768515,
-3.95028020283552));
#131436=CARTESIAN_POINT('Ctrl Pts',(-6.04062686434743,1.7384964446451,-4.00978522383035));
#131437=CARTESIAN_POINT('Ctrl Pts',(-6.00074523690707,1.75000000002681,
-4.06860622413707));
#131438=CARTESIAN_POINT('Ctrl Pts',(-5.91786775054758,1.77390538695136,
-4.19084137137646));
#131439=CARTESIAN_POINT('Ctrl Pts',(-5.83096594687763,1.79806013262182,
-4.31096365888321));
#131440=CARTESIAN_POINT('Ctrl Pts',(-5.74021653072587,1.82239946043817,
-4.42859054095511));
#131441=CARTESIAN_POINT('Ctrl Pts',(-5.71308776811837,1.82967549453686,
-4.46375409236191));
#131442=CARTESIAN_POINT('Ctrl Pts',(-5.68561549162366,1.83696799714455,
-4.49869475799346));
#131443=CARTESIAN_POINT('Ctrl Pts',(-5.65780526140172,1.84427517382125,
-4.53340265367153));
#131444=CARTESIAN_POINT('Ctrl Pts',(-6.32789381132842,1.754230961419,-4.02588622636397));
#131445=CARTESIAN_POINT('Ctrl Pts',(-6.3038229304785,1.74998153248991,-4.01026122619341));
#131446=CARTESIAN_POINT('Ctrl Pts',(-6.27976579010753,1.74566717064373,
-3.99463251394121));
#131447=CARTESIAN_POINT('Ctrl Pts',(-6.25569926639605,1.74127713116377,
-3.97903971038985));
#131448=CARTESIAN_POINT('Ctrl Pts',(-6.2327495497864,1.73709081147847,-3.96417049093199));
#131449=CARTESIAN_POINT('Ctrl Pts',(-6.20979647155677,1.73283723878647,
-3.94932520550051));
#131450=CARTESIAN_POINT('Ctrl Pts',(-6.18684026140042,1.72851290763057,
-3.93450559067464));
#131451=CARTESIAN_POINT('Ctrl Pts',(-6.16388338136915,1.7241884502883,-3.91968554340421));
#131452=CARTESIAN_POINT('Ctrl Pts',(-6.14092319847239,1.71979319997889,
-3.90489105636516));
#131453=CARTESIAN_POINT('Ctrl Pts',(-6.11795999885005,1.71532338484833,
-3.89012409187889));
#131454=CARTESIAN_POINT('Ctrl Pts',(-6.190819606,1.714555786,-4.233645309));
#131455=CARTESIAN_POINT('Ctrl Pts',(-6.419996035,1.779135389,-3.898522779));
#131456=CARTESIAN_POINT('Ctrl Pts',(-6.611657462,1.844275173,-3.540619381));
#131457=CARTESIAN_POINT('Ctrl Pts',(-6.115455858,1.714555786,-3.894059533));
#131458=CARTESIAN_POINT('Ctrl Pts',(-6.32624977,1.779135389,-3.563016607));
#131459=CARTESIAN_POINT('Ctrl Pts',(-6.500076484,1.844275173,-3.21115333));
#131460=CARTESIAN_POINT('Origin',(0.179588712885957,1.87498562990572,0.0829923124906845));
#131461=CARTESIAN_POINT('Ctrl Pts',(-6.829542535,1.844275173,-3.099572351));
#131462=CARTESIAN_POINT('Ctrl Pts',(-6.953114514,1.796786772,-2.827296052));
#131463=CARTESIAN_POINT('Ctrl Pts',(-7.054618843,1.75,-2.54604654));
#131464=CARTESIAN_POINT('Ctrl Pts',(-7.092950272,1.73233175,-2.439837317));
#131465=CARTESIAN_POINT('Ctrl Pts',(-7.128067036,1.714550109,-2.332522311));
#131466=CARTESIAN_POINT('Ctrl Pts',(-6.500076484,1.844275173,-3.21115333));
#131467=CARTESIAN_POINT('Ctrl Pts',(-6.62809690900001,1.796786772,-2.952011995));
#131468=CARTESIAN_POINT('Ctrl Pts',(-6.735081219,1.75,-2.683501626));
#131469=CARTESIAN_POINT('Ctrl Pts',(-6.775482072,1.73233175,-2.58210313));
#131470=CARTESIAN_POINT('Ctrl Pts',(-6.812812143,1.714550109,-2.479534373));
#131471=CARTESIAN_POINT('',(-6.81118718672704,1.71532338720686,-2.48399459038574));
#131472=CARTESIAN_POINT('Ctrl Pts',(-6.81118718300311,1.71532338937562,
-2.48399459670162));
#131473=CARTESIAN_POINT('Ctrl Pts',(-6.78676279055767,1.72693520765252,
-2.55096700918865));
#131474=CARTESIAN_POINT('Ctrl Pts',(-6.76138566003139,1.73849644464502,
-2.61748245733183));
#131475=CARTESIAN_POINT('Ctrl Pts',(-6.73508121901305,1.75000000000424,
-2.68350162607721));
#131476=CARTESIAN_POINT('Ctrl Pts',(-6.68041833199122,1.77390537542953,
-2.82069512751682));
#131477=CARTESIAN_POINT('Ctrl Pts',(-6.62137101549202,1.79806010944939,
-2.95669027739262));
#131478=CARTESIAN_POINT('Ctrl Pts',(-6.55802960725091,1.82239942545539,
-3.09107548762239));
#131479=CARTESIAN_POINT('Ctrl Pts',(-6.53909419508274,1.82967547114592,
-3.13124888154695));
#131480=CARTESIAN_POINT('Ctrl Pts',(-6.51977538511073,1.83696798539964,
-3.17127844552307));
#131481=CARTESIAN_POINT('Ctrl Pts',(-6.50007648272107,1.84427517376508,
-3.21115333112861));
#131482=CARTESIAN_POINT('Ctrl Pts',(-7.04539770492697,1.75423096145248,
-2.57145312545857));
#131483=CARTESIAN_POINT('Ctrl Pts',(-7.01853067466854,1.7499815325047,-2.56136795692046));
#131484=CARTESIAN_POINT('Ctrl Pts',(-6.99167626573207,1.74566717065564,
-2.55127620925494));
#131485=CARTESIAN_POINT('Ctrl Pts',(-6.96482041212451,1.7412771311639,-2.5412215479421));
#131486=CARTESIAN_POINT('Ctrl Pts',(-6.93921080451857,1.73709081147356,
-2.53163347323051));
#131487=CARTESIAN_POINT('Ctrl Pts',(-6.91360305898445,1.73283723877157,
-2.52206949564413));
#131488=CARTESIAN_POINT('Ctrl Pts',(-6.88799777319566,1.72851290761252,
-2.5125312617467));
#131489=CARTESIAN_POINT('Ctrl Pts',(-6.86239174019579,1.72418845026124,
-2.5029927495054));
#131490=CARTESIAN_POINT('Ctrl Pts',(-6.83678797627367,1.71979319995007,
-2.49347990990502));
#131491=CARTESIAN_POINT('Ctrl Pts',(-6.81118718266381,1.71532338473148,
-2.48399459871635));
#131492=CARTESIAN_POINT('Ctrl Pts',(-6.95619028,1.714555786,-2.803821818));
#131493=CARTESIAN_POINT('Ctrl Pts',(-7.107967253,1.779135389,-2.42726811));
#131494=CARTESIAN_POINT('Ctrl Pts',(-7.218209092,1.844275173,-2.036530753));
#131495=CARTESIAN_POINT('Ctrl Pts',(-6.809587591,1.714555786,-2.488376347));
#131496=CARTESIAN_POINT('Ctrl Pts',(-6.944288814,1.779135389,-2.119758561));
#131497=CARTESIAN_POINT('Ctrl Pts',(-7.038411352,1.844275173,-1.738754046));
#131498=CARTESIAN_POINT('Origin',(0.193230873444549,1.874985638441,0.0424457232433673));
#131499=CARTESIAN_POINT('Ctrl Pts',(-7.336188059,1.844275173,-1.558956307));
#131500=CARTESIAN_POINT('Ctrl Pts',(-7.39833963800001,1.796786772,-1.266481354));
#131501=CARTESIAN_POINT('Ctrl Pts',(-7.43701052,1.75,-0.969986869));
#131502=CARTESIAN_POINT('Ctrl Pts',(-7.451613939,1.73233175,-0.858020634));
#131503=CARTESIAN_POINT('Ctrl Pts',(-7.462840138,1.714550109,-0.745665527));
#131504=CARTESIAN_POINT('Ctrl Pts',(-7.038411352,1.844275173,-1.738754046));
#131505=CARTESIAN_POINT('Ctrl Pts',(-7.107731005,1.796786772,-1.458150685));
#131506=CARTESIAN_POINT('Ctrl Pts',(-7.154492288,1.75,-1.172919475));
#131507=CARTESIAN_POINT('Ctrl Pts',(-7.172150913,1.73233175,-1.06520663));
#131508=CARTESIAN_POINT('Ctrl Pts',(-7.186558977,1.714550109,-0.957011012));
#131509=CARTESIAN_POINT('',(-7.18593082598847,1.71532338697828,-0.961716270654875));
#131510=CARTESIAN_POINT('Ctrl Pts',(-7.18593082403205,1.71532338941653,
-0.961716276704436));
#131511=CARTESIAN_POINT('Ctrl Pts',(-7.1764745489304,1.72693520766661,-1.03237343373525));
#131512=CARTESIAN_POINT('Ctrl Pts',(-7.16598957642124,1.73849644464473,
-1.1027891205401));
#131513=CARTESIAN_POINT('Ctrl Pts',(-7.15449228845151,1.74999999991563,
-1.17291947499682));
#131514=CARTESIAN_POINT('Ctrl Pts',(-7.13059994450386,1.77390536878919,
-1.31865633427296));
#131515=CARTESIAN_POINT('Ctrl Pts',(-7.10216806696628,1.79806009648014,
-1.46416538209603));
#131516=CARTESIAN_POINT('Ctrl Pts',(-7.06919640414973,1.82239940603252,
-1.6090252331022));
#131517=CARTESIAN_POINT('Ctrl Pts',(-7.05933977535074,1.82967545822364,
-1.6523299880728));
#131518=CARTESIAN_POINT('Ctrl Pts',(-7.04907779246522,1.83696797900477,
-1.69557669487067));
#131519=CARTESIAN_POINT('Ctrl Pts',(-7.03841135156546,1.8442751739085,-1.7387540481104));
#131520=CARTESIAN_POINT('Ctrl Pts',(-7.43346663201529,1.75423096142758,
-0.996781734613964));
#131521=CARTESIAN_POINT('Ctrl Pts',(-7.40505972491879,1.7499815325007,-0.992707968931453));
#131522=CARTESIAN_POINT('Ctrl Pts',(-7.37666372970027,1.74566717065144,
-0.988625064820829));
#131523=CARTESIAN_POINT('Ctrl Pts',(-7.34827429605648,1.74127713115956,
-0.984578690565064));
#131524=CARTESIAN_POINT('Ctrl Pts',(-7.32120227423994,1.73709081147489,
-0.980720088329301));
#131525=CARTESIAN_POINT('Ctrl Pts',(-7.29413725113095,1.73283723877859,
-0.976884619551812));
#131526=CARTESIAN_POINT('Ctrl Pts',(-7.26708016439697,1.72851290762386,
-0.973073763836603));
#131527=CARTESIAN_POINT('Ctrl Pts',(-7.24002228807107,1.72418845027458,
-0.96926279691131));
#131528=CARTESIAN_POINT('Ctrl Pts',(-7.21297214663693,1.71979319996398,
-0.965476414649176));
#131529=CARTESIAN_POINT('Ctrl Pts',(-7.18593082378778,1.71532338478122,
-0.961716278323274));
#131530=CARTESIAN_POINT('Ctrl Pts',(-7.39629722700001,1.714555786,-1.242894736));
#131531=CARTESIAN_POINT('Ctrl Pts',(-7.463577823,1.779135389,-0.842517081));
#131532=CARTESIAN_POINT('Ctrl Pts',(-7.48724528700001,1.844275173,-0.437216209));
#131533=CARTESIAN_POINT('Ctrl Pts',(-7.185310576,1.714555786,-0.966339449));
#131534=CARTESIAN_POINT('Ctrl Pts',(-7.237620632,1.779135389,-0.57738296));
#131535=CARTESIAN_POINT('Ctrl Pts',(-7.24763792900001,1.844275173,-0.185052556));
#131536=CARTESIAN_POINT('Origin',(0.197838004389101,1.87498562398033,-8.55452297409201E-5));
#131537=CARTESIAN_POINT('Ctrl Pts',(-7.499801582,1.844275173,0.054554802));
#131538=CARTESIAN_POINT('Ctrl Pts',(-7.497626623,1.796786772,0.353552605));
#131539=CARTESIAN_POINT('Ctrl Pts',(-7.471655851,1.75,0.651428311));
#131540=CARTESIAN_POINT('Ctrl Pts',(-7.461848419,1.73233175,0.76391614));
#131541=CARTESIAN_POINT('Ctrl Pts',(-7.448659129,1.714550109,0.876057748));
#131542=CARTESIAN_POINT('Ctrl Pts',(-7.247637929,1.844275173,-0.185052556));
#131543=CARTESIAN_POINT('Ctrl Pts',(-7.255015499,1.796786772,0.103892131));
#131544=CARTESIAN_POINT('Ctrl Pts',(-7.23936725,1.75,0.392507087));
#131545=CARTESIAN_POINT('Ctrl Pts',(-7.233457948,1.73233175,0.501497748));
#131546=CARTESIAN_POINT('Ctrl Pts',(-7.2242703,1.714550109,0.610261121));
#131547=CARTESIAN_POINT('',(-7.22466832593348,1.71532338696753,0.605530834702192));
#131548=CARTESIAN_POINT('Ctrl Pts',(-7.22466832530966,1.71532338955417,
0.605530828374252));
#131549=CARTESIAN_POINT('Ctrl Pts',(-7.23062233283012,1.72693520771164,
0.534492776723643));
#131550=CARTESIAN_POINT('Ctrl Pts',(-7.23551978458698,1.73849644464494,
0.463469410197625));
#131551=CARTESIAN_POINT('Ctrl Pts',(-7.23936725010701,1.74999999995834,
0.392507087148465));
#131552=CARTESIAN_POINT('Ctrl Pts',(-7.24736260576629,1.77390535047713,
0.245041440907815));
#131553=CARTESIAN_POINT('Ctrl Pts',(-7.25087559512114,1.79806005925618,
0.0968224154203942));
#131554=CARTESIAN_POINT('Ctrl Pts',(-7.24981538563083,1.82239934968363,
-0.0517385105763896));
#131555=CARTESIAN_POINT('Ctrl Pts',(-7.24949844297524,1.82967542051086,
-0.0961498225221249));
#131556=CARTESIAN_POINT('Ctrl Pts',(-7.24877314242756,1.8369679600195,-0.140591582761845));
#131557=CARTESIAN_POINT('Ctrl Pts',(-7.24763792873457,1.8442751737337,-0.185052557496855));
#131558=CARTESIAN_POINT('Ctrl Pts',(-7.47395492118855,1.75423096142584,
0.624498063269636));
#131559=CARTESIAN_POINT('Ctrl Pts',(-7.44533641265144,1.74998153250237,
0.622369941210248));
#131560=CARTESIAN_POINT('Ctrl Pts',(-7.41672659636858,1.74566717064329,
0.620253089576169));
#131561=CARTESIAN_POINT('Ctrl Pts',(-7.38813104109155,1.7412771311558,0.618101972734666));
#131562=CARTESIAN_POINT('Ctrl Pts',(-7.3608624625947,1.73709081145649,0.616050678473018));
#131563=CARTESIAN_POINT('Ctrl Pts',(-7.33360569219016,1.73283723875479,
0.61397829614577));
#131564=CARTESIAN_POINT('Ctrl Pts',(-7.30636196376475,1.72851290761384,
0.611883582297337));
#131565=CARTESIAN_POINT('Ctrl Pts',(-7.27911744015338,1.72418845025495,
0.609788807308702));
#131566=CARTESIAN_POINT('Ctrl Pts',(-7.25188575564588,1.71979319995443,
0.607671685225234));
#131567=CARTESIAN_POINT('Ctrl Pts',(-7.22466832570712,1.71532338479073,
0.605530826510677));
#131568=CARTESIAN_POINT('Ctrl Pts',(-7.490561537,1.714555786,0.376148724));
#131569=CARTESIAN_POINT('Ctrl Pts',(-7.470199788,1.779135389,0.781629111));
#131570=CARTESIAN_POINT('Ctrl Pts',(-7.406186214,1.844275173,1.182542078));
#131571=CARTESIAN_POINT('Ctrl Pts',(-7.225056424,1.714555786,0.600882408));
#131572=CARTESIAN_POINT('Ctrl Pts',(-7.192529353,1.779135389,0.991990426));
#131573=CARTESIAN_POINT('Ctrl Pts',(-7.117973011,1.844275173,1.377301786));
#131574=CARTESIAN_POINT('Origin',(0.193194100687983,1.87498565212922,-0.0426128425397729));
#131575=CARTESIAN_POINT('Ctrl Pts',(-7.312732719,1.844275173,1.665514988));
#131576=CARTESIAN_POINT('Ctrl Pts',(-7.24633292000001,1.796786772,1.957054837));
#131577=CARTESIAN_POINT('Ctrl Pts',(-7.156934859,1.75,2.242383426));
#131578=CARTESIAN_POINT('Ctrl Pts',(-7.123175161,1.73233175,2.350133045));
#131579=CARTESIAN_POINT('Ctrl Pts',(-7.086187098,1.714550109,2.456817537));
#131580=CARTESIAN_POINT('Ctrl Pts',(-7.117973011,1.844275173,1.377301786));
#131581=CARTESIAN_POINT('Ctrl Pts',(-7.063063531,1.796786772,1.661077066));
#131582=CARTESIAN_POINT('Ctrl Pts',(-6.985737446,1.75,1.939580454));
#131583=CARTESIAN_POINT('Ctrl Pts',(-6.95653653,1.73233175,2.044752649));
#131584=CARTESIAN_POINT('Ctrl Pts',(-6.924182773,1.714550109,2.148998121));
#131585=CARTESIAN_POINT('',(-6.92558836542192,1.71532338722248,2.14446399150146));
#131586=CARTESIAN_POINT('Ctrl Pts',(-6.92558836637386,1.71532338940864,
2.14446398387456));
#131587=CARTESIAN_POINT('Ctrl Pts',(-6.94667425374691,1.72693520766414,
2.07636669827668));
#131588=CARTESIAN_POINT('Ctrl Pts',(-6.96672513021646,1.73849644464487,
2.00805662611619));
#131589=CARTESIAN_POINT('Ctrl Pts',(-6.98573744593035,1.74999999995786,
1.93958045425087));
#131590=CARTESIAN_POINT('Ctrl Pts',(-7.02524659969686,1.77390533277599,
1.79728134347411));
#131591=CARTESIAN_POINT('Ctrl Pts',(-7.06054014363285,1.7980600235061,1.65328289302275));
#131592=CARTESIAN_POINT('Ctrl Pts',(-7.09144091274129,1.8223992956843,1.50796743465552));
#131593=CARTESIAN_POINT('Ctrl Pts',(-7.10067852414962,1.82967538443001,
1.46452619436445));
#131594=CARTESIAN_POINT('Ctrl Pts',(-7.1095238684046,1.83696794194513,1.42096743216677));
#131595=CARTESIAN_POINT('Ctrl Pts',(-7.11797301163307,1.84427517374057,
1.37730178497811));
#131596=CARTESIAN_POINT('Ctrl Pts',(-7.16496938531472,1.75423096140909,
2.21657702477027));
#131597=CARTESIAN_POINT('Ctrl Pts',(-7.1374774448394,1.74998153246282,2.20834652356057));
#131598=CARTESIAN_POINT('Ctrl Pts',(-7.10999157065123,1.74566717061902,
2.20012889801882));
#131599=CARTESIAN_POINT('Ctrl Pts',(-7.08252699007765,1.74127713114131,
2.1918808740247));
#131600=CARTESIAN_POINT('Ctrl Pts',(-7.0563369033927,1.7370908114499,2.18401559959216));
#131601=CARTESIAN_POINT('Ctrl Pts',(-7.03016288205566,1.73283723875281,
2.17613226848579));
#131602=CARTESIAN_POINT('Ctrl Pts',(-7.00400639833485,1.72851290760386,
2.16822993156721));
#131603=CARTESIAN_POINT('Ctrl Pts',(-6.97784915130021,1.72418845025975,
2.16032736403801));
#131604=CARTESIAN_POINT('Ctrl Pts',(-6.95170924709586,1.71979319996095,
2.15240573186988));
#131605=CARTESIAN_POINT('Ctrl Pts',(-6.92558836665804,1.71532338478933,
2.14446398239877));
#131606=CARTESIAN_POINT('Ctrl Pts',(-7.234575514,1.714555786,1.977603887));
#131607=CARTESIAN_POINT('Ctrl Pts',(-7.127523515,1.779135389,2.369227193));
#131608=CARTESIAN_POINT('Ctrl Pts',(-6.978822105,1.844275173,2.747006012));
#131609=CARTESIAN_POINT('Ctrl Pts',(-6.926966664,1.714555786,2.140007671));
#131610=CARTESIAN_POINT('Ctrl Pts',(-6.811123395,1.779135389,2.514979442));
#131611=CARTESIAN_POINT('Ctrl Pts',(-6.655479587,1.844275173,2.875255027));
#131612=CARTESIAN_POINT('Origin',(0.179516811567976,1.87498563076573,-0.0831475948476074));
#131613=CARTESIAN_POINT('Ctrl Pts',(-6.783728602,1.844275173,3.198597545));
#131614=CARTESIAN_POINT('Ctrl Pts',(-6.656208743,1.796786772,3.46904736));
#131615=CARTESIAN_POINT('Ctrl Pts',(-6.507563547,1.75,3.728487185));
#131616=CARTESIAN_POINT('Ctrl Pts',(-6.451430149,1.73233175,3.82646034));
#131617=CARTESIAN_POINT('Ctrl Pts',(-6.392372834,1.714550109,3.922699268));
#131618=CARTESIAN_POINT('Ctrl Pts',(-6.655479587,1.844275173,2.875255027));
#131619=CARTESIAN_POINT('Ctrl Pts',(-6.540850562,1.796786772,3.140591884));
#131620=CARTESIAN_POINT('Ctrl Pts',(-6.405462322,1.75,3.395961195));
#131621=CARTESIAN_POINT('Ctrl Pts',(-6.354335194,1.73233175,3.492397189));
#131622=CARTESIAN_POINT('Ctrl Pts',(-6.300328155,1.714550109,3.587250358));
#131623=CARTESIAN_POINT('',(-6.30267559026525,1.71532338700246,3.58312439402828));
#131624=CARTESIAN_POINT('Ctrl Pts',(-6.30267559237097,1.71532338942935,
3.58312438803456));
#131625=CARTESIAN_POINT('Ctrl Pts',(-6.3379074070704,1.72693520767085,3.52115202098277));
#131626=CARTESIAN_POINT('Ctrl Pts',(-6.37217415129364,1.73849644464501,
3.45874934597489));
#131627=CARTESIAN_POINT('Ctrl Pts',(-6.40546232218141,1.75000000000019,
3.39596119494342));
#131628=CARTESIAN_POINT('Ctrl Pts',(-6.47463803525355,1.77390538761063,
3.26548195919798));
#131629=CARTESIAN_POINT('Ctrl Pts',(-6.54006198665916,1.7980601341064,3.13243687131316));
#131630=CARTESIAN_POINT('Ctrl Pts',(-6.60147896312938,1.82239946276566,
2.9971612401855));
#131631=CARTESIAN_POINT('Ctrl Pts',(-6.61983904091199,1.8296754960881,2.95672175175188));
#131632=CARTESIAN_POINT('Ctrl Pts',(-6.63784129172376,1.83696799791638,
2.91608316627399));
#131633=CARTESIAN_POINT('Ctrl Pts',(-6.65547958721565,1.84427517380786,
2.87525502605794));
#131634=CARTESIAN_POINT('Ctrl Pts',(-6.52095784396122,1.75423096140536,
3.70501130873352));
#131635=CARTESIAN_POINT('Ctrl Pts',(-6.4958779642362,1.7499815324682,3.69106327754831));
#131636=CARTESIAN_POINT('Ctrl Pts',(-6.47080124111415,1.74566717063294,
3.67712912506784));
#131637=CARTESIAN_POINT('Ctrl Pts',(-6.44575184852816,1.74127713116918,
3.66316986236279));
#131638=CARTESIAN_POINT('Ctrl Pts',(-6.4218648730107,1.73709081148772,3.64985837924667));
#131639=CARTESIAN_POINT('Ctrl Pts',(-6.39799746888694,1.73283723880349,
3.63653271520437));
#131640=CARTESIAN_POINT('Ctrl Pts',(-6.37415127804237,1.72851290766362,
3.62319225975418));
#131641=CARTESIAN_POINT('Ctrl Pts',(-6.35030439132123,1.72418845033167,
3.60985141500447));
#131642=CARTESIAN_POINT('Ctrl Pts',(-6.32647854029341,1.71979320004113,
3.59649567952216));
#131643=CARTESIAN_POINT('Ctrl Pts',(-6.30267559296041,1.7153233848871,3.58312438664675));
#131644=CARTESIAN_POINT('Ctrl Pts',(-6.640308781,1.714555786,3.48658849));
#131645=CARTESIAN_POINT('Ctrl Pts',(-6.451572163,1.779135389,3.846042846));
#131646=CARTESIAN_POINT('Ctrl Pts',(-6.225136031,1.844275173,4.183022998));
#131647=CARTESIAN_POINT('Ctrl Pts',(-6.304979642,1.714555786,3.579068554));
#131648=CARTESIAN_POINT('Ctrl Pts',(-6.111236877,1.779135389,3.920370815));
#131649=CARTESIAN_POINT('Ctrl Pts',(-5.881783334,1.844275173,4.238764539));
#131650=CARTESIAN_POINT('Origin',(0.157445675832952,1.87498564300627,-0.11979455520069));
#131651=CARTESIAN_POINT('Ctrl Pts',(-5.937524875,1.844275173,4.582117236));
#131652=CARTESIAN_POINT('Ctrl Pts',(-5.75484764300001,1.796786772,4.818831084));
#131653=CARTESIAN_POINT('Ctrl Pts',(-5.553905796,1.75,5.040251027));
#131654=CARTESIAN_POINT('Ctrl Pts',(-5.478023433,1.73233175,5.123866603));
#131655=CARTESIAN_POINT('Ctrl Pts',(-5.399658321,1.714550109,5.20515994100001));
#131656=CARTESIAN_POINT('Ctrl Pts',(-5.881783334,1.844275173,4.238764539));
#131657=CARTESIAN_POINT('Ctrl Pts',(-5.712794691,1.796786772,4.473256116));
#131658=CARTESIAN_POINT('Ctrl Pts',(-5.5256749,1.75,4.693550565));
#131659=CARTESIAN_POINT('Ctrl Pts',(-5.455012208,1.73233175,4.776741117));
#131660=CARTESIAN_POINT('Ctrl Pts',(-5.38187719599999,1.714550109,4.857766756));
#131661=CARTESIAN_POINT('',(-5.3850567085804,1.7153233869507,4.85424188252398));
#131662=CARTESIAN_POINT('Ctrl Pts',(-5.38505671164049,1.71532338934533,
4.85424187730532));
#131663=CARTESIAN_POINT('Ctrl Pts',(-5.43278705369071,1.72693520764284,
4.80129218921946));
#131664=CARTESIAN_POINT('Ctrl Pts',(-5.47966739144009,1.73849644464498,
4.74771479141373));
#131665=CARTESIAN_POINT('Ctrl Pts',(-5.52567489996523,1.74999999999131,
4.69355056504093));
#131666=CARTESIAN_POINT('Ctrl Pts',(-5.62128238601438,1.77390535875058,
4.58099273040823));
#131667=CARTESIAN_POINT('Ctrl Pts',(-5.713777415179,1.7980600758039,4.46512252189255));
#131668=CARTESIAN_POINT('Ctrl Pts',(-5.80283865954232,1.82239937461986,
4.34621254500967));
#131669=CARTESIAN_POINT('Ctrl Pts',(-5.82946289357073,1.82967543720348,
4.31066524185358));
#131670=CARTESIAN_POINT('Ctrl Pts',(-5.85578046393677,1.83696796843011,
4.27484657200368));
#131671=CARTESIAN_POINT('Ctrl Pts',(-5.88178333413084,1.84427517383409,
4.23876453736655));
#131672=CARTESIAN_POINT('Ctrl Pts',(-5.57203356106891,1.75423096144802,
5.02020338136438));
#131673=CARTESIAN_POINT('Ctrl Pts',(-5.55053844964282,1.74998153248361,
5.00119001457047));
#131674=CARTESIAN_POINT('Ctrl Pts',(-5.52904343725145,1.74566717064368,
4.98219088070449));
#131675=CARTESIAN_POINT('Ctrl Pts',(-5.50758051440559,1.74127713116268,
4.96317309889159));
#131676=CARTESIAN_POINT('Ctrl Pts',(-5.48711357848799,1.73709081146249,
4.94503783723804));
#131677=CARTESIAN_POINT('Ctrl Pts',(-5.46666880488506,1.73283723875101,
4.92689293344726));
#131678=CARTESIAN_POINT('Ctrl Pts',(-5.44624792837025,1.72851290759493,
4.90873814434882));
#131679=CARTESIAN_POINT('Ctrl Pts',(-5.4258264558248,1.72418845022322,4.89058282536075));
#131680=CARTESIAN_POINT('Ctrl Pts',(-5.40542872828474,1.71979319990471,
4.87241748589314));
#131681=CARTESIAN_POINT('Ctrl Pts',(-5.38505671417874,1.71532338465106,
4.85424187602781));
#131682=CARTESIAN_POINT('Ctrl Pts',(-5.735548589,1.714555786,4.83254409));
#131683=CARTESIAN_POINT('Ctrl Pts',(-5.473952467,1.779135389,5.143021809));
#131684=CARTESIAN_POINT('Ctrl Pts',(-5.180369514,1.844275173,5.423446478));
#131685=CARTESIAN_POINT('Ctrl Pts',(-5.388178779,1.714555786,4.85077617));
#131686=CARTESIAN_POINT('Ctrl Pts',(-5.125595715,1.779135389,5.142450006));
#131687=CARTESIAN_POINT('Ctrl Pts',(-4.833061429,1.844275173,5.404074132));
#131688=CARTESIAN_POINT('Origin',(0.128012269137338,1.87498564545476,-0.150839850589362));
#131689=CARTESIAN_POINT('Ctrl Pts',(-4.813689083,1.844275173,5.751382217));
#131690=CARTESIAN_POINT('Ctrl Pts',(-4.584396264,1.796786772,5.943291623));
#131691=CARTESIAN_POINT('Ctrl Pts',(-4.340553583,1.75,6.116338332));
#131692=CARTESIAN_POINT('Ctrl Pts',(-4.24847043,1.73233175,6.181686558));
#131693=CARTESIAN_POINT('Ctrl Pts',(-4.154461786,1.714550109,6.244233121));
#131694=CARTESIAN_POINT('Ctrl Pts',(-4.833061429,1.844275173,5.404074132));
#131695=CARTESIAN_POINT('Ctrl Pts',(-4.61761489,1.796786772,5.596755863));
#131696=CARTESIAN_POINT('Ctrl Pts',(-4.38751306,1.75,5.771674726));
#131697=CARTESIAN_POINT('Ctrl Pts',(-4.300618913,1.73233175,5.83772994));
#131698=CARTESIAN_POINT('Ctrl Pts',(-4.21177564,1.714550109,5.901139378));
#131699=CARTESIAN_POINT('',(-4.21563856057858,1.71532338724087,5.89838041754561));
#131700=CARTESIAN_POINT('Ctrl Pts',(-4.21563856641281,1.71532338948522,
5.89838041212843));
#131701=CARTESIAN_POINT('Ctrl Pts',(-4.27363561602965,1.72693520768896,
5.85692927020594));
#131702=CARTESIAN_POINT('Ctrl Pts',(-4.33093747372644,1.73849644464486,
5.81468236861823));
#131703=CARTESIAN_POINT('Ctrl Pts',(-4.38751305996885,1.7499999999554,5.77167472619238));
#131704=CARTESIAN_POINT('Ctrl Pts',(-4.50508187020585,1.77390535177738,
5.68230124087691));
#131705=CARTESIAN_POINT('Ctrl Pts',(-4.62032305475982,1.79806006190976,
5.58902373835267));
#131706=CARTESIAN_POINT('Ctrl Pts',(-4.73286419640703,1.82239935371937,
5.4920393752814));
#131707=CARTESIAN_POINT('Ctrl Pts',(-4.76650762263189,1.8296754232205,5.46304654460459));
#131708=CARTESIAN_POINT('Ctrl Pts',(-4.79990989018178,1.83696796139774,
5.43372276736845));
#131709=CARTESIAN_POINT('Ctrl Pts',(-4.83306143023905,1.8442751737759,5.40407413082299));
#131710=CARTESIAN_POINT('Ctrl Pts',(-4.36256718214353,1.75423096135179,
6.10065632342319));
#131711=CARTESIAN_POINT('Ctrl Pts',(-4.34566192601552,1.74998153244077,
6.07746666510283));
#131712=CARTESIAN_POINT('Ctrl Pts',(-4.32875370718173,1.74566717061137,
6.05429092807392));
#131713=CARTESIAN_POINT('Ctrl Pts',(-4.31188083645815,1.74127713113457,
6.03110387735127));
#131714=CARTESIAN_POINT('Ctrl Pts',(-4.29579095138311,1.73709081146119,
6.00899282183094));
#131715=CARTESIAN_POINT('Ctrl Pts',(-4.27972478328063,1.73283723877417,
5.98687711382543));
#131716=CARTESIAN_POINT('Ctrl Pts',(-4.26368407855432,1.72851290761985,
5.96475688867575));
#131717=CARTESIAN_POINT('Ctrl Pts',(-4.24764290579709,1.72418845029148,
5.94263601810869));
#131718=CARTESIAN_POINT('Ctrl Pts',(-4.23162707695028,1.71979319999226,
5.92051046568219));
#131719=CARTESIAN_POINT('Ctrl Pts',(-4.21563856675955,1.71532338489521,
5.89838041096121));
#131720=CARTESIAN_POINT('Ctrl Pts',(-4.56260052,1.714555786,5.9525353));
#131721=CARTESIAN_POINT('Ctrl Pts',(-4.240376838,1.779135389,6.199518789));
#131722=CARTESIAN_POINT('Ctrl Pts',(-3.893374677,1.844275173,6.410275628));
#131723=CARTESIAN_POINT('Ctrl Pts',(-4.219432665,1.714555786,5.895666882));
#131724=CARTESIAN_POINT('Ctrl Pts',(-3.900287394,1.779135389,6.124073949));
#131725=CARTESIAN_POINT('Ctrl Pts',(-3.558350943,1.844275173,6.316695225));
#131726=CARTESIAN_POINT('Origin',(0.0925933313251481,1.87498563513127,-0.174832223587613));
#131727=CARTESIAN_POINT('Ctrl Pts',(-3.46477054,1.844275173,6.651718958));
#131728=CARTESIAN_POINT('Ctrl Pts',(-3.19958361,1.796786772,6.78985045));
#131729=CARTESIAN_POINT('Ctrl Pts',(-2.924241908,1.75,6.906432456));
#131730=CARTESIAN_POINT('Ctrl Pts',(-2.820263672,1.73233175,6.95045772));
#131731=CARTESIAN_POINT('Ctrl Pts',(-2.715007236,1.714550109,6.991332899));
#131732=CARTESIAN_POINT('Ctrl Pts',(-3.558350943,1.844275173,6.316695225));
#131733=CARTESIAN_POINT('Ctrl Pts',(-3.306520548,1.796786772,6.45855752700001));
#131734=CARTESIAN_POINT('Ctrl Pts',(-3.044195986,1.75,6.579921793));
#131735=CARTESIAN_POINT('Ctrl Pts',(-2.945133458,1.73233175,6.62575299900001));
#131736=CARTESIAN_POINT('Ctrl Pts',(-2.844736136,1.714550109,6.668581282));
#131737=CARTESIAN_POINT('',(-2.84910183972128,1.7153233869967,6.66671723749229));
#131738=CARTESIAN_POINT('Ctrl Pts',(-2.849101845019,1.71532338948331,6.66671723400881));
#131739=CARTESIAN_POINT('Ctrl Pts',(-2.91465372686627,1.72693520768767,
6.63870284816572));
#131740=CARTESIAN_POINT('Ctrl Pts',(-2.97969773415148,1.73849644464538,
6.60976186158683));
#131741=CARTESIAN_POINT('Ctrl Pts',(-3.04419598661781,1.75000000011019,
6.57992179271417));
#131742=CARTESIAN_POINT('Ctrl Pts',(-3.17822933764657,1.77390545484905,
6.51791136105184));
#131743=CARTESIAN_POINT('Ctrl Pts',(-3.3108287147856,1.79806026946321,6.45158778029257));
#131744=CARTESIAN_POINT('Ctrl Pts',(-3.44158802289031,1.82239966718631,
6.38106353848644));
#131745=CARTESIAN_POINT('Ctrl Pts',(-3.48067692002918,1.82967563268207,
6.35998117828039));
#131746=CARTESIAN_POINT('Ctrl Pts',(-3.51960144497907,1.83696806636762,
6.3385237776968));
#131747=CARTESIAN_POINT('Ctrl Pts',(-3.5583509445948,1.84427517386462,6.31669522442253));
#131748=CARTESIAN_POINT('Ctrl Pts',(-2.94911201020307,1.75423096146604,
6.89584935662685));
#131749=CARTESIAN_POINT('Ctrl Pts',(-2.93758708077107,1.74998153251673,
6.86956772922766));
#131750=CARTESIAN_POINT('Ctrl Pts',(-2.92605626518683,1.7456671706699,6.8432990608362));
#131751=CARTESIAN_POINT('Ctrl Pts',(-2.91456240336107,1.74127713118637,
6.81702694207591));
#131752=CARTESIAN_POINT('Ctrl Pts',(-2.90360191419132,1.7370908114843,6.79197398098211));
#131753=CARTESIAN_POINT('Ctrl Pts',(-2.89266558762335,1.7328372387758,6.76692157463651));
#131754=CARTESIAN_POINT('Ctrl Pts',(-2.88175510013895,1.72851290761327,
6.74187023065704));
#131755=CARTESIAN_POINT('Ctrl Pts',(-2.87084429429732,1.72418845027103,
6.71681815570412));
#131756=CARTESIAN_POINT('Ctrl Pts',(-2.85995924627466,1.71979319997136,
6.69176695657303));
#131757=CARTESIAN_POINT('Ctrl Pts',(-2.8491018461973,1.7153233848865,6.6667172331805));
#131758=CARTESIAN_POINT('Ctrl Pts',(-3.176310322,1.714555786,6.794192575));
#131759=CARTESIAN_POINT('Ctrl Pts',(-2.808525901,1.779135389,6.96613316));
#131760=CARTESIAN_POINT('Ctrl Pts',(-2.424329967,1.844275173,7.097367414));
#131761=CARTESIAN_POINT('Ctrl Pts',(-2.853390569,1.714555786,6.664882764));
#131762=CARTESIAN_POINT('Ctrl Pts',(-2.492605969,1.779135389,6.819343002));
#131763=CARTESIAN_POINT('Ctrl Pts',(-2.117255923,1.844275173,6.933954669));
#131764=CARTESIAN_POINT('Origin',(0.0528448728486269,1.87498564167741,-0.190649775606609));
#131765=CARTESIAN_POINT('Ctrl Pts',(-1.953843178,1.844275173,7.241028714));
#131766=CARTESIAN_POINT('Ctrl Pts',(-1.665161983,1.796786772,7.318923417));
#131767=CARTESIAN_POINT('Ctrl Pts',(-1.371195932,1.75,7.373589473));
#131768=CARTESIAN_POINT('Ctrl Pts',(-1.260184519,1.73233175,7.39423320399999));
#131769=CARTESIAN_POINT('Ctrl Pts',(-1.148601964,1.714550109,7.411525722));
#131770=CARTESIAN_POINT('Ctrl Pts',(-2.117255923,1.844275173,6.933954669));
#131771=CARTESIAN_POINT('Ctrl Pts',(-1.84081698,1.796786772,7.018364219));
#131772=CARTESIAN_POINT('Ctrl Pts',(-1.558535692,1.75,7.080499029));
#131773=CARTESIAN_POINT('Ctrl Pts',(-1.451936835,1.73233175,7.103963212));
#131774=CARTESIAN_POINT('Ctrl Pts',(-1.344679932,1.714550109,7.124207737));
#131775=CARTESIAN_POINT('',(-1.34934428253352,1.71532338697916,7.12332576961706));
#131776=CARTESIAN_POINT('Ctrl Pts',(-1.34934428819312,1.715323389353,7.12332576731145));
#131777=CARTESIAN_POINT('Ctrl Pts',(-1.41938586838029,1.72693520764564,
7.11005805973543));
#131778=CARTESIAN_POINT('Ctrl Pts',(-1.48913063995742,1.73849644464481,
7.09577623625125));
#131779=CARTESIAN_POINT('Ctrl Pts',(-1.55853569163772,1.74999999993995,
7.08049902907975));
#131780=CARTESIAN_POINT('Ctrl Pts',(-1.70276500374618,1.77390531831854,
7.04875175653017));
#131781=CARTESIAN_POINT('Ctrl Pts',(-1.84652107666297,1.79805999435931,
7.01248396251438));
#131782=CARTESIAN_POINT('Ctrl Pts',(-1.98938313034179,1.82239925163071,
6.97171820711546));
#131783=CARTESIAN_POINT('Ctrl Pts',(-2.0320910514752,1.82967535506913,6.95953148137767));
#131784=CARTESIAN_POINT('Ctrl Pts',(-2.07471906307088,1.83696792734425,
6.94694313302838));
#131785=CARTESIAN_POINT('Ctrl Pts',(-2.11725592454464,1.8442751739537,6.93395466887861));
#131786=CARTESIAN_POINT('Ctrl Pts',(-1.39775963841141,1.75423096140856,
7.36860013775094));
#131787=CARTESIAN_POINT('Ctrl Pts',(-1.39215392831724,1.74998153249677,
7.34045544110522));
#131788=CARTESIAN_POINT('Ctrl Pts',(-1.38653968409113,1.74566717064396,
7.31232213507187));
#131789=CARTESIAN_POINT('Ctrl Pts',(-1.38096227129005,1.74127713116199,
7.28419340331715));
#131790=CARTESIAN_POINT('Ctrl Pts',(-1.3756436783369,1.7370908114676,7.25736998539424));
#131791=CARTESIAN_POINT('Ctrl Pts',(-1.37034856376125,1.73283723876874,
7.23055230350191));
#131792=CARTESIAN_POINT('Ctrl Pts',(-1.36507845578425,1.72851290762297,
7.2037412138722));
#131793=CARTESIAN_POINT('Ctrl Pts',(-1.35980819399523,1.72418845026839,
7.17692934174095));
#131794=CARTESIAN_POINT('Ctrl Pts',(-1.35456289953641,1.71979319996468,
7.15012386222506));
#131795=CARTESIAN_POINT('Ctrl Pts',(-1.34934429048395,1.71532338472446,
7.12332576748435));
#131796=CARTESIAN_POINT('Ctrl Pts',(-1.641499383,1.714555786,7.31816095600001));
#131797=CARTESIAN_POINT('Ctrl Pts',(-1.245351414,1.779135389,7.407018888));
#131798=CARTESIAN_POINT('Ctrl Pts',(-0.841926282,1.844275173,7.452594188));
#131799=CARTESIAN_POINT('Ctrl Pts',(-1.353927101,1.714555786,7.122456136));
#131800=CARTESIAN_POINT('Ctrl Pts',(-0.96837306,1.779135389,7.195747154));
#131801=CARTESIAN_POINT('Ctrl Pts',(-0.577160368,1.844275173,7.2269901));
#131802=CARTESIAN_POINT('Origin',(0.0106252857440335,1.87498562053249,-0.197552244875694));
#131803=CARTESIAN_POINT('Ctrl Pts',(-0.35155628,1.844275173,7.491756015));
#131804=CARTESIAN_POINT('Ctrl Pts',(-0.052879233,1.796786772,7.505771659));
#131805=CARTESIAN_POINT('Ctrl Pts',(0.245965642,1.75,7.495965642));
#131806=CARTESIAN_POINT('Ctrl Pts',(0.358819462,1.73233175,7.492262562));
#131807=CARTESIAN_POINT('Ctrl Pts',(0.471510658,1.714550109,7.485163839));
#131808=CARTESIAN_POINT('Ctrl Pts',(-0.577160368,1.844275173,7.2269901));
#131809=CARTESIAN_POINT('Ctrl Pts',(-0.289038857,1.796786772,7.25000000000001));
#131810=CARTESIAN_POINT('Ctrl Pts',(0.,1.75,7.25));
#131811=CARTESIAN_POINT('Ctrl Pts',(0.10915074,1.73233175,7.25));
#131812=CARTESIAN_POINT('Ctrl Pts',(0.218252011,1.714550109,7.246714156));
#131813=CARTESIAN_POINT('Ctrl Pts',(0.213507107014918,1.71532338944195,
7.2468555054415));
#131814=CARTESIAN_POINT('Ctrl Pts',(0.142250895423482,1.72693520767621,
7.24895485834218));
#131815=CARTESIAN_POINT('Ctrl Pts',(0.0710665482432402,1.73849644464489,
7.24999999999807));
#131816=CARTESIAN_POINT('Ctrl Pts',(1.97018677014537E-10,1.74999999996597,
7.2500000000132));
#131817=CARTESIAN_POINT('Ctrl Pts',(-0.147682176765806,1.77390534111371,
7.25000000004464));
#131818=CARTESIAN_POINT('Ctrl Pts',(-0.295873957336015,1.79806004030465,
7.2454834246082));
#131819=CARTESIAN_POINT('Ctrl Pts',(-0.444159548931349,1.82239932104086,
7.23638185097581));
#131820=CARTESIAN_POINT('Ctrl Pts',(-0.488488627306059,1.82967540141882,
7.23366099073213));
#131821=CARTESIAN_POINT('Ctrl Pts',(-0.532826001291235,1.83696795052539,
7.23053072198764));
#131822=CARTESIAN_POINT('Ctrl Pts',(-0.577160369311128,1.84427517387865,
7.22699009993985));
#131823=CARTESIAN_POINT('Ctrl Pts',(-1.356373314,4.042807359,7.121990693));
#131824=CARTESIAN_POINT('Ctrl Pts',(-0.967555641,4.108510123,7.196040483));
#131825=CARTESIAN_POINT('Ctrl Pts',(-0.572987507000001,4.173674111,7.22732214));
#131826=CARTESIAN_POINT('Ctrl Pts',(-1.160767276,4.042807359,7.409630175));
#131827=CARTESIAN_POINT('Ctrl Pts',(-0.756246224,4.108510123,7.473001057));
#131828=CARTESIAN_POINT('Ctrl Pts',(-0.347230585,4.173674111,7.49195775000001));
#131829=CARTESIAN_POINT('',(-0.57767741387148,4.17289950682494,7.2269487950413));
#131830=CARTESIAN_POINT('Ctrl Pts',(-0.577677421570388,4.17289950544926,
7.22694879416544));
#131831=CARTESIAN_POINT('Ctrl Pts',(-0.581165056550137,4.16602041298585,
7.26840987604015));
#131832=CARTESIAN_POINT('Ctrl Pts',(-0.584634097524575,4.15930620363512,
7.30992460671165));
#131833=CARTESIAN_POINT('Ctrl Pts',(-0.5915309518297,4.14619777610803,7.39295902153762));
#131834=CARTESIAN_POINT('Ctrl Pts',(-0.594962596891404,4.13979627490491,
7.43452487823737));
#131835=CARTESIAN_POINT('Ctrl Pts',(-0.598375443565973,4.13354310001741,
7.47609168121553));
#131836=CARTESIAN_POINT('Origin',(0.0411432879379811,4.01786903905992,-0.19371389706037));
#131837=CARTESIAN_POINT('Ctrl Pts',(-2.122257426,4.173681702,6.932425508));
#131838=CARTESIAN_POINT('Ctrl Pts',(-1.744480471,4.108088716,7.04807622));
#131839=CARTESIAN_POINT('Ctrl Pts',(-1.356373314,4.042807359,7.121990693));
#131840=CARTESIAN_POINT('Ctrl Pts',(-1.34295702550999,4.0405506793621,7.12454580664703));
#131841=CARTESIAN_POINT('Ctrl Pts',(-1.32954073702,4.03829399972412,7.1271009202939));
#131842=CARTESIAN_POINT('Ctrl Pts',(-2.43008400264692,4.173681702,7.09595388132405));
#131843=CARTESIAN_POINT('Ctrl Pts',(-2.04339570073195,4.108088716,7.22837935535182));
#131844=CARTESIAN_POINT('Ctrl Pts',(-1.64460712498496,4.042807359,7.31800089883344));
#131845=CARTESIAN_POINT('Ctrl Pts',(-1.63082159569944,4.0405506793621,7.32109898259864));
#131846=CARTESIAN_POINT('Ctrl Pts',(-1.61703606641398,4.03829399972412,
7.32419706636394));
#131847=CARTESIAN_POINT('',(-2.11775200231854,4.17289950637609,6.93380317648907));
#131848=CARTESIAN_POINT('Origin',(0.0562465567860779,4.16071258307181,-0.191024216299545));
#131849=CARTESIAN_POINT('Ctrl Pts',(-2.19152447788009,4.13354310002878,
7.1726717795594));
#131850=CARTESIAN_POINT('Ctrl Pts',(-2.17925578861821,4.13979627445688,
7.13281044940035));
#131851=CARTESIAN_POINT('Ctrl Pts',(-2.16696894385799,4.14619777521132,
7.09295408430292));
#131852=CARTESIAN_POINT('Ctrl Pts',(-2.14238339093939,4.15930620199799,
7.01334359200757));
#131853=CARTESIAN_POINT('Ctrl Pts',(-2.13007101043476,4.16602041351798,
6.97354518103625));
#131854=CARTESIAN_POINT('Ctrl Pts',(-2.11775200767413,4.17289950597958,
6.93380317476033));
#131855=CARTESIAN_POINT('Ctrl Pts',(-2.85697152392,4.042807359,6.66067269852999));
#131856=CARTESIAN_POINT('Ctrl Pts',(-2.49333902583,4.108510123,6.81664608632));
#131857=CARTESIAN_POINT('Ctrl Pts',(-2.11488790018,4.173674111,6.93210619159));
#131858=CARTESIAN_POINT('Ctrl Pts',(-2.855679535,4.042807359,6.66390234));
#131859=CARTESIAN_POINT('Ctrl Pts',(-2.491870718,4.108510123,6.81980519300001));
#131860=CARTESIAN_POINT('Ctrl Pts',(-2.113252,4.173674111,6.935175988));
#131861=CARTESIAN_POINT('Ctrl Pts',(-2.726480643,4.042807359,6.986866487));
#131862=CARTESIAN_POINT('Ctrl Pts',(-2.345039935,4.108510123,7.135715861));
#131863=CARTESIAN_POINT('Ctrl Pts',(-1.949661982,4.173674111,7.242155629));
#131864=CARTESIAN_POINT('Origin',(0.0818241170220929,4.01786906021735,-0.180340324830033));
#131865=CARTESIAN_POINT('Ctrl Pts',(-3.56290679,4.173681702,6.314126639));
#131866=CARTESIAN_POINT('Ctrl Pts',(-3.218823535,4.108088716,6.50828438));
#131867=CARTESIAN_POINT('Ctrl Pts',(-2.855679535,4.042807359,6.66390234));
#131868=CARTESIAN_POINT('Ctrl Pts',(-2.84312618582388,4.04055067936573,
6.66928182194095));
#131869=CARTESIAN_POINT('Ctrl Pts',(-2.83057283664774,4.03829399973139,
6.67466130388175));
#131870=CARTESIAN_POINT('Ctrl Pts',(-3.89869031899568,4.173681702,6.40765819510463));
#131871=CARTESIAN_POINT('Ctrl Pts',(-3.54951013729434,4.108088716,6.62011418952331));
#131872=CARTESIAN_POINT('Ctrl Pts',(-3.17931099982446,4.042807359,6.79336818647261));
#131873=CARTESIAN_POINT('Ctrl Pts',(-3.16651376501578,4.04055067936573,
6.79935732003907));
#131874=CARTESIAN_POINT('Ctrl Pts',(-3.15371653020715,4.03829399973139,
6.80534645360562));
#131875=CARTESIAN_POINT('',(-3.55880278961537,4.17289951177096,6.31644066991972));
#131876=CARTESIAN_POINT('Origin',(0.0959961150006616,4.16071256757818,-0.174466852259469));
#131877=CARTESIAN_POINT('Ctrl Pts',(-3.68220026361106,4.13354309997035,
6.53386571769809));
#131878=CARTESIAN_POINT('Ctrl Pts',(-3.6616494017322,4.13979627441468,6.4975737287741));
#131879=CARTESIAN_POINT('Ctrl Pts',(-3.64108187621462,4.14619777516013,
6.46129049185571));
#131880=CARTESIAN_POINT('Ctrl Pts',(-3.59995721709266,4.15930620195124,
6.38882641575838));
#131881=CARTESIAN_POINT('Ctrl Pts',(-3.57937721046934,4.16602041369041,
6.35260526619195));
#131882=CARTESIAN_POINT('Ctrl Pts',(-3.55880286240089,4.17289950613706,
6.31644062743981));
#131883=CARTESIAN_POINT('Ctrl Pts',(-4.22202485949,4.042807359,5.89078544632999));
#131884=CARTESIAN_POINT('Ctrl Pts',(-3.90042355506,4.108510123,6.1212825017));
#131885=CARTESIAN_POINT('Ctrl Pts',(-3.55564091525,4.173674111,6.31539901854001));
#131886=CARTESIAN_POINT('Ctrl Pts',(-4.221457354,4.042807359,5.89421732));
#131887=CARTESIAN_POINT('Ctrl Pts',(-3.89966869,4.108510123,6.124683393));
#131888=CARTESIAN_POINT('Ctrl Pts',(-3.554703177,4.173674111,6.318748715));
#131889=CARTESIAN_POINT('Ctrl Pts',(-4.164706805,4.042807359,6.237404687));
#131890=CARTESIAN_POINT('Ctrl Pts',(-3.824182184,4.108510123,6.464772523));
#131891=CARTESIAN_POINT('Ctrl Pts',(-3.460929352,4.173674111,6.653718361));
#131892=CARTESIAN_POINT('Origin',(0.118679043510761,4.0178690429932,-0.158534450043609));
#131893=CARTESIAN_POINT('Ctrl Pts',(-4.836958592,4.173681702,5.400586226));
#131894=CARTESIAN_POINT('Ctrl Pts',(-4.54265798800001,4.108088716,5.664172395));
#131895=CARTESIAN_POINT('Ctrl Pts',(-4.221457354,4.042807359,5.89421732));
#131896=CARTESIAN_POINT('Ctrl Pts',(-4.21035392510298,4.04055067943894,
5.90216963141373));
#131897=CARTESIAN_POINT('Ctrl Pts',(-4.19925049620598,4.03829399987781,
5.91012194282748));
#131898=CARTESIAN_POINT('Ctrl Pts',(-5.18499820863676,4.173681702,5.41974753300654));
#131899=CARTESIAN_POINT('Ctrl Pts',(-4.88965342356855,4.108088716,5.70229984158404));
#131900=CARTESIAN_POINT('Ctrl Pts',(-4.5653538246012,4.042807359,5.95108512861541));
#131901=CARTESIAN_POINT('Ctrl Pts',(-4.55414326908762,4.04055067943894,
5.95968526651294));
#131902=CARTESIAN_POINT('Ctrl Pts',(-4.54293271357389,4.03829399987781,
5.96828540441047));
#131903=CARTESIAN_POINT('',(-4.83344804812553,4.17289950636361,5.4037283423453));
#131904=CARTESIAN_POINT('Origin',(0.131257016296314,4.1607126306623,-0.149751590677861));
#131905=CARTESIAN_POINT('Ctrl Pts',(-5.00070045707408,4.13354310000987,
5.5895433562025));
#131906=CARTESIAN_POINT('Ctrl Pts',(-4.97282835816321,4.13979627444877,
5.55851768164219));
#131907=CARTESIAN_POINT('Ctrl Pts',(-4.94494186657699,4.14619777519739,
5.52750413664097));
#131908=CARTESIAN_POINT('Ctrl Pts',(-4.88920104484026,4.15930620198616,
5.46557481653246));
#131909=CARTESIAN_POINT('Ctrl Pts',(-4.86131571175525,4.16602041350881,
5.43462459145768));
#131910=CARTESIAN_POINT('Ctrl Pts',(-4.83344805214332,4.17289950595417,
5.40372833863019));
#131911=CARTESIAN_POINT('Ctrl Pts',(-5.38966100413,4.042807359,4.84545161372));
#131912=CARTESIAN_POINT('Ctrl Pts',(-5.12512861464,4.108510123,5.13969454897));
#131913=CARTESIAN_POINT('Ctrl Pts',(-4.83013611373001,4.173674111,5.40339080558));
#131914=CARTESIAN_POINT('Ctrl Pts',(-5.389844518,4.042807359,4.848925249));
#131915=CARTESIAN_POINT('Ctrl Pts',(-5.125122489,4.108510123,5.143178203));
#131916=CARTESIAN_POINT('Ctrl Pts',(-4.829940385,4.173674111,5.406863774));
#131917=CARTESIAN_POINT('Ctrl Pts',(-5.408195905,4.042807359,5.196288777));
#131918=CARTESIAN_POINT('Ctrl Pts',(-5.124509925,4.108510123,5.491543606));
#131919=CARTESIAN_POINT('Ctrl Pts',(-4.810367512,4.173674111,5.75416061600001));
#131920=CARTESIAN_POINT('Origin',(0.149984530496082,4.0178690506638,-0.129315426812652));
#131921=CARTESIAN_POINT('Ctrl Pts',(-5.88483958600001,4.173681702,4.234520403));
#131922=CARTESIAN_POINT('Ctrl Pts',(-5.654082801,4.108088716,4.555210005));
#131923=CARTESIAN_POINT('Ctrl Pts',(-5.389844518,4.042807359,4.848925249));
#131924=CARTESIAN_POINT('Ctrl Pts',(-5.3807101926145,4.04055067934832,4.85907854919147));
#131925=CARTESIAN_POINT('Ctrl Pts',(-5.37157586722897,4.03829399969656,
4.86923184938294));
#131926=CARTESIAN_POINT('Ctrl Pts',(-6.22886134497027,4.173681702,4.17841550046807));
#131927=CARTESIAN_POINT('Ctrl Pts',(-6.00116195121418,4.108088716,4.51785229157821));
#131928=CARTESIAN_POINT('Ctrl Pts',(-5.73792577853392,4.042807359,4.83053594383522));
#131929=CARTESIAN_POINT('Ctrl Pts',(-5.72882609461528,4.04055067934832,
4.84134495375618));
#131930=CARTESIAN_POINT('Ctrl Pts',(-5.71972641069679,4.03829399969656,
4.85215396367713));
#131931=CARTESIAN_POINT('',(-5.88208653312298,4.17289951178147,4.23834378550683));
#131932=CARTESIAN_POINT('Origin',(0.160380289703171,4.16071263034052,-0.118033961145265));
#131933=CARTESIAN_POINT('Ctrl Pts',(-6.08537345500513,4.13354310000783,
4.38386016046888));
#131934=CARTESIAN_POINT('Ctrl Pts',(-6.05148338734865,4.13979627444683,
4.359551526254));
#131935=CARTESIAN_POINT('Ctrl Pts',(-6.01758187087438,4.14619777522652,
4.33525783186004));
#131936=CARTESIAN_POINT('Ctrl Pts',(-5.94983126543378,4.15930620203592,
4.28675901346378));
#131937=CARTESIAN_POINT('Ctrl Pts',(-5.91594449174928,4.16602041372458,
4.26252690899275));
#131938=CARTESIAN_POINT('Ctrl Pts',(-5.88208658157426,4.17289950620119,
4.23834371608479));
#131939=CARTESIAN_POINT('Ctrl Pts',(-6.30528259168001,4.042807359,3.57354984844));
#131940=CARTESIAN_POINT('Ctrl Pts',(-6.11018835478,4.108510123,3.91778019304));
#131941=CARTESIAN_POINT('Ctrl Pts',(-5.87877951616001,4.173674111,4.23872604476));
#131942=CARTESIAN_POINT('Ctrl Pts',(-6.306208544,4.042807359,3.576902822));
#131943=CARTESIAN_POINT('Ctrl Pts',(-6.110931255,4.108510123,3.921183718));
#131944=CARTESIAN_POINT('Ctrl Pts',(-5.87933494900001,4.173674111,4.242159893));
#131945=CARTESIAN_POINT('Ctrl Pts',(-6.398803776,4.042807359,3.912200178));
#131946=CARTESIAN_POINT('Ctrl Pts',(-6.185221277,4.108510123,4.261536214));
#131947=CARTESIAN_POINT('Ctrl Pts',(-5.934878233,4.173674111,4.585544717));
#131948=CARTESIAN_POINT('Origin',(0.174276787464549,4.01786905587483,-0.094049750877061));
#131949=CARTESIAN_POINT('Ctrl Pts',(-6.657552022,4.173681702,2.870453113));
#131950=CARTESIAN_POINT('Ctrl Pts',(-6.501128988,4.108088716,3.233251058));
#131951=CARTESIAN_POINT('Ctrl Pts',(-6.306208544,4.042807359,3.576902822));
#131952=CARTESIAN_POINT('Ctrl Pts',(-6.29947043335256,4.04055067931237,
3.58878235378487));
#131953=CARTESIAN_POINT('Ctrl Pts',(-6.2927323227051,4.03829399962467,3.60066188556971));
#131954=CARTESIAN_POINT('Ctrl Pts',(-6.98146984730646,4.173681702,2.74170540229433));
#131955=CARTESIAN_POINT('Ctrl Pts',(-6.83206281608218,4.108088716,3.12215498942187));
#131956=CARTESIAN_POINT('Ctrl Pts',(-6.64219870107257,4.042807359,3.48411626705964));
#131957=CARTESIAN_POINT('Ctrl Pts',(-6.63563538021891,4.04055067931237,
3.4966287315747));
#131958=CARTESIAN_POINT('Ctrl Pts',(-6.62907205936524,4.03829399962466,
3.5091411960898));
#131959=CARTESIAN_POINT('',(-6.65568527962966,4.17289950637162,2.87477885958419));
#131960=CARTESIAN_POINT('Origin',(0.18200448439748,4.16071258288865,-0.0807973746653828));
#131961=CARTESIAN_POINT('Ctrl Pts',(-6.88550115417661,4.13354309998774,
2.97319253546826));
#131962=CARTESIAN_POINT('Ctrl Pts',(-6.84717777957122,4.13979627444384,
2.95673758635237));
#131963=CARTESIAN_POINT('Ctrl Pts',(-6.80884643569607,4.14619777519811,
2.94029968905659));
#131964=CARTESIAN_POINT('Ctrl Pts',(-6.73225398929105,4.15930620203543,
2.90749912360423));
#131965=CARTESIAN_POINT('Ctrl Pts',(-6.69395028459455,4.16602041351321,
2.89111820751232));
#131966=CARTESIAN_POINT('Ctrl Pts',(-6.65568528188716,4.17289950599813,
2.87477885414013));
#131967=CARTESIAN_POINT('Ctrl Pts',(-6.92607617273,4.042807359,2.13455286448));
#131968=CARTESIAN_POINT('Ctrl Pts',(-6.80954247911,4.108510123,2.51267478814));
#131969=CARTESIAN_POINT('Ctrl Pts',(-6.65253772200001,4.173674111,2.87586316486001));
#131970=CARTESIAN_POINT('Ctrl Pts',(-6.927701267,4.042807359,2.137628395));
#131971=CARTESIAN_POINT('Ctrl Pts',(-6.810999668,4.108510123,2.515839039));
#131972=CARTESIAN_POINT('Ctrl Pts',(-6.653818345,4.173674111,2.87909733));
#131973=CARTESIAN_POINT('Ctrl Pts',(-7.090210694,4.042807359,2.445181447));
#131974=CARTESIAN_POINT('Ctrl Pts',(-6.956718557,4.108510123,2.832264125));
#131975=CARTESIAN_POINT('Ctrl Pts',(-6.781880645,4.173674111,3.202513844));
#131976=CARTESIAN_POINT('Origin',(0.19042057799295,4.01786904786398,-0.0543866950544405));
#131977=CARTESIAN_POINT('Ctrl Pts',(-7.118964725,4.173681702,1.372166625));
#131978=CARTESIAN_POINT('Ctrl Pts',(-7.044189608,4.108088716,1.760108884));
#131979=CARTESIAN_POINT('Ctrl Pts',(-6.927701267,4.042807359,2.137628395));
#131980=CARTESIAN_POINT('Ctrl Pts',(-6.92367443794669,4.04055067938082,
2.15067868417093));
#131981=CARTESIAN_POINT('Ctrl Pts',(-6.91964760889334,4.03829399976158,
2.16372897334185));
#131982=CARTESIAN_POINT('Ctrl Pts',(-7.4076325789629,4.173681702,1.17679620739295));
#131983=CARTESIAN_POINT('Ctrl Pts',(-7.34350401581941,4.108088716,1.58046918964557));
#131984=CARTESIAN_POINT('Ctrl Pts',(-7.23588979397176,4.042807359,1.97478318634262));
#131985=CARTESIAN_POINT('Ctrl Pts',(-7.23216973004631,4.04055067938082,
1.98841403595727));
#131986=CARTESIAN_POINT('Ctrl Pts',(-7.22844966612089,4.03829399976157,
2.00204488557198));
#131987=CARTESIAN_POINT('',(-7.11807151787488,4.17289951178047,1.37679261006278));
#131988=CARTESIAN_POINT('Origin',(0.195118497292496,4.16071260882338,-0.0397828217243851));
#131989=CARTESIAN_POINT('Ctrl Pts',(-7.36367047159053,4.13354310001364,
1.42350173179299));
#131990=CARTESIAN_POINT('Ctrl Pts',(-7.3227057484912,4.13979627446707,1.41566988296896));
#131991=CARTESIAN_POINT('Ctrl Pts',(-7.28173690833156,4.14619777517845,
1.40785640051236));
#131992=CARTESIAN_POINT('Ctrl Pts',(-7.19988399878459,4.15930620199099,
1.39228780605833));
#131993=CARTESIAN_POINT('Ctrl Pts',(-7.1589543988164,4.16602041376379,1.38452403064383));
#131994=CARTESIAN_POINT('Ctrl Pts',(-7.1180715326786,4.17289950622846,1.37679252684336));
#131995=CARTESIAN_POINT('Ctrl Pts',(-7.22301412936999,4.042807359,0.5957465609));
#131996=CARTESIAN_POINT('Ctrl Pts',(-7.19048996598,4.108510123,0.990079504110001));
#131997=CARTESIAN_POINT('Ctrl Pts',(-7.11523065735001,4.173674111,1.37852811994));
#131998=CARTESIAN_POINT('Ctrl Pts',(-7.225262378,4.042807359,0.59840084));
#131999=CARTESIAN_POINT('Ctrl Pts',(-7.192593307,4.108510123,0.992856524000001));
#132000=CARTESIAN_POINT('Ctrl Pts',(-7.11717659000001,4.173674111,1.381411376));
#132001=CARTESIAN_POINT('Ctrl Pts',(-7.450087241,4.042807359,0.86382875));
#132002=CARTESIAN_POINT('Ctrl Pts',(-7.402927409,4.108510123,1.270558513));
#132003=CARTESIAN_POINT('Ctrl Pts',(-7.311769855,4.173674111,1.669736982));
#132004=CARTESIAN_POINT('Origin',(0.197660024976012,4.01786908484965,-0.0121803578723476));
#132005=CARTESIAN_POINT('Ctrl Pts',(-7.247502549,4.173681702,-0.190280849));
#132006=CARTESIAN_POINT('Ctrl Pts',(-7.257871751,4.108088716,0.204665976));
#132007=CARTESIAN_POINT('Ctrl Pts',(-7.225262378,4.042807359,0.59840084));
#132008=CARTESIAN_POINT('Ctrl Pts',(-7.22413512038967,4.04055067941005,
0.612011669680603));
#132009=CARTESIAN_POINT('Ctrl Pts',(-7.22300786277932,4.03829399982003,
0.625622499361206));
#132010=CARTESIAN_POINT('Ctrl Pts',(-7.48742264462432,4.173681702,-0.443138670805177));
#132011=CARTESIAN_POINT('Ctrl Pts',(-7.51157113006956,4.108088716,-0.0351175931109789));
#132012=CARTESIAN_POINT('Ctrl Pts',(-7.49123872278329,4.042807359,0.373111438402523));
#132013=CARTESIAN_POINT('Ctrl Pts',(-7.4905358616504,4.04055067941005,0.387223309934955));
#132014=CARTESIAN_POINT('Ctrl Pts',(-7.48983300051752,4.03829399982002,
0.401335181467389));
#132015=CARTESIAN_POINT('',(-7.24762467318051,4.17289950634919,-0.185571082546173));
#132016=CARTESIAN_POINT('Origin',(0.199108805722675,4.16071257662121,0.00309198393094883));
#132017=CARTESIAN_POINT('Ctrl Pts',(-7.49752274180161,4.13354309997187,
-0.192750430437809));
#132018=CARTESIAN_POINT('Ctrl Pts',(-7.45583213525102,4.13979627442737,
-0.19159297045491));
#132019=CARTESIAN_POINT('Ctrl Pts',(-7.41414145586947,4.14619777517913,
-0.190416688450836));
#132020=CARTESIAN_POINT('Ctrl Pts',(-7.33085543430957,4.15930620200286,
-0.188025341891005));
#132021=CARTESIAN_POINT('Ctrl Pts',(-7.28921376519328,4.16602041349394,
-0.186808950522999));
#132022=CARTESIAN_POINT('Ctrl Pts',(-7.24762467294151,4.17289950595543,
-0.185571088387518));
#132023=CARTESIAN_POINT('Ctrl Pts',(-7.18221197363,4.042807359,-0.970916189530001));
#132024=CARTESIAN_POINT('Ctrl Pts',(-7.23521813274001,4.108510123,-0.57881079857));
#132025=CARTESIAN_POINT('Ctrl Pts',(-7.24522331535001,4.173674111,-0.18326536814));
#132026=CARTESIAN_POINT('Ctrl Pts',(-7.184978251,4.042807359,-0.968807273));
#132027=CARTESIAN_POINT('Ctrl Pts',(-7.237869276,4.108510123,-0.57655086));
#132028=CARTESIAN_POINT('Ctrl Pts',(-7.247743568,4.173674111,-0.180867839));
#132029=CARTESIAN_POINT('Ctrl Pts',(-7.461605988,4.042807359,-0.75791562));
#132030=CARTESIAN_POINT('Ctrl Pts',(-7.502983602,4.108510123,-0.350557003));
#132031=CARTESIAN_POINT('Ctrl Pts',(-7.499768833,4.173674111,0.058885075));
#132032=CARTESIAN_POINT('Origin',(0.195657217993492,4.01786906992177,0.0305954721080647));
#132033=CARTESIAN_POINT('Ctrl Pts',(-7.037155209,4.173681702,-1.743831002));
#132034=CARTESIAN_POINT('Ctrl Pts',(-7.13218387800001,4.108088716,-1.360346886));
#132035=CARTESIAN_POINT('Ctrl Pts',(-7.18497825100001,4.042807359,-0.968807273));
#132036=CARTESIAN_POINT('Ctrl Pts',(-7.18680327408043,4.04055067942458,
-0.955272329974366));
#132037=CARTESIAN_POINT('Ctrl Pts',(-7.18862829716087,4.03829399984908,
-0.941737386948719));
#132038=CARTESIAN_POINT('Ctrl Pts',(-7.21710914931246,4.173681702,-2.04235287662919));
#132039=CARTESIAN_POINT('Ctrl Pts',(-7.32840552681098,4.108088716,-1.64906231605176));
#132040=CARTESIAN_POINT('Ctrl Pts',(-7.39630565439742,4.042807359,-1.24600658618435));
#132041=CARTESIAN_POINT('Ctrl Pts',(-7.39865286098343,4.04055067942458,
-1.23207354809886));
#132042=CARTESIAN_POINT('Ctrl Pts',(-7.40100006756945,4.03829399984908,
-1.21814051001333));
#132043=CARTESIAN_POINT('',(-7.03828695718376,4.17289951177251,-1.73925752363152));
#132044=CARTESIAN_POINT('Origin',(0.193788930123852,4.16071258056698,0.0458221794985492));
#132045=CARTESIAN_POINT('Ctrl Pts',(-7.28079918183226,4.13354309998201,
-1.7999897968914));
#132046=CARTESIAN_POINT('Ctrl Pts',(-7.24033209814515,4.13979627444535,
-1.78989714956336));
#132047=CARTESIAN_POINT('Ctrl Pts',(-7.19986898956744,4.14619777519187,
-1.77978610465057));
#132048=CARTESIAN_POINT('Ctrl Pts',(-7.11904421763658,4.15930620201941,
-1.75954663372673));
#132049=CARTESIAN_POINT('Ctrl Pts',(-7.07863759428674,4.16602041375186,
-1.74940695265407));
#132050=CARTESIAN_POINT('Ctrl Pts',(-7.03828693559596,4.17289950621262,
-1.73925760568948));
#132051=CARTESIAN_POINT('Ctrl Pts',(-6.80557756794,4.042807359,-2.49217997837));
#132052=CARTESIAN_POINT('Ctrl Pts',(-6.94163554200999,4.108510123,-2.12063655002));
#132053=CARTESIAN_POINT('Ctrl Pts',(-7.03643738356,4.173674111,-1.73648957142));
#132054=CARTESIAN_POINT('Ctrl Pts',(-6.808732526,4.042807359,-2.490715035));
#132055=CARTESIAN_POINT('Ctrl Pts',(-6.944710523,4.108510123,-2.118999365));
#132056=CARTESIAN_POINT('Ctrl Pts',(-7.039414112,4.173674111,-1.734689875));
#132057=CARTESIAN_POINT('Ctrl Pts',(-7.12422833200001,4.042807359,-2.344220698));
#132058=CARTESIAN_POINT('Ctrl Pts',(-7.252208622,4.108510123,-1.955280863));
#132059=CARTESIAN_POINT('Ctrl Pts',(-7.33708695600001,4.173674111,-1.554720233));
#132060=CARTESIAN_POINT('Origin',(0.184505509730328,4.01786907984804,0.0719406205453618));
#132061=CARTESIAN_POINT('Ctrl Pts',(-6.497758313,4.173681702,-3.215841555));
#132062=CARTESIAN_POINT('Ctrl Pts',(-6.67300301300001,4.108088716,-2.86175144));
#132063=CARTESIAN_POINT('Ctrl Pts',(-6.808732526,4.042807359,-2.490715035));
#132064=CARTESIAN_POINT('Ctrl Pts',(-6.81342449392482,4.04055067932614,
-2.47788885687033));
#132065=CARTESIAN_POINT('Ctrl Pts',(-6.81811646184952,4.03829399965221,
-2.46506267874058));
#132066=CARTESIAN_POINT('Ctrl Pts',(-6.60933165069055,4.173681702,-3.54606893239908));
#132067=CARTESIAN_POINT('Ctrl Pts',(-6.80257182679263,4.108088716,-3.1858987174254));
#132068=CARTESIAN_POINT('Ctrl Pts',(-6.95552955382461,4.042807359,-2.80686272653251));
#132069=CARTESIAN_POINT('Ctrl Pts',(-6.96081707555239,4.04055067932614,
-2.793760014585));
#132070=CARTESIAN_POINT('Ctrl Pts',(-6.96610459728,4.03829399965221,-2.7806573026375));
#132071=CARTESIAN_POINT('',(-6.49984676413174,4.17289951180422,-3.21161829486362));
#132072=CARTESIAN_POINT('Origin',(0.179407972082283,4.16071260285053,0.0864098315335438));
#132073=CARTESIAN_POINT('Ctrl Pts',(-6.72363354399547,4.13354310000101,
-3.32306364090028));
#132074=CARTESIAN_POINT('Ctrl Pts',(-6.68628217907727,4.13979627445217,
-3.30450772734517));
#132075=CARTESIAN_POINT('Ctrl Pts',(-6.64893865122487,4.14619777519857,
-3.28593470078994));
#132076=CARTESIAN_POINT('Ctrl Pts',(-6.57435440562825,4.15930620201408,
-3.24879348059528));
#132077=CARTESIAN_POINT('Ctrl Pts',(-6.53707219854965,4.16602041373077,
-3.23020462996973));
#132078=CARTESIAN_POINT('Ctrl Pts',(-6.49984672556043,4.17289950620038,
-3.21161837004206));
#132079=CARTESIAN_POINT('Ctrl Pts',(-6.11072191959001,4.042807359,-3.89691220109));
#132080=CARTESIAN_POINT('Ctrl Pts',(-6.32346978797,4.108510123,-3.56330369453));
#132081=CARTESIAN_POINT('Ctrl Pts',(-6.49863546028999,4.173674111,-3.20851745189));
#132082=CARTESIAN_POINT('Ctrl Pts',(-6.11411803600001,4.042807359,-3.89615973));
#132083=CARTESIAN_POINT('Ctrl Pts',(-6.326824824,4.108510123,-3.562365816));
#132084=CARTESIAN_POINT('Ctrl Pts',(-6.501929476,4.173674111,-3.20739974));
#132085=CARTESIAN_POINT('Ctrl Pts',(-6.453729677,4.042807359,-3.820912621));
#132086=CARTESIAN_POINT('Ctrl Pts',(-6.662328427,4.108510123,-3.468577963));
#132087=CARTESIAN_POINT('Ctrl Pts',(-6.831331047,4.173674111,-3.095628551));
#132088=CARTESIAN_POINT('Origin',(0.164726898386173,4.01786907394915,0.109921998321732));
#132089=CARTESIAN_POINT('Ctrl Pts',(-5.65453346,4.173681702,-4.537482931));
#132090=CARTESIAN_POINT('Ctrl Pts',(-5.901799944,4.108088716,-4.229343677));
#132091=CARTESIAN_POINT('Ctrl Pts',(-6.114118036,4.042807359,-3.89615973));
#132092=CARTESIAN_POINT('Ctrl Pts',(-6.12145755719561,4.04055067941673,
-3.88464205565578));
#132093=CARTESIAN_POINT('Ctrl Pts',(-6.12879707839122,4.03829399983337,
-3.8731243813116));
#132094=CARTESIAN_POINT('Ctrl Pts',(-5.69250915066893,4.173681702,-4.88397474512415));
#132095=CARTESIAN_POINT('Ctrl Pts',(-5.95865742732614,4.108088716,-4.57376603597331));
#132096=CARTESIAN_POINT('Ctrl Pts',(-6.18952062274081,4.042807359,-4.23647308634029));
#132097=CARTESIAN_POINT('Ctrl Pts',(-6.19750122062614,4.04055067941672,
-4.22481336987599));
#132098=CARTESIAN_POINT('Ctrl Pts',(-6.20548181851142,4.03829399983338,
-4.21315365341175));
#132099=CARTESIAN_POINT('',(-5.65748091122045,4.1728995063871,-4.5338074256061));
#132100=CARTESIAN_POINT('Origin',(0.156637907631271,4.16071263150207,0.122957005372363));
#132101=CARTESIAN_POINT('Ctrl Pts',(-5.85207827440955,4.13354310000206,
-4.69075472210398));
#132102=CARTESIAN_POINT('Ctrl Pts',(-5.81958913659606,4.13979627445759,
-4.66460319612005));
#132103=CARTESIAN_POINT('Ctrl Pts',(-5.78711133136791,4.14619777521706,
-4.63843664194184));
#132104=CARTESIAN_POINT('Ctrl Pts',(-5.72225508847915,4.15930620204372,
-4.58613035472719));
#132105=CARTESIAN_POINT('Ctrl Pts',(-5.68984057334137,4.16602041350361,
-4.55996152965675));
#132106=CARTESIAN_POINT('Ctrl Pts',(-5.657480907676,4.17289950597006,-4.53380742988185));
#132107=CARTESIAN_POINT('Ctrl Pts',(-5.13013570587,4.042807359,-5.11942914009));
#132108=CARTESIAN_POINT('Ctrl Pts',(-5.40962561367999,4.108510123,-4.83935471788));
#132109=CARTESIAN_POINT('Ctrl Pts',(-5.65696456552999,4.173674111,-4.5305186224));
#132110=CARTESIAN_POINT('Ctrl Pts',(-5.133614182,4.042807359,-5.119424326));
#132111=CARTESIAN_POINT('Ctrl Pts',(-5.413103827,4.108510123,-4.83916));
#132112=CARTESIAN_POINT('Ctrl Pts',(-5.660421844,4.173674111,-4.530135158));
#132113=CARTESIAN_POINT('Ctrl Pts',(-5.481461795,4.042807359,-5.118942917));
#132114=CARTESIAN_POINT('Ctrl Pts',(-5.760925159,4.108510123,-4.819688212));
#132115=CARTESIAN_POINT('Ctrl Pts',(-6.00614969100001,4.173674111,-4.491788718));
#132116=CARTESIAN_POINT('Origin',(0.137245792838453,4.01786906965473,0.142763576683332));
#132117=CARTESIAN_POINT('Ctrl Pts',(-4.546908906,4.173681702,-5.646956649));
#132118=CARTESIAN_POINT('Ctrl Pts',(-4.854635269,4.108088716,-5.399176504));
#132119=CARTESIAN_POINT('Ctrl Pts',(-5.133614182,4.042807359,-5.119424326));
#132120=CARTESIAN_POINT('Ctrl Pts',(-5.14325806887437,4.0405506793996,-5.10975370850253));
#132121=CARTESIAN_POINT('Ctrl Pts',(-5.15290195574862,4.03829399979913,
-5.10008309100504));
#132122=CARTESIAN_POINT('Ctrl Pts',(-4.50951124921801,4.173681702,-5.99351132775443));
#132123=CARTESIAN_POINT('Ctrl Pts',(-4.83612282993789,4.108088716,-5.7477691379534));
#132124=CARTESIAN_POINT('Ctrl Pts',(-5.13409658570113,4.042807359,-5.46799067275003));
#132125=CARTESIAN_POINT('Ctrl Pts',(-5.14439709609169,4.0405506793996,-5.45831914654295));
#132126=CARTESIAN_POINT('Ctrl Pts',(-5.15469760648239,4.03829399979914,
-5.44864762033589));
#132127=CARTESIAN_POINT('',(-4.55057757302164,4.17289950635597,-5.6440006891764));
#132128=CARTESIAN_POINT('Origin',(0.126543657505769,4.16071261389245,0.153754834376969));
#132129=CARTESIAN_POINT('Ctrl Pts',(-4.7068863288185,4.13354310002961,-5.83911132633498));
#132130=CARTESIAN_POINT('Ctrl Pts',(-4.68077857400211,4.13979627448026,
-5.8065870041996));
#132131=CARTESIAN_POINT('Ctrl Pts',(-4.65468511743214,4.14619777522813,
-5.7740504414094));
#132132=CARTESIAN_POINT('Ctrl Pts',(-4.60258948287892,4.15930620202736,
-5.70902487101796));
#132133=CARTESIAN_POINT('Ctrl Pts',(-4.57655832475415,4.16602041348794,
-5.67649969586828));
#132134=CARTESIAN_POINT('Ctrl Pts',(-4.55057756827482,4.17289950593458,
-5.64400069288196));
#132135=CARTESIAN_POINT('Ctrl Pts',(-3.90967004782,4.042807359,-6.102567263));
#132136=CARTESIAN_POINT('Ctrl Pts',(-4.24283335879,4.108510123,-5.88912289343));
#132137=CARTESIAN_POINT('Ctrl Pts',(-4.55078029527,4.173674111,-5.64067777754));
#132138=CARTESIAN_POINT('Ctrl Pts',(-3.913068234,4.042807359,-6.103310331));
#132139=CARTESIAN_POINT('Ctrl Pts',(-4.246272112,4.108510123,-5.889680441));
#132140=CARTESIAN_POINT('Ctrl Pts',(-4.554239178,4.173674111,-5.641046491));
#132141=CARTESIAN_POINT('Ctrl Pts',(-4.252886852,4.042807359,-6.177617131));
#132142=CARTESIAN_POINT('Ctrl Pts',(-4.590147433,4.108510123,-5.945435198));
#132143=CARTESIAN_POINT('Ctrl Pts',(-4.900127451,4.173674111,-5.677917837));
#132144=CARTESIAN_POINT('Origin',(0.103347005926283,4.01786907058862,0.168929478668518));
#132145=CARTESIAN_POINT('Ctrl Pts',(-3.226675946,4.173681702,-6.49238495));
#132146=CARTESIAN_POINT('Ctrl Pts',(-3.580473244,4.108088716,-6.316549838));
#132147=CARTESIAN_POINT('Ctrl Pts',(-3.913068234,4.042807359,-6.103310331));
#132148=CARTESIAN_POINT('Ctrl Pts',(-3.92456554946237,4.0405506793211,-6.09593895754359));
#132149=CARTESIAN_POINT('Ctrl Pts',(-3.9360628649248,4.03829399964212,-6.08856758408716));
#132150=CARTESIAN_POINT('Ctrl Pts',(-3.11565361346413,4.173681702,-6.82279798221495));
#132151=CARTESIAN_POINT('Ctrl Pts',(-3.48745650442695,4.108088716,-6.65301294327412));
#132152=CARTESIAN_POINT('Ctrl Pts',(-3.83860789814411,4.042807359,-6.44383109203186));
#132153=CARTESIAN_POINT('Ctrl Pts',(-3.85074668095807,4.0405506793211,-6.43659998571625));
#132154=CARTESIAN_POINT('Ctrl Pts',(-3.86288546377205,4.03829399964212,
-6.42936887940052));
#132155=CARTESIAN_POINT('',(-3.2308943560275,4.17289951171542,-6.49028671834694));
#132156=CARTESIAN_POINT('Origin',(0.0905324415274239,4.16071263741196,0.177363367578599));
#132157=CARTESIAN_POINT('Ctrl Pts',(-3.34160561000943,4.13354310003923,
-6.71443757429057));
#132158=CARTESIAN_POINT('Ctrl Pts',(-3.32310000783745,4.1397962744689,-6.67706125735356));
#132159=CARTESIAN_POINT('Ctrl Pts',(-3.30461100089086,4.14619777523478,
-6.6396760594406));
#132160=CARTESIAN_POINT('Ctrl Pts',(-3.26771190878886,4.15930620202176,
-6.56497172952417));
#132161=CARTESIAN_POINT('Ctrl Pts',(-3.24928129517904,4.16602041374647,
-6.52761104404165));
#132162=CARTESIAN_POINT('Ctrl Pts',(-3.23089427937063,4.17289950621232,
-6.49028675509605));
#132163=CARTESIAN_POINT('Ctrl Pts',(-2.50639256418,4.042807359,-6.80035612293));
#132164=CARTESIAN_POINT('Ctrl Pts',(-2.87765093218,4.108510123,-6.6635222283));
#132165=CARTESIAN_POINT('Ctrl Pts',(-3.23180659552,4.173674111,-6.48708510932001));
#132166=CARTESIAN_POINT('Ctrl Pts',(-2.509551565,4.042807359,-6.801812328));
#132167=CARTESIAN_POINT('Ctrl Pts',(-2.880889433,4.108510123,-6.66480597100001));
#132168=CARTESIAN_POINT('Ctrl Pts',(-3.235105349,4.173674111,-6.48818876));
#132169=CARTESIAN_POINT('Ctrl Pts',(-2.825451647,4.042807359,-6.947432835));
#132170=CARTESIAN_POINT('Ctrl Pts',(-3.204739515,4.108510123,-6.793180241));
#132171=CARTESIAN_POINT('Ctrl Pts',(-3.564980697,4.173674111,-6.59855382800001));
#132172=CARTESIAN_POINT('Origin',(0.0646159969929783,4.01786908411667,0.187196633203744));
#132173=CARTESIAN_POINT('Ctrl Pts',(-1.755567205,4.173681702,-7.034236546));
#132174=CARTESIAN_POINT('Ctrl Pts',(-2.13889227,4.108088716,-6.93856832300001));
#132175=CARTESIAN_POINT('Ctrl Pts',(-2.509551565,4.042807359,-6.801812328));
#132176=CARTESIAN_POINT('Ctrl Pts',(-2.5223647071198,4.04055067930441,-6.79708487606959));
#132177=CARTESIAN_POINT('Ctrl Pts',(-2.53517784923958,4.03829399960873,
-6.79235742413929));
#132178=CARTESIAN_POINT('Ctrl Pts',(-1.57611147796785,4.173681702,-7.33305818576814));
#132179=CARTESIAN_POINT('Ctrl Pts',(-1.97572058815388,4.108088716,-7.2471692583663));
#132180=CARTESIAN_POINT('Ctrl Pts',(-2.36363017270524,4.042807359,-7.11836513186759));
#132181=CARTESIAN_POINT('Ctrl Pts',(-2.37703963175169,4.04055067930441,
-7.11391256423821));
#132182=CARTESIAN_POINT('Ctrl Pts',(-2.39044909079814,4.03829399960874,
-7.10945999660886));
#132183=CARTESIAN_POINT('',(-1.7601380483259,4.17289951177404,-7.03309420339446));
#132184=CARTESIAN_POINT('Origin',(0.050287931064856,4.16071264270228,0.192678423367151));
#132185=CARTESIAN_POINT('Ctrl Pts',(-1.82007512674651,4.13354310004032,
-7.27580418456825));
#132186=CARTESIAN_POINT('Ctrl Pts',(-1.81003697857167,4.13979627448677,
-7.23532354751039));
#132187=CARTESIAN_POINT('Ctrl Pts',(-1.80001694685657,4.14619777523088,
-7.19483780481292));
#132188=CARTESIAN_POINT('Ctrl Pts',(-1.78003975777084,4.1593062020288,-7.11394780620897));
#132189=CARTESIAN_POINT('Ctrl Pts',(-1.77007148471205,4.1660204137524,-7.0734985555225));
#132190=CARTESIAN_POINT('Ctrl Pts',(-1.76013796597784,4.17289950621194,
-7.03309422269299));
#132191=CARTESIAN_POINT('Ctrl Pts',(-0.9859189489,4.042807359,-7.1801678884));
#132192=CARTESIAN_POINT('Ctrl Pts',(-1.37791274627,4.108510123,-7.12634266953999));
#132193=CARTESIAN_POINT('Ctrl Pts',(-1.76171721181001,4.173674111,-7.03016355056001));
#132194=CARTESIAN_POINT('Ctrl Pts',(-0.988691053,4.042807359,-7.18226914));
#132195=CARTESIAN_POINT('Ctrl Pts',(-1.380799566,4.108510123,-7.128292581));
#132196=CARTESIAN_POINT('Ctrl Pts',(-1.76470159,4.173674111,-7.031950533));
#132197=CARTESIAN_POINT('Ctrl Pts',(-1.265901463,4.042807359,-7.3923943));
#132198=CARTESIAN_POINT('Ctrl Pts',(-1.669481539,4.108510123,-7.323283727));
#132199=CARTESIAN_POINT('Ctrl Pts',(-2.063139409,4.173674111,-7.210648777));
#132200=CARTESIAN_POINT('Origin',(0.0228636093082184,4.01786908234283,0.196710782424259));
#132201=CARTESIAN_POINT('Ctrl Pts',(-0.202370093,4.173681702,-7.24717506));
#132202=CARTESIAN_POINT('Ctrl Pts',(-0.597299071,4.108088716,-7.236147064));
#132203=CARTESIAN_POINT('Ctrl Pts',(-0.988691053000001,4.042807359,-7.18226914));
#132204=CARTESIAN_POINT('Ctrl Pts',(-1.00222089300913,4.04055067936321,
-7.18040666011983));
#132205=CARTESIAN_POINT('Ctrl Pts',(-1.01575073301826,4.03829399972634,
-7.17854418023955));
#132206=CARTESIAN_POINT('Ctrl Pts',(0.0371278792295015,4.173681702,-7.50043273830741));
#132207=CARTESIAN_POINT('Ctrl Pts',(-0.371602173148536,4.108088716,-7.50245599257189));
#132208=CARTESIAN_POINT('Ctrl Pts',(-0.778131726340653,4.042807359,-7.46005233013564));
#132209=CARTESIAN_POINT('Ctrl Pts',(-0.7921848497224,4.04055067936321,-7.45858649845042));
#132210=CARTESIAN_POINT('Ctrl Pts',(-0.806237973104149,4.03829399972634,
-7.45712066676505));
#132211=CARTESIAN_POINT('',(-0.207079563622813,4.17289950638492,-7.24704202295315));
#132212=CARTESIAN_POINT('Origin',(0.00769208186321351,4.16071261746617,
0.198984214355209));
#132213=CARTESIAN_POINT('Ctrl Pts',(-0.213439952651149,4.13354310325808,
-7.49696225529674));
#132214=CARTESIAN_POINT('Ctrl Pts',(-0.212338631208263,4.13979627774058,
-7.45527012810047));
#132215=CARTESIAN_POINT('Ctrl Pts',(-0.21125610081469,4.14619777521567,
-7.41357693052393));
#132216=CARTESIAN_POINT('Ctrl Pts',(-0.209134926115335,4.15930620200786,
-7.33028359035146));
#132217=CARTESIAN_POINT('Ctrl Pts',(-0.208095099130585,4.16602041357748,
-7.2886371377501));
#132218=CARTESIAN_POINT('Ctrl Pts',(-0.207079557951058,4.172899506042,-7.24704202303491));
#132219=CARTESIAN_POINT('Ctrl Pts',(0.580655139860001,4.042807359,-7.22424298406));
#132220=CARTESIAN_POINT('Ctrl Pts',(0.18625510917,4.108510123,-7.25594324748));
#132221=CARTESIAN_POINT('Ctrl Pts',(-0.20925188932,4.173674111,-7.24451935813));
#132222=CARTESIAN_POINT('Ctrl Pts',(0.578399553,4.042807359,-7.22689103));
#132223=CARTESIAN_POINT('Ctrl Pts',(0.183854955,4.108510123,-7.258468152));
#132224=CARTESIAN_POINT('Ctrl Pts',(-0.211782346,4.173674111,-7.24690611500001));
#132225=CARTESIAN_POINT('Ctrl Pts',(0.352840867,4.042807359,-7.491695624));
#132226=CARTESIAN_POINT('Ctrl Pts',(-0.056160462,4.108510123,-7.510958604));
#132227=CARTESIAN_POINT('Ctrl Pts',(-0.464828014,4.173674111,-7.485581802));
#132228=CARTESIAN_POINT('Origin',(-0.0199579329223511,4.01786909089896,
0.197026828565895));
#132229=CARTESIAN_POINT('Ctrl Pts',(1.360289621,4.173681702,-7.121243722));
#132230=CARTESIAN_POINT('Ctrl Pts',(0.972223169,4.108088716,-7.195371611));
#132231=CARTESIAN_POINT('Ctrl Pts',(0.578399553,4.042807359,-7.22689103));
#132232=CARTESIAN_POINT('Ctrl Pts',(0.564785654758208,4.04055067932115,
-7.22798060956172));
#132233=CARTESIAN_POINT('Ctrl Pts',(0.551171756516431,4.03829399964222,
-7.22907018912331));
#132234=CARTESIAN_POINT('Ctrl Pts',(1.64863117716287,4.173681702,-7.31709539294683));
#132235=CARTESIAN_POINT('Ctrl Pts',(1.24989194723257,4.108088716,-7.40693622353508));
#132236=CARTESIAN_POINT('Ctrl Pts',(0.843751293891402,4.042807359,-7.4529157718641));
#132237=CARTESIAN_POINT('Ctrl Pts',(0.829711613938738,4.04055067932115,
-7.45450521664782));
#132238=CARTESIAN_POINT('Ctrl Pts',(0.815671933986074,4.03829399964222,
-7.45609466143153));
#132239=CARTESIAN_POINT('',(1.35566157838182,4.17289951177391,-7.12212620752211));
#132240=CARTESIAN_POINT('Origin',(-0.0352634846856975,4.16071259653434,
0.19598567199083));
#132241=CARTESIAN_POINT('Ctrl Pts',(1.40317543510752,4.13354310004224,-7.36757074577745));
#132242=CARTESIAN_POINT('Ctrl Pts',(1.39528843329839,4.13979627446409,-7.32661660577024));
#132243=CARTESIAN_POINT('Ctrl Pts',(1.3873828455856,4.14619777522124,-7.28566543866845));
#132244=CARTESIAN_POINT('Ctrl Pts',(1.37154882246648,4.15930620197364,-7.20386346053619));
#132245=CARTESIAN_POINT('Ctrl Pts',(1.36361158256332,4.1660204136406,-7.16296714596945));
#132246=CARTESIAN_POINT('Ctrl Pts',(1.35566166098924,4.17289950607299,-7.12212619048186));
#132247=CARTESIAN_POINT('Ctrl Pts',(2.12007843989,4.042807359,-6.9305205064));
#132248=CARTESIAN_POINT('Ctrl Pts',(1.74171388206,4.108510123,-7.04626398314));
#132249=CARTESIAN_POINT('Ctrl Pts',(1.35299781883,4.173674111,-7.12012949179001));
#132250=CARTESIAN_POINT('Ctrl Pts',(2.118444839,4.042807359,-6.933591527));
#132251=CARTESIAN_POINT('Ctrl Pts',(1.739912622,4.108510123,-7.049245819));
#132252=CARTESIAN_POINT('Ctrl Pts',(1.351039605,4.173674111,-7.12300442100001));
#132253=CARTESIAN_POINT('Ctrl Pts',(1.95508475,4.042807359,-7.240693587));
#132254=CARTESIAN_POINT('Ctrl Pts',(1.559786616,4.108510123,-7.347429405));
#132255=CARTESIAN_POINT('Ctrl Pts',(1.155218222,4.173674111,-7.41049734200001));
#132256=CARTESIAN_POINT('Origin',(-0.0618462821909793,4.01786907401881,
0.188130101067273));
#132257=CARTESIAN_POINT('Ctrl Pts',(2.859343703,4.173681702,-6.662330943));
#132258=CARTESIAN_POINT('Ctrl Pts',(2.496285335,4.108088716,-6.818148579));
#132259=CARTESIAN_POINT('Ctrl Pts',(2.118444839,4.042807359,-6.933591527));
#132260=CARTESIAN_POINT('Ctrl Pts',(2.1053834537122,4.04055067935632,-6.93758221841224));
#132261=CARTESIAN_POINT('Ctrl Pts',(2.09232206842445,4.03829399971256,-6.94157290982447));
#132262=CARTESIAN_POINT('Ctrl Pts',(3.18304631452949,4.173681702,-6.79161879846189));
#132263=CARTESIAN_POINT('Ctrl Pts',(2.81294250805857,4.108088716,-6.96507634840558));
#132264=CARTESIAN_POINT('Ctrl Pts',(2.42618144212599,4.042807359,-7.09728915532336));
#132265=CARTESIAN_POINT('Ctrl Pts',(2.41281168597241,4.04055067935632,-7.10185955587442));
#132266=CARTESIAN_POINT('Ctrl Pts',(2.3994419298189,4.03829399971257,-7.10642995642561));
#132267=CARTESIAN_POINT('',(2.85501356984558,4.17289951177047,-6.6641876880865));
#132268=CARTESIAN_POINT('Origin',(-0.0765701649059569,4.16071261020573,
0.183823023449187));
#132269=CARTESIAN_POINT('Ctrl Pts',(2.95417989991717,4.13354310002489,-6.89367979482904));
#132270=CARTESIAN_POINT('Ctrl Pts',(2.93767336231485,4.13979627446358,-6.85537861209491));
#132271=CARTESIAN_POINT('Ctrl Pts',(2.92114931248078,4.14619777520393,-6.8170843284045));
#132272=CARTESIAN_POINT('Ctrl Pts',(2.888100472612,4.15930620198082,-6.74059868211742));
#132273=CARTESIAN_POINT('Ctrl Pts',(2.87155730183866,4.16602041376059,-6.70236477214455));
#132274=CARTESIAN_POINT('Ctrl Pts',(2.85501364662232,4.17289950620053,-6.66418765381247));
#132275=CARTESIAN_POINT('Ctrl Pts',(3.56036922856,4.042807359,-6.31273459326));
#132276=CARTESIAN_POINT('Ctrl Pts',(3.21573205004,4.108510123,-6.50710924714));
#132277=CARTESIAN_POINT('Ctrl Pts',(2.85198285308,4.173674111,-6.66281028394001));
#132278=CARTESIAN_POINT('Ctrl Pts',(3.559433999,4.042807359,-6.316084991));
#132279=CARTESIAN_POINT('Ctrl Pts',(3.214613909,4.108510123,-6.510408587));
#132280=CARTESIAN_POINT('Ctrl Pts',(2.850688446,4.173674111,-6.66603895700001));
#132281=CARTESIAN_POINT('Ctrl Pts',(3.465911043,4.042807359,-6.651124765));
#132282=CARTESIAN_POINT('Ctrl Pts',(3.102799805,4.108510123,-6.840342573));
#132283=CARTESIAN_POINT('Ctrl Pts',(2.721247738,4.173674111,-6.988906263));
#132284=CARTESIAN_POINT('Origin',(-0.1008426060641,4.01786904378294,0.170436281909311));
#132285=CARTESIAN_POINT('Ctrl Pts',(4.224698052,4.173681702,-5.891894973));
#132286=CARTESIAN_POINT('Ctrl Pts',(3.903623972,4.108088716,-6.122116497));
#132287=CARTESIAN_POINT('Ctrl Pts',(3.559433999,4.042807359,-6.316084991));
#132288=CARTESIAN_POINT('Ctrl Pts',(3.54753586259605,4.04055067940109,-6.32279019388423));
#132289=CARTESIAN_POINT('Ctrl Pts',(3.53563772619209,4.03829399980212,-6.32949539676845));
#132290=CARTESIAN_POINT('Ctrl Pts',(4.56862574298852,4.173681702,-5.94857365764975));
#132291=CARTESIAN_POINT('Ctrl Pts',(4.24446300427223,4.108088716,-6.19753724418816));
#132292=CARTESIAN_POINT('Ctrl Pts',(3.89516604182199,4.042807359,-6.40980118682287));
#132293=CARTESIAN_POINT('Ctrl Pts',(3.88309136437426,4.0405506794011,-6.4171388362061));
#132294=CARTESIAN_POINT('Ctrl Pts',(3.87101668692651,4.03829399980211,-6.42447648558946));
#132295=CARTESIAN_POINT('',(4.22086836463542,4.1728995063624,-5.89463911385087));
#132296=CARTESIAN_POINT('Origin',(-0.114296549845329,4.16071257439138,0.16306507739361));
#132297=CARTESIAN_POINT('Ctrl Pts',(4.36705019567237,4.13354310002302,-6.09744803842827));
#132298=CARTESIAN_POINT('Ctrl Pts',(4.34269594963005,4.13979627447705,-6.06359073367165));
#132299=CARTESIAN_POINT('Ctrl Pts',(4.31832608394857,4.14619777521901,-6.02974393134162));
#132300=CARTESIAN_POINT('Ctrl Pts',(4.26960775467346,4.15930620202782,-5.96215100045011));
#132301=CARTESIAN_POINT('Ctrl Pts',(4.2452321948314,4.16602041350905,-5.92836727220656));
#132302=CARTESIAN_POINT('Ctrl Pts',(4.22086836934866,4.17289950595936,-5.89463911036402));
#132303=CARTESIAN_POINT('Ctrl Pts',(4.83418110893999,4.042807359,-5.39977222598));
#132304=CARTESIAN_POINT('Ctrl Pts',(4.53938616098,4.108510123,-5.6636893146));
#132305=CARTESIAN_POINT('Ctrl Pts',(4.2176123393,4.173674111,-5.89394547327));
#132306=CARTESIAN_POINT('Ctrl Pts',(4.833987981,4.042807359,-5.40324534));
#132307=CARTESIAN_POINT('Ctrl Pts',(4.539003422,4.108510123,-5.667151885));
#132308=CARTESIAN_POINT('Ctrl Pts',(4.217042264,4.173674111,-5.897376921));
#132309=CARTESIAN_POINT('Ctrl Pts',(4.814675187,4.042807359,-5.750556742));
#132310=CARTESIAN_POINT('Ctrl Pts',(4.500729524,4.108510123,-6.013408925));
#132311=CARTESIAN_POINT('Ctrl Pts',(4.160034734,4.173674111,-6.240521694));
#132312=CARTESIAN_POINT('Origin',(-0.135123824914297,4.0178690631926,0.144773525234887));
#132313=CARTESIAN_POINT('Ctrl Pts',(5.392510215,4.173681702,-4.845960543));
#132314=CARTESIAN_POINT('Ctrl Pts',(5.12843349100001,4.108088716,-5.139821051));
#132315=CARTESIAN_POINT('Ctrl Pts',(4.833987981,4.042807359,-5.40324534));
#132316=CARTESIAN_POINT('Ctrl Pts',(4.82380943690371,4.04055067941645,-5.41235152654575));
#132317=CARTESIAN_POINT('Ctrl Pts',(4.81363089280759,4.03829399983284,-5.4214577130914));
#132318=CARTESIAN_POINT('Ctrl Pts',(5.74058131055242,4.173681702,-4.82737982414742));
#132319=CARTESIAN_POINT('Ctrl Pts',(5.47751712737947,4.108088716,-5.14020818726269));
#132320=CARTESIAN_POINT('Ctrl Pts',(5.182017007808,4.042807359,-5.42259803764837));
#132321=CARTESIAN_POINT('Ctrl Pts',(5.17180200742472,4.04055067941645,-5.43235983549166));
#132322=CARTESIAN_POINT('Ctrl Pts',(5.16158700704133,4.03829399983283,-5.44212163333497));
#132323=CARTESIAN_POINT('',(5.38935991988585,4.17289951176709,-4.84946385508664));
#132324=CARTESIAN_POINT('Origin',(-0.146678535111375,4.16071263738005,0.134682317308428));
#132325=CARTESIAN_POINT('Ctrl Pts',(5.57572207796147,4.13354310000542,-5.01610638889035));
#132326=CARTESIAN_POINT('Ctrl Pts',(5.54465890095454,4.13979627444771,-4.98827609211711));
#132327=CARTESIAN_POINT('Ctrl Pts',(5.51358272710208,4.14619777520086,-4.96045940989693));
#132328=CARTESIAN_POINT('Ctrl Pts',(5.45147292314858,4.15930620201029,-4.9049197648852));
#132329=CARTESIAN_POINT('Ctrl Pts',(5.42040474616916,4.16602041376432,-4.87716590519808));
#132330=CARTESIAN_POINT('Ctrl Pts',(5.38935997551831,4.17289950624065,-4.84946379136899));
#132331=CARTESIAN_POINT('Ctrl Pts',(5.88195205285999,4.042807359,-4.23432251066));
#132332=CARTESIAN_POINT('Ctrl Pts',(5.65078362047,4.108510123,-4.55544156500999));
#132333=CARTESIAN_POINT('Ctrl Pts',(5.38603095943,4.173674111,-4.84948632227001));
#132334=CARTESIAN_POINT('Ctrl Pts',(5.882510057,4.042807359,-4.237755942));
#132335=CARTESIAN_POINT('Ctrl Pts',(5.65115418,4.108510123,-4.55890546));
#132336=CARTESIAN_POINT('Ctrl Pts',(5.386211872,4.173674111,-4.85296009400001));
#132337=CARTESIAN_POINT('Ctrl Pts',(5.938310471,4.042807359,-4.581099076));
#132338=CARTESIAN_POINT('Ctrl Pts',(5.688210133,4.108510123,-4.905294959));
#132339=CARTESIAN_POINT('Ctrl Pts',(5.40430312900001,4.173674111,-5.200337267));
#132340=CARTESIAN_POINT('Origin',(-0.163086559530075,4.01786906831046,0.112341029565017));
#132341=CARTESIAN_POINT('Ctrl Pts',(6.30817459400001,4.173681702,-3.573434383));
#132342=CARTESIAN_POINT('Ctrl Pts',(6.11344316000001,4.108088716,-3.917193286));
#132343=CARTESIAN_POINT('Ctrl Pts',(5.882510057,4.042807359,-4.237755942));
#132344=CARTESIAN_POINT('Ctrl Pts',(5.87452704205408,4.04055067928692,-4.24883731769155));
#132345=CARTESIAN_POINT('Ctrl Pts',(5.86654402710806,4.03829399957376,-4.25991869338303));
#132346=CARTESIAN_POINT('Ctrl Pts',(6.64411367476263,4.173681702,-3.48046307510273));
#132347=CARTESIAN_POINT('Ctrl Pts',(6.45444863851461,4.108088716,-3.84252870800095));
#132348=CARTESIAN_POINT('Ctrl Pts',(6.22656261649925,4.042807359,-4.18184023157307));
#132349=CARTESIAN_POINT('Ctrl Pts',(6.21868493462476,4.04055067928692,-4.19356972781599));
#132350=CARTESIAN_POINT('Ctrl Pts',(6.21080725275035,4.03829399957376,-4.20529922405897));
#132351=CARTESIAN_POINT('',(6.30585109886971,4.17289950635719,-3.5775329418795));
#132352=CARTESIAN_POINT('Origin',(-0.172201855024702,4.1607126089196,0.100001893504828));
#132353=CARTESIAN_POINT('Ctrl Pts',(6.52367939274731,4.13354309997313,-3.7002171795232));
#132354=CARTESIAN_POINT('Ctrl Pts',(6.48735976437488,4.13979627442715,-3.67971520436029));
#132355=CARTESIAN_POINT('Ctrl Pts',(6.45103036979152,4.14619777517902,-3.65922931941917));
#132356=CARTESIAN_POINT('Ctrl Pts',(6.37843327653972,4.15930620198339,-3.61833993218304));
#132357=CARTESIAN_POINT('Ctrl Pts',(6.34212519835251,4.16602041343716,-3.59791368279754));
#132358=CARTESIAN_POINT('Ctrl Pts',(6.30585110154139,4.17289950588202,-3.577532936964));
#132359=CARTESIAN_POINT('Ctrl Pts',(6.65468945644,4.042807359,-2.87088058177));
#132360=CARTESIAN_POINT('Ctrl Pts',(6.49795671792,4.108510123,-3.23418643029));
#132361=CARTESIAN_POINT('Ctrl Pts',(6.30260475782,4.173674111,-3.57827058098));
#132362=CARTESIAN_POINT('Ctrl Pts',(6.655972501,4.042807359,-2.874113787));
#132363=CARTESIAN_POINT('Ctrl Pts',(6.499063249,4.108510123,-3.237489682));
#132364=CARTESIAN_POINT('Ctrl Pts',(6.303528199,4.173674111,-3.581624247));
#132365=CARTESIAN_POINT('Ctrl Pts',(6.784276957,4.042807359,-3.19743431));
#132366=CARTESIAN_POINT('Ctrl Pts',(6.609716357,4.108510123,-3.567814853));
#132367=CARTESIAN_POINT('Ctrl Pts',(6.395872317,4.173674111,-3.916990849));
#132368=CARTESIAN_POINT('Origin',(-0.183423764448718,4.0178690710966,0.0746558063975883));
#132369=CARTESIAN_POINT('Ctrl Pts',(6.92887574,4.173681702,-2.133818404));
#132370=CARTESIAN_POINT('Ctrl Pts',(6.812595022,4.108088716,-2.511401917));
#132371=CARTESIAN_POINT('Ctrl Pts',(6.655972501,4.042807359,-2.874113787));
#132372=CARTESIAN_POINT('Ctrl Pts',(6.65055829288174,4.0405506793681,-2.88665219807012));
#132373=CARTESIAN_POINT('Ctrl Pts',(6.64514408476364,4.03829399973613,-2.89919060914025));
#132374=CARTESIAN_POINT('Ctrl Pts',(7.23697466922762,4.173681702,-1.97080374093111));
#132375=CARTESIAN_POINT('Ctrl Pts',(7.1295773034183,4.108088716,-2.36517685756169));
#132376=CARTESIAN_POINT('Ctrl Pts',(6.97996107817811,4.042807359,-2.74554422463711));
#132377=CARTESIAN_POINT('Ctrl Pts',(6.97478906730675,4.0405506793681,-2.7586929600398));
#132378=CARTESIAN_POINT('Ctrl Pts',(6.96961705643524,4.03829399973613,-2.77184169544254));
#132379=CARTESIAN_POINT('',(6.92748761210297,4.17289951179661,-2.13832069848568));
#132380=CARTESIAN_POINT('Origin',(-0.189673230629527,4.16071259632617,0.0606455671723691));
#132381=CARTESIAN_POINT('Ctrl Pts',(7.16659670980132,4.13354310001635,-2.211309927262));
#132382=CARTESIAN_POINT('Ctrl Pts',(7.12671889557544,4.13979627446342,-2.19909492345641));
#132383=CARTESIAN_POINT('Ctrl Pts',(7.08683500233852,4.14619777522031,-2.18689773310916));
#132384=CARTESIAN_POINT('Ctrl Pts',(7.00714517929606,4.1593062020332,-2.16257054614862));
#132385=CARTESIAN_POINT('Ctrl Pts',(6.96729492228005,4.16602041379438,-2.15042701411706));
#132386=CARTESIAN_POINT('Ctrl Pts',(6.92748763585173,4.17289950626471,-2.13832061725355));
#132387=CARTESIAN_POINT('Ctrl Pts',(7.11626097776,4.042807359,-1.37319946697));
#132388=CARTESIAN_POINT('Ctrl Pts',(7.04129258152,4.108510123,-1.76170433195));
#132389=CARTESIAN_POINT('Ctrl Pts',(6.92447576331001,4.173674111,-2.13973888338));
#132390=CARTESIAN_POINT('Ctrl Pts',(7.118209069,4.042807359,-1.376081265));
#132391=CARTESIAN_POINT('Ctrl Pts',(7.043083344,4.108510123,-1.764692484));
#132392=CARTESIAN_POINT('Ctrl Pts',(6.926098554,4.173674111,-2.14281563));
#132393=CARTESIAN_POINT('Ctrl Pts',(7.313018193,4.042807359,-1.664261068));
#132394=CARTESIAN_POINT('Ctrl Pts',(7.222159592,4.108510123,-2.063507689));
#132395=CARTESIAN_POINT('Ctrl Pts',(7.08837762300001,4.173674111,-2.450490292));
#132396=CARTESIAN_POINT('Origin',(-0.19518439295879,4.01786909364984,0.0334797583197854));
#132397=CARTESIAN_POINT('Ctrl Pts',(7.225590357,4.173681702,-0.594427447));
#132398=CARTESIAN_POINT('Ctrl Pts',(7.193197511,4.108088716,-0.988180185000001));
#132399=CARTESIAN_POINT('Ctrl Pts',(7.118209069,4.042807359,-1.376081265));
#132400=CARTESIAN_POINT('Ctrl Pts',(7.11561682978209,4.0405506793131,-1.38949043000508));
#132401=CARTESIAN_POINT('Ctrl Pts',(7.11302459056408,4.03829399962612,-1.40289959501017));
#132402=CARTESIAN_POINT('Ctrl Pts',(7.49144277026395,4.173681702,-0.368991814859853));
#132403=CARTESIAN_POINT('Ctrl Pts',(7.47133485840943,4.108088716,-0.777231965446189));
#132404=CARTESIAN_POINT('Ctrl Pts',(7.40698431742471,4.042807359,-1.18086962076656));
#132405=CARTESIAN_POINT('Ctrl Pts',(7.40475981466687,4.0405506793131,-1.19482277584016));
#132406=CARTESIAN_POINT('Ctrl Pts',(7.40253531190902,4.03829399962611,-1.20877593091373));
#132407=CARTESIAN_POINT('',(7.22520254318857,4.17289951177379,-0.599122887178798));
#132408=CARTESIAN_POINT('Origin',(-0.198275918900978,4.16071258780606,0.0184535848791907));
#132409=CARTESIAN_POINT('Ctrl Pts',(7.47441192954827,4.13354310003169,-0.619004280640486));
#132410=CARTESIAN_POINT('Ctrl Pts',(7.432840571704,4.13979627447792,-0.615647408031067));
#132411=CARTESIAN_POINT('Ctrl Pts',(7.3912671063394,4.14619777523392,-0.612309239198264));
#132412=CARTESIAN_POINT('Ctrl Pts',(7.30821076097249,4.15930620204402,-0.60568176445075));
#132413=CARTESIAN_POINT('Ctrl Pts',(7.26668168060823,4.16602041376777,-0.602388768625244));
#132414=CARTESIAN_POINT('Ctrl Pts',(7.22520254895009,4.17289950623539,-0.599122802339564));
#132415=CARTESIAN_POINT('Ctrl Pts',(7.24508404466,4.042807359,0.18869092816));
#132416=CARTESIAN_POINT('Ctrl Pts',(7.25538543020001,4.108510123,-0.20684689829));
#132417=CARTESIAN_POINT('Ctrl Pts',(7.22256597768,4.173674111,-0.601155374030001));
#132418=CARTESIAN_POINT('Ctrl Pts',(7.247606092,4.042807359,0.186295287));
#132419=CARTESIAN_POINT('Ctrl Pts',(7.25777669,4.108510123,-0.209380228));
#132420=CARTESIAN_POINT('Ctrl Pts',(7.22481223800001,4.173674111,-0.603811336000001));
#132421=CARTESIAN_POINT('Ctrl Pts',(7.49981082600001,4.042807359,-0.053268829));
#132422=CARTESIAN_POINT('Ctrl Pts',(7.49690267000001,4.108510123,-0.462713199));
#132423=CARTESIAN_POINT('Ctrl Pts',(7.44943827000001,4.173674111,-0.869407533));
#132424=CARTESIAN_POINT('Origin',(-0.197818151014114,4.01786906839711,-0.00926186170131144));
#132425=CARTESIAN_POINT('Ctrl Pts',(7.1844444,4.173681702,0.972758276));
#132426=CARTESIAN_POINT('Ctrl Pts',(7.23745408,4.108088716,0.581247754));
#132427=CARTESIAN_POINT('Ctrl Pts',(7.247606092,4.042807359,0.186295287));
#132428=CARTESIAN_POINT('Ctrl Pts',(7.24795703198754,4.04055067937703,0.172642366391681));
#132429=CARTESIAN_POINT('Ctrl Pts',(7.24830797197519,4.038293999754,0.158989445783361));
#132430=CARTESIAN_POINT('Ctrl Pts',(7.39561933502162,4.173681702,1.25007375973637));
#132431=CARTESIAN_POINT('Ctrl Pts',(7.46374109865901,4.108088716,0.847055430001624));
#132432=CARTESIAN_POINT('Ctrl Pts',(7.48766520227535,4.042807359,0.439021134686341));
#132433=CARTESIAN_POINT('Ctrl Pts',(7.48849222302995,4.04055067937703,0.424915994688794));
#132434=CARTESIAN_POINT('Ctrl Pts',(7.48931924378469,4.038293999754,0.410810854691255));
#132435=CARTESIAN_POINT('',(7.18507502384416,4.17289950633231,0.968089322403721));
#132436=CARTESIAN_POINT('Origin',(-0.197607384198897,4.16071259388392,-0.0246013163387804));
#132437=CARTESIAN_POINT('Ctrl Pts',(7.4327319551077,4.13354309998286,1.00224531859311));
#132438=CARTESIAN_POINT('Ctrl Pts',(7.39141088416451,4.13979627442906,0.996587096134489));
#132439=CARTESIAN_POINT('Ctrl Pts',(7.35009177569022,4.14619777518784,0.990910154106153));
#132440=CARTESIAN_POINT('Ctrl Pts',(7.2675525304276,4.15930620198021,0.979528022672306));
#132441=CARTESIAN_POINT('Ctrl Pts',(7.22628648180661,4.16602041341854,0.973816505420604));
#132442=CARTESIAN_POINT('Ctrl Pts',(7.18507502301303,4.17289950585988,0.968089327816833));
#132443=CARTESIAN_POINT('Ctrl Pts',(7.03513503368,4.042807359,1.74175834578));
#132444=CARTESIAN_POINT('Ctrl Pts',(7.13022451851,4.108510123,1.3576824667));
#132445=CARTESIAN_POINT('Ctrl Pts',(7.18293703368,4.173674111,0.965537491470001));
#132446=CARTESIAN_POINT('Ctrl Pts',(7.038113109,4.042807359,1.739960879));
#132447=CARTESIAN_POINT('Ctrl Pts',(7.133104463,4.108510123,1.355722415));
#132448=CARTESIAN_POINT('Ctrl Pts',(7.18570173100001,4.173674111,0.963426504000001));
#132449=CARTESIAN_POINT('Ctrl Pts',(7.335920641,4.042807359,1.560214201));
#132450=CARTESIAN_POINT('Ctrl Pts',(7.421098912,4.108510123,1.159717245));
#132451=CARTESIAN_POINT('Ctrl Pts',(7.462171463,4.173674111,0.752327757));
#132452=CARTESIAN_POINT('Origin',(-0.191202134330626,4.01786908337155,-0.0515703590211958));
#132453=CARTESIAN_POINT('Ctrl Pts',(6.807361808,4.173681702,2.494458903));
#132454=CARTESIAN_POINT('Ctrl Pts',(6.94329534,4.108088716,2.123497195));
#132455=CARTESIAN_POINT('Ctrl Pts',(7.038113109,4.042807359,1.739960879));
#132456=CARTESIAN_POINT('Ctrl Pts',(7.04139081861473,4.04055067933166,1.72670259752172));
#132457=CARTESIAN_POINT('Ctrl Pts',(7.04466852822935,4.03829399966326,1.71344431604344));
#132458=CARTESIAN_POINT('Ctrl Pts',(6.95398495829392,4.173681702,2.81068727388919));
#132459=CARTESIAN_POINT('Ctrl Pts',(7.10715110139243,4.108088716,2.43173545453254));
#132460=CARTESIAN_POINT('Ctrl Pts',(7.21823118476982,4.042807359,2.03838374951113));
#132461=CARTESIAN_POINT('Ctrl Pts',(7.22207105846783,4.04055067933166,2.02478616459523));
#132462=CARTESIAN_POINT('Ctrl Pts',(7.22591093216596,4.03829399966326,2.01118857967941));
#132463=CARTESIAN_POINT('',(6.80898137486375,4.1728995063478,2.49003467242114));
#132464=CARTESIAN_POINT('Origin',(-0.187698734055647,4.16071265495012,-0.0665058597055171));
#132465=CARTESIAN_POINT('Ctrl Pts',(7.04350569533256,4.13354309996481,2.57663104013005));
#132466=CARTESIAN_POINT('Ctrl Pts',(7.00436703867137,4.13979627440061,2.56222229503698));
#132467=CARTESIAN_POINT('Ctrl Pts',(6.96523432263822,4.1461977751729,2.54779568983075));
#132468=CARTESIAN_POINT('Ctrl Pts',(6.88707162095704,4.15930620196764,2.51893616842301));
#132469=CARTESIAN_POINT('Ctrl Pts',(6.8479981567205,4.16602041347153,2.50448720246409));
#132470=CARTESIAN_POINT('Ctrl Pts',(6.8089813728981,4.17289950593006,2.49003467752891));
#132471=CARTESIAN_POINT('Ctrl Pts',(6.49623092821,4.042807359,3.21338307884));
#132472=CARTESIAN_POINT('Ctrl Pts',(6.67166223484,4.108510123,2.85872810885));
#132473=CARTESIAN_POINT('Ctrl Pts',(6.80744193786,4.173674111,2.48708289756));
#132474=CARTESIAN_POINT('Ctrl Pts',(6.49952578,4.042807359,3.212267834));
#132475=CARTESIAN_POINT('Ctrl Pts',(6.674896201,4.108510123,2.857432985));
#132476=CARTESIAN_POINT('Ctrl Pts',(6.810595798,4.173674111,2.485615592));
#132477=CARTESIAN_POINT('Ctrl Pts',(6.829010959,4.042807359,3.10074335));
#132478=CARTESIAN_POINT('Ctrl Pts',(6.998292817,4.108510123,2.7279206));
#132479=CARTESIAN_POINT('Ctrl Pts',(7.125981812,4.173674111,2.338885036));
#132480=CARTESIAN_POINT('Origin',(-0.175646128157292,4.01786907295784,-0.0914676050620089));
#132481=CARTESIAN_POINT('Ctrl Pts',(6.111974543,4.173681702,3.899521405));
#132482=CARTESIAN_POINT('Ctrl Pts',(6.324475827,4.108088716,3.566454266));
#132483=CARTESIAN_POINT('Ctrl Pts',(6.49952578,4.042807359,3.212267834));
#132484=CARTESIAN_POINT('Ctrl Pts',(6.5055769970589,4.04055067938178,3.20002413474375));
#132485=CARTESIAN_POINT('Ctrl Pts',(6.51162821411791,4.0382939997635,3.18778043548744));
#132486=CARTESIAN_POINT('Ctrl Pts',(6.18718997383367,4.173681702,4.23987617474425));
#132487=CARTESIAN_POINT('Ctrl Pts',(6.41823861690002,4.108088716,3.90271023113911));
#132488=CARTESIAN_POINT('Ctrl Pts',(6.61128069909999,4.042807359,3.54243380476379));
#132489=CARTESIAN_POINT('Ctrl Pts',(6.61795387736068,4.04055067938178,3.529979583441));
#132490=CARTESIAN_POINT('Ctrl Pts',(6.62462705562136,4.0382939997635,3.51752536211824));
#132491=CARTESIAN_POINT('',(6.11450736626476,4.17289951176952,3.89554870260983));
#132492=CARTESIAN_POINT('Origin',(-0.169013702511757,4.16071260599231,-0.105300696633516));
#132493=CARTESIAN_POINT('Ctrl Pts',(6.32493293725509,4.13354310001343,4.030536358256));
#132494=CARTESIAN_POINT('Ctrl Pts',(6.28980677482503,4.13979627446321,4.00805082736618));
#132495=CARTESIAN_POINT('Ctrl Pts',(6.25469025369967,4.14619777521526,3.98554913111775));
#132496=CARTESIAN_POINT('Ctrl Pts',(6.18455889639565,4.1593062020154,3.94056165900709));
#132497=CARTESIAN_POINT('Ctrl Pts',(6.14950504726379,4.16602041375794,3.91805086130808));
#132498=CARTESIAN_POINT('Ctrl Pts',(6.11450731972724,4.17289950620169,3.89554877328798));
#132499=CARTESIAN_POINT('Ctrl Pts',(5.65357028333,4.042807359,4.53475359029));
#132500=CARTESIAN_POINT('Ctrl Pts',(5.90114043883001,4.108510123,4.22610280245));
#132501=CARTESIAN_POINT('Ctrl Pts',(6.11363842303001,4.173674111,3.89233507207));
#132502=CARTESIAN_POINT('Ctrl Pts',(5.657027848,4.042807359,4.534372715));
#132503=CARTESIAN_POINT('Ctrl Pts',(5.90457721,4.108510123,4.225533165));
#132504=CARTESIAN_POINT('Ctrl Pts',(6.117033975,4.173674111,3.891580058));
#132505=CARTESIAN_POINT('Ctrl Pts',(6.002784315,4.042807359,4.496285186));
#132506=CARTESIAN_POINT('Ctrl Pts',(6.24825432699999,4.108510123,4.16856942));
#132507=CARTESIAN_POINT('Ctrl Pts',(6.45658917200001,4.173674111,3.816078651));
#132508=CARTESIAN_POINT('Origin',(-0.151876743933352,4.01786908548743,-0.127087835198143));
#132509=CARTESIAN_POINT('Ctrl Pts',(5.13079814199999,4.173681702,5.122246619));
#132510=CARTESIAN_POINT('Ctrl Pts',(5.409930853,4.108088716,4.8426479));
#132511=CARTESIAN_POINT('Ctrl Pts',(5.657027848,4.042807359,4.534372715));
#132512=CARTESIAN_POINT('Ctrl Pts',(5.66556962431573,4.04055067939498,4.52371609947151));
#132513=CARTESIAN_POINT('Ctrl Pts',(5.67411140063149,4.03829399978988,4.51305948394299));
#132514=CARTESIAN_POINT('Ctrl Pts',(5.13108886245636,4.173681702,5.47081317818954));
#132515=CARTESIAN_POINT('Ctrl Pts',(5.42921642824447,4.108088716,5.19119861552039));
#132516=CARTESIAN_POINT('Ctrl Pts',(5.69519407555069,4.042807359,4.88084359396338));
#132517=CARTESIAN_POINT('Ctrl Pts',(5.70438852798938,4.04055067939498,4.87011508157252));
#132518=CARTESIAN_POINT('Ctrl Pts',(5.71358298042812,4.03829399978988,4.85938656918154));
#132519=CARTESIAN_POINT('',(5.13412576263134,4.17289951176391,5.11891127869527));
#132520=CARTESIAN_POINT('Origin',(-0.142425679370615,4.16071261417797,-0.139171734135627));
#132521=CARTESIAN_POINT('Ctrl Pts',(5.31061334460018,4.13354310000474,5.29597827577731));
#132522=CARTESIAN_POINT('Ctrl Pts',(5.28114213686151,4.13979627444847,5.26646735746395));
#132523=CARTESIAN_POINT('Ctrl Pts',(5.25168382007216,4.1461977752049,5.23694272427037));
#132524=CARTESIAN_POINT('Ctrl Pts',(5.19286307176349,4.15930620201472,5.17793086538721));
#132525=CARTESIAN_POINT('Ctrl Pts',(5.16346791838434,4.16602041375355,5.14841081626259));
#132526=CARTESIAN_POINT('Ctrl Pts',(5.13412570209188,4.17289950622626,5.11891133762066));
#132527=CARTESIAN_POINT('Ctrl Pts',(4.54655497634,4.042807359,5.64408406444999));
#132528=CARTESIAN_POINT('Ctrl Pts',(4.85468787541999,4.108510123,5.39586962442));
#132529=CARTESIAN_POINT('Ctrl Pts',(5.13396797045,4.173674111,5.11558598396));
#132530=CARTESIAN_POINT('Ctrl Pts',(4.550013582,4.042807359,5.644455368));
#132531=CARTESIAN_POINT('Ctrl Pts',(4.858166752,4.108510123,5.396052109));
#132532=CARTESIAN_POINT('Ctrl Pts',(5.137446442,4.173674111,5.115578565));
#132533=CARTESIAN_POINT('Ctrl Pts',(4.895874148,4.042807359,5.681585723));
#132534=CARTESIAN_POINT('Ctrl Pts',(5.20605441,4.108510123,5.414300567));
#132535=CARTESIAN_POINT('Ctrl Pts',(5.485293597,4.173674111,5.114836669));
#132536=CARTESIAN_POINT('Origin',(-0.121005699289965,4.01786904130105,-0.156765469005895));
#132537=CARTESIAN_POINT('Ctrl Pts',(3.909711322,4.173681702,6.105461275));
#132538=CARTESIAN_POINT('Ctrl Pts',(4.242423525,4.108088716,5.89240469999999));
#132539=CARTESIAN_POINT('Ctrl Pts',(4.550013582,4.042807359,5.644455368));
#132540=CARTESIAN_POINT('Ctrl Pts',(4.56064651363442,4.04055067940265,5.63588412768856));
#132541=CARTESIAN_POINT('Ctrl Pts',(4.57127944526878,4.03829399980524,5.62731288737714));
#132542=CARTESIAN_POINT('Ctrl Pts',(3.83506373905209,4.173681702,6.4459410374688));
#132543=CARTESIAN_POINT('Ctrl Pts',(4.18633011316431,4.108088716,6.23695232226666));
#132544=CARTESIAN_POINT('Ctrl Pts',(4.51280650719211,4.042807359,5.99103056005124));
#132545=CARTESIAN_POINT('Ctrl Pts',(4.52409231145965,4.04055067940265,5.98252940981719));
#132546=CARTESIAN_POINT('Ctrl Pts',(4.53537811572727,4.03829399980525,5.97402825958322));
#132547=CARTESIAN_POINT('',(3.91367807798151,4.17289950635246,6.10291929574919));
#132548=CARTESIAN_POINT('Origin',(-0.10917812640765,4.16071260748246,-0.166535413895311));
#132549=CARTESIAN_POINT('Ctrl Pts',(4.04797537441707,4.13354309997486,6.31378613519414));
#132550=CARTESIAN_POINT('Ctrl Pts',(4.02553716221962,4.13979627442888,6.27862972721912));
#132551=CARTESIAN_POINT('Ctrl Pts',(4.00311448798317,4.14619777516769,6.24346269633418));
#132552=CARTESIAN_POINT('Ctrl Pts',(3.95835474138069,4.15930620198404,6.1731857797458));
#132553=CARTESIAN_POINT('Ctrl Pts',(3.93599276900521,4.16602041351721,6.13803680496813));
#132554=CARTESIAN_POINT('Ctrl Pts',(3.91367807337261,4.17289950597883,6.10291929860463));
#132555=CARTESIAN_POINT('Ctrl Pts',(3.22694781191,4.042807359,6.48950344034));
#132556=CARTESIAN_POINT('Ctrl Pts',(3.5812355014,4.108510123,6.31333158117999));
#132557=CARTESIAN_POINT('Ctrl Pts',(3.91423888132,4.173674111,6.09963778095));
#132558=CARTESIAN_POINT('Ctrl Pts',(3.230245738,4.042807359,6.490609561));
#132559=CARTESIAN_POINT('Ctrl Pts',(3.584593815,4.108510123,6.314257655));
#132560=CARTESIAN_POINT('Ctrl Pts',(3.917637623,4.173674111,6.100378304));
#132561=CARTESIAN_POINT('Ctrl Pts',(3.560038347,4.042807359,6.601221627));
#132562=CARTESIAN_POINT('Ctrl Pts',(3.920425175,4.108510123,6.406865037));
#132563=CARTESIAN_POINT('Ctrl Pts',(4.25751179100001,4.173674111,6.174430609));
#132564=CARTESIAN_POINT('Origin',(-0.0844766574966155,4.01786906872095,
-0.179112931320975));
#132565=CARTESIAN_POINT('Ctrl Pts',(2.505810746,4.173681702,6.803191347));
#132566=CARTESIAN_POINT('Ctrl Pts',(2.876545188,4.108088716,6.66663920500001));
#132567=CARTESIAN_POINT('Ctrl Pts',(3.230245738,4.042807359,6.490609561));
#132568=CARTESIAN_POINT('Ctrl Pts',(3.2424726411516,4.04055067936057,6.48452447742013));
#132569=CARTESIAN_POINT('Ctrl Pts',(3.25469954430317,4.03829399972108,6.47843939384023));
#132570=CARTESIAN_POINT('Ctrl Pts',(2.35971529781498,4.173681702,7.11966385829063));
#132571=CARTESIAN_POINT('Ctrl Pts',(2.74769565534635,4.108088716,6.99107307035044));
#132572=CARTESIAN_POINT('Ctrl Pts',(3.11940512216221,4.042807359,6.82108359598885));
#132573=CARTESIAN_POINT('Ctrl Pts',(3.13225456684441,4.04055067936057,6.81520731211027));
#132574=CARTESIAN_POINT('Ctrl Pts',(3.14510401152666,4.03829399972108,6.80933102823169));
#132575=CARTESIAN_POINT('',(2.51023128580415,4.1728995117299,6.80156150582057));
#132576=CARTESIAN_POINT('Origin',(-0.0708253644546503,4.16071265875346,
-0.186111902591437));
#132577=CARTESIAN_POINT('Ctrl Pts',(2.59605857474129,4.13354310001904,7.03636837218138));
#132578=CARTESIAN_POINT('Ctrl Pts',(2.58170254394118,4.13979627446724,6.99721034916009));
#132579=CARTESIAN_POINT('Ctrl Pts',(2.56736397139921,4.14619777521901,6.95804529166872));
#132580=CARTESIAN_POINT('Ctrl Pts',(2.53875814241895,4.15930620203028,6.87978938791505));
#132581=CARTESIAN_POINT('Ctrl Pts',(2.52447497067071,4.16602041375511,6.84065501247579));
#132582=CARTESIAN_POINT('Ctrl Pts',(2.51023120599506,4.1728995062256,6.80156153393056));
#132583=CARTESIAN_POINT('Ctrl Pts',(1.75645215384,4.042807359,7.03148084821));
#132584=CARTESIAN_POINT('Ctrl Pts',(2.14032853641,4.108510123,6.93558916912));
#132585=CARTESIAN_POINT('Ctrl Pts',(2.51148433258,4.173674111,6.79847729497001));
#132586=CARTESIAN_POINT('Ctrl Pts',(1.759435193,4.042807359,7.033270065));
#132587=CARTESIAN_POINT('Ctrl Pts',(2.143409256,4.108510123,6.93721553));
#132588=CARTESIAN_POINT('Ctrl Pts',(2.514644423,4.173674111,6.79993113400001));
#132589=CARTESIAN_POINT('Ctrl Pts',(2.057739109,4.042807359,7.212191744));
#132590=CARTESIAN_POINT('Ctrl Pts',(2.451481215,4.108510123,7.099851618));
#132591=CARTESIAN_POINT('Ctrl Pts',(2.830653465,4.173674111,6.945315037));
#132592=CARTESIAN_POINT('Origin',(-0.0439977612037606,4.01786909908604,
-0.193085675719032));
#132593=CARTESIAN_POINT('Ctrl Pts',(0.984741244,4.173681702,7.182811753));
#132594=CARTESIAN_POINT('Ctrl Pts',(1.376162796,4.108088716,7.129149071));
#132595=CARTESIAN_POINT('Ctrl Pts',(1.759435193,4.042807359,7.033270065));
#132596=CARTESIAN_POINT('Ctrl Pts',(1.77268435110923,4.04055067934542,7.02995567001672));
#132597=CARTESIAN_POINT('Ctrl Pts',(1.78593350921839,4.03829399969076,7.02664127503343));
#132598=CARTESIAN_POINT('Ctrl Pts',(0.77402919142123,4.173681702,7.4604791102965));
#132599=CARTESIAN_POINT('Ctrl Pts',(1.18058200259842,4.108088716,7.41829901202046));
#132600=CARTESIAN_POINT('Ctrl Pts',(1.5801438198671,4.042807359,7.3321903451503));
#132601=CARTESIAN_POINT('Ctrl Pts',(1.59395607906664,4.04055067934542,7.32921369629466));
#132602=CARTESIAN_POINT('Ctrl Pts',(1.60776833826625,4.03829399969076,7.32623704743884));
#132603=CARTESIAN_POINT('',(0.989408801939575,4.17289951177892,7.18217030221119));
#132604=CARTESIAN_POINT('Origin',(-0.0291609472063403,4.16071258635768,
-0.196986017737631));
#132605=CARTESIAN_POINT('Ctrl Pts',(1.02275296161709,4.13354310000798,7.42993784453988));
#132606=CARTESIAN_POINT('Ctrl Pts',(1.01715038425056,4.13979627445525,7.3886091920938));
#132607=CARTESIAN_POINT('Ctrl Pts',(1.01156636914356,4.14619777522442,7.34727742251048));
#132608=CARTESIAN_POINT('Ctrl Pts',(1.00045203447617,4.1593062020231,7.26470169062957));
#132609=CARTESIAN_POINT('Ctrl Pts',(0.994915529196611,4.1660204137004,7.22341179562296));
#132610=CARTESIAN_POINT('Ctrl Pts',(0.989408718002346,4.17289950615059,
7.18217031248019));
#132611=CARTESIAN_POINT('Ctrl Pts',(0.20382674536,4.042807359,7.24467402586));
#132612=CARTESIAN_POINT('Ctrl Pts',(0.59934218743,4.108510123,7.23354631689));
#132613=CARTESIAN_POINT('Ctrl Pts',(0.991295567150001,4.173674111,7.17942756589));
#132614=CARTESIAN_POINT('Ctrl Pts',(0.206355414,4.042807359,7.247062677));
#132615=CARTESIAN_POINT('Ctrl Pts',(0.602001262,4.108510123,7.235796918));
#132616=CARTESIAN_POINT('Ctrl Pts',(0.994069244,4.173674111,7.181526741));
#132617=CARTESIAN_POINT('Ctrl Pts',(0.459222278,4.042807359,7.485927791));
#132618=CARTESIAN_POINT('Ctrl Pts',(0.867908719,4.108510123,7.460857029));
#132619=CARTESIAN_POINT('Ctrl Pts',(1.271436929,4.173674111,7.39144425200001));
#132620=CARTESIAN_POINT('Origin',(-0.00146140008758431,4.01786907736225,
-0.19802964222655));
#132621=CARTESIAN_POINT('Ctrl Pts',(-0.579724377070001,4.173681702,7.22431773469001));
#132622=CARTESIAN_POINT('Ctrl Pts',(-0.18604099109,4.108088716,7.25590934798001));
#132623=CARTESIAN_POINT('Ctrl Pts',(0.20874406514,4.042807359,7.24453400836));
#132624=CARTESIAN_POINT('Ctrl Pts',(0.222391198647374,4.04055067937027,
7.2441407797511));
#132625=CARTESIAN_POINT('Ctrl Pts',(0.236038332154748,4.03829399974047,
7.24374755114209));
#132626=CARTESIAN_POINT('Ctrl Pts',(-0.582373663,4.173681702,7.22657186500001));
#132627=CARTESIAN_POINT('Ctrl Pts',(-0.18856744,4.108088716,7.25830784900001));
#132628=CARTESIAN_POINT('Ctrl Pts',(0.206355414,4.042807359,7.247062677));
#132629=CARTESIAN_POINT('Ctrl Pts',(0.220007310971782,4.04055067937027,
7.24667394809255));
#132630=CARTESIAN_POINT('Ctrl Pts',(0.233659207943565,4.03829399974047,
7.24628521918494));
#132631=CARTESIAN_POINT('Ctrl Pts',(-0.847849659089798,4.173681702,7.45245065089739));
#132632=CARTESIAN_POINT('Ctrl Pts',(-0.441734353150908,4.108088716,7.49865353618934));
#132633=CARTESIAN_POINT('Ctrl Pts',(-0.0330032499787613,4.042807359,7.50045202179791));
#132634=CARTESIAN_POINT('Ctrl Pts',(-0.0188740223254308,4.04055067937027,
7.50051419277634));
#132635=CARTESIAN_POINT('Ctrl Pts',(-0.00474479467210093,4.03829399974047,
7.50057636375477));
#132636=CARTESIAN_POINT('Origin',(0.0138668838850882,4.16071273333814,-0.198651015243198));
#132637=CARTESIAN_POINT('Ctrl Pts',(0.213507122,1.715323387,7.246855505));
#132638=CARTESIAN_POINT('Ctrl Pts',(0.605805226,1.779910221,7.235297604));
#132639=CARTESIAN_POINT('Ctrl Pts',(0.994563149000001,1.845052736,7.181458358));
#132640=CARTESIAN_POINT('Ctrl Pts',(0.466609588000001,1.715323387,7.48547096));
#132641=CARTESIAN_POINT('Ctrl Pts',(0.871824797,1.779910221,7.460211721));
#132642=CARTESIAN_POINT('Ctrl Pts',(1.27194527,1.845052736,7.391356792));
#132643=CARTESIAN_POINT('',(0.466609584806905,1.71532338744763,7.48547096129464));
#132644=CARTESIAN_POINT('',(1.0255415441568,1.80506741731045,7.42955345467621));
#132645=CARTESIAN_POINT('Origin',(-0.0371219255234506,1.87497458960283,
-0.186844580707713));
#132646=CARTESIAN_POINT('Ctrl Pts',(0.989922562716042,1.84427517372254,
7.18209950661362));
#132647=CARTESIAN_POINT('Ctrl Pts',(0.995813103391253,1.83740483626466,
7.22328556358072));
#132648=CARTESIAN_POINT('Ctrl Pts',(1.00173105596826,1.83070797850139,7.26452308862856));
#132649=CARTESIAN_POINT('Ctrl Pts',(1.01360302452397,1.81765000112593,7.34699349044738));
#132650=CARTESIAN_POINT('Ctrl Pts',(1.01956408258325,1.81128114572236,7.38827527131803));
#132651=CARTESIAN_POINT('Ctrl Pts',(1.02554154127133,1.8050674173951,7.4295534551068));
#132652=CARTESIAN_POINT('',(0.340058346905326,1.71532338829773,7.36616323287369));
#132653=CARTESIAN_POINT('Origin',(-6.84673671924596E-14,1.80614392400061,
1.4658413372004E-13));
#132654=CARTESIAN_POINT('',(1.0294825429089,1.6256495872185,7.42900839215824));
#132655=CARTESIAN_POINT('Origin',(-0.0480202436087657,1.48225709598333,
-0.179766005105065));
#132656=CARTESIAN_POINT('',(1.58774795233212,1.71532338734617,7.33001067177152));
#132657=CARTESIAN_POINT('Origin',(-0.0635989656301628,1.87485301774001,
-0.1735270144933));
#132658=CARTESIAN_POINT('Ctrl Pts',(1.0255415464473,1.80506741659162,7.42955345421685));
#132659=CARTESIAN_POINT('Ctrl Pts',(1.14143634970523,1.78658581162503,7.41355586629499));
#132660=CARTESIAN_POINT('Ctrl Pts',(1.25671458271972,1.76822051520836,7.39487847462538));
#132661=CARTESIAN_POINT('Ctrl Pts',(1.37119593248245,1.74999999995591,7.37358947262711));
#132662=CARTESIAN_POINT('Ctrl Pts',(1.44347393988503,1.73849644457293,7.36014862272757));
#132663=CARTESIAN_POINT('Ctrl Pts',(1.51567409001699,1.72693520694185,7.34562253447594));
#132664=CARTESIAN_POINT('Ctrl Pts',(1.58774795046836,1.71532338729505,7.33001067089588));
#132665=CARTESIAN_POINT('Ctrl Pts',(0.9851997,1.845058467,7.182748885));
#132666=CARTESIAN_POINT('Ctrl Pts',(1.273922751,1.797173233,7.143147075));
#132667=CARTESIAN_POINT('Ctrl Pts',(1.558535692,1.75,7.080499029));
#132668=CARTESIAN_POINT('Ctrl Pts',(1.662816028,1.732716033,7.057545191));
#132669=CARTESIAN_POINT('Ctrl Pts',(1.766375162,1.715323387,7.03153033));
#132670=CARTESIAN_POINT('Ctrl Pts',(0.774939815000001,1.845058467,7.459857122));
#132671=CARTESIAN_POINT('Ctrl Pts',(1.074801713,1.797173233,7.428707072));
#132672=CARTESIAN_POINT('Ctrl Pts',(1.371195932,1.75,7.373589473));
#132673=CARTESIAN_POINT('Ctrl Pts',(1.479792853,1.732716033,7.353394742));
#132674=CARTESIAN_POINT('Ctrl Pts',(1.587747952,1.715323387,7.330010671));
#132675=CARTESIAN_POINT('',(1.67706156174498,1.71532338778839,7.18077049939182));
#132676=CARTESIAN_POINT('Ctrl Pts',(1.766375162,1.715323387,7.03153033));
#132677=CARTESIAN_POINT('Ctrl Pts',(2.147016947,1.779910221,6.935910151));
#132678=CARTESIAN_POINT('Ctrl Pts',(2.51511208,1.845052736,6.799758174));
#132679=CARTESIAN_POINT('Ctrl Pts',(2.064855503,1.715323387,7.21015754));
#132680=CARTESIAN_POINT('Ctrl Pts',(2.455167015,1.779910221,7.098379556));
#132681=CARTESIAN_POINT('Ctrl Pts',(2.83113112,1.845052736,6.945120343));
#132682=CARTESIAN_POINT('',(2.06485550015272,1.71532338744839,7.21015754195452));
#132683=CARTESIAN_POINT('',(2.59869932952182,1.80506741729831,7.03539350645313));
#132684=CARTESIAN_POINT('Origin',(-0.0764201321297411,1.87497455512894,
-0.174496271270764));
#132685=CARTESIAN_POINT('Ctrl Pts',(2.51071781620877,1.84427517367611,6.80138192209821));
#132686=CARTESIAN_POINT('Ctrl Pts',(2.52532442072709,1.83740483780848,6.84033877097677));
#132687=CARTESIAN_POINT('Ctrl Pts',(2.53996885979272,1.83070798172457,6.8793399903243));
#132688=CARTESIAN_POINT('Ctrl Pts',(2.56929197405064,1.81765000114506,6.95733017689152));
#132689=CARTESIAN_POINT('Ctrl Pts',(2.58398802854539,1.81128114570797,6.99636536159158));
#132690=CARTESIAN_POINT('Ctrl Pts',(2.59869932691265,1.80506741737884,7.03539350744946));
#132691=CARTESIAN_POINT('',(1.9156153246616,1.71532338829994,7.12084393710865));
#132692=CARTESIAN_POINT('Origin',(2.94902990916057E-14,1.806143924,1.23165366794353E-13));
#132693=CARTESIAN_POINT('',(2.60243101765133,1.62564958721911,7.0340139887338));
#132694=CARTESIAN_POINT('Origin',(-0.085541867002264,1.48225708216688,-0.165240028068662));
#132695=CARTESIAN_POINT('',(3.12636290849826,1.7153233873471,6.81732021967138));
#132696=CARTESIAN_POINT('Origin',(-0.0994150821221096,1.87485304671307,
-0.155797783110659));
#132697=CARTESIAN_POINT('Ctrl Pts',(2.59869933156525,1.80506741660997,7.03539350555662));
#132698=CARTESIAN_POINT('Ctrl Pts',(2.70844556999549,1.78658581162499,6.99485597570313));
#132699=CARTESIAN_POINT('Ctrl Pts',(2.81701357488237,1.76822051520318,6.95183383867207));
#132700=CARTESIAN_POINT('Ctrl Pts',(2.92424190825311,1.75000000000266,6.90643245527506));
#132701=CARTESIAN_POINT('Ctrl Pts',(2.99194071041716,1.73849644464936,6.8777682092977));
#132702=CARTESIAN_POINT('Ctrl Pts',(3.05933018184855,1.72693520694185,6.8480608352413));
#132703=CARTESIAN_POINT('Ctrl Pts',(3.12636290648176,1.71532338729505,6.8173202192276));
#132704=CARTESIAN_POINT('Ctrl Pts',(2.506244968,1.845058467,6.803031395));
#132705=CARTESIAN_POINT('Ctrl Pts',(2.779704616,1.797173233,6.702288531));
#132706=CARTESIAN_POINT('Ctrl Pts',(3.044195986,1.75,6.579921793));
#132707=CARTESIAN_POINT('Ctrl Pts',(3.14110391,1.732716033,6.535087413));
#132708=CARTESIAN_POINT('Ctrl Pts',(3.236649463,1.715323387,6.487418613));
#132709=CARTESIAN_POINT('Ctrl Pts',(2.360470923,1.845058467,7.118860655));
#132710=CARTESIAN_POINT('Ctrl Pts',(2.646625875,1.797173233,7.023977432));
#132711=CARTESIAN_POINT('Ctrl Pts',(2.924241908,1.75,6.906432456));
#132712=CARTESIAN_POINT('Ctrl Pts',(3.025958623,1.732716033,6.863364738));
#132713=CARTESIAN_POINT('Ctrl Pts',(3.126362908,1.715323387,6.817320219));
#132714=CARTESIAN_POINT('',(3.18150618989582,1.71532338778839,6.6523694138977));
#132715=CARTESIAN_POINT('Ctrl Pts',(3.236649463,1.715323387,6.487418613));
#132716=CARTESIAN_POINT('Ctrl Pts',(3.587836542,1.779910221,6.312207247));
#132717=CARTESIAN_POINT('Ctrl Pts',(3.918057165,1.845052736,6.100108856));
#132718=CARTESIAN_POINT('Ctrl Pts',(3.566551069,1.715323387,6.597705167));
#132719=CARTESIAN_POINT('Ctrl Pts',(3.923708353,1.779910221,6.40463505300001));
#132720=CARTESIAN_POINT('Ctrl Pts',(4.257936425,1.845052736,6.174137786));
#132721=CARTESIAN_POINT('',(3.56655106664231,1.7153233874486,6.59770516952165));
#132722=CARTESIAN_POINT('',(4.0503448225298,1.80506741733711,6.31226637702187));
#132723=CARTESIAN_POINT('Origin',(-0.112144917130483,1.87497457603044,-0.153988411054592));
#132724=CARTESIAN_POINT('Ctrl Pts',(3.91411469427357,1.84427517371797,6.10263927834585));
#132725=CARTESIAN_POINT('Ctrl Pts',(3.93675437769205,1.83740483719272,6.13754535275076));
#132726=CARTESIAN_POINT('Ctrl Pts',(3.95944054978277,1.83070798041905,6.17248662756391));
#132727=CARTESIAN_POINT('Ctrl Pts',(4.00484368626686,1.81765000114176,6.24234983715179));
#132728=CARTESIAN_POINT('Ctrl Pts',(4.02758756590525,1.81128114575264,6.2773131833951));
#132729=CARTESIAN_POINT('Ctrl Pts',(4.05034482005215,1.80506741742345,6.31226637865036));
#132730=CARTESIAN_POINT('',(3.40160025879484,1.71532338830053,6.5425618937461));
#132731=CARTESIAN_POINT('Origin',(7.93635990259389E-13,1.80614392399917,
1.20693385841086E-12));
#132732=CARTESIAN_POINT('',(4.0536927102926,1.62564958721554,6.31011690930612));
#132733=CARTESIAN_POINT('Origin',(-0.119063806186307,1.48225703862391,-0.142988065447516));
#132734=CARTESIAN_POINT('',(4.51879260962798,1.7153233873466,5.98585945055491));
#132735=CARTESIAN_POINT('Origin',(-0.130582748919531,1.87485301701732,-0.130784038236786));
#132736=CARTESIAN_POINT('Ctrl Pts',(4.05034482445065,1.80506741660596,6.31226637562157));
#132737=CARTESIAN_POINT('Ctrl Pts',(4.14881088633035,1.78658581163939,6.24908439319196));
#132738=CARTESIAN_POINT('Ctrl Pts',(4.24559214392768,1.76822051521793,6.18372917775308));
#132739=CARTESIAN_POINT('Ctrl Pts',(4.34055358295998,1.75000000001201,6.11633833187862));
#132740=CARTESIAN_POINT('Ctrl Pts',(4.40050765881071,1.73849644466465,6.07379100026899));
#132741=CARTESIAN_POINT('Ctrl Pts',(4.45993539460349,1.72693520694186,6.03029142298064));
#132742=CARTESIAN_POINT('Ctrl Pts',(4.51879260756621,1.71532338729505,5.98585945054844));
#132743=CARTESIAN_POINT('Ctrl Pts',(3.910101007,1.845058467,6.105211717));
#132744=CARTESIAN_POINT('Ctrl Pts',(4.155510583,1.797173233,5.948038425));
#132745=CARTESIAN_POINT('Ctrl Pts',(4.38751306,1.75,5.771674726));
#132746=CARTESIAN_POINT('Ctrl Pts',(4.472517264,1.732716033,5.707056211));
#132747=CARTESIAN_POINT('Ctrl Pts',(4.555581632,1.715323387,5.639962411));
#132748=CARTESIAN_POINT('Ctrl Pts',(3.835629033,1.845058467,6.444994175));
#132749=CARTESIAN_POINT('Ctrl Pts',(4.094696754,1.797173233,6.290814413));
#132750=CARTESIAN_POINT('Ctrl Pts',(4.340553583,1.75,6.116338332));
#132751=CARTESIAN_POINT('Ctrl Pts',(4.430633931,1.732716033,6.052411428));
#132752=CARTESIAN_POINT('Ctrl Pts',(4.518792609,1.715323387,5.98585945));
#132753=CARTESIAN_POINT('',(4.53718712434111,1.71532338778839,5.81291092750188));
#132754=CARTESIAN_POINT('Ctrl Pts',(4.555581632,1.715323387,5.639962411));
#132755=CARTESIAN_POINT('Ctrl Pts',(4.860892888,1.779910221,5.393352549));
#132756=CARTESIAN_POINT('Ctrl Pts',(5.137798252,1.845052736,5.115225227));
#132757=CARTESIAN_POINT('Ctrl Pts',(4.901478671,1.715323387,5.676751433));
#132758=CARTESIAN_POINT('Ctrl Pts',(5.208781448,1.779910221,5.41141693200001));
#132759=CARTESIAN_POINT('Ctrl Pts',(5.485645355,1.845052736,5.11445940800001));
#132760=CARTESIAN_POINT('',(4.90147866925435,1.71532338744861,5.67675143596386));
#132761=CARTESIAN_POINT('',(5.31260069305792,1.80506741735431,5.29398468727746));
#132762=CARTESIAN_POINT('Origin',(-0.142626191119171,1.87497457881845,-0.126280623933815));
#132763=CARTESIAN_POINT('Ctrl Pts',(5.13449192012045,1.84427517373959,5.11854400406275));
#132764=CARTESIAN_POINT('Ctrl Pts',(5.16410607728195,1.83740483654798,5.14776713411668));
#132765=CARTESIAN_POINT('Ctrl Pts',(5.1937732038837,1.83070797905741,5.17701464835099));
#132766=CARTESIAN_POINT('Ctrl Pts',(5.2531333385214,1.81765000563682,5.23548413644653));
#132767=CARTESIAN_POINT('Ctrl Pts',(5.28286154154871,1.81128115488623,5.26474077435008));
#132768=CARTESIAN_POINT('Ctrl Pts',(5.31260069112421,1.80506741744112,5.29398468919549));
#132769=CARTESIAN_POINT('',(4.72853014526859,1.71532338830053,5.65835692720741));
#132770=CARTESIAN_POINT('Origin',(-3.70797142990043E-13,1.80614392399972,
-5.24753851482984E-13));
#132771=CARTESIAN_POINT('',(5.3154082369853,1.62564958723406,5.29116577603139));
#132772=CARTESIAN_POINT('Origin',(-0.147018238527079,1.48225708010876,-0.114049756782595));
#132773=CARTESIAN_POINT('',(5.69992859077017,1.71532338735754,4.8745065462909));
#132774=CARTESIAN_POINT('Origin',(-0.155644556101205,1.87485301895261,-0.0996550053948186));
#132775=CARTESIAN_POINT('Ctrl Pts',(5.31260069456111,1.80506741667151,5.29398468568869));
#132776=CARTESIAN_POINT('Ctrl Pts',(5.39518241618632,1.78658581165965,5.21111257035019));
#132777=CARTESIAN_POINT('Ctrl Pts',(5.47565154239998,1.76822051521757,5.12648021422536));
#132778=CARTESIAN_POINT('Ctrl Pts',(5.5539057960115,1.74999999998492,5.04025102627439));
#132779=CARTESIAN_POINT('Ctrl Pts',(5.60331176043689,1.73849644462036,4.9858100722164));
#132780=CARTESIAN_POINT('Ctrl Pts',(5.65199898542071,1.72693520694185,4.93055228506105));
#132781=CARTESIAN_POINT('Ctrl Pts',(5.69992858871765,1.71532338729505,4.87450654684407));
#132782=CARTESIAN_POINT('Ctrl Pts',(5.131125069,1.845058467,5.121919125));
#132783=CARTESIAN_POINT('Ctrl Pts',(5.337009493,1.797173233,4.915664652));
#132784=CARTESIAN_POINT('Ctrl Pts',(5.5256749,1.75,4.693550565));
#132785=CARTESIAN_POINT('Ctrl Pts',(5.594800682,1.732716033,4.612169403));
#132786=CARTESIAN_POINT('Ctrl Pts',(5.661499867,1.715323387,4.528787835));
#132787=CARTESIAN_POINT('Ctrl Pts',(5.131437393,1.845058467,5.469766932));
#132788=CARTESIAN_POINT('Ctrl Pts',(5.351304163,1.797173233,5.263499904));
#132789=CARTESIAN_POINT('Ctrl Pts',(5.553905796,1.75,5.040251027));
#132790=CARTESIAN_POINT('Ctrl Pts',(5.628137721,1.732716033,4.958454085));
#132791=CARTESIAN_POINT('Ctrl Pts',(5.69992859,1.715323387,4.874506546));
#132792=CARTESIAN_POINT('',(5.6807142316068,1.71532338778839,4.70164718674625));
#132793=CARTESIAN_POINT('Ctrl Pts',(5.661499867,1.715323387,4.528787835));
#132794=CARTESIAN_POINT('Ctrl Pts',(5.906659286,1.779910221,4.222310679));
#132795=CARTESIAN_POINT('Ctrl Pts',(6.117301603,1.845052736,3.891159352));
#132796=CARTESIAN_POINT('Ctrl Pts',(6.00721857800001,1.715323387,4.490359112));
#132797=CARTESIAN_POINT('Ctrl Pts',(6.250297713,1.779910221,4.165166971));
#132798=CARTESIAN_POINT('Ctrl Pts',(6.456851606,1.845052736,3.815634592));
#132799=CARTESIAN_POINT('',(6.00721857692768,1.71532338744743,4.4903591152651));
#132800=CARTESIAN_POINT('',(6.32644526003464,1.80506741731562,4.02816215775166));
#132801=CARTESIAN_POINT('Origin',(-0.166438120757657,1.87497456263235,-0.0926677379795166));
#132802=CARTESIAN_POINT('Ctrl Pts',(6.11478601007336,1.84427517366593,3.89511130188059));
#132803=CARTESIAN_POINT('Ctrl Pts',(6.14998991154671,1.83740483692664,3.91728504138385));
#132804=CARTESIAN_POINT('Ctrl Pts',(6.18525078550277,1.83070797992551,3.93947120792344));
#132805=CARTESIAN_POINT('Ctrl Pts',(6.25579235404182,1.81765000111118,3.98381305591478));
#132806=CARTESIAN_POINT('Ctrl Pts',(6.2911148683189,1.81128114571037,4.00599502240091));
#132807=CARTESIAN_POINT('Ctrl Pts',(6.32644525851615,1.80506741739896,4.02816216019523));
#132808=CARTESIAN_POINT('',(5.83435921754669,1.71532338829715,4.50957347990846));
#132809=CARTESIAN_POINT('Origin',(-6.34908792207511E-13,1.80614392400067,
-4.53196508098941E-13));
#132810=CARTESIAN_POINT('',(6.32858118252632,1.62564958718437,4.024805611846));
#132811=CARTESIAN_POINT('Origin',(-0.168098257326036,1.48225710020701,-0.0797786914912602));
#132812=CARTESIAN_POINT('',(6.61454224581474,1.71532338735652,3.53522713313313));
#132813=CARTESIAN_POINT('Origin',(-0.17342861253934,1.87485299658896,-0.0638661794487672));
#132814=CARTESIAN_POINT('Ctrl Pts',(6.32644526115658,1.80506741660584,4.02816215574145));
#132815=CARTESIAN_POINT('Ctrl Pts',(6.38928121287247,1.7865858116304,3.92947491541144));
#132816=CARTESIAN_POINT('Ctrl Pts',(6.44967556073724,1.76822051520956,3.82952273321842));
#132817=CARTESIAN_POINT('Ctrl Pts',(6.50756354678065,1.75000000001832,3.72848718457675));
#132818=CARTESIAN_POINT('Ctrl Pts',(6.54411123116617,1.73849644467496,3.66469820839607));
#132819=CARTESIAN_POINT('Ctrl Pts',(6.57978138511481,1.72693520694185,3.60026600275635));
#132820=CARTESIAN_POINT('Ctrl Pts',(6.61454224392906,1.71532338729505,3.53522713409992));
#132821=CARTESIAN_POINT('Ctrl Pts',(6.112223425,1.845058467,3.899131288));
#132822=CARTESIAN_POINT('Ctrl Pts',(6.268955771,1.797173233,3.653439864));
#132823=CARTESIAN_POINT('Ctrl Pts',(6.405462322,1.75,3.395961195));
#132824=CARTESIAN_POINT('Ctrl Pts',(6.455477438,1.732716033,3.30162268));
#132825=CARTESIAN_POINT('Ctrl Pts',(6.502692661,1.715323387,3.205852173));
#132826=CARTESIAN_POINT('Ctrl Pts',(6.187305443,1.845058467,4.238779465));
#132827=CARTESIAN_POINT('Ctrl Pts',(6.357690537,1.797173233,3.99006999));
#132828=CARTESIAN_POINT('Ctrl Pts',(6.507563547,1.75,3.728487185));
#132829=CARTESIAN_POINT('Ctrl Pts',(6.562476046,1.732716033,3.632644941));
#132830=CARTESIAN_POINT('Ctrl Pts',(6.614542245,1.715323387,3.535227133));
#132831=CARTESIAN_POINT('',(6.55861745522722,1.71532338778839,3.37053964866614));
#132832=CARTESIAN_POINT('Ctrl Pts',(6.502692661,1.715323387,3.205852173));
#132833=CARTESIAN_POINT('Ctrl Pts',(6.676236859,1.779910221,2.853838255));
#132834=CARTESIAN_POINT('Ctrl Pts',(6.810766729,1.845052736,2.48514719));
#132835=CARTESIAN_POINT('Ctrl Pts',(6.832067621,1.715323387,3.094002589));
#132836=CARTESIAN_POINT('Ctrl Pts',(6.999557003,1.779910221,2.724158431));
#132837=CARTESIAN_POINT('Ctrl Pts',(7.126142651,1.845052736,2.338394944));
#132838=CARTESIAN_POINT('',(6.83206762065268,1.71532338744779,3.09400259242416));
#132839=CARTESIAN_POINT('',(7.04447227761881,1.80506741731637,2.57398724268056));
#132840=CARTESIAN_POINT('Origin',(-0.182467701556788,1.87497457397358,-0.0547219325918286));
#132841=CARTESIAN_POINT('Ctrl Pts',(6.80915950284082,1.84427517370896,2.48954752285449));
#132842=CARTESIAN_POINT('Ctrl Pts',(6.84830704640822,1.83740483848713,2.50363505160379));
#132843=CARTESIAN_POINT('Ctrl Pts',(6.88751290039156,1.83070798310218,2.51772246887146));
#132844=CARTESIAN_POINT('Ctrl Pts',(6.96593745123682,1.81765000117452,2.54586328409677));
#132845=CARTESIAN_POINT('Ctrl Pts',(7.00520261195919,1.81128114573483,2.55993335230123));
#132846=CARTESIAN_POINT('Ctrl Pts',(7.04447227667578,1.80506741739832,2.57398724535184));
#132847=CARTESIAN_POINT('',(6.66738013753733,1.71532338829819,3.14992738832937));
#132848=CARTESIAN_POINT('Origin',(-6.5746019739521E-13,1.80614392400017,
-3.50414142147315E-13));
#132849=CARTESIAN_POINT('',(7.04583670518615,1.62564958718578,2.57025001060835));
#132850=CARTESIAN_POINT('Origin',(-0.181318472582188,1.48225706044545,-0.041777424151937));
#132851=CARTESIAN_POINT('',(7.21986725682524,1.71532338735623,2.03064442895894));
#132852=CARTESIAN_POINT('Origin',(-0.183103012008832,1.87485300201219,-0.0250909106018232));
#132853=CARTESIAN_POINT('Ctrl Pts',(7.04447227826771,1.80506741661818,2.57398724050962));
#132854=CARTESIAN_POINT('Ctrl Pts',(7.08462432078263,1.78658581163429,2.46409938080374));
#132855=CARTESIAN_POINT('Ctrl Pts',(7.12211991779882,1.76822051520959,2.3535010254003));
#132856=CARTESIAN_POINT('Ctrl Pts',(7.15693485866943,1.75000000001996,2.24238342560448));
#132857=CARTESIAN_POINT('Ctrl Pts',(7.17891533426046,1.73849644467764,2.17222912820569));
#132858=CARTESIAN_POINT('Ctrl Pts',(7.19990052025176,1.72693520694185,2.10163528313927));
#132859=CARTESIAN_POINT('Ctrl Pts',(7.21986725519057,1.71532338729505,2.03064443030443));
#132860=CARTESIAN_POINT('Ctrl Pts',(6.807521008,1.845058467,2.494024404));
#132861=CARTESIAN_POINT('Ctrl Pts',(6.907772645,1.797173233,2.220384289));
#132862=CARTESIAN_POINT('Ctrl Pts',(6.985737446,1.75,1.939580454));
#132863=CARTESIAN_POINT('Ctrl Pts',(7.014303243,1.732716033,1.83669575));
#132864=CARTESIAN_POINT('Ctrl Pts',(7.039826773,1.715323387,1.733014427));
#132865=CARTESIAN_POINT('Ctrl Pts',(6.953861968,1.845058467,2.809591382));
#132866=CARTESIAN_POINT('Ctrl Pts',(7.06679836700001,1.797173233,2.530068838));
#132867=CARTESIAN_POINT('Ctrl Pts',(7.156934859,1.75,2.242383426));
#132868=CARTESIAN_POINT('Ctrl Pts',(7.18996028500001,1.732716033,2.136977356));
#132869=CARTESIAN_POINT('Ctrl Pts',(7.21986725600001,1.715323387,2.030644429));
#132870=CARTESIAN_POINT('',(7.12984701574349,1.71532338778839,1.88182942328867));
#132871=CARTESIAN_POINT('Ctrl Pts',(7.039826773,1.715323387,1.733014427));
#132872=CARTESIAN_POINT('Ctrl Pts',(7.133641018,1.779910221,1.351923526));
#132873=CARTESIAN_POINT('Ctrl Pts',(7.18576797400001,1.845052736,0.962932308));
#132874=CARTESIAN_POINT('Ctrl Pts',(7.337456775,1.715323387,1.552973944));
#132875=CARTESIAN_POINT('Ctrl Pts',(7.421524787,1.779910221,1.15577127));
#132876=CARTESIAN_POINT('Ctrl Pts',(7.462223187,1.845052736,0.751814547));
#132877=CARTESIAN_POINT('',(7.33745677540195,1.71532338744823,1.55297394741524));
#132878=CARTESIAN_POINT('',(7.43310760101885,1.80506741731817,0.99945554461675));
#132879=CARTESIAN_POINT('Origin',(-0.189965455514084,1.87497461017791,-0.0142174232791398));
#132880=CARTESIAN_POINT('Ctrl Pts',(7.18514426466047,1.84427517372893,0.967575270075705));
#132881=CARTESIAN_POINT('Ctrl Pts',(7.22640497351326,1.83740483668611,0.972917876941878));
#132882=CARTESIAN_POINT('Ctrl Pts',(7.26772260749884,1.83070797936229,0.978247840077157));
#132883=CARTESIAN_POINT('Ctrl Pts',(7.35036305583967,1.81765000113681,0.988871775213704));
#132884=CARTESIAN_POINT('Ctrl Pts',(7.39173486735399,1.8112811457412,0.994172043980483));
#132885=CARTESIAN_POINT('Ctrl Pts',(7.43310760065318,1.80506741740517,0.999455547582473));
#132886=CARTESIAN_POINT('',(7.1886417721921,1.71532338829947,1.64299419341015));
#132887=CARTESIAN_POINT('Origin',(6.38811920028459E-13,1.80614392400006,
-5.39390580811538E-15));
#132888=CARTESIAN_POINT('',(7.43363673487287,1.62564958721554,0.995512375212924));
#132889=CARTESIAN_POINT('Origin',(-0.186060401123735,1.48225706441154,-0.00182260911100379));
#132890=CARTESIAN_POINT('',(7.48759929982863,1.71532338734673,0.43111104887891));
#132891=CARTESIAN_POINT('Origin',(-0.184216316486344,1.87485304405876,0.0148574046167898));
#132892=CARTESIAN_POINT('Ctrl Pts',(7.4331076011919,1.805067416582,0.999455542227304));
#132893=CARTESIAN_POINT('Ctrl Pts',(7.44869826958329,1.78658581162576,0.883505297448109));
#132894=CARTESIAN_POINT('Ctrl Pts',(7.46154186313188,1.76822051521192,0.767432225427406));
#132895=CARTESIAN_POINT('Ctrl Pts',(7.47165585077362,1.74999999996564,0.651428310507613));
#132896=CARTESIAN_POINT('Ctrl Pts',(7.47804133522892,1.73849644458883,0.57818902898479));
#132897=CARTESIAN_POINT('Ctrl Pts',(7.48336030927677,1.72693520694185,0.504734434407505));
#132898=CARTESIAN_POINT('Ctrl Pts',(7.4875992984897,1.71532338729505,0.431111050447745));
#132899=CARTESIAN_POINT('Ctrl Pts',(7.184506474,1.845058467,0.972299712));
#132900=CARTESIAN_POINT('Ctrl Pts',(7.223589747,1.797173233,0.683506012));
#132901=CARTESIAN_POINT('Ctrl Pts',(7.23936725,1.75,0.392507087));
#132902=CARTESIAN_POINT('Ctrl Pts',(7.245148025,1.732716033,0.285886968));
#132903=CARTESIAN_POINT('Ctrl Pts',(7.24778641,1.715323387,0.179142852));
#132904=CARTESIAN_POINT('Ctrl Pts',(7.395263635,1.845058467,1.249029928));
#132905=CARTESIAN_POINT('Ctrl Pts',(7.44547056,1.797173233,0.951764478));
#132906=CARTESIAN_POINT('Ctrl Pts',(7.471655851,1.75,0.651428311));
#132907=CARTESIAN_POINT('Ctrl Pts',(7.481249972,1.732716033,0.541387086));
#132908=CARTESIAN_POINT('Ctrl Pts',(7.487599299,1.715323387,0.431111049));
#132909=CARTESIAN_POINT('',(7.36769285470163,1.71532338778839,0.305126945631507));
#132910=CARTESIAN_POINT('Ctrl Pts',(7.24778641,1.715323387,0.179142852));
#132911=CARTESIAN_POINT('Ctrl Pts',(7.25748405,1.779910221,-0.213205645));
#132912=CARTESIAN_POINT('Ctrl Pts',(7.22477069400001,1.845052736,-0.604308219));
#132913=CARTESIAN_POINT('Ctrl Pts',(7.499754606,1.715323387,-0.060670037));
#132914=CARTESIAN_POINT('Ctrl Pts',(7.496470321,1.779910221,-0.46665847));
#132915=CARTESIAN_POINT('Ctrl Pts',(7.449378459,1.845052736,-0.869919863));
#132916=CARTESIAN_POINT('',(7.49975460711691,1.71532338744859,-0.0606700337169635));
#132917=CARTESIAN_POINT('',(7.47417907449485,1.80506741732727,-0.621809583799175));
#132918=CARTESIAN_POINT('Origin',(-0.188580229757588,1.87497455775272,0.0269519145656917));
#132919=CARTESIAN_POINT('Ctrl Pts',(7.22515966610095,1.84427517370307,-0.599639727402906));
#132920=CARTESIAN_POINT('Ctrl Pts',(7.26660422586505,1.83740483653573,-0.603291860843548));
#132921=CARTESIAN_POINT('Ctrl Pts',(7.30810166197752,1.83070797908474,-0.606968579461518));
#132922=CARTESIAN_POINT('Ctrl Pts',(7.3910938530514,1.81765000112985,-0.614358279513735));
#132923=CARTESIAN_POINT('Ctrl Pts',(7.43263781590535,1.81128114572277,-0.618075644573826));
#132924=CARTESIAN_POINT('Ctrl Pts',(7.47417907476336,1.80506741741021,-0.621809580950034));
#132925=CARTESIAN_POINT('',(7.37377050793477,1.71532338830053,0.0592364156205474));
#132926=CARTESIAN_POINT('Origin',(-3.72531866466019E-13,1.8061439240005,
9.02598308594182E-14));
#132927=CARTESIAN_POINT('',(7.47384817270388,1.6256495872157,-0.625774312001561));
#132928=CARTESIAN_POINT('Origin',(-0.182101997659883,1.48225706935401,0.0382174822994667));
#132929=CARTESIAN_POINT('',(7.40521952078754,1.71532338734622,-1.18858060629072));
#132930=CARTESIAN_POINT('Origin',(-0.176715334484012,1.87485302405344,0.0541110863609406));
#132931=CARTESIAN_POINT('Ctrl Pts',(7.47417907417002,1.80506741662168,-0.621809586066532));
#132932=CARTESIAN_POINT('Ctrl Pts',(7.46447936625317,1.7865858116396,-0.738400511443372));
#132933=CARTESIAN_POINT('Ctrl Pts',(7.45207040425345,1.76822051521369,-0.854520852749165));
#132934=CARTESIAN_POINT('Ctrl Pts',(7.4370105196625,1.750000000046,-0.96998686897824));
#132935=CARTESIAN_POINT('Ctrl Pts',(7.42750243431284,1.7384964447202,-1.04288654643311));
#132936=CARTESIAN_POINT('Ctrl Pts',(7.41690648710136,1.72693520694185,-1.11576723638024));
#132937=CARTESIAN_POINT('Ctrl Pts',(7.40521951981277,1.71532338729505,-1.18858060447645));
#132938=CARTESIAN_POINT('Ctrl Pts',(7.225552402,1.845058467,-0.594888634));
#132939=CARTESIAN_POINT('Ctrl Pts',(7.201639821,1.797173233,-0.885332247));
#132940=CARTESIAN_POINT('Ctrl Pts',(7.154492288,1.75,-1.172919475));
#132941=CARTESIAN_POINT('Ctrl Pts',(7.137217738,1.732716033,-1.278289571));
#132942=CARTESIAN_POINT('Ctrl Pts',(7.116847609,1.715323387,-1.383105243));
#132943=CARTESIAN_POINT('Ctrl Pts',(7.490870995,1.845058467,-0.369934777));
#132944=CARTESIAN_POINT('Ctrl Pts',(7.476000825,1.797173233,-0.67104333));
#132945=CARTESIAN_POINT('Ctrl Pts',(7.43701052,1.75,-0.969986869));
#132946=CARTESIAN_POINT('Ctrl Pts',(7.422724725,1.732716033,-1.079517843));
#132947=CARTESIAN_POINT('Ctrl Pts',(7.40521952,1.715323387,-1.188580606));
#132948=CARTESIAN_POINT('',(7.26103356365033,1.71532338778839,-1.28584292929801));
#132949=CARTESIAN_POINT('Ctrl Pts',(7.116847609,1.715323387,-1.383105243));
#132950=CARTESIAN_POINT('Ctrl Pts',(7.04197519500001,1.779910221,-1.768365556));
#132951=CARTESIAN_POINT('Ctrl Pts',(6.925951166,1.845052736,-2.143291965));
#132952=CARTESIAN_POINT('Ctrl Pts',(7.311372246,1.715323387,-1.671477154));
#132953=CARTESIAN_POINT('Ctrl Pts',(7.220889234,1.779910221,-2.067267779));
#132954=CARTESIAN_POINT('Ctrl Pts',(7.088209075,1.845052736,-2.450977787));
#132955=CARTESIAN_POINT('',(7.31137224780019,1.7153233874486,-1.67147715106331));
#132956=CARTESIAN_POINT('',(7.16576624136519,1.80506741729005,-2.21399958686633));
#132957=CARTESIAN_POINT('Origin',(-0.178377524981393,1.87497455155373,0.0668609764454212));
#132958=CARTESIAN_POINT('Ctrl Pts',(6.92733463178518,1.84427517371465,-2.13881623762417));
#132959=CARTESIAN_POINT('Ctrl Pts',(6.96702514232173,1.83740483617331,-2.15129234207367));
#132960=CARTESIAN_POINT('Ctrl Pts',(7.00676200825457,1.83070797831737,-2.16380382392064));
#132961=CARTESIAN_POINT('Ctrl Pts',(7.08622531640099,1.81765000111462,-2.18886162321189));
#132962=CARTESIAN_POINT('Ctrl Pts',(7.12599888080652,1.81128114571596,-2.20142280227942));
#132963=CARTESIAN_POINT('Ctrl Pts',(7.16576624227572,1.80506741737912,-2.21399958403128));
#132964=CARTESIAN_POINT('',(7.21410992918197,1.71532338830053,-1.52729119055528));
#132965=CARTESIAN_POINT('Origin',(-1.3162214373974E-12,1.80614392400089,
4.32596666821716E-13));
#132966=CARTESIAN_POINT('',(7.1645907762973,1.62564958719313,-2.21780048786883));
#132967=CARTESIAN_POINT('Origin',(-0.169628947985297,1.48225708989375,0.0764705232282592));
#132968=CARTESIAN_POINT('',(6.97657990728278,1.7153233872797,-2.75269555326827));
#132969=CARTESIAN_POINT('Origin',(-0.160951713078892,1.87485303486766,0.0908346270390281));
#132970=CARTESIAN_POINT('Ctrl Pts',(7.16576624052238,1.80506741655413,-2.21399958912398));
#132971=CARTESIAN_POINT('Ctrl Pts',(7.11406920084479,1.77740267790226,-2.38132071423326));
#132972=CARTESIAN_POINT('Ctrl Pts',(7.05461884250418,1.75,-2.54604654021329));
#132973=CARTESIAN_POINT('Ctrl Pts',(7.01712111950104,1.732716033,-2.64994571820598));
#132974=CARTESIAN_POINT('Ctrl Pts',(6.97657990649811,1.715323387,-2.75269555219859));
#132975=CARTESIAN_POINT('Ctrl Pts',(6.92873953,1.845058467,-2.134260649));
#132976=CARTESIAN_POINT('Ctrl Pts',(6.84294922100001,1.797173233,-2.412773354));
#132977=CARTESIAN_POINT('Ctrl Pts',(6.735081219,1.75,-2.683501626));
#132978=CARTESIAN_POINT('Ctrl Pts',(6.695559082,1.732716033,-2.78269471));
#132979=CARTESIAN_POINT('Ctrl Pts',(6.653132924,1.715323387,-2.880680874));
#132980=CARTESIAN_POINT('Ctrl Pts',(7.236213552,1.845058467,-1.971601742));
#132981=CARTESIAN_POINT('Ctrl Pts',(7.1569616,1.797173233,-2.262473898));
#132982=CARTESIAN_POINT('Ctrl Pts',(7.054618843,1.75,-2.54604654));
#132983=CARTESIAN_POINT('Ctrl Pts',(7.01712112,1.732716033,-2.649945718));
#132984=CARTESIAN_POINT('Ctrl Pts',(6.976579907,1.715323387,-2.752695552));
#132985=CARTESIAN_POINT('',(6.81485641363876,1.71532338778839,-2.81668821750318));
#132986=CARTESIAN_POINT('Ctrl Pts',(6.653132924,1.715323387,-2.880680874));
#132987=CARTESIAN_POINT('Ctrl Pts',(6.497191406,1.779910221,-3.24083866));
#132988=CARTESIAN_POINT('Ctrl Pts',(6.303281859,1.845052736,-3.582057761));
#132989=CARTESIAN_POINT('Ctrl Pts',(6.781118246,1.715323387,-3.204127858));
#132990=CARTESIAN_POINT('Ctrl Pts',(6.607667391,1.779910221,-3.571213945));
#132991=CARTESIAN_POINT('Ctrl Pts',(6.395602912,1.845052736,-3.917430713));
#132992=CARTESIAN_POINT('',(6.78111824838966,1.7153233874486,-3.20412785551618));
#132993=CARTESIAN_POINT('',(6.52229014260304,1.80506741731559,-3.70266543055499));
#132994=CARTESIAN_POINT('Origin',(-0.159834165078843,1.87497459574732,0.103643782784949));
#132995=CARTESIAN_POINT('Ctrl Pts',(6.30559512922781,1.84427517371725,-3.57798407800257));
#132996=CARTESIAN_POINT('Ctrl Pts',(6.34167569827233,1.83740483728647,-3.59870078122464));
#132997=CARTESIAN_POINT('Ctrl Pts',(6.37779393284573,1.83070798060367,-3.61946199927444));
#132998=CARTESIAN_POINT('Ctrl Pts',(6.45001275928298,1.81765000115535,-3.66101623075933));
#132999=CARTESIAN_POINT('Ctrl Pts',(6.48615615778852,1.8112811457277,-3.68183387727167));
#133000=CARTESIAN_POINT('Ctrl Pts',(6.52229014402864,1.80506741739754,-3.70266542810664));
#133001=CARTESIAN_POINT('',(6.71712558835053,1.71532338830053,-3.0424043586026));
#133002=CARTESIAN_POINT('Origin',(-7.41594285980085E-13,1.80614392400039,
4.57966997657877E-13));
#133003=CARTESIAN_POINT('',(6.52032507813897,1.62564958718767,-3.70612477802065));
#133004=CARTESIAN_POINT('Origin',(-0.149224148019865,1.48225708657861,0.111147861824504));
#133005=CARTESIAN_POINT('',(6.22172317159653,1.71532338734596,-4.18809751359268));
#133006=CARTESIAN_POINT('Origin',(-0.137661888875984,1.87485299115467,0.123310757861001));
#133007=CARTESIAN_POINT('Ctrl Pts',(6.52229014136684,1.80506741661758,-3.70266543245436));
#133008=CARTESIAN_POINT('Ctrl Pts',(6.46453166599464,1.78658581163406,-3.80440768893434));
#133009=CARTESIAN_POINT('Ctrl Pts',(6.40451193142273,1.76822051520921,-3.90458526841971));
#133010=CARTESIAN_POINT('Ctrl Pts',(6.34236102849571,1.74999999995533,-4.00305590530895));
#133011=CARTESIAN_POINT('Ctrl Pts',(6.30312194351028,1.73849644457198,-4.06522552017018));
#133012=CARTESIAN_POINT('Ctrl Pts',(6.26290351519366,1.72693520694186,-4.12692111936024));
#133013=CARTESIAN_POINT('Ctrl Pts',(6.22172317147024,1.71532338729505,-4.18809751153858));
#133014=CARTESIAN_POINT('Ctrl Pts',(6.307946499,1.845058467,-3.573837008));
#133015=CARTESIAN_POINT('Ctrl Pts',(6.164289921,1.797173233,-3.82739586));
#133016=CARTESIAN_POINT('Ctrl Pts',(6.000745237,1.75,-4.068606224));
#133017=CARTESIAN_POINT('Ctrl Pts',(5.940823524,1.732716033,-4.156984138));
#133018=CARTESIAN_POINT('Ctrl Pts',(5.87832513800001,1.715323387,-4.24355907));
#133019=CARTESIAN_POINT('Ctrl Pts',(6.643198806,1.845058467,-3.481078802));
#133020=CARTESIAN_POINT('Ctrl Pts',(6.503270805,1.797173233,-3.748113702));
#133021=CARTESIAN_POINT('Ctrl Pts',(6.342361029,1.75,-4.003055905));
#133022=CARTESIAN_POINT('Ctrl Pts',(6.28340473,1.732716033,-4.096465076));
#133023=CARTESIAN_POINT('Ctrl Pts',(6.221723171,1.715323387,-4.188097513));
#133024=CARTESIAN_POINT('',(6.05002415171423,1.71532338778839,-4.21582829549779));
#133025=CARTESIAN_POINT('Ctrl Pts',(5.878325138,1.715323387,-4.24355907));
#133026=CARTESIAN_POINT('Ctrl Pts',(5.648606168,1.779910221,-4.56177375));
#133027=CARTESIAN_POINT('Ctrl Pts',(5.385878098,1.845052736,-4.853330517));
#133028=CARTESIAN_POINT('Ctrl Pts',(5.933786694,1.715323387,-4.586957104));
#133029=CARTESIAN_POINT('Ctrl Pts',(5.685478366,1.779910221,-4.908174115));
#133030=CARTESIAN_POINT('Ctrl Pts',(5.403945465,1.845052736,-5.200708934));
#133031=CARTESIAN_POINT('',(5.93378669687623,1.71532338744858,-4.5869571020615));
#133032=CARTESIAN_POINT('',(5.57383900614683,1.80506741730661,-5.01819875357225));
#133033=CARTESIAN_POINT('Origin',(-0.133817050721352,1.8749745499756,0.135580323984583));
#133034=CARTESIAN_POINT('Ctrl Pts',(5.38901300709274,1.84427517363401,-4.84984936019252));
#133035=CARTESIAN_POINT('Ctrl Pts',(5.41979654877647,1.83740483829925,-4.87783796967003));
#133036=CARTESIAN_POINT('Ctrl Pts',(5.45060730516344,1.83070798279121,-4.90587814936565));
#133037=CARTESIAN_POINT('Ctrl Pts',(5.51220477455614,1.81765000115592,-4.96198578808963));
#133038=CARTESIAN_POINT('Ctrl Pts',(5.54302798188949,1.81128114573603,-4.99008649174508));
#133039=CARTESIAN_POINT('Ctrl Pts',(5.57383900811601,1.80506741739091,-5.01819875143265));
#133040=CARTESIAN_POINT('',(5.90605592086241,1.71532338830053,-4.41525808049581));
#133041=CARTESIAN_POINT('Origin',(-7.43329009456062E-13,1.80614392399978,
7.86263415486488E-13));
#133042=CARTESIAN_POINT('',(5.5711762260882,1.62564958718905,-5.02115479264374));
#133043=CARTESIAN_POINT('Origin',(-0.121842006482895,1.48225709229395,0.140628193630493));
#133044=CARTESIAN_POINT('',(5.17594557531704,1.71532338735862,-5.42766869075742));
#133045=CARTESIAN_POINT('Origin',(-0.107935379387698,1.87485296552199,0.150021153472114));
#133046=CARTESIAN_POINT('Ctrl Pts',(5.57383900449109,1.80506741658938,-5.01819875520795));
#133047=CARTESIAN_POINT('Ctrl Pts',(5.49555931254626,1.78658581162276,-5.1051459692823));
#133048=CARTESIAN_POINT('Ctrl Pts',(5.41540758776006,1.76822051520736,-5.19007898388589));
#133049=CARTESIAN_POINT('Ctrl Pts',(5.33354146241272,1.7500000000465,-5.27288682476711));
#133050=CARTESIAN_POINT('Ctrl Pts',(5.28185513600857,1.73849644472102,-5.32516770431212));
#133051=CARTESIAN_POINT('Ctrl Pts',(5.22931426207082,1.72693520694185,-5.37677512226718));
#133052=CARTESIAN_POINT('Ctrl Pts',(5.17594557577341,1.71532338729505,-5.42766868867384));
#133053=CARTESIAN_POINT('Ctrl Pts',(5.392200901,1.845058467,-4.846304721));
#133054=CARTESIAN_POINT('Ctrl Pts',(5.197395276,1.797173233,-5.06305359));
#133055=CARTESIAN_POINT('Ctrl Pts',(4.985821077,1.75,-5.263467316));
#133056=CARTESIAN_POINT('Ctrl Pts',(4.908301662,1.732716033,-5.336897607));
#133057=CARTESIAN_POINT('Ctrl Pts',(4.828653401,1.715323387,-5.40801315900001));
#133058=CARTESIAN_POINT('Ctrl Pts',(5.739555467,1.845058467,-4.827784486));
#133059=CARTESIAN_POINT('Ctrl Pts',(5.54549429500001,1.797173233,-5.05849587400001));
#133060=CARTESIAN_POINT('Ctrl Pts',(5.333541463,1.75,-5.272886825));
#133061=CARTESIAN_POINT('Ctrl Pts',(5.255883319,1.732716033,-5.351438279));
#133062=CARTESIAN_POINT('Ctrl Pts',(5.175945575,1.715323387,-5.42766869));
#133063=CARTESIAN_POINT('',(5.00229948441995,1.71532338778839,-5.41784092780546));
#133064=CARTESIAN_POINT('Ctrl Pts',(4.828653401,1.715323387,-5.408013159));
#133065=CARTESIAN_POINT('Ctrl Pts',(4.535898384,1.779910221,-5.669405369));
#133066=CARTESIAN_POINT('Ctrl Pts',(4.216636664,1.845052736,-5.897666932));
#133067=CARTESIAN_POINT('Ctrl Pts',(4.808997871,1.715323387,-5.755305333));
#133068=CARTESIAN_POINT('Ctrl Pts',(4.497442691,1.779910221,-6.015633519));
#133069=CARTESIAN_POINT('Ctrl Pts',(4.159605534,1.845052736,-6.240807784));
#133070=CARTESIAN_POINT('',(4.80899787421697,1.7153233874486,-5.75530533174012));
#133071=CARTESIAN_POINT('',(4.36476135241826,1.80506741731031,-6.09908667995287));
#133072=CARTESIAN_POINT('Origin',(-0.101542619938455,1.87497458295353,0.161177119256457));
#133073=CARTESIAN_POINT('Ctrl Pts',(4.22044662611338,1.84427517372663,-5.89494107521926));
#133074=CARTESIAN_POINT('Ctrl Pts',(4.24449374406009,1.83740483775101,-5.92889288124366));
#133075=CARTESIAN_POINT('Ctrl Pts',(4.26855635477787,1.83070798156074,-5.96290090268123));
#133076=CARTESIAN_POINT('Ctrl Pts',(4.31665222094061,1.81765000116853,-6.03093840455445));
#133077=CARTESIAN_POINT('Ctrl Pts',(4.34071397812627,1.81128114573728,-6.06500820782899));
#133078=CARTESIAN_POINT('Ctrl Pts',(4.36476135477305,1.80506741739355,-6.0990866783064));
#133079=CARTESIAN_POINT('',(4.81882564214694,1.71532338830053,-5.58165924069315));
#133080=CARTESIAN_POINT('Origin',(5.08707659330199E-13,1.8061439240005,
-7.70217223333702E-13));
#133081=CARTESIAN_POINT('',(4.36152536599515,1.6256495872286,-6.10140118956462));
#133082=CARTESIAN_POINT('Origin',(-0.0887624671539777,1.48225710253061,
0.163532757542503));
#133083=CARTESIAN_POINT('',(3.88814651615066,1.71532338735835,-6.41344811180768));
#133084=CARTESIAN_POINT('Origin',(-0.0731616365055499,1.87485299007194,
0.169716425058697));
#133085=CARTESIAN_POINT('Ctrl Pts',(4.3647613504681,1.805067416603,-6.09908668117183));
#133086=CARTESIAN_POINT('Ctrl Pts',(4.26962071314246,1.78658581162838,-6.16717329779867));
#133087=CARTESIAN_POINT('Ctrl Pts',(4.17308480344671,1.76822051520836,-6.23289037410551));
#133088=CARTESIAN_POINT('Ctrl Pts',(4.07533142468709,1.74999999999323,-6.29616341695472));
#133089=CARTESIAN_POINT('Ctrl Pts',(4.01361465257327,1.73849644463394,-6.33611096694137));
#133090=CARTESIAN_POINT('Ctrl Pts',(3.95120808549899,1.72693520694185,-6.3752170969759));
#133091=CARTESIAN_POINT('Ctrl Pts',(3.88814651704041,1.71532338729505,-6.41344810987111));
#133092=CARTESIAN_POINT('Ctrl Pts',(4.224321981,1.845058467,-5.892164611));
#133093=CARTESIAN_POINT('Ctrl Pts',(3.987476203,1.797173233,-6.061968561));
#133094=CARTESIAN_POINT('Ctrl Pts',(3.737765465,1.75,-6.212214527));
#133095=CARTESIAN_POINT('Ctrl Pts',(3.646273069,1.732716033,-6.267263675));
#133096=CARTESIAN_POINT('Ctrl Pts',(3.553199198,1.715323387,-6.319594564));
#133097=CARTESIAN_POINT('Ctrl Pts',(4.567536894,1.845058467,-5.948748333));
#133098=CARTESIAN_POINT('Ctrl Pts',(4.328416635,1.797173233,-6.13234840100001));
#133099=CARTESIAN_POINT('Ctrl Pts',(4.075331425,1.75,-6.296163417));
#133100=CARTESIAN_POINT('Ctrl Pts',(3.98260264499999,1.732716033,-6.356184177));
#133101=CARTESIAN_POINT('Ctrl Pts',(3.888146516,1.715323387,-6.41344811100001));
#133102=CARTESIAN_POINT('',(3.72067285279307,1.71532338778839,-6.36652133995858));
#133103=CARTESIAN_POINT('Ctrl Pts',(3.553199198,1.715323387,-6.319594564));
#133104=CARTESIAN_POINT('Ctrl Pts',(3.211097032,1.779910221,-6.511941894));
#133105=CARTESIAN_POINT('Ctrl Pts',(2.850229985,1.845052736,-6.66623499700001));
#133106=CARTESIAN_POINT('Ctrl Pts',(3.459345652,1.715323387,-6.654541882));
#133107=CARTESIAN_POINT('Ctrl Pts',(3.099111595,1.779910221,-6.84180858500001));
#133108=CARTESIAN_POINT('Ctrl Pts',(2.720767072,1.845052736,-6.989093399));
#133109=CARTESIAN_POINT('',(3.4593456554125,1.7153233874486,-6.65454188146125));
#133110=CARTESIAN_POINT('',(2.95159230918543,1.80506741736312,-6.89478809203611));
#133111=CARTESIAN_POINT('Origin',(-0.0645203327015181,1.87497455206243,
0.179237619153348));
#133112=CARTESIAN_POINT('Ctrl Pts',(2.85453685143102,1.84427517369847,-6.66439189757178));
#133113=CARTESIAN_POINT('Ctrl Pts',(2.87072312970937,1.83740483635783,-6.70271935640467));
#133114=CARTESIAN_POINT('Ctrl Pts',(2.88691245442373,1.83070797872001,-6.74110504825094));
#133115=CARTESIAN_POINT('Ctrl Pts',(2.91925780734436,1.81765000115226,-6.81789104434923));
#133116=CARTESIAN_POINT('Ctrl Pts',(2.93543301336312,1.81128114575983,-6.85633688103594));
#133117=CARTESIAN_POINT('Ctrl Pts',(2.9515923118759,1.80506741744797,-6.89478809091914));
#133118=CARTESIAN_POINT('',(3.50627243214405,1.71532338830053,-6.48706821913863));
#133119=CARTESIAN_POINT('Origin',(1.26634813746307E-13,1.80614392399972,
-3.70363462121048E-13));
#133120=CARTESIAN_POINT('',(2.94793442701481,1.62564958720091,-6.89635284844599));
#133121=CARTESIAN_POINT('Origin',(-0.0515325910989406,1.48225709321937,
0.178790863984528));
#133122=CARTESIAN_POINT('',(2.41854204810154,1.71532338734699,-7.09934182683035));
#133123=CARTESIAN_POINT('Origin',(-0.0349672952353988,1.87485305299441,
0.18147657222317));
#133124=CARTESIAN_POINT('Ctrl Pts',(2.9515923069852,1.80506741664557,-6.89478809282103));
#133125=CARTESIAN_POINT('Ctrl Pts',(2.844039395054,1.78658581166052,-6.940830457713));
#133126=CARTESIAN_POINT('Ctrl Pts',(2.73563321256291,1.76822051522611,-6.98425873842889));
#133127=CARTESIAN_POINT('Ctrl Pts',(2.62656341956293,1.75000000000633,-7.02503840575027));
#133128=CARTESIAN_POINT('Ctrl Pts',(2.55770200869291,1.73849644465536,-7.05078472224044));
#133129=CARTESIAN_POINT('Ctrl Pts',(2.48834781076598,1.72693520694185,-7.07556100547006));
#133130=CARTESIAN_POINT('Ctrl Pts',(2.41854204925877,1.71532338729505,-7.09934182512115));
#133131=CARTESIAN_POINT('Ctrl Pts',(2.85891846,1.845058467,-6.662513432));
#133132=CARTESIAN_POINT('Ctrl Pts',(2.591107176,1.797173233,-6.777432619));
#133133=CARTESIAN_POINT('Ctrl Pts',(2.314936093,1.75,-6.870485491));
#133134=CARTESIAN_POINT('Ctrl Pts',(2.213748799,1.732716033,-6.90457946));
#133135=CARTESIAN_POINT('Ctrl Pts',(2.11160135,1.715323387,-6.935678751));
#133136=CARTESIAN_POINT('Ctrl Pts',(3.181945371,1.845058467,-6.791555319));
#133137=CARTESIAN_POINT('Ctrl Pts',(2.908947024,1.797173233,-6.919459133));
#133138=CARTESIAN_POINT('Ctrl Pts',(2.62656342,1.75,-7.025038406));
#133139=CARTESIAN_POINT('Ctrl Pts',(2.523099898,1.732716033,-7.063721967));
#133140=CARTESIAN_POINT('Ctrl Pts',(2.418542048,1.715323387,-7.099341826));
#133141=CARTESIAN_POINT('',(2.2650716943629,1.71532338778839,-7.01751028999674));
#133142=CARTESIAN_POINT('Ctrl Pts',(2.11160135,1.715323387,-6.935678751));
#133143=CARTESIAN_POINT('Ctrl Pts',(1.736148353,1.779910221,-7.049987254));
#133144=CARTESIAN_POINT('Ctrl Pts',(1.35054972,1.845052736,-7.123097322));
#133145=CARTESIAN_POINT('Ctrl Pts',(1.947938275,1.715323387,-7.242619448));
#133146=CARTESIAN_POINT('Ctrl Pts',(1.555869484,1.779910221,-7.348068286));
#133147=CARTESIAN_POINT('Ctrl Pts',(1.154708565,1.845052736,-7.410576774));
#133148=CARTESIAN_POINT('',(1.94793827842462,1.71532338744861,-7.24261944822413));
#133149=CARTESIAN_POINT('',(1.40041008981262,1.80506741730835,-7.36809687579697));
#133150=CARTESIAN_POINT('Origin',(-0.0244810838891019,1.87497458259997,
0.188917070257419));
#133151=CARTESIAN_POINT('Ctrl Pts',(1.35515210599349,1.84427517370281,-7.12222316244358));
#133152=CARTESIAN_POINT('Ctrl Pts',(1.36272068687216,1.83740483687102,-7.163134114833));
#133153=CARTESIAN_POINT('Ctrl Pts',(1.37027972446643,1.83070797976688,-7.20410259313213));
#133154=CARTESIAN_POINT('Ctrl Pts',(1.38536214280713,1.81765000114587,-7.28604667632506));
#133155=CARTESIAN_POINT('Ctrl Pts',(1.39289446305999,1.81128114571295,-7.32707086193457));
#133156=CARTESIAN_POINT('Ctrl Pts',(1.40041009257676,1.80506741738948,-7.36809687530289));
#133157=CARTESIAN_POINT('',(2.0297698203071,1.71532338830053,-7.08914909726467));
#133158=CARTESIAN_POINT('Origin',(5.0415401020576E-15,1.80614392400089,
1.70002900645727E-13));
#133159=CARTESIAN_POINT('',(1.39650135063366,1.6256495872356,-7.36883871276101));
#133160=CARTESIAN_POINT('Origin',(-0.0118930177375121,1.48225706706544,
0.185688717421748));
#133161=CARTESIAN_POINT('',(0.835849240922742,1.71532338734683,-7.4532782088336));
#133162=CARTESIAN_POINT('Origin',(0.00486236476819724,1.87485299080187,
0.184750327284376));
#133163=CARTESIAN_POINT('Ctrl Pts',(1.40041008758366,1.80506741661815,-7.36809687607145));
#133164=CARTESIAN_POINT('Ctrl Pts',(1.2854739556344,1.78658581163196,-7.38994209922501));
#133165=CARTESIAN_POINT('Ctrl Pts',(1.17026645276057,1.76822051520721,-7.40905092596894));
#133166=CARTESIAN_POINT('Ctrl Pts',(1.05498022756264,1.7499999999812,-7.42543040576093));
#133167=CARTESIAN_POINT('Ctrl Pts',(0.982194060839949,1.73849644461428,
-7.43577161995214));
#133168=CARTESIAN_POINT('Ctrl Pts',(0.909135157054965,1.72693520694186,
-7.44505954502194));
#133169=CARTESIAN_POINT('Ctrl Pts',(0.83584924241827,1.71532338729505,-7.45327820741229));
#133170=CARTESIAN_POINT('Ctrl Pts',(1.35983509,1.845058467,-7.121330531));
#133171=CARTESIAN_POINT('Ctrl Pts',(1.073580856,1.797173233,-7.175991461));
#133172=CARTESIAN_POINT('Ctrl Pts',(0.783862884,1.75,-7.207500189));
#133173=CARTESIAN_POINT('Ctrl Pts',(0.677712097,1.732716033,-7.21904478299999));
#133174=CARTESIAN_POINT('Ctrl Pts',(0.57126737,1.715323387,-7.227458308));
#133175=CARTESIAN_POINT('Ctrl Pts',(1.64756962,1.845058467,-7.316796727));
#133176=CARTESIAN_POINT('Ctrl Pts',(1.353458284,1.797173233,-7.383023646));
#133177=CARTESIAN_POINT('Ctrl Pts',(1.054980228,1.75,-7.425430406));
#133178=CARTESIAN_POINT('Ctrl Pts',(0.945619802999998,1.732716033,-7.440967968));
#133179=CARTESIAN_POINT('Ctrl Pts',(0.835849241000001,1.715323387,-7.453278208));
#133180=CARTESIAN_POINT('',(0.703558300649563,1.71532338778839,-7.3403682584649));
#133181=CARTESIAN_POINT('Ctrl Pts',(0.57126737,1.715323387,-7.227458308));
#133182=CARTESIAN_POINT('Ctrl Pts',(0.180019305,1.779910221,-7.258383046));
#133183=CARTESIAN_POINT('Ctrl Pts',(-0.212280749,1.845052736,-7.246891532));
#133184=CARTESIAN_POINT('Ctrl Pts',(0.34544747,1.715323387,-7.49204017899999));
#133185=CARTESIAN_POINT('Ctrl Pts',(-0.0601233540000001,1.779910221,-7.510740481));
#133186=CARTESIAN_POINT('Ctrl Pts',(-0.465342831,1.845052736,-7.485549816));
#133187=CARTESIAN_POINT('Ctrl Pts',(-0.207598045964949,1.84427517368269,
-7.24702718706223));
#133188=CARTESIAN_POINT('Ctrl Pts',(-0.209001059456788,1.83740483775766,
-7.28860867995657));
#133189=CARTESIAN_POINT('Ctrl Pts',(-0.210425759463398,1.83070798161786,
-7.33024430134279));
#133190=CARTESIAN_POINT('Ctrl Pts',(-0.213311515592232,1.81765000115136,
-7.41351486354743));
#133191=CARTESIAN_POINT('Ctrl Pts',(-0.214774283997516,1.81128114568937,
-7.45519915300969));
#133192=CARTESIAN_POINT('Ctrl Pts',(-0.216253745842921,1.80506741735323,
-7.49688163937647));
#133193=CARTESIAN_POINT('',(0.458357428105106,1.71532338830053,-7.35974924299522));
#133194=CARTESIAN_POINT('Ctrl Pts',(-0.202832658,1.845058467,-7.247162128));
#133195=CARTESIAN_POINT('Ctrl Pts',(-0.494144911,1.797173233,-7.23900891800001));
#133196=CARTESIAN_POINT('Ctrl Pts',(-0.783862884,1.75,-7.207500189));
#133197=CARTESIAN_POINT('Ctrl Pts',(-0.890013671,1.732716033,-7.195955596));
#133198=CARTESIAN_POINT('Ctrl Pts',(-0.995778438,1.715323387,-7.18128994700001));
#133199=CARTESIAN_POINT('Ctrl Pts',(0.036155345,1.845058467,-7.499912852));
#133200=CARTESIAN_POINT('Ctrl Pts',(-0.265316662,1.797173233,-7.501366179));
#133201=CARTESIAN_POINT('Ctrl Pts',(-0.565932667,1.75,-7.478617534));
#133202=CARTESIAN_POINT('Ctrl Pts',(-0.676076422,1.732716033,-7.470282578));
#133203=CARTESIAN_POINT('Ctrl Pts',(-0.785926947,1.715323387,-7.458707585));
#133204=CARTESIAN_POINT('',(-0.890852697336977,1.71532338778839,-7.31999876541133));
#133205=CARTESIAN_POINT('Ctrl Pts',(-0.995778438,1.715323387,-7.181289947));
#133206=CARTESIAN_POINT('Ctrl Pts',(-1.384527244,1.779910221,-7.127384913));
#133207=CARTESIAN_POINT('Ctrl Pts',(-1.765185206,1.845052736,-7.03182915));
#133208=CARTESIAN_POINT('Ctrl Pts',(-1.273196075,1.715323387,-7.391141438));
#133209=CARTESIAN_POINT('Ctrl Pts',(-1.673304891,1.779910221,-7.322218799));
#133210=CARTESIAN_POINT('Ctrl Pts',(-2.063635314,1.845052736,-7.210506868));
#133211=CARTESIAN_POINT('',(-1.27319607194735,1.71532338744859,-7.39114143963449));
#133212=CARTESIAN_POINT('',(-1.82280580273647,1.8050674173212,-7.27512054905735));
#133213=CARTESIAN_POINT('Origin',(0.0571057831376345,1.87497457696,0.181735794365157));
#133214=CARTESIAN_POINT('Ctrl Pts',(-1.76064114318867,1.84427517368998,
-7.03296827585413));
#133215=CARTESIAN_POINT('Ctrl Pts',(-1.77095014927405,1.83740483626804,
-7.07327601879132));
#133216=CARTESIAN_POINT('Ctrl Pts',(-1.78129197126079,1.83070797853862,
-7.11363196432593));
#133217=CARTESIAN_POINT('Ctrl Pts',(-1.8020109648533,1.81765000112568,-7.19433533587172));
#133218=CARTESIAN_POINT('Ctrl Pts',(-1.81240042460075,1.81128114572588,
-7.23473061744994));
#133219=CARTESIAN_POINT('Ctrl Pts',(-1.82280579992674,1.80506741740548,
-7.27512054979416));
#133220=CARTESIAN_POINT('',(-1.13448724847587,1.71532338830053,-7.28621569374938));
#133221=CARTESIAN_POINT('Origin',(-2.75387351811318E-14,1.80614392399994,
-5.09575021068187E-13));
#133222=CARTESIAN_POINT('',(-1.82666476757934,1.6256495872379,-7.27415258434626));
#133223=CARTESIAN_POINT('Origin',(0.0671749039816039,1.48225703765185,0.173520398716352));
#133224=CARTESIAN_POINT('',(-2.37095406541176,1.71532338734599,-7.11537608473305));
#133225=CARTESIAN_POINT('Origin',(0.081987519381812,1.8748529725513,0.165632892873371));
#133226=CARTESIAN_POINT('Ctrl Pts',(-1.82280580495611,1.80506741660434,
-7.27512054836361));
#133227=CARTESIAN_POINT('Ctrl Pts',(-1.93629158428473,1.78658581163235,
-7.24668630654801));
#133228=CARTESIAN_POINT('Ctrl Pts',(-2.04887467011018,1.76822051521175,
-7.21565463296981));
#133229=CARTESIAN_POINT('Ctrl Pts',(-2.16038317911473,1.750000000003,-7.18211281673717));
#133230=CARTESIAN_POINT('Ctrl Pts',(-2.23078427757153,1.73849644464992,
-7.16093613064846));
#133231=CARTESIAN_POINT('Ctrl Pts',(-2.30099064162491,1.72693520694186,
-7.13868898533399));
#133232=CARTESIAN_POINT('Ctrl Pts',(-2.37095406346605,1.71532338729505,
-7.11537608406213));
#133233=CARTESIAN_POINT('Ctrl Pts',(-1.756016176,1.845058467,-7.034124479));
#133234=CARTESIAN_POINT('Ctrl Pts',(-2.038765011,1.797173233,-6.96353836300001));
#133235=CARTESIAN_POINT('Ctrl Pts',(-2.314936093,1.75,-6.870485491));
#133236=CARTESIAN_POINT('Ctrl Pts',(-2.416123388,1.732716033,-6.836391522));
#133237=CARTESIAN_POINT('Ctrl Pts',(-2.516262752,1.715323387,-6.79933245));
#133238=CARTESIAN_POINT('Ctrl Pts',(-1.576949515,1.845058467,-7.332341388));
#133239=CARTESIAN_POINT('Ctrl Pts',(-1.871685696,1.797173233,-7.268953167));
#133240=CARTESIAN_POINT('Ctrl Pts',(-2.160383179,1.75,-7.182112817));
#133241=CARTESIAN_POINT('Ctrl Pts',(-2.266160065,1.732716033,-7.150295076));
#133242=CARTESIAN_POINT('Ctrl Pts',(-2.370954065,1.715323387,-7.115376084));
#133243=CARTESIAN_POINT('',(-2.44360841309735,1.71532338778839,-6.95735426538529));
#133244=CARTESIAN_POINT('Ctrl Pts',(-2.516262752,1.715323387,-6.79933245));
#133245=CARTESIAN_POINT('Ctrl Pts',(-2.884334839,1.779910221,-6.663118183));
#133246=CARTESIAN_POINT('Ctrl Pts',(-3.235551564,1.845052736,-6.487966251));
#133247=CARTESIAN_POINT('Ctrl Pts',(-2.832306387,1.715323387,-6.944641137));
#133248=CARTESIAN_POINT('Ctrl Pts',(-3.208244551,1.779910221,-6.791318303));
#133249=CARTESIAN_POINT('Ctrl Pts',(-3.565434502,1.845052736,-6.598308633));
#133250=CARTESIAN_POINT('',(-2.83230638441011,1.71532338744861,-6.9446411392509));
#133251=CARTESIAN_POINT('',(-3.34412548260674,1.80506741730588,-6.71318290765383));
#133252=CARTESIAN_POINT('Origin',(0.0948385256196937,1.87497459905246,0.165210909860477));
#133253=CARTESIAN_POINT('Ctrl Pts',(-3.23135861816427,1.8442751737878,-6.49005558377446));
#133254=CARTESIAN_POINT('Ctrl Pts',(-3.25009157661077,1.83740483705531,
-6.52720481882866));
#133255=CARTESIAN_POINT('Ctrl Pts',(-3.26886694551241,1.83070798005969,
-6.56439407438189));
#133256=CARTESIAN_POINT('Ctrl Pts',(-3.30645038374621,1.81765000117055,
-6.63875668311628));
#133257=CARTESIAN_POINT('Ctrl Pts',(-3.32528073507912,1.81128114574275,
-6.67597411881968));
#133258=CARTESIAN_POINT('Ctrl Pts',(-3.34412548002259,1.80506741739003,
-6.71318290897665));
#133259=CARTESIAN_POINT('',(-2.67428456193206,1.71532338830053,-6.87198679644513));
#133260=CARTESIAN_POINT('Origin',(5.24103330179493E-13,1.80614392400078,
1.3240276930393E-12));
#133261=CARTESIAN_POINT('',(-3.3476861434657,1.62564958723185,-6.71140801018691));
#133262=CARTESIAN_POINT('Origin',(0.102905981622565,1.48225706127344,0.155022634375567));
#133263=CARTESIAN_POINT('',(-3.84511800556868,1.7153233873472,-6.43933750761235));
#133264=CARTESIAN_POINT('Origin',(0.115677207984717,1.87485304760366,0.144136193360177));
#133265=CARTESIAN_POINT('Ctrl Pts',(-3.34412548462044,1.80506741659049,
-6.71318290649401));
#133266=CARTESIAN_POINT('Ctrl Pts',(-3.44884550812391,1.78658581162302,
-6.66101735348689));
#133267=CARTESIAN_POINT('Ctrl Pts',(-3.55212557167422,1.76822051520746,
-6.60650914783531));
#133268=CARTESIAN_POINT('Ctrl Pts',(-3.65381657476143,1.75000000007832,
-6.54978048744543));
#133269=CARTESIAN_POINT('Ctrl Pts',(-3.71801937267495,1.73849644477304,
-6.51396474497676));
#133270=CARTESIAN_POINT('Ctrl Pts',(-3.78180187253556,1.72693520694185,
-6.4771454331214));
#133271=CARTESIAN_POINT('Ctrl Pts',(-3.84511800351527,1.71532338729505,
-6.43933750739044));
#133272=CARTESIAN_POINT('Ctrl Pts',(-3.22709033,1.845058467,-6.492178987));
#133273=CARTESIAN_POINT('Ctrl Pts',(-3.488054726,1.797173233,-6.362460494));
#133274=CARTESIAN_POINT('Ctrl Pts',(-3.737765465,1.75,-6.212214527));
#133275=CARTESIAN_POINT('Ctrl Pts',(-3.82925786,1.732716033,-6.157165379));
#133276=CARTESIAN_POINT('Ctrl Pts',(-3.919089417,1.715323387,-6.099445724));
#133277=CARTESIAN_POINT('Ctrl Pts',(-3.116317967,1.845058467,-6.82191779));
#133278=CARTESIAN_POINT('Ctrl Pts',(-3.390536786,1.797173233,-6.69665198300001));
#133279=CARTESIAN_POINT('Ctrl Pts',(-3.653816575,1.75,-6.549780488));
#133280=CARTESIAN_POINT('Ctrl Pts',(-3.750280582,1.732716033,-6.495967724));
#133281=CARTESIAN_POINT('Ctrl Pts',(-3.845118005,1.715323387,-6.439337507));
#133282=CARTESIAN_POINT('',(-3.88210371514274,1.71532338778839,-6.26939161293474));
#133283=CARTESIAN_POINT('Ctrl Pts',(-3.919089417,1.715323387,-6.09944572399999));
#133284=CARTESIAN_POINT('Ctrl Pts',(-4.249274143,1.779910221,-5.887291453));
#133285=CARTESIAN_POINT('Ctrl Pts',(-4.554627128,1.845052736,-5.640733261));
#133286=CARTESIAN_POINT('Ctrl Pts',(-4.2589812,1.715323387,-6.173417136));
#133287=CARTESIAN_POINT('Ctrl Pts',(-4.593170261,1.779910221,-5.942863312));
#133288=CARTESIAN_POINT('Ctrl Pts',(-4.900517936,1.845052736,-5.677580819));
#133289=CARTESIAN_POINT('',(-4.25898119793413,1.7153233874486,-6.17341713876038));
#133290=CARTESIAN_POINT('',(-4.70907757189762,1.80506741732327,-5.83734429464129));
#133291=CARTESIAN_POINT('Origin',(0.128136703404839,1.87497456693746,0.140960870615262));
#133292=CARTESIAN_POINT('Ctrl Pts',(-4.55098135569827,1.84427517364945,
-5.6436751063504));
#133293=CARTESIAN_POINT('Ctrl Pts',(-4.57726232901562,1.83740483857874,
-5.67592877290656));
#133294=CARTESIAN_POINT('Ctrl Pts',(-4.60359332343685,1.83070798334266,
-5.7082124060049));
#133295=CARTESIAN_POINT('Ctrl Pts',(-4.65628385777715,1.81765000116681,
-5.77275714641575));
#133296=CARTESIAN_POINT('Ctrl Pts',(-4.68267461446684,1.81128114574686,
-5.80505649027571));
#133297=CARTESIAN_POINT('Ctrl Pts',(-4.70907756966156,1.80506741740742,
-5.837344296486));
#133298=CARTESIAN_POINT('',(-4.08903530174211,1.71532338830053,-6.13643143450315));
#133299=CARTESIAN_POINT('Origin',(6.15393153102772E-13,1.80614392400067,
8.7733639797527E-13));
#133300=CARTESIAN_POINT('',(-4.71217343633271,1.62564958722512,-5.83484545661086));
#133301=CARTESIAN_POINT('Origin',(0.133825473295058,1.48225708072422,0.129276671077776));
#133302=CARTESIAN_POINT('',(-5.13948850268995,1.71532338734785,-5.46220266446694));
#133303=CARTESIAN_POINT('Origin',(0.143957591572755,1.87485301735426,0.115899004336963));
#133304=CARTESIAN_POINT('Ctrl Pts',(-4.70907757360896,1.80506741660989,
-5.83734429307193));
#133305=CARTESIAN_POINT('Ctrl Pts',(-4.80013524921256,1.78658581163547,
-5.76388663229429));
#133306=CARTESIAN_POINT('Ctrl Pts',(-4.88928302912086,1.76822051521265,
-5.68845063738575));
#133307=CARTESIAN_POINT('Ctrl Pts',(-4.97640156834857,1.74999999992805,
-5.61118770152768));
#133308=CARTESIAN_POINT('Ctrl Pts',(-5.03140401600431,1.73849644452739,
-5.56240760784191));
#133309=CARTESIAN_POINT('Ctrl Pts',(-5.08578025209878,1.72693520694185,
-5.51273775897613));
#133310=CARTESIAN_POINT('Ctrl Pts',(-5.13948850063391,1.71532338729505,
-5.46220266470048));
#133311=CARTESIAN_POINT('Ctrl Pts',(-4.54726932600001,1.845058467,-5.646666422));
#133312=CARTESIAN_POINT('Ctrl Pts',(-4.77424687800001,1.797173233,-5.463881043));
#133313=CARTESIAN_POINT('Ctrl Pts',(-4.985821077,1.75,-5.263467316));
#133314=CARTESIAN_POINT('Ctrl Pts',(-5.063340492,1.732716033,-5.190037026));
#133315=CARTESIAN_POINT('Ctrl Pts',(-5.138663817,1.715323387,-5.114355695));
#133316=CARTESIAN_POINT('Ctrl Pts',(-4.509970855,1.845058467,-5.992508897));
#133317=CARTESIAN_POINT('Ctrl Pts',(-4.75085014500001,1.797173233,-5.811222796));
#133318=CARTESIAN_POINT('Ctrl Pts',(-4.976401568,1.75,-5.611187702));
#133319=CARTESIAN_POINT('Ctrl Pts',(-5.059042148,1.732716033,-5.537896141));
#133320=CARTESIAN_POINT('Ctrl Pts',(-5.139488502,1.715323387,-5.462202664));
#133321=CARTESIAN_POINT('',(-5.13907616299444,1.71532338778839,-5.28827917610415));
#133322=CARTESIAN_POINT('Ctrl Pts',(-5.138663817,1.715323387,-5.114355695));
#133323=CARTESIAN_POINT('Ctrl Pts',(-5.41552211,1.779910221,-4.836181517));
#133324=CARTESIAN_POINT('Ctrl Pts',(-5.660733389,1.845052736,-4.529745854));
#133325=CARTESIAN_POINT('Ctrl Pts',(-5.486510786,1.715323387,-5.11353101));
#133326=CARTESIAN_POINT('Ctrl Pts',(-5.763324435,1.779910221,-4.816526637));
#133327=CARTESIAN_POINT('Ctrl Pts',(-6.006458598,1.845052736,-4.491375636));
#133328=CARTESIAN_POINT('',(-5.48651078462152,1.7153233873907,-5.11353101378422));
#133329=CARTESIAN_POINT('',(-5.85383842782573,1.80506741729938,-4.68855794995681));
#133330=CARTESIAN_POINT('Origin',(0.155443364178303,1.87497454573908,0.110119684231014));
#133331=CARTESIAN_POINT('Ctrl Pts',(-5.65780526184909,1.84427517371848,
-4.53340265369336));
#133332=CARTESIAN_POINT('Ctrl Pts',(-5.69040539293009,1.83740483709969,
-4.55925262052202));
#133333=CARTESIAN_POINT('Ctrl Pts',(-5.72306081876345,1.83070798022868,
-4.58512110127154));
#133334=CARTESIAN_POINT('Ctrl Pts',(-5.78839467371819,1.81765000111874,
-4.63682990163741));
#133335=CARTESIAN_POINT('Ctrl Pts',(-5.82111183336738,1.8112811457063,-4.66270087204328));
#133336=CARTESIAN_POINT('Ctrl Pts',(-5.85383842605123,1.80506741738274,
-4.68855795222277));
#133337=CARTESIAN_POINT('',(-5.31258729586815,1.71532338830053,-5.11394335885062));
#133338=CARTESIAN_POINT('Origin',(3.67327696038089E-13,1.80614392400011,
2.68882138776405E-13));
#133339=CARTESIAN_POINT('',(-5.85632473619675,1.6256495871923,-4.68545201434567));
#133340=CARTESIAN_POINT('Origin',(0.158487672707834,1.48225704678402,0.0974859784145793));
#133341=CARTESIAN_POINT('',(-6.19354222877295,1.71532338734701,-4.2296612953197));
#133342=CARTESIAN_POINT('Origin',(0.165506588390246,1.87485294691966,0.082242575767319));
#133343=CARTESIAN_POINT('Ctrl Pts',(-5.85383842914288,1.80506741659236,
-4.68855794806636));
#133344=CARTESIAN_POINT('Ctrl Pts',(-5.9269760013645,1.78658581162182,-4.5972429780145));
#133345=CARTESIAN_POINT('Ctrl Pts',(-5.99782304696224,1.76822051520559,
-4.50440649736151));
#133346=CARTESIAN_POINT('Ctrl Pts',(-6.06629555573099,1.75000000004347,
-4.41022201567403));
#133347=CARTESIAN_POINT('Ctrl Pts',(-6.10952579750693,1.73849644471606,
-4.35075847315401));
#133348=CARTESIAN_POINT('Ctrl Pts',(-6.15195319866596,1.72693520694185,
-4.29056059386023));
#133349=CARTESIAN_POINT('Ctrl Pts',(-6.19354222681643,1.71532338729505,
-4.22966129597777));
#133350=CARTESIAN_POINT('Ctrl Pts',(-5.654823062,1.845058467,-4.53712201));
#133351=CARTESIAN_POINT('Ctrl Pts',(-5.837200552,1.797173233,-4.309816588));
#133352=CARTESIAN_POINT('Ctrl Pts',(-6.000745237,1.75,-4.068606224));
#133353=CARTESIAN_POINT('Ctrl Pts',(-6.06066694900001,1.732716033,-3.98022831));
#133354=CARTESIAN_POINT('Ctrl Pts',(-6.117960008,1.715323387,-3.890124078));
#133355=CARTESIAN_POINT('Ctrl Pts',(-5.692742518,1.845058467,-4.882896949));
#133356=CARTESIAN_POINT('Ctrl Pts',(-5.889019031,1.797173233,-4.654067289));
#133357=CARTESIAN_POINT('Ctrl Pts',(-6.066295556,1.75,-4.410222016));
#133358=CARTESIAN_POINT('Ctrl Pts',(-6.131248525,1.732716033,-4.320878689));
#133359=CARTESIAN_POINT('Ctrl Pts',(-6.193542228,1.715323387,-4.229661295));
#133360=CARTESIAN_POINT('',(-6.15575112068274,1.71532338778839,-4.05989268243235));
#133361=CARTESIAN_POINT('Ctrl Pts',(-6.117960008,1.715323387,-3.890124078));
#133362=CARTESIAN_POINT('Ctrl Pts',(-6.328546282,1.779910221,-3.558937109));
#133363=CARTESIAN_POINT('Ctrl Pts',(-6.502150048,1.845052736,-3.206952564));
#133364=CARTESIAN_POINT('Ctrl Pts',(-6.457497225,1.715323387,-3.814541858));
#133365=CARTESIAN_POINT('Ctrl Pts',(-6.663991964,1.779910221,-3.46497453));
#133366=CARTESIAN_POINT('Ctrl Pts',(-6.83154393200001,1.845052736,-3.095158721));
#133367=CARTESIAN_POINT('',(-6.45749722428321,1.7153233874486,-3.81454186137344));
#133368=CARTESIAN_POINT('',(-6.72488030527665,1.80506741733644,-3.32053984683611));
#133369=CARTESIAN_POINT('Origin',(0.175481749968587,1.87497455746621,0.0741294710234985));
#133370=CARTESIAN_POINT('Ctrl Pts',(-6.5000764830721,1.84427517365532,-3.21115333069245));
#133371=CARTESIAN_POINT('Ctrl Pts',(-6.53747141464812,1.83740483805641,
-3.22939087266828));
#133372=CARTESIAN_POINT('Ctrl Pts',(-6.57492432724293,1.83070798225605,
-3.24763460848772));
#133373=CARTESIAN_POINT('Ctrl Pts',(-6.64984658819208,1.81765000117118,
-3.28408964401682));
#133374=CARTESIAN_POINT('Ctrl Pts',(-6.6873603328519,1.81128114575583,-3.30232254337401));
#133375=CARTESIAN_POINT('Ctrl Pts',(-6.7248803040286,1.80506741742015,-3.3205398494351));
#133376=CARTESIAN_POINT('',(-6.28772861225752,1.71532338830053,-3.85233297492452));
#133377=CARTESIAN_POINT('Origin',(-4.49293380277993E-13,1.80614392399933,
-2.08600497986211E-13));
#133378=CARTESIAN_POINT('',(-6.72664080054466,1.62564958722407,-3.3169720436542));
#133379=CARTESIAN_POINT('Origin',(0.175738525450879,1.48225710692865,0.0611364500891559));
#133380=CARTESIAN_POINT('',(-6.95799280382239,1.71532338734776,-2.79934566613531));
#133381=CARTESIAN_POINT('Origin',(0.179317325664667,1.87485305229205,0.0447409567436702));
#133382=CARTESIAN_POINT('Ctrl Pts',(-6.72488030617135,1.80506741662604,
-3.32053984470728));
#133383=CARTESIAN_POINT('Ctrl Pts',(-6.77667794310486,1.78658581164461,
-3.21563735165099));
#133384=CARTESIAN_POINT('Ctrl Pts',(-6.82591152482656,1.7682205152171,-3.10974131575523));
#133385=CARTESIAN_POINT('Ctrl Pts',(-6.87253630462811,1.75000000004312,
-3.0030392496445));
#133386=CARTESIAN_POINT('Ctrl Pts',(-6.90197294320774,1.7384964447155,-2.9356727075413));
#133387=CARTESIAN_POINT('Ctrl Pts',(-6.93046765080973,1.72693520694185,
-2.86776158452171));
#133388=CARTESIAN_POINT('Ctrl Pts',(-6.95799280205429,1.71532338729505,
-2.79934566720934));
#133389=CARTESIAN_POINT('Ctrl Pts',(-6.497963557,1.845058467,-3.215426816));
#133390=CARTESIAN_POINT('Ctrl Pts',(-6.627213216,1.797173233,-2.954229899));
#133391=CARTESIAN_POINT('Ctrl Pts',(-6.735081219,1.75,-2.683501626));
#133392=CARTESIAN_POINT('Ctrl Pts',(-6.77460335600001,1.732716033,-2.584308542));
#133393=CARTESIAN_POINT('Ctrl Pts',(-6.811187188,1.715323387,-2.483994583));
#133394=CARTESIAN_POINT('Ctrl Pts',(-6.609327869,1.845058467,-3.544966167));
#133395=CARTESIAN_POINT('Ctrl Pts',(-6.75182393300001,1.797173233,-3.279292768));
#133396=CARTESIAN_POINT('Ctrl Pts',(-6.872536305,1.75,-3.00303925));
#133397=CARTESIAN_POINT('Ctrl Pts',(-6.916764535,1.732716033,-2.901821752));
#133398=CARTESIAN_POINT('Ctrl Pts',(-6.957992803,1.715323387,-2.799345666));
#133399=CARTESIAN_POINT('',(-6.88458999724559,1.71532338778839,-2.64167011995074));
#133400=CARTESIAN_POINT('Ctrl Pts',(-6.811187188,1.715323387,-2.483994583));
#133401=CARTESIAN_POINT('Ctrl Pts',(-6.945654664,1.779910221,-2.115280757));
#133402=CARTESIAN_POINT('Ctrl Pts',(-7.039533398,1.845052736,-1.734205737));
#133403=CARTESIAN_POINT('Ctrl Pts',(-7.126538271,1.715323387,-2.337188968));
#133404=CARTESIAN_POINT('Ctrl Pts',(-7.253058636,1.779910221,-1.951404065));
#133405=CARTESIAN_POINT('Ctrl Pts',(-7.337193864,1.845052736,-1.554215624));
#133406=CARTESIAN_POINT('',(-7.12653827101836,1.71532338744859,-2.33718897145734));
#133407=CARTESIAN_POINT('',(-7.28147425196933,1.80506741742003,-1.79725699571591));
#133408=CARTESIAN_POINT('Origin',(0.18731449796178,1.8749745675529,0.0346728987575037));
#133409=CARTESIAN_POINT('Ctrl Pts',(-7.03841135207602,1.84427517370752,
-1.73875404728259));
#133410=CARTESIAN_POINT('Ctrl Pts',(-7.07885255315508,1.8374048364221,-1.74852640324277));
#133411=CARTESIAN_POINT('Ctrl Pts',(-7.1193517128608,1.83070797883412,-1.75829234444339));
#133412=CARTESIAN_POINT('Ctrl Pts',(-7.20035906684401,1.81765000112338,
-1.7777890052515));
#133413=CARTESIAN_POINT('Ctrl Pts',(-7.24091529479374,1.81128114578685,
-1.78753128332844));
#133414=CARTESIAN_POINT('Ctrl Pts',(-7.28147425231075,1.80506741742304,
-1.79725699429402));
#133415=CARTESIAN_POINT('',(-6.96886272684528,1.71532338830053,-2.41059178317464));
#133416=CARTESIAN_POINT('Ctrl Pts',(-7.037266498,1.845058467,-1.743381837));
#133417=CARTESIAN_POINT('Ctrl Pts',(-7.10734475600001,1.797173233,-1.460506703));
#133418=CARTESIAN_POINT('Ctrl Pts',(-7.154492288,1.75,-1.172919475));
#133419=CARTESIAN_POINT('Ctrl Pts',(-7.171766839,1.732716033,-1.067549379));
#133420=CARTESIAN_POINT('Ctrl Pts',(-7.185930826,1.715323387,-0.961716262));
#133421=CARTESIAN_POINT('Ctrl Pts',(-7.216868393,1.845058467,-2.041276707));
#133422=CARTESIAN_POINT('Ctrl Pts',(-7.298921051,1.797173233,-1.751182163));
#133423=CARTESIAN_POINT('Ctrl Pts',(-7.357424895,1.75,-1.455437707));
#133424=CARTESIAN_POINT('Ctrl Pts',(-7.37886032399999,1.732716033,-1.347078855));
#133425=CARTESIAN_POINT('Ctrl Pts',(-7.397095368,1.715323387,-1.238135744));
#133426=CARTESIAN_POINT('',(-7.39709536883243,1.71532338734766,-1.23813574395633));
#133427=CARTESIAN_POINT('Ctrl Pts',(-7.28147425154384,1.80506741796643,
-1.79725699772192));
#133428=CARTESIAN_POINT('Ctrl Pts',(-7.30950995424651,1.78658581254366,
-1.68367210305473));
#133429=CARTESIAN_POINT('Ctrl Pts',(-7.33482796555722,1.7682205156674,-1.5696680900927));
#133430=CARTESIAN_POINT('Ctrl Pts',(-7.35742489468803,1.74999999998162,
-1.45543770641869));
#133431=CARTESIAN_POINT('Ctrl Pts',(-7.3716915062426,1.73849644461496,-1.38331814875904));
#133432=CARTESIAN_POINT('Ctrl Pts',(-7.38492113915213,1.72693520694185,
-1.31086923046406));
#133433=CARTESIAN_POINT('Ctrl Pts',(-7.39709536733612,1.71532338729505,
-1.23813574538403));
#133434=CARTESIAN_POINT('',(-7.29151309772682,1.71532338778839,-1.09992599818185));
#133435=CARTESIAN_POINT('Origin',(-1.04907402209697E-12,1.80614392399972,
-3.31657444563316E-13));
#133436=CARTESIAN_POINT('',(-7.2824266169875,1.62564958719531,-1.79339414632113));
#133437=CARTESIAN_POINT('Origin',(0.184772441701598,1.48225711658612,0.0219285383639398));
#133438=CARTESIAN_POINT('Origin',(0.184742667814161,1.87485301774908,0.00514695786866456));
#133439=CARTESIAN_POINT('Ctrl Pts',(-7.185930826,1.715323387,-0.961716262));
#133440=CARTESIAN_POINT('Ctrl Pts',(-7.237991953,1.779910221,-0.572716228));
#133441=CARTESIAN_POINT('Ctrl Pts',(-7.24775599,1.845052736,-0.180369377));
#133442=CARTESIAN_POINT('Ctrl Pts',(-7.462350308,1.715323387,-0.750551720000001));
#133443=CARTESIAN_POINT('Ctrl Pts',(-7.502980346,1.779910221,-0.346588114));
#133444=CARTESIAN_POINT('Ctrl Pts',(-7.49976476500001,1.845052736,0.059400869));
#133445=CARTESIAN_POINT('',(-7.46235030875524,1.71532338744859,-0.750551723384883));
#133446=CARTESIAN_POINT('',(-7.32414056605716,1.71532338830053,-0.856133999065891));
#133447=CARTESIAN_POINT('',(-7.49759455823745,1.80506741730981,-0.189936395315711));
#133448=CARTESIAN_POINT('Origin',(0.190388983215062,1.87497459522639,-0.00640480722740908));
#133449=CARTESIAN_POINT('Ctrl Pts',(-7.24763792913635,1.84427517364804,
-0.18505255738451));
#133450=CARTESIAN_POINT('Ctrl Pts',(-7.28923440489062,1.83740483639556,
-0.185902778062715));
#133451=CARTESIAN_POINT('Ctrl Pts',(-7.33088610523764,1.83070797884176,
-0.186734274565161));
#133452=CARTESIAN_POINT('Ctrl Pts',(-7.41419075820685,1.81765000112243,
-0.188360927322157));
#133453=CARTESIAN_POINT('Ctrl Pts',(-7.45589310646488,1.81128114570684,
-0.189157046000084));
#133454=CARTESIAN_POINT('Ctrl Pts',(-7.49759455819688,1.80506741739137,
-0.189936398137077));
#133455=CARTESIAN_POINT('Origin',(-8.14452671971111E-13,1.80614392400033,
-4.03052157621486E-14));
#133456=CARTESIAN_POINT('',(-7.49031797585143,1.71532338730065,0.380968029371306));
#133457=CARTESIAN_POINT('Ctrl Pts',(-7.49759455815538,1.80506741661502,
-0.189936393060656));
#133458=CARTESIAN_POINT('Ctrl Pts',(-7.50055740688098,1.78658581163115,
-0.0729802056970346));
#133459=CARTESIAN_POINT('Ctrl Pts',(-7.50077600416531,1.76822051520785,
0.0438010778798551));
#133460=CARTESIAN_POINT('Ctrl Pts',(-7.49828847350378,1.75000000007189,
0.160218486994678));
#133461=CARTESIAN_POINT('Ctrl Pts',(-7.49671796620267,1.73849644476259,
0.233718828343446));
#133462=CARTESIAN_POINT('Ctrl Pts',(-7.49406392199738,1.72693520698401,
0.307317911773481));
#133463=CARTESIAN_POINT('Ctrl Pts',(-7.49031797471166,1.71532338742604,
0.380968027657659));
#133464=CARTESIAN_POINT('',(-7.49769425871342,1.62564958721909,-0.185959132152087));
#133465=CARTESIAN_POINT('Origin',(0.185166703010033,1.48225708291231,-0.0183047507892071));
#133466=CARTESIAN_POINT('Origin',(0.181530033628547,1.87485303207714,-0.0346875888160002));
#133467=CARTESIAN_POINT('Ctrl Pts',(-7.247514679,1.845058467,-0.189818262));
#133468=CARTESIAN_POINT('Ctrl Pts',(-7.25514475400001,1.797173233,0.101508163));
#133469=CARTESIAN_POINT('Ctrl Pts',(-7.23936725,1.75,0.392507087));
#133470=CARTESIAN_POINT('Ctrl Pts',(-7.233586475,1.732716033,0.499127207));
#133471=CARTESIAN_POINT('Ctrl Pts',(-7.224668324,1.715323387,0.605530844));
#133472=CARTESIAN_POINT('Ctrl Pts',(-7.486956173,1.845058467,-0.442139416));
#133473=CARTESIAN_POINT('Ctrl Pts',(-7.504728734,1.797173233,-0.141188225));
#133474=CARTESIAN_POINT('Ctrl Pts',(-7.498288474,1.75,0.160218487));
#133475=CARTESIAN_POINT('Ctrl Pts',(-7.49592880400001,1.732716033,0.270651952));
#133476=CARTESIAN_POINT('Ctrl Pts',(-7.490317975,1.715323387,0.38096803));
#133477=CARTESIAN_POINT('',(-7.35749314923284,1.71532338764623,0.493249440985084));
#133478=CARTESIAN_POINT('Ctrl Pts',(-7.224668324,1.715323387,0.605530843));
#133479=CARTESIAN_POINT('Ctrl Pts',(-7.191888783,1.779910221,0.996627876));
#133480=CARTESIAN_POINT('Ctrl Pts',(-7.117081567,1.845052736,1.381900854));
#133481=CARTESIAN_POINT('Ctrl Pts',(-7.449231138,1.715323387,0.871180493));
#133482=CARTESIAN_POINT('Ctrl Pts',(-7.402071035,1.779910221,1.274433911));
#133483=CARTESIAN_POINT('Ctrl Pts',(-7.311655002,1.845052736,1.670239842));
#133484=CARTESIAN_POINT('',(-7.44923113946963,1.71532338744859,0.871180489875332));
#133485=CARTESIAN_POINT('',(-7.36313567458969,1.8050674173157,1.42626541414909));
#133486=CARTESIAN_POINT('Origin',(0.184560763126078,1.8749745822392,-0.0471830341014413));
#133487=CARTESIAN_POINT('Ctrl Pts',(-7.11797301180835,1.84427517372359,
1.37730178494788));
#133488=CARTESIAN_POINT('Ctrl Pts',(-7.15877975547646,1.83740483677234,
1.38541345408613));
#133489=CARTESIAN_POINT('Ctrl Pts',(-7.19963640712206,1.83070797954891,
1.39355528121711));
#133490=CARTESIAN_POINT('Ctrl Pts',(-7.28134313007023,1.81765000113501,
1.40987469709975));
#133491=CARTESIAN_POINT('Ctrl Pts',(-7.32224164240428,1.81128114574182,
1.41806196319935));
#133492=CARTESIAN_POINT('Ctrl Pts',(-7.3631356751902,1.8050674174027,1.42626541122143));
#133493=CARTESIAN_POINT('',(-7.33694973181313,1.71532338830053,0.738355659920048));
#133494=CARTESIAN_POINT('Origin',(3.1788807697275E-13,1.80614392400006,
-9.44340092234874E-14));
#133495=CARTESIAN_POINT('',(-7.36237804979227,1.62564958720817,1.43017112447915));
#133496=CARTESIAN_POINT('Origin',(0.176902554139877,1.48225709057109,-0.0576821485220025));
#133497=CARTESIAN_POINT('',(-7.23330163873855,1.71532338734751,1.98225816138769));
#133498=CARTESIAN_POINT('Origin',(0.169829105003895,1.87485302319861,-0.0729001907297283));
#133499=CARTESIAN_POINT('Ctrl Pts',(-7.36313567399073,1.80506741657942,
1.42626541646893));
#133500=CARTESIAN_POINT('Ctrl Pts',(-7.3408871297091,1.78658581162416,1.54112415805627));
#133501=CARTESIAN_POINT('Ctrl Pts',(-7.31599609245516,1.76822051521171,
1.65522215227455));
#133502=CARTESIAN_POINT('Ctrl Pts',(-7.28854041727265,1.75000000006627,
1.76838304205611));
#133503=CARTESIAN_POINT('Ctrl Pts',(-7.27120622654293,1.73849644475334,
1.83982737395459));
#133504=CARTESIAN_POINT('Ctrl Pts',(-7.25279260523698,1.72693520694185,
1.91113521043703));
#133505=CARTESIAN_POINT('Ctrl Pts',(-7.23330163797866,1.71532338729505,
1.9822581594651));
#133506=CARTESIAN_POINT('Ctrl Pts',(-7.118877129,1.845058467,1.372621005));
#133507=CARTESIAN_POINT('Ctrl Pts',(-7.063702247,1.797173233,1.65877662));
#133508=CARTESIAN_POINT('Ctrl Pts',(-6.985737446,1.75,1.939580454));
#133509=CARTESIAN_POINT('Ctrl Pts',(-6.957171648,1.732716033,2.042465159));
#133510=CARTESIAN_POINT('Ctrl Pts',(-6.92558836200001,1.715323387,2.144463998));
#133511=CARTESIAN_POINT('Ctrl Pts',(-7.406962203,1.845058467,1.177671822));
#133512=CARTESIAN_POINT('Ctrl Pts',(-7.359623641,1.797173233,1.475407516));
#133513=CARTESIAN_POINT('Ctrl Pts',(-7.288540418,1.75,1.768383042));
#133514=CARTESIAN_POINT('Ctrl Pts',(-7.262495985,1.732716033,1.875727375));
#133515=CARTESIAN_POINT('Ctrl Pts',(-7.23330163800001,1.715323387,1.982258161));
#133516=CARTESIAN_POINT('',(-7.07944499863658,1.71532338778837,2.06336108417793));
#133517=CARTESIAN_POINT('Ctrl Pts',(-6.925588362,1.715323387,2.144463998));
#133518=CARTESIAN_POINT('Ctrl Pts',(-6.809500887,1.779910221,2.519370767));
#133519=CARTESIAN_POINT('Ctrl Pts',(-6.65362032,1.845052736,2.879554937));
#133520=CARTESIAN_POINT('Ctrl Pts',(-7.0877942,1.715323387,2.452177274));
#133521=CARTESIAN_POINT('Ctrl Pts',(-6.955049108,1.779910221,2.835864823));
#133522=CARTESIAN_POINT('Ctrl Pts',(-6.781660377,1.845052736,3.202980258));
#133523=CARTESIAN_POINT('',(-7.08779420210665,1.71532338744858,2.45217727124133));
#133524=CARTESIAN_POINT('',(-6.88438475017486,1.80506741732249,2.97577663915184));
#133525=CARTESIAN_POINT('Origin',(0.170103244568237,1.87497457945223,-0.0857551769196505));
#133526=CARTESIAN_POINT('Ctrl Pts',(-6.65547958725748,1.8442751737515,2.8752550263023));
#133527=CARTESIAN_POINT('Ctrl Pts',(-6.69358851776623,1.83740483771236,
2.89194929058825));
#133528=CARTESIAN_POINT('Ctrl Pts',(-6.73173970549045,1.83070798145379,
2.90868373622113));
#133529=CARTESIAN_POINT('Ctrl Pts',(-6.80802798945147,1.81765000117156,
2.94218614845364));
#133530=CARTESIAN_POINT('Ctrl Pts',(-6.84621029723544,1.81128114574425,
2.95897397223806));
#133531=CARTESIAN_POINT('Ctrl Pts',(-6.88438475134653,1.80506741740601,
2.97577663652078));
#133532=CARTESIAN_POINT('',(-7.00669128353107,1.71532338830053,2.29832062828375));
#133533=CARTESIAN_POINT('Origin',(-1.26634813746307E-13,1.80614392400033,
1.52655665885959E-13));
#133534=CARTESIAN_POINT('',(-6.88280522652421,1.62564958718962,2.97942816863293));
#133535=CARTESIAN_POINT('Origin',(0.160366736514282,1.48225709015059,-0.0943624016382039));
#133536=CARTESIAN_POINT('',(-6.63806415663428,1.71532338734785,3.49086010453999));
#133537=CARTESIAN_POINT('Origin',(0.150187169775896,1.87485301589997,-0.107704045557256));
#133538=CARTESIAN_POINT('Ctrl Pts',(-6.88438474913271,1.80506741661292,
2.97577664120878));
#133539=CARTESIAN_POINT('Ctrl Pts',(-6.83796512925141,1.78658581163562,
3.08316726987123));
#133540=CARTESIAN_POINT('Ctrl Pts',(-6.78912833450483,1.76822051521236,
3.18924687890002));
#133541=CARTESIAN_POINT('Ctrl Pts',(-6.73798831140334,1.75000000001485,
3.29385997111074));
#133542=CARTESIAN_POINT('Ctrl Pts',(-6.70570096511747,1.73849644466928,
3.35990763580892));
#133543=CARTESIAN_POINT('Ctrl Pts',(-6.67238876701024,1.72693520694185,
3.42558995016916));
#133544=CARTESIAN_POINT('Ctrl Pts',(-6.63806415630943,1.71532338729505,
3.49086010249632));
#133545=CARTESIAN_POINT('Ctrl Pts',(-6.657368796,1.845058467,2.870878039));
#133546=CARTESIAN_POINT('Ctrl Pts',(-6.541968873,1.797173233,3.138482526));
#133547=CARTESIAN_POINT('Ctrl Pts',(-6.405462322,1.75,3.395961195));
#133548=CARTESIAN_POINT('Ctrl Pts',(-6.355447207,1.732716033,3.49029971));
#133549=CARTESIAN_POINT('Ctrl Pts',(-6.302675585,1.715323387,3.583124401));
#133550=CARTESIAN_POINT('Ctrl Pts',(-6.980626913,1.845058467,2.742416435));
#133551=CARTESIAN_POINT('Ctrl Pts',(-6.87039072700001,1.797173233,3.023014843));
#133552=CARTESIAN_POINT('Ctrl Pts',(-6.737988312,1.75,3.293859971));
#133553=CARTESIAN_POINT('Ctrl Pts',(-6.689476925,1.732716033,3.39309587));
#133554=CARTESIAN_POINT('Ctrl Pts',(-6.638064156,1.715323387,3.490860104));
#133555=CARTESIAN_POINT('',(-6.47036986816281,1.71532338778839,3.53699225677551));
#133556=CARTESIAN_POINT('Ctrl Pts',(-6.30267558499999,1.715323387,3.583124401));
#133557=CARTESIAN_POINT('Ctrl Pts',(-6.108708297,1.779910221,3.924310682));
#133558=CARTESIAN_POINT('Ctrl Pts',(-5.879043182,1.845052736,4.242564232));
#133559=CARTESIAN_POINT('Ctrl Pts',(-6.394939882,1.715323387,3.918512972));
#133560=CARTESIAN_POINT('Ctrl Pts',(-6.182816816,1.779910221,4.264693848));
#133561=CARTESIAN_POINT('Ctrl Pts',(-5.93456285000001,1.845052736,4.585952876));
#133562=CARTESIAN_POINT('',(-6.39493988465156,1.71532338744858,3.9185129697532));
#133563=CARTESIAN_POINT('',(-6.08372764672891,1.80506741727164,4.386143855119));
#133564=CARTESIAN_POINT('Origin',(0.147691334341582,1.8749745505013,-0.120317322450024));
#133565=CARTESIAN_POINT('Ctrl Pts',(-5.88178333421817,1.84427517375015,
4.23876453771839));
#133566=CARTESIAN_POINT('Ctrl Pts',(-5.9154125277128,1.83740483730708,4.26326079454293));
#133567=CARTESIAN_POINT('Ctrl Pts',(-5.94907435305998,1.83070798061871,
4.2878053775091));
#133568=CARTESIAN_POINT('Ctrl Pts',(-6.01637702711119,1.81765000111501,
4.33692424505133));
#133569=CARTESIAN_POINT('Ctrl Pts',(-6.050057767914,1.81128114569571,4.36152764629411));
#133570=CARTESIAN_POINT('Ctrl Pts',(-6.08372764844526,1.80506741735516,
4.38614385279247));
#133571=CARTESIAN_POINT('',(-6.34880773763066,1.71532338830053,3.75081867950825));
#133572=CARTESIAN_POINT('Origin',(-1.50487261540988E-13,1.80614392399994,
-3.46944695195361E-15));
#133573=CARTESIAN_POINT('',(-6.08140007977468,1.6256495872305,4.38937046332154));
#133574=CARTESIAN_POINT('Origin',(0.13633236409473,1.48225708328908,-0.126630402607792));
#133575=CARTESIAN_POINT('',(-5.73243817153204,1.71532338734572,4.83623330865244));
#133576=CARTESIAN_POINT('Origin',(0.123522468779412,1.87485301057633,-0.137471620468915));
#133577=CARTESIAN_POINT('Ctrl Pts',(-6.08372764527108,1.80506741655844,
4.38614385691246));
#133578=CARTESIAN_POINT('Ctrl Pts',(-6.0153074796744,1.7865858116006,4.48104490613826));
#133579=CARTESIAN_POINT('Ctrl Pts',(-5.94480848178056,1.76822051519547,
4.57414596570128));
#133580=CARTESIAN_POINT('Ctrl Pts',(-5.87237536131294,1.75000000001473,
4.66531966898703));
#133581=CARTESIAN_POINT('Ctrl Pts',(-5.8266445793839,1.73849644466908,4.72288235120746));
#133582=CARTESIAN_POINT('Ctrl Pts',(-5.77999144574739,1.72693520694185,
4.77986791146979));
#133583=CARTESIAN_POINT('Ctrl Pts',(-5.73243817162547,1.71532338729505,
4.83623330659798));
#133584=CARTESIAN_POINT('Ctrl Pts',(-5.884569297,1.845058467,4.234896006));
#133585=CARTESIAN_POINT('Ctrl Pts',(-5.714340306,1.797173233,4.471436477));
#133586=CARTESIAN_POINT('Ctrl Pts',(-5.5256749,1.75,4.693550565));
#133587=CARTESIAN_POINT('Ctrl Pts',(-5.456549118,1.732716033,4.774931727));
#133588=CARTESIAN_POINT('Ctrl Pts',(-5.385056702,1.715323387,4.854241888));
#133589=CARTESIAN_POINT('Ctrl Pts',(-6.227885267,1.845058467,4.178928703));
#133590=CARTESIAN_POINT('Ctrl Pts',(-6.05990597900001,1.797173233,4.429269354));
#133591=CARTESIAN_POINT('Ctrl Pts',(-5.872375362,1.75,4.665319669));
#133592=CARTESIAN_POINT('Ctrl Pts',(-5.803665359,1.732716033,4.751806974));
#133593=CARTESIAN_POINT('Ctrl Pts',(-5.732438171,1.715323387,4.836233308));
#133594=CARTESIAN_POINT('',(-5.55874743329838,1.71532338778837,4.84523760167309));
#133595=CARTESIAN_POINT('Ctrl Pts',(-5.385056702,1.715323387,4.854241888));
#133596=CARTESIAN_POINT('Ctrl Pts',(-5.122279297,1.779910221,5.145754191));
#133597=CARTESIAN_POINT('Ctrl Pts',(-4.829568519,1.845052736,5.407195939));
#133598=CARTESIAN_POINT('Ctrl Pts',(-5.403065283,1.715323387,5.201623357));
#133599=CARTESIAN_POINT('Ctrl Pts',(-5.121482881,1.779910221,5.494110528));
#133600=CARTESIAN_POINT('Ctrl Pts',(-4.80997176,1.845052736,5.754491434));
#133601=CARTESIAN_POINT('',(-5.40306528606363,1.71532338744859,5.2016233553958));
#133602=CARTESIAN_POINT('',(-4.99860219952518,1.80506741735075,5.59141985937217));
#133603=CARTESIAN_POINT('Origin',(0.118373688949022,1.87497455816666,-0.149253604198235));
#133604=CARTESIAN_POINT('Ctrl Pts',(-4.83306143014279,1.84427517370204,
5.40407413113599));
#133605=CARTESIAN_POINT('Ctrl Pts',(-4.86063842297015,1.83740483668169,
5.4352269642911));
#133606=CARTESIAN_POINT('Ctrl Pts',(-4.88823689644891,1.83070797937978,
5.46643400908832));
#133607=CARTESIAN_POINT('Ctrl Pts',(-4.94340696136198,1.81765000116022,
5.52887258420017));
#133608=CARTESIAN_POINT('Ctrl Pts',(-4.97101126108887,1.81128114575866,
5.5601411352121));
#133609=CARTESIAN_POINT('Ctrl Pts',(-4.9986022017135,1.80506741743534,5.59141985745866));
#133610=CARTESIAN_POINT('',(-5.39406099803711,1.71532338830053,5.02793261655969));
#133611=CARTESIAN_POINT('Origin',(7.46364775539021E-13,1.80614392399945,
-7.6588041464376E-13));
#133612=CARTESIAN_POINT('',(-4.99563542483045,1.62564958722827,5.59407067324546));
#133613=CARTESIAN_POINT('Origin',(0.105923124203066,1.48225704987208,-0.152977207608697));
#133614=CARTESIAN_POINT('',(-4.55876974925633,1.715323387357,5.95546961878356));
#133615=CARTESIAN_POINT('Origin',(0.0910824517940872,1.87485302966038,-0.160811540123007));
#133616=CARTESIAN_POINT('Ctrl Pts',(-4.99860219769392,1.80506741663509,
5.59141986081333));
#133617=CARTESIAN_POINT('Ctrl Pts',(-4.91138073706177,1.78658581165296,
5.66939386310148));
#133618=CARTESIAN_POINT('Ctrl Pts',(-4.82251599075879,1.76822051522225,
5.74516307094973));
#133619=CARTESIAN_POINT('Ctrl Pts',(-4.73217666580145,1.75000000003504,
5.81863420380799));
#133620=CARTESIAN_POINT('Ctrl Pts',(-4.67514077019381,1.73849644470229,
5.86502033598252));
#133621=CARTESIAN_POINT('Ctrl Pts',(-4.6173281493075,1.72693520694185,5.91064456103527));
#133622=CARTESIAN_POINT('Ctrl Pts',(-4.55876974991222,1.71532338729505,
5.95546961676522));
#133623=CARTESIAN_POINT('Ctrl Pts',(-4.836613879,1.845058467,5.400894943));
#133624=CARTESIAN_POINT('Ctrl Pts',(-4.619515538,1.797173233,5.59531102800001));
#133625=CARTESIAN_POINT('Ctrl Pts',(-4.38751306,1.75,5.771674726));
#133626=CARTESIAN_POINT('Ctrl Pts',(-4.302508856,1.732716033,5.836293242));
#133627=CARTESIAN_POINT('Ctrl Pts',(-4.215638554,1.715323387,5.898380421));
#133628=CARTESIAN_POINT('Ctrl Pts',(-5.183934627,1.845058467,5.42003891));
#133629=CARTESIAN_POINT('Ctrl Pts',(-4.966066761,1.797173233,5.62841615400001));
#133630=CARTESIAN_POINT('Ctrl Pts',(-4.732176666,1.75,5.818634204));
#133631=CARTESIAN_POINT('Ctrl Pts',(-4.646480852,1.732716033,5.888328864));
#133632=CARTESIAN_POINT('Ctrl Pts',(-4.558769749,1.715323387,5.95546961800001));
#133633=CARTESIAN_POINT('',(-4.38720414758359,1.71532338778839,5.92692502239899));
#133634=CARTESIAN_POINT('Ctrl Pts',(-4.215638554,1.715323387,5.898380421));
#133635=CARTESIAN_POINT('Ctrl Pts',(-3.89633821,1.779910221,6.126587953));
#133636=CARTESIAN_POINT('Ctrl Pts',(-3.554268599,1.845052736,6.318993173));
#133637=CARTESIAN_POINT('Ctrl Pts',(-4.158549356,1.715323387,6.241511616));
#133638=CARTESIAN_POINT('Ctrl Pts',(-3.820674098,1.779910221,6.466628707));
#133639=CARTESIAN_POINT('Ctrl Pts',(-3.460471736,1.845052736,6.653956369));
#133640=CARTESIAN_POINT('',(-4.15854935933182,1.71532338744847,6.24151161509755));
#133641=CARTESIAN_POINT('',(-3.6797476691896,1.80506741728958,6.53524728577702));
#133642=CARTESIAN_POINT('Origin',(0.0835210239221201,1.87497457238564,-0.17121091276438));
#133643=CARTESIAN_POINT('Ctrl Pts',(-3.55835094392698,1.84427517370894,
6.31669522493168));
#133644=CARTESIAN_POINT('Ctrl Pts',(-3.57858625937572,1.83740483824043,
6.35304795193762));
#133645=CARTESIAN_POINT('Ctrl Pts',(-3.59883089848952,1.8307079825938,6.38945823950481));
#133646=CARTESIAN_POINT('Ctrl Pts',(-3.63928868009485,1.81765000115139,
6.46229698630404));
#133647=CARTESIAN_POINT('Ctrl Pts',(-3.659525792586,1.81128114571434,6.4987686045792));
#133648=CARTESIAN_POINT('Ctrl Pts',(-3.6797476716983,1.80506741737228,6.53524728440042));
#133649=CARTESIAN_POINT('',(-4.18709396168286,1.71532338830019,6.06994601389012));
#133650=CARTESIAN_POINT('Origin',(1.49403059368503E-13,1.8061439239995,
-3.35235311732518E-13));
#133651=CARTESIAN_POINT('',(-3.67628040958788,1.62564958722685,6.53719835590227));
#133652=CARTESIAN_POINT('Origin',(0.0705612289384649,1.48225705527937,-0.172171196500804));
#133653=CARTESIAN_POINT('',(-3.17193832019193,1.71532338734682,6.79623478881418));
#133654=CARTESIAN_POINT('Origin',(0.0543832873494848,1.87485296704309,-0.176631898520114));
#133655=CARTESIAN_POINT('Ctrl Pts',(-3.67974766713166,1.80506741658449,
6.53524728677746));
#133656=CARTESIAN_POINT('Ctrl Pts',(-3.57780329029907,1.78658581161492,
6.59264826446448));
#133657=CARTESIAN_POINT('Ctrl Pts',(-3.47472801243772,1.76822051520117,
6.64754273669236));
#133658=CARTESIAN_POINT('Ctrl Pts',(-3.37070664861048,1.74999999999575,
6.69987587087804));
#133659=CARTESIAN_POINT('Ctrl Pts',(-3.30503257263167,1.73849644463805,
6.73291648972614));
#133660=CARTESIAN_POINT('Ctrl Pts',(-3.23876371927812,1.72693520694185,
6.76504604108847));
#133661=CARTESIAN_POINT('Ctrl Pts',(-3.17193832115523,1.71532338729505,
6.79623478698976));
#133662=CARTESIAN_POINT('Ctrl Pts',(-3.56250377,1.845058467,6.314354036));
#133663=CARTESIAN_POINT('Ctrl Pts',(-3.308687357,1.797173233,6.457555054));
#133664=CARTESIAN_POINT('Ctrl Pts',(-3.044195986,1.75,6.579921793));
#133665=CARTESIAN_POINT('Ctrl Pts',(-2.947288063,1.732716033,6.62475617200001));
#133666=CARTESIAN_POINT('Ctrl Pts',(-2.849101831,1.715323387,6.66671724));
#133667=CARTESIAN_POINT('Ctrl Pts',(-3.897588966,1.845058467,6.40771412100001));
#133668=CARTESIAN_POINT('Ctrl Pts',(-3.640019782,1.797173233,6.56438447000001));
#133669=CARTESIAN_POINT('Ctrl Pts',(-3.370706649,1.75,6.699875871));
#133670=CARTESIAN_POINT('Ctrl Pts',(-3.272032063,1.732716033,6.74951904200001));
#133671=CARTESIAN_POINT('Ctrl Pts',(-3.17193832,1.715323387,6.796234788));
#133672=CARTESIAN_POINT('',(-3.01052007105196,1.71532338778838,6.7314760159893));
#133673=CARTESIAN_POINT('Ctrl Pts',(-2.849101831,1.715323387,6.66671724));
#133674=CARTESIAN_POINT('Ctrl Pts',(-2.488208678,1.779910221,6.820949271));
#133675=CARTESIAN_POINT('Ctrl Pts',(-2.11277503,1.845052736,6.93532131));
#133676=CARTESIAN_POINT('Ctrl Pts',(-2.719584283,1.715323387,6.989553729));
#133677=CARTESIAN_POINT('Ctrl Pts',(-2.341214841,1.779910221,7.136774514));
#133678=CARTESIAN_POINT('Ctrl Pts',(-1.949163901,1.845052736,7.242289699));
#133679=CARTESIAN_POINT('',(-2.71958428645445,1.71532338744809,6.98955372882641));
#133680=CARTESIAN_POINT('',(-2.1888322280156,1.80506741730229,7.17349381209083));
#133681=CARTESIAN_POINT('Origin',(0.0447630880302707,1.87497458410537,-0.185162737521352));
#133682=CARTESIAN_POINT('Ctrl Pts',(-2.11725592328195,1.84427517370612,
6.93395466941367));
#133683=CARTESIAN_POINT('Ctrl Pts',(-2.12920338796688,1.83740483743912,
6.9738074892125));
#133684=CARTESIAN_POINT('Ctrl Pts',(-2.14114758477622,1.83070798093934,
7.01371852897689));
#133685=CARTESIAN_POINT('Ctrl Pts',(-2.16500130557034,1.81765000112972,
7.0935515635659));
#133686=CARTESIAN_POINT('Ctrl Pts',(-2.17692496579604,1.81128114571579,
7.1335208765333));
#133687=CARTESIAN_POINT('Ctrl Pts',(-2.18883223079566,1.80506741738623,
7.17349381127575));
#133688=CARTESIAN_POINT('',(-2.78434306451125,1.71532338829908,6.8281354814371));
#133689=CARTESIAN_POINT('Origin',(1.44632569809566E-13,1.8061439240005,
-3.90746462963776E-13));
#133690=CARTESIAN_POINT('',(-2.18502660827602,1.62564958721219,7.17465390913889));
#133691=CARTESIAN_POINT('Origin',(0.0318997603712604,1.48225709287231,-0.183314302122269));
#133692=CARTESIAN_POINT('',(-1.63679058102413,1.71532338734606,7.31921557284011));
#133693=CARTESIAN_POINT('Origin',(0.0151411834314741,1.8748529928791,-0.184193113374613));
#133694=CARTESIAN_POINT('Ctrl Pts',(-2.18883222576068,1.80506741658859,
7.17349381263113));
#133695=CARTESIAN_POINT('Ctrl Pts',(-2.07693173832936,1.78658581162109,
7.20763775979279));
#133696=CARTESIAN_POINT('Ctrl Pts',(-1.96446561443443,1.76822051520548,
7.23909069180446));
#133697=CARTESIAN_POINT('Ctrl Pts',(-1.85162613527359,1.749999999943,7.26783878785127));
#133698=CARTESIAN_POINT('Ctrl Pts',(-1.78038472563909,1.73849644455183,
7.28598895035891));
#133699=CARTESIAN_POINT('Ctrl Pts',(-1.70875829796959,1.72693520694185,
7.30312148604251));
#133700=CARTESIAN_POINT('Ctrl Pts',(-1.63679058234637,1.71532338729505,
7.3192155712624));
#133701=CARTESIAN_POINT('Ctrl Pts',(-2.121814945,1.845058467,6.932560951));
#133702=CARTESIAN_POINT('Ctrl Pts',(-1.843148632,1.797173233,7.01785098300001));
#133703=CARTESIAN_POINT('Ctrl Pts',(-1.558535692,1.75,7.080499029));
#133704=CARTESIAN_POINT('Ctrl Pts',(-1.454255355,1.732716033,7.103452867));
#133705=CARTESIAN_POINT('Ctrl Pts',(-1.349344274,1.715323387,7.12332577));
#133706=CARTESIAN_POINT('Ctrl Pts',(-2.428996377,1.845058467,7.095771741));
#133707=CARTESIAN_POINT('Ctrl Pts',(-2.143769523,1.797173233,7.193409464));
#133708=CARTESIAN_POINT('Ctrl Pts',(-1.851626136,1.75,7.267838788));
#133709=CARTESIAN_POINT('Ctrl Pts',(-1.744586692,1.732716033,7.29510921));
#133710=CARTESIAN_POINT('Ctrl Pts',(-1.636790581,1.715323387,7.319215572));
#133711=CARTESIAN_POINT('',(-1.49306742272831,1.71532338778839,7.2212706719866));
#133712=CARTESIAN_POINT('Ctrl Pts',(-1.349344274,1.715323387,7.12332577));
#133713=CARTESIAN_POINT('Ctrl Pts',(-0.963733275,1.779910221,7.196370583));
#133714=CARTESIAN_POINT('Ctrl Pts',(-0.572490449,1.845052736,7.22736153));
#133715=CARTESIAN_POINT('Ctrl Pts',(-1.153454472,1.715323387,7.41077207700001));
#133716=CARTESIAN_POINT('Ctrl Pts',(-0.75228298,1.779910221,7.473212677));
#133717=CARTESIAN_POINT('Ctrl Pts',(-0.346715327,1.845052736,7.491981613));
#133718=CARTESIAN_POINT('',(-1.15345447538118,1.71532338744759,7.41077207758618));
#133719=CARTESIAN_POINT('',(-0.595569424149683,1.80506741729189,7.4763157408475));
#133720=CARTESIAN_POINT('Origin',(0.00391204345537494,1.87497458607747,
-0.190456472670194));
#133721=CARTESIAN_POINT('Ctrl Pts',(-0.577160368713407,1.84427517375144,
7.22699010014981));
#133722=CARTESIAN_POINT('Ctrl Pts',(-0.58026133036698,1.83740483693944,
7.26847953832023));
#133723=CARTESIAN_POINT('Ctrl Pts',(-0.583346585006129,1.83070797985232,
7.31002513333623));
#133724=CARTESIAN_POINT('Ctrl Pts',(-0.589480875960759,1.81765000113372,
7.39311955382139));
#133725=CARTESIAN_POINT('Ctrl Pts',(-0.592533546807837,1.81128114573694,
7.43471764077701));
#133726=CARTESIAN_POINT('Ctrl Pts',(-0.595569427165579,1.80506741737982,
7.47631574064053));
#133727=CARTESIAN_POINT('',(-1.25139938098489,1.71532338829759,7.26704892212499));
#133728=CARTESIAN_POINT('Origin',(4.1165801236559E-16,1.80614392399939,
-6.8434841127285E-13));
#133729=CARTESIAN_POINT('',(-0.591603391254012,1.62564958716999,7.47663061959824));
#133730=CARTESIAN_POINT('Origin',(-0.00825319872770208,1.48225709597672,
-0.185885931764933));
#133731=CARTESIAN_POINT('',(-0.0251083328437023,1.715323387346,7.49995797182605));
#133732=CARTESIAN_POINT('Origin',(-0.0248088887949483,1.87485302402727,
-0.183141684585254));
#133733=CARTESIAN_POINT('Ctrl Pts',(-0.595569421727552,1.80506741654646,
7.47631574089619));
#133734=CARTESIAN_POINT('Ctrl Pts',(-0.478945166287782,1.78658581160554,
7.4856061244765));
#133735=CARTESIAN_POINT('Ctrl Pts',(-0.362346987204218,1.76822051520377,
7.49214681237726));
#133736=CARTESIAN_POINT('Ctrl Pts',(-0.24596564175084,1.75000000004052,
7.49596564148352));
#133737=CARTESIAN_POINT('Ctrl Pts',(-0.17248806913491,1.73849644471125,
7.49837666576198));
#133738=CARTESIAN_POINT('Ctrl Pts',(-0.0988532380978183,1.72693520694185,
7.49971108777194));
#133739=CARTESIAN_POINT('Ctrl Pts',(-0.0251083344734459,1.71532338729505,
7.49995797056906));
#133740=CARTESIAN_POINT('Ctrl Pts',(-0.581912411,1.845058467,7.226609021));
#133741=CARTESIAN_POINT('Ctrl Pts',(-0.291426326,1.797173233,7.25));
#133742=CARTESIAN_POINT('Ctrl Pts',(0.,1.75,7.25));
#133743=CARTESIAN_POINT('Ctrl Pts',(0.106776717,1.732716033,7.25));
#133744=CARTESIAN_POINT('Ctrl Pts',(0.213507122,1.715323387,7.246855505));
#133745=CARTESIAN_POINT('Ctrl Pts',(-0.846826616,1.845058467,7.452038961));
#133746=CARTESIAN_POINT('Ctrl Pts',(-0.547278984,1.797173233,7.48607862600001));
#133747=CARTESIAN_POINT('Ctrl Pts',(-0.245965642,1.75,7.495965642));
#133748=CARTESIAN_POINT('Ctrl Pts',(-0.135566387,1.732716033,7.49958818));
#133749=CARTESIAN_POINT('Ctrl Pts',(-0.025108333,1.715323387,7.499957971));
#133750=CARTESIAN_POINT('',(0.094199399372222,1.71532338778839,7.37340673793776));
#133751=CARTESIAN_POINT('Ctrl Pts',(-1.648780528,4.042023177,7.316523954));
#133752=CARTESIAN_POINT('Ctrl Pts',(-1.249332754,4.10772842,7.406539611));
#133753=CARTESIAN_POINT('Ctrl Pts',(-0.842459476,4.172899507,7.452533934));
#133754=CARTESIAN_POINT('Ctrl Pts',(-1.361013652,4.042023177,7.12110538));
#133755=CARTESIAN_POINT('Ctrl Pts',(-0.972234813,4.10772842,7.19541032));
#133756=CARTESIAN_POINT('Ctrl Pts',(-0.577677420999999,4.172899507,7.226948789));
#133757=CARTESIAN_POINT('',(-0.84245946624551,4.17289950600422,7.45253393658569));
#133758=CARTESIAN_POINT('',(-0.710068431037417,4.17289950413623,7.33974136318938));
#133759=CARTESIAN_POINT('',(-1.40346520264162,4.08221031165715,7.36751555261981));
#133760=CARTESIAN_POINT('Origin',(0.045787793001877,4.01787921770315,-0.185145958812898));
#133761=CARTESIAN_POINT('Ctrl Pts',(-1.35637331540347,4.0428073592789,7.12199069258409));
#133762=CARTESIAN_POINT('Ctrl Pts',(-1.36425141320857,4.04969801218673,
7.16284458526961));
#133763=CARTESIAN_POINT('Ctrl Pts',(-1.37211768790064,4.05642175344562,
7.20375431976348));
#133764=CARTESIAN_POINT('Ctrl Pts',(-1.38781116925284,4.0695455071114,7.28558294300322));
#133765=CARTESIAN_POINT('Ctrl Pts',(-1.39564719791905,4.07595289336076,
7.32654784736749));
#133766=CARTESIAN_POINT('Ctrl Pts',(-1.40346520397192,4.08221031165702,
7.36751555236596));
#133767=CARTESIAN_POINT('Ctrl Pts',(-1.954361232,4.172899507,7.240888908));
#133768=CARTESIAN_POINT('Ctrl Pts',(-1.55978046,4.107307013,7.347388728));
#133769=CARTESIAN_POINT('Ctrl Pts',(-1.155963477,4.04203077,7.410381126));
#133770=CARTESIAN_POINT('Ctrl Pts',(-2.117752007,4.172899507,6.933803173));
#133771=CARTESIAN_POINT('Ctrl Pts',(-1.739905385,4.107307013,7.049206714));
#133772=CARTESIAN_POINT('Ctrl Pts',(-1.351755947,4.04203077,7.122868513));
#133773=CARTESIAN_POINT('',(-1.95436122762896,4.17289950692266,7.24088891073579));
#133774=CARTESIAN_POINT('Origin',(0.0483827730459563,4.16071411101886,-0.186743460649631));
#133775=CARTESIAN_POINT('',(-2.03605662078521,4.17289950678353,7.08734604013078));
#133776=CARTESIAN_POINT('Origin',(6.59737021957429E-14,4.26419218499978,
-5.49039980146659E-13));
#133777=CARTESIAN_POINT('',(-1.39881673462662,4.26310680662278,7.36839953685386));
#133778=CARTESIAN_POINT('Origin',(0.0196658883634099,4.16071717757456,-0.19146588038788));
#133779=CARTESIAN_POINT('Origin',(0.0716636017910904,4.01799492241726,-0.170731827707776));
#133780=CARTESIAN_POINT('Ctrl Pts',(-3.183069331,4.042023177,6.791028614));
#133781=CARTESIAN_POINT('Ctrl Pts',(-2.812311129,4.10772842,6.964809219));
#133782=CARTESIAN_POINT('Ctrl Pts',(-2.424837742,4.172899507,7.09719394700001));
#133783=CARTESIAN_POINT('Ctrl Pts',(-2.860021067,4.042023177,6.66204019));
#133784=CARTESIAN_POINT('Ctrl Pts',(-2.496305027,4.10772842,6.81818388));
#133785=CARTESIAN_POINT('Ctrl Pts',(-2.117752007,4.172899507,6.933803173));
#133786=CARTESIAN_POINT('',(-2.42483773306114,4.17289950600422,7.09719395161998));
#133787=CARTESIAN_POINT('',(-2.27129485780885,4.17289950413623,7.01549856540382));
#133788=CARTESIAN_POINT('',(-2.95445102732462,4.08221031165033,6.89356360063074));
#133789=CARTESIAN_POINT('Origin',(0.0845180867257572,4.01787922293851,-0.170974027477583));
#133790=CARTESIAN_POINT('Ctrl Pts',(-2.85567953540613,4.04280735926973,
6.66390233981684));
#133791=CARTESIAN_POINT('Ctrl Pts',(-2.87215582770793,4.04969801251677,
6.7021075347925));
#133792=CARTESIAN_POINT('Ctrl Pts',(-2.88863257781732,4.05642175415592,
6.74036980808426));
#133793=CARTESIAN_POINT('Ctrl Pts',(-2.92154988751123,4.06954550710655,
6.81691168458022));
#133794=CARTESIAN_POINT('Ctrl Pts',(-2.93800895763356,4.07595289335613,
6.85523433760006));
#133795=CARTESIAN_POINT('Ctrl Pts',(-2.95445102856625,4.08221031165021,
6.89356360009814));
#133796=CARTESIAN_POINT('Ctrl Pts',(-3.465246429,4.172899507,6.651471054));
#133797=CARTESIAN_POINT('Ctrl Pts',(-3.102785048,4.107307013,6.84030417));
#133798=CARTESIAN_POINT('Ctrl Pts',(-2.721950586,4.04203077,6.988632556));
#133799=CARTESIAN_POINT('Ctrl Pts',(-3.558802862,4.172899507,6.316440627));
#133800=CARTESIAN_POINT('Ctrl Pts',(-3.214598434,4.107307013,6.510371952));
#133801=CARTESIAN_POINT('Ctrl Pts',(-2.851358824,4.04203077,6.665752235));
#133802=CARTESIAN_POINT('',(-3.46524642532133,4.17289950685238,6.65147105763285));
#133803=CARTESIAN_POINT('Origin',(0.0873959770846583,4.16071398744577,-0.171976766965011));
#133804=CARTESIAN_POINT('',(-3.5120246466758,4.17289950678353,6.48395583986313));
#133805=CARTESIAN_POINT('Origin',(-4.71411104596697E-13,4.26419218499956,
8.28330459778925E-13));
#133806=CARTESIAN_POINT('',(-2.95010126897283,4.26310680661376,6.89542620135548));
#133807=CARTESIAN_POINT('Origin',(0.0603656250039425,4.16071714725873,-0.182762002467465));
#133808=CARTESIAN_POINT('Origin',(0.106690365472132,4.01799501511567,-0.151334504317661));
#133809=CARTESIAN_POINT('Ctrl Pts',(-4.568521349,4.042023177,5.947992324));
#133810=CARTESIAN_POINT('Ctrl Pts',(-4.243788962,4.10772842,6.197412088));
#133811=CARTESIAN_POINT('Ctrl Pts',(-3.89383329,4.172899507,6.40999706));
#133812=CARTESIAN_POINT('Ctrl Pts',(-4.225297077,4.042023177,5.891465405));
#133813=CARTESIAN_POINT('Ctrl Pts',(-3.903650793,4.10772842,6.122146739));
#133814=CARTESIAN_POINT('Ctrl Pts',(-3.558802862,4.172899507,6.31644062700001));
#133815=CARTESIAN_POINT('',(-3.89383328225289,4.17289950600423,6.40999706643631));
#133816=CARTESIAN_POINT('',(-3.72631806086074,4.17289950413623,6.36321885236559));
#133817=CARTESIAN_POINT('',(-4.36729000625335,4.0822103116468,6.0972762766455));
#133818=CARTESIAN_POINT('Origin',(0.119296556422939,4.01787916433398,-0.148807985082576));
#133819=CARTESIAN_POINT('Ctrl Pts',(-4.22145735396844,4.04280735933467,
5.89421731982391));
#133820=CARTESIAN_POINT('Ctrl Pts',(-4.24576142183867,4.04969801097169,
5.92798737493316));
#133821=CARTESIAN_POINT('Ctrl Pts',(-4.27007820568629,4.05642175081999,
5.96181307371015));
#133822=CARTESIAN_POINT('Ctrl Pts',(-4.31868018038231,4.06954550707837,
6.0294892121902));
#133823=CARTESIAN_POINT('Ctrl Pts',(-4.34299268432752,4.07595289333869,
6.06337768937981));
#133824=CARTESIAN_POINT('Ctrl Pts',(-4.36729000735009,4.08221031164667,
6.09727627585942));
#133825=CARTESIAN_POINT('Ctrl Pts',(-4.814100554,4.172899507,5.751037807));
#133826=CARTESIAN_POINT('Ctrl Pts',(-4.500706857,4.107307013,6.01337459200001));
#133827=CARTESIAN_POINT('Ctrl Pts',(-4.160662311,4.04203077,6.240103295));
#133828=CARTESIAN_POINT('Ctrl Pts',(-4.83344805100001,4.172899507,5.403728337));
#133829=CARTESIAN_POINT('Ctrl Pts',(-4.538980434,4.107307013,5.667119433));
#133830=CARTESIAN_POINT('Ctrl Pts',(-4.217635331,4.04203077,5.89695279));
#133831=CARTESIAN_POINT('',(-4.81410055117865,4.17289950692264,5.75103781132326));
#133832=CARTESIAN_POINT('Origin',(0.122322701494825,4.16071408995026,-0.149168563028286));
#133833=CARTESIAN_POINT('',(-4.82377430351141,4.17289950678353,5.57738307112526));
#133834=CARTESIAN_POINT('Origin',(-1.34441069388203E-13,4.26419218500022,
1.7650811368064E-13));
#133835=CARTESIAN_POINT('',(-4.36344234637331,4.26310680660557,6.10003040005731));
#133836=CARTESIAN_POINT('Origin',(0.0982427970437966,4.16071715899573,-0.165512377509088));
#133837=CARTESIAN_POINT('Origin',(0.136728528293678,4.01799496612477,-0.124861216573521));
#133838=CARTESIAN_POINT('Ctrl Pts',(-5.74035438700001,4.042023177,4.826834523));
#133839=CARTESIAN_POINT('Ctrl Pts',(-5.476831939,4.10772842,5.140230856));
#133840=CARTESIAN_POINT('Ctrl Pts',(-5.180757521,4.172899507,5.423075834));
#133841=CARTESIAN_POINT('Ctrl Pts',(-5.39300289,4.042023177,4.845412245));
#133842=CARTESIAN_POINT('Ctrl Pts',(-5.128466186,4.10772842,5.139844821));
#133843=CARTESIAN_POINT('Ctrl Pts',(-4.83344805100001,4.172899507,5.403728337));
#133844=CARTESIAN_POINT('',(-5.18075751483706,4.17289950600424,5.42307584194055));
#133845=CARTESIAN_POINT('',(-5.00710277312053,4.17289950413623,5.41340209741281));
#133846=CARTESIAN_POINT('',(-5.57591935849747,4.08221031169378,5.01588709046708));
#133847=CARTESIAN_POINT('Origin',(0.148496838195578,4.01787919839837,-0.119683774713932));
#133848=CARTESIAN_POINT('Ctrl Pts',(-5.38984451854537,4.04280735924304,
4.84892524811203));
#133849=CARTESIAN_POINT('Ctrl Pts',(-5.42083994034192,4.04969801218734,
4.87668112718648));
#133850=CARTESIAN_POINT('Ctrl Pts',(-5.4518597438633,4.05642175349626,4.90448861664555));
#133851=CARTESIAN_POINT('Ctrl Pts',(-5.51387378821012,4.06954550710964,
4.96013452549735));
#133852=CARTESIAN_POINT('Ctrl Pts',(-5.54490290021431,4.0759528933765,4.98800423927055));
#133853=CARTESIAN_POINT('Ctrl Pts',(-5.57591935941457,4.08221031169365,
5.01588708944694));
#133854=CARTESIAN_POINT('Ctrl Pts',(-5.937852687,4.172899507,4.58169242400001));
#133855=CARTESIAN_POINT('Ctrl Pts',(-5.688180615,4.107307013,4.905266302));
#133856=CARTESIAN_POINT('Ctrl Pts',(-5.404826091,4.04203077,5.199793739));
#133857=CARTESIAN_POINT('Ctrl Pts',(-5.882086581,4.172899507,4.238343716));
#133858=CARTESIAN_POINT('Ctrl Pts',(-5.651124753,4.107307013,4.558878708));
#133859=CARTESIAN_POINT('Ctrl Pts',(-5.38669989800001,4.04203077,4.852418387));
#133860=CARTESIAN_POINT('',(-5.93785268519229,4.17289950685237,4.58169242882394));
#133861=CARTESIAN_POINT('Origin',(0.151529528601895,4.16071399372597,-0.119385194429135));
#133862=CARTESIAN_POINT('',(-5.90996963479971,4.17289950678353,4.41001806892829));
#133863=CARTESIAN_POINT('Origin',(3.14418630020796E-13,4.26419218500067,
-4.08961059461532E-13));
#133864=CARTESIAN_POINT('',(-5.57275370974783,4.26310680605755,5.01940395734865));
#133865=CARTESIAN_POINT('Origin',(0.131526048152067,4.16071715478734,-0.140523359004434));
#133866=CARTESIAN_POINT('Origin',(0.160373400530025,4.0179949732781,-0.0925494642866742));
#133867=CARTESIAN_POINT('Ctrl Pts',(-6.643774834,4.042023177,3.479979305));
#133868=CARTESIAN_POINT('Ctrl Pts',(-6.453784342,4.10772842,3.842698142));
#133869=CARTESIAN_POINT('Ctrl Pts',(-6.225435289,4.172899507,4.18257761));
#133870=CARTESIAN_POINT('Ctrl Pts',(-6.308537883,4.042023177,3.572792994));
#133871=CARTESIAN_POINT('Ctrl Pts',(-6.113480201,4.10772842,3.917209472));
#133872=CARTESIAN_POINT('Ctrl Pts',(-5.882086581,4.172899507,4.238343716));
#133873=CARTESIAN_POINT('',(-6.22543528466732,4.17289950600422,4.18257761909796));
#133874=CARTESIAN_POINT('',(-6.05376092498255,4.17289950413623,4.210460677403));
#133875=CARTESIAN_POINT('',(-6.52382491778054,4.08221031166323,3.69996059879415));
#133876=CARTESIAN_POINT('Origin',(0.170753419546019,4.01787914189447,-0.0849631041525056));
#133877=CARTESIAN_POINT('Ctrl Pts',(-6.30620854436298,4.04280735921502,
3.57690282142814));
#133878=CARTESIAN_POINT('Ctrl Pts',(-6.34244600490884,4.04969801238145,
3.59734668483609));
#133879=CARTESIAN_POINT('Ctrl Pts',(-6.37871837213589,4.05642175393434,
3.61783571071886));
#133880=CARTESIAN_POINT('Ctrl Pts',(-6.451244785248,4.06954550708461,3.6588494613919));
#133881=CARTESIAN_POINT('Ctrl Pts',(-6.48753961835998,4.07595289334855,
3.67939725488016));
#133882=CARTESIAN_POINT('Ctrl Pts',(-6.52382491844971,4.08221031166311,
3.6999605976134));
#133883=CARTESIAN_POINT('Ctrl Pts',(-6.783957428,4.172899507,3.198112195));
#133884=CARTESIAN_POINT('Ctrl Pts',(-6.609681369,4.107307013,3.567793211));
#133885=CARTESIAN_POINT('Ctrl Pts',(-6.396266209,4.04203077,3.916347607));
#133886=CARTESIAN_POINT('Ctrl Pts',(-6.65568528000001,4.172899507,2.874778854));
#133887=CARTESIAN_POINT('Ctrl Pts',(-6.499028759,4.107307013,3.237469881));
#133888=CARTESIAN_POINT('Ctrl Pts',(-6.303888365,4.04203077,3.580990293));
#133889=CARTESIAN_POINT('',(-6.78395742727015,4.17289950685237,3.19811220011488));
#133890=CARTESIAN_POINT('Origin',(0.173651161295976,4.16071398741859,-0.0840196800174137));
#133891=CARTESIAN_POINT('',(-6.71982135455063,4.17289950678353,3.03644552328143));
#133892=CARTESIAN_POINT('Origin',(1.86049092798513E-13,4.26419218500022,
-1.0321604682062E-13));
#133893=CARTESIAN_POINT('',(-6.52148930308317,4.26310680659818,3.70407576406289));
#133894=CARTESIAN_POINT('Origin',(0.158659732795933,4.16071715051203,-0.108963977755514));
#133895=CARTESIAN_POINT('Origin',(0.176518966636331,4.01799497241305,-0.0559099629043863));
#133896=CARTESIAN_POINT('Ctrl Pts',(-7.236539753,4.042023177,1.970404122));
#133897=CARTESIAN_POINT('Ctrl Pts',(-7.128964961,4.10772842,2.365485134));
#133898=CARTESIAN_POINT('Ctrl Pts',(-6.979018621,4.172899507,2.746506705));
#133899=CARTESIAN_POINT('Ctrl Pts',(-6.929092656,4.042023177,2.133113913));
#133900=CARTESIAN_POINT('Ctrl Pts',(-6.812634675,4.10772842,2.511409761));
#133901=CARTESIAN_POINT('Ctrl Pts',(-6.65568528,4.172899507,2.874778854));
#133902=CARTESIAN_POINT('',(-6.97901861874018,4.17289950600424,2.74650671479494));
#133903=CARTESIAN_POINT('',(-6.81735194381297,4.17289950413623,2.81064279571972));
#133904=CARTESIAN_POINT('',(-7.16668367558851,4.08221031168703,2.21102806139634));
#133905=CARTESIAN_POINT('Origin',(0.185026142951854,4.01787919238931,-0.0462698970781572));
#133906=CARTESIAN_POINT('Ctrl Pts',(-6.92770126735829,4.04280735924753,
2.13762839408099));
#133907=CARTESIAN_POINT('Ctrl Pts',(-6.96748634201239,4.04969801232502,
2.14980430828143));
#133908=CARTESIAN_POINT('Ctrl Pts',(-7.00731521574551,4.05642175377696,
2.16201682517382));
#133909=CARTESIAN_POINT('Ctrl Pts',(-7.08696274687549,4.06954550711632,
2.18648066255977));
#133910=CARTESIAN_POINT('Ctrl Pts',(-7.12682619520053,4.07595289337755,
2.19874574381524));
#133911=CARTESIAN_POINT('Ctrl Pts',(-7.16668367599155,4.0822103116869,2.21102806008848));
#133912=CARTESIAN_POINT('Ctrl Pts',(-7.31285186,4.172899507,1.664991795));
#133913=CARTESIAN_POINT('Ctrl Pts',(-7.222120769,4.107307013,2.063494074));
#133914=CARTESIAN_POINT('Ctrl Pts',(-7.088624029,4.04203077,2.449777414));
#133915=CARTESIAN_POINT('Ctrl Pts',(-7.118071532,4.172899507,1.376792527));
#133916=CARTESIAN_POINT('Ctrl Pts',(-7.043045404,4.107307013,1.764680561));
#133917=CARTESIAN_POINT('Ctrl Pts',(-6.926314018,4.04203077,2.142119073));
#133918=CARTESIAN_POINT('',(-7.31285186038333,4.17289950685237,1.66499180012521));
#133919=CARTESIAN_POINT('Origin',(0.187653197368192,4.16071405450739,-0.0447255136504804));
#133920=CARTESIAN_POINT('',(-7.2154616962758,4.17289950678353,1.52089215969156));
#133921=CARTESIAN_POINT('Origin',(6.40112962635442E-13,4.26419218500022,
-2.50992802930394E-13));
#133922=CARTESIAN_POINT('',(-7.16528730476381,4.26310680663001,2.21554910444215));
#133923=CARTESIAN_POINT('Origin',(0.178374116608985,4.16071715854707,-0.0723092164665737));
#133924=CARTESIAN_POINT('Origin',(0.184411326266831,4.01799491751039,-0.0166565351205841));
#133925=CARTESIAN_POINT('Ctrl Pts',(-7.490932116,4.042023177,0.368695032));
#133926=CARTESIAN_POINT('Ctrl Pts',(-7.470803103,4.10772842,0.77766467));
#133927=CARTESIAN_POINT('Ctrl Pts',(-7.4062708,4.172899507,1.182012199));
#133928=CARTESIAN_POINT('Ctrl Pts',(-7.225650757,4.042023177,0.593692797));
#133929=CARTESIAN_POINT('Ctrl Pts',(-7.193237924,4.10772842,0.988179322000001));
#133930=CARTESIAN_POINT('Ctrl Pts',(-7.118071532,4.172899507,1.376792527));
#133931=CARTESIAN_POINT('',(-7.40627079988748,4.17289950600422,1.18201220907727));
#133932=CARTESIAN_POINT('',(-7.26217116295607,4.17289950413623,1.27940238027803));
#133933=CARTESIAN_POINT('',(-7.47443626910764,4.08221031167934,0.618710309512847));
#133934=CARTESIAN_POINT('Origin',(0.190646650037835,4.01787918147397,-0.00541292423114959));
#133935=CARTESIAN_POINT('Ctrl Pts',(-7.22526237813834,4.04280735921943,
0.598400839381963));
#133936=CARTESIAN_POINT('Ctrl Pts',(-7.26673476055614,4.04969801214614,
0.601739472284816));
#133937=CARTESIAN_POINT('Ctrl Pts',(-7.30825778633643,4.05642175343086,
0.605104436638636));
#133938=CARTESIAN_POINT('Ctrl Pts',(-7.39130220628258,4.06954550709366,
0.611874458356977));
#133939=CARTESIAN_POINT('Ctrl Pts',(-7.43287029924927,4.07595289336291,
0.615283325785464));
#133940=CARTESIAN_POINT('Ctrl Pts',(-7.47443626921981,4.08221031167921,
0.61871030815259));
#133941=CARTESIAN_POINT('Ctrl Pts',(-7.49980546600001,4.172899507,0.054018228));
#133942=CARTESIAN_POINT('Ctrl Pts',(-7.49686182800001,4.107307013,0.462708249));
#133943=CARTESIAN_POINT('Ctrl Pts',(-7.449525667,4.04203077,0.868658351));
#133944=CARTESIAN_POINT('Ctrl Pts',(-7.247624671,4.172899507,-0.185571088));
#133945=CARTESIAN_POINT('Ctrl Pts',(-7.257737073,4.107307013,0.209376739));
#133946=CARTESIAN_POINT('Ctrl Pts',(-7.224872925,4.04203077,0.603084746));
#133947=CARTESIAN_POINT('',(-7.49980546748518,4.17289950685237,0.0540182329483246));
#133948=CARTESIAN_POINT('Origin',(0.192880559441947,4.16071398945195,-0.00333997202822588));
#133949=CARTESIAN_POINT('',(-7.37371506848807,4.17289950678353,-0.0657764313371442));
#133950=CARTESIAN_POINT('Origin',(8.59555482346508E-13,4.264192185,1.95698492133634E-14));
#133951=CARTESIAN_POINT('',(-7.47404443556447,4.26310680659394,0.623425831355525));
#133952=CARTESIAN_POINT('Origin',(0.1897483654665,4.16071713900448,-0.0322735214081868));
#133953=CARTESIAN_POINT('Origin',(0.183680685919455,4.01799491410986,0.0233758684203914));
#133954=CARTESIAN_POINT('Ctrl Pts',(-7.39505682,4.042023177,-1.250253828));
#133955=CARTESIAN_POINT('Ctrl Pts',(-7.463314795,4.10772842,-0.846518529));
#133956=CARTESIAN_POINT('Ctrl Pts',(-7.487213987,4.172899507,-0.437751883));
#133957=CARTESIAN_POINT('Ctrl Pts',(-7.18434546000001,4.042023177,-0.973488735));
#133958=CARTESIAN_POINT('Ctrl Pts',(-7.237493363,4.10772842,-0.581257285));
#133959=CARTESIAN_POINT('Ctrl Pts',(-7.247624671,4.172899507,-0.185571088));
#133960=CARTESIAN_POINT('',(-7.48721398905837,4.17289950600422,-0.437751873144494));
#133961=CARTESIAN_POINT('',(-7.3674193297415,4.17289950413623,-0.311661467971566));
#133962=CARTESIAN_POINT('',(-7.43269253070425,4.08221031161394,-1.00253764896776));
#133963=CARTESIAN_POINT('Origin',(0.187352954992916,4.01787920562906,0.0356969993917453));
#133964=CARTESIAN_POINT('Ctrl Pts',(-7.18497825126012,4.04280735926989,
-0.968807273831972));
#133965=CARTESIAN_POINT('Ctrl Pts',(-7.22619874119893,4.04969801241923,
-0.974462032846668));
#133966=CARTESIAN_POINT('Ctrl Pts',(-7.26747435131031,4.05642175395236,
-0.980101962884917));
#133967=CARTESIAN_POINT('Ctrl Pts',(-7.35003259022942,4.06954550707542,
-0.991342315626475));
#133968=CARTESIAN_POINT('Ctrl Pts',(-7.39136164998044,4.07595289332165,
-0.99694905686827));
#133969=CARTESIAN_POINT('Ctrl Pts',(-7.43269253052555,4.08221031161382,
-1.00253765028944));
#133970=CARTESIAN_POINT('Ctrl Pts',(-7.336076504,4.172899507,-1.55948117));
#133971=CARTESIAN_POINT('Ctrl Pts',(-7.421057961,4.107307013,-1.159713301));
#133972=CARTESIAN_POINT('Ctrl Pts',(-7.462095765,4.04203077,-0.753078211));
#133973=CARTESIAN_POINT('Ctrl Pts',(-7.03828693500001,4.172899507,-1.739257605));
#133974=CARTESIAN_POINT('Ctrl Pts',(-7.133065024,4.107307013,-1.355717306));
#133975=CARTESIAN_POINT('Ctrl Pts',(-7.185604805,4.04203077,-0.964149153));
#133976=CARTESIAN_POINT('',(-7.33607650652361,4.17289950685235,-1.55948116547139));
#133977=CARTESIAN_POINT('Origin',(0.18908886836307,4.16071403517206,0.0382017074795551));
#133978=CARTESIAN_POINT('',(-7.1871817192009,4.17289950678353,-1.64936938880332));
#133979=CARTESIAN_POINT('Origin',(3.62123525610158E-13,4.26419218500022,
3.63749828868887E-14));
#133980=CARTESIAN_POINT('',(-7.43332355565574,4.26310680663769,-0.997848140298518));
#133981=CARTESIAN_POINT('Origin',(0.192249680943634,4.16071712908807,0.00927126714342946));
#133982=CARTESIAN_POINT('Origin',(0.174360938573022,4.01799497386905,0.0623152207350958));
#133983=CARTESIAN_POINT('Ctrl Pts',(-6.953396885,4.042023177,-2.810742208));
#133984=CARTESIAN_POINT('Ctrl Pts',(-7.106850181,4.10772842,-2.431119463));
#133985=CARTESIAN_POINT('Ctrl Pts',(-7.21806337,4.172899507,-2.037047174));
#133986=CARTESIAN_POINT('Ctrl Pts',(-6.807108153,4.042023177,-2.495151015));
#133987=CARTESIAN_POINT('Ctrl Pts',(-6.94333165600001,4.10772842,-2.123514947));
#133988=CARTESIAN_POINT('Ctrl Pts',(-7.038286935,4.172899507,-1.739257605));
#133989=CARTESIAN_POINT('',(-7.21806337412925,4.17289950600421,-2.03704716480384));
#133990=CARTESIAN_POINT('',(-7.12817515699226,4.17289950413623,-1.88815237254077));
#133991=CARTESIAN_POINT('',(-7.04340435027309,4.08221031169495,-2.57690806135675));
#133992=CARTESIAN_POINT('Origin',(0.175299420682953,4.0178792215071,0.0751379209236386));
#133993=CARTESIAN_POINT('Ctrl Pts',(-6.80873252634046,4.04280735930085,
-2.49071503621283));
#133994=CARTESIAN_POINT('Ctrl Pts',(-6.84777370212766,4.04969801315263,
-2.50509877828202));
#133995=CARTESIAN_POINT('Ctrl Pts',(-6.88687189803305,4.05642175546742,
-2.5194798876564));
#133996=CARTESIAN_POINT('Ctrl Pts',(-6.96508361896581,4.06954550714206,
-2.54820502489215));
#133997=CARTESIAN_POINT('Ctrl Pts',(-7.00424114463182,4.0759528933933,-2.56256520981103));
#133998=CARTESIAN_POINT('Ctrl Pts',(-7.04340434980117,4.08221031169484,
-2.5769080626454));
#133999=CARTESIAN_POINT('Ctrl Pts',(-6.829320759,4.172899507,-3.100060963));
#134000=CARTESIAN_POINT('Ctrl Pts',(-6.998253671,4.107307013,-2.727907945));
#134001=CARTESIAN_POINT('Ctrl Pts',(-7.125746559,4.04203077,-2.339601672));
#134002=CARTESIAN_POINT('Ctrl Pts',(-6.499846725,4.172899507,-3.21161837));
#134003=CARTESIAN_POINT('Ctrl Pts',(-6.67485878100001,4.107307013,-2.857419517));
#134004=CARTESIAN_POINT('Ctrl Pts',(-6.81034579,4.04203077,-2.48630051));
#134005=CARTESIAN_POINT('',(-6.82932076240721,4.17289950685237,-3.10006095915154));
#134006=CARTESIAN_POINT('Origin',(0.176456086776277,4.16071403607459,0.0779571854405042));
#134007=CARTESIAN_POINT('',(-6.6645837414277,4.17289950678353,-3.15583966770859));
#134008=CARTESIAN_POINT('Origin',(8.87744738831131E-13,4.26419218500111,
3.38921599118969E-13));
#134009=CARTESIAN_POINT('',(-7.0450287277557,4.26310680662765,-2.57246384257894));
#134010=CARTESIAN_POINT('Origin',(0.185761950671148,4.16071713387759,0.0503825143463937));
#134011=CARTESIAN_POINT('Origin',(0.156888685719833,4.01799496418505,0.0983408227819893));
#134012=CARTESIAN_POINT('Ctrl Pts',(-6.18660384,4.042023177,-4.239803406));
#134013=CARTESIAN_POINT('Ctrl Pts',(-6.418077152,4.10772842,-3.902043953));
#134014=CARTESIAN_POINT('Ctrl Pts',(-6.611404132,4.172899507,-3.541092403));
#134015=CARTESIAN_POINT('Ctrl Pts',(-6.111578035,4.042023177,-3.900142807));
#134016=CARTESIAN_POINT('Ctrl Pts',(-6.324507477,4.10772842,-3.56647941));
#134017=CARTESIAN_POINT('Ctrl Pts',(-6.499846725,4.172899507,-3.21161837));
#134018=CARTESIAN_POINT('',(-6.61140413801019,4.17289950600422,-3.54109239490403));
#134019=CARTESIAN_POINT('',(-6.55562543653299,4.17289950413623,-3.37635537090293));
#134020=CARTESIAN_POINT('',(-6.32477440992221,4.08221031163205,-4.03078511625019));
#134021=CARTESIAN_POINT('Origin',(0.155048372953193,4.01787918526179,0.111065323303753));
#134022=CARTESIAN_POINT('Ctrl Pts',(-6.11411803582838,4.04280735932927,
-3.89615973118788));
#134023=CARTESIAN_POINT('Ctrl Pts',(-6.14915437016196,4.04969801296718,
-3.91859988748003));
#134024=CARTESIAN_POINT('Ctrl Pts',(-6.1842469572818,4.05642175505077,-3.94104973009006));
#134025=CARTESIAN_POINT('Ctrl Pts',(-6.25445507828098,4.06954550710154,
-3.98591649891152));
#134026=CARTESIAN_POINT('Ctrl Pts',(-6.28961010744197,4.07595289334218,
-4.00835866113015));
#134027=CARTESIAN_POINT('Ctrl Pts',(-6.32477440920043,4.08221031163192,
-4.03078511738196));
#134028=CARTESIAN_POINT('Ctrl Pts',(-6.00323356500001,4.172899507,-4.49568535));
#134029=CARTESIAN_POINT('Ctrl Pts',(-6.248218817,4.107307013,-4.168548645));
#134030=CARTESIAN_POINT('Ctrl Pts',(-6.456205362,4.04203077,-3.81672796));
#134031=CARTESIAN_POINT('Ctrl Pts',(-5.657480906,4.172899507,-4.533807429));
#134032=CARTESIAN_POINT('Ctrl Pts',(-5.904543561,4.107307013,-4.225511967));
#134033=CARTESIAN_POINT('Ctrl Pts',(-6.116642575,4.04203077,-3.892195218));
#134034=CARTESIAN_POINT('',(-6.00323356915964,4.17289950685237,-4.49568534697083));
#134035=CARTESIAN_POINT('Origin',(0.155572222910411,4.16071401278495,0.114067469851924));
#134036=CARTESIAN_POINT('',(-5.83035723468127,4.17289950678352,-4.51474639055731));
#134037=CARTESIAN_POINT('Origin',(9.14632952708772E-13,4.26419218500022,
5.24970691917481E-13));
#134038=CARTESIAN_POINT('',(-6.32731618628048,4.26310680660589,-4.02679399416042));
#134039=CARTESIAN_POINT('Origin',(0.170588519435007,4.16071713402905,0.0891381260390134));
#134040=CARTESIAN_POINT('Origin',(0.132080173369563,4.01799495212349,0.129767979784806));
#134041=CARTESIAN_POINT('Ctrl Pts',(-5.130532076,4.042023177,-5.47061610999999));
#134042=CARTESIAN_POINT('Ctrl Pts',(-5.429201969,4.10772842,-5.190513205));
#134043=CARTESIAN_POINT('Ctrl Pts',(-5.695602984,4.172899507,-4.879560087));
#134044=CARTESIAN_POINT('Ctrl Pts',(-5.130277321,4.042023177,-5.122768257));
#134045=CARTESIAN_POINT('Ctrl Pts',(-5.409956358,4.10772842,-4.84267926));
#134046=CARTESIAN_POINT('Ctrl Pts',(-5.657480906,4.172899507,-4.533807429));
#134047=CARTESIAN_POINT('',(-5.69560299159702,4.17289950600423,-4.87956008041204));
#134048=CARTESIAN_POINT('',(-5.67654195619809,4.17289950413623,-4.70668374449444));
#134049=CARTESIAN_POINT('',(-5.31040504833037,4.08221031160588,-5.29618713926893));
#134050=CARTESIAN_POINT('Origin',(0.127547362614432,4.01787918058668,0.141799201134928));
#134051=CARTESIAN_POINT('Ctrl Pts',(-5.13361418158609,4.04280735933178,
-5.11942432679469));
#134052=CARTESIAN_POINT('Ctrl Pts',(-5.16300740977581,4.04969801160511,
-5.14887161527873));
#134053=CARTESIAN_POINT('Ctrl Pts',(-5.1924534920505,4.05642175216957,-5.17834045498303));
#134054=CARTESIAN_POINT('Ctrl Pts',(-5.25137516991062,4.06954550705694,
-5.23725094732631));
#134055=CARTESIAN_POINT('Ctrl Pts',(-5.28088389259553,4.07595289330727,
-5.26672571649307));
#134056=CARTESIAN_POINT('Ctrl Pts',(-5.31040504739098,4.08221031160576,
-5.29618714021025));
#134057=CARTESIAN_POINT('Ctrl Pts',(-4.896441841,4.172899507,-5.681096487));
#134058=CARTESIAN_POINT('Ctrl Pts',(-5.206024196,4.107307013,-5.414272644));
#134059=CARTESIAN_POINT('Ctrl Pts',(-5.484779179,4.04203077,-5.11538829));
#134060=CARTESIAN_POINT('Ctrl Pts',(-4.550577568,4.172899507,-5.64400069100001));
#134061=CARTESIAN_POINT('Ctrl Pts',(-4.85813844599999,4.107307013,-5.396024174));
#134062=CARTESIAN_POINT('Ctrl Pts',(-5.136931951,4.04203077,-5.116095203));
#134063=CARTESIAN_POINT('',(-4.89644184573234,4.17289950685235,-5.68109648492861));
#134064=CARTESIAN_POINT('Origin',(0.127413845258664,4.16071401356712,0.144844019211612));
#134065=CARTESIAN_POINT('',(-4.72350970347312,4.17289950678353,-5.66254858985659));
#134066=CARTESIAN_POINT('Origin',(7.67615138119737E-13,4.26419218499978,
8.51315545835618E-13));
#134067=CARTESIAN_POINT('',(-5.31374537261658,4.26310680661091,-5.29283573454961));
#134068=CARTESIAN_POINT('Origin',(0.14743797145068,4.16071715078108,0.12372539659845));
#134069=CARTESIAN_POINT('Origin',(0.101096018227911,4.01799493201509,0.155127520179251));
#134070=CARTESIAN_POINT('Ctrl Pts',(-3.834562334,4.042023177,-6.445628884));
#134071=CARTESIAN_POINT('Ctrl Pts',(-4.186463335,4.10772842,-6.236279827));
#134072=CARTESIAN_POINT('Ctrl Pts',(-4.513481772,4.172899507,-5.989864965));
#134073=CARTESIAN_POINT('Ctrl Pts',(-3.909090541,4.042023177,-6.105858756));
#134074=CARTESIAN_POINT('Ctrl Pts',(-4.242441693,4.10772842,-5.89244081));
#134075=CARTESIAN_POINT('Ctrl Pts',(-4.550577568,4.172899507,-5.64400069100001));
#134076=CARTESIAN_POINT('',(-4.51348178085793,4.17289950600422,-5.98986496017105));
#134077=CARTESIAN_POINT('',(-4.53202968383958,4.17289950413623,-5.81693281721745));
#134078=CARTESIAN_POINT('',(-4.0477270485313,4.08221031162645,-6.31394533827614));
#134079=CARTESIAN_POINT('Origin',(0.0940831213956261,4.01787919159973,0.16590348653861));
#134080=CARTESIAN_POINT('Ctrl Pts',(-3.91306823383849,4.04280735934069,
-6.10331033138982));
#134081=CARTESIAN_POINT('Ctrl Pts',(-3.93544396832325,4.04969801166272,
-6.13838783415081));
#134082=CARTESIAN_POINT('Ctrl Pts',(-3.95786668829155,4.05642175228402,
-6.17349774639542));
#134083=CARTESIAN_POINT('Ctrl Pts',(-4.00274679512569,4.06954550706758,
-6.24369736271112));
#134084=CARTESIAN_POINT('Ctrl Pts',(-4.02522941608651,4.07595289331948,
-6.27882653129195));
#134085=CARTESIAN_POINT('Ctrl Pts',(-4.04772704740326,4.08221031162632,
-6.31394533899881));
#134086=CARTESIAN_POINT('Ctrl Pts',(-3.560697939,4.172899507,-6.600865866));
#134087=CARTESIAN_POINT('Ctrl Pts',(-3.92040167,4.107307013,-6.406831272));
#134088=CARTESIAN_POINT('Ctrl Pts',(-4.256890817,4.04203077,-6.174858749));
#134089=CARTESIAN_POINT('Ctrl Pts',(-3.23089428,4.172899507,-6.49028675400001));
#134090=CARTESIAN_POINT('Ctrl Pts',(-3.584572177,4.107307013,-6.314224288));
#134091=CARTESIAN_POINT('Ctrl Pts',(-3.917024099,4.04203077,-6.100772263));
#134092=CARTESIAN_POINT('',(-3.56069794407931,4.17289950685236,-6.60086586499261));
#134093=CARTESIAN_POINT('Origin',(0.0932976583525053,4.16071400382663,0.168847627684026));
#134094=CARTESIAN_POINT('',(-3.39579610831299,4.17289950678352,-6.54557631061581));
#134095=CARTESIAN_POINT('Origin',(4.91360424570431E-13,4.26419218500067,
7.63278329429795E-13));
#134096=CARTESIAN_POINT('',(-4.05170973090138,4.2631068066114,-6.31139035807637));
#134097=CARTESIAN_POINT('Origin',(0.11739369948572,4.16071712351179,0.152527655333695));
#134098=CARTESIAN_POINT('Origin',(0.0653845985702356,4.01799498159655,0.17323333309049));
#134099=CARTESIAN_POINT('Ctrl Pts',(-2.359292718,4.042023177,-7.119251215));
#134100=CARTESIAN_POINT('Ctrl Pts',(-2.747970329,4.10772842,-6.990444937));
#134101=CARTESIAN_POINT('Ctrl Pts',(-3.120315168,4.172899507,-6.820090414));
#134102=CARTESIAN_POINT('Ctrl Pts',(-2.505119032,4.042023177,-6.803446085));
#134103=CARTESIAN_POINT('Ctrl Pts',(-2.876555169,4.10772842,-6.666678376));
#134104=CARTESIAN_POINT('Ctrl Pts',(-3.23089428,4.172899507,-6.490286754));
#134105=CARTESIAN_POINT('',(-3.12031517768316,4.17289950600422,-6.82009041119266));
#134106=CARTESIAN_POINT('',(-3.17560473983395,4.17289950413623,-6.65518857644464));
#134107=CARTESIAN_POINT('',(-2.59578183050533,4.08221031170026,-7.03647047076548));
#134108=CARTESIAN_POINT('Origin',(0.0562190675631685,4.01787921877911,0.182249585017943));
#134109=CARTESIAN_POINT('Ctrl Pts',(-2.50955156393116,4.04280735929469,
-6.80181232839606));
#134110=CARTESIAN_POINT('Ctrl Pts',(-2.52386354156956,4.04969801243914,
-6.84087986467192));
#134111=CARTESIAN_POINT('Ctrl Pts',(-2.53821443956852,4.05642175397371,
-6.87998915422951));
#134112=CARTESIAN_POINT('Ctrl Pts',(-2.56695442848329,4.06954550713191,
-6.95819542901028));
#134113=CARTESIAN_POINT('Ctrl Pts',(-2.58135968549397,4.0759528933911,-6.99733639606272));
#134114=CARTESIAN_POINT('Ctrl Pts',(-2.59578182921528,4.08221031170013,
-7.03647047124092));
#134115=CARTESIAN_POINT('Ctrl Pts',(-2.058459759,4.172899507,-7.211986094));
#134116=CARTESIAN_POINT('Ctrl Pts',(-2.451465519,4.107307013,-7.09981359));
#134117=CARTESIAN_POINT('Ctrl Pts',(-2.829954972,4.04203077,-6.945599676));
#134118=CARTESIAN_POINT('Ctrl Pts',(-1.760137966,4.172899507,-7.033094222));
#134119=CARTESIAN_POINT('Ctrl Pts',(-2.143395296,4.107307013,-6.937178292));
#134120=CARTESIAN_POINT('Ctrl Pts',(-2.513960553,4.04203077,-6.800183993));
#134121=CARTESIAN_POINT('',(-2.05845976415483,4.17289950685236,-7.21198609410644));
#134122=CARTESIAN_POINT('Origin',(0.0548191946948218,4.16071399001688,0.184956388900183));
#134123=CARTESIAN_POINT('',(-1.90929886120836,4.17289950678353,-7.12254015834624));
#134124=CARTESIAN_POINT('Origin',(2.99239799605999E-14,4.26419218500089,
5.03069808033274E-14));
#134125=CARTESIAN_POINT('',(-2.60022064544648,4.26310680662107,-7.03483138298938));
#134126=CARTESIAN_POINT('Origin',(0.0818601306484634,4.16071714532607,0.174197752453119));
#134127=CARTESIAN_POINT('Origin',(0.0266158912002012,4.01799497142736,0.18323895048609));
#134128=CARTESIAN_POINT('Ctrl Pts',(-0.773705198,4.042023177,-7.459985273));
#134129=CARTESIAN_POINT('Ctrl Pts',(-1.180985284,4.10772842,-7.41774461));
#134130=CARTESIAN_POINT('Ctrl Pts',(-1.581246094,4.172899507,-7.331416015));
#134131=CARTESIAN_POINT('Ctrl Pts',(-0.984010941,4.042023177,-7.18291183800001));
#134132=CARTESIAN_POINT('Ctrl Pts',(-1.376164122,4.10772842,-7.129189471));
#134133=CARTESIAN_POINT('Ctrl Pts',(-1.760137966,4.172899507,-7.033094222));
#134134=CARTESIAN_POINT('',(-1.58124610403693,4.17289950600423,-7.33141601435202));
#134135=CARTESIAN_POINT('',(-1.67069204708794,4.17289950413623,-7.18225511452511));
#134136=CARTESIAN_POINT('',(-1.02246073937731,4.08221031165689,-7.429978063712));
#134137=CARTESIAN_POINT('Origin',(0.0157264105232788,4.01787917543695,0.190074088263203));
#134138=CARTESIAN_POINT('Ctrl Pts',(-0.988691052623827,4.04280735930237,
-7.1822691405059));
#134139=CARTESIAN_POINT('Ctrl Pts',(-0.994270058771183,4.04969801240803,
-7.22349995134818));
#134140=CARTESIAN_POINT('Ctrl Pts',(-0.999878099569674,4.05642175390003,
-7.26477990599238));
#134141=CARTESIAN_POINT('Ctrl Pts',(-1.01113412626995,4.06954550710363,
-7.34733600980363));
#134142=CARTESIAN_POINT('Ctrl Pts',(-1.0167884454357,4.07595289335518,-7.38865858715136));
#134143=CARTESIAN_POINT('Ctrl Pts',(-1.02246073803572,4.08221031165677,
-7.42997806389619));
#134144=CARTESIAN_POINT('Ctrl Pts',(-0.459970288,4.172899507,-7.485881867));
#134145=CARTESIAN_POINT('Ctrl Pts',(-0.867901564,4.107307013,-7.46081651499999));
#134146=CARTESIAN_POINT('Ctrl Pts',(-1.270693578,4.04203077,-7.391572081));
#134147=CARTESIAN_POINT('Ctrl Pts',(-0.207079558,4.172899507,-7.247042021));
#134148=CARTESIAN_POINT('Ctrl Pts',(-0.601995634,4.107307013,-7.23575754900001));
#134149=CARTESIAN_POINT('Ctrl Pts',(-0.993347006,4.04203077,-7.181626677));
#134150=CARTESIAN_POINT('',(-0.459970293037299,4.17289950685236,-7.48588186821977));
#134151=CARTESIAN_POINT('Origin',(0.0137773947320928,4.16071402757819,0.192416766574395));
#134152=CARTESIAN_POINT('',(-0.333524921664125,4.17289950678352,-7.36646194406049));
#134153=CARTESIAN_POINT('Origin',(-1.62386380384016E-13,4.26419218499956,
-1.11802928026705E-12));
#134154=CARTESIAN_POINT('',(-1.02714813218712,4.26310680660984,-7.42933151171826));
#134155=CARTESIAN_POINT('Origin',(0.0424989310837132,4.1607171084661,0.187722585433427));
#134156=CARTESIAN_POINT('Origin',(-0.0133973344608364,4.0179949710456,0.184676628010878));
#134157=CARTESIAN_POINT('Ctrl Pts',(0.848059918,4.042023177,-7.451898709));
#134158=CARTESIAN_POINT('Ctrl Pts',(0.441221319,4.10772842,-7.49819879));
#134159=CARTESIAN_POINT('Ctrl Pts',(0.031760289,4.172899507,-7.499932752));
#134160=CARTESIAN_POINT('Ctrl Pts',(0.583108408,4.042023177,-7.22651261599999));
#134161=CARTESIAN_POINT('Ctrl Pts',(0.188574829,4.10772842,-7.25834759));
#134162=CARTESIAN_POINT('Ctrl Pts',(-0.207079558,4.172899507,-7.247042021));
#134163=CARTESIAN_POINT('',(0.0317602790403005,4.17289950600422,-7.4999327535199));
#134164=CARTESIAN_POINT('',(-0.0876596520429175,4.17289950413623,-7.37348738629144));
#134165=CARTESIAN_POINT('',(0.598669479685729,4.08221031163955,-7.47606814066269));
#134166=CARTESIAN_POINT('Origin',(-0.0255015617587158,4.01787924343035,
0.189010783131128));
#134167=CARTESIAN_POINT('Ctrl Pts',(0.578399553974621,4.0428073592547,-7.22689102994081));
#134168=CARTESIAN_POINT('Ctrl Pts',(0.581814387242482,4.04969801196833,
-7.2683572062548));
#134169=CARTESIAN_POINT('Ctrl Pts',(0.585211429059266,4.05642175301284,
-7.30987761848275));
#134170=CARTESIAN_POINT('Ctrl Pts',(0.591965684311098,4.06954550708528,
-7.39292332495118));
#134171=CARTESIAN_POINT('Ctrl Pts',(0.595326692553784,4.07595289334113,
-7.43449531494571));
#134172=CARTESIAN_POINT('Ctrl Pts',(0.598669481027308,4.08221031163943,
-7.47606814055483));
#134173=CARTESIAN_POINT('Ctrl Pts',(1.160026882,4.172899507,-7.409746125));
#134174=CARTESIAN_POINT('Ctrl Pts',(0.756244503,4.107307013,-7.472959952));
#134175=CARTESIAN_POINT('Ctrl Pts',(0.347984036,4.04203077,-7.49192279100001));
#134176=CARTESIAN_POINT('Ctrl Pts',(1.355661661,4.172899507,-7.12212619));
#134177=CARTESIAN_POINT('Ctrl Pts',(0.967552675,4.107307013,-7.196000825));
#134178=CARTESIAN_POINT('Ctrl Pts',(0.573714344,4.04203077,-7.227264479));
#134179=CARTESIAN_POINT('',(1.16002687738136,4.17289950685236,-7.40974612725279));
#134180=CARTESIAN_POINT('Origin',(-0.0279086400380241,4.16071403958437,
0.190880066307909));
#134181=CARTESIAN_POINT('',(1.25784427281764,4.17289950678353,-7.2659361572719));
#134182=CARTESIAN_POINT('Origin',(1.11986225956491E-13,4.26419218500089,
-5.11309744544164E-13));
#134183=CARTESIAN_POINT('',(0.59395268554274,4.26310680660941,-7.47644435575336));
#134184=CARTESIAN_POINT('Origin',(0.001150519444039,4.16071710816118,0.192469726632061));
#134185=CARTESIAN_POINT('Origin',(-0.0527841183711129,4.01799497364709,
0.17747896038271));
#134186=CARTESIAN_POINT('Ctrl Pts',(2.430170694,4.042023177,-7.09536964500001));
#134187=CARTESIAN_POINT('Ctrl Pts',(2.042796905,4.10772842,-7.228045528));
#134188=CARTESIAN_POINT('Ctrl Pts',(1.643281596,4.172899507,-7.317760969));
#134189=CARTESIAN_POINT('Ctrl Pts',(2.122962255,4.042023177,-6.932209696));
#134190=CARTESIAN_POINT('Ctrl Pts',(1.744496231,4.10772842,-7.048113443));
#134191=CARTESIAN_POINT('Ctrl Pts',(1.355661661,4.172899507,-7.12212619));
#134192=CARTESIAN_POINT('',(1.64328158659124,4.17289950600421,-7.31776097262514));
#134193=CARTESIAN_POINT('',(1.49947161132239,4.17289950413623,-7.21994358306752));
#134194=CARTESIAN_POINT('',(2.19180657900837,4.08221031164392,-7.1725855806994));
#134195=CARTESIAN_POINT('Origin',(-0.0655370874021338,4.01787918223643,
0.17910972065395));
#134196=CARTESIAN_POINT('Ctrl Pts',(2.11844483962398,4.04280735919209,-6.93359152718499));
#134197=CARTESIAN_POINT('Ctrl Pts',(2.13069383942245,4.04969801264247,-6.97335416331008));
#134198=CARTESIAN_POINT('Ctrl Pts',(2.14293712315487,4.05642175450617,-7.0131735929134));
#134199=CARTESIAN_POINT('Ctrl Pts',(2.16738583696148,4.06954550708139,-7.09282576247492));
#134200=CARTESIAN_POINT('Ctrl Pts',(2.17960501571345,4.07595289334154,-7.13270330499154));
#134201=CARTESIAN_POINT('Ctrl Pts',(2.19180658029741,4.0822103116438,-7.17258558030506));
#134202=CARTESIAN_POINT('Ctrl Pts',(2.725782484,4.172899507,-6.987138889));
#134203=CARTESIAN_POINT('Ctrl Pts',(2.345029417,4.107307013,-7.135676088));
#134204=CARTESIAN_POINT('Ctrl Pts',(1.950390303,4.04203077,-7.241959518));
#134205=CARTESIAN_POINT('Ctrl Pts',(2.855013647,4.172899507,-6.664187653));
#134206=CARTESIAN_POINT('Ctrl Pts',(2.491859296,4.107307013,-6.8197671));
#134207=CARTESIAN_POINT('Ctrl Pts',(2.113949448,4.04203077,-6.934963427));
#134208=CARTESIAN_POINT('',(2.72578247997462,4.17289950685236,-6.98713889219217));
#134209=CARTESIAN_POINT('Origin',(-0.0682896670251204,4.16071402437646,
0.180417702860357));
#134210=CARTESIAN_POINT('',(2.79039806673785,4.17289950678351,-6.82566327049396));
#134211=CARTESIAN_POINT('Origin',(-3.10732342634346E-13,4.26419218500044,
8.50014503228635E-13));
#134212=CARTESIAN_POINT('',(2.18728093607448,4.26310680608004,-7.17396697094151));
#134213=CARTESIAN_POINT('Origin',(-0.0402517053402771,4.16071713026298,
0.188217278569863));
#134214=CARTESIAN_POINT('Origin',(-0.0897029231216462,4.01799491305414,
0.161982952090527));
#134215=CARTESIAN_POINT('Ctrl Pts',(3.89864939,4.042023177,-6.407068982));
#134216=CARTESIAN_POINT('Ctrl Pts',(3.548853577,4.10772842,-6.61991689));
#134217=CARTESIAN_POINT('Ctrl Pts',(3.177964882,4.172899507,-6.793418816));
#134218=CARTESIAN_POINT('Ctrl Pts',(3.563548747,4.042023177,-6.313764355));
#134219=CARTESIAN_POINT('Ctrl Pts',(3.218846929,4.10772842,-6.508317345));
#134220=CARTESIAN_POINT('Ctrl Pts',(2.855013647,4.172899507,-6.664187653));
#134221=CARTESIAN_POINT('',(3.17796487359751,4.17289950600422,-6.79341882156139));
#134222=CARTESIAN_POINT('',(3.01648924849091,4.17289950413623,-6.7288032416768));
#134223=CARTESIAN_POINT('',(3.68245723873874,4.0822103116389,-6.53372089046924));
#134224=CARTESIAN_POINT('Origin',(-0.102508252357332,4.01787918946685,0.160833875721125));
#134225=CARTESIAN_POINT('Ctrl Pts',(3.55943399894128,4.04280735921392,-6.31608499055302));
#134226=CARTESIAN_POINT('Ctrl Pts',(3.57994441221785,4.04969801158654,-6.35228481986496));
#134227=CARTESIAN_POINT('Ctrl Pts',(3.60046145125465,4.05642175224883,-6.38854134233796));
#134228=CARTESIAN_POINT('Ctrl Pts',(3.6414614367487,4.06954550705898,-6.46107555004328));
#134229=CARTESIAN_POINT('Ctrl Pts',(3.66196743080507,4.07595289332575,-6.49739401557589));
#134230=CARTESIAN_POINT('Ctrl Pts',(3.68245723991077,4.08221031163877,-6.53372088980819));
#134231=CARTESIAN_POINT('Ctrl Pts',(4.164083527,4.172899507,-6.23782080400001));
#134232=CARTESIAN_POINT('Ctrl Pts',(3.824163362,4.107307013,-6.46473594));
#134233=CARTESIAN_POINT('Ctrl Pts',(3.461598487,4.04203077,-6.653370267));
#134234=CARTESIAN_POINT('Ctrl Pts',(4.220868368,4.172899507,-5.894639109));
#134235=CARTESIAN_POINT('Ctrl Pts',(3.899649346,4.107307013,-6.124648645));
#134236=CARTESIAN_POINT('Ctrl Pts',(3.555338625,4.04203077,-6.318391192));
#134237=CARTESIAN_POINT('',(4.1640835237513,4.17289950685234,-6.23782080798759));
#134238=CARTESIAN_POINT('Origin',(-0.105477635539921,4.16071403000556,0.161519491255585));
#134239=CARTESIAN_POINT('',(4.19247594860009,4.17289950678352,-6.06622995573972));
#134240=CARTESIAN_POINT('Origin',(3.38921599118969E-13,4.26419218499978,
-6.4098032437343E-13));
#134241=CARTESIAN_POINT('',(3.67833436109936,4.26310680662289,-6.53604286388211));
#134242=CARTESIAN_POINT('Origin',(-0.0797718658867791,4.16071714068479,
0.175164068949367));
#134243=CARTESIAN_POINT('Origin',(-0.122427020027684,4.01799493636923,0.138912015982894));
#134244=CARTESIAN_POINT('Ctrl Pts',(5.184831573,4.042023177,-5.419180894));
#134245=CARTESIAN_POINT('Ctrl Pts',(4.88896980099999,4.10772842,-5.702248296));
#134246=CARTESIAN_POINT('Ctrl Pts',(4.56405006300001,4.172899507,-5.951423949));
#134247=CARTESIAN_POINT('Ctrl Pts',(4.837507661,4.042023177,-5.40009441));
#134248=CARTESIAN_POINT('Ctrl Pts',(4.542687921,4.10772842,-5.66419956100001));
#134249=CARTESIAN_POINT('Ctrl Pts',(4.220868368,4.172899507,-5.894639109));
#134250=CARTESIAN_POINT('',(4.56405005599778,4.17289950600422,-5.95142395623466));
#134251=CARTESIAN_POINT('',(4.39245920140799,4.17289950413623,-5.92303153945049));
#134252=CARTESIAN_POINT('',(5.00092029153408,4.08221031166126,-5.58934667322293));
#134253=CARTESIAN_POINT('Origin',(-0.134686198386177,4.01787920240881,0.135037443744226));
#134254=CARTESIAN_POINT('Ctrl Pts',(4.83398798137622,4.0428073592445,-5.40324533971125));
#134255=CARTESIAN_POINT('Ctrl Pts',(4.86180076688022,4.04969801186075,-5.43418970570736));
#134256=CARTESIAN_POINT('Ctrl Pts',(4.8896322108278,4.05642175280369,-5.46518801533919));
#134257=CARTESIAN_POINT('Ctrl Pts',(4.94526634776557,4.06954550707249,-5.52721262610302));
#134258=CARTESIAN_POINT('Ctrl Pts',(4.97310031961993,4.07595289334174,-5.55827380351772));
#134259=CARTESIAN_POINT('Ctrl Pts',(5.00092029254455,4.08221031166114,-5.58934667231826));
#134260=CARTESIAN_POINT('Ctrl Pts',(5.407676652,4.172899507,-5.19682915100001));
#134261=CARTESIAN_POINT('Ctrl Pts',(5.12448367900001,4.107307013,-5.491511925));
#134262=CARTESIAN_POINT('Ctrl Pts',(4.810946174,4.04203077,-5.753676817));
#134263=CARTESIAN_POINT('Ctrl Pts',(5.389359975,4.172899507,-4.84946379100001));
#134264=CARTESIAN_POINT('Ctrl Pts',(5.125096127,4.107307013,-5.143148427));
#134265=CARTESIAN_POINT('Ctrl Pts',(4.83048412,4.04203077,-5.406378008));
#134266=CARTESIAN_POINT('',(5.40767664967603,4.17289950685236,-5.19682915561212));
#134267=CARTESIAN_POINT('Origin',(-0.13773348277981,4.16071402875705,0.135068604265487));
#134268=CARTESIAN_POINT('',(5.39851831441093,4.17289950678353,-5.023146470021));
#134269=CARTESIAN_POINT('Origin',(-1.61762964134837E-13,4.26419218499978,
1.77375475418629E-13));
#134270=CARTESIAN_POINT('',(4.99739295983041,4.26310680661695,-5.59250065718638));
#134271=CARTESIAN_POINT('Origin',(-0.115561917034222,4.1607171309572,0.153920221420748));
#134272=CARTESIAN_POINT('Origin',(-0.149426904978411,4.0179949497126,0.109346319510427));
#134273=CARTESIAN_POINT('Ctrl Pts',(6.228576794,4.042023177,-4.17789793));
#134274=CARTESIAN_POINT('Ctrl Pts',(6.00048323,4.10772842,-4.517948909));
#134275=CARTESIAN_POINT('Ctrl Pts',(5.736725335,4.172899507,-4.831147114));
#134276=CARTESIAN_POINT('Ctrl Pts',(5.88527009200001,4.042023177,-4.233922052));
#134277=CARTESIAN_POINT('Ctrl Pts',(5.654117875,4.10772842,-4.555230101));
#134278=CARTESIAN_POINT('Ctrl Pts',(5.389359975,4.172899507,-4.849463791));
#134279=CARTESIAN_POINT('',(5.73672532969533,4.17289950600421,-4.8311471225858));
#134280=CARTESIAN_POINT('',(5.563042643484,4.17289950413623,-4.84030546573553));
#134281=CARTESIAN_POINT('',(6.08554586918542,4.08221031174222,-4.38362081754647));
#134282=CARTESIAN_POINT('Origin',(-0.160566649509389,4.01787920792561,0.102927005237378));
#134283=CARTESIAN_POINT('Ctrl Pts',(5.88251005789048,4.0428073592437,-4.23775594170643));
#134284=CARTESIAN_POINT('Ctrl Pts',(5.91632472470477,4.04969801284624,-4.26199792235454));
#134285=CARTESIAN_POINT('Ctrl Pts',(5.95016921108538,4.05642175488811,-4.28628857520854));
#134286=CARTESIAN_POINT('Ctrl Pts',(6.01783610026202,4.06954550714686,-4.33490338265932));
#134287=CARTESIAN_POINT('Ctrl Pts',(6.05169656428838,4.0759528934186,-4.35925488582192));
#134288=CARTESIAN_POINT('Ctrl Pts',(6.08554587000034,4.08221031174209,-4.38362081641441));
#134289=CARTESIAN_POINT('Ctrl Pts',(6.39841282800001,4.172899507,-3.912839543));
#134290=CARTESIAN_POINT('Ctrl Pts',(6.18518883400001,4.107307013,-4.261510916));
#134291=CARTESIAN_POINT('Ctrl Pts',(5.935339364,4.04203077,-4.584947834));
#134292=CARTESIAN_POINT('Ctrl Pts',(6.30585110000001,4.172899507,-3.577532936));
#134293=CARTESIAN_POINT('Ctrl Pts',(6.110899109,4.107307013,-3.921160304));
#134294=CARTESIAN_POINT('Ctrl Pts',(5.879761546,4.04203077,-4.241568597));
#134295=CARTESIAN_POINT('',(6.3984128267292,4.17289950685238,-3.91283954796789));
#134296=CARTESIAN_POINT('Origin',(-0.163549219894527,4.16071400496938,0.102302234735868));
#134297=CARTESIAN_POINT('',(6.35213196467917,4.17289950678353,-3.74518623834807));
#134298=CARTESIAN_POINT('Origin',(-4.0766001685455E-13,4.26419218500044,
3.18321757841744E-13));
#134299=CARTESIAN_POINT('',(6.082779017676,4.26310680662323,-4.3874593349363));
#134300=CARTESIAN_POINT('Origin',(-0.145948342705643,4.16071718925756,0.125479155657017));
#134301=CARTESIAN_POINT('Origin',(-0.169439547415214,4.01799495272587,0.0746674649441564));
#134302=CARTESIAN_POINT('Ctrl Pts',(6.98108068700001,4.042023177,-2.741261103));
#134303=CARTESIAN_POINT('Ctrl Pts',(6.831420733,4.10772842,-3.122395253));
#134304=CARTESIAN_POINT('Ctrl Pts',(6.641157706,4.172899507,-3.484971208));
#134305=CARTESIAN_POINT('Ctrl Pts',(6.657843835,4.042023177,-2.869776205));
#134306=CARTESIAN_POINT('Ctrl Pts',(6.501167561,4.10772842,-3.233263144));
#134307=CARTESIAN_POINT('Ctrl Pts',(6.3058511,4.172899507,-3.577532936));
#134308=CARTESIAN_POINT('',(6.64115770268627,4.17289950600422,-3.48497121750205));
#134309=CARTESIAN_POINT('',(6.47350439459849,4.17289950413623,-3.53125208740169));
#134310=CARTESIAN_POINT('',(6.88561808514311,4.08221031165632,-2.97292172430832));
#134311=CARTESIAN_POINT('Origin',(-0.178938489425086,4.01787919383781,0.066003326674286));
#134312=CARTESIAN_POINT('Ctrl Pts',(6.65597250213183,4.04280735929249,-2.87411378637647));
#134313=CARTESIAN_POINT('Ctrl Pts',(6.69420791073327,4.0496980130125,-2.89051984944257));
#134314=CARTESIAN_POINT('Ctrl Pts',(6.73248290502452,4.05642175518567,-2.90696703653915));
#134315=CARTESIAN_POINT('Ctrl Pts',(6.80901852467154,4.06954550710853,-2.93989887499767));
#134316=CARTESIAN_POINT('Ctrl Pts',(6.8473222031756,4.07595289335837,-2.95640205462647));
#134317=CARTESIAN_POINT('Ctrl Pts',(6.8856180856794,4.0822103116562,-2.97292172306514));
#134318=CARTESIAN_POINT('Ctrl Pts',(7.08996633,4.172899507,-2.445889906));
#134319=CARTESIAN_POINT('Ctrl Pts',(6.95668143399999,4.107307013,-2.832246392));
#134320=CARTESIAN_POINT('Ctrl Pts',(6.782202682,4.04203077,-3.201831785));
#134321=CARTESIAN_POINT('Ctrl Pts',(6.927487635,4.172899507,-2.138320617));
#134322=CARTESIAN_POINT('Ctrl Pts',(6.81096324000001,4.107307013,-2.515823084));
#134323=CARTESIAN_POINT('Ctrl Pts',(6.654107857,4.04203077,-2.878428153));
#134324=CARTESIAN_POINT('',(7.08996632982761,4.17289950685234,-2.44588991117874));
#134325=CARTESIAN_POINT('Origin',(-0.181717264224633,4.16071400914111,0.0647521217746));
#134326=CARTESIAN_POINT('',(7.00872698291568,4.17289950678351,-2.29210526022896));
#134327=CARTESIAN_POINT('Origin',(3.30898503042576E-13,4.26419218499911,
-1.23599047663348E-13));
#134328=CARTESIAN_POINT('',(6.88374108936043,4.26310680610879,-2.97726529079439));
#134329=CARTESIAN_POINT('Origin',(-0.169510333814914,4.16071715532136,0.0911709032238156));
#134330=CARTESIAN_POINT('Origin',(-0.181529238467207,4.01799496167259,0.0364971912151618));
#134331=CARTESIAN_POINT('Ctrl Pts',(7.407157006,4.042023177,-1.176445953));
#134332=CARTESIAN_POINT('Ctrl Pts',(7.342928594,4.10772842,-1.580841865));
#134333=CARTESIAN_POINT('Ctrl Pts',(7.235056924,4.172899507,-1.975841922));
#134334=CARTESIAN_POINT('Ctrl Pts',(7.1191042,4.042023177,-1.371442812));
#134335=CARTESIAN_POINT('Ctrl Pts',(7.044229877,4.10772842,-1.760112396));
#134336=CARTESIAN_POINT('Ctrl Pts',(6.92748763500001,4.172899507,-2.138320617));
#134337=CARTESIAN_POINT('',(7.23505692281089,4.17289950600423,-1.97584193198538));
#134338=CARTESIAN_POINT('',(7.08127227460583,4.17289950413623,-2.05708128634764));
#134339=CARTESIAN_POINT('',(7.36372645293057,4.08221031170477,-1.42321211529242));
#134340=CARTESIAN_POINT('Origin',(-0.188944138865323,4.01787924544133,0.0259938208454624));
#134341=CARTESIAN_POINT('Ctrl Pts',(7.11820906946345,4.04280735927478,-1.37608126440439));
#134342=CARTESIAN_POINT('Ctrl Pts',(7.15907737229309,4.04969801268933,-1.38388427975716));
#134343=CARTESIAN_POINT('Ctrl Pts',(7.19999317533954,4.05642175451896,-1.39171894787107));
#134344=CARTESIAN_POINT('Ctrl Pts',(7.2818188109592,4.06954550713737,-1.40742796310531));
#134345=CARTESIAN_POINT('Ctrl Pts',(7.32277466663668,4.07595289339688,-1.41531114890485));
#134346=CARTESIAN_POINT('Ctrl Pts',(7.36372645319145,4.08221031170464,-1.42321211394033));
#134347=CARTESIAN_POINT('Ctrl Pts',(7.450000887,4.172899507,-0.864573176000001));
#134348=CARTESIAN_POINT('Ctrl Pts',(7.402887342,4.107307013,-1.270549175));
#134349=CARTESIAN_POINT('Ctrl Pts',(7.31193774100001,4.04203077,-1.669001641));
#134350=CARTESIAN_POINT('Ctrl Pts',(7.225202548,4.172899507,-0.599122803));
#134351=CARTESIAN_POINT('Ctrl Pts',(7.1925543,4.107307013,-0.992848772000001));
#134352=CARTESIAN_POINT('Ctrl Pts',(7.11731548,4.04203077,-1.380695607));
#134353=CARTESIAN_POINT('',(7.45000088794504,4.17289950685238,-0.864573181094501));
#134354=CARTESIAN_POINT('Origin',(-0.191388568438923,4.16071400365763,0.0241744027929161));
#134355=CARTESIAN_POINT('',(7.33760171763272,4.17289950678353,-0.731847988169358));
#134356=CARTESIAN_POINT('Origin',(-1.65752828129584E-12,4.264192185,3.55780942901118E-13));
#134357=CARTESIAN_POINT('',(7.36282707779088,4.26310680606226,-1.42785763063805));
#134358=CARTESIAN_POINT('Origin',(-0.185146489275991,4.16071714815283,0.0525997026355554));
#134359=CARTESIAN_POINT('Origin',(-0.18513120911127,4.01799500061643,-0.00337946912520898));
#134360=CARTESIAN_POINT('Ctrl Pts',(7.486882896,4.042023177,0.443378502));
#134361=CARTESIAN_POINT('Ctrl Pts',(7.511089276,4.10772842,0.034629932));
#134362=CARTESIAN_POINT('Ctrl Pts',(7.49065292200001,4.172899507,-0.374324464));
#134363=CARTESIAN_POINT('Ctrl Pts',(7.247483165,4.042023177,0.191017723));
#134364=CARTESIAN_POINT('Ctrl Pts',(7.25791183400001,4.10772842,-0.204660748));
#134365=CARTESIAN_POINT('Ctrl Pts',(7.225202548,4.172899507,-0.599122803));
#134366=CARTESIAN_POINT('',(7.49065292297682,4.17289950600421,-0.374324474032694));
#134367=CARTESIAN_POINT('',(7.35792773384199,4.17289950413623,-0.486723651005898));
#134368=CARTESIAN_POINT('',(7.49751515522338,4.08221031172839,0.193045309743851));
#134369=CARTESIAN_POINT('Origin',(-0.190114426969782,4.01787920023827,-0.0152313257799268));
#134370=CARTESIAN_POINT('Ctrl Pts',(7.24760609256059,4.04280735932244,0.186295288436253));
#134371=CARTESIAN_POINT('Ctrl Pts',(7.28919633568094,4.04969801290351,0.187460180072133));
#134372=CARTESIAN_POINT('Ctrl Pts',(7.33083977311272,4.05642175490914,0.188604370186818));
#134373=CARTESIAN_POINT('Ctrl Pts',(7.41412934245488,4.06954550718391,0.190852715569519));
#134374=CARTESIAN_POINT('Ctrl Pts',(7.45582232480963,4.07595289343287,0.191958132496257));
#134375=CARTESIAN_POINT('Ctrl Pts',(7.49751515518722,4.08221031172826,0.193045311131656));
#134376=CARTESIAN_POINT('Ctrl Pts',(7.461681683,4.172899507,0.757170034));
#134377=CARTESIAN_POINT('Ctrl Pts',(7.502942465,4.107307013,0.350557509));
#134378=CARTESIAN_POINT('Ctrl Pts',(7.499774717,4.04203077,-0.058130836));
#134379=CARTESIAN_POINT('Ctrl Pts',(7.185075021,4.172899507,0.968089328));
#134380=CARTESIAN_POINT('Ctrl Pts',(7.237829515,4.107307013,0.576550044));
#134381=CARTESIAN_POINT('Ctrl Pts',(7.247725342,4.04203077,0.181596731));
#134382=CARTESIAN_POINT('',(7.46168168499956,4.17289950692262,0.757170029229101));
#134383=CARTESIAN_POINT('Origin',(-0.192110981246819,4.16071410180708,-0.0175336851590434));
#134384=CARTESIAN_POINT('',(7.32337835184357,4.17289950678352,0.862629682328062));
#134385=CARTESIAN_POINT('Origin',(-1.01394587170844E-12,4.264192185,-4.13352078260099E-14));
#134386=CARTESIAN_POINT('',(7.49763545621552,4.26310680660134,0.188315065718333));
#134387=CARTESIAN_POINT('Origin',(-0.192125296875894,4.16071714821591,0.0115689275453297));
#134388=CARTESIAN_POINT('Origin',(-0.18007633025845,4.01799492518908,-0.0430982007787728));
#134389=CARTESIAN_POINT('Ctrl Pts',(7.216530463,4.042023177,2.042471071));
#134390=CARTESIAN_POINT('Ctrl Pts',(7.328039771,4.10772842,1.648482471));
#134391=CARTESIAN_POINT('Ctrl Pts',(7.395994314,4.172899507,1.24469599));
#134392=CARTESIAN_POINT('Ctrl Pts',(7.036977872,4.042023177,1.744546481));
#134393=CARTESIAN_POINT('Ctrl Pts',(7.1322219,4.10772842,1.360360608));
#134394=CARTESIAN_POINT('Ctrl Pts',(7.185075021,4.172899507,0.968089328));
#134395=CARTESIAN_POINT('',(7.39599431711138,4.17289950600422,1.24469598041833));
#134396=CARTESIAN_POINT('',(7.29053467013232,4.17289950413623,1.10639264165444));
#134397=CARTESIAN_POINT('',(7.28072838184259,4.0822103116604,1.80027615080325));
#134398=CARTESIAN_POINT('Origin',(-0.18239528671673,4.01787920662655,-0.0557441918224923));
#134399=CARTESIAN_POINT('Ctrl Pts',(7.03811310959639,4.04280735930236,1.73996088057068));
#134400=CARTESIAN_POINT('Ctrl Pts',(7.07848058142537,4.04969801334083,1.75003921115477));
#134401=CARTESIAN_POINT('Ctrl Pts',(7.11890445475128,4.05642175586792,1.76010875955354));
#134402=CARTESIAN_POINT('Ctrl Pts',(7.19976342610926,4.06954550711907,1.78020933350753));
#134403=CARTESIAN_POINT('Ctrl Pts',(7.24024401768039,4.07595289336593,1.79025166508122));
#134404=CARTESIAN_POINT('Ctrl Pts',(7.28072838151672,4.08221031166027,1.80027615211935));
#134405=CARTESIAN_POINT('Ctrl Pts',(7.124462536,4.172899507,2.343508816));
#134406=CARTESIAN_POINT('Ctrl Pts',(7.252168337,4.107307013,1.955272514));
#134407=CARTESIAN_POINT('Ctrl Pts',(7.336930563,4.04203077,1.555458103));
#134408=CARTESIAN_POINT('Ctrl Pts',(6.80898137100001,4.172899507,2.490034677));
#134409=CARTESIAN_POINT('Ctrl Pts',(6.944671867,4.107307013,2.118990022));
#134410=CARTESIAN_POINT('Ctrl Pts',(7.039239622,4.04203077,1.735397808));
#134411=CARTESIAN_POINT('',(7.12446253898564,4.17289950685236,2.34350881178721));
#134412=CARTESIAN_POINT('Origin',(-0.18385034724122,4.16071403008887,-0.058421934317176));
#134413=CARTESIAN_POINT('',(6.96672195306173,4.17289950678352,2.41677174776338));
#134414=CARTESIAN_POINT('Origin',(9.11163505756818E-13,4.264192185,2.70183181383388E-13));
#134415=CARTESIAN_POINT('',(7.28186273324354,4.26310680661245,1.79568235838605));
#134416=CARTESIAN_POINT('Origin',(-0.190120374725622,4.16071715608105,-0.0300027826587959));
#134417=CARTESIAN_POINT('Origin',(-0.166601488256943,4.01799499817148,-0.0808016891777477));
#134418=CARTESIAN_POINT('Ctrl Pts',(6.608741086,4.042023177,3.546059963));
#134419=CARTESIAN_POINT('Ctrl Pts',(6.802339271,4.10772842,3.185253802));
#134420=CARTESIAN_POINT('Ctrl Pts',(6.95550723200001,4.172899507,2.805515843));
#134421=CARTESIAN_POINT('Ctrl Pts',(6.497431315,4.042023177,3.216502185));
#134422=CARTESIAN_POINT('Ctrl Pts',(6.673037196,4.10772842,2.861773014));
#134423=CARTESIAN_POINT('Ctrl Pts',(6.808981371,4.172899507,2.490034677));
#134424=CARTESIAN_POINT('',(6.95550723709794,4.17289950600422,2.80551583431232));
#134425=CARTESIAN_POINT('',(6.88224430779956,4.17289950413623,2.64777524362585));
#134426=CARTESIAN_POINT('',(6.72350284208098,4.08221031170637,3.32332808042156));
#134427=CARTESIAN_POINT('Origin',(-0.166147856588221,4.01787924998038,-0.0936506027297385));
#134428=CARTESIAN_POINT('Ctrl Pts',(6.49952577937696,4.04280735929061,3.21226783447011));
#134429=CARTESIAN_POINT('Ctrl Pts',(6.53678293033991,4.04969801171788,3.23078834846234));
#134430=CARTESIAN_POINT('Ctrl Pts',(6.57409705013473,4.05642175244788,3.24931240921773));
#134431=CARTESIAN_POINT('Ctrl Pts',(6.64874457416989,4.06954550713273,3.28632534165753));
#134432=CARTESIAN_POINT('Ctrl Pts',(6.68611994776028,4.07595289339519,3.30483501987673));
#134433=CARTESIAN_POINT('Ctrl Pts',(6.72350284147008,4.08221031170624,3.32332808165651));
#134434=CARTESIAN_POINT('Ctrl Pts',(6.45411144,4.172899507,3.82026773));
#134435=CARTESIAN_POINT('Ctrl Pts',(6.662290879,4.107307013,3.468561149));
#134436=CARTESIAN_POINT('Ctrl Pts',(6.83101969100001,4.04203077,3.09631555));
#134437=CARTESIAN_POINT('Ctrl Pts',(6.114507319,4.172899507,3.895548773));
#134438=CARTESIAN_POINT('Ctrl Pts',(6.32678908000001,4.107307013,3.562348381));
#134439=CARTESIAN_POINT('Ctrl Pts',(6.50160688,4.04203077,3.208053611));
#134440=CARTESIAN_POINT('',(6.45411144382979,4.17289950685223,3.82026772651186));
#134441=CARTESIAN_POINT('Origin',(-0.166993061533895,4.16071401829543,-0.0965784589115737));
#134442=CARTESIAN_POINT('',(6.28430937880036,4.17289950678351,3.85790825263968));
#134443=CARTESIAN_POINT('Origin',(2.77555756156289E-13,4.26419218499978,
1.33790548084711E-13));
#134444=CARTESIAN_POINT('',(6.72559820178816,4.26310680658169,3.31908553998013));
#134445=CARTESIAN_POINT('Origin',(-0.179225866214101,4.16071716216026,-0.0701716498773386));
#134446=CARTESIAN_POINT('Origin',(-0.145336718269771,4.01799492185903,-0.114727121590696));
#134447=CARTESIAN_POINT('Ctrl Pts',(5.691934321,4.042023177,4.883839032));
#134448=CARTESIAN_POINT('Ctrl Pts',(5.95856894700001,4.10772842,4.573086206));
#134449=CARTESIAN_POINT('Ctrl Pts',(6.189788363,4.172899507,4.235152893));
#134450=CARTESIAN_POINT('Ctrl Pts',(5.654072091,4.042023177,4.538057821));
#134451=CARTESIAN_POINT('Ctrl Pts',(5.90182869,4.10772842,4.229372095));
#134452=CARTESIAN_POINT('Ctrl Pts',(6.114507319,4.172899507,3.895548773));
#134453=CARTESIAN_POINT('',(6.18978836985319,4.17289950600421,4.23515288559372));
#134454=CARTESIAN_POINT('',(6.15214785067221,4.17289950413623,4.06535081836292));
#134455=CARTESIAN_POINT('',(5.85189378122471,4.08221031161528,4.69098488189386));
#134456=CARTESIAN_POINT('Origin',(-0.142131104059078,4.01787918315488,-0.127177865467208));
#134457=CARTESIAN_POINT('Ctrl Pts',(5.65702784793379,4.04280735922081,4.53437271583437));
#134458=CARTESIAN_POINT('Ctrl Pts',(5.6894325894266,4.04969801272765,4.56046942051071));
#134459=CARTESIAN_POINT('Ctrl Pts',(5.72189220651359,4.05642175465624,4.58658183659266));
#134460=CARTESIAN_POINT('Ctrl Pts',(5.78683781525976,4.06954550706718,4.63877642906093));
#134461=CARTESIAN_POINT('Ctrl Pts',(5.8193603396521,4.07595289331887,4.66488796167648));
#134462=CARTESIAN_POINT('Ctrl Pts',(5.8518937803898,4.08221031161516,4.69098488293473));
#134463=CARTESIAN_POINT('Ctrl Pts',(5.481973265,4.172899507,5.11839517));
#134464=CARTESIAN_POINT('Ctrl Pts',(5.760892103,4.107307013,4.81966372));
#134465=CARTESIAN_POINT('Ctrl Pts',(6.005697929,4.04203077,4.492392723));
#134466=CARTESIAN_POINT('Ctrl Pts',(5.134125702,4.172899507,5.118911337));
#134467=CARTESIAN_POINT('Ctrl Pts',(5.413072667,4.107307013,4.839135289));
#134468=CARTESIAN_POINT('Ctrl Pts',(5.659966227,4.04203077,4.530704394));
#134469=CARTESIAN_POINT('',(5.48197326948944,4.17289950685236,5.11839516742479));
#134470=CARTESIAN_POINT('Origin',(-0.14232717713363,4.16071403116877,-0.130218946123016));
#134471=CARTESIAN_POINT('',(5.30804948257176,4.17289950678352,5.11865325446259));
#134472=CARTESIAN_POINT('Origin',(-5.24753851482984E-14,4.26419218500022,
2.34187669256869E-14));
#134473=CARTESIAN_POINT('',(5.85485217362851,4.26310680661815,4.68729197077568));
#134474=CARTESIAN_POINT('Origin',(-0.159950766863188,4.16071718815307,-0.107059299983618));
#134475=CARTESIAN_POINT('Origin',(-0.117275699508936,4.01799490700237,-0.143287822644464));
#134476=CARTESIAN_POINT('Ctrl Pts',(4.508979033,4.042023177,5.993255216));
#134477=CARTESIAN_POINT('Ctrl Pts',(4.836182561,4.10772842,5.747086181));
#134478=CARTESIAN_POINT('Ctrl Pts',(5.134641869,4.172899507,5.466758901));
#134479=CARTESIAN_POINT('Ctrl Pts',(4.54633474,4.042023177,5.647418918));
#134480=CARTESIAN_POINT('Ctrl Pts',(4.854657234,4.10772842,5.399210438));
#134481=CARTESIAN_POINT('Ctrl Pts',(5.134125702,4.172899507,5.118911337));
#134482=CARTESIAN_POINT('',(5.13464187728293,4.17289950600421,5.46675889524292));
#134483=CARTESIAN_POINT('',(5.13438379809265,4.17289950413623,5.29283510678433));
#134484=CARTESIAN_POINT('',(4.70665667160418,4.0822103116914,5.83929644515874));
#134485=CARTESIAN_POINT('Origin',(-0.111469018216903,4.01787921396925,-0.154758873994295));
#134486=CARTESIAN_POINT('Ctrl Pts',(4.55001358209104,4.0428073593046,5.64445536825661));
#134487=CARTESIAN_POINT('Ctrl Pts',(4.57605069418501,4.049698011634,5.67690800270813));
#134488=CARTESIAN_POINT('Ctrl Pts',(4.60213802041595,4.05642175225397,5.70938777661076));
#134489=CARTESIAN_POINT('Ctrl Pts',(4.6543449520232,4.06954550710832,5.77432348696933));
#134490=CARTESIAN_POINT('Ctrl Pts',(4.68049391020144,4.07595289337418,5.80681592801612));
#134491=CARTESIAN_POINT('Ctrl Pts',(4.70665667053675,4.08221031169127,5.83929644601857));
#134492=CARTESIAN_POINT('Ctrl Pts',(4.253504114,4.172899507,6.177192142));
#134493=CARTESIAN_POINT('Ctrl Pts',(4.590120416,4.107307013,5.94540417200001));
#134494=CARTESIAN_POINT('Ctrl Pts',(4.899556408,4.04203077,5.678410606));
#134495=CARTESIAN_POINT('Ctrl Pts',(3.913678072,4.172899507,6.102919297));
#134496=CARTESIAN_POINT('Ctrl Pts',(4.246246993,4.107307013,5.889649609));
#134497=CARTESIAN_POINT('Ctrl Pts',(4.553671844,4.04203077,5.641504474));
#134498=CARTESIAN_POINT('',(4.25350411889082,4.17289950685237,6.1771921404623));
#134499=CARTESIAN_POINT('Origin',(-0.111006536517217,4.16071400427737,-0.157770777196192));
#134500=CARTESIAN_POINT('',(4.08359109188653,4.17289950678353,6.14005572024055));
#134501=CARTESIAN_POINT('Origin',(8.32667268468867E-14,4.26419218500044,
1.6002824065886E-13));
#134502=CARTESIAN_POINT('',(4.71033976528965,4.26310680660776,5.83632583827294));
#134503=CARTESIAN_POINT('Origin',(-0.133196765032976,4.16071716528115,-0.138941155871057));
#134504=CARTESIAN_POINT('Origin',(-0.0837313970627712,4.01799493508786,
-0.165148863663684));
#134505=CARTESIAN_POINT('Ctrl Pts',(3.115188897,4.042023177,6.822433447));
#134506=CARTESIAN_POINT('Ctrl Pts',(3.487661654,4.10772842,6.652358794));
#134507=CARTESIAN_POINT('Ctrl Pts',(3.839405228,4.172899507,6.442745339));
#134508=CARTESIAN_POINT('Ctrl Pts',(3.226015829,4.042023177,6.492712982));
#134509=CARTESIAN_POINT('Ctrl Pts',(3.580487401,4.10772842,6.316587701));
#134510=CARTESIAN_POINT('Ctrl Pts',(3.913678072,4.172899507,6.102919297));
#134511=CARTESIAN_POINT('',(3.8394052373347,4.17289950600421,6.44274533515021));
#134512=CARTESIAN_POINT('',(3.87654166492425,4.17289950413623,6.27283230877697));
#134513=CARTESIAN_POINT('',(3.34134152675702,4.08221031164381,6.71456899555679));
#134514=CARTESIAN_POINT('Origin',(-0.0755942808618143,4.01787919564236,
-0.175103132993055));
#134515=CARTESIAN_POINT('Ctrl Pts',(3.23024573729236,4.04280735935761,6.49060956175588));
#134516=CARTESIAN_POINT('Ctrl Pts',(3.24869776186493,4.04969801266095,6.52790068627852));
#134517=CARTESIAN_POINT('Ctrl Pts',(3.26719299297759,4.05642175437212,6.56522911152584));
#134518=CARTESIAN_POINT('Ctrl Pts',(3.30422009156699,4.0695455071151,6.63986959601397));
#134519=CARTESIAN_POINT('Ctrl Pts',(3.32277278728129,4.0759528933535,6.67722363469553));
#134520=CARTESIAN_POINT('Ctrl Pts',(3.34134152555005,4.08221031164368,6.71456899615694));
#134521=CARTESIAN_POINT('Ctrl Pts',(2.826145837,4.172899507,6.947150474));
#134522=CARTESIAN_POINT('Ctrl Pts',(3.204719799,4.107307013,6.793144133));
#134523=CARTESIAN_POINT('Ctrl Pts',(3.564317074,4.04203077,6.598912319));
#134524=CARTESIAN_POINT('Ctrl Pts',(2.510231206,4.172899507,6.801561533));
#134525=CARTESIAN_POINT('Ctrl Pts',(2.880871529,4.107307013,6.66477046000001));
#134526=CARTESIAN_POINT('Ctrl Pts',(3.234452827,4.04203077,6.488514076));
#134527=CARTESIAN_POINT('',(2.82614584213299,4.17289950685239,6.9471504735488));
#134528=CARTESIAN_POINT('Origin',(-0.0744951406898375,4.16071401400292,
-0.177945158959567));
#134529=CARTESIAN_POINT('',(2.66818852025341,4.17289950678353,6.87435600398385));
#134530=CARTESIAN_POINT('Origin',(1.83880688453542E-13,4.26419218500044,
1.34007388519208E-13));
#134531=CARTESIAN_POINT('',(3.34557710444455,4.26310680660674,6.71245959639363));
#134532=CARTESIAN_POINT('Origin',(-0.100214494169487,4.16071715590041,-0.164326227237381));
#134533=CARTESIAN_POINT('Origin',(-0.0462715741382319,4.01799497278107,
-0.179287317113798));
#134534=CARTESIAN_POINT('Ctrl Pts',(1.57573599,4.042023177,7.332602273));
#134535=CARTESIAN_POINT('Ctrl Pts',(1.976061564,4.10772842,7.24657450400001));
#134536=CARTESIAN_POINT('Ctrl Pts',(2.364642265,4.172899507,7.117476165));
#134537=CARTESIAN_POINT('Ctrl Pts',(1.754852004,4.042023177,7.034415004));
#134538=CARTESIAN_POINT('Ctrl Pts',(2.138897957,4.10772842,6.938608343));
#134539=CARTESIAN_POINT('Ctrl Pts',(2.510231206,4.172899507,6.801561533));
#134540=CARTESIAN_POINT('',(2.36464227492406,4.17289950600422,7.11747616326049));
#134541=CARTESIAN_POINT('',(2.43743675205796,4.17289950413623,6.95951884320089));
#134542=CARTESIAN_POINT('',(1.8197889658224,4.08221031167589,7.27587576289585));
#134543=CARTESIAN_POINT('Origin',(-0.0361848468469295,4.0178791970496,-0.187259532776093));
#134544=CARTESIAN_POINT('Ctrl Pts',(1.75943519295772,4.04280735931344,7.03327006476682));
#134545=CARTESIAN_POINT('Ctrl Pts',(1.76943932797021,4.04969801137569,7.0736559761413));
#134546=CARTESIAN_POINT('Ctrl Pts',(1.77947764045624,4.0564217516996,7.11408760265159));
#134547=CARTESIAN_POINT('Ctrl Pts',(1.79959357205713,4.06954550710117,7.19494278222298));
#134548=CARTESIAN_POINT('Ctrl Pts',(1.80968250185344,4.07595289336307,7.23541178557499));
#134549=CARTESIAN_POINT('Ctrl Pts',(1.81978896449978,4.08221031167577,7.27587576322622));
#134550=CARTESIAN_POINT('Ctrl Pts',(1.266640122,4.172899507,7.392267771));
#134551=CARTESIAN_POINT('Ctrl Pts',(1.669470046,4.107307013,7.323244224));
#134552=CARTESIAN_POINT('Ctrl Pts',(2.062414236,4.04203077,7.210856227));
#134553=CARTESIAN_POINT('Ctrl Pts',(0.989408718000001,4.172899507,7.18217031200001));
#134554=CARTESIAN_POINT('Ctrl Pts',(1.380789714,4.107307013,7.128254051));
#134555=CARTESIAN_POINT('Ctrl Pts',(1.76399439,4.04203077,7.03212797));
#134556=CARTESIAN_POINT('',(1.26664012712354,4.1728995068524,7.39226777166522));
#134557=CARTESIAN_POINT('Origin',(-0.0345005551398,4.16071403657584,-0.189799287105015));
#134558=CARTESIAN_POINT('',(1.12802441867854,4.17289950678353,7.28721904170456));
#134559=CARTESIAN_POINT('Origin',(1.58293517182884E-14,4.26419218500133,
-3.62557206479153E-13));
#134560=CARTESIAN_POINT('',(1.8243789766821,4.26310680660485,7.27472620408612));
#134561=CARTESIAN_POINT('Origin',(-0.0625461994119189,4.16071710752316,
-0.182027287696495));
#134562=CARTESIAN_POINT('Origin',(-0.00664832895622192,4.0179949497113,
-0.185042884422192));
#134563=CARTESIAN_POINT('Ctrl Pts',(-0.03739658,4.042023177,7.499906766));
#134564=CARTESIAN_POINT('Ctrl Pts',(0.372063032,4.10772842,7.50194844300001));
#134565=CARTESIAN_POINT('Ctrl Pts',(0.779311259,4.172899507,7.459401716));
#134566=CARTESIAN_POINT('Ctrl Pts',(0.201633249,4.042023177,7.247195598));
#134567=CARTESIAN_POINT('Ctrl Pts',(0.597296021,4.10772842,7.236187371));
#134568=CARTESIAN_POINT('Ctrl Pts',(0.989408718,4.172899507,7.18217031200001));
#134569=CARTESIAN_POINT('',(0.779311269060809,4.17289950600422,7.4594017164365));
#134570=CARTESIAN_POINT('',(0.884360005917485,4.17289950413623,7.32078601189595));
#134571=CARTESIAN_POINT('',(0.21314509586863,4.08221031164964,7.49697066538411));
#134572=CARTESIAN_POINT('Origin',(0.00491640757449785,4.01787918214174,
-0.190660168586786));
#134573=CARTESIAN_POINT('Ctrl Pts',(0.206355413397366,4.04280735932038,
7.24706267725279));
#134574=CARTESIAN_POINT('Ctrl Pts',(0.207443880494177,4.04969801231471,
7.28865498727906));
#134575=CARTESIAN_POINT('Ctrl Pts',(0.208555898644855,4.05642175367949,
7.33029929207554));
#134576=CARTESIAN_POINT('Ctrl Pts',(0.210820057400983,4.06954550711118,
7.41358844048726));
#134577=CARTESIAN_POINT('Ctrl Pts',(0.211973474311316,4.07595289335646,
7.45528012253599));
#134578=CARTESIAN_POINT('Ctrl Pts',(0.213145094518449,4.08221031164952,
7.49697066542207));
#134579=CARTESIAN_POINT('Ctrl Pts',(-0.352092277,4.172899507,7.49173084300001));
#134580=CARTESIAN_POINT('Ctrl Pts',(0.0561577300000001,4.107307013,7.510917554));
#134581=CARTESIAN_POINT('Ctrl Pts',(0.4640752,4.04203077,7.485628511));
#134582=CARTESIAN_POINT('Ctrl Pts',(-0.577677421000001,4.172899507,7.226948789));
#134583=CARTESIAN_POINT('Ctrl Pts',(-0.183856294,4.107307013,7.258428405));
#134584=CARTESIAN_POINT('Ctrl Pts',(0.211053536,4.04203077,7.246927377));
#134585=CARTESIAN_POINT('',(-0.352092272134449,4.17289950685238,7.49173084475307));
#134586=CARTESIAN_POINT('Origin',(0.00710727529755324,4.160714013686,-0.192778466708976));
#134587=CARTESIAN_POINT('',(-0.464884850334537,4.17289950678353,7.3593398159157));
#134588=CARTESIAN_POINT('Origin',(-3.27700106633744E-14,4.26419218499956,
2.03830008427275E-13));
#134589=CARTESIAN_POINT('',(0.217874915136567,4.26310680605619,7.49683469969476));
#134590=CARTESIAN_POINT('Origin',(-0.0219534128396459,4.16071715851607,
-0.191217207783373));
#134591=CARTESIAN_POINT('Origin',(0.0332858491263909,4.01799497996062,-0.182145603627001));
#134592=CARTESIAN_POINT('Ctrl Pts',(0.458515569029856,1.71660033198358,
7.48597550365515));
#134593=CARTESIAN_POINT('Ctrl Pts',(0.462562578514928,1.71596185949179,
7.48572323182757));
#134594=CARTESIAN_POINT('Ctrl Pts',(0.466609588,1.715323387,7.48547096));
#134595=CARTESIAN_POINT('Ctrl Pts',(0.873461406,1.651136808,7.46010970200001));
#134596=CARTESIAN_POINT('Ctrl Pts',(1.275167733,1.585954698,7.39080153));
#134597=CARTESIAN_POINT('Ctrl Pts',(0.205671117258217,1.71660033198358,
7.24708636966053));
#134598=CARTESIAN_POINT('Ctrl Pts',(0.209589119629109,1.71596185949179,
7.24697093733027));
#134599=CARTESIAN_POINT('Ctrl Pts',(0.213507122,1.715323387,7.246855505));
#134600=CARTESIAN_POINT('Ctrl Pts',(0.607389665,1.651136808,7.235250923));
#134601=CARTESIAN_POINT('Ctrl Pts',(0.997694124000001,1.585954698,7.18102405200001));
#134602=CARTESIAN_POINT('',(0.993027300490256,1.58673401522208,7.18167089043044));
#134603=CARTESIAN_POINT('Origin',(-0.043636971062415,1.48222902514883,-0.188849083665119));
#134604=CARTESIAN_POINT('Ctrl Pts',(1.02948254309185,1.62564958676913,7.42900839219714));
#134605=CARTESIAN_POINT('Ctrl Pts',(1.02534588378697,1.62139779886715,7.40060352041928));
#134606=CARTESIAN_POINT('Ctrl Pts',(1.02118591211148,1.61707840871591,7.37221205908516));
#134607=CARTESIAN_POINT('Ctrl Pts',(1.01700107867271,1.61268792538597,7.34383535412214));
#134608=CARTESIAN_POINT('Ctrl Pts',(1.01301187494507,1.60850268534662,7.3167851838172));
#134609=CARTESIAN_POINT('Ctrl Pts',(1.00899401265604,1.60425381504717,7.28974898488846));
#134610=CARTESIAN_POINT('Ctrl Pts',(1.00499516686957,1.59993003804733,7.26272204028933));
#134611=CARTESIAN_POINT('Ctrl Pts',(1.00099621028148,1.59560614124254,7.2356943468168));
#134612=CARTESIAN_POINT('Ctrl Pts',(0.99700672008524,1.59120881937225,7.208676889702));
#134613=CARTESIAN_POINT('Ctrl Pts',(0.993027296840828,1.5867340161625,7.18167089110788));
#134614=CARTESIAN_POINT('Ctrl Pts',(0.778213576,1.585967065,7.45951631300001));
#134615=CARTESIAN_POINT('Ctrl Pts',(0.845381055,1.59657582,7.45250907));
#134616=CARTESIAN_POINT('Ctrl Pts',(0.912411464,1.607142857,7.444293474));
#134617=CARTESIAN_POINT('Ctrl Pts',(1.252691653,1.660786473,7.402586957));
#134618=CARTESIAN_POINT('Ctrl Pts',(1.587747952,1.715323387,7.330010671));
#134619=CARTESIAN_POINT('Ctrl Pts',(1.59177351427215,1.71597862537066,7.32913869706712));
#134620=CARTESIAN_POINT('Ctrl Pts',(1.59579907654429,1.71663386374133,7.32826672313425));
#134621=CARTESIAN_POINT('Ctrl Pts',(0.988351829,1.585967065,7.182315829));
#134622=CARTESIAN_POINT('Ctrl Pts',(1.053023321,1.59657582,7.173416445));
#134623=CARTESIAN_POINT('Ctrl Pts',(1.117524075,1.607142857,7.163353959));
#134624=CARTESIAN_POINT('Ctrl Pts',(1.444962461,1.660786473,7.112271703));
#134625=CARTESIAN_POINT('Ctrl Pts',(1.766375162,1.715323387,7.03153033));
#134626=CARTESIAN_POINT('Ctrl Pts',(1.77023680210883,1.71597862537066,7.03056025593805));
#134627=CARTESIAN_POINT('Ctrl Pts',(1.77409844221766,1.71663386374133,7.02959018187611));
#134628=CARTESIAN_POINT('Ctrl Pts',(1.7663751461876,1.71532338431697,7.0315303339722));
#134629=CARTESIAN_POINT('Ctrl Pts',(1.62199423020245,1.69082500709975,7.0677999438676));
#134630=CARTESIAN_POINT('Ctrl Pts',(1.47679252529511,1.66647815902139,7.09954383997699));
#134631=CARTESIAN_POINT('Ctrl Pts',(1.33119287040896,1.64234940160257,7.12674017636573));
#134632=CARTESIAN_POINT('Ctrl Pts',(1.26004864791652,1.63055938954785,7.14002909664876));
#134633=CARTESIAN_POINT('Ctrl Pts',(1.18880939776744,1.61882139759851,7.15223304210549));
#134634=CARTESIAN_POINT('Ctrl Pts',(1.1175240745291,1.60714285692684,7.16335395910296));
#134635=CARTESIAN_POINT('Ctrl Pts',(1.07611863033894,1.60035948101443,7.16981344483863));
#134636=CARTESIAN_POINT('Ctrl Pts',(1.03461671586149,1.59355605143323,7.17592022024356));
#134637=CARTESIAN_POINT('Ctrl Pts',(0.993027300662214,1.58673401459539,
7.18167089093061));
#134638=CARTESIAN_POINT('Ctrl Pts',(2.05705917966293,1.71660033198358,7.21239026252005));
#134639=CARTESIAN_POINT('Ctrl Pts',(2.06095734133147,1.71596185949179,7.21127390126003));
#134640=CARTESIAN_POINT('Ctrl Pts',(2.064855503,1.715323387,7.21015754));
#134641=CARTESIAN_POINT('Ctrl Pts',(2.456743431,1.651136808,7.0979281));
#134642=CARTESIAN_POINT('Ctrl Pts',(2.834158878,1.585954698,6.94388532800001));
#134643=CARTESIAN_POINT('Ctrl Pts',(1.75877198777081,1.71660033198358,7.03344030656226));
#134644=CARTESIAN_POINT('Ctrl Pts',(1.7625735748854,1.71596185949179,7.03248531828113));
#134645=CARTESIAN_POINT('Ctrl Pts',(1.766375162,1.715323387,7.03153033));
#134646=CARTESIAN_POINT('Ctrl Pts',(2.148554308,1.651136808,6.93552395300001));
#134647=CARTESIAN_POINT('Ctrl Pts',(2.518076491,1.585954698,6.798660955));
#134648=CARTESIAN_POINT('',(2.51365782700824,1.5867340152172,6.80029590006137));
#134649=CARTESIAN_POINT('Origin',(-0.0832136971996106,1.48222899362148,
-0.175053107338738));
#134650=CARTESIAN_POINT('Ctrl Pts',(2.60243101783764,1.62564958677363,7.03401398873212));
#134651=CARTESIAN_POINT('Ctrl Pts',(2.59228486354879,1.62139779887973,7.00716246659475));
#134652=CARTESIAN_POINT('Ctrl Pts',(2.58211882471485,1.6170784087356,6.98032905281386));
#134653=CARTESIAN_POINT('Ctrl Pts',(2.57193167755893,1.61268792541243,6.95351539495929));
#134654=CARTESIAN_POINT('Ctrl Pts',(2.56222075215246,1.60850268538428,6.92795520354208));
#134655=CARTESIAN_POINT('Ctrl Pts',(2.55248484170892,1.60425381508471,6.90241481758498));
#134656=CARTESIAN_POINT('Ctrl Pts',(2.54276949248601,1.59993003809904,6.87687938164382));
#134657=CARTESIAN_POINT('Ctrl Pts',(2.53305387406628,1.59560614130841,6.85134323815648));
#134658=CARTESIAN_POINT('Ctrl Pts',(2.52334970118557,1.59120881945939,6.82581505672652));
#134659=CARTESIAN_POINT('Ctrl Pts',(2.51365782285346,1.58673401618092,6.80029590129333));
#134660=CARTESIAN_POINT('Ctrl Pts',(2.363594881,1.585967065,7.117824052));
#134661=CARTESIAN_POINT('Ctrl Pts',(2.427685672,1.59657582,7.096541612));
#134662=CARTESIAN_POINT('Ctrl Pts',(2.491382836,1.607142857,7.074108535));
#134663=CARTESIAN_POINT('Ctrl Pts',(2.814741796,1.660786473,6.96022691200001));
#134664=CARTESIAN_POINT('Ctrl Pts',(3.126362908,1.715323387,6.817320219));
#134665=CARTESIAN_POINT('Ctrl Pts',(3.13010690623377,1.71597862537066,6.81560325443765));
#134666=CARTESIAN_POINT('Ctrl Pts',(3.13385090446755,1.71663386374133,6.81388628987529));
#134667=CARTESIAN_POINT('Ctrl Pts',(2.509230308,1.585967065,6.801930848));
#134668=CARTESIAN_POINT('Ctrl Pts',(2.570476711,1.59657582,6.779337068));
#134669=CARTESIAN_POINT('Ctrl Pts',(2.631306337,1.607142857,6.755644082));
#134670=CARTESIAN_POINT('Ctrl Pts',(2.940108221,1.660786473,6.635366527));
#134671=CARTESIAN_POINT('Ctrl Pts',(3.236649463,1.715323387,6.487418613));
#134672=CARTESIAN_POINT('Ctrl Pts',(3.24021228285891,1.71597862537066,6.48564108026112));
#134673=CARTESIAN_POINT('Ctrl Pts',(3.24377510271782,1.71663386374133,6.48386354752224));
#134674=CARTESIAN_POINT('Ctrl Pts',(3.23664944837323,1.71532338430999,6.48741862029747));
#134675=CARTESIAN_POINT('Ctrl Pts',(3.10344096466667,1.69082500573501,6.55387789944305));
#134676=CARTESIAN_POINT('Ctrl Pts',(2.96845798684327,1.66647815635029,6.61609371823778));
#134677=CARTESIAN_POINT('Ctrl Pts',(2.83210877192866,1.64234939768718,6.67395384374131));
#134678=CARTESIAN_POINT('Ctrl Pts',(2.7654845940745,1.6305593869447,6.70222597786856));
#134679=CARTESIAN_POINT('Ctrl Pts',(2.6985343728361,1.61882139630545,6.72945893164121));
#134680=CARTESIAN_POINT('Ctrl Pts',(2.63130633664155,1.60714285693915,6.75564408215498));
#134681=CARTESIAN_POINT('Ctrl Pts',(2.59225752655057,1.60035948100455,6.7708534952413));
#134682=CARTESIAN_POINT('Ctrl Pts',(2.55303868056522,1.5935560515235,6.78573918205019));
#134683=CARTESIAN_POINT('Ctrl Pts',(2.51365782710389,1.58673401460554,6.80029590003346));
#134684=CARTESIAN_POINT('Ctrl Pts',(3.55941698871103,1.71660033198358,6.6015616687789));
#134685=CARTESIAN_POINT('Ctrl Pts',(3.56298402885552,1.71596185949179,6.59963341788945));
#134686=CARTESIAN_POINT('Ctrl Pts',(3.566551069,1.715323387,6.59770516700001));
#134687=CARTESIAN_POINT('Ctrl Pts',(3.925150863,1.651136808,6.403855268));
#134688=CARTESIAN_POINT('Ctrl Pts',(4.260627904,1.585954698,6.172280767));
#134689=CARTESIAN_POINT('Ctrl Pts',(3.22963463525794,1.71660033198358,6.49091839309238));
#134690=CARTESIAN_POINT('Ctrl Pts',(3.23314204912897,1.71596185949179,6.48916850304618));
#134691=CARTESIAN_POINT('Ctrl Pts',(3.236649463,1.715323387,6.487418613));
#134692=CARTESIAN_POINT('Ctrl Pts',(3.58925494,1.651136808,6.311499592));
#134693=CARTESIAN_POINT('Ctrl Pts',(3.9207164,1.585954698,6.098400028));
#134694=CARTESIAN_POINT('',(3.91675250661477,1.58673401523444,6.10094663162891));
#134695=CARTESIAN_POINT('Origin',(-0.118899482557115,1.48222899061809,-0.153072010682567));
#134696=CARTESIAN_POINT('Ctrl Pts',(4.05369271047275,1.62564958678609,6.31011690926927));
#134697=CARTESIAN_POINT('Ctrl Pts',(4.03801148411028,1.62139779885104,6.28607428389982));
#134698=CARTESIAN_POINT('Ctrl Pts',(4.02231473077999,1.61707840870115,6.26205361824685));
#134699=CARTESIAN_POINT('Ctrl Pts',(4.00660160957958,1.61268792537235,6.23805678428026));
#134700=CARTESIAN_POINT('Ctrl Pts',(3.99162303459156,1.6085026853468,6.21518173784873));
#134701=CARTESIAN_POINT('Ctrl Pts',(3.97662431624528,1.60425381506014,6.1923314048936));
#134702=CARTESIAN_POINT('Ctrl Pts',(3.96164674257624,1.59993003808297,6.16948148613296));
#134703=CARTESIAN_POINT('Ctrl Pts',(3.94666875390263,1.59560614130087,6.14663093423766));
#134704=CARTESIAN_POINT('Ctrl Pts',(3.93170365482691,1.59120881945928,6.12378569777082));
#134705=CARTESIAN_POINT('Ctrl Pts',(3.91675250287728,1.58673401620365,6.10094663327425));
#134706=CARTESIAN_POINT('Ctrl Pts',(3.838457116,1.585967065,6.44331024900001));
#134707=CARTESIAN_POINT('Ctrl Pts',(3.896474404,1.59657582,6.408747755));
#134708=CARTESIAN_POINT('Ctrl Pts',(3.953859916,1.607142857,6.373146144));
#134709=CARTESIAN_POINT('Ctrl Pts',(4.24517774,1.660786473,6.192414392));
#134710=CARTESIAN_POINT('Ctrl Pts',(4.518792609,1.715323387,5.98585945));
#134711=CARTESIAN_POINT('Ctrl Pts',(4.52207997800942,1.71597862537066,5.9833777781612));
#134712=CARTESIAN_POINT('Ctrl Pts',(4.52536734701884,1.71663386374133,5.9808961063224));
#134713=CARTESIAN_POINT('Ctrl Pts',(3.912779966,1.585967065,6.103495141));
#134714=CARTESIAN_POINT('Ctrl Pts',(3.967737468,1.59657582,6.068263424));
#134715=CARTESIAN_POINT('Ctrl Pts',(4.022051639,1.607142857,6.032047796));
#134716=CARTESIAN_POINT('Ctrl Pts',(4.297777787,1.660786473,5.848198986));
#134717=CARTESIAN_POINT('Ctrl Pts',(4.555581632,1.715323387,5.639962411));
#134718=CARTESIAN_POINT('Ctrl Pts',(4.55867903812293,1.71597862537066,5.63746053503914));
#134719=CARTESIAN_POINT('Ctrl Pts',(4.56177644424584,1.71663386374133,5.63495865907829));
#134720=CARTESIAN_POINT('Ctrl Pts',(4.55558161941369,1.71532338433744,5.63996242116637));
#134721=CARTESIAN_POINT('Ctrl Pts',(4.43977427164447,1.69082500902195,5.73350379309277));
#134722=CARTESIAN_POINT('Ctrl Pts',(4.32132169862116,1.66647816281935,5.8232823794762));
#134723=CARTESIAN_POINT('Ctrl Pts',(4.20059848569967,1.64234940725285,5.90910080807064));
#134724=CARTESIAN_POINT('Ctrl Pts',(4.14160960169909,1.63055939331314,5.95103419608245));
#134725=CARTESIAN_POINT('Ctrl Pts',(4.08207890368759,1.61882139949784,5.99202278842587));
#134726=CARTESIAN_POINT('Ctrl Pts',(4.02205163891606,1.60714285698474,6.03204779607983));
#134727=CARTESIAN_POINT('Ctrl Pts',(3.98718534275932,1.6003594810294,6.05529596109391));
#134728=CARTESIAN_POINT('Ctrl Pts',(3.95208339400105,1.59355605150957,6.07826452157217));
#134729=CARTESIAN_POINT('Ctrl Pts',(3.91675250664303,1.58673401458826,6.10094663147859));
#134730=CARTESIAN_POINT('Ctrl Pts',(4.89534041542821,1.71660033198358,5.68205138827747));
#134731=CARTESIAN_POINT('Ctrl Pts',(4.8984095432141,1.71596185949179,5.67940141063874));
#134732=CARTESIAN_POINT('Ctrl Pts',(4.901478671,1.715323387,5.676751433));
#134733=CARTESIAN_POINT('Ctrl Pts',(5.210022603,1.651136808,5.410345282));
#134734=CARTESIAN_POINT('Ctrl Pts',(5.487874705,1.585954698,5.11206721600001));
#134735=CARTESIAN_POINT('Ctrl Pts',(4.54948315630955,1.71660033198358,5.64488834877326));
#134736=CARTESIAN_POINT('Ctrl Pts',(4.55253239415478,1.71596185949179,5.64242537988663));
#134737=CARTESIAN_POINT('Ctrl Pts',(4.555581632,1.715323387,5.639962411));
#134738=CARTESIAN_POINT('Ctrl Pts',(4.862125999,1.651136808,5.392356525));
#134739=CARTESIAN_POINT('Ctrl Pts',(5.140027969,1.585954698,5.112984694));
#134740=CARTESIAN_POINT('',(5.13670419287797,1.58673401524605,5.11632387916256));
#134741=CARTESIAN_POINT('Origin',(-0.149025739088519,1.48222905383165,-0.123933542996065));
#134742=CARTESIAN_POINT('Ctrl Pts',(5.3154082371546,1.62564958678922,5.29116577595053));
#134743=CARTESIAN_POINT('Ctrl Pts',(5.29492517538635,1.6213977988818,5.27105625408232));
#134744=CARTESIAN_POINT('Ctrl Pts',(5.27443167040395,1.61707840872797,5.25097151622125));
#134745=CARTESIAN_POINT('Ctrl Pts',(5.25392730332914,1.61268792539793,5.2309135715011));
#134746=CARTESIAN_POINT('Ctrl Pts',(5.23438146031953,1.60850268536628,5.21179328180062));
#134747=CARTESIAN_POINT('Ctrl Pts',(5.21482125764764,1.6042538150562,5.19270145794555));
#134748=CARTESIAN_POINT('Ctrl Pts',(5.19528179427944,1.59993003806774,5.17360549318183));
#134749=CARTESIAN_POINT('Ctrl Pts',(5.1757417895041,1.59560614127438,5.15450899929958));
#134750=CARTESIAN_POINT('Ctrl Pts',(5.15621551555659,1.59120881943709,5.13541492577162));
#134751=CARTESIAN_POINT('Ctrl Pts',(5.13670419026838,1.58673401624022,5.11632388192909));
#134752=CARTESIAN_POINT('Ctrl Pts',(5.13383736200001,1.585967065,5.46751442));
#134753=CARTESIAN_POINT('Ctrl Pts',(5.18306832399999,1.59657582,5.421287976));
#134754=CARTESIAN_POINT('Ctrl Pts',(5.2314589,1.607142857,5.374182522));
#134755=CARTESIAN_POINT('Ctrl Pts',(5.477113891,1.660786473,5.135051457));
#134756=CARTESIAN_POINT('Ctrl Pts',(5.69992859,1.715323387,4.874506546));
#134757=CARTESIAN_POINT('Ctrl Pts',(5.70260561606592,1.71597862537066,4.87137620710755));
#134758=CARTESIAN_POINT('Ctrl Pts',(5.70528264213185,1.71663386374133,4.86824586821509));
#134759=CARTESIAN_POINT('Ctrl Pts',(5.133372382,1.585967065,5.119666785));
#134760=CARTESIAN_POINT('Ctrl Pts',(5.179471231,1.59657582,5.073444527));
#134761=CARTESIAN_POINT('Ctrl Pts',(5.224730277,1.607142857,5.026399659));
#134762=CARTESIAN_POINT('Ctrl Pts',(5.454488042,1.660786473,4.787576161));
#134763=CARTESIAN_POINT('Ctrl Pts',(5.661499867,1.715323387,4.528787835));
#134764=CARTESIAN_POINT('Ctrl Pts',(5.66398702809828,1.71597862537066,4.52567860074675));
#134765=CARTESIAN_POINT('Ctrl Pts',(5.66647418919657,1.71663386374133,4.5225693664935));
#134766=CARTESIAN_POINT('Ctrl Pts',(5.6614998570788,1.71532338438628,4.52878784740263));
#134767=CARTESIAN_POINT('Ctrl Pts',(5.56850864601704,1.69082500771115,4.64503743717996));
#134768=CARTESIAN_POINT('Ctrl Pts',(5.47212516562663,1.66647816026213,4.75818085749009));
#134769=CARTESIAN_POINT('Ctrl Pts',(5.37267281462158,1.64234940357072,4.86794482593811));
#134770=CARTESIAN_POINT('Ctrl Pts',(5.32407750161806,1.63055939084648,4.92157869531712));
#134771=CARTESIAN_POINT('Ctrl Pts',(5.27474993895569,1.61882139826002,4.97440633186802));
#134772=CARTESIAN_POINT('Ctrl Pts',(5.22473027694185,1.60714285698642,5.02639965906045));
#134773=CARTESIAN_POINT('Ctrl Pts',(5.19567680415667,1.60035948108635,5.05659951771608));
#134774=CARTESIAN_POINT('Ctrl Pts',(5.16633308073874,1.5935560515154,5.08657696779505));
#134775=CARTESIAN_POINT('Ctrl Pts',(5.13670419294588,1.58673401465026,5.11632387909356));
#134776=CARTESIAN_POINT('Ctrl Pts',(6.00236316514702,1.71660033198358,4.49685470076832));
#134777=CARTESIAN_POINT('Ctrl Pts',(6.00479087157351,1.71596185949179,4.49360690638416));
#134778=CARTESIAN_POINT('Ctrl Pts',(6.007218578,1.715323387,4.490359112));
#134779=CARTESIAN_POINT('Ctrl Pts',(6.251279477,1.651136808,4.163853564));
#134780=CARTESIAN_POINT('Ctrl Pts',(6.458514584,1.585954698,3.812819084));
#134781=CARTESIAN_POINT('Ctrl Pts',(5.65660290128854,1.71660033198358,4.53490959909924));
#134782=CARTESIAN_POINT('Ctrl Pts',(5.65905138414427,1.71596185949179,4.53184871704962));
#134783=CARTESIAN_POINT('Ctrl Pts',(5.661499867,1.715323387,4.528787835));
#134784=CARTESIAN_POINT('Ctrl Pts',(5.907649451,1.651136808,4.221072859));
#134785=CARTESIAN_POINT('Ctrl Pts',(6.118997541,1.585954698,3.888491878));
#134786=CARTESIAN_POINT('',(6.11646929978026,1.58673401524938,3.89246750857916));
#134787=CARTESIAN_POINT('Origin',(-0.172183501602985,1.48222899636219,-0.0889997952577576));
#134788=CARTESIAN_POINT('Ctrl Pts',(6.32858118267442,1.62564958672614,4.02480561173429));
#134789=CARTESIAN_POINT('Ctrl Pts',(6.30425405066538,1.62139779884577,4.00956949215637));
#134790=CARTESIAN_POINT('Ctrl Pts',(6.27992204751377,1.61707840870175,3.9943598220441));
#134791=CARTESIAN_POINT('Ctrl Pts',(6.25558519594434,1.61268792537898,3.97917865369961));
#134792=CARTESIAN_POINT('Ctrl Pts',(6.23238602679848,1.60850268535536,3.96470716418705));
#134793=CARTESIAN_POINT('Ctrl Pts',(6.20917895297853,1.60425381506262,3.95026656197384));
#134794=CARTESIAN_POINT('Ctrl Pts',(6.18599124343742,1.59993003808074,3.93581745729565));
#134795=CARTESIAN_POINT('Ctrl Pts',(6.16280289140197,1.59560614129391,3.92136795225588));
#134796=CARTESIAN_POINT('Ctrl Pts',(6.13962846950894,1.59120881944976,3.90691785921443));
#134797=CARTESIAN_POINT('Ctrl Pts',(6.11646929696361,1.58673401627534,3.89246751191927));
#134798=CARTESIAN_POINT('Ctrl Pts',(6.18916508,1.585967065,4.236063694));
#134799=CARTESIAN_POINT('Ctrl Pts',(6.22730773,1.59657582,4.180334797));
#134800=CARTESIAN_POINT('Ctrl Pts',(6.264440681,1.607142857,4.123928098));
#134801=CARTESIAN_POINT('Ctrl Pts',(6.45294628400001,1.660786473,3.837579223));
#134802=CARTESIAN_POINT('Ctrl Pts',(6.614542245,1.715323387,3.535227133));
#134803=CARTESIAN_POINT('Ctrl Pts',(6.61648375335508,1.71597862537066,3.53159449821581));
#134804=CARTESIAN_POINT('Ctrl Pts',(6.61842526171017,1.71663386374133,3.52796186343163));
#134805=CARTESIAN_POINT('Ctrl Pts',(6.113934011,1.585967065,3.896448499));
#134806=CARTESIAN_POINT('Ctrl Pts',(6.149018675,1.59657582,3.841397003));
#134807=CARTESIAN_POINT('Ctrl Pts',(6.183106334,1.607142857,3.785722661));
#134808=CARTESIAN_POINT('Ctrl Pts',(6.35615249700001,1.660786473,3.503091595));
#134809=CARTESIAN_POINT('Ctrl Pts',(6.502692661,1.715323387,3.205852173));
#134810=CARTESIAN_POINT('Ctrl Pts',(6.50445328020731,1.71597862537066,3.20228096479836));
#134811=CARTESIAN_POINT('Ctrl Pts',(6.50621389941464,1.71663386374133,3.19870975659673));
#134812=CARTESIAN_POINT('Ctrl Pts',(6.50269265359969,1.71532338424588,3.20585218801065));
#134813=CARTESIAN_POINT('Ctrl Pts',(6.43686575043932,1.69082500755083,3.33937428870625));
#134814=CARTESIAN_POINT('Ctrl Pts',(6.36705815283194,1.66647816004792,3.47059207839789));
#134815=CARTESIAN_POINT('Ctrl Pts',(6.29352695091531,1.64234940326824,3.59916914265701));
#134816=CARTESIAN_POINT('Ctrl Pts',(6.2575974662105,1.63055939066046,3.66199563730517));
#134817=CARTESIAN_POINT('Ctrl Pts',(6.22077953525197,1.61882139818087,3.72419216051023));
#134818=CARTESIAN_POINT('Ctrl Pts',(6.18310633402413,1.60714285700432,3.78572266101966));
#134819=CARTESIAN_POINT('Ctrl Pts',(6.16122419188576,1.60035948107341,3.82146210164454));
#134820=CARTESIAN_POINT('Ctrl Pts',(6.13901077410713,1.59355605150694,3.85704672843223));
#134821=CARTESIAN_POINT('Ctrl Pts',(6.11646929960905,1.5867340145087,3.89246750832756));
#134822=CARTESIAN_POINT('Ctrl Pts',(6.8287220845867,1.71660033198358,3.10139008475842));
#134823=CARTESIAN_POINT('Ctrl Pts',(6.83039485279336,1.71596185949179,3.09769633687921));
#134824=CARTESIAN_POINT('Ctrl Pts',(6.832067621,1.715323387,3.094002589));
#134825=CARTESIAN_POINT('Ctrl Pts',(7.00023347,1.651136808,2.72266468));
#134826=CARTESIAN_POINT('Ctrl Pts',(7.127161499,1.585954698,2.33528777));
#134827=CARTESIAN_POINT('Ctrl Pts',(6.49922618194217,1.71660033198358,3.21288351652541));
#134828=CARTESIAN_POINT('Ctrl Pts',(6.50095942147109,1.71596185949179,3.2093678447627));
#134829=CARTESIAN_POINT('Ctrl Pts',(6.502692661,1.715323387,3.205852173));
#134830=CARTESIAN_POINT('Ctrl Pts',(6.676937781,1.651136808,2.852416518));
#134831=CARTESIAN_POINT('Ctrl Pts',(6.81184959,1.585954698,2.482177504));
#134832=CARTESIAN_POINT('',(6.81023510037855,1.5867340152209,2.48660368285477));
#134833=CARTESIAN_POINT('Origin',(-0.187290311837918,1.48222900552861,-0.0499046892512461));
#134834=CARTESIAN_POINT('Ctrl Pts',(7.0458367053091,1.6256495867156,2.57025001046618));
#134835=CARTESIAN_POINT('Ctrl Pts',(7.01880301281208,1.62139779885643,2.56059971734374));
#134836=CARTESIAN_POINT('Ctrl Pts',(6.9917702488842,1.61707840870187,2.5509763023171));
#134837=CARTESIAN_POINT('Ctrl Pts',(6.96473887695019,1.61268792536728,2.54138176494955));
#134838=CARTESIAN_POINT('Ctrl Pts',(6.93897114900315,1.60850268532848,2.53223574641715));
#134839=CARTESIAN_POINT('Ctrl Pts',(6.91320234107661,1.60425381501464,2.52312159228064));
#134840=CARTESIAN_POINT('Ctrl Pts',(6.8874506169071,1.59993003802148,2.51399497175813));
#134841=CARTESIAN_POINT('Ctrl Pts',(6.86169817919846,1.59560614122338,2.50486809835155));
#134842=CARTESIAN_POINT('Ctrl Pts',(6.83595921954746,1.59120881937249,2.49573765613442));
#134843=CARTESIAN_POINT('Ctrl Pts',(6.81023509907772,1.58673401608377,2.48660368644794));
#134844=CARTESIAN_POINT('Ctrl Pts',(6.955094316,1.585967065,2.806539337));
#134845=CARTESIAN_POINT('Ctrl Pts',(6.980365147,1.59657582,2.743913808));
#134846=CARTESIAN_POINT('Ctrl Pts',(7.004504177,1.607142857,2.68084338));
#134847=CARTESIAN_POINT('Ctrl Pts',(7.127046081,1.660786473,2.36066605));
#134848=CARTESIAN_POINT('Ctrl Pts',(7.219867256,1.715323387,2.030644429));
#134849=CARTESIAN_POINT('Ctrl Pts',(7.22098246386582,1.71597862537066,2.02667935629295));
#134850=CARTESIAN_POINT('Ctrl Pts',(7.22209767173163,1.71663386374133,2.0227142835859));
#134851=CARTESIAN_POINT('Ctrl Pts',(6.808614881,1.585967065,2.491036613));
#134852=CARTESIAN_POINT('Ctrl Pts',(6.83104484,1.59657582,2.429730024));
#134853=CARTESIAN_POINT('Ctrl Pts',(6.852367211,1.607142857,2.368029478));
#134854=CARTESIAN_POINT('Ctrl Pts',(6.96061032600001,1.660786473,2.05480636));
#134855=CARTESIAN_POINT('Ctrl Pts',(7.039826773,1.715323387,1.733014427));
#134856=CARTESIAN_POINT('Ctrl Pts',(7.04077852570941,1.71597862537066,1.7291482305762));
#134857=CARTESIAN_POINT('Ctrl Pts',(7.04173027841881,1.71663386374133,1.7252820341524));
#134858=CARTESIAN_POINT('Ctrl Pts',(7.0398267723587,1.71532338598808,1.73301443434052));
#134859=CARTESIAN_POINT('Ctrl Pts',(7.03674478447241,1.71320157782646,1.74553404158354));
#134860=CARTESIAN_POINT('Ctrl Pts',(7.03578215386801,1.71254943786671,1.74938028347368));
#134861=CARTESIAN_POINT('Ctrl Pts',(7.03187812797395,1.70989962932953,1.76500933389786));
#134862=CARTESIAN_POINT('Ctrl Pts',(7.02986684988547,1.70854407402951,1.77300311029435));
#134863=CARTESIAN_POINT('Ctrl Pts',(7.02379362923113,1.70447938484232,1.79696818020817));
#134864=CARTESIAN_POINT('Ctrl Pts',(7.01969082021462,1.70177120841212,1.81292922855852));
#134865=CARTESIAN_POINT('Ctrl Pts',(7.00722572551858,1.69365497346663,1.86074508438884));
#134866=CARTESIAN_POINT('Ctrl Pts',(6.99870059694122,1.68825095320109,1.89255771623979));
#134867=CARTESIAN_POINT('Ctrl Pts',(6.97250587998078,1.6720751488223,1.98770859903185));
#134868=CARTESIAN_POINT('Ctrl Pts',(6.95419024702157,1.66132115703357,2.0508687956172));
#134869=CARTESIAN_POINT('Ctrl Pts',(6.89678398291717,1.62920290563523,2.23921117229545));
#134870=CARTESIAN_POINT('Ctrl Pts',(6.85518854199609,1.60803075408737,2.36348655623575));
#134871=CARTESIAN_POINT('Ctrl Pts',(6.81023510083827,1.58673401461604,2.486603682918));
#134872=CARTESIAN_POINT('Ctrl Pts',(7.33577754858687,1.71660033198358,1.56090791565573));
#134873=CARTESIAN_POINT('Ctrl Pts',(7.33661716179344,1.71596185949179,1.55694092982786));
#134874=CARTESIAN_POINT('Ctrl Pts',(7.337456775,1.715323387,1.552973944));
#134875=CARTESIAN_POINT('Ctrl Pts',(7.421864326,1.651136808,1.154167022));
#134876=CARTESIAN_POINT('Ctrl Pts',(7.462550264,1.585954698,0.748560994));
#134877=CARTESIAN_POINT('Ctrl Pts',(7.03795286930082,1.71660033198358,1.74062657215131));
#134878=CARTESIAN_POINT('Ctrl Pts',(7.03888982115041,1.71596185949179,1.73682049957566));
#134879=CARTESIAN_POINT('Ctrl Pts',(7.039826773,1.715323387,1.733014427));
#134880=CARTESIAN_POINT('Ctrl Pts',(7.134019921,1.651136808,1.350384351));
#134881=CARTESIAN_POINT('Ctrl Pts',(7.186187123,1.585954698,0.959799268000001));
#134882=CARTESIAN_POINT('',(7.18556187676617,1.58673401523149,0.964469033473924));
#134883=CARTESIAN_POINT('Origin',(-0.19363951953293,1.48222901693015,-0.00847605363484161));
#134884=CARTESIAN_POINT('Ctrl Pts',(7.43363673495881,1.62564958676892,0.995512375047741));
#134885=CARTESIAN_POINT('Ctrl Pts',(7.40516054742324,1.62139779886505,0.991899144976718));
#134886=CARTESIAN_POINT('Ctrl Pts',(7.37669104475956,1.6170784087111,0.988311965239451));
#134887=CARTESIAN_POINT('Ctrl Pts',(7.34822910937733,1.61268792537966,0.984752688798697));
#134888=CARTESIAN_POINT('Ctrl Pts',(7.32109769297018,1.60850268534258,0.981359798964417));
#134889=CARTESIAN_POINT('Ctrl Pts',(7.29397207171134,1.60425381504701,0.977998260824985));
#134890=CARTESIAN_POINT('Ctrl Pts',(7.26686045491275,1.59993003805526,0.974620875143033));
#134891=CARTESIAN_POINT('Ctrl Pts',(7.23974808689459,1.59560614125856,0.971243395879125));
#134892=CARTESIAN_POINT('Ctrl Pts',(7.21264811464815,1.59120881939792,0.967859533782329));
#134893=CARTESIAN_POINT('Ctrl Pts',(7.18556187633388,1.58673401612646,0.964469036847194));
#134894=CARTESIAN_POINT('Ctrl Pts',(7.395811073,1.585967065,1.24578432));
#134895=CARTESIAN_POINT('Ctrl Pts',(7.407028448,1.59657582,1.17919046));
#134896=CARTESIAN_POINT('Ctrl Pts',(7.417044844,1.607142857,1.112405405));
#134897=CARTESIAN_POINT('Ctrl Pts',(7.467893124,1.660786473,0.773370756));
#134898=CARTESIAN_POINT('Ctrl Pts',(7.487599299,1.715323387,0.431111049));
#134899=CARTESIAN_POINT('Ctrl Pts',(7.48783606050798,1.71597862537066,0.426998940772556));
#134900=CARTESIAN_POINT('Ctrl Pts',(7.48807282201595,1.71663386374133,0.422886832545111));
#134901=CARTESIAN_POINT('Ctrl Pts',(7.184932486,1.585967065,0.969146623));
#134902=CARTESIAN_POINT('Ctrl Pts',(7.193658941,1.59657582,0.90445157));
#134903=CARTESIAN_POINT('Ctrl Pts',(7.201219013,1.607142857,0.839609869));
#134904=CARTESIAN_POINT('Ctrl Pts',(7.239597753,1.660786473,0.510440663));
#134905=CARTESIAN_POINT('Ctrl Pts',(7.24778641,1.715323387,0.179142852));
#134906=CARTESIAN_POINT('Ctrl Pts',(7.24788479331283,1.71597862537066,0.175162446400145));
#134907=CARTESIAN_POINT('Ctrl Pts',(7.24798317662565,1.71663386374133,0.17118204080029));
#134908=CARTESIAN_POINT('Ctrl Pts',(7.24778640958819,1.71532338425733,0.179142868661036));
#134909=CARTESIAN_POINT('Ctrl Pts',(7.24410800451256,1.69082500283194,0.327964273211171));
#134910=CARTESIAN_POINT('Ctrl Pts',(7.23584926208652,1.66647815067575,0.47636579160891));
#134911=CARTESIAN_POINT('Ctrl Pts',(7.2231022543405,1.64234938933421,0.623934152985415));
#134912=CARTESIAN_POINT('Ctrl Pts',(7.21687369910933,1.63055938138335,0.69604030585824));
#134913=CARTESIAN_POINT('Ctrl Pts',(7.20957429458728,1.61882139352168,0.767947761171279));
#134914=CARTESIAN_POINT('Ctrl Pts',(7.20121901293751,1.60714285691265,0.839609869535977));
#134915=CARTESIAN_POINT('Ctrl Pts',(7.19636592023945,1.60035948103039,0.881234180183976));
#134916=CARTESIAN_POINT('Ctrl Pts',(7.19114716532452,1.59355605149237,0.922857084704198));
#134917=CARTESIAN_POINT('Ctrl Pts',(7.18556187702628,1.5867340145481,0.964469033396799));
#134918=CARTESIAN_POINT('Ctrl Pts',(7.49982020834237,1.71660033198358,-0.052560573154935));
#134919=CARTESIAN_POINT('Ctrl Pts',(7.49978740717118,1.71596185949179,-0.0566153050774675));
#134920=CARTESIAN_POINT('Ctrl Pts',(7.499754606,1.715323387,-0.060670037));
#134921=CARTESIAN_POINT('Ctrl Pts',(7.496457056,1.651136808,-0.468298203));
#134922=CARTESIAN_POINT('Ctrl Pts',(7.448998472,1.585954698,-0.873167661));
#134923=CARTESIAN_POINT('Ctrl Pts',(7.24759270333538,1.71660033198358,0.186979863312151));
#134924=CARTESIAN_POINT('Ctrl Pts',(7.24768955666769,1.71596185949179,0.183061357656076));
#134925=CARTESIAN_POINT('Ctrl Pts',(7.24778641,1.715323387,0.179142852));
#134926=CARTESIAN_POINT('Ctrl Pts',(7.257523218,1.651136808,-0.214790287));
#134927=CARTESIAN_POINT('Ctrl Pts',(7.224506533,1.585954698,-0.607458115));
#134928=CARTESIAN_POINT('',(7.22489976600227,1.58673401521042,-0.602763116913948));
#134929=CARTESIAN_POINT('Origin',(-0.190934634282323,1.48222905617907,0.0333488860263628));
#134930=CARTESIAN_POINT('Ctrl Pts',(7.47384817275646,1.62564958676686,-0.625774312182214));
#134931=CARTESIAN_POINT('Ctrl Pts',(7.44526100500499,1.6213977988801,-0.623181528288945));
#134932=CARTESIAN_POINT('Ctrl Pts',(7.41668596593912,1.61707840874644,-0.620564740192384));
#134933=CARTESIAN_POINT('Ctrl Pts',(7.38812431561075,1.6126879254332,-0.617922327910765));
#134934=CARTESIAN_POINT('Ctrl Pts',(7.36089784559814,1.60850268540349,-0.615403441294639));
#134935=CARTESIAN_POINT('Ctrl Pts',(7.33368377491949,1.60425381509984,-0.612855181841118));
#134936=CARTESIAN_POINT('Ctrl Pts',(7.30647997453032,1.59993003809602,-0.610325409987345));
#134937=CARTESIAN_POINT('Ctrl Pts',(7.27927542036728,1.59560614128724,-0.607795568037634));
#134938=CARTESIAN_POINT('Ctrl Pts',(7.25208160005015,1.59120881941603,-0.605274624400682));
#134939=CARTESIAN_POINT('Ctrl Pts',(7.22489976652123,1.58673401614243,-0.602763113096493));
#134940=CARTESIAN_POINT('Ctrl Pts',(7.490707924,1.585967065,-0.373222187));
#134941=CARTESIAN_POINT('Ctrl Pts',(7.487347331,1.59657582,-0.440670524));
#134942=CARTESIAN_POINT('Ctrl Pts',(7.482772737,1.607142857,-0.50804741));
#134943=CARTESIAN_POINT('Ctrl Pts',(7.459549785,1.660786473,-0.850086495));
#134944=CARTESIAN_POINT('Ctrl Pts',(7.40521952,1.715323387,-1.188580606));
#134945=CARTESIAN_POINT('Ctrl Pts',(7.40456676443124,1.71597862537066,-1.19264747215549));
#134946=CARTESIAN_POINT('Ctrl Pts',(7.40391400886248,1.71663386374133,-1.19671433831097));
#134947=CARTESIAN_POINT('Ctrl Pts',(7.225290633,1.585967065,-0.598059586));
#134948=CARTESIAN_POINT('Ctrl Pts',(7.219905545,1.59657582,-0.663118034));
#134949=CARTESIAN_POINT('Ctrl Pts',(7.213349817,1.607142857,-0.728068964));
#134950=CARTESIAN_POINT('Ctrl Pts',(7.180069635,1.660786473,-1.057792671));
#134951=CARTESIAN_POINT('Ctrl Pts',(7.116847609,1.715323387,-1.383105243));
#134952=CARTESIAN_POINT('Ctrl Pts',(7.11608802261588,1.71597862537066,-1.38701373843915));
#134953=CARTESIAN_POINT('Ctrl Pts',(7.11532843623176,1.71663386374133,-1.39092223387829));
#134954=CARTESIAN_POINT('Ctrl Pts',(7.11684761207532,1.71532338434715,-1.38310522717576));
#134955=CARTESIAN_POINT('Ctrl Pts',(7.14524739863188,1.69082501198697,-1.23697248985002));
#134956=CARTESIAN_POINT('Ctrl Pts',(7.16908367371738,1.66647816873387,-1.09026518511952));
#134957=CARTESIAN_POINT('Ctrl Pts',(7.18835751572347,1.64234941611947,-0.94340671439929));
#134958=CARTESIAN_POINT('Ctrl Pts',(7.19777528077458,1.63055939921329,-0.871647354092652));
#134959=CARTESIAN_POINT('Ctrl Pts',(7.20610451662223,1.61882140247104,-0.799851844908871));
#134960=CARTESIAN_POINT('Ctrl Pts',(7.2133498171633,1.60714285707959,-0.728068964315511));
#134961=CARTESIAN_POINT('Ctrl Pts',(7.21755818397531,1.60035948117327,-0.686374535307469));
#134962=CARTESIAN_POINT('Ctrl Pts',(7.22140913456291,1.59355605158198,-0.644602873176996));
#134963=CARTESIAN_POINT('Ctrl Pts',(7.22489976573252,1.58673401461327,-0.602763116988815));
#134964=CARTESIAN_POINT('Ctrl Pts',(7.31317960960073,1.71660033198358,-1.66357138748205));
#134965=CARTESIAN_POINT('Ctrl Pts',(7.31227592780037,1.71596185949179,-1.66752427074103));
#134966=CARTESIAN_POINT('Ctrl Pts',(7.311372246,1.715323387,-1.671477154));
#134967=CARTESIAN_POINT('Ctrl Pts',(7.220523785,1.651136808,-2.068866324));
#134968=CARTESIAN_POINT('Ctrl Pts',(7.087139791,1.585954698,-2.454067967));
#134969=CARTESIAN_POINT('Ctrl Pts',(7.11834315687191,1.71660033198358,-1.37540981543085));
#134970=CARTESIAN_POINT('Ctrl Pts',(7.11759538293595,1.71596185949179,-1.37925752921543));
#134971=CARTESIAN_POINT('Ctrl Pts',(7.116847609,1.715323387,-1.383105243));
#134972=CARTESIAN_POINT('Ctrl Pts',(7.04167279500001,1.651136808,-1.769921571));
#134973=CARTESIAN_POINT('Ctrl Pts',(6.925016046,1.585954698,-2.146311431));
#134974=CARTESIAN_POINT('',(6.92640937099897,1.58673401527515,-2.14181073446729));
#134975=CARTESIAN_POINT('Origin',(-0.179301677008858,1.4822289963032,0.0736145282351569));
#134976=CARTESIAN_POINT('Ctrl Pts',(7.16459077630825,1.62564958672988,-2.21780048805578));
#134977=CARTESIAN_POINT('Ctrl Pts',(7.13722933254449,1.62139779886377,-2.20912292591444));
#134978=CARTESIAN_POINT('Ctrl Pts',(7.1098848940126,1.61707840872217,-2.20042452820074));
#134979=CARTESIAN_POINT('Ctrl Pts',(7.08255903964804,1.61268792540122,-2.19170398356328));
#134980=CARTESIAN_POINT('Ctrl Pts',(7.05651059551737,1.60850268537298,-2.18339110094496));
#134981=CARTESIAN_POINT('Ctrl Pts',(7.03048057511913,1.60425381506448,-2.17505219774219));
#134982=CARTESIAN_POINT('Ctrl Pts',(7.00445661063308,1.59993003806697,-2.16673355763766));
#134983=CARTESIAN_POINT('Ctrl Pts',(6.97843192506457,1.59560614126451,-2.15841468703692));
#134984=CARTESIAN_POINT('Ctrl Pts',(6.95241580953442,1.59120881940851,-2.15010681410913));
#134985=CARTESIAN_POINT('Ctrl Pts',(6.92640937246645,1.58673401608731,-2.14181072954637));
#134986=CARTESIAN_POINT('Ctrl Pts',(7.235347597,1.585967065,-1.97477724));
#134987=CARTESIAN_POINT('Ctrl Pts',(7.217566175,1.59657582,-2.039926244));
#134988=CARTESIAN_POINT('Ctrl Pts',(7.198614493,1.607142857,-2.104744493));
#134989=CARTESIAN_POINT('Ctrl Pts',(7.102406188,1.660786473,-2.433794646));
#134990=CARTESIAN_POINT('Ctrl Pts',(6.976579907,1.715323387,-2.752695552));
#134991=CARTESIAN_POINT('Ctrl Pts',(6.97506815649374,1.71597862537066,-2.75652701393514));
#134992=CARTESIAN_POINT('Ctrl Pts',(6.97355640598748,1.71663386374133,-2.76035847587028));
#134993=CARTESIAN_POINT('Ctrl Pts',(6.927802221,1.585967065,-2.137301193));
#134994=CARTESIAN_POINT('Ctrl Pts',(6.90855739,1.59657582,-2.199680976));
#134995=CARTESIAN_POINT('Ctrl Pts',(6.888192401,1.607142857,-2.261704102));
#134996=CARTESIAN_POINT('Ctrl Pts',(6.78480944,1.660786473,-2.576564797));
#134997=CARTESIAN_POINT('Ctrl Pts',(6.653132924,1.715323387,-2.880680874));
#134998=CARTESIAN_POINT('Ctrl Pts',(6.65155088535002,1.71597862537066,-2.88433470235535));
#134999=CARTESIAN_POINT('Ctrl Pts',(6.64996884670004,1.71663386374133,-2.8879885307107));
#135000=CARTESIAN_POINT('Ctrl Pts',(6.65313292612395,1.71532338611517,-2.88068086759738));
#135001=CARTESIAN_POINT('Ctrl Pts',(6.71228296416041,1.69082501192151,-2.7440697389745));
#135002=CARTESIAN_POINT('Ctrl Pts',(6.76709969595371,1.66647816771549,-2.60591645951733));
#135003=CARTESIAN_POINT('Ctrl Pts',(6.81749315660543,1.64234941497924,-2.46663476376996));
#135004=CARTESIAN_POINT('Ctrl Pts',(6.84211688048578,1.6305593982336,-2.39857763942654));
#135005=CARTESIAN_POINT('Ctrl Pts',(6.86568529500849,1.61882140184801,-2.33025121065281));
#135006=CARTESIAN_POINT('Ctrl Pts',(6.88819240103793,1.60714285700126,-2.26170410208723));
#135007=CARTESIAN_POINT('Ctrl Pts',(6.9012654487764,1.60035948085629,-2.22188913820699));
#135008=CARTESIAN_POINT('Ctrl Pts',(6.91400603931158,1.593556051179,-2.18192191381413));
#135009=CARTESIAN_POINT('Ctrl Pts',(6.926409371,1.586734015,-2.141810735));
#135010=CARTESIAN_POINT('Ctrl Pts',(6.78458286054717,1.71660033198358,-3.19679545366646));
#135011=CARTESIAN_POINT('Ctrl Pts',(6.78285055327358,1.71596185949179,-3.20046165583323));
#135012=CARTESIAN_POINT('Ctrl Pts',(6.78111824600001,1.715323387,-3.204127858));
#135013=CARTESIAN_POINT('Ctrl Pts',(6.606966847,1.651136808,-3.572696556));
#135014=CARTESIAN_POINT('Ctrl Pts',(6.39389433,1.585954698,-3.920218782));
#135015=CARTESIAN_POINT('Ctrl Pts',(6.6562477962472,1.71660033198358,-2.87348685982246));
#135016=CARTESIAN_POINT('Ctrl Pts',(6.6546903601236,1.71596185949179,-2.87708386691123));
#135017=CARTESIAN_POINT('Ctrl Pts',(6.653132924,1.715323387,-2.880680874));
#135018=CARTESIAN_POINT('Ctrl Pts',(6.496561579,1.651136808,-3.242293289));
#135019=CARTESIAN_POINT('Ctrl Pts',(6.301719506,1.585954698,-3.58480561));
#135020=CARTESIAN_POINT('',(6.30404777345953,1.58673401521883,-3.58070965999336));
#135021=CARTESIAN_POINT('Origin',(-0.159284671104115,1.48222897082287,0.110437985497804));
#135022=CARTESIAN_POINT('Ctrl Pts',(6.52032507811018,1.62564958671635,-3.70612477820676));
#135023=CARTESIAN_POINT('Ctrl Pts',(6.49546874906344,1.62139779884951,-3.69176819098134));
#135024=CARTESIAN_POINT('Ctrl Pts',(6.47063350665613,1.61707840869391,-3.67739491099258));
#135025=CARTESIAN_POINT('Ctrl Pts',(6.44582117486303,1.61268792535999,-3.6630039969133));
#135026=CARTESIAN_POINT('Ctrl Pts',(6.42216875293301,1.60850268532869,-3.64928581941188));
#135027=CARTESIAN_POINT('Ctrl Pts',(6.39853991765919,1.60425381501957,-3.6355461902282));
#135028=CARTESIAN_POINT('Ctrl Pts',(6.37491264077159,1.5999300380313,-3.62182765219868));
#135029=CARTESIAN_POINT('Ctrl Pts',(6.35128470921003,1.5956061412381,-3.60810873405046));
#135030=CARTESIAN_POINT('Ctrl Pts',(6.32766278316444,1.59120881939816,-3.59440239872991));
#135031=CARTESIAN_POINT('Ctrl Pts',(6.30404777520744,1.58673401614287,-3.58070965616356));
#135032=CARTESIAN_POINT('Ctrl Pts',(6.641670459,1.585967065,-3.483993903));
#135033=CARTESIAN_POINT('Ctrl Pts',(6.610299646,1.59657582,-3.54379728));
#135034=CARTESIAN_POINT('Ctrl Pts',(6.577857036,1.607142857,-3.603026063));
#135035=CARTESIAN_POINT('Ctrl Pts',(6.41316197200001,1.660786473,-3.903701264));
#135036=CARTESIAN_POINT('Ctrl Pts',(6.221723171,1.715323387,-4.188097513));
#135037=CARTESIAN_POINT('Ctrl Pts',(6.21942311331706,1.71597862537066,-4.19151441581224));
#135038=CARTESIAN_POINT('Ctrl Pts',(6.21712305563413,1.71663386374133,-4.1949313186245));
#135039=CARTESIAN_POINT('Ctrl Pts',(6.306377476,1.585967065,-3.576604972));
#135040=CARTESIAN_POINT('Ctrl Pts',(6.274172769,1.59657582,-3.633389281));
#135041=CARTESIAN_POINT('Ctrl Pts',(6.240950764,1.607142857,-3.68958447));
#135042=CARTESIAN_POINT('Ctrl Pts',(6.072299097,1.660786473,-3.974859616));
#135043=CARTESIAN_POINT('Ctrl Pts',(5.878325138,1.715323387,-4.24355907));
#135044=CARTESIAN_POINT('Ctrl Pts',(5.87599462144663,1.71597862537066,-4.24678738233974));
#135045=CARTESIAN_POINT('Ctrl Pts',(5.87366410489327,1.71663386374133,-4.25001569467948));
#135046=CARTESIAN_POINT('Ctrl Pts',(5.87832514762602,1.71532338429359,-4.2435590566657));
#135047=CARTESIAN_POINT('Ctrl Pts',(5.96545964263553,1.6908250109101,-4.12285733223717));
#135048=CARTESIAN_POINT('Ctrl Pts',(6.04869366166071,1.66647816661746,-3.99971797539809));
#135049=CARTESIAN_POINT('Ctrl Pts',(6.12785040151841,1.64234941292913,-3.87452570760659));
#135050=CARTESIAN_POINT('Ctrl Pts',(6.16652870330467,1.63055939708763,-3.81335309838025));
#135051=CARTESIAN_POINT('Ctrl Pts',(6.20423426152324,1.61882140138784,-3.75169061978853));
#135052=CARTESIAN_POINT('Ctrl Pts',(6.24095076432877,1.60714285701179,-3.68958446996873));
#135053=CARTESIAN_POINT('Ctrl Pts',(6.26227721078558,1.60035948109084,-3.6535106782366));
#135054=CARTESIAN_POINT('Ctrl Pts',(6.28331170442055,1.59355605152486,-3.61721671655659));
#135055=CARTESIAN_POINT('Ctrl Pts',(6.30404777321125,1.58673401456331,-3.58070965997483));
#135056=CARTESIAN_POINT('Ctrl Pts',(5.93874655798517,1.71660033198358,-4.5805409169344));
#135057=CARTESIAN_POINT('Ctrl Pts',(5.93626662599258,1.71596185949179,-4.5837490104672));
#135058=CARTESIAN_POINT('Ctrl Pts',(5.933786694,1.715323387,-4.586957104));
#135059=CARTESIAN_POINT('Ctrl Pts',(5.68447548200001,1.651136808,-4.909471467));
#135060=CARTESIAN_POINT('Ctrl Pts',(5.401677476,1.585954698,-5.203064524));
#135061=CARTESIAN_POINT('Ctrl Pts',(5.88291368665965,1.71660033198358,-4.23720285334885));
#135062=CARTESIAN_POINT('Ctrl Pts',(5.88061941232983,1.71596185949179,-4.24038096167442));
#135063=CARTESIAN_POINT('Ctrl Pts',(5.878325138,1.715323387,-4.24355907));
#135064=CARTESIAN_POINT('Ctrl Pts',(5.647678364,1.651136808,-4.563058976));
#135065=CARTESIAN_POINT('Ctrl Pts',(5.383761566,1.585954698,-4.855678264));
#135066=CARTESIAN_POINT('',(5.38691590788117,1.58673401522098,-4.85217858289702));
#135067=CARTESIAN_POINT('Origin',(-0.131819883971023,1.48222899047365,0.142097578797142));
#135068=CARTESIAN_POINT('Ctrl Pts',(5.57117622601978,1.62564958674757,-5.02115479281309));
#135069=CARTESIAN_POINT('Ctrl Pts',(5.54998726590558,1.62139779884887,-5.00179047884981));
#135070=CARTESIAN_POINT('Ctrl Pts',(5.5288224880741,1.61707840870451,-4.98241439515562));
#135071=CARTESIAN_POINT('Ctrl Pts',(5.50768387604366,1.61268792538439,-4.96302601473718));
#135072=CARTESIAN_POINT('Ctrl Pts',(5.48753343727595,1.60850268535182,-4.94454398896063));
#135073=CARTESIAN_POINT('Ctrl Pts',(5.46741064525574,1.60425381505338,-4.92604608340411));
#135074=CARTESIAN_POINT('Ctrl Pts',(5.44728484120158,1.59993003807154,-4.90756911092237));
#135075=CARTESIAN_POINT('Ctrl Pts',(5.42715847949359,1.59560614128475,-4.88909162647329));
#135076=CARTESIAN_POINT('Ctrl Pts',(5.40703527793745,1.59120881944353,-4.87062772170985));
#135077=CARTESIAN_POINT('Ctrl Pts',(5.38691591042844,1.58673401610884,-4.85217858048633));
#135078=CARTESIAN_POINT('Ctrl Pts',(5.737436191,1.585967065,-4.830302884));
#135079=CARTESIAN_POINT('Ctrl Pts',(5.693942853,1.59657582,-4.881964294));
#135080=CARTESIAN_POINT('Ctrl Pts',(5.649526295,1.607142857,-4.932834139));
#135081=CARTESIAN_POINT('Ctrl Pts',(5.42404543,1.660786473,-5.19107515));
#135082=CARTESIAN_POINT('Ctrl Pts',(5.175945575,1.715323387,-5.42766869));
#135083=CARTESIAN_POINT('Ctrl Pts',(5.17296475828653,1.71597862537066,-5.43051126311771));
#135084=CARTESIAN_POINT('Ctrl Pts',(5.16998394157306,1.71663386374133,-5.43335383623542));
#135085=CARTESIAN_POINT('Ctrl Pts',(5.39007353,1.585967065,-4.848670677));
#135086=CARTESIAN_POINT('Ctrl Pts',(5.346414803,1.59657582,-4.89720434));
#135087=CARTESIAN_POINT('Ctrl Pts',(5.301889206,1.607142857,-4.944943968));
#135088=CARTESIAN_POINT('Ctrl Pts',(5.075854798,1.660786473,-5.187294417));
#135089=CARTESIAN_POINT('Ctrl Pts',(4.828653401,1.715323387,-5.408013159));
#135090=CARTESIAN_POINT('Ctrl Pts',(4.82568337888624,1.71597862537066,-5.41066500301309));
#135091=CARTESIAN_POINT('Ctrl Pts',(4.82271335677248,1.71663386374133,-5.41331684702618));
#135092=CARTESIAN_POINT('Ctrl Pts',(4.82865341292025,1.71532338437019,-5.40801314835676));
#135093=CARTESIAN_POINT('Ctrl Pts',(4.93969804922549,1.69082501233844,-5.30886470972604));
#135094=CARTESIAN_POINT('Ctrl Pts',(5.04745741921797,1.66647816940417,-5.20649714239737));
#135095=CARTESIAN_POINT('Ctrl Pts',(5.15167614981874,1.64234941710383,-5.10124816592978));
#135096=CARTESIAN_POINT('Ctrl Pts',(5.20260048333634,1.6305593998735,-5.04982042401502));
#135097=CARTESIAN_POINT('Ctrl Pts',(5.25268012264772,1.61882140281017,-4.99770515434739));
#135098=CARTESIAN_POINT('Ctrl Pts',(5.30188920605868,1.60714285710216,-4.94494396844451));
#135099=CARTESIAN_POINT('Ctrl Pts',(5.33047185070332,1.60035948118248,-4.91429811729116));
#135100=CARTESIAN_POINT('Ctrl Pts',(5.35881669862536,1.5935560516734,-4.88337448286254));
#135101=CARTESIAN_POINT('Ctrl Pts',(5.3869159075036,1.58673401462794,-4.85217858268661));
#135102=CARTESIAN_POINT('Ctrl Pts',(4.81522106667948,1.71660033198358,-5.75010537695528));
#135103=CARTESIAN_POINT('Ctrl Pts',(4.81210946883974,1.71596185949179,-5.75270535497764));
#135104=CARTESIAN_POINT('Ctrl Pts',(4.808997871,1.715323387,-5.755305333));
#135105=CARTESIAN_POINT('Ctrl Pts',(4.496184362,1.651136808,-6.016684949));
#135106=CARTESIAN_POINT('Ctrl Pts',(4.156884187,1.585954698,-6.242620752));
#135107=CARTESIAN_POINT('Ctrl Pts',(4.83450107061284,1.71660033198358,-5.40279194947145));
#135108=CARTESIAN_POINT('Ctrl Pts',(4.83157723580641,1.71596185949179,-5.40540255423573));
#135109=CARTESIAN_POINT('Ctrl Pts',(4.828653401,1.715323387,-5.40801315900001));
#135110=CARTESIAN_POINT('Ctrl Pts',(4.534715986,1.651136808,-5.670461097));
#135111=CARTESIAN_POINT('Ctrl Pts',(4.214064918,1.585954698,-5.899504798));
#135112=CARTESIAN_POINT('',(4.21789784021562,1.5867340152838,-5.89676502875833));
#135113=CARTESIAN_POINT('Origin',(-0.0981910441401429,1.48222903544964,
0.167112545806996));
#135114=CARTESIAN_POINT('Ctrl Pts',(4.36152536588842,1.62564958678343,-6.10140118971835));
#135115=CARTESIAN_POINT('Ctrl Pts',(4.34499454697019,1.62139779888937,-6.07793460252609));
#135116=CARTESIAN_POINT('Ctrl Pts',(4.32848987505951,1.61707840874017,-6.05446171928497));
#135117=CARTESIAN_POINT('Ctrl Pts',(4.31201340060561,1.61268792541011,-6.03098245170926));
#135118=CARTESIAN_POINT('Ctrl Pts',(4.29630715704654,1.60850268537488,-6.00860077678453));
#135119=CARTESIAN_POINT('Ctrl Pts',(4.28063132748528,1.6042538150622,-5.98620953662333));
#135120=CARTESIAN_POINT('Ctrl Pts',(4.26494805633297,1.59993003807245,-5.963838092623));
#135121=CARTESIAN_POINT('Ctrl Pts',(4.24926435062233,1.59560614127776,-5.94146602874581));
#135122=CARTESIAN_POINT('Ctrl Pts',(4.23358081196648,1.59120881943565,-5.91910790639485));
#135123=CARTESIAN_POINT('Ctrl Pts',(4.21789784426445,1.58673401613719,-5.89676502585763));
#135124=CARTESIAN_POINT('Ctrl Pts',(4.564925784,1.585967065,-5.950752271));
#135125=CARTESIAN_POINT('Ctrl Pts',(4.51134362,1.59657582,-5.99185608300001));
#135126=CARTESIAN_POINT('Ctrl Pts',(4.457029984,1.607142857,-6.031988372));
#135127=CARTESIAN_POINT('Ctrl Pts',(4.181306552,1.660786473,-6.235720132));
#135128=CARTESIAN_POINT('Ctrl Pts',(3.888146516,1.715323387,-6.41344811100001));
#135129=CARTESIAN_POINT('Ctrl Pts',(3.88462431992685,1.71597862537066,-6.41558343885118));
#135130=CARTESIAN_POINT('Ctrl Pts',(3.8811021238537,1.71663386374133,-6.41771876670236));
#135131=CARTESIAN_POINT('Ctrl Pts',(4.221735737,1.585967065,-5.894017931));
#135132=CARTESIAN_POINT('Ctrl Pts',(4.168664423,1.59657582,-5.932031568));
#135133=CARTESIAN_POINT('Ctrl Pts',(4.114917201,1.607142857,-5.969083383));
#135134=CARTESIAN_POINT('Ctrl Pts',(3.842069169,1.660786473,-6.157177096));
#135135=CARTESIAN_POINT('Ctrl Pts',(3.553199198,1.715323387,-6.319594564));
#135136=CARTESIAN_POINT('Ctrl Pts',(3.54972854527601,1.71597862537066,-6.32154594242049));
#135137=CARTESIAN_POINT('Ctrl Pts',(3.54625789255202,1.71663386374133,-6.32349732084099));
#135138=CARTESIAN_POINT('Ctrl Pts',(3.55319920437648,1.71532338607709,-6.31959456096104));
#135139=CARTESIAN_POINT('Ctrl Pts',(3.68296167347084,1.69082501162648,-6.24663546560832));
#135140=CARTESIAN_POINT('Ctrl Pts',(3.81020769735712,1.66647816717725,-6.16982626951713));
#135141=CARTESIAN_POINT('Ctrl Pts',(3.93461527411236,1.64234941421584,-6.08944189945254));
#135142=CARTESIAN_POINT('Ctrl Pts',(3.99540446547425,1.6305593977285,-6.05016373825198));
#135143=CARTESIAN_POINT('Ctrl Pts',(4.05551650849235,1.61882140160225,-6.01003253971538));
#135144=CARTESIAN_POINT('Ctrl Pts',(4.11491720092053,1.60714285701562,-5.96908338305479));
#135145=CARTESIAN_POINT('Ctrl Pts',(4.1494195531229,1.60035948087342,-5.94529843739841));
#135146=CARTESIAN_POINT('Ctrl Pts',(4.1837493825457,1.59355605118872,-5.92119108391622));
#135147=CARTESIAN_POINT('Ctrl Pts',(4.21789784,1.586734015,-5.896765029));
#135148=CARTESIAN_POINT('Ctrl Pts',(3.46654118966067,1.71660033198358,-6.65080130115457));
#135149=CARTESIAN_POINT('Ctrl Pts',(3.46294342083033,1.71596185949179,-6.65267159157729));
#135150=CARTESIAN_POINT('Ctrl Pts',(3.459345652,1.715323387,-6.654541882));
#135151=CARTESIAN_POINT('Ctrl Pts',(3.097656658,1.651136808,-6.84256493));
#135152=CARTESIAN_POINT('Ctrl Pts',(2.717719614,1.585954698,-6.990278972));
#135153=CARTESIAN_POINT('Ctrl Pts',(3.56003255805081,1.71660033198358,-6.31575249957073));
#135154=CARTESIAN_POINT('Ctrl Pts',(3.5566158780254,1.71596185949179,-6.31767353178537));
#135155=CARTESIAN_POINT('Ctrl Pts',(3.553199198,1.715323387,-6.319594564));
#135156=CARTESIAN_POINT('Ctrl Pts',(3.209715328,1.651136808,-6.512718759));
#135157=CARTESIAN_POINT('Ctrl Pts',(2.847323279,1.585954698,-6.667477045));
#135158=CARTESIAN_POINT('',(2.85165556048068,1.58673401523959,-6.66562529465689));
#135159=CARTESIAN_POINT('Origin',(-0.0599712233341998,1.48222903854166,
0.184313888207516));
#135160=CARTESIAN_POINT('Ctrl Pts',(2.94793442687893,1.6256495867408,-6.89635284857505));
#135161=CARTESIAN_POINT('Ctrl Pts',(2.93683471205565,1.62139779887027,-6.86988125968827));
#135162=CARTESIAN_POINT('Ctrl Pts',(2.92576188631293,1.61707840873292,-6.84340914287658));
#135163=CARTESIAN_POINT('Ctrl Pts',(2.91471797125889,1.61268792541888,-6.81693685259069));
#135164=CARTESIAN_POINT('Ctrl Pts',(2.90419032953264,1.60850268539221,-6.79170207068234));
#135165=CARTESIAN_POINT('Ctrl Pts',(2.89369444699762,1.6042538150892,-6.76646448526372));
#135166=CARTESIAN_POINT('Ctrl Pts',(2.88318704114662,1.59993003808792,-6.74124463351249));
#135167=CARTESIAN_POINT('Ctrl Pts',(2.8726793441522,1.5956061412817,-6.7160240829595));
#135168=CARTESIAN_POINT('Ctrl Pts',(2.86216881324473,1.5912088194187,-6.69081718391987));
#135169=CARTESIAN_POINT('Ctrl Pts',(2.85165556371443,1.5867340161584,-6.66562529299552));
#135170=CARTESIAN_POINT('Ctrl Pts',(3.178964521,1.585967065,-6.792951095));
#135171=CARTESIAN_POINT('Ctrl Pts',(3.117798973,1.59657582,-6.821575341));
#135172=CARTESIAN_POINT('Ctrl Pts',(3.056127904,1.607142857,-6.849093534));
#135173=CARTESIAN_POINT('Ctrl Pts',(2.743054426,1.660786473,-6.98878977));
#135174=CARTESIAN_POINT('Ctrl Pts',(2.418542048,1.715323387,-7.099341826));
#135175=CARTESIAN_POINT('Ctrl Pts',(2.41464316655942,1.71597862537066,-7.10067006303679));
#135176=CARTESIAN_POINT('Ctrl Pts',(2.41074428511884,1.71663386374133,-7.10199830007359));
#135177=CARTESIAN_POINT('Ctrl Pts',(2.855994272,1.585967065,-6.663767457));
#135178=CARTESIAN_POINT('Ctrl Pts',(2.795991928,1.59657582,-6.689483593));
#135179=CARTESIAN_POINT('Ctrl Pts',(2.735536241,1.607142857,-6.714115092));
#135180=CARTESIAN_POINT('Ctrl Pts',(2.428632656,1.660786473,-6.839157018));
#135181=CARTESIAN_POINT('Ctrl Pts',(2.11160135,1.715323387,-6.935678751));
#135182=CARTESIAN_POINT('Ctrl Pts',(2.10779235053235,1.71597862537066,-6.93683841953322));
#135183=CARTESIAN_POINT('Ctrl Pts',(2.1039833510647,1.71663386374133,-6.93799808806643));
#135184=CARTESIAN_POINT('Ctrl Pts',(2.1116013570794,1.71532338594482,-6.93567874963665));
#135185=CARTESIAN_POINT('Ctrl Pts',(2.12393574773601,1.71320157779459,-6.93192348391174));
#135186=CARTESIAN_POINT('Ctrl Pts',(2.12772423295924,1.71254943784492,-6.93075403377145));
#135187=CARTESIAN_POINT('Ctrl Pts',(2.14311900235626,1.70989962930861,-6.92600959375084));
#135188=CARTESIAN_POINT('Ctrl Pts',(2.15099216679657,1.70854407400994,-6.92356849105429));
#135189=CARTESIAN_POINT('Ctrl Pts',(2.17459329235689,1.70447938482579,-6.91620673459527));
#135190=CARTESIAN_POINT('Ctrl Pts',(2.19030881086288,1.70177120839844,-6.91124582897896));
#135191=CARTESIAN_POINT('Ctrl Pts',(2.23737969405122,1.69365497345755,-6.8962103172014));
#135192=CARTESIAN_POINT('Ctrl Pts',(2.26868412879233,1.68825095319847,-6.88597539031003));
#135193=CARTESIAN_POINT('Ctrl Pts',(2.36227728757173,1.67207515293314,-6.8546677331669));
#135194=CARTESIAN_POINT('Ctrl Pts',(2.42435327818651,1.66132115912265,-6.83295953415283));
#135195=CARTESIAN_POINT('Ctrl Pts',(2.60931157749119,1.62920289813894,-6.76544079017663));
#135196=CARTESIAN_POINT('Ctrl Pts',(2.73115276257568,1.60803074733088,-6.7171782188802));
#135197=CARTESIAN_POINT('Ctrl Pts',(2.8516555605562,1.5867340146619,-6.66562529507205));
#135198=CARTESIAN_POINT('Ctrl Pts',(1.95576969930549,1.71660033198358,-7.24051314774188));
#135199=CARTESIAN_POINT('Ctrl Pts',(1.95185398715275,1.71596185949179,-7.24156629787095));
#135200=CARTESIAN_POINT('Ctrl Pts',(1.947938275,1.715323387,-7.242619448));
#135201=CARTESIAN_POINT('Ctrl Pts',(1.554285971,1.651136808,-7.34849418));
#135202=CARTESIAN_POINT('Ctrl Pts',(1.151477492,1.585954698,-7.41107951600001));
#135203=CARTESIAN_POINT('Ctrl Pts',(2.11910088016766,1.71660033198358,-6.93339548231832));
#135204=CARTESIAN_POINT('Ctrl Pts',(2.11535111508383,1.71596185949179,-6.93453711665916));
#135205=CARTESIAN_POINT('Ctrl Pts',(2.11160135,1.715323387,-6.935678751));
#135206=CARTESIAN_POINT('Ctrl Pts',(1.734631949,1.651136808,-7.050448931));
#135207=CARTESIAN_POINT('Ctrl Pts',(1.347443968,1.585954698,-7.123685476));
#135208=CARTESIAN_POINT('',(1.35207303377562,1.58673401519647,-7.12280833071507));
#135209=CARTESIAN_POINT('Origin',(-0.0189470888890086,1.48222904029177,
0.192896751804501));
#135210=CARTESIAN_POINT('Ctrl Pts',(1.39650135047031,1.6256495867804,-7.36883871285757));
#135211=CARTESIAN_POINT('Ctrl Pts',(1.39135174990273,1.62139779887436,-7.34059990434166));
#135212=CARTESIAN_POINT('Ctrl Pts',(1.38622852329221,1.6170784087104,-7.31236636061691));
#135213=CARTESIAN_POINT('Ctrl Pts',(1.38113356873396,1.61268792536747,-7.28413886241582));
#135214=CARTESIAN_POINT('Ctrl Pts',(1.37627678961722,1.6085026853288,-7.2572309239418));
#135215=CARTESIAN_POINT('Ctrl Pts',(1.3714516299737,1.60425381503388,-7.23032707476029));
#135216=CARTESIAN_POINT('Ctrl Pts',(1.366611404198,1.59993003804022,-7.20343806747254));
#135217=CARTESIAN_POINT('Ctrl Pts',(1.36177104430736,1.59560614124161,-7.17654831513328));
#135218=CARTESIAN_POINT('Ctrl Pts',(1.35692498200514,1.59120881937363,-7.14967128595165));
#135219=CARTESIAN_POINT('Ctrl Pts',(1.35207303748469,1.58673401603004,-7.12280833022491));
#135220=CARTESIAN_POINT('Ctrl Pts',(1.64435841,1.585967065,-7.317519076));
#135221=CARTESIAN_POINT('Ctrl Pts',(1.578469512,1.59657582,-7.332325318));
#135222=CARTESIAN_POINT('Ctrl Pts',(1.51232468,1.607142857,-7.345942694));
#135223=CARTESIAN_POINT('Ctrl Pts',(1.176540125,1.660786473,-7.415071367));
#135224=CARTESIAN_POINT('Ctrl Pts',(0.835849241,1.715323387,-7.453278208));
#135225=CARTESIAN_POINT('Ctrl Pts',(0.831755981529315,1.71597862537066,
-7.453737247326));
#135226=CARTESIAN_POINT('Ctrl Pts',(0.82766272205863,1.71663386374133,-7.45419628665201));
#135227=CARTESIAN_POINT('Ctrl Pts',(1.356709689,1.585967065,-7.121926623));
#135228=CARTESIAN_POINT('Ctrl Pts',(1.292581958,1.59657582,-7.134142799));
#135229=CARTESIAN_POINT('Ctrl Pts',(1.228244647,1.607142857,-7.145202243));
#135230=CARTESIAN_POINT('Ctrl Pts',(0.901635979,1.660786473,-7.201345559));
#135231=CARTESIAN_POINT('Ctrl Pts',(0.57126737,1.715323387,-7.227458308));
#135232=CARTESIAN_POINT('Ctrl Pts',(0.567298128376246,1.71597862537066,
-7.22777204183371));
#135233=CARTESIAN_POINT('Ctrl Pts',(0.563328886752492,1.71663386374133,
-7.22808577566744));
#135234=CARTESIAN_POINT('Ctrl Pts',(0.571267377071571,1.71532338597849,
-7.22745830826502));
#135235=CARTESIAN_POINT('Ctrl Pts',(0.584120668103141,1.71320157775186,
-7.22644236793295));
#135236=CARTESIAN_POINT('Ctrl Pts',(0.58807197768213,1.71254943783057,-7.22611467124006));
#135237=CARTESIAN_POINT('Ctrl Pts',(0.604126740209036,1.70989962930403,
-7.22479057396694));
#135238=CARTESIAN_POINT('Ctrl Pts',(0.612340599370621,1.7085440740024,-7.22409904052771));
#135239=CARTESIAN_POINT('Ctrl Pts',(0.636972503771454,1.70447938481183,
-7.22198294221739));
#135240=CARTESIAN_POINT('Ctrl Pts',(0.653387050275347,1.70177120837809,
-7.2205163917624));
#135241=CARTESIAN_POINT('Ctrl Pts',(0.702589632971672,1.69365497342768,
-7.21595125041875));
#135242=CARTESIAN_POINT('Ctrl Pts',(0.735362394227467,1.68825095315395,
-7.21268513857028));
#135243=CARTESIAN_POINT('Ctrl Pts',(0.833497639285269,1.67207514933648,
-7.20222919738827));
#135244=CARTESIAN_POINT('Ctrl Pts',(0.898788938037303,1.66132115724861,
-7.19437302764026));
#135245=CARTESIAN_POINT('Ctrl Pts',(1.09393752057592,1.62920290096259,-7.16819340536559));
#135246=CARTESIAN_POINT('Ctrl Pts',(1.22330512767297,1.608030754495,-7.14725144361751));
#135247=CARTESIAN_POINT('Ctrl Pts',(1.35207303373849,1.58673401467295,-7.1228083309756));
#135248=CARTESIAN_POINT('Ctrl Pts',(0.353548592258207,1.71660033198358,
-7.49166664761222));
#135249=CARTESIAN_POINT('Ctrl Pts',(0.349498031129103,1.71596185949179,
-7.49185341330611));
#135250=CARTESIAN_POINT('Ctrl Pts',(0.34544747,1.715323387,-7.492040179));
#135251=CARTESIAN_POINT('Ctrl Pts',(-0.0617614,1.651136808,-7.51081600900001));
#135252=CARTESIAN_POINT('Ctrl Pts',(-0.468606438,1.585954698,-7.485346218));
#135253=CARTESIAN_POINT('Ctrl Pts',(0.579082400613263,1.71660033198358,
-7.22684059819051));
#135254=CARTESIAN_POINT('Ctrl Pts',(0.575174885306631,1.71596185949179,
-7.22714945309525));
#135255=CARTESIAN_POINT('Ctrl Pts',(0.57126737,1.715323387,-7.22745830800001));
#135256=CARTESIAN_POINT('Ctrl Pts',(0.178439107,1.651136808,-7.258507946));
#135257=CARTESIAN_POINT('Ctrl Pts',(-0.215440326,1.585954698,-7.246798291));
#135258=CARTESIAN_POINT('',(-0.210730924768195,1.58673401520766,-7.24693676522288));
#135259=CARTESIAN_POINT('Origin',(0.02296298988262,1.48222898981416,0.192460243053221));
#135260=CARTESIAN_POINT('Ctrl Pts',(-0.220230577341825,1.62564958673025,
-7.49676586842819));
#135261=CARTESIAN_POINT('Ctrl Pts',(-0.219189274043533,1.62139779886349,
-7.46808025586321));
#135262=CARTESIAN_POINT('Ctrl Pts',(-0.218123345138537,1.6170784087238,
-7.43940545450373));
#135263=CARTESIAN_POINT('Ctrl Pts',(-0.217031104751607,1.61268792540798,
-7.41074263500274));
#135264=CARTESIAN_POINT('Ctrl Pts',(-0.215989923663357,1.60850268537158,
-7.38341972517653));
#135265=CARTESIAN_POINT('Ctrl Pts',(-0.21491874152865,1.60425381506126,
-7.3561076063082));
#135266=CARTESIAN_POINT('Ctrl Pts',(-0.21386546378962,1.59993003805682,
-7.32880674356716));
#135267=CARTESIAN_POINT('Ctrl Pts',(-0.212812156865946,1.59560614124741,
-7.3015051243628));
#135268=CARTESIAN_POINT('Ctrl Pts',(-0.211767154034744,1.59120881937963,
-7.27421470500947));
#135269=CARTESIAN_POINT('Ctrl Pts',(-0.21073092149889,1.58673401597724,
-7.24693676549605));
#135270=CARTESIAN_POINT('Ctrl Pts',(0.032863927,1.585967065,-7.499927997));
#135271=CARTESIAN_POINT('Ctrl Pts',(-0.03466743,1.59657582,-7.500223913));
#135272=CARTESIAN_POINT('Ctrl Pts',(-0.102193166,1.607142857,-7.499303738));
#135273=CARTESIAN_POINT('Ctrl Pts',(-0.444987886,1.660786473,-7.494632467));
#135274=CARTESIAN_POINT('Ctrl Pts',(-0.785926947,1.715323387,-7.458707585));
#135275=CARTESIAN_POINT('Ctrl Pts',(-0.790023188214287,1.71597862537067,
-7.4582759624636));
#135276=CARTESIAN_POINT('Ctrl Pts',(-0.794119429428574,1.71663386374134,
-7.4578443399272));
#135277=CARTESIAN_POINT('Ctrl Pts',(-0.206013131,1.585967065,-7.247072415));
#135278=CARTESIAN_POINT('Ctrl Pts',(-0.271267708,1.59657582,-7.245217418));
#135279=CARTESIAN_POINT('Ctrl Pts',(-0.336478302,1.607142857,-7.242187677));
#135280=CARTESIAN_POINT('Ctrl Pts',(-0.667520194,1.660786473,-7.226807185));
#135281=CARTESIAN_POINT('Ctrl Pts',(-0.995778438,1.715323387,-7.181289947));
#135282=CARTESIAN_POINT('Ctrl Pts',(-0.999722324464808,1.71597862537067,
-7.18074307629029));
#135283=CARTESIAN_POINT('Ctrl Pts',(-1.00366621092962,1.71663386374134,
-7.18019620558059));
#135284=CARTESIAN_POINT('Ctrl Pts',(-0.995778431195552,1.71532338603152,
-7.18128994909741));
#135285=CARTESIAN_POINT('Ctrl Pts',(-0.983007246198175,1.71320157786637,
-7.18306083844871));
#135286=CARTESIAN_POINT('Ctrl Pts',(-0.979077870701436,1.71254943790544,
-7.18359021791031));
#135287=CARTESIAN_POINT('Ctrl Pts',(-0.963113817753805,1.70989962936613,
-7.18574837665296));
#135288=CARTESIAN_POINT('Ctrl Pts',(-0.954943334809972,1.70854407406466,
-7.1868387477902));
#135289=CARTESIAN_POINT('Ctrl Pts',(-0.930432412067507,1.70447938487425,
-7.19006725398254));
#135290=CARTESIAN_POINT('Ctrl Pts',(-0.914086363547438,1.70177120844069,
-7.19216363292857));
#135291=CARTESIAN_POINT('Ctrl Pts',(-0.865052739460746,1.69365497349035,
-7.19828232285063));
#135292=CARTESIAN_POINT('Ctrl Pts',(-0.832344069660024,1.68825095321702,
-7.20213774575369));
#135293=CARTESIAN_POINT('Ctrl Pts',(-0.734255462670462,1.6720751508552,
-7.21302243439045));
#135294=CARTESIAN_POINT('Ctrl Pts',(-0.668801789500237,1.66132115804658,
-7.21938563741333));
#135295=CARTESIAN_POINT('Ctrl Pts',(-0.47258780643187,1.62920289831347,
-7.23576925835512));
#135296=CARTESIAN_POINT('Ctrl Pts',(-0.341742814072663,1.60803074768566,
-7.24312712082469));
#135297=CARTESIAN_POINT('Ctrl Pts',(-0.210730924864113,1.58673401470343,
-7.2469367657027));
#135298=CARTESIAN_POINT('Ctrl Pts',(-1.26520405425852,1.71660033198358,
-7.39251814139622));
#135299=CARTESIAN_POINT('Ctrl Pts',(-1.26920006462926,1.71596185949179,
-7.39182978969811));
#135300=CARTESIAN_POINT('Ctrl Pts',(-1.273196075,1.715323387,-7.39114143800001));
#135301=CARTESIAN_POINT('Ctrl Pts',(-1.674920877,1.651136808,-7.321940429));
#135302=CARTESIAN_POINT('Ctrl Pts',(-2.066778852,1.585954698,-7.209606451));
#135303=CARTESIAN_POINT('Ctrl Pts',(-0.988013329107109,1.71660033198358,
-7.18236667945575));
#135304=CARTESIAN_POINT('Ctrl Pts',(-0.991895883553554,1.71596185949179,
-7.18182831322788));
#135305=CARTESIAN_POINT('Ctrl Pts',(-0.995778438,1.715323387,-7.181289947));
#135306=CARTESIAN_POINT('Ctrl Pts',(-1.386097349,1.651136808,-7.12716719800001));
#135307=CARTESIAN_POINT('Ctrl Pts',(-1.76825087,1.585954698,-7.031058872));
#135308=CARTESIAN_POINT('',(-1.7636813391673,1.58673401524348,-7.0322064913939));
#135309=CARTESIAN_POINT('Origin',(0.0637993173099696,1.4822290083721,0.183023894089098));
#135310=CARTESIAN_POINT('Ctrl Pts',(-1.82666476776868,1.62564958678102,
-7.27415258436543));
#135311=CARTESIAN_POINT('Ctrl Pts',(-1.81948125070448,1.62139779891109,
-7.24636147483946));
#135312=CARTESIAN_POINT('Ctrl Pts',(-1.81227600790523,1.61707840876749,
-7.21858621756028));
#135313=CARTESIAN_POINT('Ctrl Pts',(-1.80504764454274,1.61268792544544,
-7.19082831818906));
#135314=CARTESIAN_POINT('Ctrl Pts',(-1.79815718774571,1.60850268542199,
-7.16436802603133));
#135315=CARTESIAN_POINT('Ctrl Pts',(-1.7912397511775,1.60425381510532,-7.13792472184617));
#135316=CARTESIAN_POINT('Ctrl Pts',(-1.7843422201044,1.59993003810657,-7.11148856171909));
#135317=CARTESIAN_POINT('Ctrl Pts',(-1.77744449791178,1.5956061413029,-7.08505166908843));
#135318=CARTESIAN_POINT('Ctrl Pts',(-1.77055729322817,1.59120881945812,
-7.05862392934178));
#135319=CARTESIAN_POINT('Ctrl Pts',(-1.7636813350497,1.58673401625577,-7.03220649222103));
#135320=CARTESIAN_POINT('Ctrl Pts',(-1.580167237,1.585967065,-7.331648621));
#135321=CARTESIAN_POINT('Ctrl Pts',(-1.646183361,1.59657582,-7.317420373));
#135322=CARTESIAN_POINT('Ctrl Pts',(-1.711932572,1.607142857,-7.302005674));
#135323=CARTESIAN_POINT('Ctrl Pts',(-2.045708757,1.660786473,-7.223752884));
#135324=CARTESIAN_POINT('Ctrl Pts',(-2.370954065,1.715323387,-7.115376084));
#135325=CARTESIAN_POINT('Ctrl Pts',(-2.37486175229012,1.71597862537066,
-7.11407398176059));
#135326=CARTESIAN_POINT('Ctrl Pts',(-2.37876943958024,1.71663386374133,
-7.11277187952119));
#135327=CARTESIAN_POINT('Ctrl Pts',(-1.759103005,1.585967065,-7.033353156));
#135328=CARTESIAN_POINT('Ctrl Pts',(-1.822433198,1.59657582,-7.017513722));
#135329=CARTESIAN_POINT('Ctrl Pts',(-1.885467899,1.607142857,-7.000536465));
#135330=CARTESIAN_POINT('Ctrl Pts',(-2.205463864,1.660786473,-6.914351339));
#135331=CARTESIAN_POINT('Ctrl Pts',(-2.516262752,1.715323387,-6.79933245));
#135332=CARTESIAN_POINT('Ctrl Pts',(-2.51999687155391,1.71597862537066,
-6.79795054581994));
#135333=CARTESIAN_POINT('Ctrl Pts',(-2.52373099110783,1.71663386374133,
-6.79656864163989));
#135334=CARTESIAN_POINT('Ctrl Pts',(-2.5162627369183,1.71532338435357,-6.79933245558136));
#135335=CARTESIAN_POINT('Ctrl Pts',(-2.37664964043737,1.69082501025532,
-6.85099976765249));
#135336=CARTESIAN_POINT('Ctrl Pts',(-2.23573125128583,1.66647816528029,
-6.89825663970194));
#135337=CARTESIAN_POINT('Ctrl Pts',(-2.09392556770815,1.64234941096584,
-6.94103563718671));
#135338=CARTESIAN_POINT('Ctrl Pts',(-2.02463516259193,1.63055939579003,
-6.96193870673513));
#135339=CARTESIAN_POINT('Ctrl Pts',(-1.95513298040099,1.61882140076076,
-6.98177343537018));
#135340=CARTESIAN_POINT('Ctrl Pts',(-1.88546789921594,1.60714285706073,
-7.00053646515667));
#135341=CARTESIAN_POINT('Ctrl Pts',(-1.84500356901233,1.60035948112099,
-7.01143480091374));
#135342=CARTESIAN_POINT('Ctrl Pts',(-1.80440519902882,1.59355605149649,
-7.0219929241046));
#135343=CARTESIAN_POINT('Ctrl Pts',(-1.76368133918351,1.58673401465524,
-7.03220649106564));
#135344=CARTESIAN_POINT('Ctrl Pts',(-2.82479716579741,1.71660033198358,
-6.94770370202509));
#135345=CARTESIAN_POINT('Ctrl Pts',(-2.8285517763987,1.71596185949179,-6.94617241951255));
#135346=CARTESIAN_POINT('Ctrl Pts',(-2.832306387,1.715323387,-6.944641137));
#135347=CARTESIAN_POINT('Ctrl Pts',(-3.209762915,1.651136808,-6.790699053));
#135348=CARTESIAN_POINT('Ctrl Pts',(-3.568310983,1.585954698,-6.596753499));
#135349=CARTESIAN_POINT('Ctrl Pts',(-2.50891065267966,1.71660033198358,
-6.80205327793971));
#135350=CARTESIAN_POINT('Ctrl Pts',(-2.51258670233983,1.71596185949179,
-6.80069286396985));
#135351=CARTESIAN_POINT('Ctrl Pts',(-2.516262752,1.715323387,-6.79933245));
#135352=CARTESIAN_POINT('Ctrl Pts',(-2.885821433,1.651136808,-6.662568032));
#135353=CARTESIAN_POINT('Ctrl Pts',(-3.238379968,1.585954698,-6.486554955));
#135354=CARTESIAN_POINT('',(-3.23416397512505,1.58673401528033,-6.48865805732195));
#135355=CARTESIAN_POINT('Origin',(0.101652530209534,1.48222898518188,0.16503009862893));
#135356=CARTESIAN_POINT('Ctrl Pts',(-3.3476861436547,1.62564958677245,-6.71140801016537));
#135357=CARTESIAN_POINT('Ctrl Pts',(-3.33469630621779,1.62139779889616,
-6.68581088513764));
#135358=CARTESIAN_POINT('Ctrl Pts',(-3.32168865877955,1.61707840874773,
-6.66023391214072));
#135359=CARTESIAN_POINT('Ctrl Pts',(-3.30866216274858,1.6126879254223,-6.63467886147285));
#135360=CARTESIAN_POINT('Ctrl Pts',(-3.29624462038393,1.60850268538805,
-6.61031844071623));
#135361=CARTESIAN_POINT('Ctrl Pts',(-3.28380438072982,1.6042538150954,-6.58598041070878));
#135362=CARTESIAN_POINT('Ctrl Pts',(-3.27138511704215,1.59993003810284,
-6.56164507859974));
#135363=CARTESIAN_POINT('Ctrl Pts',(-3.2589655092365,1.59560614130533,-6.53730907219748));
#135364=CARTESIAN_POINT('Ctrl Pts',(-3.24655814078463,1.59120881943997,
-6.51297974367117));
#135365=CARTESIAN_POINT('Ctrl Pts',(-3.2341639711417,1.58673401616681,-6.48865805919337));
#135366=CARTESIAN_POINT('Ctrl Pts',(-3.119311536,1.585967065,-6.820549504));
#135367=CARTESIAN_POINT('Ctrl Pts',(-3.180725587,1.59657582,-6.792462389));
#135368=CARTESIAN_POINT('Ctrl Pts',(-3.241623914,1.607142857,-6.763273941));
#135369=CARTESIAN_POINT('Ctrl Pts',(-3.55077456,1.660786473,-6.615098643));
#135370=CARTESIAN_POINT('Ctrl Pts',(-3.845118005,1.715323387,-6.439337507));
#135371=CARTESIAN_POINT('Ctrl Pts',(-3.84865441924078,1.71597862537066,
-6.43722580995057));
#135372=CARTESIAN_POINT('Ctrl Pts',(-3.85219083348155,1.71663386374133,
-6.43511411290114));
#135373=CARTESIAN_POINT('Ctrl Pts',(-3.229939179,1.585967065,-6.49076212));
#135374=CARTESIAN_POINT('Ctrl Pts',(-3.288383736,1.59657582,-6.461678884));
#135375=CARTESIAN_POINT('Ctrl Pts',(-3.346295113,1.607142857,-6.431547949));
#135376=CARTESIAN_POINT('Ctrl Pts',(-3.640282496,1.660786473,-6.278588109));
#135377=CARTESIAN_POINT('Ctrl Pts',(-3.919089417,1.715323387,-6.09944572399999));
#135378=CARTESIAN_POINT('Ctrl Pts',(-3.92243916635777,1.71597862537066,
-6.09729340264818));
#135379=CARTESIAN_POINT('Ctrl Pts',(-3.92578891571553,1.71663386374133,
-6.09514108129637));
#135380=CARTESIAN_POINT('Ctrl Pts',(-3.9190894113225,1.71532338611378,-6.09944572779726));
#135381=CARTESIAN_POINT('Ctrl Pts',(-3.79384736364693,1.69082501703781,
-6.17991775846372));
#135382=CARTESIAN_POINT('Ctrl Pts',(-3.66638243065307,1.66647817789189,
-6.25636306151695));
#135383=CARTESIAN_POINT('Ctrl Pts',(-3.53708834177104,1.64234943014875,
-6.32862592241045));
#135384=CARTESIAN_POINT('Ctrl Pts',(-3.47391141500436,1.63055940832857,
-6.36393569960209));
#135385=CARTESIAN_POINT('Ctrl Pts',(-3.41029800108025,1.61882140691879,
-6.39824763726708));
#135386=CARTESIAN_POINT('Ctrl Pts',(-3.34629511360955,1.60714285711122,
-6.43154794868285));
#135387=CARTESIAN_POINT('Ctrl Pts',(-3.30911963545218,1.60035948098744,
-6.45089012269899));
#135388=CARTESIAN_POINT('Ctrl Pts',(-3.2717401159293,1.5935560511928,-6.46992885310997));
#135389=CARTESIAN_POINT('Ctrl Pts',(-3.234163976,1.586734015,-6.488658057));
#135390=CARTESIAN_POINT('Ctrl Pts',(-4.25230590117908,1.71660033198358,
-6.17802236055207));
#135391=CARTESIAN_POINT('Ctrl Pts',(-4.25564355058954,1.71596185949179,
-6.17571974827603));
#135392=CARTESIAN_POINT('Ctrl Pts',(-4.2589812,1.715323387,-6.173417136));
#135393=CARTESIAN_POINT('Ctrl Pts',(-4.594520006,1.651136808,-5.941932136));
#135394=CARTESIAN_POINT('Ctrl Pts',(-4.90299285900001,1.585954698,-5.675443685));
#135395=CARTESIAN_POINT('Ctrl Pts',(-3.91249410326131,1.71660033198358,
-6.10368342451692));
#135396=CARTESIAN_POINT('Ctrl Pts',(-3.91579176013065,1.71596185949179,
-6.10156457425846));
#135397=CARTESIAN_POINT('Ctrl Pts',(-3.919089417,1.715323387,-6.09944572400001));
#135398=CARTESIAN_POINT('Ctrl Pts',(-4.250607714,1.651136808,-5.88643459));
#135399=CARTESIAN_POINT('Ctrl Pts',(-4.55708601800001,1.585954698,-5.63874693700001));
#135400=CARTESIAN_POINT('',(-4.55342069719549,1.58673401524202,-5.64170718400532));
#135401=CARTESIAN_POINT('Origin',(0.134752473701915,1.48222900232617,0.139319403200179));
#135402=CARTESIAN_POINT('Ctrl Pts',(-4.71217343650642,1.62564958679273,
-5.83484545654915));
#135403=CARTESIAN_POINT('Ctrl Pts',(-4.69398466915291,1.62139779886915,
-5.81263920890564));
#135404=CARTESIAN_POINT('Ctrl Pts',(-4.67578284009688,1.61707840871869,
-5.79045647096182));
#135405=CARTESIAN_POINT('Ctrl Pts',(-4.65756731577416,1.61268792538905,
-5.76829919469481));
#135406=CARTESIAN_POINT('Ctrl Pts',(-4.64020331825134,1.60850268535374,
-5.74717771153594));
#135407=CARTESIAN_POINT('Ctrl Pts',(-4.62282196747897,1.60425381505011,
-5.72608297484968));
#135408=CARTESIAN_POINT('Ctrl Pts',(-4.60546168216947,1.59993003806062,
-5.7049863638248));
#135409=CARTESIAN_POINT('Ctrl Pts',(-4.58810091583422,1.59560614126618,
-5.68388916824656));
#135410=CARTESIAN_POINT('Ctrl Pts',(-4.57075353820189,1.59120881941508,
-5.66279586335943));
#135411=CARTESIAN_POINT('Ctrl Pts',(-4.55342069426911,1.58673401611734,
-5.64170718630423));
#135412=CARTESIAN_POINT('Ctrl Pts',(-4.512600295,1.585967065,-5.99052907300001));
#135413=CARTESIAN_POINT('Ctrl Pts',(-4.566540621,1.59657582,-5.949896413));
#135414=CARTESIAN_POINT('Ctrl Pts',(-4.619740525,1.607142857,-5.908299035));
#135415=CARTESIAN_POINT('Ctrl Pts',(-4.889810092,1.660786473,-5.697129743));
#135416=CARTESIAN_POINT('Ctrl Pts',(-5.139488502,1.715323387,-5.462202664));
#135417=CARTESIAN_POINT('Ctrl Pts',(-5.14248828439617,1.71597862537066,
-5.45938011271906));
#135418=CARTESIAN_POINT('Ctrl Pts',(-5.14548806679234,1.71663386374133,
-5.45655756143813));
#135419=CARTESIAN_POINT('Ctrl Pts',(-4.549746986,1.585967065,-5.644670262));
#135420=CARTESIAN_POINT('Ctrl Pts',(-4.600573106,1.59657582,-5.603703124));
#135421=CARTESIAN_POINT('Ctrl Pts',(-4.650653287,1.607142857,-5.561827398));
#135422=CARTESIAN_POINT('Ctrl Pts',(-4.904885564,1.660786473,-5.349245077));
#135423=CARTESIAN_POINT('Ctrl Pts',(-5.138663817,1.715323387,-5.114355695));
#135424=CARTESIAN_POINT('Ctrl Pts',(-5.14147256561369,1.71597862537066,
-5.11153359663286));
#135425=CARTESIAN_POINT('Ctrl Pts',(-5.14428131422739,1.71663386374133,
-5.10871149826573));
#135426=CARTESIAN_POINT('Ctrl Pts',(-5.13866380557472,1.71532338433466,
-5.11435570647959));
#135427=CARTESIAN_POINT('Ctrl Pts',(-5.03364892658114,1.69082500890268,
-5.21986971217025));
#135428=CARTESIAN_POINT('Ctrl Pts',(-4.92559750013,1.66647816264222,-5.3219289887372));
#135429=CARTESIAN_POINT('Ctrl Pts',(-4.81486057615405,1.6423494070885,-5.42029682131852));
#135430=CARTESIAN_POINT('Ctrl Pts',(-4.76075128450724,1.63055939320285,
-5.46836221405928));
#135431=CARTESIAN_POINT('Ctrl Pts',(-4.70600120464847,1.61882139945801,
-5.5155469299307));
#135432=CARTESIAN_POINT('Ctrl Pts',(-4.6506532871449,1.60714285703281,-5.56182739798854));
#135433=CARTESIAN_POINT('Ctrl Pts',(-4.61850494796888,1.60035948119918,
-5.58870899100399));
#135434=CARTESIAN_POINT('Ctrl Pts',(-4.58609210673901,1.59355605171779,
-5.61533809689503));
#135435=CARTESIAN_POINT('Ctrl Pts',(-4.55342069759857,1.58673401469568,
-5.64170718436339));
#135436=CARTESIAN_POINT('Ctrl Pts',(-5.48098153912164,1.71660033198358,
-5.11946355990375));
#135437=CARTESIAN_POINT('Ctrl Pts',(-5.48374616256082,1.71596185949179,
-5.11649728545188));
#135438=CARTESIAN_POINT('Ctrl Pts',(-5.486510786,1.715323387,-5.113531011));
#135439=CARTESIAN_POINT('Ctrl Pts',(-5.76444244800001,1.651136808,-4.815327076));
#135440=CARTESIAN_POINT('Ctrl Pts',(-6.008416238,1.585954698,-4.488756433));
#135441=CARTESIAN_POINT('Ctrl Pts',(-5.13313367838099,1.71660033198358,
-5.11991211792546));
#135442=CARTESIAN_POINT('Ctrl Pts',(-5.13589874769049,1.71596185949179,
-5.11713390646273));
#135443=CARTESIAN_POINT('Ctrl Pts',(-5.13866381700001,1.715323387,-5.114355695));
#135444=CARTESIAN_POINT('Ctrl Pts',(-5.416640303,1.651136808,-4.835058009));
#135445=CARTESIAN_POINT('Ctrl Pts',(-5.662707791,1.585954698,-4.52727738));
#135446=CARTESIAN_POINT('',(-5.65976452852026,1.58673401523511,-4.53095635414236));
#135447=CARTESIAN_POINT('Origin',(0.161551673038854,1.48222901763502,0.107094477920148));
#135448=CARTESIAN_POINT('Ctrl Pts',(-5.85632473635433,1.62564958674453,
-4.68545201425031));
#135449=CARTESIAN_POINT('Ctrl Pts',(-5.83378752536501,1.62139779883973,
-4.66767498378072));
#135450=CARTESIAN_POINT('Ctrl Pts',(-5.81124261200344,1.61707840867752,
-4.64992372110351));
#135451=CARTESIAN_POINT('Ctrl Pts',(-5.78868979708449,1.61268792533566,
-4.63220026889469));
#135452=CARTESIAN_POINT('Ctrl Pts',(-5.76719126574319,1.6085026853083,-4.61530534051628));
#135453=CARTESIAN_POINT('Ctrl Pts',(-5.74568153657526,1.60425381501317,
-4.59844026372362));
#135454=CARTESIAN_POINT('Ctrl Pts',(-5.72419197744197,1.5999300380356,-4.5815688279632));
#135455=CARTESIAN_POINT('Ctrl Pts',(-5.70270182286744,1.59560614125309,
-4.56469692472233));
#135456=CARTESIAN_POINT('Ctrl Pts',(-5.68122558035585,1.59120881941638,
-4.54782594303467));
#135457=CARTESIAN_POINT('Ctrl Pts',(-5.65976452599462,1.58673401627607,
-4.53095635732274));
#135458=CARTESIAN_POINT('Ctrl Pts',(-5.69488488000001,1.585967065,-4.88039816));
#135459=CARTESIAN_POINT('Ctrl Pts',(-5.73882929,1.59657582,-4.82911989400001));
#135460=CARTESIAN_POINT('Ctrl Pts',(-5.781843203,1.607142857,-4.777058632));
#135461=CARTESIAN_POINT('Ctrl Pts',(-6.000203538,1.660786473,-4.512769388));
#135462=CARTESIAN_POINT('Ctrl Pts',(-6.193542228,1.715323387,-4.229661295));
#135463=CARTESIAN_POINT('Ctrl Pts',(-6.19586511206018,1.71597862537066,
-4.22625986884708));
#135464=CARTESIAN_POINT('Ctrl Pts',(-6.19818799612036,1.71663386374133,
-4.22285844269416));
#135465=CARTESIAN_POINT('Ctrl Pts',(-5.656813681,1.585967065,-4.53463989500001));
#135466=CARTESIAN_POINT('Ctrl Pts',(-5.697644791,1.59657582,-4.483704433));
#135467=CARTESIAN_POINT('Ctrl Pts',(-5.737552082,1.607142857,-4.43204198));
#135468=CARTESIAN_POINT('Ctrl Pts',(-5.940141634,1.660786473,-4.169777291));
#135469=CARTESIAN_POINT('Ctrl Pts',(-6.117960008,1.715323387,-3.890124078));
#135470=CARTESIAN_POINT('Ctrl Pts',(-6.12009642190956,1.71597862537066,
-3.88676416079535));
#135471=CARTESIAN_POINT('Ctrl Pts',(-6.12223283581911,1.71663386374133,
-3.8834042435907));
#135472=CARTESIAN_POINT('Ctrl Pts',(-6.11795999903966,1.71532338425187,
-3.89012409209184));
#135473=CARTESIAN_POINT('Ctrl Pts',(-6.0380827030761,1.69082500927857,-4.01574633149173));
#135474=CARTESIAN_POINT('Ctrl Pts',(-5.95449718812239,1.66647816346924,
-4.13864737958845));
#135475=CARTESIAN_POINT('Ctrl Pts',(-5.86749540988425,1.64234940833118,
-4.25852059023017));
#135476=CARTESIAN_POINT('Ctrl Pts',(-5.8249838006051,1.6305593940166,-4.31709414122001));
#135477=CARTESIAN_POINT('Ctrl Pts',(-5.78165706483856,1.61882139983996,
-4.37494535553091));
#135478=CARTESIAN_POINT('Ctrl Pts',(-5.73755208192497,1.60714285697828,
-4.43204198016065));
#135479=CARTESIAN_POINT('Ctrl Pts',(-5.71193410050092,1.60035948104102,
-4.46520603929647));
#135480=CARTESIAN_POINT('Ctrl Pts',(-5.68600352387605,1.59355605151279,
-4.49818037433353));
#135481=CARTESIAN_POINT('Ctrl Pts',(-5.6597645284826,1.58673401451738,-4.53095635396281));
#135482=CARTESIAN_POINT('Ctrl Pts',(-6.45337257147076,1.71660033198358,
-3.82152433181392));
#135483=CARTESIAN_POINT('Ctrl Pts',(-6.45543489823538,1.71596185949179,
-3.81803309490696));
#135484=CARTESIAN_POINT('Ctrl Pts',(-6.457497225,1.715323387,-3.814541858));
#135485=CARTESIAN_POINT('Ctrl Pts',(-6.664825969,1.651136808,-3.463562675));
#135486=CARTESIAN_POINT('Ctrl Pts',(-6.832892752,1.585954698,-3.092179918));
#135487=CARTESIAN_POINT('Ctrl Pts',(-6.1137536276454,1.71660033198358,-3.8967394111811));
#135488=CARTESIAN_POINT('Ctrl Pts',(-6.11585681782271,1.71596185949179,
-3.89343174459055));
#135489=CARTESIAN_POINT('Ctrl Pts',(-6.117960008,1.715323387,-3.890124078));
#135490=CARTESIAN_POINT('Ctrl Pts',(-6.329396811,1.651136808,-3.557599489));
#135491=CARTESIAN_POINT('Ctrl Pts',(-6.503547641,1.585954698,-3.204117364));
#135492=CARTESIAN_POINT('',(-6.50146406149294,1.58673401531619,-3.20834303967259));
#135493=CARTESIAN_POINT('Origin',(0.180796891847448,1.48222900349585,0.0698618628709807));
#135494=CARTESIAN_POINT('Ctrl Pts',(-6.72664080068503,1.625649586757,-3.31697204352363));
#135495=CARTESIAN_POINT('Ctrl Pts',(-6.70080896102677,1.6213977988843,-3.3044554644234));
#135496=CARTESIAN_POINT('Ctrl Pts',(-6.67497513854352,1.61707840873839,
-3.29196570633431));
#135497=CARTESIAN_POINT('Ctrl Pts',(-6.64913957764186,1.61268792541326,
-3.27950480713941));
#135498=CARTESIAN_POINT('Ctrl Pts',(-6.62451175980181,1.60850268538798,
-3.26762642150408));
#135499=CARTESIAN_POINT('Ctrl Pts',(-6.59987942312048,1.60425381509443,
-3.25577959675733));
#135500=CARTESIAN_POINT('Ctrl Pts',(-6.57526541791268,1.59993003811615,
-3.24392222576583));
#135501=CARTESIAN_POINT('Ctrl Pts',(-6.5506507306901,1.59560614133292,-3.2320645262255));
#135502=CARTESIAN_POINT('Ctrl Pts',(-6.52604982838255,1.59120881949136,
-3.22020473601114));
#135503=CARTESIAN_POINT('Ctrl Pts',(-6.50146405949292,1.58673401619063,
-3.20834304338622));
#135504=CARTESIAN_POINT('Ctrl Pts',(-6.610882977,1.585967065,-3.542065254));
#135505=CARTESIAN_POINT('Ctrl Pts',(-6.64277668,1.59657582,-3.482539096));
#135506=CARTESIAN_POINT('Ctrl Pts',(-6.673593319,1.607142857,-3.422448278));
#135507=CARTESIAN_POINT('Ctrl Pts',(-6.830034135,1.660786473,-3.117396951));
#135508=CARTESIAN_POINT('Ctrl Pts',(-6.957992803,1.715323387,-2.799345666));
#135509=CARTESIAN_POINT('Ctrl Pts',(-6.95953017325041,1.71597862537066,
-2.7955244119083));
#135510=CARTESIAN_POINT('Ctrl Pts',(-6.96106754350082,1.71663386374133,
-2.7917031578166));
#135511=CARTESIAN_POINT('Ctrl Pts',(-6.499374055,1.585967065,-3.212574807));
#135512=CARTESIAN_POINT('Ctrl Pts',(-6.528300937,1.59657582,-3.154052706));
#135513=CARTESIAN_POINT('Ctrl Pts',(-6.556169318,1.607142857,-3.095019205));
#135514=CARTESIAN_POINT('Ctrl Pts',(-6.697643284,1.660786473,-2.795335353));
#135515=CARTESIAN_POINT('Ctrl Pts',(-6.811187188,1.715323387,-2.483994583));
#135516=CARTESIAN_POINT('Ctrl Pts',(-6.81255137084789,1.71597862537066,
-2.48025395295892));
#135517=CARTESIAN_POINT('Ctrl Pts',(-6.81391555369579,1.71663386374133,
-2.47651332291784));
#135518=CARTESIAN_POINT('Ctrl Pts',(-6.81118718586599,1.71532338609523,
-2.483994589877));
#135519=CARTESIAN_POINT('Ctrl Pts',(-6.7601824533748,1.69082501482219,-2.62385108575496));
#135520=CARTESIAN_POINT('Ctrl Pts',(-6.70497122496998,1.66647817350564,
-2.76184716434788));
#135521=CARTESIAN_POINT('Ctrl Pts',(-6.64577271151913,1.64234942362513,
-2.8976205874493));
#135522=CARTESIAN_POINT('Ctrl Pts',(-6.61684656990636,1.63055940398956,
-2.96396349092682));
#135523=CARTESIAN_POINT('Ctrl Pts',(-6.58696907752558,1.6188214047438,-3.02977617227563));
#135524=CARTESIAN_POINT('Ctrl Pts',(-6.55616931819621,1.6071428570744,-3.09501920458437));
#135525=CARTESIAN_POINT('Ctrl Pts',(-6.53827956256854,1.60035948094352,
-3.13291501639681));
#135526=CARTESIAN_POINT('Ctrl Pts',(-6.52004373512448,1.59355605121258,
-3.17069273876414));
#135527=CARTESIAN_POINT('Ctrl Pts',(-6.501464062,1.586734015,-3.208343039));
#135528=CARTESIAN_POINT('Ctrl Pts',(-7.12401107506173,1.71660033198358,
-2.34489487403908));
#135529=CARTESIAN_POINT('Ctrl Pts',(-7.12527467303087,1.71596185949179,
-2.34104192101954));
#135530=CARTESIAN_POINT('Ctrl Pts',(-7.126538271,1.715323387,-2.337188968));
#135531=CARTESIAN_POINT('Ctrl Pts',(-7.253569634,1.651136808,-1.949845932));
#135532=CARTESIAN_POINT('Ctrl Pts',(-7.337870794,1.585954698,-1.551016507));
#135533=CARTESIAN_POINT('Ctrl Pts',(-6.80850125154208,1.71660033198358,
-2.49135950079383));
#135534=CARTESIAN_POINT('Ctrl Pts',(-6.80984421977104,1.71596185949179,
-2.48767704189691));
#135535=CARTESIAN_POINT('Ctrl Pts',(-6.811187188,1.715323387,-2.483994583));
#135536=CARTESIAN_POINT('Ctrl Pts',(-6.94619776,1.651136808,-2.113791572));
#135537=CARTESIAN_POINT('Ctrl Pts',(-7.040288831,1.585954698,-1.731136382));
#135538=CARTESIAN_POINT('',(-7.03916235977438,1.5867340151941,-1.73571117135257));
#135539=CARTESIAN_POINT('Origin',(0.191587870767866,1.48222903349934,0.0293624495522038));
#135540=CARTESIAN_POINT('Ctrl Pts',(-7.28242661707383,1.62564958676879,
-1.79339414618027));
#135541=CARTESIAN_POINT('Ctrl Pts',(-7.25450801706566,1.62139779883678,
-1.78672327941274));
#135542=CARTESIAN_POINT('Ctrl Pts',(-7.22659324614458,1.61707840868643,
-1.78007903323404));
#135543=CARTESIAN_POINT('Ctrl Pts',(-7.19868298126379,1.61268792535802,
-1.77346334495163));
#135544=CARTESIAN_POINT('Ctrl Pts',(-7.17207744626429,1.60850268532689,
-1.7671569223184));
#135545=CARTESIAN_POINT('Ctrl Pts',(-7.14547428273646,1.60425381502804,
-1.76088229411126));
#135546=CARTESIAN_POINT('Ctrl Pts',(-7.11888675499135,1.59993003803373,
-1.75459342542346));
#135547=CARTESIAN_POINT('Ctrl Pts',(-7.09229849054833,1.59560614123448,
-1.74830438248116));
#135548=CARTESIAN_POINT('Ctrl Pts',(-7.0657232393096,1.59120881937443,-1.74201033436875));
#135549=CARTESIAN_POINT('Ctrl Pts',(-7.03916235886331,1.58673401603955,
-1.73571117489813));
#135550=CARTESIAN_POINT('Ctrl Pts',(-7.21776353400001,1.585967065,-2.038109313));
#135551=CARTESIAN_POINT('Ctrl Pts',(-7.236115215,1.59657582,-1.97311864));
#135552=CARTESIAN_POINT('Ctrl Pts',(-7.253293629,1.607142857,-1.907808045));
#135553=CARTESIAN_POINT('Ctrl Pts',(-7.340499928,1.660786473,-1.576258498));
#135554=CARTESIAN_POINT('Ctrl Pts',(-7.397095368,1.715323387,-1.238135744));
#135555=CARTESIAN_POINT('Ctrl Pts',(-7.39777533870557,1.71597862537066,
-1.23407333954463));
#135556=CARTESIAN_POINT('Ctrl Pts',(-7.39845530941115,1.71663386374133,
-1.23001093508926));
#135557=CARTESIAN_POINT('Ctrl Pts',(-7.038030922,1.585967065,-1.740293292));
#135558=CARTESIAN_POINT('Ctrl Pts',(-7.053700988,1.59657582,-1.67692098));
#135559=CARTESIAN_POINT('Ctrl Pts',(-7.068227363,1.607142857,-1.613276771));
#135560=CARTESIAN_POINT('Ctrl Pts',(-7.141970577,1.660786473,-1.290186641));
#135561=CARTESIAN_POINT('Ctrl Pts',(-7.185930826,1.715323387,-0.961716262));
#135562=CARTESIAN_POINT('Ctrl Pts',(-7.18645899013354,1.71597862537066,
-0.957769826821296));
#135563=CARTESIAN_POINT('Ctrl Pts',(-7.18698715426708,1.71663386374133,
-0.953823391642592));
#135564=CARTESIAN_POINT('Ctrl Pts',(-7.18593082383186,1.7153233843102,-0.96171627820039));
#135565=CARTESIAN_POINT('Ctrl Pts',(-7.16618356659928,1.69082501418126,
-1.10926751150146));
#135566=CARTESIAN_POINT('Ctrl Pts',(-7.14192822398185,1.66647817310497,
-1.25590609992664));
#135567=CARTESIAN_POINT('Ctrl Pts',(-7.11330101035654,1.64234942258282,
-1.40123115002223));
#135568=CARTESIAN_POINT('Ctrl Pts',(-7.09931290954574,1.63055940350657,
-1.47224125522062));
#135569=CARTESIAN_POINT('Ctrl Pts',(-7.08428171779415,1.61882140460229,
-1.54293804795029));
#135570=CARTESIAN_POINT('Ctrl Pts',(-7.06822736322912,1.60714285705965,
-1.61327677087489));
#135571=CARTESIAN_POINT('Ctrl Pts',(-7.05890234030263,1.60035948115203,
-1.65413236680542));
#135572=CARTESIAN_POINT('Ctrl Pts',(-7.04921395033693,1.59355605159159,
-1.69494702943989));
#135573=CARTESIAN_POINT('Ctrl Pts',(-7.03916236003226,1.58673401462371,
-1.7357111713207));
#135574=CARTESIAN_POINT('Ctrl Pts',(-7.46153873851908,1.71660033198358,
-0.758620738679522));
#135575=CARTESIAN_POINT('Ctrl Pts',(-7.46194452325954,1.71596185949179,
-0.754586229339761));
#135576=CARTESIAN_POINT('Ctrl Pts',(-7.462350308,1.715323387,-0.75055172));
#135577=CARTESIAN_POINT('Ctrl Pts',(-7.503144445,1.651136808,-0.34495656));
#135578=CARTESIAN_POINT('Ctrl Pts',(-7.49973815400001,1.585954698,0.062670712));
#135579=CARTESIAN_POINT('Ctrl Pts',(-7.18489092487628,1.71660033198358,
-0.969486389062758));
#135580=CARTESIAN_POINT('Ctrl Pts',(-7.18541087543814,1.71596185949179,
-0.965601325531379));
#135581=CARTESIAN_POINT('Ctrl Pts',(-7.185930826,1.715323387,-0.961716262));
#135582=CARTESIAN_POINT('Ctrl Pts',(-7.23820222100001,1.651136808,-0.571145109));
#135583=CARTESIAN_POINT('Ctrl Pts',(-7.247833941,1.585954698,-0.177209386));
#135584=CARTESIAN_POINT('',(-7.24771725026763,1.58673401517814,-0.18191937719729));
#135585=CARTESIAN_POINT('Origin',(0.193420936396731,1.48222900303388,-0.0125097447096686));
#135586=CARTESIAN_POINT('Ctrl Pts',(-7.49769425876711,1.62564958680033,
-0.185959131992468));
#135587=CARTESIAN_POINT('Ctrl Pts',(-7.46899434096227,1.62139779886003,
-0.185445900051847));
#135588=CARTESIAN_POINT('Ctrl Pts',(-7.4403038853534,1.61707840871034,-0.184957843259731));
#135589=CARTESIAN_POINT('Ctrl Pts',(-7.41162396954117,1.61268792538127,
-0.184496708034791));
#135590=CARTESIAN_POINT('Ctrl Pts',(-7.38428476270878,1.60850268534733,
-0.184057129642196));
#135591=CARTESIAN_POINT('Ctrl Pts',(-7.35695470676653,1.60425381504928,
-0.183648092577493));
#135592=CARTESIAN_POINT('Ctrl Pts',(-7.32963685977038,1.5999300380482,-0.183221786703882));
#135593=CARTESIAN_POINT('Ctrl Pts',(-7.30231825584026,1.59560614124216,
-0.182795469018011));
#135594=CARTESIAN_POINT('Ctrl Pts',(-7.27501128491269,1.59120881936851,
-0.18236146569843));
#135595=CARTESIAN_POINT('Ctrl Pts',(-7.24771725040738,1.58673401593797,
-0.18191938037661));
#135596=CARTESIAN_POINT('Ctrl Pts',(-7.487149489,1.585967065,-0.438853645));
#135597=CARTESIAN_POINT('Ctrl Pts',(-7.491101045,1.59657582,-0.37143735));
#135598=CARTESIAN_POINT('Ctrl Pts',(-7.49383799,1.607142857,-0.303960829));
#135599=CARTESIAN_POINT('Ctrl Pts',(-7.507732102,1.660786473,0.038584051));
#135600=CARTESIAN_POINT('Ctrl Pts',(-7.49031797500001,1.715323387,0.38096803));
#135601=CARTESIAN_POINT('Ctrl Pts',(-7.49010875149683,1.71597862537053,
0.385081631303059));
#135602=CARTESIAN_POINT('Ctrl Pts',(-7.48989952799365,1.71663386374106,
0.389195232606118));
#135603=CARTESIAN_POINT('Ctrl Pts',(-7.247597285,1.585967065,-0.186637596));
#135604=CARTESIAN_POINT('Ctrl Pts',(-7.24927782,1.59657582,-0.121378293));
#135605=CARTESIAN_POINT('Ctrl Pts',(-7.249782953,1.607142857,-0.056099309));
#135606=CARTESIAN_POINT('Ctrl Pts',(-7.252347264,1.660786473,0.275289765));
#135607=CARTESIAN_POINT('Ctrl Pts',(-7.224668324,1.715323387,0.605530844));
#135608=CARTESIAN_POINT('Ctrl Pts',(-7.22433577303198,1.71597862537053,
0.609498553402951));
#135609=CARTESIAN_POINT('Ctrl Pts',(-7.22400322206396,1.71663386374106,
0.613466262805901));
#135610=CARTESIAN_POINT('Ctrl Pts',(-7.2246683254307,1.71532338418104,0.605530826930147));
#135611=CARTESIAN_POINT('Ctrl Pts',(-7.23710190400368,1.69082501017366,
0.457184159018169));
#135612=CARTESIAN_POINT('Ctrl Pts',(-7.24493660034943,1.66647816530689,
0.308759694131952));
#135613=CARTESIAN_POINT('Ctrl Pts',(-7.24821926433237,1.64234941111953,
0.160678235119607));
#135614=CARTESIAN_POINT('Ctrl Pts',(-7.24982326999497,1.63055939589135,
0.0883213018436355));
#135615=CARTESIAN_POINT('Ctrl Pts',(-7.25034121939894,1.6188214008152,0.016046122256376));
#135616=CARTESIAN_POINT('Ctrl Pts',(-7.24978295328257,1.60714285707412,
-0.0560993088255138));
#135617=CARTESIAN_POINT('Ctrl Pts',(-7.24945868958999,1.60035948119099,
-0.0980043278327279));
#135618=CARTESIAN_POINT('Ctrl Pts',(-7.24877075450675,1.59355605165188,
-0.139947483342351));
#135619=CARTESIAN_POINT('Ctrl Pts',(-7.24771725015678,1.58673401461714,
-0.181919377103323));
#135620=CARTESIAN_POINT('Ctrl Pts',(-7.45017314305326,1.71660033198358,
0.863125660047407));
#135621=CARTESIAN_POINT('Ctrl Pts',(-7.44970214052664,1.71596185949179,
0.867153076523704));
#135622=CARTESIAN_POINT('Ctrl Pts',(-7.449231138,1.715323387,0.871180493));
#135623=CARTESIAN_POINT('Ctrl Pts',(-7.401880561,1.651136808,1.276062597));
#135624=CARTESIAN_POINT('Ctrl Pts',(-7.31092609300001,1.585954698,1.673427518));
#135625=CARTESIAN_POINT('Ctrl Pts',(-7.22532308280471,1.71660033198358,
0.597718829193276));
#135626=CARTESIAN_POINT('Ctrl Pts',(-7.22499570340235,1.71596185949179,
0.601624836096638));
#135627=CARTESIAN_POINT('Ctrl Pts',(-7.224668324,1.715323387,0.605530843000001));
#135628=CARTESIAN_POINT('Ctrl Pts',(-7.191756391,1.651136808,0.998207464));
#135629=CARTESIAN_POINT('Ctrl Pts',(-7.116478391,1.585954698,1.385003724));
#135630=CARTESIAN_POINT('',(-7.11737693714463,1.58673401526929,1.38037876528236));
#135631=CARTESIAN_POINT('Origin',(0.18620950884611,1.48222902396052,-0.0537970276721317));
#135632=CARTESIAN_POINT('Ctrl Pts',(-7.36237804982027,1.62564958676894,
1.43017112466105));
#135633=CARTESIAN_POINT('Ctrl Pts',(-7.33423879050121,1.62139779885538,
1.42450272340483));
#135634=CARTESIAN_POINT('Ctrl Pts',(-7.3061141840004,1.61707840869336,1.41881176988085));
#135635=CARTESIAN_POINT('Ctrl Pts',(-7.2780056582292,1.6126879253501,1.41309678996554));
#135636=CARTESIAN_POINT('Ctrl Pts',(-7.25121113052638,1.60850268530843,
1.40764897000841));
#135637=CARTESIAN_POINT('Ctrl Pts',(-7.22443210526534,1.60425381500575,
1.40217328992506));
#135638=CARTESIAN_POINT('Ctrl Pts',(-7.1976612912563,1.59993003802629,1.39671709932095));
#135639=CARTESIAN_POINT('Ctrl Pts',(-7.17088973547085,1.59560614124188,
1.39126075753453));
#135640=CARTESIAN_POINT('Ctrl Pts',(-7.14412788854287,1.59120881940184,
1.38581442237808));
#135641=CARTESIAN_POINT('Ctrl Pts',(-7.11737693823206,1.58673401602446,
1.38037876113075));
#135642=CARTESIAN_POINT('Ctrl Pts',(-7.406444656,1.585967065,1.180922331));
#135643=CARTESIAN_POINT('Ctrl Pts',(-7.395811316,1.59657582,1.247611939));
#135644=CARTESIAN_POINT('Ctrl Pts',(-7.383978815,1.607142857,1.314099258));
#135645=CARTESIAN_POINT('Ctrl Pts',(-7.323911067,1.660786473,1.651622452));
#135646=CARTESIAN_POINT('Ctrl Pts',(-7.233301638,1.715323387,1.982258161));
#135647=CARTESIAN_POINT('Ctrl Pts',(-7.23221300334376,1.71597862537067,
1.98623061171932));
#135648=CARTESIAN_POINT('Ctrl Pts',(-7.23112436868752,1.71663386374133,
1.99020306243864));
#135649=CARTESIAN_POINT('Ctrl Pts',(-7.118274054,1.585967065,1.375745066));
#135650=CARTESIAN_POINT('Ctrl Pts',(-7.105886478,1.59657582,1.439839908));
#135651=CARTESIAN_POINT('Ctrl Pts',(-7.09234675,1.607142857,1.503701295));
#135652=CARTESIAN_POINT('Ctrl Pts',(-7.02361225300001,1.660786473,1.827893927));
#135653=CARTESIAN_POINT('Ctrl Pts',(-6.925588362,1.715323387,2.144463998));
#135654=CARTESIAN_POINT('Ctrl Pts',(-6.9244106456623,1.71597862537067,2.14826745592069));
#135655=CARTESIAN_POINT('Ctrl Pts',(-6.92323292932461,1.71663386374133,
2.15207091384138));
#135656=CARTESIAN_POINT('Ctrl Pts',(-6.92558836451754,1.71532338603359,
2.14446399142624));
#135657=CARTESIAN_POINT('Ctrl Pts',(-6.96962140931418,1.69082500736844,
2.00225841314585));
#135658=CARTESIAN_POINT('Ctrl Pts',(-7.00917981241695,1.66647815876397,
1.85898823668409));
#135659=CARTESIAN_POINT('Ctrl Pts',(-7.04421886888584,1.64234940171621,
1.71507449825301));
#135660=CARTESIAN_POINT('Ctrl Pts',(-7.06133997073513,1.63055938941156,
1.64475406096102));
#135661=CARTESIAN_POINT('Ctrl Pts',(-7.07738283337217,1.6188213974299,1.57427999703851));
#135662=CARTESIAN_POINT('Ctrl Pts',(-7.09234675007792,1.60714285693919,
1.50370129463249));
#135663=CARTESIAN_POINT('Ctrl Pts',(-7.10103840820445,1.60035948078227,
1.46270628192017));
#135664=CARTESIAN_POINT('Ctrl Pts',(-7.10938309562888,1.59355605118676,
1.42159584729182));
#135665=CARTESIAN_POINT('Ctrl Pts',(-7.117376937,1.586734015,1.380378766));
#135666=CARTESIAN_POINT('Ctrl Pts',(-7.09044573248517,1.71660033198358,
2.44451326180714));
#135667=CARTESIAN_POINT('Ctrl Pts',(-7.08911996624259,1.71596185949179,
2.44834526790357));
#135668=CARTESIAN_POINT('Ctrl Pts',(-7.0877942,1.715323387,2.452177274));
#135669=CARTESIAN_POINT('Ctrl Pts',(-6.954512969,1.651136808,2.837414485));
#135670=CARTESIAN_POINT('Ctrl Pts',(-6.780263254,1.585954698,3.205936713));
#135671=CARTESIAN_POINT('Ctrl Pts',(-6.92790716496715,1.71660033198358,
2.13697537852514));
#135672=CARTESIAN_POINT('Ctrl Pts',(-6.92674776348357,1.71596185949179,
2.14071968826257));
#135673=CARTESIAN_POINT('Ctrl Pts',(-6.92558836200001,1.715323387,2.144463998));
#135674=CARTESIAN_POINT('Ctrl Pts',(-6.809032025,1.651136808,2.520884965));
#135675=CARTESIAN_POINT('Ctrl Pts',(-6.65236422,1.585954698,2.882455599));
#135676=CARTESIAN_POINT('',(-6.65423598885696,1.58673401523155,2.87813192899063));
#135677=CARTESIAN_POINT('Origin',(0.170291263072342,1.48222902846579,-0.0925688321982565));
#135678=CARTESIAN_POINT('Ctrl Pts',(-6.88280522651745,1.62564958674772,
2.97942816881734));
#135679=CARTESIAN_POINT('Ctrl Pts',(-6.85654238608057,1.62139779883964,
2.9678431826258));
#135680=CARTESIAN_POINT('Ctrl Pts',(-6.83029870404631,1.61707840869647,
2.95623932143671));
#135681=CARTESIAN_POINT('Ctrl Pts',(-6.80407589172505,1.61268792537165,
2.94461545246392));
#135682=CARTESIAN_POINT('Ctrl Pts',(-6.77907892536435,1.60850268533586,
2.93353496810799));
#135683=CARTESIAN_POINT('Ctrl Pts',(-6.75410308807487,1.60425381503204,
2.92243060758177));
#135684=CARTESIAN_POINT('Ctrl Pts',(-6.72913108036632,1.59993003804053,
2.91134704614054));
#135685=CARTESIAN_POINT('Ctrl Pts',(-6.70415838072451,1.59560614124426,
2.90026317759203));
#135686=CARTESIAN_POINT('Ctrl Pts',(-6.67919301180922,1.59120881939051,
2.88919116886698));
#135687=CARTESIAN_POINT('Ctrl Pts',(-6.6542359904442,1.58673401620649,2.87813192527157));
#135688=CARTESIAN_POINT('Ctrl Pts',(-6.979422703,1.585967065,2.745479691));
#135689=CARTESIAN_POINT('Ctrl Pts',(-6.95470167,1.59657582,2.808324279));
#135690=CARTESIAN_POINT('Ctrl Pts',(-6.928852998,1.607142857,2.870713524));
#135691=CARTESIAN_POINT('Ctrl Pts',(-6.797632091,1.660786473,3.187432823));
#135692=CARTESIAN_POINT('Ctrl Pts',(-6.638064156,1.715323387,3.490860104));
#135693=CARTESIAN_POINT('Ctrl Pts',(-6.63614701353499,1.71597862537066,
3.49450565675749));
#135694=CARTESIAN_POINT('Ctrl Pts',(-6.63422987106999,1.71663386374133,
3.49815120951497));
#135695=CARTESIAN_POINT('Ctrl Pts',(-6.65610824,1.585967065,2.873799418));
#135696=CARTESIAN_POINT('Ctrl Pts',(-6.630231782,1.59657582,2.933732796));
#135697=CARTESIAN_POINT('Ctrl Pts',(-6.603280295,1.607142857,2.993190497));
#135698=CARTESIAN_POINT('Ctrl Pts',(-6.46646094,1.660786473,3.2950278));
#135699=CARTESIAN_POINT('Ctrl Pts',(-6.30267558499999,1.715323387,3.583124401));
#135700=CARTESIAN_POINT('Ctrl Pts',(-6.30070777198533,1.71597862537066,
3.58658576200464));
#135701=CARTESIAN_POINT('Ctrl Pts',(-6.29873995897067,1.71663386374133,
3.59004712300929));
#135702=CARTESIAN_POINT('Ctrl Pts',(-6.3026755931018,1.71532338430228,3.58312438674902));
#135703=CARTESIAN_POINT('Ctrl Pts',(-6.37624917261175,1.69082500352122,
3.45370928555288));
#135704=CARTESIAN_POINT('Ctrl Pts',(-6.44568158368489,1.66647815192422,
3.32229255612157));
#135705=CARTESIAN_POINT('Ctrl Pts',(-6.51083865543083,1.64234939105966,
3.18927578061367));
#135706=CARTESIAN_POINT('Ctrl Pts',(-6.54267628004166,1.63055938254416,
3.1242799474357));
#135707=CARTESIAN_POINT('Ctrl Pts',(-6.57349390040191,1.6188213941053,3.05890228911775));
#135708=CARTESIAN_POINT('Ctrl Pts',(-6.60328029523312,1.6071428569086,2.9931904964857));
#135709=CARTESIAN_POINT('Ctrl Pts',(-6.62058146193252,1.60035948096017,
2.95502237623406));
#135710=CARTESIAN_POINT('Ctrl Pts',(-6.63756858308226,1.59355605142897,
2.91666694263408));
#135711=CARTESIAN_POINT('Ctrl Pts',(-6.65423598891596,1.58673401453857,
2.87813192913883));
#135712=CARTESIAN_POINT('Ctrl Pts',(-6.39917695920962,1.71660033198358,
3.91159814126253));
#135713=CARTESIAN_POINT('Ctrl Pts',(-6.39705842060482,1.71596185949179,
3.91505555663127));
#135714=CARTESIAN_POINT('Ctrl Pts',(-6.394939882,1.715323387,3.918512972));
#135715=CARTESIAN_POINT('Ctrl Pts',(-6.181960079,1.651136808,4.266092026));
#135716=CARTESIAN_POINT('Ctrl Pts',(-5.93256284,1.585954698,4.588539871));
#135717=CARTESIAN_POINT('Ctrl Pts',(-6.30655000747555,1.71660033198358,
3.57630933537954));
#135718=CARTESIAN_POINT('Ctrl Pts',(-6.30461279623777,1.71596185949179,
3.57971686818977));
#135719=CARTESIAN_POINT('Ctrl Pts',(-6.302675585,1.715323387,3.583124401));
#135720=CARTESIAN_POINT('Ctrl Pts',(-6.107924889,1.651136808,3.925688688));
#135721=CARTESIAN_POINT('Ctrl Pts',(-5.87719289300001,1.585954698,4.245127054));
#135722=CARTESIAN_POINT('',(-5.87995036171793,1.58673401520821,4.24130684438252));
#135723=CARTESIAN_POINT('Origin',(0.146410562493575,1.48222898979575,-0.127012328747914));
#135724=CARTESIAN_POINT('Ctrl Pts',(-6.08140007972267,1.62564958678031,
4.38937046350252));
#135725=CARTESIAN_POINT('Ctrl Pts',(-6.05824167964871,1.62139779889533,
4.37241059342073));
#135726=CARTESIAN_POINT('Ctrl Pts',(-6.03510604752352,1.61707840874886,
4.35543640811371));
#135727=CARTESIAN_POINT('Ctrl Pts',(-6.01199509829649,1.61268792542109,
4.33844716915636));
#135728=CARTESIAN_POINT('Ctrl Pts',(-5.98996452384715,1.60850268539175,
4.3222521314705));
#135729=CARTESIAN_POINT('Ctrl Pts',(-5.96795971712767,1.60425381508137,
4.30603831801684));
#135730=CARTESIAN_POINT('Ctrl Pts',(-5.94595417929556,1.59993003808504,
4.28984564058481));
#135731=CARTESIAN_POINT('Ctrl Pts',(-5.92394803172507,1.59560614128375,
4.27365251447949));
#135732=CARTESIAN_POINT('Ctrl Pts',(-5.90194649400798,1.59120881942668,
4.25747254677786));
#135733=CARTESIAN_POINT('Ctrl Pts',(-5.87995036393212,1.58673401603956,
4.24130684150147));
#135734=CARTESIAN_POINT('Ctrl Pts',(-6.22605070100001,1.585967065,4.181661472));
#135735=CARTESIAN_POINT('Ctrl Pts',(-6.188397903,1.59657582,4.237722498));
#135736=CARTESIAN_POINT('Ctrl Pts',(-6.149741715,1.607142857,4.293096416));
#135737=CARTESIAN_POINT('Ctrl Pts',(-5.953503393,1.660786473,4.574202378));
#135738=CARTESIAN_POINT('Ctrl Pts',(-5.73243817100001,1.715323387,4.836233308));
#135739=CARTESIAN_POINT('Ctrl Pts',(-5.72978216417361,1.71597862537067,
4.83938150079355));
#135740=CARTESIAN_POINT('Ctrl Pts',(-5.72712615734723,1.71663386374133,
4.84252969358709));
#135741=CARTESIAN_POINT('Ctrl Pts',(-5.88271020300001,1.585967065,4.237478103));
#135742=CARTESIAN_POINT('Ctrl Pts',(-5.844554817,1.59657582,4.290447598));
#135743=CARTESIAN_POINT('Ctrl Pts',(-5.805451792,1.607142857,4.342721438));
#135744=CARTESIAN_POINT('Ctrl Pts',(-5.6069451,1.660786473,4.608089836));
#135745=CARTESIAN_POINT('Ctrl Pts',(-5.385056702,1.715323387,4.854241888));
#135746=CARTESIAN_POINT('Ctrl Pts',(-5.38239080505587,1.71597862537067,
4.85719930266941));
#135747=CARTESIAN_POINT('Ctrl Pts',(-5.37972490811174,1.71663386374133,
4.86015671733883));
#135748=CARTESIAN_POINT('Ctrl Pts',(-5.38505671266411,1.71532338437892,
4.85424187616975));
#135749=CARTESIAN_POINT('Ctrl Pts',(-5.48473056372628,1.69082501355794,
4.74366861817509));
#135750=CARTESIAN_POINT('Ctrl Pts',(-5.58079035829832,1.66647817182258,
4.63025030234907));
#135751=CARTESIAN_POINT('Ctrl Pts',(-5.67301873404316,1.64234942068528,
4.51435027910742));
#135752=CARTESIAN_POINT('Ctrl Pts',(-5.71808423471452,1.63055940224687,
4.45771811429886));
#135753=CARTESIAN_POINT('Ctrl Pts',(-5.76223565778625,1.61882140398259,
4.40049377946256));
#135754=CARTESIAN_POINT('Ctrl Pts',(-5.80545179213163,1.60714285708149,
4.34272143834067));
#135755=CARTESIAN_POINT('Ctrl Pts',(-5.83055348496221,1.60035948120359,
4.3091649072749));
#135756=CARTESIAN_POINT('Ctrl Pts',(-5.85538874093021,1.59355605170177,
4.27535793163229));
#135757=CARTESIAN_POINT('Ctrl Pts',(-5.87995036172034,1.58673401468259,
4.24130684448956));
#135758=CARTESIAN_POINT('Ctrl Pts',(-5.40868978391049,1.71660033198358,
5.19578103749289));
#135759=CARTESIAN_POINT('Ctrl Pts',(-5.40587753345524,1.71596185949179,
5.19870219724644));
#135760=CARTESIAN_POINT('Ctrl Pts',(-5.40306528300001,1.715323387,5.201623357));
#135761=CARTESIAN_POINT('Ctrl Pts',(-5.120345607,1.651136808,5.495291845));
#135762=CARTESIAN_POINT('Ctrl Pts',(-4.807462382,1.585954698,5.756588004));
#135763=CARTESIAN_POINT('Ctrl Pts',(-5.39030558027708,1.71660033198358,
4.84841904112145));
#135764=CARTESIAN_POINT('Ctrl Pts',(-5.38768114113854,1.71596185949179,
4.85133046456072));
#135765=CARTESIAN_POINT('Ctrl Pts',(-5.385056702,1.715323387,4.854241888));
#135766=CARTESIAN_POINT('Ctrl Pts',(-5.121217974,1.651136808,5.14693157));
#135767=CARTESIAN_POINT('Ctrl Pts',(-4.827210557,1.585954698,5.409301086));
#135768=CARTESIAN_POINT('',(-4.83072478968181,1.58673401528728,5.40616296532268));
#135769=CARTESIAN_POINT('Origin',(0.115683554224224,1.48222901566629,-0.155516667237091));
#135770=CARTESIAN_POINT('Ctrl Pts',(-4.99563542474065,1.62564958676171,
5.59407067341435));
#135771=CARTESIAN_POINT('Ctrl Pts',(-4.9766643259881,1.62139779890127,5.57252894419362));
#135772=CARTESIAN_POINT('Ctrl Pts',(-4.95771854011771,1.61707840875737,
5.55097812899299));
#135773=CARTESIAN_POINT('Ctrl Pts',(-4.93880009614803,1.61268792543274,
5.52941791819071));
#135774=CARTESIAN_POINT('Ctrl Pts',(-4.92076603853601,1.60850268539144,
5.50886558923814));
#135775=CARTESIAN_POINT('Ctrl Pts',(-4.90276118250712,1.60425381508363,
5.4883004627315));
#135776=CARTESIAN_POINT('Ctrl Pts',(-4.88475106888786,1.59993003810558,
5.46775582088404));
#135777=CARTESIAN_POINT('Ctrl Pts',(-4.86674045623727,1.59560614132261,
5.44721060977753));
#135778=CARTESIAN_POINT('Ctrl Pts',(-4.84873151701052,1.59120881949219,
5.42667924040514));
#135779=CARTESIAN_POINT('Ctrl Pts',(-4.83072479286547,1.58673401610626,
5.4061629624154));
#135780=CARTESIAN_POINT('Ctrl Pts',(-5.181555488,1.585967065,5.422313411));
#135781=CARTESIAN_POINT('Ctrl Pts',(-5.13273152800001,1.59657582,5.468969522));
#135782=CARTESIAN_POINT('Ctrl Pts',(-5.083075345,1.607142857,5.514738891));
#135783=CARTESIAN_POINT('Ctrl Pts',(-4.830995493,1.660786473,5.747087313));
#135784=CARTESIAN_POINT('Ctrl Pts',(-4.558769749,1.715323387,5.955469618));
#135785=CARTESIAN_POINT('Ctrl Pts',(-4.5554990697505,1.71597862537066,5.95797324484628));
#135786=CARTESIAN_POINT('Ctrl Pts',(-4.552228390501,1.71663386374133,5.96047687169255));
#135787=CARTESIAN_POINT('Ctrl Pts',(-4.834243174,1.585967065,5.403017021));
#135788=CARTESIAN_POINT('Ctrl Pts',(-4.785592964,1.59657582,5.446545839));
#135789=CARTESIAN_POINT('Ctrl Pts',(-4.736166816,1.607142857,5.489191552));
#135790=CARTESIAN_POINT('Ctrl Pts',(-4.485254739,1.660786473,5.705682713));
#135791=CARTESIAN_POINT('Ctrl Pts',(-4.215638554,1.715323387,5.898380421));
#135792=CARTESIAN_POINT('Ctrl Pts',(-4.21239922751805,1.71597862537066,
5.90069560392768));
#135793=CARTESIAN_POINT('Ctrl Pts',(-4.20915990103609,1.71663386374133,
5.90301078685534));
#135794=CARTESIAN_POINT('Ctrl Pts',(-4.21563855917688,1.71532338609041,
5.89838041591));
#135795=CARTESIAN_POINT('Ctrl Pts',(-4.33675209913449,1.69082500967298,
5.81181921265613));
#135796=CARTESIAN_POINT('Ctrl Pts',(-4.45494767587929,1.66647816324636,
5.7217025528292));
#135797=CARTESIAN_POINT('Ctrl Pts',(-4.56993489988004,1.6423494082958,5.62833856611449));
#135798=CARTESIAN_POINT('Ctrl Pts',(-4.62612101649552,1.63055939378575,
5.58271819488782));
#135799=CARTESIAN_POINT('Ctrl Pts',(-4.68154172496527,1.61882139960798,
5.53632299966429));
#135800=CARTESIAN_POINT('Ctrl Pts',(-4.73616681628953,1.60714285693547,
5.48919155190664));
#135801=CARTESIAN_POINT('Ctrl Pts',(-4.7678953096723,1.60035948077783,5.46181567431286));
#135802=CARTESIAN_POINT('Ctrl Pts',(-4.79941743244761,1.59355605119151,
5.43413793201519));
#135803=CARTESIAN_POINT('Ctrl Pts',(-4.830724789,1.586734015,5.406162966));
#135804=CARTESIAN_POINT('Ctrl Pts',(-4.16529828519659,1.71660033198358,
6.23701498812772));
#135805=CARTESIAN_POINT('Ctrl Pts',(-4.16192382059829,1.71596185949179,
6.23926330206386));
#135806=CARTESIAN_POINT('Ctrl Pts',(-4.158549356,1.715323387,6.241511616));
#135807=CARTESIAN_POINT('Ctrl Pts',(-3.819309465,1.651136808,6.467537924));
#135808=CARTESIAN_POINT('Ctrl Pts',(-3.457570326,1.585954698,6.65546448));
#135809=CARTESIAN_POINT('Ctrl Pts',(-4.22201645637774,1.71660033198358,
5.893822062747));
#135810=CARTESIAN_POINT('Ctrl Pts',(-4.21882750518887,1.71596185949179,
5.8961012418735));
#135811=CARTESIAN_POINT('Ctrl Pts',(-4.215638554,1.715323387,5.898380421));
#135812=CARTESIAN_POINT('Ctrl Pts',(-3.895048599,1.651136808,6.127509652));
#135813=CARTESIAN_POINT('Ctrl Pts',(-3.551513221,1.585954698,6.320542211));
#135814=CARTESIAN_POINT('',(-3.55561989738265,1.58673401525583,6.3182329131868));
#135815=CARTESIAN_POINT('Origin',(0.0795475509393828,1.48222904884081,-0.17674948871494));
#135816=CARTESIAN_POINT('Ctrl Pts',(-3.67628040946491,1.62564958677506,
6.53719835604483));
#135817=CARTESIAN_POINT('Ctrl Pts',(-3.66238367936959,1.62139779888063,
6.51208203505397));
#135818=CARTESIAN_POINT('Ctrl Pts',(-3.64851362369125,1.61707840872687,
6.48696228194679));
#135819=CARTESIAN_POINT('Ctrl Pts',(-3.6346722904589,1.61268792539826,6.46183923059958));
#135820=CARTESIAN_POINT('Ctrl Pts',(-3.62147800234549,1.60850268536232,
6.43789061436456));
#135821=CARTESIAN_POINT('Ctrl Pts',(-3.60831498411565,1.60425381504979,
6.4139357772996));
#135822=CARTESIAN_POINT('Ctrl Pts',(-3.59514242756208,1.59993003806146,
6.38999981577955));
#135823=CARTESIAN_POINT('Ctrl Pts',(-3.58196950601816,1.59560614126824,
6.36606319103251));
#135824=CARTESIAN_POINT('Ctrl Pts',(-3.56879524322245,1.59120881943395,
6.34214044413688));
#135825=CARTESIAN_POINT('Ctrl Pts',(-3.55561990060144,1.58673401625832,
6.31823291137706));
#135826=CARTESIAN_POINT('Ctrl Pts',(-3.894776499,1.585967065,6.409424001));
#135827=CARTESIAN_POINT('Ctrl Pts',(-3.837064332,1.59657582,6.44449361));
#135828=CARTESIAN_POINT('Ctrl Pts',(-3.778730021,1.607142857,6.478518305));
#135829=CARTESIAN_POINT('Ctrl Pts',(-3.482595614,1.660786473,6.651244833));
#135830=CARTESIAN_POINT('Ctrl Pts',(-3.17193832,1.715323387,6.796234788));
#135831=CARTESIAN_POINT('Ctrl Pts',(-3.16820590163919,1.71597862537067,
6.79797678209004));
#135832=CARTESIAN_POINT('Ctrl Pts',(-3.16447348327838,1.71663386374133,
6.79971877618008));
#135833=CARTESIAN_POINT('Ctrl Pts',(-3.559732308,1.585967065,6.315916869));
#135834=CARTESIAN_POINT('Ctrl Pts',(-3.502862104,1.59657582,6.347969651));
#135835=CARTESIAN_POINT('Ctrl Pts',(-3.445423944,1.607142857,6.378993169));
#135836=CARTESIAN_POINT('Ctrl Pts',(-3.153838851,1.660786473,6.536484208));
#135837=CARTESIAN_POINT('Ctrl Pts',(-2.849101831,1.715323387,6.66671724));
#135838=CARTESIAN_POINT('Ctrl Pts',(-2.8454405422724,1.71597862537067,6.66828193578925));
#135839=CARTESIAN_POINT('Ctrl Pts',(-2.84177925354481,1.71663386374133,
6.6698466315785));
#135840=CARTESIAN_POINT('Ctrl Pts',(-2.84910184639505,1.71532338424484,
6.66671723342074));
#135841=CARTESIAN_POINT('Ctrl Pts',(-2.98599189749724,1.69082501201072,
6.60821562268897));
#135842=CARTESIAN_POINT('Ctrl Pts',(-3.1207965283895,1.66647816885366,6.54561440386231));
#135843=CARTESIAN_POINT('Ctrl Pts',(-3.25316589951571,1.64234941630276,
6.47915207685954));
#135844=CARTESIAN_POINT('Ctrl Pts',(-3.31784546089788,1.63055939933424,
6.44667663240888));
#135845=CARTESIAN_POINT('Ctrl Pts',(-3.38194407384616,1.61882140252272,
6.41327993798857));
#135846=CARTESIAN_POINT('Ctrl Pts',(-3.44542394381593,1.60714285705506,
6.37899316919607));
#135847=CARTESIAN_POINT('Ctrl Pts',(-3.48229564501008,1.6003594811509,6.35907801375703));
#135848=CARTESIAN_POINT('Ctrl Pts',(-3.51903069410623,1.59355605158396,
6.33882368660111));
#135849=CARTESIAN_POINT('Ctrl Pts',(-3.55561989734046,1.58673401463352,
6.31823291331802));
#135850=CARTESIAN_POINT('Ctrl Pts',(-2.72714206803972,1.71660033198358,
6.98661305006529));
#135851=CARTESIAN_POINT('Ctrl Pts',(-2.72336317551986,1.71596185949179,
6.98808338953265));
#135852=CARTESIAN_POINT('Ctrl Pts',(-2.719584283,1.715323387,6.989553729));
#135853=CARTESIAN_POINT('Ctrl Pts',(-2.339686658,1.651136808,7.137369119));
#135854=CARTESIAN_POINT('Ctrl Pts',(-1.946006124,1.585954698,7.243138834));
#135855=CARTESIAN_POINT('Ctrl Pts',(-2.85631053383156,1.71660033198358,
6.66363651409478));
#135856=CARTESIAN_POINT('Ctrl Pts',(-2.85270618241578,1.71596185949179,
6.66517687704739));
#135857=CARTESIAN_POINT('Ctrl Pts',(-2.849101831,1.715323387,6.66671724));
#135858=CARTESIAN_POINT('Ctrl Pts',(-2.48675108,1.651136808,6.821572194));
#135859=CARTESIAN_POINT('Ctrl Pts',(-2.109751075,1.585954698,6.936241807));
#135860=CARTESIAN_POINT('',(-2.11425816856513,1.5867340151998,6.93486931357578));
#135861=CARTESIAN_POINT('Origin',(0.0396917784304465,1.48222903682356,-0.189717322672631));
#135862=CARTESIAN_POINT('Ctrl Pts',(-2.18502660812398,1.62564958673401,
7.17465390925617));
#135863=CARTESIAN_POINT('Ctrl Pts',(-2.17685404271359,1.62139779888482,
7.14713740763033));
#135864=CARTESIAN_POINT('Ctrl Pts',(-2.16870826565351,1.61707840873381,
7.11962328841482));
#135865=CARTESIAN_POINT('Ctrl Pts',(-2.160591248555,1.61268792540409,7.09211212254638));
#135866=CARTESIAN_POINT('Ctrl Pts',(-2.15285368017845,1.60850268536363,
7.06588702970223));
#135867=CARTESIAN_POINT('Ctrl Pts',(-2.14514798794446,1.6042538150484,7.03966258355752));
#135868=CARTESIAN_POINT('Ctrl Pts',(-2.1374289226582,1.59993003804401,7.01345452121582));
#135869=CARTESIAN_POINT('Ctrl Pts',(-2.12970964348897,1.59560614123467,
6.9872457326906));
#135870=CARTESIAN_POINT('Ctrl Pts',(-2.12198607104548,1.59120881937031,
6.96105020924954));
#135871=CARTESIAN_POINT('Ctrl Pts',(-2.11425817195538,1.58673401592903,
6.9348693128284));
#135872=CARTESIAN_POINT('Ctrl Pts',(-2.42588209,1.585967065,7.096837048));
#135873=CARTESIAN_POINT('Ctrl Pts',(-2.361980272,1.59657582,7.118680339));
#135874=CARTESIAN_POINT('Ctrl Pts',(-2.297695481,1.607142857,7.139369403));
#135875=CARTESIAN_POINT('Ctrl Pts',(-1.971353434,1.660786473,7.244397537));
#135876=CARTESIAN_POINT('Ctrl Pts',(-1.636790581,1.715323387,7.319215572));
#135877=CARTESIAN_POINT('Ctrl Pts',(-1.6327709472766,1.71597862537066,7.32011447961603));
#135878=CARTESIAN_POINT('Ctrl Pts',(-1.6287513135532,1.71663386374133,7.32101338723207));
#135879=CARTESIAN_POINT('Ctrl Pts',(-2.118772315,1.585967065,6.933491464));
#135880=CARTESIAN_POINT('Ctrl Pts',(-2.056341304,1.59657582,6.952569456));
#135881=CARTESIAN_POINT('Ctrl Pts',(-1.993576877,1.607142857,6.970520155));
#135882=CARTESIAN_POINT('Ctrl Pts',(-1.674952964,1.660786473,7.061646965));
#135883=CARTESIAN_POINT('Ctrl Pts',(-1.349344274,1.715323387,7.12332577));
#135884=CARTESIAN_POINT('Ctrl Pts',(-1.34543222082607,1.71597862537066,
7.12406681522476));
#135885=CARTESIAN_POINT('Ctrl Pts',(-1.34152016765215,1.71663386374133,
7.12480786044952));
#135886=CARTESIAN_POINT('Ctrl Pts',(-1.34934428967406,1.71532338437472,
7.12332576703092));
#135887=CARTESIAN_POINT('Ctrl Pts',(-1.49561004609945,1.69082501186417,
7.09561920558352));
#135888=CARTESIAN_POINT('Ctrl Pts',(-1.64072043248348,1.66647816847583,
7.06346057892067));
#135889=CARTESIAN_POINT('Ctrl Pts',(-1.78428251795239,1.64234941574856,
7.02700760592775));
#135890=CARTESIAN_POINT('Ctrl Pts',(-1.85443116652592,1.63055939897599,
7.00919561341184));
#135891=CARTESIAN_POINT('Ctrl Pts',(-1.92421049037672,1.618821402371,6.99035902258183));
#135892=CARTESIAN_POINT('Ctrl Pts',(-1.99357687675647,1.60714285712086,
6.97052015546866));
#135893=CARTESIAN_POINT('Ctrl Pts',(-2.03386770756363,1.60035948126202,
6.95899693115295));
#135894=CARTESIAN_POINT('Ctrl Pts',(-2.07409799246674,1.5935560517563,6.94711308871186));
#135895=CARTESIAN_POINT('Ctrl Pts',(-2.11425816857299,1.58673401473019,
6.93486931386321));
#135896=CARTESIAN_POINT('Ctrl Pts',(-1.16146771926858,1.71660033198358,
7.40952484987453));
#135897=CARTESIAN_POINT('Ctrl Pts',(-1.15746109563429,1.71596185949179,
7.41014846343726));
#135898=CARTESIAN_POINT('Ctrl Pts',(-1.153454472,1.715323387,7.41077207700001));
#135899=CARTESIAN_POINT('Ctrl Pts',(-0.750662703,1.651136808,7.47346486600001));
#135900=CARTESIAN_POINT('Ctrl Pts',(-0.343448839,1.585954698,7.492132066));
#135901=CARTESIAN_POINT('Ctrl Pts',(-1.35704670638058,1.71660033198358,
7.12186672777106));
#135902=CARTESIAN_POINT('Ctrl Pts',(-1.35319549019029,1.71596185949179,
7.12259624888553));
#135903=CARTESIAN_POINT('Ctrl Pts',(-1.349344274,1.715323387,7.12332577000001));
#135904=CARTESIAN_POINT('Ctrl Pts',(-0.962175844,1.651136808,7.196665601));
#135905=CARTESIAN_POINT('Ctrl Pts',(-0.569339312,1.585954698,7.227610445));
#135906=CARTESIAN_POINT('',(-0.574036078793354,1.58673401524049,7.22723893187494));
#135907=CARTESIAN_POINT('Origin',(-0.00201981579105066,1.48222903402286,
-0.193814356406586));
#135908=CARTESIAN_POINT('Ctrl Pts',(-0.591603391086984,1.62564958670864,
7.47663061967719));
#135909=CARTESIAN_POINT('Ctrl Pts',(-0.589537129951309,1.62139779883426,
7.44800057857977));
#135910=CARTESIAN_POINT('Ctrl Pts',(-0.587496518870869,1.61707840868329,
7.4193786228778));
#135911=CARTESIAN_POINT('Ctrl Pts',(-0.585483360458298,1.61268792535319,
7.39076573401896));
#135912=CARTESIAN_POINT('Ctrl Pts',(-0.583564311790205,1.60850268531728,
7.36349042080358));
#135913=CARTESIAN_POINT('Ctrl Pts',(-0.581676255042661,1.60425381501644,
7.33622259159249));
#135914=CARTESIAN_POINT('Ctrl Pts',(-0.579771615869591,1.59993003803003,
7.30896788832829));
#135915=CARTESIAN_POINT('Ctrl Pts',(-0.577866923922012,1.59560614123866,
7.28171242987984));
#135916=CARTESIAN_POINT('Ctrl Pts',(-0.575955187441002,1.59120881938927,
7.25446900346002));
#135917=CARTESIAN_POINT('Ctrl Pts',(-0.574036082484844,1.58673401613979,
7.22723893149673));
#135918=CARTESIAN_POINT('Ctrl Pts',(-0.84355613,1.585967065,7.452409882));
#135919=CARTESIAN_POINT('Ctrl Pts',(-0.776452639,1.59657582,7.460005487));
#135920=CARTESIAN_POINT('Ctrl Pts',(-0.709223254,1.607142857,7.466391523));
#135921=CARTESIAN_POINT('Ctrl Pts',(-0.367932958,1.660786473,7.498810264));
#135922=CARTESIAN_POINT('Ctrl Pts',(-0.025108333,1.715323387,7.499957971));
#135923=CARTESIAN_POINT('Ctrl Pts',(-0.0209894375174155,1.71597862537066,
7.49997176022292));
#135924=CARTESIAN_POINT('Ctrl Pts',(-0.016870542034831,1.71663386374133,
7.49998554944585));
#135925=CARTESIAN_POINT('Ctrl Pts',(-0.578740883,1.585967065,7.226863704));
#135926=CARTESIAN_POINT('Ctrl Pts',(-0.51366827,1.59657582,7.232074841));
#135927=CARTESIAN_POINT('Ctrl Pts',(-0.448512371,1.607142857,7.236113367));
#135928=CARTESIAN_POINT('Ctrl Pts',(-0.117748137,1.660786473,7.256614959));
#135929=CARTESIAN_POINT('Ctrl Pts',(0.213507122,1.715323387,7.246855505));
#135930=CARTESIAN_POINT('Ctrl Pts',(0.217487016355248,1.71597862537066,
7.24673824921362));
#135931=CARTESIAN_POINT('Ctrl Pts',(0.221466910710496,1.71663386374133,
7.24662099342725));
#135932=CARTESIAN_POINT('Ctrl Pts',(0.213507114912512,1.71532338597331,
7.2468555060868));
#135933=CARTESIAN_POINT('Ctrl Pts',(0.200619328248611,1.71320157779897,
7.24723520642678));
#135934=CARTESIAN_POINT('Ctrl Pts',(0.196655750649506,1.71254943779287,
7.24733664243004));
#135935=CARTESIAN_POINT('Ctrl Pts',(0.180551941733234,1.70989962927072,
7.24775613221961));
#135936=CARTESIAN_POINT('Ctrl Pts',(0.17231146465773,1.70854407397244,7.24795672696019));
#135937=CARTESIAN_POINT('Ctrl Pts',(0.147595163082729,1.70447938479062,
7.2485162106093));
#135938=CARTESIAN_POINT('Ctrl Pts',(0.131118277380395,1.70177120836391,
7.24883298177625));
#135939=CARTESIAN_POINT('Ctrl Pts',(0.081710543770135,1.69365497342894,
7.24961433639062));
#135940=CARTESIAN_POINT('Ctrl Pts',(0.0487767691046939,1.68825095317067,
7.2499107293857));
#135941=CARTESIAN_POINT('Ctrl Pts',(-0.0499137006149773,1.67207514746497,
7.25012636772878));
#135942=CARTESIAN_POINT('Ctrl Pts',(-0.115671654201335,1.66132115636037,
7.24937548198048));
#135943=CARTESIAN_POINT('Ctrl Pts',(-0.312506753462951,1.62920290478646,
7.24444859976342));
#135944=CARTESIAN_POINT('Ctrl Pts',(-0.443380249615298,1.60803075453319,
7.23761650001668));
#135945=CARTESIAN_POINT('Ctrl Pts',(-0.574036078744983,1.58673401461205,
7.22723893255561));
#135946=CARTESIAN_POINT('Ctrl Pts',(-1.354636469,4.302796438,7.122321253));
#135947=CARTESIAN_POINT('Ctrl Pts',(-0.968989539,4.238074114,7.195669727));
#135948=CARTESIAN_POINT('Ctrl Pts',(-0.577677421000001,4.172899507,7.226948789));
#135949=CARTESIAN_POINT('Ctrl Pts',(-0.564250173365847,4.17066314490592,
7.22802207983848));
#135950=CARTESIAN_POINT('Ctrl Pts',(-0.550822925731692,4.16842678281185,
7.22909537067707));
#135951=CARTESIAN_POINT('Ctrl Pts',(-1.64281292560515,4.302796438,7.31839524783626));
#135952=CARTESIAN_POINT('Ctrl Pts',(-1.24654932631986,4.238074114,7.40734739431102));
#135953=CARTESIAN_POINT('Ctrl Pts',(-0.842997787615108,4.172899507,7.45299255686155));
#135954=CARTESIAN_POINT('Ctrl Pts',(-0.829150563892455,4.17066314490592,
7.45455879739607));
#135955=CARTESIAN_POINT('Ctrl Pts',(-0.815303340169794,4.16842678281185,
7.45612503793064));
#135956=CARTESIAN_POINT('',(-1.35005064870962,4.30202682597625,7.12319192827134));
#135957=CARTESIAN_POINT('Origin',(0.0137705755161144,4.16072147847015,-0.198015518509984));
#135958=CARTESIAN_POINT('Ctrl Pts',(-1.39881673453704,4.26310680820179,
7.36839953710498));
#135959=CARTESIAN_POINT('Ctrl Pts',(-1.39323107349379,4.26736775487504,
7.34024242578059));
#135960=CARTESIAN_POINT('Ctrl Pts',(-1.38763724397555,4.27169422775334,
7.3120967623594));
#135961=CARTESIAN_POINT('Ctrl Pts',(-1.38203469282476,4.27608953503156,
7.28396366972715));
#135962=CARTESIAN_POINT('Ctrl Pts',(-1.37669475276436,4.28027881894546,
7.25714927315551));
#135963=CARTESIAN_POINT('Ctrl Pts',(-1.37133665373562,4.28452899137152,
7.23034791613796));
#135964=CARTESIAN_POINT('Ctrl Pts',(-1.36599630035225,4.2888490835118,7.20355436555762));
#135965=CARTESIAN_POINT('Ctrl Pts',(-1.36065581289424,4.2931692841121,7.17676014229977));
#135966=CARTESIAN_POINT('Ctrl Pts',(-1.35534004338375,4.29756059498722,
7.14997233931333));
#135967=CARTESIAN_POINT('Ctrl Pts',(-1.35005064905555,4.30202682552111,
7.12319192419185));
#135968=CARTESIAN_POINT('Ctrl Pts',(-2.1253965081304,4.17158344184794,6.93146835656078));
#135969=CARTESIAN_POINT('Ctrl Pts',(-2.1215742575652,4.17224147442397,6.93263576478039));
#135970=CARTESIAN_POINT('Ctrl Pts',(-2.117752007,4.172899507,6.933803173));
#135971=CARTESIAN_POINT('Ctrl Pts',(-1.787314404,4.229787119,7.034726848));
#135972=CARTESIAN_POINT('Ctrl Pts',(-1.448776863,4.285714286,7.103769816));
#135973=CARTESIAN_POINT('Ctrl Pts',(-1.397161514,4.294241258,7.114296498));
#135974=CARTESIAN_POINT('Ctrl Pts',(-1.345398651,4.302795611,7.12407204299999));
#135975=CARTESIAN_POINT('Ctrl Pts',(-1.96234429440288,4.17158344184794,
7.23873422950782));
#135976=CARTESIAN_POINT('Ctrl Pts',(-1.95835276320144,4.17224147442397,
7.23981156875392));
#135977=CARTESIAN_POINT('Ctrl Pts',(-1.954361232,4.172899507,7.240888908));
#135978=CARTESIAN_POINT('Ctrl Pts',(-1.609289139,4.229787119,7.334026025));
#135979=CARTESIAN_POINT('Ctrl Pts',(-1.256923902,4.285714286,7.393926041));
#135980=CARTESIAN_POINT('Ctrl Pts',(-1.203200304,4.294241258,7.403058737));
#135981=CARTESIAN_POINT('Ctrl Pts',(-1.14934967,4.302795611,7.411409808));
#135982=CARTESIAN_POINT('Ctrl Pts',(-2.11775200214645,4.17289950776325,
6.93380317514373));
#135983=CARTESIAN_POINT('Ctrl Pts',(-2.10540223265424,4.17502562443694,
6.93757509482064));
#135984=CARTESIAN_POINT('Ctrl Pts',(-2.10156372697733,4.1756853482417,6.9387313149784));
#135985=CARTESIAN_POINT('Ctrl Pts',(-2.08608302136244,4.17834651467031,
6.94340162287339));
#135986=CARTESIAN_POINT('Ctrl Pts',(-2.07815766815513,4.17970788576612,
6.94577779488903));
#135987=CARTESIAN_POINT('Ctrl Pts',(-2.05437518968315,4.18379006162331,
6.95286388617765));
#135988=CARTESIAN_POINT('Ctrl Pts',(-2.03850584321999,4.18650992790924,
6.95753315333298));
#135989=CARTESIAN_POINT('Ctrl Pts',(-1.99087453841738,4.19466138435571,
6.97137084369471));
#135990=CARTESIAN_POINT('Ctrl Pts',(-1.95906505357515,4.20008900935301,
6.98037657298076));
#135991=CARTESIAN_POINT('Ctrl Pts',(-1.86356284657613,4.2163361933017,7.0067103780558));
#135992=CARTESIAN_POINT('Ctrl Pts',(-1.79969087995045,4.22713823017249,
7.0233874035499));
#135993=CARTESIAN_POINT('Ctrl Pts',(-1.6077998448799,4.25939963184753,7.07070041929629));
#135994=CARTESIAN_POINT('Ctrl Pts',(-1.47928066971532,4.28067055419012,
7.0986991046817));
#135995=CARTESIAN_POINT('Ctrl Pts',(-1.3500506490493,4.30202682560965,7.12319193038323));
#135996=CARTESIAN_POINT('Ctrl Pts',(-2.854054357,4.302796438,6.664598542));
#135997=CARTESIAN_POINT('Ctrl Pts',(-2.493191391,4.238074114,6.81913486));
#135998=CARTESIAN_POINT('Ctrl Pts',(-2.117752007,4.172899507,6.933803173));
#135999=CARTESIAN_POINT('Ctrl Pts',(-2.10486940628411,4.17066314482125,
6.93773783237272));
#136000=CARTESIAN_POINT('Ctrl Pts',(-2.09198680556821,4.16842678264244,
6.94167249174543));
#136001=CARTESIAN_POINT('Ctrl Pts',(-3.17764352088934,4.302796438,6.79413901620324));
#136002=CARTESIAN_POINT('Ctrl Pts',(-2.80976642583978,4.238074114,6.96619647104542));
#136003=CARTESIAN_POINT('Ctrl Pts',(-2.42546205857017,4.172899507,7.09752612644045));
#136004=CARTESIAN_POINT('Ctrl Pts',(-2.412275270162,4.17066314482125,7.10203249307303));
#136005=CARTESIAN_POINT('Ctrl Pts',(-2.3990884817538,4.16842678264244,7.10653885970545));
#136006=CARTESIAN_POINT('',(-2.84976291967314,4.30202682599171,6.66643467681058));
#136007=CARTESIAN_POINT('Origin',(0.056016144692978,4.16072142213443,-0.190425882582227));
#136008=CARTESIAN_POINT('Ctrl Pts',(-2.95010126893415,4.26310680820208,
6.8954262016237));
#136009=CARTESIAN_POINT('Ctrl Pts',(-2.93859325105434,4.26736775488116,
6.86912813973383));
#136010=CARTESIAN_POINT('Ctrl Pts',(-2.92707971648568,4.27169422776909,
6.84284301422454));
#136011=CARTESIAN_POINT('Ctrl Pts',(-2.91556036655634,4.27608953505766,
6.81657204049201));
#136012=CARTESIAN_POINT('Ctrl Pts',(-2.90458096871979,4.28027881896961,
6.79153247889068));
#136013=CARTESIAN_POINT('Ctrl Pts',(-2.89358663965223,4.28452899140393,
6.76650955559758));
#136014=CARTESIAN_POINT('Ctrl Pts',(-2.88261131919965,4.2888490834973,6.74149044156445));
#136015=CARTESIAN_POINT('Ctrl Pts',(-2.87163572320134,4.29316928405064,
6.71647069940297));
#136016=CARTESIAN_POINT('Ctrl Pts',(-2.86068564753187,4.29756059489377,
6.69145191373861));
#136017=CARTESIAN_POINT('Ctrl Pts',(-2.84976291926378,4.3020268255214,6.66643467296296));
#136018=CARTESIAN_POINT('Ctrl Pts',(-3.56576672243298,4.17158344184794,
6.31251705551099));
#136019=CARTESIAN_POINT('Ctrl Pts',(-3.56228479221649,4.17224147442397,
6.31447884125549));
#136020=CARTESIAN_POINT('Ctrl Pts',(-3.558802862,4.172899507,6.31644062700001));
#136021=CARTESIAN_POINT('Ctrl Pts',(-3.257786313,4.229787119,6.486039079));
#136022=CARTESIAN_POINT('Ctrl Pts',(-2.94200579,4.285714286,6.626243425));
#136023=CARTESIAN_POINT('Ctrl Pts',(-2.893860104,4.294241258,6.647619773));
#136024=CARTESIAN_POINT('Ctrl Pts',(-2.845408881,4.302795611,6.668294257));
#136025=CARTESIAN_POINT('Ctrl Pts',(-3.47257965967507,4.17158344184794,
6.64765062822451));
#136026=CARTESIAN_POINT('Ctrl Pts',(-3.46891304433754,4.17224147442397,
6.64956084111226));
#136027=CARTESIAN_POINT('Ctrl Pts',(-3.465246429,4.172899507,6.651471054));
#136028=CARTESIAN_POINT('Ctrl Pts',(-3.148263656,4.229787119,6.81661097799999));
#136029=CARTESIAN_POINT('Ctrl Pts',(-2.817013256,4.285714286,6.950858675));
#136030=CARTESIAN_POINT('Ctrl Pts',(-2.766508945,4.294241258,6.971326838));
#136031=CARTESIAN_POINT('Ctrl Pts',(-2.715712542,4.302795611,6.99105896000001));
#136032=CARTESIAN_POINT('Ctrl Pts',(-3.55880256580312,4.17289956297677,
6.31644079388295));
#136033=CARTESIAN_POINT('Ctrl Pts',(-3.42907978966191,4.1974152208008,6.3895290666609));
#136034=CARTESIAN_POINT('Ctrl Pts',(-3.29736278114992,4.22178367600239,
6.45847127992605));
#136035=CARTESIAN_POINT('Ctrl Pts',(-3.16405329923453,4.24593816410288,
6.52313319819443));
#136036=CARTESIAN_POINT('Ctrl Pts',(-3.09049910662304,4.259265527203,6.55881074432697));
#136037=CARTESIAN_POINT('Ctrl Pts',(-3.01646035691276,4.27252780772309,
6.59318611782242));
#136038=CARTESIAN_POINT('Ctrl Pts',(-2.94200579035202,4.28571428590791,
6.62624342520531));
#136039=CARTESIAN_POINT('Ctrl Pts',(-2.91137508270563,4.29113922027103,
6.63984324526649));
#136040=CARTESIAN_POINT('Ctrl Pts',(-2.88062613755849,4.29657697957941,
6.65324128930027));
#136041=CARTESIAN_POINT('Ctrl Pts',(-2.8497629196197,4.30202682581219,6.66643467675972));
#136042=CARTESIAN_POINT('Ctrl Pts',(-4.220019834,4.302796438,5.89524661));
#136043=CARTESIAN_POINT('Ctrl Pts',(-3.900814385,4.238074114,6.123744826));
#136044=CARTESIAN_POINT('Ctrl Pts',(-3.558802862,4.172899507,6.316440627));
#136045=CARTESIAN_POINT('Ctrl Pts',(-3.54706728522262,4.17066314490999,
6.3230526743003));
#136046=CARTESIAN_POINT('Ctrl Pts',(-3.53533170844517,4.16842678281997,
6.32966472160044));
#136047=CARTESIAN_POINT('Ctrl Pts',(-4.5638910363296,4.302796438,5.95219639508923));
#136048=CARTESIAN_POINT('Ctrl Pts',(-4.24160196994199,4.238074114,6.19931394307104));
#136049=CARTESIAN_POINT('Ctrl Pts',(-3.89451441912942,4.172899507,6.41018726365446));
#136050=CARTESIAN_POINT('Ctrl Pts',(-3.88260466660029,4.17066314490999,
6.41742304337996));
#136051=CARTESIAN_POINT('Ctrl Pts',(-3.87069491407125,4.16842678281997,
6.42465882310546));
#136052=CARTESIAN_POINT('',(-4.21622344309948,4.30202682597525,5.89796234949526));
#136053=CARTESIAN_POINT('Origin',(0.0956423205124818,4.16072145579759,-0.173931787777442));
#136054=CARTESIAN_POINT('Ctrl Pts',(-4.36344234639725,4.26310680820233,
6.10003040032616));
#136055=CARTESIAN_POINT('Ctrl Pts',(-4.34655007361737,4.26736775485972,
6.07682105633263));
#136056=CARTESIAN_POINT('Ctrl Pts',(-4.32965519414465,4.27169422775199,
6.05362553204985));
#136057=CARTESIAN_POINT('Ctrl Pts',(-4.31275767749974,4.27608953504627,
6.03044507880318));
#136058=CARTESIAN_POINT('Ctrl Pts',(-4.29665220633118,4.28027881897436,
6.0083511741612));
#136059=CARTESIAN_POINT('Ctrl Pts',(-4.28053572977285,4.28452899142628,
5.98627672859719));
#136060=CARTESIAN_POINT('Ctrl Pts',(-4.26443863631163,4.28884908353792,
5.96420191693393));
#136061=CARTESIAN_POINT('Ctrl Pts',(-4.24834113871776,4.29316928410953,
5.94212655106178));
#136062=CARTESIAN_POINT('Ctrl Pts',(-4.23226877044292,4.29756059497319,
5.92004663319214));
#136063=CARTESIAN_POINT('Ctrl Pts',(-4.21622344160556,4.30202682552111,
5.89796234547385));
#136064=CARTESIAN_POINT('Ctrl Pts',(-4.83940564834472,4.17158344184794,
5.39839947227737));
#136065=CARTESIAN_POINT('Ctrl Pts',(-4.83642684967236,4.17224147442397,
5.40106390463868));
#136066=CARTESIAN_POINT('Ctrl Pts',(-4.83344805100001,4.172899507,5.403728337));
#136067=CARTESIAN_POINT('Ctrl Pts',(-4.575927756,4.229787119,5.634071332));
#136068=CARTESIAN_POINT('Ctrl Pts',(-4.297669796,4.285714286,5.838881257));
#136069=CARTESIAN_POINT('Ctrl Pts',(-4.255245012,4.294241258,5.870107737));
#136070=CARTESIAN_POINT('Ctrl Pts',(-4.212370955,4.302795611,5.900714443));
#136071=CARTESIAN_POINT('Ctrl Pts',(-4.82044105921187,4.17158344184794,
5.74573027284353));
#136072=CARTESIAN_POINT('Ctrl Pts',(-4.81727080660594,4.17224147442397,
5.74838403992177));
#136073=CARTESIAN_POINT('Ctrl Pts',(-4.81410055400001,4.172899507,5.751037807));
#136074=CARTESIAN_POINT('Ctrl Pts',(-4.540028864,4.229787119,5.980458777));
#136075=CARTESIAN_POINT('Ctrl Pts',(-4.2453822,4.285714286,6.182776882));
#136076=CARTESIAN_POINT('Ctrl Pts',(-4.200458702,4.294241258,6.213623445));
#136077=CARTESIAN_POINT('Ctrl Pts',(-4.155091715,4.302795611,6.243813966));
#136078=CARTESIAN_POINT('Ctrl Pts',(-4.83344804756002,4.17289950774314,
5.40372834137236));
#136079=CARTESIAN_POINT('Ctrl Pts',(-4.82382348853918,4.17502562436276,
5.41233717634408));
#136080=CARTESIAN_POINT('Ctrl Pts',(-4.82082523943908,4.17568534815515,
5.41499827998668));
#136081=CARTESIAN_POINT('Ctrl Pts',(-4.8087363428629,4.17834651459899,5.42573711625745));
#136082=CARTESIAN_POINT('Ctrl Pts',(-4.80254121582195,4.17970788569747,
5.43122144101507));
#136083=CARTESIAN_POINT('Ctrl Pts',(-4.78393219541999,4.18379006156185,
5.44763860682258));
#136084=CARTESIAN_POINT('Ctrl Pts',(-4.77149014101508,4.18650992785334,
5.45853968456259));
#136085=CARTESIAN_POINT('Ctrl Pts',(-4.73407143490589,4.1946613843129,5.49109829800729));
#136086=CARTESIAN_POINT('Ctrl Pts',(-4.70898333589813,4.20008900932188,
5.51262813258871));
#136087=CARTESIAN_POINT('Ctrl Pts',(-4.63336514813262,4.21633619542157,
5.57662839111951));
#136088=CARTESIAN_POINT('Ctrl Pts',(-4.5823990272295,4.22713823126396,5.61858318778587));
#136089=CARTESIAN_POINT('Ctrl Pts',(-4.42810970281214,4.25939962410648,
5.7420962384294));
#136090=CARTESIAN_POINT('Ctrl Pts',(-4.32322521667029,4.28067054359089,
5.82147094945651));
#136091=CARTESIAN_POINT('Ctrl Pts',(-4.21622344427235,4.30202682562769,
5.89796235123299));
#136092=CARTESIAN_POINT('Ctrl Pts',(-5.388661875,4.302796438,4.85023949900001));
#136093=CARTESIAN_POINT('Ctrl Pts',(-5.126039633,4.238074114,5.142015289));
#136094=CARTESIAN_POINT('Ctrl Pts',(-4.83344805100001,4.172899507,5.403728337));
#136095=CARTESIAN_POINT('Ctrl Pts',(-4.82340824000853,4.17066314486255,
5.41270860060828));
#136096=CARTESIAN_POINT('Ctrl Pts',(-4.81336842901706,4.16842678272508,
5.42168886421645));
#136097=CARTESIAN_POINT('Ctrl Pts',(-5.73673607986641,4.302796438,4.83193568617792));
#136098=CARTESIAN_POINT('Ctrl Pts',(-5.47510492068605,4.238074114,5.1425583858957));
#136099=CARTESIAN_POINT('Ctrl Pts',(-5.181463613887,4.172899507,5.42311516817079));
#136100=CARTESIAN_POINT('Ctrl Pts',(-5.17138778327219,4.17066314486254,
5.43274202430646));
#136101=CARTESIAN_POINT('Ctrl Pts',(-5.1613119526574,4.16842678272508,5.44236888044202));
#136102=CARTESIAN_POINT('',(-5.38553804416647,4.30202682608494,4.85370785869225));
#136103=CARTESIAN_POINT('Origin',(0.130796620685834,4.16072143753726,-0.149305274772075));
#136104=CARTESIAN_POINT('Ctrl Pts',(-5.57275370959191,4.2631068065418,5.0194039576247));
#136105=CARTESIAN_POINT('Ctrl Pts',(-5.55126704606305,4.26736775488585,
5.00036857440293));
#136106=CARTESIAN_POINT('Ctrl Pts',(-5.52978080737595,4.27169422776882,
4.98134724825959));
#136107=CARTESIAN_POINT('Ctrl Pts',(-5.50829523230219,4.27608953519676,
4.96234120710692));
#136108=CARTESIAN_POINT('Ctrl Pts',(-5.4927902460748,4.27926139263606,4.9486255674139));
#136109=CARTESIAN_POINT('Ctrl Pts',(-5.47728190210849,4.2824699864591,4.93492215050233));
#136110=CARTESIAN_POINT('Ctrl Pts',(-5.46178013446649,4.285714286,4.92121979118411));
#136111=CARTESIAN_POINT('Ctrl Pts',(-5.45680768340001,4.2867549492618,4.9168245304209));
#136112=CARTESIAN_POINT('Ctrl Pts',(-5.45183604222683,4.28779988859445,
4.91242936939491));
#136113=CARTESIAN_POINT('Ctrl Pts',(-5.44686554586364,4.28884908281018,
4.90803394274152));
#136114=CARTESIAN_POINT('Ctrl Pts',(-5.42639884426299,4.29316928412718,
4.88993516967156));
#136115=CARTESIAN_POINT('Ctrl Pts',(-5.40595570935508,4.29756059498149,
4.87182655211498));
#136116=CARTESIAN_POINT('Ctrl Pts',(-5.38553804287315,4.30202682632576,
4.85370785966905));
#136117=CARTESIAN_POINT('Ctrl Pts',(-5.88675934464407,4.17158344184794,
4.23185872984859));
#136118=CARTESIAN_POINT('Ctrl Pts',(-5.88442296282203,4.17224147442397,
4.23510122292429));
#136119=CARTESIAN_POINT('Ctrl Pts',(-5.882086581,4.172899507,4.238343716));
#136120=CARTESIAN_POINT('Ctrl Pts',(-5.680103902,4.229787119,4.518660671));
#136121=CARTESIAN_POINT('Ctrl Pts',(-5.452379538,4.285714286,4.77849949));
#136122=CARTESIAN_POINT('Ctrl Pts',(-5.417659393,4.294241258,4.818115986));
#136123=CARTESIAN_POINT('Ctrl Pts',(-5.382367244,4.302795611,4.85722378));
#136124=CARTESIAN_POINT('Ctrl Pts',(-5.942903991763,4.17158344184794,4.57514595584757));
#136125=CARTESIAN_POINT('Ctrl Pts',(-5.9403783393815,4.17224147442397,4.57841918992378));
#136126=CARTESIAN_POINT('Ctrl Pts',(-5.937852687,4.172899507,4.581692424));
#136127=CARTESIAN_POINT('Ctrl Pts',(-5.719507368,4.229787119,4.864666971));
#136128=CARTESIAN_POINT('Ctrl Pts',(-5.475241792,4.285714286,5.125595314));
#136129=CARTESIAN_POINT('Ctrl Pts',(-5.43799968,4.294241258,5.165377926));
#136130=CARTESIAN_POINT('Ctrl Pts',(-5.40018341600001,4.302795611,5.20461517));
#136131=CARTESIAN_POINT('Ctrl Pts',(-5.88208638225256,4.17289956298542,
4.23834399206812));
#136132=CARTESIAN_POINT('Ctrl Pts',(-5.79504213826813,4.197415223681,4.35914630590836));
#136133=CARTESIAN_POINT('Ctrl Pts',(-5.70444709207052,4.22178368168539,
4.47702311374695));
#136134=CARTESIAN_POINT('Ctrl Pts',(-5.61060950626881,4.24593817251312,
4.59168389254803));
#136135=CARTESIAN_POINT('Ctrl Pts',(-5.55883415213957,4.25926553282117,
4.65494854685941));
#136136=CARTESIAN_POINT('Ctrl Pts',(-5.50607225823275,4.27252781056818,
4.71723484194515));
#136137=CARTESIAN_POINT('Ctrl Pts',(-5.45237953796616,4.28571428600831,
4.77849949003861));
#136138=CARTESIAN_POINT('Ctrl Pts',(-5.43029027710596,4.29113922040459,
4.80370385236194));
#136139=CARTESIAN_POINT('Ctrl Pts',(-5.40800898232443,4.2965769798951,4.82877473577457));
#136140=CARTESIAN_POINT('Ctrl Pts',(-5.38553804393672,4.30202682606781,
4.85370785848893));
#136141=CARTESIAN_POINT('Ctrl Pts',(-6.305336075,4.302796438,3.57844058));
#136142=CARTESIAN_POINT('Ctrl Pts',(-6.111576965,4.238074114,3.919850833));
#136143=CARTESIAN_POINT('Ctrl Pts',(-5.882086581,4.172899507,4.238343716));
#136144=CARTESIAN_POINT('Ctrl Pts',(-5.87421198671132,4.1706631449394,4.24927228822925));
#136145=CARTESIAN_POINT('Ctrl Pts',(-5.86633739242265,4.16842678287881,
4.26020086045845));
#136146=CARTESIAN_POINT('Ctrl Pts',(-6.6413377196824,4.302796438,3.48573903474629));
#136147=CARTESIAN_POINT('Ctrl Pts',(-6.45259804968316,4.238074114,3.84534251319503));
#136148=CARTESIAN_POINT('Ctrl Pts',(-6.22613332948798,4.172899507,4.18246423546578));
#136149=CARTESIAN_POINT('Ctrl Pts',(-6.21836255599781,4.1706631449394,4.19403202642291));
#136150=CARTESIAN_POINT('Ctrl Pts',(-6.21059178250765,4.16842678287881,
4.20559981738003));
#136151=CARTESIAN_POINT('',(-6.3030308728385,4.30202682607316,3.58249938071131));
#136152=CARTESIAN_POINT('Origin',(0.159834808439206,4.16072143984921,-0.117697143487096));
#136153=CARTESIAN_POINT('Ctrl Pts',(-6.52148930321773,4.26310680820184,
3.70407576429898));
#136154=CARTESIAN_POINT('Ctrl Pts',(-6.49641294089323,4.26736775487178,
3.69010441533625));
#136155=CARTESIAN_POINT('Ctrl Pts',(-6.47134001560251,4.27169422777064,
3.67614670344654));
#136156=CARTESIAN_POINT('Ctrl Pts',(-6.44627102503695,4.27608953507197,
3.66220377698965));
#136157=CARTESIAN_POINT('Ctrl Pts',(-6.42237710548024,4.28027881899269,
3.64891440411782));
#136158=CARTESIAN_POINT('Ctrl Pts',(-6.3984813683556,4.28452899143848,3.63564731287308));
#136159=CARTESIAN_POINT('Ctrl Pts',(-6.37460306918202,4.28884908356176,
3.62237175053091));
#136160=CARTESIAN_POINT('Ctrl Pts',(-6.35072417052129,4.29316928414502,
3.60909585489328));
#136161=CARTESIAN_POINT('Ctrl Pts',(-6.32686616717162,4.29756059498849,
3.59580527662949));
#136162=CARTESIAN_POINT('Ctrl Pts',(-6.30303086975177,4.30202682552141,
3.58249937757921));
#136163=CARTESIAN_POINT('Ctrl Pts',(-6.65885471669918,4.17158344184794,
2.86744097718168));
#136164=CARTESIAN_POINT('Ctrl Pts',(-6.65726999834959,4.17224147442397,
2.87110991559084));
#136165=CARTESIAN_POINT('Ctrl Pts',(-6.65568528,4.172899507,2.874778854));
#136166=CARTESIAN_POINT('Ctrl Pts',(-6.518684703,4.229787119,3.191962459));
#136167=CARTESIAN_POINT('Ctrl Pts',(-6.352142073,4.285714286,3.494680397));
#136168=CARTESIAN_POINT('Ctrl Pts',(-6.326750041,4.294241258,3.540834488));
#136169=CARTESIAN_POINT('Ctrl Pts',(-6.300690023,4.302795611,3.586614732));
#136170=CARTESIAN_POINT('Ctrl Pts',(-6.78748333890467,4.17158344184794,
3.19063289841924));
#136171=CARTESIAN_POINT('Ctrl Pts',(-6.78572038345234,4.17224147442397,
3.19437254670962));
#136172=CARTESIAN_POINT('Ctrl Pts',(-6.783957428,4.172899507,3.198112195));
#136173=CARTESIAN_POINT('Ctrl Pts',(-6.631548065,4.229787119,3.521408744));
#136174=CARTESIAN_POINT('Ctrl Pts',(-6.449085162,4.285714286,3.828746606));
#136175=CARTESIAN_POINT('Ctrl Pts',(-6.421265836,4.294241258,3.875605075));
#136176=CARTESIAN_POINT('Ctrl Pts',(-6.392768543,4.302795611,3.922054354));
#136177=CARTESIAN_POINT('Ctrl Pts',(-6.65568527858334,4.17289950772645,
2.87477885888926));
#136178=CARTESIAN_POINT('Ctrl Pts',(-6.65056502153285,4.17502562427833,
2.8866332729685));
#136179=CARTESIAN_POINT('Ctrl Pts',(-6.64896125271127,4.1756853480929,2.89030735746956));
#136180=CARTESIAN_POINT('Ctrl Pts',(-6.6424987876089,4.17834651454824,2.90512965729521));
#136181=CARTESIAN_POINT('Ctrl Pts',(-6.63917905077847,4.17970788564625,
2.91270836196509));
#136182=CARTESIAN_POINT('Ctrl Pts',(-6.6291833502722,4.18379006150965,2.93542190296867));
#136183=CARTESIAN_POINT('Ctrl Pts',(-6.62246849125797,4.18650992780003,
2.95053973621401));
#136184=CARTESIAN_POINT('Ctrl Pts',(-6.60217920028303,4.19466138425825,
2.99580084035583));
#136185=CARTESIAN_POINT('Ctrl Pts',(-6.58845000118158,4.20008900926453,
3.02587500834143));
#136186=CARTESIAN_POINT('Ctrl Pts',(-6.54669380299953,4.21633619562176,
3.11571132414243));
#136187=CARTESIAN_POINT('Ctrl Pts',(-6.51805456655974,4.22713823132758,
3.17518858420653));
#136188=CARTESIAN_POINT('Ctrl Pts',(-6.42988713789993,4.25939962926024,
3.3520704264618));
#136189=CARTESIAN_POINT('Ctrl Pts',(-6.3680251256942,4.28067055054578,3.46814882480474));
#136190=CARTESIAN_POINT('Ctrl Pts',(-6.30303087435391,4.30202682552899,
3.58249938167426));
#136191=CARTESIAN_POINT('Ctrl Pts',(-6.927179768,4.302796438,2.139317756));
#136192=CARTESIAN_POINT('Ctrl Pts',(-6.811343751,4.238074114,2.514398508));
#136193=CARTESIAN_POINT('Ctrl Pts',(-6.65568528000001,4.172899507,2.874778854));
#136194=CARTESIAN_POINT('Ctrl Pts',(-6.65034410928241,4.17066314491703,
2.88714472743355));
#136195=CARTESIAN_POINT('Ctrl Pts',(-6.64500293856484,4.16842678283405,
2.89951060086715));
#136196=CARTESIAN_POINT('Ctrl Pts',(-7.23539778916921,4.302796438,1.97655309987432));
#136197=CARTESIAN_POINT('Ctrl Pts',(-7.12837486615929,4.238074114,2.36832269907274));
#136198=CARTESIAN_POINT('Ctrl Pts',(-6.9796759695216,4.172899507,2.7462459230242));
#136199=CARTESIAN_POINT('Ctrl Pts',(-6.97457360543338,4.17066314491702,
2.75921375217153));
#136200=CARTESIAN_POINT('Ctrl Pts',(-6.96947124134512,4.16842678283406,
2.77218158131886));
#136201=CARTESIAN_POINT('',(-6.92580098261212,4.3020268259686,2.14377721513266));
#136202=CARTESIAN_POINT('Origin',(0.181399492165553,4.16072144628749,-0.0805857300572521));
#136203=CARTESIAN_POINT('Ctrl Pts',(-7.16528730494324,4.26310680820237,
2.21554910463716));
#136204=CARTESIAN_POINT('Ctrl Pts',(-7.13779378704632,4.26736775490308,
2.20729507488378));
#136205=CARTESIAN_POINT('Ctrl Pts',(-7.11030655738358,4.27169422779421,
2.19905362431567));
#136206=CARTESIAN_POINT('Ctrl Pts',(-7.08282634888507,4.27608953508727,
2.19082576765599));
#136207=CARTESIAN_POINT('Ctrl Pts',(-7.05663423357179,4.28027881900277,
2.18298357932531));
#136208=CARTESIAN_POINT('Ctrl Pts',(-7.03044513306719,4.28452899143874,
2.17516354243805));
#136209=CARTESIAN_POINT('Ctrl Pts',(-7.0042712418177,4.28884908356817,2.16733148377025));
#136210=CARTESIAN_POINT('Ctrl Pts',(-6.97809669344815,4.29316928415757,
2.15949922847128));
#136211=CARTESIAN_POINT('Ctrl Pts',(-6.95193939554079,4.29756059500922,
2.15164814193842));
#136212=CARTESIAN_POINT('Ctrl Pts',(-6.92580098108579,4.30202682519232,
2.14377721262106));
#136213=CARTESIAN_POINT('Ctrl Pts',(-7.11958944241024,4.17158344184794,
1.36894487045972));
#136214=CARTESIAN_POINT('Ctrl Pts',(-7.11883048720513,4.17224147442397,
1.37286869872986));
#136215=CARTESIAN_POINT('Ctrl Pts',(-7.118071532,4.172899507,1.376792527));
#136216=CARTESIAN_POINT('Ctrl Pts',(-7.052459052,4.229787119,1.71601163));
#136217=CARTESIAN_POINT('Ctrl Pts',(-6.954885505,4.285714286,2.047453934));
#136218=CARTESIAN_POINT('Ctrl Pts',(-6.94000889,4.294241258,2.097987503));
#136219=CARTESIAN_POINT('Ctrl Pts',(-6.924399539,4.302795611,2.148299564));
#136220=CARTESIAN_POINT('Ctrl Pts',(-7.31468750940415,4.17158344184794,
1.65692939362537));
#136221=CARTESIAN_POINT('Ctrl Pts',(-7.31376968470208,4.17224147442397,
1.66096059431268));
#136222=CARTESIAN_POINT('Ctrl Pts',(-7.31285186,4.172899507,1.664991795));
#136223=CARTESIAN_POINT('Ctrl Pts',(-7.233504944,4.229787119,2.013493357));
#136224=CARTESIAN_POINT('Ctrl Pts',(-7.121376478,4.285714286,2.352869961));
#136225=CARTESIAN_POINT('Ctrl Pts',(-7.104280738,4.294241258,2.404613239));
#136226=CARTESIAN_POINT('Ctrl Pts',(-7.08643491800001,4.302795611,2.456102635));
#136227=CARTESIAN_POINT('Ctrl Pts',(-7.11807146745239,4.17289956296434,
1.37679286071363));
#136228=CARTESIAN_POINT('Ctrl Pts',(-7.08979582541024,4.19741522461937,
1.52297900648501));
#136229=CARTESIAN_POINT('Ctrl Pts',(-7.05706917398433,4.22178368355328,
1.66800097785143));
#136230=CARTESIAN_POINT('Ctrl Pts',(-7.02004929737975,4.24593817527534,
1.81146566714692));
#136231=CARTESIAN_POINT('Ctrl Pts',(-6.99962339875592,4.25926553464218,
1.89062301364352));
#136232=CARTESIAN_POINT('Ctrl Pts',(-6.9778913386645,4.27252781145132,1.96930666269499));
#136233=CARTESIAN_POINT('Ctrl Pts',(-6.95488550517666,4.2857142859596,2.04745393395531));
#136234=CARTESIAN_POINT('Ctrl Pts',(-6.94542087204743,4.29113922043585,
2.07960383435806));
#136235=CARTESIAN_POINT('Ctrl Pts',(-6.93572590721988,4.29657697986723,
2.11171322429797));
#136236=CARTESIAN_POINT('Ctrl Pts',(-6.92580098234181,4.30202682588361,
2.14377721466289));
#136237=CARTESIAN_POINT('Ctrl Pts',(-7.225116234,4.302796438,0.600162811));
#136238=CARTESIAN_POINT('Ctrl Pts',(-7.19261967400001,4.238074114,0.991375703));
#136239=CARTESIAN_POINT('Ctrl Pts',(-7.118071532,4.172899507,1.376792527));
#136240=CARTESIAN_POINT('Ctrl Pts',(-7.11551353207835,4.17066314489725,
1.39001748712837));
#136241=CARTESIAN_POINT('Ctrl Pts',(-7.11295553215668,4.1684267827945,1.40324244725675));
#136242=CARTESIAN_POINT('Ctrl Pts',(-7.49113869911339,4.302796438,0.374945738428264));
#136243=CARTESIAN_POINT('Ctrl Pts',(-7.47083679599638,4.238074114,0.780562747110289));
#136244=CARTESIAN_POINT('Ctrl Pts',(-7.40685671966933,4.172899507,1.18161620345787));
#136245=CARTESIAN_POINT('Ctrl Pts',(-7.40466134597066,4.17066314489725,
1.19537770954496));
#136246=CARTESIAN_POINT('Ctrl Pts',(-7.40246597227197,4.1684267827945,1.20913921563204));
#136247=CARTESIAN_POINT('',(-7.2247283364511,4.30202682595718,0.604814408909641));
#136248=CARTESIAN_POINT('Origin',(0.194481632606994,4.1607214752105,-0.0397060957560117));
#136249=CARTESIAN_POINT('Ctrl Pts',(-7.47404443578633,4.26310680820214,
0.623425831514019));
#136250=CARTESIAN_POINT('Ctrl Pts',(-7.44541932874542,4.26736775483642,
0.621275069824007));
#136251=CARTESIAN_POINT('Ctrl Pts',(-7.41680306703337,4.27169422772008,
0.619135241647022));
#136252=CARTESIAN_POINT('Ctrl Pts',(-7.38819658462309,4.2760895350054,0.617007180217377));
#136253=CARTESIAN_POINT('Ctrl Pts',(-7.36093098775278,4.28027881891818,
0.614978868444409));
#136254=CARTESIAN_POINT('Ctrl Pts',(-7.33367309711141,4.28452899135015,
0.612971542138589));
#136255=CARTESIAN_POINT('Ctrl Pts',(-7.30642747581962,4.288849083484,0.610949205513844));
#136256=CARTESIAN_POINT('Ctrl Pts',(-7.27918117050091,4.29316928407784,
0.608926818116439));
#136257=CARTESIAN_POINT('Ctrl Pts',(-7.25194766417651,4.29756059492796,
0.606882331437864));
#136258=CARTESIAN_POINT('Ctrl Pts',(-7.22472833267039,4.3020268255214,0.604814407460073));
#136259=CARTESIAN_POINT('Ctrl Pts',(-7.24742007933239,4.17158344184794,
-0.193561576570007));
#136260=CARTESIAN_POINT('Ctrl Pts',(-7.24752237516619,4.17224147442397,
-0.189566332285004));
#136261=CARTESIAN_POINT('Ctrl Pts',(-7.247624671,4.172899507,-0.185571088));
#136262=CARTESIAN_POINT('Ctrl Pts',(-7.256468254,4.229787119,0.159822005));
#136263=CARTESIAN_POINT('Ctrl Pts',(-7.23242622,4.285714286,0.5044908));
#136264=CARTESIAN_POINT('Ctrl Pts',(-7.22876063600001,4.294241258,0.557040955));
#136265=CARTESIAN_POINT('Ctrl Pts',(-7.224331829,4.302795611,0.609532297));
#136266=CARTESIAN_POINT('Ctrl Pts',(-7.4998650209685,4.17158344184794,0.0457497107196035));
#136267=CARTESIAN_POINT('Ctrl Pts',(-7.49983524348425,4.17224147442397,
0.0498839693598018));
#136268=CARTESIAN_POINT('Ctrl Pts',(-7.499805466,4.172899507,0.054018228));
#136269=CARTESIAN_POINT('Ctrl Pts',(-7.497231171,4.229787119,0.411429259));
#136270=CARTESIAN_POINT('Ctrl Pts',(-7.460680145,4.285714286,0.766975733));
#136271=CARTESIAN_POINT('Ctrl Pts',(-7.455107369,4.294241258,0.82118436));
#136272=CARTESIAN_POINT('Ctrl Pts',(-7.448747472,4.302795611,0.875306286));
#136273=CARTESIAN_POINT('Ctrl Pts',(-7.24762467222106,4.17289950769165,
-0.185571082742715));
#136274=CARTESIAN_POINT('Ctrl Pts',(-7.24795519204109,4.17502562416708,
-0.172662368237618));
#136275=CARTESIAN_POINT('Ctrl Pts',(-7.24804235892694,4.17568534802917,
-0.168654454115379));
#136276=CARTESIAN_POINT('Ctrl Pts',(-7.24840090660423,4.17834651449988,
-0.152488580367354));
#136277=CARTESIAN_POINT('Ctrl Pts',(-7.24857021054988,4.17970788559751,
-0.144216412981057));
#136278=CARTESIAN_POINT('Ctrl Pts',(-7.24903552678746,4.18379006146066,
-0.119405075762955));
#136279=CARTESIAN_POINT('Ctrl Pts',(-7.24928909921507,4.1865099277502,-0.102865005793642));
#136280=CARTESIAN_POINT('Ctrl Pts',(-7.24987968178903,4.19466138420899,
-0.0532678880350508));
#136281=CARTESIAN_POINT('Ctrl Pts',(-7.25004721352457,4.200089009213,-0.0202085713368787));
#136282=CARTESIAN_POINT('Ctrl Pts',(-7.2498716043712,4.2163361945907,0.0788576272574867));
#136283=CARTESIAN_POINT('Ctrl Pts',(-7.24885319079528,4.22713823077996,
0.144863032802135));
#136284=CARTESIAN_POINT('Ctrl Pts',(-7.24310535697581,4.25939963221318,
0.342417208870289));
#136285=CARTESIAN_POINT('Ctrl Pts',(-7.23570096849353,4.28067055518881,
0.473742302818427));
#136286=CARTESIAN_POINT('Ctrl Pts',(-7.22472833839899,4.30202682550461,
0.604814409146449));
#136287=CARTESIAN_POINT('Ctrl Pts',(-7.185214296,4.302796438,-0.967055079));
#136288=CARTESIAN_POINT('Ctrl Pts',(-7.237576694,4.238074114,-0.578002727000001));
#136289=CARTESIAN_POINT('Ctrl Pts',(-7.247624671,4.172899507,-0.185571088));
#136290=CARTESIAN_POINT('Ctrl Pts',(-7.24796945123017,4.17066314479459,
-0.172105425128183));
#136291=CARTESIAN_POINT('Ctrl Pts',(-7.24831423146048,4.16842678258919,
-0.158639762256362));
#136292=CARTESIAN_POINT('Ctrl Pts',(-7.39660228961032,4.302796438,-1.24419366777359));
#136293=CARTESIAN_POINT('Ctrl Pts',(-7.46397070149007,4.238074114,-0.843695450120858));
#136294=CARTESIAN_POINT('Ctrl Pts',(-7.48770108087874,4.172899507,-0.438264575817995));
#136295=CARTESIAN_POINT('Ctrl Pts',(-7.48851535082266,4.17066314479459,
-0.424352865016336));
#136296=CARTESIAN_POINT('Ctrl Pts',(-7.48932962076643,4.16842678258918,
-0.410441154214679));
#136297=CARTESIAN_POINT('',(-7.18583542224986,4.30202682602123,-0.962428846804123));
#136298=CARTESIAN_POINT('Origin',(0.198470723781902,4.16072144092381,0.00303002836568644));
#136299=CARTESIAN_POINT('Ctrl Pts',(-7.43332355589999,4.26310680820188,
-0.997848140191728));
#136300=CARTESIAN_POINT('Ctrl Pts',(-7.40490533771934,4.26736775491181,
-0.993795066420131));
#136301=CARTESIAN_POINT('Ctrl Pts',(-7.3764981084869,4.27169422779882,-0.989733216274674));
#136302=CARTESIAN_POINT('Ctrl Pts',(-7.34810295942663,4.27608953509018,
-0.985661976730497));
#136303=CARTESIAN_POINT('Ctrl Pts',(-7.32103878997482,4.28027881900884,
-0.981781570374166));
#136304=CARTESIAN_POINT('Ctrl Pts',(-7.2939866578393,4.28452899145251,-0.977882325800221));
#136305=CARTESIAN_POINT('Ctrl Pts',(-7.26694328144623,4.28884908358092,
-0.974000378013041));
#136306=CARTESIAN_POINT('Ctrl Pts',(-7.23989922610386,4.2931692841693,-0.970118332765922));
#136307=CARTESIAN_POINT('Ctrl Pts',(-7.21286291982685,4.29756059502628,
-0.966260621572241));
#136308=CARTESIAN_POINT('Ctrl Pts',(-7.18583541843999,4.30202682552111,
-0.962428847399571));
#136309=CARTESIAN_POINT('Ctrl Pts',(-7.03636940770779,4.17158344184794,
-1.7470172992385));
#136310=CARTESIAN_POINT('Ctrl Pts',(-7.0373281713539,4.17224147442397,-1.74313745211925));
#136311=CARTESIAN_POINT('Ctrl Pts',(-7.038286935,4.172899507,-1.739257605));
#136312=CARTESIAN_POINT('Ctrl Pts',(-7.121173066,4.229787119,-1.403840719));
#136313=CARTESIAN_POINT('Ctrl Pts',(-7.171786724,4.285714286,-1.062061763));
#136314=CARTESIAN_POINT('Ctrl Pts',(-7.179503569,4.294241258,-1.009952209));
#136315=CARTESIAN_POINT('Ctrl Pts',(-7.186462392,4.302795611,-0.957736023));
#136316=CARTESIAN_POINT('Ctrl Pts',(-7.33435717978959,4.17158344184794,
-1.56756917649812));
#136317=CARTESIAN_POINT('Ctrl Pts',(-7.33521684189479,4.17224147442397,
-1.56352517324906));
#136318=CARTESIAN_POINT('Ctrl Pts',(-7.336076504,4.172899507,-1.55948117));
#136319=CARTESIAN_POINT('Ctrl Pts',(-7.410395202,4.229787119,-1.209872813));
#136320=CARTESIAN_POINT('Ctrl Pts',(-7.4511307,4.285714286,-0.854781429));
#136321=CARTESIAN_POINT('Ctrl Pts',(-7.457341465,4.294241258,-0.800642187));
#136322=CARTESIAN_POINT('Ctrl Pts',(-7.462764873,4.302795611,-0.746418412));
#136323=CARTESIAN_POINT('Ctrl Pts',(-7.03828701704771,4.17289956295234,
-1.73925727478107));
#136324=CARTESIAN_POINT('Ctrl Pts',(-7.07400671165685,4.19741522660035,
-1.59470967625666));
#136325=CARTESIAN_POINT('Ctrl Pts',(-7.10519795470142,4.22178368756786,
-1.44934972323286));
#136326=CARTESIAN_POINT('Ctrl Pts',(-7.13183888559359,4.2459381813504,-1.30360044244046));
#136327=CARTESIAN_POINT('Ctrl Pts',(-7.14653814647385,4.25926553867801,
-1.22318258053661));
#136328=CARTESIAN_POINT('Ctrl Pts',(-7.15985306735223,4.2725278134871,-1.14264619181022));
#136329=CARTESIAN_POINT('Ctrl Pts',(-7.17178672404415,4.28571428603967,
-1.06206176275147));
#136330=CARTESIAN_POINT('Ctrl Pts',(-7.17669624850512,4.29113922041278,
-1.02890920747046));
#136331=CARTESIAN_POINT('Ctrl Pts',(-7.18137971989326,4.29657697980703,
-0.995696704394958));
#136332=CARTESIAN_POINT('Ctrl Pts',(-7.18583542232086,4.30202682589502,
-0.962428846792947));
#136333=CARTESIAN_POINT('Ctrl Pts',(-6.809339722,4.302796438,-2.489054549));
#136334=CARTESIAN_POINT('Ctrl Pts',(-6.944112672,4.238074114,-2.120354393));
#136335=CARTESIAN_POINT('Ctrl Pts',(-7.03828693500001,4.172899507,-1.739257605));
#136336=CARTESIAN_POINT('Ctrl Pts',(-7.04151837395981,4.17066314477596,
-1.72618087926869));
#136337=CARTESIAN_POINT('Ctrl Pts',(-7.04474981291962,4.16842678255194,
-1.71310415353744));
#136338=CARTESIAN_POINT('Ctrl Pts',(-6.95620897777936,4.302796438,-2.80515596191518));
#136339=CARTESIAN_POINT('Ctrl Pts',(-7.10809763203523,4.238074114,-2.42850338715821));
#136340=CARTESIAN_POINT('Ctrl Pts',(-7.21842886209782,4.172899507,-2.03765259113535));
#136341=CARTESIAN_POINT('Ctrl Pts',(-7.22221470149757,4.17066314477596,
-2.02424117224549));
#136342=CARTESIAN_POINT('Ctrl Pts',(-7.2260005408973,4.16842678255194,-2.01082975335561));
#136343=CARTESIAN_POINT('',(-6.81094083021135,4.30202682600845,-2.48466999876099));
#136344=CARTESIAN_POINT('Origin',(0.193179002053649,4.16072148814982,0.045624470169838));
#136345=CARTESIAN_POINT('Ctrl Pts',(-7.04502872801916,4.26310680820185,
-2.57246384252604));
#136346=CARTESIAN_POINT('Ctrl Pts',(-7.01814620294762,4.26736775489512,
-2.56239645050777));
#136347=CARTESIAN_POINT('Ctrl Pts',(-6.99127629662423,4.27169422777541,
-2.55232284955793));
#136348=CARTESIAN_POINT('Ctrl Pts',(-6.96442020648899,4.2760895350602,-2.54224267560679));
#136349=CARTESIAN_POINT('Ctrl Pts',(-6.93882295490606,4.28027881897259,
-2.53263499454347));
#136350=CARTESIAN_POINT('Ctrl Pts',(-6.91324150887699,4.28452899140873,
-2.52301150334713));
#136351=CARTESIAN_POINT('Ctrl Pts',(-6.88766489559402,4.28884908352697,
-2.51340678675703));
#136352=CARTESIAN_POINT('Ctrl Pts',(-6.86208764018609,4.2931692841052,-2.50380182903149));
#136353=CARTESIAN_POINT('Ctrl Pts',(-6.83651272154255,4.29756059496695,
-2.49422230234871));
#136354=CARTESIAN_POINT('Ctrl Pts',(-6.81094082624314,4.30202682552111,
-2.48466999852055));
#136355=CARTESIAN_POINT('Ctrl Pts',(-6.49630592356605,4.17158344184794,
-3.21878443522406));
#136356=CARTESIAN_POINT('Ctrl Pts',(-6.49807632428302,4.17224147442397,
-3.21520140261203));
#136357=CARTESIAN_POINT('Ctrl Pts',(-6.499846725,4.172899507,-3.21161837));
#136358=CARTESIAN_POINT('Ctrl Pts',(-6.652899739,4.229787119,-2.901861412));
#136359=CARTESIAN_POINT('Ctrl Pts',(-6.775802451,4.285714286,-2.578953498));
#136360=CARTESIAN_POINT('Ctrl Pts',(-6.794540894,4.294241258,-2.52972113));
#136361=CARTESIAN_POINT('Ctrl Pts',(-6.81256196000001,4.302795611,-2.480221671));
#136362=CARTESIAN_POINT('Ctrl Pts',(-6.82590294932948,4.17158344184794,
-3.10759027252605));
#136363=CARTESIAN_POINT('Ctrl Pts',(-6.82761185416474,4.17224147442397,
-3.10382561776302));
#136364=CARTESIAN_POINT('Ctrl Pts',(-6.829320759,4.172899507,-3.100060963));
#136365=CARTESIAN_POINT('Ctrl Pts',(-6.977057389,4.229787119,-2.774602578));
#136366=CARTESIAN_POINT('Ctrl Pts',(-7.093174665,4.285714286,-2.436569961));
#136367=CARTESIAN_POINT('Ctrl Pts',(-7.11087856200001,4.294241258,-2.385031595));
#136368=CARTESIAN_POINT('Ctrl Pts',(-7.127831683,4.302795611,-2.333241414));
#136369=CARTESIAN_POINT('Ctrl Pts',(-6.49984687581053,4.17289956305412,
-3.21161806478148));
#136370=CARTESIAN_POINT('Ctrl Pts',(-6.56580492407541,4.19741522640325,
-3.07812858848471));
#136371=CARTESIAN_POINT('Ctrl Pts',(-6.62751502573194,4.22178368708935,
-2.94287226689012));
#136372=CARTESIAN_POINT('Ctrl Pts',(-6.68486489301122,4.2459381806137,-2.80625753724418));
#136373=CARTESIAN_POINT('Ctrl Pts',(-6.7165079571281,4.25926553817461,-2.73087970544478));
#136374=CARTESIAN_POINT('Ctrl Pts',(-6.74682452604478,4.27252781322038,
-2.65508852572861));
#136375=CARTESIAN_POINT('Ctrl Pts',(-6.77580245114839,4.28571428601294,
-2.57895349787146));
#136376=CARTESIAN_POINT('Ctrl Pts',(-6.78772401284233,4.291139220383,-2.54763143360634));
#136377=CARTESIAN_POINT('Ctrl Pts',(-6.79943769358361,4.29657697979264,
-2.51620222834178));
#136378=CARTESIAN_POINT('Ctrl Pts',(-6.81094083028747,4.30202682596771,
-2.48466999878171));
#136379=CARTESIAN_POINT('Ctrl Pts',(-6.115067991,4.302796438,-3.894668594));
#136380=CARTESIAN_POINT('Ctrl Pts',(-6.32594966,4.238074114,-3.563560643));
#136381=CARTESIAN_POINT('Ctrl Pts',(-6.499846725,4.172899507,-3.21161837));
#136382=CARTESIAN_POINT('Ctrl Pts',(-6.50581372401252,4.17066314484168,
-3.19954203509781));
#136383=CARTESIAN_POINT('Ctrl Pts',(-6.5117807230249,4.16842678268336,-3.18746570019562));
#136384=CARTESIAN_POINT('Ctrl Pts',(-6.19055106550287,4.302796438,-4.23495228059749));
#136385=CARTESIAN_POINT('Ctrl Pts',(-6.41985781636945,4.238074114,-3.89975720418037));
#136386=CARTESIAN_POINT('Ctrl Pts',(-6.61163093230066,4.172899507,-3.5417622357951));
#136387=CARTESIAN_POINT('Ctrl Pts',(-6.61821131934391,4.17066314484168,
-3.5294782123538));
#136388=CARTESIAN_POINT('Ctrl Pts',(-6.62479170638728,4.16842678268338,
-3.51719418891246));
#136389=CARTESIAN_POINT('',(-6.1175742154234,4.30202682597258,-3.89073074407606));
#136390=CARTESIAN_POINT('Origin',(0.178854686864315,4.1607214229367,0.0860855762359175));
#136391=CARTESIAN_POINT('Ctrl Pts',(-6.32731618655374,4.26310680820184,
-4.02679399416409));
#136392=CARTESIAN_POINT('Ctrl Pts',(-6.30322635167546,4.2673677548649,-4.01118302401819));
#136393=CARTESIAN_POINT('Ctrl Pts',(-6.27915017526903,4.27169422775724,
-3.9955687026238));
#136394=CARTESIAN_POINT('Ctrl Pts',(-6.25508890503238,4.27608953505144,
-3.97995093197959));
#136395=CARTESIAN_POINT('Ctrl Pts',(-6.23215547048255,4.28027881895734,
-3.96506522073654));
#136396=CARTESIAN_POINT('Ctrl Pts',(-6.20924087068471,4.2845289913791,-3.95016746669878));
#136397=CARTESIAN_POINT('Ctrl Pts',(-6.18632695457098,4.28884908350346,
-3.93528908736913));
#136398=CARTESIAN_POINT('Ctrl Pts',(-6.16341246318179,4.29316928408781,
-3.92041033450374));
#136399=CARTESIAN_POINT('Ctrl Pts',(-6.14049478700705,4.29756059494739,
-3.90555692044372));
#136400=CARTESIAN_POINT('Ctrl Pts',(-6.11757421157827,4.30202682552139,
-3.8907307430016));
#136401=CARTESIAN_POINT('Ctrl Pts',(-5.6524823943449,4.17158344184794,-4.54004478794309));
#136402=CARTESIAN_POINT('Ctrl Pts',(-5.65498165017245,4.17224147442397,
-4.53692610847154));
#136403=CARTESIAN_POINT('Ctrl Pts',(-5.657480906,4.172899507,-4.533807429));
#136404=CARTESIAN_POINT('Ctrl Pts',(-5.873544215,4.229787119,-4.264194291));
#136405=CARTESIAN_POINT('Ctrl Pts',(-6.062989186,4.285714286,-3.975256234));
#136406=CARTESIAN_POINT('Ctrl Pts',(-6.091873039,4.294241258,-3.931203103));
#136407=CARTESIAN_POINT('Ctrl Pts',(-6.120113703,4.302795611,-3.88673491));
#136408=CARTESIAN_POINT('Ctrl Pts',(-5.9982770828366,4.17158344184794,-4.50230390039397));
#136409=CARTESIAN_POINT('Ctrl Pts',(-6.0007553239183,4.17224147442397,-4.49899462519698));
#136410=CARTESIAN_POINT('Ctrl Pts',(-6.003233565,4.172899507,-4.49568535));
#136411=CARTESIAN_POINT('Ctrl Pts',(-6.217480127,4.229787119,-4.20959501));
#136412=CARTESIAN_POINT('Ctrl Pts',(-6.403549666,4.285714286,-3.904427189));
#136413=CARTESIAN_POINT('Ctrl Pts',(-6.431918881,4.294241258,-3.857899576));
#136414=CARTESIAN_POINT('Ctrl Pts',(-6.45960900600001,4.302795611,-3.810964641));
#136415=CARTESIAN_POINT('Ctrl Pts',(-5.65748091034017,4.17289950777047,
-4.53380742519254));
#136416=CARTESIAN_POINT('Ctrl Pts',(-5.66555605643019,4.17502562434964,
-4.52373090866465));
#136417=CARTESIAN_POINT('Ctrl Pts',(-5.6680509353656,4.17568534813323,-4.52059298754607));
#136418=CARTESIAN_POINT('Ctrl Pts',(-5.67811954256308,4.17834651458591,
-4.50794043144338));
#136419=CARTESIAN_POINT('Ctrl Pts',(-5.68326042665598,4.17970788568245,
-4.50145747473345));
#136420=CARTESIAN_POINT('Ctrl Pts',(-5.69864604318714,4.18379006154285,
-4.48198693861613));
#136421=CARTESIAN_POINT('Ctrl Pts',(-5.70885753428319,4.18650992783038,
-4.4689729591054));
#136422=CARTESIAN_POINT('Ctrl Pts',(-5.73934258974514,4.19466138428471,
-4.42984644292587));
#136423=CARTESIAN_POINT('Ctrl Pts',(-5.75948260660457,4.20008900928439,
-4.40362953603836));
#136424=CARTESIAN_POINT('Ctrl Pts',(-5.81929511903045,4.21633619593903,
-4.32465734190559));
#136425=CARTESIAN_POINT('Ctrl Pts',(-5.85842913392724,4.22713823148072,
-4.27149458167131));
#136426=CARTESIAN_POINT('Ctrl Pts',(-5.97340800784085,4.25939963040738,
-4.11074464354552));
#136427=CARTESIAN_POINT('Ctrl Pts',(-6.04698798485694,4.28067055282548,
-4.00171670482559));
#136428=CARTESIAN_POINT('Ctrl Pts',(-6.11757421701856,4.30202682553039,
-3.89073074500549));
#136429=CARTESIAN_POINT('Ctrl Pts',(-5.134862478,4.302796438,-5.11817226500001));
#136430=CARTESIAN_POINT('Ctrl Pts',(-5.41199227200001,4.238074114,-4.840138759));
#136431=CARTESIAN_POINT('Ctrl Pts',(-5.657480906,4.172899507,-4.533807429));
#136432=CARTESIAN_POINT('Ctrl Pts',(-5.66590445502806,4.17066314481695,
-4.52329616037206));
#136433=CARTESIAN_POINT('Ctrl Pts',(-5.67432800405597,4.1684267826339,-4.51278489174419));
#136434=CARTESIAN_POINT('Ctrl Pts',(-5.13542986618061,4.302796438,-5.46672693770758));
#136435=CARTESIAN_POINT('Ctrl Pts',(-5.4314325856829,4.238074114,-5.18866270937467));
#136436=CARTESIAN_POINT('Ctrl Pts',(-5.69568048758393,4.172899507,-4.88026301484536));
#136437=CARTESIAN_POINT('Ctrl Pts',(-5.70474773082427,4.17066314481695,
-4.86968077360362));
#136438=CARTESIAN_POINT('Ctrl Pts',(-5.71381497406465,4.1684267826339,-4.85909853236175));
#136439=CARTESIAN_POINT('',(-5.13815662914318,4.30202682605394,-5.11486524284701));
#136440=CARTESIAN_POINT('Origin',(0.156167497269551,4.16072142532751,0.122521574995526));
#136441=CARTESIAN_POINT('Ctrl Pts',(-5.31374537287912,4.26310680820188,
-5.29283573461444));
#136442=CARTESIAN_POINT('Ctrl Pts',(-5.29357464216325,4.2673677548786,-5.27241113771949));
#136443=CARTESIAN_POINT('Ctrl Pts',(-5.27341797098531,4.2716942277604,-5.25198620429076));
#136444=CARTESIAN_POINT('Ctrl Pts',(-5.25327659895758,4.27608953504662,
-5.23156110664844));
#136445=CARTESIAN_POINT('Ctrl Pts',(-5.23407932319175,4.28027881897093,
-5.21209340447583));
#136446=CARTESIAN_POINT('Ctrl Pts',(-5.21490303063397,4.28452899142244,
-5.19261799002205));
#136447=CARTESIAN_POINT('Ctrl Pts',(-5.19572324093142,4.28884908354616,
-5.17316164412882));
#136448=CARTESIAN_POINT('Ctrl Pts',(-5.1765429697024,4.29316928412982,-5.15370480976592));
#136449=CARTESIAN_POINT('Ctrl Pts',(-5.15735414107386,4.29756059498671,
-5.13427203714466));
#136450=CARTESIAN_POINT('Ctrl Pts',(-5.13815662496132,4.3020268255211,-5.11486524163069));
#136451=CARTESIAN_POINT('Ctrl Pts',(-4.5443550709688,4.17158344184794,-5.64901769170602));
#136452=CARTESIAN_POINT('Ctrl Pts',(-4.5474663194844,4.17224147442397,-5.64650919135301));
#136453=CARTESIAN_POINT('Ctrl Pts',(-4.550577568,4.172899507,-5.644000691));
#136454=CARTESIAN_POINT('Ctrl Pts',(-4.819548292,4.229787119,-5.42713818300001));
#136455=CARTESIAN_POINT('Ctrl Pts',(-5.066677286,4.285714286,-5.185680407));
#136456=CARTESIAN_POINT('Ctrl Pts',(-5.104355971,4.294241258,-5.148866388));
#136457=CARTESIAN_POINT('Ctrl Pts',(-5.14149573100001,4.302795611,-5.111508744));
#136458=CARTESIAN_POINT('Ctrl Pts',(-4.8901784459381,4.17158344184794,-5.6864948022092));
#136459=CARTESIAN_POINT('Ctrl Pts',(-4.89331014346905,4.17224147442397,
-5.6837956446046));
#136460=CARTESIAN_POINT('Ctrl Pts',(-4.896441841,4.172899507,-5.681096487));
#136461=CARTESIAN_POINT('Ctrl Pts',(-5.167180404,4.229787119,-5.447751458));
#136462=CARTESIAN_POINT('Ctrl Pts',(-5.414501802,4.285714286,-5.189717742));
#136463=CARTESIAN_POINT('Ctrl Pts',(-5.452209822,4.294241258,-5.150376461));
#136464=CARTESIAN_POINT('Ctrl Pts',(-5.48934219,4.302795611,-5.110491397));
#136465=CARTESIAN_POINT('Ctrl Pts',(-4.55057757175014,4.17289950779316,
-5.64400068797639));
#136466=CARTESIAN_POINT('Ctrl Pts',(-4.81954829372672,4.22978711939077,
-5.42713818131292));
#136467=CARTESIAN_POINT('Ctrl Pts',(-5.066677286,4.285714286,-5.185680407));
#136468=CARTESIAN_POINT('Ctrl Pts',(-5.10266266459496,4.29385804992617,
-5.15052083571143));
#136469=CARTESIAN_POINT('Ctrl Pts',(-5.13815662986677,4.3020268261311,-5.11486524162382));
#136470=CARTESIAN_POINT('Ctrl Pts',(-3.914556502,4.302796438,-6.102355889));
#136471=CARTESIAN_POINT('Ctrl Pts',(-4.24497614,4.238074114,-5.890397365));
#136472=CARTESIAN_POINT('Ctrl Pts',(-4.550577568,4.172899507,-5.64400069100001));
#136473=CARTESIAN_POINT('Ctrl Pts',(-4.56106379122528,4.17066314481382,
-5.63554598402288));
#136474=CARTESIAN_POINT('Ctrl Pts',(-4.57155001445054,4.16842678262765,
-5.62709127704577));
#136475=CARTESIAN_POINT('Ctrl Pts',(-3.84018167302776,4.302796438,-6.44288351854466));
#136476=CARTESIAN_POINT('Ctrl Pts',(-4.18903960369835,4.238074114,-6.23495211221143));
#136477=CARTESIAN_POINT('Ctrl Pts',(-4.51340635488503,4.172899507,-5.9905681197649));
#136478=CARTESIAN_POINT('Ctrl Pts',(-4.52453648010094,4.17066314481382,
-5.98218247472962));
#136479=CARTESIAN_POINT('Ctrl Pts',(-4.53566660531688,4.16842678262766,
-5.9737968296945));
#136480=CARTESIAN_POINT('',(-3.91848454918051,4.30202682597578,-6.0998343282999));
#136481=CARTESIAN_POINT('Origin',(0.126177966822555,4.1607214641731,0.153228623991858));
#136482=CARTESIAN_POINT('Ctrl Pts',(-4.0517097311445,4.26310680820184,-6.31139035819562));
#136483=CARTESIAN_POINT('Ctrl Pts',(-4.03640126539844,4.26736775488148,
-6.28710716620262));
#136484=CARTESIAN_POINT('Ctrl Pts',(-4.02110660284375,4.27169422777429,
-6.26282666784151));
#136485=CARTESIAN_POINT('Ctrl Pts',(-4.00582691709567,4.2760895350694,-6.23854929794492));
#136486=CARTESIAN_POINT('Ctrl Pts',(-3.99126344352812,4.28027881897674,
-6.21540989307706));
#136487=CARTESIAN_POINT('Ctrl Pts',(-3.9767221205835,4.28452899140062,-6.19226746695518));
#136488=CARTESIAN_POINT('Ctrl Pts',(-3.96217328298514,4.28884908352118,
-6.16914291186207));
#136489=CARTESIAN_POINT('Ctrl Pts',(-3.94762408012453,4.29316928410171,
-6.14601777620528));
#136490=CARTESIAN_POINT('Ctrl Pts',(-3.93306134734588,4.29756059496636,
-6.1229143001681));
#136491=CARTESIAN_POINT('Ctrl Pts',(-3.91848454655754,4.3020268255211,-6.09983432616156));
#136492=CARTESIAN_POINT('Ctrl Pts',(-3.22373875465859,4.17158344184793,
-6.49384880706528));
#136493=CARTESIAN_POINT('Ctrl Pts',(-3.22731651732929,4.17224147442396,
-6.49206778053264));
#136494=CARTESIAN_POINT('Ctrl Pts',(-3.23089428,4.172899507,-6.490286754));
#136495=CARTESIAN_POINT('Ctrl Pts',(-3.540195646,4.229787119,-6.336315127));
#136496=CARTESIAN_POINT('Ctrl Pts',(-3.833453187,4.285714286,-6.153627927));
#136497=CARTESIAN_POINT('Ctrl Pts',(-3.878164891,4.294241258,-6.125774403));
#136498=CARTESIAN_POINT('Ctrl Pts',(-3.922467133,4.302795611,-6.097274111));
#136499=CARTESIAN_POINT('Ctrl Pts',(-3.55342050042447,4.17158344184793,
-6.60479152680991));
#136500=CARTESIAN_POINT('Ctrl Pts',(-3.55705921971224,4.17224147442396,
-6.60282869640496));
#136501=CARTESIAN_POINT('Ctrl Pts',(-3.560697939,4.172899507,-6.600865866));
#136502=CARTESIAN_POINT('Ctrl Pts',(-3.875269069,4.229787119,-6.431177102));
#136503=CARTESIAN_POINT('Ctrl Pts',(-4.172277851,4.285714286,-6.232342861));
#136504=CARTESIAN_POINT('Ctrl Pts',(-4.217561491,4.294241258,-6.202027467));
#136505=CARTESIAN_POINT('Ctrl Pts',(-4.262399835,4.302795611,-6.171057255));
#136506=CARTESIAN_POINT('Ctrl Pts',(-3.23089458435371,4.17289956251625,
-6.49028660284023));
#136507=CARTESIAN_POINT('Ctrl Pts',(-3.54019579132273,4.22978714684626,
-6.33631503609226));
#136508=CARTESIAN_POINT('Ctrl Pts',(-3.833453187,4.285714286,-6.153627927));
#136509=CARTESIAN_POINT('Ctrl Pts',(-3.876155517,4.29385805,-6.127026159));
#136510=CARTESIAN_POINT('Ctrl Pts',(-3.91848454655754,4.3020268255211,-6.09983432616156));
#136511=CARTESIAN_POINT('Ctrl Pts',(-2.511210214,4.302796438,-6.801200134));
#136512=CARTESIAN_POINT('Ctrl Pts',(-2.879469642,4.238074114,-6.665227538));
#136513=CARTESIAN_POINT('Ctrl Pts',(-3.23089428,4.172899507,-6.49028675400001));
#136514=CARTESIAN_POINT('Ctrl Pts',(-3.24295285297228,4.17066314486295,
-6.48428394150031));
#136515=CARTESIAN_POINT('Ctrl Pts',(-3.25501142594456,4.16842678272591,
-6.47828112900057));
#136516=CARTESIAN_POINT('Ctrl Pts',(-2.36537085379952,4.302796438,-7.11777802662557));
#136517=CARTESIAN_POINT('Ctrl Pts',(-2.75077178539864,4.238074114,-6.98970208423936));
#136518=CARTESIAN_POINT('Ctrl Pts',(-3.12009035661109,4.172899507,-6.82076091693253));
#136519=CARTESIAN_POINT('Ctrl Pts',(-3.1327629312101,4.17066314486295,-6.81496397165978));
#136520=CARTESIAN_POINT('Ctrl Pts',(-3.14543550580904,4.16842678272591,
-6.80916702638693));
#136521=CARTESIAN_POINT('',(-2.5155884870915,4.30202682598825,-6.7995819405079));
#136522=CARTESIAN_POINT('Origin',(0.0902882200923827,4.16072150620521,0.176770419752994));
#136523=CARTESIAN_POINT('Ctrl Pts',(-2.60022064565508,4.26310680820217,
-7.03483138315783));
#136524=CARTESIAN_POINT('Ctrl Pts',(-2.59049025192455,4.26736775487167,
-7.00782505119042));
#136525=CARTESIAN_POINT('Ctrl Pts',(-2.58077275948663,4.27169422775182,
-6.98082431713158));
#136526=CARTESIAN_POINT('Ctrl Pts',(-2.57106922114836,4.27608953503605,
-6.95382985797731));
#136527=CARTESIAN_POINT('Ctrl Pts',(-2.56182052148295,4.28027881894382,
-6.92810072323856));
#136528=CARTESIAN_POINT('Ctrl Pts',(-2.55259410397172,4.28452899137914,
-6.90237339964067));
#136529=CARTESIAN_POINT('Ctrl Pts',(-2.5433565058699,4.2888490834871,-6.87666191378213));
#136530=CARTESIAN_POINT('Ctrl Pts',(-2.53411867584956,4.29316928405502,
-6.85094978241272));
#136531=CARTESIAN_POINT('Ctrl Pts',(-2.52486297614486,4.2975605948876,-6.82525589570485));
#136532=CARTESIAN_POINT('Ctrl Pts',(-2.51558848481664,4.30202682552139,
-6.79958193754012));
#136533=CARTESIAN_POINT('Ctrl Pts',(-1.75238399671172,4.17158344184794,
-7.03503476980878));
#136534=CARTESIAN_POINT('Ctrl Pts',(-1.75626098135586,4.17224147442397,
-7.03406449590439));
#136535=CARTESIAN_POINT('Ctrl Pts',(-1.760137966,4.172899507,-7.033094222));
#136536=CARTESIAN_POINT('Ctrl Pts',(-2.095307388,4.229787119,-6.949213017));
#136537=CARTESIAN_POINT('Ctrl Pts',(-2.420981077,4.285714286,-6.833838645));
#136538=CARTESIAN_POINT('Ctrl Pts',(-2.470635131,4.294241258,-6.816248015));
#136539=CARTESIAN_POINT('Ctrl Pts',(-2.520028332,4.302795611,-6.797937717));
#136540=CARTESIAN_POINT('Ctrl Pts',(-2.05050856186381,4.17158344184794,
-7.21425554087441));
#136541=CARTESIAN_POINT('Ctrl Pts',(-2.0544841604319,4.17224147442397,-7.2131208174372));
#136542=CARTESIAN_POINT('Ctrl Pts',(-2.058459759,4.172899507,-7.211986094));
#136543=CARTESIAN_POINT('Ctrl Pts',(-2.402154459,4.229787119,-7.11388805300001));
#136544=CARTESIAN_POINT('Ctrl Pts',(-2.734962825,4.285714286,-6.983550554));
#136545=CARTESIAN_POINT('Ctrl Pts',(-2.785704672,4.294241258,-6.963678562));
#136546=CARTESIAN_POINT('Ctrl Pts',(-2.836152401,4.302795611,-6.943071335));
#136547=CARTESIAN_POINT('Ctrl Pts',(-1.76013829606613,4.17289956297316,
-7.03309413963776));
#136548=CARTESIAN_POINT('Ctrl Pts',(-1.90457922844313,4.19741522351749,
-6.99694560958115));
#136549=CARTESIAN_POINT('Ctrl Pts',(-2.04761672121439,4.22178368138733,
-6.9564156254032));
#136550=CARTESIAN_POINT('Ctrl Pts',(-2.18886678551531,4.24593817209426,
-6.91168302222974));
#136551=CARTESIAN_POINT('Ctrl Pts',(-2.26680221137891,4.25926553253887,
-6.88700158583135));
#136552=CARTESIAN_POINT('Ctrl Pts',(-2.34419392029766,4.27252781042464,
-6.8610415487873));
#136553=CARTESIAN_POINT('Ctrl Pts',(-2.42098107728448,4.28571428600471,
-6.83383864511283));
#136554=CARTESIAN_POINT('Ctrl Pts',(-2.45257142201105,4.29113922038427,
-6.82264733202966));
#136555=CARTESIAN_POINT('Ctrl Pts',(-2.48410884525471,4.2965769796734,-6.81122821862746));
#136556=CARTESIAN_POINT('Ctrl Pts',(-2.51558848703189,4.30202682577276,
-6.79958194024593));
#136557=CARTESIAN_POINT('Ctrl Pts',(-0.990442528,4.302796438,-7.182027819));
#136558=CARTESIAN_POINT('Ctrl Pts',(-1.379322344,4.238074114,-7.12839907900001));
#136559=CARTESIAN_POINT('Ctrl Pts',(-1.760137966,4.172899507,-7.033094222));
#136560=CARTESIAN_POINT('Ctrl Pts',(-1.77320504385938,4.17066314479498,
-7.0298239885462));
#136561=CARTESIAN_POINT('Ctrl Pts',(-1.7862721217187,4.16842678258996,-7.02655375509242));
#136562=CARTESIAN_POINT('Ctrl Pts',(-0.779957921281984,4.302796438,-7.45985314610527));
#136563=CARTESIAN_POINT('Ctrl Pts',(-1.1838809356057,4.238074114,-7.41762135551125));
#136564=CARTESIAN_POINT('Ctrl Pts',(-1.58088240025405,4.172899507,-7.33202251416165));
#136565=CARTESIAN_POINT('Ctrl Pts',(-1.59450486936809,4.17066314479498,
-7.32908532708222));
#136566=CARTESIAN_POINT('Ctrl Pts',(-1.60812733848218,4.16842678258996,
-7.32614814000278));
#136567=CARTESIAN_POINT('',(-0.995066304014444,4.30202682608954,-7.18138865763276));
#136568=CARTESIAN_POINT('Origin',(0.0501768802110265,4.16072148901941,0.192046736180631));
#136569=CARTESIAN_POINT('Ctrl Pts',(-1.02714813235652,4.26310680820184,
-7.42933151192896));
#136570=CARTESIAN_POINT('Ctrl Pts',(-1.02345079285982,4.26736775487571,
-7.40086482582209));
#136571=CARTESIAN_POINT('Ctrl Pts',(-1.01976484971036,4.27169422776037,
-7.37240638024215));
#136572=CARTESIAN_POINT('Ctrl Pts',(-1.0160911854935,4.2760895350484,-7.34395706258297));
#136573=CARTESIAN_POINT('Ctrl Pts',(-1.01258971872643,4.28027881895993,
-7.31684126362888));
#136574=CARTESIAN_POINT('Ctrl Pts',(-1.00910962384362,4.28452899139447,
-7.28973202347391));
#136575=CARTESIAN_POINT('Ctrl Pts',(-1.00561520513928,4.28884908349595,
-7.26263584728086));
#136576=CARTESIAN_POINT('Ctrl Pts',(-1.00212069870427,4.29316928405743,
-7.2355389908128));
#136577=CARTESIAN_POINT('Ctrl Pts',(-0.998604818079791,4.2975605949177,
-7.20845611103672));
#136578=CARTESIAN_POINT('Ctrl Pts',(-0.995066302196107,4.3020268255211,
-7.18138865409593));
#136579=CARTESIAN_POINT('Ctrl Pts',(-0.199089711805015,4.17158344184793,
-7.24727032571477));
#136580=CARTESIAN_POINT('Ctrl Pts',(-0.203084634902507,4.17224147442396,
-7.24715617335739));
#136581=CARTESIAN_POINT('Ctrl Pts',(-0.207079558,4.172899507,-7.247042021));
#136582=CARTESIAN_POINT('Ctrl Pts',(-0.552444884,4.229787119,-7.237173429));
#136583=CARTESIAN_POINT('Ctrl Pts',(-0.895306583,4.285714286,-7.194506663));
#136584=CARTESIAN_POINT('Ctrl Pts',(-0.947581218,4.294241258,-7.188001446));
#136585=CARTESIAN_POINT('Ctrl Pts',(-0.999755805999999,4.302795611,-7.180737311));
#136586=CARTESIAN_POINT('Ctrl Pts',(-0.451717121439883,4.17158344184793,
-7.48638898311077));
#136587=CARTESIAN_POINT('Ctrl Pts',(-0.455843704719942,4.17224147442396,
-7.48613542505538));
#136588=CARTESIAN_POINT('Ctrl Pts',(-0.459970288,4.172899507,-7.48588186700001));
#136589=CARTESIAN_POINT('Ctrl Pts',(-0.816717776000001,4.229787119,-7.46396150500001));
#136590=CARTESIAN_POINT('Ctrl Pts',(-1.169763977,4.285714286,-7.408215186));
#136591=CARTESIAN_POINT('Ctrl Pts',(-1.223591399,4.294241258,-7.399715786));
#136592=CARTESIAN_POINT('Ctrl Pts',(-1.277289632,4.302795611,-7.390435115));
#136593=CARTESIAN_POINT('Ctrl Pts',(-0.20707956336158,4.17289950774601,
-7.24704202165685));
#136594=CARTESIAN_POINT('Ctrl Pts',(-0.21998723992398,4.17502562418936,
-7.24667319304932));
#136595=CARTESIAN_POINT('Ctrl Pts',(-0.223993995176412,4.17568534804455,
-7.24654324800825));
#136596=CARTESIAN_POINT('Ctrl Pts',(-0.240155571671878,4.17834651451532,
-7.24602606710527));
#136597=CARTESIAN_POINT('Ctrl Pts',(-0.248424773146666,4.17970788561247,
-7.2457472766494));
#136598=CARTESIAN_POINT('Ctrl Pts',(-0.273224914126765,4.18379006147442,
-7.24486865177658));
#136599=CARTESIAN_POINT('Ctrl Pts',(-0.289754454797499,4.18650992776272,
-7.24422639100457));
#136600=CARTESIAN_POINT('Ctrl Pts',(-0.339310807627244,4.1946613842195,
-7.24213097367978));
#136601=CARTESIAN_POINT('Ctrl Pts',(-0.372330709975183,4.20008900922057,
-7.2405084644347));
#136602=CARTESIAN_POINT('Ctrl Pts',(-0.471242108456474,4.21633619398169,
-7.23496977729559));
#136603=CARTESIAN_POINT('Ctrl Pts',(-0.537095577453983,4.22713823046721,
-7.23037939677633));
#136604=CARTESIAN_POINT('Ctrl Pts',(-0.73404881608325,4.25939962768096,
-7.2139446275718));
#136605=CARTESIAN_POINT('Ctrl Pts',(-0.864780427711907,4.28067054765987,
-7.19944130409139));
#136606=CARTESIAN_POINT('Ctrl Pts',(-0.995066304340255,4.3020268256754,
-7.18138865949419));
#136607=CARTESIAN_POINT('Ctrl Pts',(0.57663715,4.302796438,-7.227031866));
#136608=CARTESIAN_POINT('Ctrl Pts',(0.185320533,4.238074114,-7.25825460100001));
#136609=CARTESIAN_POINT('Ctrl Pts',(-0.207079558,4.172899507,-7.247042021));
#136610=CARTESIAN_POINT('Ctrl Pts',(-0.220544138690441,4.1706631447385,
-7.24665727927435));
#136611=CARTESIAN_POINT('Ctrl Pts',(-0.234008719380881,4.16842678247702,
-7.24627253754872));
#136612=CARTESIAN_POINT('Ctrl Pts',(0.841924975632872,4.302796438,-7.45311382237723));
#136613=CARTESIAN_POINT('Ctrl Pts',(0.438366870732096,4.238074114,-7.49870089635587));
#136614=CARTESIAN_POINT('Ctrl Pts',(0.0322458591927978,4.172899507,-7.50044688815672));
#136615=CARTESIAN_POINT('Ctrl Pts',(0.0183104670882274,4.1706631447385,
-7.50050679906916));
#136616=CARTESIAN_POINT('Ctrl Pts',(0.00437507498365682,4.16842678247702,
-7.50056670998151));
#136617=CARTESIAN_POINT('',(0.571984074783619,4.30202682599323,-7.22740162258272));
#136618=CARTESIAN_POINT('Origin',(0.00771940334921756,4.16072144823275,
0.198343469846251));
#136619=CARTESIAN_POINT('Ctrl Pts',(0.593952685418298,4.26310680820187,
-7.47644435599597));
#136620=CARTESIAN_POINT('Ctrl Pts',(0.59144408727556,4.26736775488579,-7.44784838639655));
#136621=CARTESIAN_POINT('Ctrl Pts',(0.588926130551418,4.27169422777635,
-7.41926291457612));
#136622=CARTESIAN_POINT('Ctrl Pts',(0.586398144197795,4.27608953506819,
-7.39068899687837));
#136623=CARTESIAN_POINT('Ctrl Pts',(0.583988653383373,4.28027881897436,
-7.3634544383824));
#136624=CARTESIAN_POINT('Ctrl Pts',(0.581559700274735,4.2845289913987,-7.33623087966888));
#136625=CARTESIAN_POINT('Ctrl Pts',(0.579147544540272,4.28884908349961,
-7.30901700028622));
#136626=CARTESIAN_POINT('Ctrl Pts',(0.576735328246355,4.29316928406052,
-7.28180243767334));
#136627=CARTESIAN_POINT('Ctrl Pts',(0.574346991003685,4.29756059491905,
-7.25459693016561));
#136628=CARTESIAN_POINT('Ctrl Pts',(0.571984075604951,4.30202682552139,
-7.22740161874865));
#136629=CARTESIAN_POINT('Ctrl Pts',(1.36351378779211,4.17158344184794,-7.120631576332));
#136630=CARTESIAN_POINT('Ctrl Pts',(1.35958772439605,4.17224147442397,-7.121378883166));
#136631=CARTESIAN_POINT('Ctrl Pts',(1.355661661,4.172899507,-7.12212619));
#136632=CARTESIAN_POINT('Ctrl Pts',(1.016249329,4.229787119,-7.186731656));
#136633=CARTESIAN_POINT('Ctrl Pts',(0.672231452,4.285714286,-7.218767545));
#136634=CARTESIAN_POINT('Ctrl Pts',(0.619780539,4.294241258,-7.223651918));
#136635=CARTESIAN_POINT('Ctrl Pts',(0.56726419,4.302795611,-7.227773609));
#136636=CARTESIAN_POINT('Ctrl Pts',(1.16819610908937,4.17158344184794,-7.40846719817912));
#136637=CARTESIAN_POINT('Ctrl Pts',(1.16411149554469,4.17224147442397,-7.40910666158956));
#136638=CARTESIAN_POINT('Ctrl Pts',(1.160026882,4.172899507,-7.409746125));
#136639=CARTESIAN_POINT('Ctrl Pts',(0.806907722,4.229787119,-7.465028413));
#136640=CARTESIAN_POINT('Ctrl Pts',(0.450131734,4.285714286,-7.486479909));
#136641=CARTESIAN_POINT('Ctrl Pts',(0.395735648,4.294241258,-7.489750525));
#136642=CARTESIAN_POINT('Ctrl Pts',(0.34129778,4.302795611,-7.492230364));
#136643=CARTESIAN_POINT('Ctrl Pts',(1.35566132646284,4.1728995630705,-7.1221262536775));
#136644=CARTESIAN_POINT('Ctrl Pts',(1.20939187737991,4.19741522958354,-7.14996791590427));
#136645=CARTESIAN_POINT('Ctrl Pts',(1.06255643070428,4.2217836932938,-7.17324378695403));
#136646=CARTESIAN_POINT('Ctrl Pts',(0.915578576336522,4.24593818969773,
-7.19195494056951));
#136647=CARTESIAN_POINT('Ctrl Pts',(0.834482868858626,4.25926554423746,
-7.20227890567774));
#136648=CARTESIAN_POINT('Ctrl Pts',(0.753343755120934,4.27252781626317,
-7.21121414472586));
#136649=CARTESIAN_POINT('Ctrl Pts',(0.672231451661361,4.28571428604748,
-7.21876754508335));
#136650=CARTESIAN_POINT('Ctrl Pts',(0.638861721101172,4.29113922036799,
-7.22187502600129));
#136651=CARTESIAN_POINT('Ctrl Pts',(0.605444369423189,4.29657697969623,
-7.22475354016177));
#136652=CARTESIAN_POINT('Ctrl Pts',(0.571984074806843,4.302026825889,-7.22740162309087));
#136653=CARTESIAN_POINT('Ctrl Pts',(2.116753915,4.302796438,-6.934107936));
#136654=CARTESIAN_POINT('Ctrl Pts',(1.741298029,4.238074114,-7.048722205));
#136655=CARTESIAN_POINT('Ctrl Pts',(1.355661661,4.172899507,-7.12212619));
#136656=CARTESIAN_POINT('Ctrl Pts',(1.34242916693796,4.17066314479019,-7.12464493012992));
#136657=CARTESIAN_POINT('Ctrl Pts',(1.32919667287593,4.16842678258039,-7.12716367025997));
#136658=CARTESIAN_POINT('Ctrl Pts',(2.42444039675729,4.302796438,-7.09787518030707));
#136659=CARTESIAN_POINT('Ctrl Pts',(2.04011712962238,4.238074114,-7.22914951711653));
#136660=CARTESIAN_POINT('Ctrl Pts',(1.64386633789201,4.172899507,-7.31815870169129));
#136661=CARTESIAN_POINT('Ctrl Pts',(1.63026962688718,4.17066314479019,-7.32121290924037));
#136662=CARTESIAN_POINT('Ctrl Pts',(1.61667291588234,4.16842678258039,-7.32426711678959));
#136663=CARTESIAN_POINT('',(2.11228911235521,4.30202682605736,-6.93546932111101));
#136664=CARTESIAN_POINT('Origin',(-0.035099148622541,4.16072145763487,0.195366131088097));
#136665=CARTESIAN_POINT('Ctrl Pts',(2.1872809357983,4.26310680658203,-7.17396697110051));
#136666=CARTESIAN_POINT('Ctrl Pts',(2.17868369939943,4.26736775489131,-7.14657883414244));
#136667=CARTESIAN_POINT('Ctrl Pts',(2.17007957965209,4.27169422777959,-7.11920296110774));
#136668=CARTESIAN_POINT('Ctrl Pts',(2.16146814827941,4.27608953521548,-7.09184052727085));
#136669=CARTESIAN_POINT('Ctrl Pts',(2.15525374053094,4.27926139264596,-7.07209452762295));
#136670=CARTESIAN_POINT('Ctrl Pts',(2.14903015416925,4.28246998646097,-7.05235727007208));
#136671=CARTESIAN_POINT('Ctrl Pts',(2.14281165749886,4.285714286,-7.03262430918845));
#136672=CARTESIAN_POINT('Ctrl Pts',(2.14081697072266,4.28675494926488,-7.02629463208906));
#136673=CARTESIAN_POINT('Ctrl Pts',(2.13882292648665,4.28779988860438,-7.01996545799532));
#136674=CARTESIAN_POINT('Ctrl Pts',(2.13683000013097,4.28884908283037,-7.01363664650976));
#136675=CARTESIAN_POINT('Ctrl Pts',(2.12862385216706,4.2931692841448,-6.98757689606371));
#136676=CARTESIAN_POINT('Ctrl Pts',(2.12044297297646,4.29756059502454,-6.96152086016398));
#136677=CARTESIAN_POINT('Ctrl Pts',(2.11228911061973,4.30202682639742,-6.93546932209822));
#136678=CARTESIAN_POINT('Ctrl Pts',(2.86236089767707,4.17158344184794,-6.66104000740502));
#136679=CARTESIAN_POINT('Ctrl Pts',(2.85868727233853,4.17224147442397,-6.66261383020251));
#136680=CARTESIAN_POINT('Ctrl Pts',(2.855013647,4.172899507,-6.664187653));
#136681=CARTESIAN_POINT('Ctrl Pts',(2.537424852,4.229787119,-6.800246298));
#136682=CARTESIAN_POINT('Ctrl Pts',(2.208336691,4.285714286,-6.905486881));
#136683=CARTESIAN_POINT('Ctrl Pts',(2.158162048,4.294241258,-6.92153245500001));
#136684=CARTESIAN_POINT('Ctrl Pts',(2.107759543,4.302795611,-6.936847246));
#136685=CARTESIAN_POINT('Ctrl Pts',(2.73348578762687,4.17158344184794,-6.98413372045932));
#136686=CARTESIAN_POINT('Ctrl Pts',(2.72963413581344,4.17224147442397,-6.98563630472967));
#136687=CARTESIAN_POINT('Ctrl Pts',(2.725782484,4.172899507,-6.987138889));
#136688=CARTESIAN_POINT('Ctrl Pts',(2.392803112,4.229787119,-7.117038888));
#136689=CARTESIAN_POINT('Ctrl Pts',(2.048979786,4.285714286,-7.214685152));
#136690=CARTESIAN_POINT('Ctrl Pts',(1.996558536,4.294241258,-7.229572853));
#136691=CARTESIAN_POINT('Ctrl Pts',(1.943926487,4.302795611,-7.243697248));
#136692=CARTESIAN_POINT('Ctrl Pts',(2.85501333397931,4.17289956286129,-6.66418778679595));
#136693=CARTESIAN_POINT('Ctrl Pts',(2.53742468986878,4.22978714683597,-6.80024635016384));
#136694=CARTESIAN_POINT('Ctrl Pts',(2.208336691,4.285714286,-6.905486881));
#136695=CARTESIAN_POINT('Ctrl Pts',(2.16041693,4.29385805,-6.920811357));
#136696=CARTESIAN_POINT('Ctrl Pts',(2.11228911319059,4.30202682552139,-6.93546931684795));
#136697=CARTESIAN_POINT('Ctrl Pts',(3.55789362,4.302796438,-6.316952824));
#136698=CARTESIAN_POINT('Ctrl Pts',(3.215854364,4.238074114,-6.509599393));
#136699=CARTESIAN_POINT('Ctrl Pts',(2.855013647,4.172899507,-6.664187653));
#136700=CARTESIAN_POINT('Ctrl Pts',(2.84263197655568,4.17066314489563,-6.66949210119473));
#136701=CARTESIAN_POINT('Ctrl Pts',(2.83025030611137,4.16842678279126,-6.67479654938961));
#136702=CARTESIAN_POINT('Ctrl Pts',(3.8935916797487,4.302796438,-6.41074778369885));
#136703=CARTESIAN_POINT('Ctrl Pts',(3.54647377862577,4.238074114,-6.62157114079839));
#136704=CARTESIAN_POINT('Ctrl Pts',(3.17862145369182,4.172899507,-6.79368154768867));
#136705=CARTESIAN_POINT('Ctrl Pts',(3.16599919116732,4.17066314489563,-6.79958724024984));
#136706=CARTESIAN_POINT('Ctrl Pts',(3.15337692864277,4.16842678279128,-6.80549293281101));
#136707=CARTESIAN_POINT('',(3.55382586057344,4.30202682596346,-6.31924218176628));
#136708=CARTESIAN_POINT('Origin',(-0.0762763638463032,4.16072146698572,
0.183253025037982));
#136709=CARTESIAN_POINT('Ctrl Pts',(3.67833436109219,4.26310680820193,-6.53604286415009));
#136710=CARTESIAN_POINT('Ctrl Pts',(3.66405048306734,4.26736775486722,-6.51114319839327));
#136711=CARTESIAN_POINT('Ctrl Pts',(3.64976251940713,4.2716942277443,-6.48625698950045));
#136712=CARTESIAN_POINT('Ctrl Pts',(3.63547030455461,4.27608953502506,-6.46138547817639));
#136713=CARTESIAN_POINT('Ctrl Pts',(3.62184801560651,4.28027881894025,-6.4376797812408));
#136714=CARTESIAN_POINT('Ctrl Pts',(3.60821268185684,4.28452899137762,-6.41399223943781));
#136715=CARTESIAN_POINT('Ctrl Pts',(3.59459665732802,4.28884908351028,-6.39030642927422));
#136716=CARTESIAN_POINT('Ctrl Pts',(3.5809802909561,4.2931692841029,-6.36662002445608));
#136717=CARTESIAN_POINT('Ctrl Pts',(3.56738939858886,4.29756059496313,-6.34293181137133));
#136718=CARTESIAN_POINT('Ctrl Pts',(3.55382585953241,4.30202682552139,-6.31924217758476));
#136719=CARTESIAN_POINT('Ctrl Pts',(4.22736719328809,4.17158344184794,-5.8899856118872));
#136720=CARTESIAN_POINT('Ctrl Pts',(4.22411778064405,4.17224147442397,-5.8923123604436));
#136721=CARTESIAN_POINT('Ctrl Pts',(4.220868368,4.172899507,-5.89463910900001));
#136722=CARTESIAN_POINT('Ctrl Pts',(3.939953209,4.229787119,-6.095788982));
#136723=CARTESIAN_POINT('Ctrl Pts',(3.641182561,4.285714286,-6.269313324));
#136724=CARTESIAN_POINT('Ctrl Pts',(3.595630297,4.294241258,-6.29576982800001));
#136725=CARTESIAN_POINT('Ctrl Pts',(3.549698402,4.302795611,-6.321561615));
#136726=CARTESIAN_POINT('Ctrl Pts',(4.17096070925658,4.17158344184794,-6.23322991204395));
#136727=CARTESIAN_POINT('Ctrl Pts',(4.16752211812829,4.17224147442397,-6.23552535802198));
#136728=CARTESIAN_POINT('Ctrl Pts',(4.164083527,4.172899507,-6.237820804));
#136729=CARTESIAN_POINT('Ctrl Pts',(3.866813688,4.229787119,-6.436264536));
#136730=CARTESIAN_POINT('Ctrl Pts',(3.55201982,4.285714286,-6.605539735));
#136731=CARTESIAN_POINT('Ctrl Pts',(3.504024566,4.294241258,-6.63134839));
#136732=CARTESIAN_POINT('Ctrl Pts',(3.455659352,4.302795611,-6.656456899));
#136733=CARTESIAN_POINT('Ctrl Pts',(4.22086836419622,4.17289950772743,-5.89463911285146));
#136734=CARTESIAN_POINT('Ctrl Pts',(4.21036944622223,4.17502562429124,-5.90215688440212));
#136735=CARTESIAN_POINT('Ctrl Pts',(4.20710105665032,4.175685348168,-5.90447822109222));
#136736=CARTESIAN_POINT('Ctrl Pts',(4.19392195323513,4.17834651461355,-5.91384706622864));
#136737=CARTESIAN_POINT('Ctrl Pts',(4.18717018248245,4.17970788571012,-5.91862943058245));
#136738=CARTESIAN_POINT('Ctrl Pts',(4.16689524109046,4.18379006157001,-5.9329383692362));
#136739=CARTESIAN_POINT('Ctrl Pts',(4.15334750871452,4.18650992785742,-5.94243032167265));
#136740=CARTESIAN_POINT('Ctrl Pts',(4.11262794730963,4.1946613843096,-5.97075240133703));
#136741=CARTESIAN_POINT('Ctrl Pts',(4.08535913123871,4.20008900930932,-5.98944352643003));
#136742=CARTESIAN_POINT('Ctrl Pts',(4.00326457661388,4.21633619514749,-6.04489284753308));
#136743=CARTESIAN_POINT('Ctrl Pts',(3.94806110930445,4.22713823109094,-6.08109129674243));
#136744=CARTESIAN_POINT('Ctrl Pts',(3.78132209108869,4.25939963061046,-6.18719871994207));
#136745=CARTESIAN_POINT('Ctrl Pts',(3.66847050410133,4.28067055425272,-6.25476813660489));
#136746=CARTESIAN_POINT('Ctrl Pts',(3.55382586154031,4.3020268255718,-6.31924218361524));
#136747=CARTESIAN_POINT('Ctrl Pts',(4.832670174,4.302796438,-5.40442402));
#136748=CARTESIAN_POINT('Ctrl Pts',(4.540040923,4.238074114,-5.666094949));
#136749=CARTESIAN_POINT('Ctrl Pts',(4.220868368,4.172899507,-5.894639109));
#136750=CARTESIAN_POINT('Ctrl Pts',(4.20991647333625,4.17066314482088,-5.90248123554604));
#136751=CARTESIAN_POINT('Ctrl Pts',(4.19896457867244,4.16842678264175,-5.91032336209221));
#136752=CARTESIAN_POINT('Ctrl Pts',(5.18068294323162,4.302796438,-5.42386094580911));
#136753=CARTESIAN_POINT('Ctrl Pts',(4.88700125593113,4.238074114,-5.7043754577779));
#136754=CARTESIAN_POINT('Ctrl Pts',(4.56474776398164,4.172899507,-5.95153939466388));
#136755=CARTESIAN_POINT('Ctrl Pts',(4.55369015190452,4.17066314482088,-5.96002042901051));
#136756=CARTESIAN_POINT('Ctrl Pts',(4.54263253982728,4.16842678264174,-5.96850146335713));
#136757=CARTESIAN_POINT('',(4.82918966053496,4.30202682607914,-5.4075343008958));
#136758=CARTESIAN_POINT('Origin',(-0.113887094330756,4.16072143125059,0.162571574944076));
#136759=CARTESIAN_POINT('Ctrl Pts',(4.99739295987823,4.26310680820187,-5.5925006574533));
#136760=CARTESIAN_POINT('Ctrl Pts',(4.97809033885805,4.26736775488714,-5.57125374342459));
#136761=CARTESIAN_POINT('Ctrl Pts',(4.9587866205154,4.27169422777249,-5.55002085012781));
#136762=CARTESIAN_POINT('Ctrl Pts',(4.93948190990831,4.27608953505775,-5.52880322466369));
#136763=CARTESIAN_POINT('Ctrl Pts',(4.92108207837028,4.28027881897154,-5.50858014325509));
#136764=CARTESIAN_POINT('Ctrl Pts',(4.90267340981735,4.28452899140277,-5.48837759677755));
#136765=CARTESIAN_POINT('Ctrl Pts',(4.88428397121445,4.2888490835086,-5.46817259061411));
#136766=CARTESIAN_POINT('Ctrl Pts',(4.8658940709274,4.29316928407441,-5.44796707718501));
#136767=CARTESIAN_POINT('Ctrl Pts',(4.84752866049303,4.29756059493458,-5.42775432148553));
#136768=CARTESIAN_POINT('Ctrl Pts',(4.82918965923875,4.3020268255211,-5.40753429774623));
#136769=CARTESIAN_POINT('Ctrl Pts',(5.39470649704281,4.17158344184794,-4.84352203473393));
#136770=CARTESIAN_POINT('Ctrl Pts',(5.39203323602141,4.17224147442397,-4.84649291286697));
#136771=CARTESIAN_POINT('Ctrl Pts',(5.389359975,4.172899507,-4.849463791));
#136772=CARTESIAN_POINT('Ctrl Pts',(5.158253733,4.229787119,-5.106299347));
#136773=CARTESIAN_POINT('Ctrl Pts',(4.903770781,4.285714286,-5.339993645));
#136774=CARTESIAN_POINT('Ctrl Pts',(4.86497087,4.294241258,-5.37562400000001));
#136775=CARTESIAN_POINT('Ctrl Pts',(4.825657309,4.302795611,-5.41068678999999));
#136776=CARTESIAN_POINT('Ctrl Pts',(5.41340614349393,4.17158344184794,-5.19086720064895));
#136777=CARTESIAN_POINT('Ctrl Pts',(5.41054139774697,4.17224147442397,-5.19384817582448));
#136778=CARTESIAN_POINT('Ctrl Pts',(5.40767665200001,4.172899507,-5.196829151));
#136779=CARTESIAN_POINT('Ctrl Pts',(5.160016353,4.229787119,-5.454537607));
#136780=CARTESIAN_POINT('Ctrl Pts',(4.888971356,4.285714286,-5.687526623));
#136781=CARTESIAN_POINT('Ctrl Pts',(4.847646301,4.294241258,-5.723049447));
#136782=CARTESIAN_POINT('Ctrl Pts',(4.805809426,4.302795611,-5.75796802300001));
#136783=CARTESIAN_POINT('Ctrl Pts',(5.389359747424,4.17289956286129,-4.84946404403705));
#136784=CARTESIAN_POINT('Ctrl Pts',(5.15825360814972,4.22978714684751,-5.10629946169107));
#136785=CARTESIAN_POINT('Ctrl Pts',(4.903770781,4.285714286,-5.339993645));
#136786=CARTESIAN_POINT('Ctrl Pts',(4.866714564,4.29385805,-5.374022748));
#136787=CARTESIAN_POINT('Ctrl Pts',(4.82918965923875,4.3020268255211,-5.40753429774623));
#136788=CARTESIAN_POINT('Ctrl Pts',(5.881476442,4.302796438,-4.239190355));
#136789=CARTESIAN_POINT('Ctrl Pts',(5.651940215,4.238074114,-4.557650202));
#136790=CARTESIAN_POINT('Ctrl Pts',(5.389359975,4.172899507,-4.84946379100001));
#136791=CARTESIAN_POINT('Ctrl Pts',(5.38034995519343,4.17066314488853,-4.85947690629275));
#136792=CARTESIAN_POINT('Ctrl Pts',(5.37133993538672,4.16842678277707,-4.86949002158551));
#136793=CARTESIAN_POINT('Ctrl Pts',(6.22553122981452,4.302796438,-4.18336039794204));
#136794=CARTESIAN_POINT('Ctrl Pts',(5.99901798618111,4.238074114,-4.52044951809392));
#136795=CARTESIAN_POINT('Ctrl Pts',(5.73743154150416,4.172899507,-4.83110987552454));
#136796=CARTESIAN_POINT('Ctrl Pts',(5.7284556221902,4.17066314488853,-4.84176968744937));
#136797=CARTESIAN_POINT('Ctrl Pts',(5.71947970287635,4.16842678277705,-4.85242949937412));
#136798=CARTESIAN_POINT('',(5.87874591915956,4.30202682596213,-4.242976127138));
#136799=CARTESIAN_POINT('Origin',(-0.146172589532412,4.16072141476489,0.134288418613644));
#136800=CARTESIAN_POINT('Ctrl Pts',(6.08277901778227,4.26310680820167,-4.38745933518201));
#136801=CARTESIAN_POINT('Ctrl Pts',(6.05936022279369,4.26736775488834,-4.37085865528994));
#136802=CARTESIAN_POINT('Ctrl Pts',(6.03594337023099,4.2716942277768,-4.35427190405316));
#136803=CARTESIAN_POINT('Ctrl Pts',(6.01252883073701,4.27608953506782,-4.33770027700124));
#136804=CARTESIAN_POINT('Ctrl Pts',(5.99021181229749,4.28027881899059,-4.32190541985338));
#136805=CARTESIAN_POINT('Ctrl Pts',(5.96789057786926,4.28452899143785,-4.30613251721398));
#136806=CARTESIAN_POINT('Ctrl Pts',(5.94558759502439,4.28884908355563,-4.2903530785531));
#136807=CARTESIAN_POINT('Ctrl Pts',(5.92328405224215,4.29316928413338,-4.27457324373456));
#136808=CARTESIAN_POINT('Ctrl Pts',(5.90100286981083,4.29756059498866,-4.25878107146336));
#136809=CARTESIAN_POINT('Ctrl Pts',(5.87874591645362,4.30202682552206,-4.24297612382547));
#136810=CARTESIAN_POINT('Ctrl Pts',(6.30979532136944,4.17158344184794,-3.57058075049655));
#136811=CARTESIAN_POINT('Ctrl Pts',(6.30782321068473,4.17224147442397,-3.57405684324828));
#136812=CARTESIAN_POINT('Ctrl Pts',(6.3058511,4.172899507,-3.577532936));
#136813=CARTESIAN_POINT('Ctrl Pts',(6.135360046,4.229787119,-3.87804483));
#136814=CARTESIAN_POINT('Ctrl Pts',(5.93706413,4.285714286,-4.160981797));
#136815=CARTESIAN_POINT('Ctrl Pts',(5.906830812,4.294241258,-4.204119968));
#136816=CARTESIAN_POINT('Ctrl Pts',(5.875973844,4.302795611,-4.246814263));
#136817=CARTESIAN_POINT('Ctrl Pts',(6.40272672408439,4.17158344184794,-3.90578530842664));
#136818=CARTESIAN_POINT('Ctrl Pts',(6.4005697760422,4.17224147442397,-3.90931242571332));
#136819=CARTESIAN_POINT('Ctrl Pts',(6.398412828,4.172899507,-3.912839543));
#136820=CARTESIAN_POINT('Ctrl Pts',(6.211942389,4.229787119,-4.217762562));
#136821=CARTESIAN_POINT('Ctrl Pts',(5.997320024,4.285714286,-4.503571086));
#136822=CARTESIAN_POINT('Ctrl Pts',(5.964597484,4.294241258,-4.547147072));
#136823=CARTESIAN_POINT('Ctrl Pts',(5.931245193,4.302795611,-4.590242963));
#136824=CARTESIAN_POINT('Ctrl Pts',(6.30585109805129,4.17289950775651,-3.57753294115029));
#136825=CARTESIAN_POINT('Ctrl Pts',(6.29947916846551,4.17502562433408,-3.58876426714043));
#136826=CARTESIAN_POINT('Ctrl Pts',(6.29748756240345,4.17568534821138,-3.59224341642849));
#136827=CARTESIAN_POINT('Ctrl Pts',(6.28946040807777,4.17834651465004,-3.60628011185563));
#136828=CARTESIAN_POINT('Ctrl Pts',(6.28534072957839,4.17970788574548,-3.6134554631478));
#136829=CARTESIAN_POINT('Ctrl Pts',(6.27294785853963,4.1837900616024,-3.63495513108321));
#136830=CARTESIAN_POINT('Ctrl Pts',(6.26463783703034,4.18650992788744,-3.64925833897672));
#136831=CARTESIAN_POINT('Ctrl Pts',(6.23957389659969,4.19466138433422,-3.69206046238253));
#136832=CARTESIAN_POINT('Ctrl Pts',(6.22267358914811,4.20008900932887,-3.72047394676422));
#136833=CARTESIAN_POINT('Ctrl Pts',(6.17144914928316,4.21633619694954,-3.80526900580106));
#136834=CARTESIAN_POINT('Ctrl Pts',(6.13654717623975,4.2271382319934,-3.86130115791271));
#136835=CARTESIAN_POINT('Ctrl Pts',(6.02977230827358,4.25939962672662,-4.02761351906478));
#136836=CARTESIAN_POINT('Ctrl Pts',(5.95572265761057,4.28067054646697,-4.13632299277107));
#136837=CARTESIAN_POINT('Ctrl Pts',(5.87874592074033,4.30202682557444,-4.24297612835655));
#136838=CARTESIAN_POINT('Ctrl Pts',(6.655271408,4.302796438,-2.87573686));
#136839=CARTESIAN_POINT('Ctrl Pts',(6.499561064,4.238074114,-3.236094797));
#136840=CARTESIAN_POINT('Ctrl Pts',(6.30585110000001,4.172899507,-3.577532936));
#136841=CARTESIAN_POINT('Ctrl Pts',(6.29920425302589,4.17066314480995,-3.58924883854929));
#136842=CARTESIAN_POINT('Ctrl Pts',(6.29255740605191,4.16842678261991,-3.60096474109857));
#136843=CARTESIAN_POINT('Ctrl Pts',(6.97928059608469,4.302796438,-2.74725056763748));
#136844=CARTESIAN_POINT('Ctrl Pts',(6.83052730232644,4.238074114,-3.12515238362164));
#136845=CARTESIAN_POINT('Ctrl Pts',(6.64183939664013,4.172899507,-3.48478302660876));
#136846=CARTESIAN_POINT('Ctrl Pts',(6.63536487354871,4.17066314480995,-3.49712317577696));
#136847=CARTESIAN_POINT('Ctrl Pts',(6.62889035045719,4.16842678261991,-3.50946332494515));
#136848=CARTESIAN_POINT('',(6.65341855241806,4.30202682601949,-2.88002110588503));
#136849=CARTESIAN_POINT('Origin',(-0.171623230891431,4.16072138151534,0.0997260640717268));
#136850=CARTESIAN_POINT('Ctrl Pts',(6.88374108930325,4.26310680659847,-2.97726529110235));
#136851=CARTESIAN_POINT('Ctrl Pts',(6.85730115750649,4.26736775493315,-2.96608707433597));
#136852=CARTESIAN_POINT('Ctrl Pts',(6.83086611675001,4.27169422781411,-2.95492204319667));
#136853=CARTESIAN_POINT('Ctrl Pts',(6.80443658539477,4.27608953524134,-2.94377128502033));
#136854=CARTESIAN_POINT('Ctrl Pts',(6.7853638114032,4.27926139266311,-2.93572438143837));
#136855=CARTESIAN_POINT('Ctrl Pts',(6.76629175820736,4.28246998646359,-2.92769013290502));
#136856=CARTESIAN_POINT('Ctrl Pts',(6.7472262747399,4.285714286,-2.91965478686889));
#136857=CARTESIAN_POINT('Ctrl Pts',(6.74111070209016,4.28675494927158,-2.9170773152643));
#136858=CARTESIAN_POINT('Ctrl Pts',(6.73499592878079,4.2877998886161,-2.91449967958568));
#136859=CARTESIAN_POINT('Ctrl Pts',(6.72888215553343,4.28884908284639,-2.91192142665916));
#136860=CARTESIAN_POINT('Ctrl Pts',(6.70370785482667,4.29316928413364,-2.90130511626555));
#136861=CARTESIAN_POINT('Ctrl Pts',(6.67855274380647,4.29756059496317,-2.89067195182173));
#136862=CARTESIAN_POINT('Ctrl Pts',(6.65341855208966,4.30202682584539,-2.88002110531445));
#136863=CARTESIAN_POINT('Ctrl Pts',(6.92984512827001,4.17158344184793,-2.13068307872255));
#136864=CARTESIAN_POINT('Ctrl Pts',(6.928666381635,4.17224147442396,-2.13450184786127));
#136865=CARTESIAN_POINT('Ctrl Pts',(6.92748763500001,4.172899507,-2.138320617));
#136866=CARTESIAN_POINT('Ctrl Pts',(6.825583742,4.229787119,-2.468457247));
#136867=CARTESIAN_POINT('Ctrl Pts',(6.692746959,4.285714286,-2.787407065));
#136868=CARTESIAN_POINT('Ctrl Pts',(6.672493911,4.294241258,-2.83603596));
#136869=CARTESIAN_POINT('Ctrl Pts',(6.651536372,4.302795611,-2.884365422));
#136870=CARTESIAN_POINT('Ctrl Pts',(7.09266291765338,4.17158344184793,-2.43807323536181));
#136871=CARTESIAN_POINT('Ctrl Pts',(7.09131462382669,4.17224147442396,-2.4419815706809));
#136872=CARTESIAN_POINT('Ctrl Pts',(7.08996633,4.172899507,-2.445889906));
#136873=CARTESIAN_POINT('Ctrl Pts',(6.973404903,4.229787119,-2.783769627));
#136874=CARTESIAN_POINT('Ctrl Pts',(6.825240674,4.285714286,-3.109033571));
#136875=CARTESIAN_POINT('Ctrl Pts',(6.80265071700001,4.294241258,-3.158625153));
#136876=CARTESIAN_POINT('Ctrl Pts',(6.779342527,4.302795611,-3.207883243));
#136877=CARTESIAN_POINT('Ctrl Pts',(6.92748753519233,4.17289956295265,-2.13832094250849));
#136878=CARTESIAN_POINT('Ctrl Pts',(6.88357214225513,4.19741522520789,-2.2805930073402));
#136879=CARTESIAN_POINT('Ctrl Pts',(6.83535770137452,4.22178368474058,-2.42122648355313));
#136880=CARTESIAN_POINT('Ctrl Pts',(6.78304357401901,4.24593817707607,-2.55984762726379));
#136881=CARTESIAN_POINT('Ctrl Pts',(6.75417899942936,4.25926553587831,-2.63633251852746));
#136882=CARTESIAN_POINT('Ctrl Pts',(6.72406713596566,4.27252781213611,-2.71220526836914));
#136883=CARTESIAN_POINT('Ctrl Pts',(6.69274695873652,4.28571428611093,-2.78740706563264));
#136884=CARTESIAN_POINT('Ctrl Pts',(6.67986179168243,4.29113922060291,-2.81834519581253));
#136885=CARTESIAN_POINT('Ctrl Pts',(6.66675202366146,4.29657697989847,-2.84921814883435));
#136886=CARTESIAN_POINT('Ctrl Pts',(6.65341855208966,4.30202682584539,-2.88002110531445));
#136887=CARTESIAN_POINT('Ctrl Pts',(7.117873279,4.302796438,-1.377817106));
#136888=CARTESIAN_POINT('Ctrl Pts',(7.043269661,4.238074114,-1.763223195));
#136889=CARTESIAN_POINT('Ctrl Pts',(6.927487635,4.172899507,-2.138320617));
#136890=CARTESIAN_POINT('Ctrl Pts',(6.92351476036112,4.17066314482709,-2.15119148380426));
#136891=CARTESIAN_POINT('Ctrl Pts',(6.91954188572229,4.16842678265418,-2.16406235060846));
#136892=CARTESIAN_POINT('Ctrl Pts',(7.40668655768233,4.302796438,-1.18268235378972));
#136893=CARTESIAN_POINT('Ctrl Pts',(7.34264875278569,4.238074114,-1.58372659622447));
#136894=CARTESIAN_POINT('Ctrl Pts',(7.23568222365171,4.172899507,-1.97551159685042));
#136895=CARTESIAN_POINT('Ctrl Pts',(7.23201183865772,4.17066314482709,-1.98895507116724));
#136896=CARTESIAN_POINT('Ctrl Pts',(7.22834145366371,4.16842678265418,-2.00239854548401));
#136897=CARTESIAN_POINT('',(7.11698472910248,4.30202682608696,-1.38239949858852));
#136898=CARTESIAN_POINT('Origin',(-0.189048592298741,4.16072148633095,0.0605005003374037));
#136899=CARTESIAN_POINT('Ctrl Pts',(7.36282707780144,4.26310680656247,-1.42785763095792));
#136900=CARTESIAN_POINT('Ctrl Pts',(7.33460231089812,4.26736775486543,-1.42262455834587));
#136901=CARTESIAN_POINT('Ctrl Pts',(7.30638515506275,4.27169422775027,-1.4174033117379));
#136902=CARTESIAN_POINT('Ctrl Pts',(7.27817644810359,4.27608953517981,-1.41219482004959));
#136903=CARTESIAN_POINT('Ctrl Pts',(7.25781973845827,4.27926139262348,-1.40843613117588));
#136904=CARTESIAN_POINT('Ctrl Pts',(7.23746645323342,4.28246998644609,-1.40468964655264));
#136905=CARTESIAN_POINT('Ctrl Pts',(7.21711934821421,4.285714286,-1.40094067775963));
#136906=CARTESIAN_POINT('Ctrl Pts',(7.21059267423742,4.28675494924643,-1.39973813337481));
#136907=CARTESIAN_POINT('Ctrl Pts',(7.20406674564231,4.28779988856547,-1.3985352569144));
#136908=CARTESIAN_POINT('Ctrl Pts',(7.19754166103911,4.28884908277022,-1.39733156264874));
#136909=CARTESIAN_POINT('Ctrl Pts',(7.17067372868453,4.2931692840602,-1.39237518613073));
#136910=CARTESIAN_POINT('Ctrl Pts',(7.14382091426537,4.29756059489632,-1.38739822434175));
#136911=CARTESIAN_POINT('Ctrl Pts',(7.11698472848189,4.30202682631765,-1.38239949983428));
#136912=CARTESIAN_POINT('Ctrl Pts',(7.22586307942343,4.17158344184794,-0.591157034752303));
#136913=CARTESIAN_POINT('Ctrl Pts',(7.22553281371172,4.17224147442397,-0.595139918876151));
#136914=CARTESIAN_POINT('Ctrl Pts',(7.225202548,4.172899507,-0.599122803));
#136915=CARTESIAN_POINT('Ctrl Pts',(7.196650728,4.229787119,-0.943447347));
#136916=CARTESIAN_POINT('Ctrl Pts',(7.135484378,4.285714286,-1.283496277));
#136917=CARTESIAN_POINT('Ctrl Pts',(7.12615861,4.294241258,-1.335342062));
#136918=CARTESIAN_POINT('Ctrl Pts',(7.11608045300001,4.302795611,-1.387046859));
#136919=CARTESIAN_POINT('Ctrl Pts',(7.45095407682186,4.17158344184794,-0.856359568123212));
#136920=CARTESIAN_POINT('Ctrl Pts',(7.45047748191092,4.17224147442397,-0.860466372061607));
#136921=CARTESIAN_POINT('Ctrl Pts',(7.450000887,4.172899507,-0.864573176));
#136922=CARTESIAN_POINT('Ctrl Pts',(7.408798753,4.229787119,-1.219610719));
#136923=CARTESIAN_POINT('Ctrl Pts',(7.334020655,4.285714286,-1.569121102));
#136924=CARTESIAN_POINT('Ctrl Pts',(7.322619563,4.294241258,-1.622409433));
#136925=CARTESIAN_POINT('Ctrl Pts',(7.310445339,4.302795611,-1.675526468));
#136926=CARTESIAN_POINT('Ctrl Pts',(7.22520252064608,4.17289956288448,-0.599123142072916));
#136927=CARTESIAN_POINT('Ctrl Pts',(7.21289813244332,4.19741522779708,-0.747509492860021));
#136928=CARTESIAN_POINT('Ctrl Pts',(7.1960429562716,4.22178369001281,-0.895219732403616));
#136929=CARTESIAN_POINT('Ctrl Pts',(7.17475134897079,4.24593818502351,-1.04184599794281));
#136930=CARTESIAN_POINT('Ctrl Pts',(7.16300360461675,4.25926554112103,-1.12274772878938));
#136931=CARTESIAN_POINT('Ctrl Pts',(7.14990614052798,4.27252781471258,-1.20331976014873));
#136932=CARTESIAN_POINT('Ctrl Pts',(7.1354843779457,4.28571428606412,-1.28349627741262));
#136933=CARTESIAN_POINT('Ctrl Pts',(7.12955124246503,4.29113922050012,-1.31648102090752));
#136934=CARTESIAN_POINT('Ctrl Pts',(7.123384745955,4.29657697988621,-1.34945039443806));
#136935=CARTESIAN_POINT('Ctrl Pts',(7.11698472873802,4.30202682609955,-1.38239949851566));
#136936=CARTESIAN_POINT('Ctrl Pts',(7.247651307,4.302796438,0.184527844));
#136937=CARTESIAN_POINT('Ctrl Pts',(7.257642797,4.238074114,-0.207905238));
#136938=CARTESIAN_POINT('Ctrl Pts',(7.225202548,4.172899507,-0.599122803));
#136939=CARTESIAN_POINT('Ctrl Pts',(7.22408941287079,4.1706631448628,-0.612546806458474));
#136940=CARTESIAN_POINT('Ctrl Pts',(7.22297627774156,4.16842678272561,-0.62597080991694));
#136941=CARTESIAN_POINT('Ctrl Pts',(7.48776408865884,4.302796438,0.437186772684723));
#136942=CARTESIAN_POINT('Ctrl Pts',(7.51143610924894,4.238074114,0.031752486387759));
#136943=CARTESIAN_POINT('Ctrl Pts',(7.49119259234274,4.172899507,-0.373867440734867));
#136944=CARTESIAN_POINT('Ctrl Pts',(7.4904979685189,4.1706631448628,-0.387785638156601));
#136945=CARTESIAN_POINT('Ctrl Pts',(7.48980334469506,4.16842678272561,-0.401703835578327));
#136946=CARTESIAN_POINT('',(7.24776860934395,4.30202682592312,0.179861575525647));
#136947=CARTESIAN_POINT('Origin',(-0.197634449238847,4.16072144827485,0.0184461769716144));
#136948=CARTESIAN_POINT('Ctrl Pts',(7.49763545645216,4.26310680820235,0.188315065585071));
#136949=CARTESIAN_POINT('Ctrl Pts',(7.4689456126465,4.26736775486193,0.18735830090538));
#136950=CARTESIAN_POINT('Ctrl Pts',(7.44026574456446,4.27169422773965,0.186391623159985));
#136951=CARTESIAN_POINT('Ctrl Pts',(7.41159687066663,4.27608953501748,0.185414304967327));
#136952=CARTESIAN_POINT('Ctrl Pts',(7.38427180671391,4.28027881893866,0.184482797081399));
#136953=CARTESIAN_POINT('Ctrl Pts',(7.35695667274408,4.28452899137757,0.183531259927492));
#136954=CARTESIAN_POINT('Ctrl Pts',(7.32965211329939,4.28884908351549,0.182595971637373));
#136955=CARTESIAN_POINT('Ctrl Pts',(7.30234686834818,4.29316928411336,0.181660659865965));
#136956=CARTESIAN_POINT('Ctrl Pts',(7.27505195801011,4.29756059497224,0.180748701676423));
#136957=CARTESIAN_POINT('Ctrl Pts',(7.24776860697028,4.30202682519232,0.179861576786871));
#136958=CARTESIAN_POINT('Ctrl Pts',(7.18400770487018,4.17158344184794,0.976010855747786));
#136959=CARTESIAN_POINT('Ctrl Pts',(7.1845413629351,4.17224147442397,0.972050091873893));
#136960=CARTESIAN_POINT('Ctrl Pts',(7.185075021,4.172899507,0.968089328));
#136961=CARTESIAN_POINT('Ctrl Pts',(7.23121032499999,4.229787119,0.625677103));
#136962=CARTESIAN_POINT('Ctrl Pts',(7.244574478,4.285714286,0.28042937));
#136963=CARTESIAN_POINT('Ctrl Pts',(7.246612053,4.294241258,0.227790947));
#136964=CARTESIAN_POINT('Ctrl Pts',(7.24788452,4.302795611,0.175128473));
#136965=CARTESIAN_POINT('Ctrl Pts',(7.46084690487036,4.17158344184793,0.765396519891662));
#136966=CARTESIAN_POINT('Ctrl Pts',(7.46126429393518,4.17224147442396,0.761283276945831));
#136967=CARTESIAN_POINT('Ctrl Pts',(7.46168168300001,4.172899507,0.757170034));
#136968=CARTESIAN_POINT('Ctrl Pts',(7.497765409,4.229787119,0.401575832));
#136969=CARTESIAN_POINT('Ctrl Pts',(7.499869982,4.285714286,0.044161726));
#136970=CARTESIAN_POINT('Ctrl Pts',(7.500190857,4.294241258,-0.010331651));
#136971=CARTESIAN_POINT('Ctrl Pts',(7.499719852,4.302795611,-0.064823938));
#136972=CARTESIAN_POINT('Ctrl Pts',(7.18507502325376,4.17289950769094,0.968089322549891));
#136973=CARTESIAN_POINT('Ctrl Pts',(7.18679928313913,4.17502562425059,0.955292014454728));
#136974=CARTESIAN_POINT('Ctrl Pts',(7.18731927076748,4.1756853480949,0.951317019401954));
#136975=CARTESIAN_POINT('Ctrl Pts',(7.18942355498595,4.17834651455219,0.935284676602476));
#136976=CARTESIAN_POINT('Ctrl Pts',(7.19048624506953,4.17970788565082,0.927079305986244));
#136977=CARTESIAN_POINT('Ctrl Pts',(7.19363141099024,4.18379006151612,0.902463723411376));
#136978=CARTESIAN_POINT('Ctrl Pts',(7.1956717930712,4.18650992780772,0.886048028029467));
#136979=CARTESIAN_POINT('Ctrl Pts',(7.20162130524362,4.19466138426959,0.836805503884857));
#136980=CARTESIAN_POINT('Ctrl Pts',(7.20536219573357,4.20008900927845,0.803958095649033));
#136981=CARTESIAN_POINT('Ctrl Pts',(7.2158985568298,4.21633619585876,0.705453633347998));
#136982=CARTESIAN_POINT('Ctrl Pts',(7.22202255225789,4.22713823146259,0.639725048026729));
#136983=CARTESIAN_POINT('Ctrl Pts',(7.23766777348088,4.25939962771955,0.442707524339282));
#136984=CARTESIAN_POINT('Ctrl Pts',(7.24450553306108,4.28067055357091,0.311351690624788));
#136985=CARTESIAN_POINT('Ctrl Pts',(7.2477686110021,4.30202682546369,0.17986157549218));
#136986=CARTESIAN_POINT('Ctrl Pts',(7.038537216,4.302796438,1.738244478));
#136987=CARTESIAN_POINT('Ctrl Pts',(7.132656622,4.238074114,1.357134138));
#136988=CARTESIAN_POINT('Ctrl Pts',(7.185075021,4.172899507,0.968089328));
#136989=CARTESIAN_POINT('Ctrl Pts',(7.18687367436045,4.17066314480402,0.954739878794608));
#136990=CARTESIAN_POINT('Ctrl Pts',(7.18867232772096,4.16842678260804,0.941390429589207));
#136991=CARTESIAN_POINT('Ctrl Pts',(7.21872209223334,4.302796438,2.03661353051088));
#136992=CARTESIAN_POINT('Ctrl Pts',(7.32899706144724,4.238074114,1.64574685777162));
#136993=CARTESIAN_POINT('Ctrl Pts',(7.39642312066713,4.172899507,1.24525834150018));
#136994=CARTESIAN_POINT('Ctrl Pts',(7.39873673783805,4.17066314480401,1.23151621985278));
#136995=CARTESIAN_POINT('Ctrl Pts',(7.40105035500898,4.16842678260803,1.21777409820541));
#136996=CARTESIAN_POINT('',(7.03965488517183,4.30202682592122,1.7337125204802));
#136997=CARTESIAN_POINT('Origin',(-0.196979586829847,4.16072142722509,-0.0244707087506646));
#136998=CARTESIAN_POINT('Ctrl Pts',(7.28186273350202,4.26310680820227,1.79568235830517));
#136999=CARTESIAN_POINT('Ctrl Pts',(7.25404931831883,4.26736775489622,1.78858049393525));
#137000=CARTESIAN_POINT('Ctrl Pts',(7.22624777665622,4.27169422779228,1.78147109270522));
#137001=CARTESIAN_POINT('Ctrl Pts',(7.19845925952399,4.27608953508906,1.77435366321102));
#137002=CARTESIAN_POINT('Ctrl Pts',(7.17197328713478,4.28027881899905,1.76756985246761));
#137003=CARTESIAN_POINT('Ctrl Pts',(7.14550131827908,4.28452899142257,1.76076861535023));
#137004=CARTESIAN_POINT('Ctrl Pts',(7.1190361837065,4.28884908354054,1.7539855203759));
#137005=CARTESIAN_POINT('Ctrl Pts',(7.09257038470169,4.29316928411851,1.74720225510555));
#137006=CARTESIAN_POINT('Ctrl Pts',(7.06610965831957,4.29756059499092,1.74044401924817));
#137007=CARTESIAN_POINT('Ctrl Pts',(7.0396548826298,4.30202682519237,1.73371252114864));
#137008=CARTESIAN_POINT('Ctrl Pts',(6.80623611384359,4.17158344184793,2.49754156239315));
#137009=CARTESIAN_POINT('Ctrl Pts',(6.8076087424218,4.17224147442396,2.49378811969657));
#137010=CARTESIAN_POINT('Ctrl Pts',(6.808981371,4.172899507,2.490034677));
#137011=CARTESIAN_POINT('Ctrl Pts',(6.927646563,4.229787119,2.165545587));
#137012=CARTESIAN_POINT('Ctrl Pts',(7.014916327,4.285714286,1.831242452));
#137013=CARTESIAN_POINT('Ctrl Pts',(7.02822197000001,4.294241258,1.780272704));
#137014=CARTESIAN_POINT('Ctrl Pts',(7.040785563,4.302795611,1.729114993));
#137015=CARTESIAN_POINT('Ctrl Pts',(7.12187882321818,4.17158344184793,2.35136351863107));
#137016=CARTESIAN_POINT('Ctrl Pts',(7.12317067960909,4.17224147442396,2.34743616731554));
#137017=CARTESIAN_POINT('Ctrl Pts',(7.124462536,4.172899507,2.343508816));
#137018=CARTESIAN_POINT('Ctrl Pts',(7.236144887,4.229787119,2.003985142));
#137019=CARTESIAN_POINT('Ctrl Pts',(7.315033724,4.285714286,1.655379601));
#137020=CARTESIAN_POINT('Ctrl Pts',(7.32706156200001,4.294241258,1.602229227));
#137021=CARTESIAN_POINT('Ctrl Pts',(7.3383158,4.302795611,1.548909688));
#137022=CARTESIAN_POINT('Ctrl Pts',(6.80898137388471,4.17289950770924,2.49003467230179));
#137023=CARTESIAN_POINT('Ctrl Pts',(6.81341636437782,4.17502562421675,2.47790722337832));
#137024=CARTESIAN_POINT('Ctrl Pts',(6.8147787014379,4.17568534806893,2.47413694343038));
#137025=CARTESIAN_POINT('Ctrl Pts',(6.82028026846994,4.1783465145361,2.45893178676429));
#137026=CARTESIAN_POINT('Ctrl Pts',(6.82308202557879,4.17970788563266,2.45114670013015));
#137027=CARTESIAN_POINT('Ctrl Pts',(6.83144528188024,4.18379006149366,2.42778273395339));
#137028=CARTESIAN_POINT('Ctrl Pts',(6.83696685021433,4.18650992778079,2.41218945028609));
#137029=CARTESIAN_POINT('Ctrl Pts',(6.8533629531749,4.19466138423686,2.36537715833159));
#137030=CARTESIAN_POINT('Ctrl Pts',(6.86407760550708,4.20008900923532,2.33410188521755));
#137031=CARTESIAN_POINT('Ctrl Pts',(6.89554317839344,4.21633619501415,2.24016541342386));
#137032=CARTESIAN_POINT('Ctrl Pts',(6.9156537019838,4.22713823099044,2.17729000179038));
#137033=CARTESIAN_POINT('Ctrl Pts',(6.97328609825812,4.25939963164881,1.98824187278948));
#137034=CARTESIAN_POINT('Ctrl Pts',(7.00820160458577,4.28067055172509,1.86142701520606));
#137035=CARTESIAN_POINT('Ctrl Pts',(7.03965488694047,4.30202682549038,1.73371252084374));
#137036=CARTESIAN_POINT('Ctrl Pts',(6.500308946,4.302796438,3.210682731));
#137037=CARTESIAN_POINT('Ctrl Pts',(6.67415535,4.238074114,2.85871543));
#137038=CARTESIAN_POINT('Ctrl Pts',(6.80898137100001,4.172899507,2.490034677));
#137039=CARTESIAN_POINT('Ctrl Pts',(6.81360770973313,4.17066314486052,2.4773839880965));
#137040=CARTESIAN_POINT('Ctrl Pts',(6.81823404846635,4.16842678272104,2.46473329919302));
#137041=CARTESIAN_POINT('Ctrl Pts',(6.61214067371357,4.302796438,3.54081050413914));
#137042=CARTESIAN_POINT('Ctrl Pts',(6.80386225587372,4.238074114,3.18278793553515));
#137043=CARTESIAN_POINT('Ctrl Pts',(6.95580512444798,4.172899507,2.80615722777803));
#137044=CARTESIAN_POINT('Ctrl Pts',(6.96101880036082,4.17066314486052,2.79323374892385));
#137045=CARTESIAN_POINT('Ctrl Pts',(6.96623247627363,4.16842678272103,2.78031027006967));
#137046=CARTESIAN_POINT('',(6.50237472155639,4.30202682607388,3.20649699365));
#137047=CARTESIAN_POINT('Origin',(-0.187113793004612,4.16072150002556,-0.0662433900295017));
#137048=CARTESIAN_POINT('Ctrl Pts',(6.72559820206182,4.26310680820237,3.31908553995907));
#137049=CARTESIAN_POINT('Ctrl Pts',(6.69996174009863,4.26736775483089,3.30617065118014));
#137050=CARTESIAN_POINT('Ctrl Pts',(6.67433849417783,4.27169422772263,3.29325095419085));
#137051=CARTESIAN_POINT('Ctrl Pts',(6.64872969411649,4.27608953501734,3.28032621653173));
#137052=CARTESIAN_POINT('Ctrl Pts',(6.6243212678066,4.28027881893362,3.26800730639257));
#137053=CARTESIAN_POINT('Ctrl Pts',(6.59993026376815,4.28452899137277,3.25567438769194));
#137054=CARTESIAN_POINT('Ctrl Pts',(6.57554203423745,4.28884908349646,3.24336065608557));
#137055=CARTESIAN_POINT('Ctrl Pts',(6.55115319241728,4.29316928408013,3.23104661533138));
#137056=CARTESIAN_POINT('Ctrl Pts',(6.52676392411202,4.29756059493291,3.21875810912994));
#137057=CARTESIAN_POINT('Ctrl Pts',(6.50237471819514,4.3020268255211,3.20649699335662));
#137058=CARTESIAN_POINT('Ctrl Pts',(6.110212485956,4.17158344184793,3.9022900024487));
#137059=CARTESIAN_POINT('Ctrl Pts',(6.112359902478,4.17224147442396,3.89891938772435));
#137060=CARTESIAN_POINT('Ctrl Pts',(6.114507319,4.172899507,3.895548773));
#137061=CARTESIAN_POINT('Ctrl Pts',(6.300153748,4.229787119,3.604155566));
#137062=CARTESIAN_POINT('Ctrl Pts',(6.457248486,4.285714286,3.296428672));
#137063=CARTESIAN_POINT('Ctrl Pts',(6.481200039,4.294241258,3.249510888));
#137064=CARTESIAN_POINT('Ctrl Pts',(6.504467298,4.302795611,3.202250017));
#137065=CARTESIAN_POINT('Ctrl Pts',(6.44989960413632,4.17158344184793,3.82738337217394));
#137066=CARTESIAN_POINT('Ctrl Pts',(6.45200552206816,4.17224147442396,3.82382555108697));
#137067=CARTESIAN_POINT('Ctrl Pts',(6.45411144,4.172899507,3.82026773));
#137068=CARTESIAN_POINT('Ctrl Pts',(6.636170272,4.229787119,3.512690335));
#137069=CARTESIAN_POINT('Ctrl Pts',(6.788154619,4.285714286,3.189193765));
#137070=CARTESIAN_POINT('Ctrl Pts',(6.811327012,4.294241258,3.139871648));
#137071=CARTESIAN_POINT('Ctrl Pts',(6.833780257,4.302795611,3.090218018));
#137072=CARTESIAN_POINT('Ctrl Pts',(6.11450750225399,4.17289956286128,3.89554848604006));
#137073=CARTESIAN_POINT('Ctrl Pts',(6.30015382568167,4.22978714685332,3.60415541375994));
#137074=CARTESIAN_POINT('Ctrl Pts',(6.457248486,4.285714286,3.296428672));
#137075=CARTESIAN_POINT('Ctrl Pts',(6.48012364,4.29385805,3.251619405));
#137076=CARTESIAN_POINT('Ctrl Pts',(6.50237471819514,4.3020268255211,3.20649699335661));
#137077=CARTESIAN_POINT('Ctrl Pts',(5.658133455,4.302796438,4.532993029));
#137078=CARTESIAN_POINT('Ctrl Pts',(5.903577993,4.238074114,4.226626366));
#137079=CARTESIAN_POINT('Ctrl Pts',(6.114507319,4.172899507,3.895548773));
#137080=CARTESIAN_POINT('Ctrl Pts',(6.12174502027726,4.17066314496693,3.88418837678026));
#137081=CARTESIAN_POINT('Ctrl Pts',(6.12898272155437,4.16842678293385,3.87282798056048));
#137082=CARTESIAN_POINT('Ctrl Pts',(5.69638290676083,4.302796438,4.87944311363592));
#137083=CARTESIAN_POINT('Ctrl Pts',(5.96058641405342,4.238074114,4.57100538662989));
#137084=CARTESIAN_POINT('Ctrl Pts',(6.18994141211535,4.172899507,4.2358433205947));
#137085=CARTESIAN_POINT('Ctrl Pts',(6.19781136075596,4.17066314496693,4.22434277223839));
#137086=CARTESIAN_POINT('Ctrl Pts',(6.20568130939647,4.16842678293385,4.21284222388206));
#137087=CARTESIAN_POINT('',(5.66105074341552,4.30202682603145,4.52934923318187));
#137088=CARTESIAN_POINT('Origin',(-0.168498607298304,4.16072146875512,-0.104918434826472));
#137089=CARTESIAN_POINT('Ctrl Pts',(5.85485217389105,4.26310680820223,4.68729197081692));
#137090=CARTESIAN_POINT('Ctrl Pts',(5.83259139768624,4.26736775487359,4.66916794326473));
#137091=CARTESIAN_POINT('Ctrl Pts',(5.81034456199046,4.271694227753,4.65104206117557));
#137092=CARTESIAN_POINT('Ctrl Pts',(5.78811291800977,4.27608953503455,4.63291436170113));
#137093=CARTESIAN_POINT('Ctrl Pts',(5.76692334865122,4.28027881894786,4.61563637066914));
#137094=CARTESIAN_POINT('Ctrl Pts',(5.74575380567805,4.2845289913801,4.5983484438477));
#137095=CARTESIAN_POINT('Ctrl Pts',(5.72458284762704,4.28884908350985,4.58107985205215));
#137096=CARTESIAN_POINT('Ctrl Pts',(5.70341135805906,4.29316928409961,4.56381082671223));
#137097=CARTESIAN_POINT('Ctrl Pts',(5.68223396277897,4.29756059496175,4.5465666472899));
#137098=CARTESIAN_POINT('Ctrl Pts',(5.66105074131829,4.30202682519241,4.52934923316963));
#137099=CARTESIAN_POINT('Ctrl Pts',(5.12848211471851,4.17158344184793,5.12457169809598));
#137100=CARTESIAN_POINT('Ctrl Pts',(5.13130390835926,4.17224147442396,5.121741517548));
#137101=CARTESIAN_POINT('Ctrl Pts',(5.134125702,4.172899507,5.118911337));
#137102=CARTESIAN_POINT('Ctrl Pts',(5.378072746,4.229787119,4.874239236));
#137103=CARTESIAN_POINT('Ctrl Pts',(5.597646882,4.285714286,4.607477551));
#137104=CARTESIAN_POINT('Ctrl Pts',(5.631124397,4.294241258,4.566805555));
#137105=CARTESIAN_POINT('Ctrl Pts',(5.664007371,4.302795611,4.52565139));
#137106=CARTESIAN_POINT('Ctrl Pts',(5.47633024678037,4.17158344184793,5.12443903217739));
#137107=CARTESIAN_POINT('Ctrl Pts',(5.47915175589019,4.17224147442396,5.12141710108869));
#137108=CARTESIAN_POINT('Ctrl Pts',(5.481973265,4.172899507,5.11839517));
#137109=CARTESIAN_POINT('Ctrl Pts',(5.725895711,4.229787119,4.857146032));
#137110=CARTESIAN_POINT('Ctrl Pts',(5.943868948,4.285714286,4.573884774));
#137111=CARTESIAN_POINT('Ctrl Pts',(5.977102382,4.294241258,4.53069716));
#137112=CARTESIAN_POINT('Ctrl Pts',(6.009704745,4.302795611,4.487031188));
#137113=CARTESIAN_POINT('Ctrl Pts',(5.13412594167712,4.17289956286129,5.11891109617975));
#137114=CARTESIAN_POINT('Ctrl Pts',(5.37807285460148,4.22978714684998,4.87423910519998));
#137115=CARTESIAN_POINT('Ctrl Pts',(5.597646882,4.285714286,4.607477551));
#137116=CARTESIAN_POINT('Ctrl Pts',(5.629619895,4.29385805,4.568633382));
#137117=CARTESIAN_POINT('Ctrl Pts',(5.66105074131829,4.30202682519241,4.52934923316963));
#137118=CARTESIAN_POINT('Ctrl Pts',(4.551389933,4.302796438,5.643345611));
#137119=CARTESIAN_POINT('Ctrl Pts',(4.85695589,4.238074114,5.39690495000001));
#137120=CARTESIAN_POINT('Ctrl Pts',(5.134125702,4.172899507,5.118911337));
#137121=CARTESIAN_POINT('Ctrl Pts',(5.14363633911191,4.17066314499645,5.10937243247936));
#137122=CARTESIAN_POINT('Ctrl Pts',(5.15314697622385,4.1684267829929,5.09983352795872));
#137123=CARTESIAN_POINT('Ctrl Pts',(4.51426860610591,4.302796438,5.9899183865558));
#137124=CARTESIAN_POINT('Ctrl Pts',(4.83860017587704,4.238074114,5.74548770562787));
#137125=CARTESIAN_POINT('Ctrl Pts',(5.13464291838638,4.172899507,5.46746608780856));
#137126=CARTESIAN_POINT('Ctrl Pts',(5.14480114980883,4.17066314499645,5.45792622234752));
#137127=CARTESIAN_POINT('Ctrl Pts',(5.15495938123141,4.16842678299289,5.44838635688648));
#137128=CARTESIAN_POINT('',(4.55502232502809,4.30202682596754,5.64041413559328));
#137129=CARTESIAN_POINT('Origin',(-0.142005119474485,4.16072144008022,-0.13868801311401));
#137130=CARTESIAN_POINT('Ctrl Pts',(4.71033976553897,4.26310680820237,5.83632583837018));
#137131=CARTESIAN_POINT('Ctrl Pts',(4.69249556405986,4.26736775487414,5.81384013165561));
#137132=CARTESIAN_POINT('Ctrl Pts',(4.67466537587514,4.27169422776848,5.79135561055881));
#137133=CARTESIAN_POINT('Ctrl Pts',(4.65685041491454,4.27608953506659,5.7688725803372));
#137134=CARTESIAN_POINT('Ctrl Pts',(4.63987050326624,4.28027881899228,5.74744340810419));
#137135=CARTESIAN_POINT('Ctrl Pts',(4.6229122856843,4.28452899144104,5.72600883746806));
#137136=CARTESIAN_POINT('Ctrl Pts',(4.6059485297059,4.28884908357724,5.70459284556887));
#137137=CARTESIAN_POINT('Ctrl Pts',(4.58898434783651,4.2931692841734,5.68317631600114));
#137138=CARTESIAN_POINT('Ctrl Pts',(4.57200905721618,4.29756059503823,5.66178278189233));
#137139=CARTESIAN_POINT('Ctrl Pts',(4.55502232147118,4.30202682552115,5.64041413303933));
#137140=CARTESIAN_POINT('Ctrl Pts',(3.90694961831175,4.17158344184794,6.10723411756125));
#137141=CARTESIAN_POINT('Ctrl Pts',(3.91031384515587,4.17224147442397,6.10507670728062));
#137142=CARTESIAN_POINT('Ctrl Pts',(3.913678072,4.172899507,6.10291929700001));
#137143=CARTESIAN_POINT('Ctrl Pts',(4.20451904,4.229787119,5.916408897));
#137144=CARTESIAN_POINT('Ctrl Pts',(4.476305531,4.285714286,5.703085901));
#137145=CARTESIAN_POINT('Ctrl Pts',(4.517743638,4.294241258,5.67056147000001));
#137146=CARTESIAN_POINT('Ctrl Pts',(4.55870475500001,4.302795611,5.637438333));
#137147=CARTESIAN_POINT('Ctrl Pts',(4.24669377469677,4.17158344184794,6.18188161995671));
#137148=CARTESIAN_POINT('Ctrl Pts',(4.25009894434839,4.17224147442397,6.17953688097836));
#137149=CARTESIAN_POINT('Ctrl Pts',(4.253504114,4.172899507,6.177192142));
#137150=CARTESIAN_POINT('Ctrl Pts',(4.547884631,4.229787119,5.974486978));
#137151=CARTESIAN_POINT('Ctrl Pts',(4.821654572,4.285714286,5.744706014));
#137152=CARTESIAN_POINT('Ctrl Pts',(4.863395087,4.294241258,5.709672308));
#137153=CARTESIAN_POINT('Ctrl Pts',(4.904622117,4.302795611,5.674035767));
#137154=CARTESIAN_POINT('Ctrl Pts',(3.91367807732903,4.17289950768826,6.10291929513916));
#137155=CARTESIAN_POINT('Ctrl Pts',(3.92454796154736,4.17502562412239,6.09594865927556));
#137156=CARTESIAN_POINT('Ctrl Pts',(3.92791418505326,4.17568534801395,6.09377161668534));
#137157=CARTESIAN_POINT('Ctrl Pts',(3.94149571326175,4.17834651449182,6.0849963033746));
#137158=CARTESIAN_POINT('Ctrl Pts',(3.94843750638517,4.17970788558933,6.08049420104513));
#137159=CARTESIAN_POINT('Ctrl Pts',(3.96923470669487,4.18379006145286,6.06695553664428));
#137160=CARTESIAN_POINT('Ctrl Pts',(3.98306704220716,4.18650992774202,6.05788334242269));
#137161=CARTESIAN_POINT('Ctrl Pts',(4.02444945824376,4.19466138420298,6.03053890013995));
#137162=CARTESIAN_POINT('Ctrl Pts',(4.05190630760384,4.20008900920532,6.01212510339892));
#137163=CARTESIAN_POINT('Ctrl Pts',(4.13380376324285,4.21633619508676,5.95638508265756));
#137164=CARTESIAN_POINT('Ctrl Pts',(4.18786418937046,4.22713823102538,5.91850077395462));
#137165=CARTESIAN_POINT('Ctrl Pts',(4.34815197388925,4.2593996277154,5.80287852399229));
#137166=CARTESIAN_POINT('Ctrl Pts',(4.45269304977008,4.28067054815198,5.72305206009217));
#137167=CARTESIAN_POINT('Ctrl Pts',(4.55502232628601,4.3020268255026,5.6404141370308));
#137168=CARTESIAN_POINT('Ctrl Pts',(3.231828475,4.302796438,6.489821624));
#137169=CARTESIAN_POINT('Ctrl Pts',(3.583227927,4.238074114,6.314830257));
#137170=CARTESIAN_POINT('Ctrl Pts',(3.913678072,4.172899507,6.102919297));
#137171=CARTESIAN_POINT('Ctrl Pts',(3.92501693864835,4.17066314490783,6.09564791233541));
#137172=CARTESIAN_POINT('Ctrl Pts',(3.93635580529665,4.16842678281565,6.08837652767085));
#137173=CARTESIAN_POINT('Ctrl Pts',(3.12107212213211,4.302796438,6.8203117322704));
#137174=CARTESIAN_POINT('Ctrl Pts',(3.49036637109628,4.238074114,6.65131740573638));
#137175=CARTESIAN_POINT('Ctrl Pts',(3.83925422858816,4.172899507,6.44343621778832));
#137176=CARTESIAN_POINT('Ctrl Pts',(3.8512257557646,4.17066314490783,6.43630310828754));
#137177=CARTESIAN_POINT('Ctrl Pts',(3.86319728294106,4.16842678281565,6.42916999878664));
#137178=CARTESIAN_POINT('',(3.23600612433553,4.30202682597445,6.48773954084562));
#137179=CARTESIAN_POINT('Origin',(-0.108871229324251,4.16072146210519,-0.165972360017885));
#137180=CARTESIAN_POINT('Ctrl Pts',(3.34557710467499,4.26310680820227,6.71245959653848));
#137181=CARTESIAN_POINT('Ctrl Pts',(3.33298385271176,4.26736775486933,6.6866636173957));
#137182=CARTESIAN_POINT('Ctrl Pts',(3.32040403182692,4.27169422775713,6.66087180846766));
#137183=CARTESIAN_POINT('Ctrl Pts',(3.30783876168844,4.27608953504649,6.63508472895175));
#137184=CARTESIAN_POINT('Ctrl Pts',(3.29586246955396,4.28027881896461,6.61050637972617));
#137185=CARTESIAN_POINT('Ctrl Pts',(3.28390852482556,4.28452899140031,6.5859274218728));
#137186=CARTESIAN_POINT('Ctrl Pts',(3.27194517730307,4.2888490835254,6.56136541780598));
#137187=CARTESIAN_POINT('Ctrl Pts',(3.25998152942953,4.29316928411046,6.53680279708701));
#137188=CARTESIAN_POINT('Ctrl Pts',(3.2480020891073,4.29756059497838,6.51226024618941));
#137189=CARTESIAN_POINT('Ctrl Pts',(3.23600612183535,4.30202682552111,6.48773953829106));
#137190=CARTESIAN_POINT('Ctrl Pts',(2.50273250095792,4.17158344184794,6.80432905678979));
#137191=CARTESIAN_POINT('Ctrl Pts',(2.50648185347896,4.17224147442397,6.80294529489489));
#137192=CARTESIAN_POINT('Ctrl Pts',(2.510231206,4.172899507,6.801561533));
#137193=CARTESIAN_POINT('Ctrl Pts',(2.834366696,4.229787119,6.681933854));
#137194=CARTESIAN_POINT('Ctrl Pts',(3.145657109,4.285714286,6.532024292));
#137195=CARTESIAN_POINT('Ctrl Pts',(3.193118207,4.294241258,6.509168232));
#137196=CARTESIAN_POINT('Ctrl Pts',(3.240242171,4.302795611,6.485624925));
#137197=CARTESIAN_POINT('Ctrl Pts',(2.81848662049146,4.17158344184794,6.95026629291661));
#137198=CARTESIAN_POINT('Ctrl Pts',(2.82231622874573,4.17224147442397,6.9487083834583));
#137199=CARTESIAN_POINT('Ctrl Pts',(2.826145837,4.172899507,6.947150474));
#137200=CARTESIAN_POINT('Ctrl Pts',(3.15721952,4.229787119,6.812467554));
#137201=CARTESIAN_POINT('Ctrl Pts',(3.473984987,4.285714286,6.646911186));
#137202=CARTESIAN_POINT('Ctrl Pts',(3.522280843,4.294241258,6.62166952500001));
#137203=CARTESIAN_POINT('Ctrl Pts',(3.570204811,4.302795611,6.59572874));
#137204=CARTESIAN_POINT('Ctrl Pts',(2.51023152525807,4.17289956251626,6.8015614158811));
#137205=CARTESIAN_POINT('Ctrl Pts',(2.83436684933752,4.22978714686279,6.68193378041409));
#137206=CARTESIAN_POINT('Ctrl Pts',(3.145657109,4.285714286,6.532024292));
#137207=CARTESIAN_POINT('Ctrl Pts',(3.190985273,4.29385805,6.510195399));
#137208=CARTESIAN_POINT('Ctrl Pts',(3.23600612183535,4.30202682552111,6.48773953829106));
#137209=CARTESIAN_POINT('Ctrl Pts',(1.76115031,4.302796438,7.032840791));
#137210=CARTESIAN_POINT('Ctrl Pts',(2.141952209,4.238074114,6.93748112));
#137211=CARTESIAN_POINT('Ctrl Pts',(2.510231206,4.172899507,6.801561533));
#137212=CARTESIAN_POINT('Ctrl Pts',(2.52286810920761,4.17066314487519,6.7968976703336));
#137213=CARTESIAN_POINT('Ctrl Pts',(2.53550501241526,4.16842678275038,6.79223380766704));
#137214=CARTESIAN_POINT('Ctrl Pts',(1.58193777457203,4.302796438,7.3317948824841));
#137215=CARTESIAN_POINT('Ctrl Pts',(1.9789269150573,4.238074114,7.24613889640495));
#137216=CARTESIAN_POINT('Ctrl Pts',(2.3643462773467,4.172899507,7.11811843102602));
#137217=CARTESIAN_POINT('Ctrl Pts',(2.37757132470284,4.17066314487519,7.11372561405092));
#137218=CARTESIAN_POINT('Ctrl Pts',(2.39079637205892,4.16842678275038,7.10933279707585));
#137219=CARTESIAN_POINT('',(1.76567787428357,4.30202682597753,7.03170545777996));
#137220=CARTESIAN_POINT('Origin',(-0.0706467007222489,4.16072148923606,
-0.185496026492233));
#137221=CARTESIAN_POINT('Ctrl Pts',(1.82437897687012,4.26310680820178,7.27472620427878));
#137222=CARTESIAN_POINT('Ctrl Pts',(1.81762552129248,4.26736775486331,7.24682614389789));
#137223=CARTESIAN_POINT('Ctrl Pts',(1.81088428609454,4.27169422775163,7.21893304355694));
#137224=CARTESIAN_POINT('Ctrl Pts',(1.80415624475797,4.27608953504463,7.19104769004101));
#137225=CARTESIAN_POINT('Ctrl Pts',(1.79774357016074,4.28027881897063,7.16446942020277));
#137226=CARTESIAN_POINT('Ctrl Pts',(1.79135285131702,4.28452899141856,7.13789536000321));
#137227=CARTESIAN_POINT('Ctrl Pts',(1.78494930497304,4.28884908355464,7.11133583589126));
#137228=CARTESIAN_POINT('Ctrl Pts',(1.77854559786201,4.29316928415071,7.08477564497745));
#137229=CARTESIAN_POINT('Ctrl Pts',(1.77212215308869,4.29756059503481,7.0582316597583));
#137230=CARTESIAN_POINT('Ctrl Pts',(1.76567787233577,4.30202682519262,7.03170545551019));
#137231=CARTESIAN_POINT('Ctrl Pts',(0.9814903926885,4.17158344184794,7.18326113271218));
#137232=CARTESIAN_POINT('Ctrl Pts',(0.98544955534425,4.17224147442397,7.18271572235609));
#137233=CARTESIAN_POINT('Ctrl Pts',(0.989408718,4.172899507,7.18217031200001));
#137234=CARTESIAN_POINT('Ctrl Pts',(1.331682516,4.229787119,7.13501901));
#137235=CARTESIAN_POINT('Ctrl Pts',(1.667921256,4.285714286,7.055532488));
#137236=CARTESIAN_POINT('Ctrl Pts',(1.719186117,4.294241258,7.043413523));
#137237=CARTESIAN_POINT('Ctrl Pts',(1.770269464,4.302795611,7.030550905));
#137238=CARTESIAN_POINT('Ctrl Pts',(1.25849016475012,4.17158344184794,7.39366423866198));
#137239=CARTESIAN_POINT('Ctrl Pts',(1.26256514337506,4.17224147442397,7.39296600483099));
#137240=CARTESIAN_POINT('Ctrl Pts',(1.266640122,4.172899507,7.392267771));
#137241=CARTESIAN_POINT('Ctrl Pts',(1.618926333,4.229787119,7.331904718));
#137242=CARTESIAN_POINT('Ctrl Pts',(1.963875725,4.285714286,7.238314178));
#137243=CARTESIAN_POINT('Ctrl Pts',(2.016468661,4.294241258,7.224044834));
#137244=CARTESIAN_POINT('Ctrl Pts',(2.068848696,4.302795611,7.209012767));
#137245=CARTESIAN_POINT('Ctrl Pts',(0.989409055158278,4.17289956303739,
7.18217026555341));
#137246=CARTESIAN_POINT('Ctrl Pts',(1.13691161755963,4.19741522444947,7.16185045047789));
#137247=CARTESIAN_POINT('Ctrl Pts',(1.28349268583219,4.22178368318658,7.1370231269043));
#137248=CARTESIAN_POINT('Ctrl Pts',(1.42875118656237,4.24593817475617,7.10782456514262));
#137249=CARTESIAN_POINT('Ctrl Pts',(1.50889827891373,4.25926553430343,7.09171411505345));
#137250=CARTESIAN_POINT('Ctrl Pts',(1.58864308271313,4.27252781130386,7.0742737736276));
#137251=CARTESIAN_POINT('Ctrl Pts',(1.66792125607932,4.28571428601319,7.05553248798125));
#137252=CARTESIAN_POINT('Ctrl Pts',(1.70053641057144,4.29113922043624,7.04782229608627));
#137253=CARTESIAN_POINT('Ctrl Pts',(1.73312358400982,4.29657697982257,7.0398799173664));
#137254=CARTESIAN_POINT('Ctrl Pts',(1.76567787434394,4.30202682585967,7.03170545794183));
#137255=CARTESIAN_POINT('Ctrl Pts',(0.208122714,4.302796438,7.247012139));
#137256=CARTESIAN_POINT('Ctrl Pts',(0.600521186,4.238074114,7.235743076));
#137257=CARTESIAN_POINT('Ctrl Pts',(0.989408718000001,4.172899507,7.18217031200001));
#137258=CARTESIAN_POINT('Ctrl Pts',(1.00275277015647,4.17066314485536,7.18033204849665));
#137259=CARTESIAN_POINT('Ctrl Pts',(1.01609682231295,4.16842678271074,7.17849378499338));
#137260=CARTESIAN_POINT('Ctrl Pts',(-0.0311662251568304,4.302796438,7.5004514520176));
#137261=CARTESIAN_POINT('Ctrl Pts',(0.374955034168565,4.238074114,7.50213898580997));
#137262=CARTESIAN_POINT('Ctrl Pts',(0.778884123161325,4.172899507,7.45996533761075));
#137263=CARTESIAN_POINT('Ctrl Pts',(0.792744302229845,4.17066314485536,
7.45851821648986));
#137264=CARTESIAN_POINT('Ctrl Pts',(0.806604481298361,4.16842678271073,
7.45707109536911));
#137265=CARTESIAN_POINT('',(0.212788490584648,4.30202682621549,7.24687664241124));
#137266=CARTESIAN_POINT('Origin',(-0.0291188721727571,4.16072147706576,
-0.196346383455754));
#137267=CARTESIAN_POINT('Ctrl Pts',(0.217874915450326,4.2631068065521,7.49683469975628));
#137268=CARTESIAN_POINT('Ctrl Pts',(0.217277039860373,4.26736775487693,
7.46813513417208));
#137269=CARTESIAN_POINT('Ctrl Pts',(0.216689603126521,4.27169422777341,
7.43944499266939));
#137270=CARTESIAN_POINT('Ctrl Pts',(0.216113386426567,4.2760895352188,7.41076525225242));
#137271=CARTESIAN_POINT('Ctrl Pts',(0.215697561767632,4.27926139264598,
7.39006862322674));
#137272=CARTESIAN_POINT('Ctrl Pts',(0.215293226590095,4.28246998645481,
7.36937734793203));
#137273=CARTESIAN_POINT('Ctrl Pts',(0.21488544015339,4.285714286,7.3486917695344));
#137274=CARTESIAN_POINT('Ctrl Pts',(0.214754635844401,4.2867549492685,7.34205652434719));
#137275=CARTESIAN_POINT('Ctrl Pts',(0.214623383247917,4.28779988861281,
7.33542196099898));
#137276=CARTESIAN_POINT('Ctrl Pts',(0.214491187080227,4.28884908284614,
7.32878809821868));
#137277=CARTESIAN_POINT('Ctrl Pts',(0.213946851210435,4.29316928414664,
7.30147225745247));
#137278=CARTESIAN_POINT('Ctrl Pts',(0.213379755318496,4.29756059501892,
7.27416800514923));
#137279=CARTESIAN_POINT('Ctrl Pts',(0.212788492433934,4.30202682634648,
7.24687664195078));
#137280=CARTESIAN_POINT('Ctrl Pts',(-0.585645114452639,4.17158344184794,
7.22631190105834));
#137281=CARTESIAN_POINT('Ctrl Pts',(-0.58166126772632,4.17224147442397,
7.22663034502917));
#137282=CARTESIAN_POINT('Ctrl Pts',(-0.577677420999999,4.172899507,7.226948789));
#137283=CARTESIAN_POINT('Ctrl Pts',(-0.233269659,4.229787119,7.25447860700001));
#137284=CARTESIAN_POINT('Ctrl Pts',(0.112195259,4.285714286,7.249131826));
#137285=CARTESIAN_POINT('Ctrl Pts',(0.164866796,4.294241258,7.24831662500001));
#137286=CARTESIAN_POINT('Ctrl Pts',(0.217520925,4.302795611,7.246736138));
#137287=CARTESIAN_POINT('Ctrl Pts',(-0.360351892041105,4.17158344184794,
7.49134266211465));
#137288=CARTESIAN_POINT('Ctrl Pts',(-0.356222084520552,4.17224147442397,
7.49153675255733));
#137289=CARTESIAN_POINT('Ctrl Pts',(-0.352092277,4.172899507,7.491730843));
#137290=CARTESIAN_POINT('Ctrl Pts',(0.00493395,4.229787119,7.508510167));
#137291=CARTESIAN_POINT('Ctrl Pts',(0.361937816,4.285714286,7.491261644));
#137292=CARTESIAN_POINT('Ctrl Pts',(0.416368646,4.294241258,7.488631836));
#137293=CARTESIAN_POINT('Ctrl Pts',(0.470755515,4.302795611,7.485211369));
#137294=CARTESIAN_POINT('Ctrl Pts',(-0.577677413703493,4.17289950809451,
7.22694879031625));
#137295=CARTESIAN_POINT('Ctrl Pts',(-0.56480552482683,4.17502562458467,
7.22797768913303));
#137296=CARTESIAN_POINT('Ctrl Pts',(-0.560808210063437,4.17568534806879,
7.228281712103));
#137297=CARTESIAN_POINT('Ctrl Pts',(-0.544685456375747,4.17834651453278,
7.22951493671606));
#137298=CARTESIAN_POINT('Ctrl Pts',(-0.536434586763961,4.17970788563026,
7.23013183848652));
#137299=CARTESIAN_POINT('Ctrl Pts',(-0.511684829216335,4.18379006149283,
7.23193973104456));
#137300=CARTESIAN_POINT('Ctrl Pts',(-0.495182744814378,4.18650992778213,
7.23308839294241));
#137301=CARTESIAN_POINT('Ctrl Pts',(-0.445690338987542,4.19466138423982,
7.23636324326149));
#137302=CARTESIAN_POINT('Ctrl Pts',(-0.412688576604694,4.20008900924327,
7.23832032466424));
#137303=CARTESIAN_POINT('Ctrl Pts',(-0.31375816172737,4.216336194307,7.24350830895865));
#137304=CARTESIAN_POINT('Ctrl Pts',(-0.247794422042017,4.22713823064889,
7.24606484978825));
#137305=CARTESIAN_POINT('Ctrl Pts',(-0.0502188363241316,4.25939962529463,
7.25102081240762));
#137306=CARTESIAN_POINT('Ctrl Pts',(0.0813145238869553,4.2806705478024,
7.25073708286748));
#137307=CARTESIAN_POINT('Ctrl Pts',(0.212788490677497,4.30202682582528,
7.24687664341437));
#137308=CARTESIAN_POINT('Ctrl Pts',(0.208833664,1.716084912,7.24699168599999));
#137309=CARTESIAN_POINT('Ctrl Pts',(0.602705566,1.651909459,7.235641637));
#137310=CARTESIAN_POINT('Ctrl Pts',(0.993027302,1.586734015,7.18167089));
#137311=CARTESIAN_POINT('Ctrl Pts',(1.00632215130568,1.58451405739453,7.17983257846853));
#137312=CARTESIAN_POINT('Ctrl Pts',(1.01961700061136,1.58229409978908,7.17799426693693));
#137313=CARTESIAN_POINT('Ctrl Pts',(-0.0304295583832685,1.716084912,7.50045357073996));
#137314=CARTESIAN_POINT('Ctrl Pts',(0.377217924081657,1.651909459,7.50210740824932));
#137315=CARTESIAN_POINT('Ctrl Pts',(0.782643448641818,1.586734015,7.45957096278917));
#137316=CARTESIAN_POINT('Ctrl Pts',(0.796452751984597,1.58451405739453,
7.45812211795109));
#137317=CARTESIAN_POINT('Ctrl Pts',(0.810262055327374,1.58229409978908,
7.45667327311299));
#137318=CARTESIAN_POINT('',(0.221461492134119,1.67637478032017,7.49672960736312));
#137319=CARTESIAN_POINT('',(0.783069556218465,1.5867340154113,7.45900811558597));
#137320=CARTESIAN_POINT('Origin',(-0.0362756096552462,1.48219936157375,
-0.185156248438731));
#137321=CARTESIAN_POINT('',(0.888048434082533,1.58673401622023,7.32033950208015));
#137322=CARTESIAN_POINT('Ctrl Pts',(0.221461497219396,1.67637477933497,
7.4967296070682));
#137323=CARTESIAN_POINT('Ctrl Pts',(0.220241943763555,1.68255913647788,
7.45504166138719));
#137324=CARTESIAN_POINT('Ctrl Pts',(0.218971997975702,1.68889233601893,
7.41335297032202));
#137325=CARTESIAN_POINT('Ctrl Pts',(0.216324551305769,1.70186464078375,
7.33007576431632));
#137326=CARTESIAN_POINT('Ctrl Pts',(0.214945489005334,1.70851143074018,
7.28843788680386));
#137327=CARTESIAN_POINT('Ctrl Pts',(0.213507121522031,1.71532338698339,
7.24685550635322));
#137328=CARTESIAN_POINT('Ctrl Pts',(0.993027301999999,1.586734015,7.18167089));
#137329=CARTESIAN_POINT('Ctrl Pts',(1.055355172,1.596957843,7.173052662));
#137330=CARTESIAN_POINT('Ctrl Pts',(1.117524075,1.607142857,7.163353959));
#137331=CARTESIAN_POINT('Ctrl Pts',(1.447313794,1.661171687,7.111904882));
#137332=CARTESIAN_POINT('Ctrl Pts',(1.770981213,1.716105035,7.03037165));
#137333=CARTESIAN_POINT('Ctrl Pts',(1.270364528,1.586734015,7.391628641));
#137334=CARTESIAN_POINT('Ctrl Pts',(1.334514567,1.596957843,7.380603475));
#137335=CARTESIAN_POINT('Ctrl Pts',(1.398463589,1.607142857,7.36846657));
#137336=CARTESIAN_POINT('Ctrl Pts',(1.737696375,1.661171687,7.304083473));
#137337=CARTESIAN_POINT('Ctrl Pts',(2.06957851,1.716105035,7.208803284));
#137338=CARTESIAN_POINT('',(1.27036453248219,1.5867340145549,7.39162863951456));
#137339=CARTESIAN_POINT('',(1.82785910999321,1.67637477921978,7.27385256010028));
#137340=CARTESIAN_POINT('Ctrl Pts',(1.27036453168524,1.58673401558733,7.39162864036663));
#137341=CARTESIAN_POINT('Ctrl Pts',(1.31316981756271,1.59355605166269,7.38427189684406));
#137342=CARTESIAN_POINT('Ctrl Pts',(1.35587255570895,1.60035948085478,7.37654993560476));
#137343=CARTESIAN_POINT('Ctrl Pts',(1.39846358896283,1.60714285699732,7.36846656998833));
#137344=CARTESIAN_POINT('Ctrl Pts',(1.5420458747753,1.63001087929659,7.34121604280571));
#137345=CARTESIAN_POINT('Ctrl Pts',(1.68530485402972,1.65310706305942,7.30967526843382));
#137346=CARTESIAN_POINT('Ctrl Pts',(1.82785910592338,1.67637477811409,7.27385256090117));
#137347=CARTESIAN_POINT('Ctrl Pts',(1.76637516206954,1.71532338708051,7.03153033114753));
#137348=CARTESIAN_POINT('Ctrl Pts',(1.77671888970243,1.70851142704495,7.07183135470349));
#137349=CARTESIAN_POINT('Ctrl Pts',(1.78701662973198,1.70186463305822,7.11219933048093));
#137350=CARTESIAN_POINT('Ctrl Pts',(1.80750430589202,1.68889233606769,7.19296039064618));
#137351=CARTESIAN_POINT('Ctrl Pts',(1.81770639724589,1.68255913656091,7.23340142230929));
#137352=CARTESIAN_POINT('Ctrl Pts',(1.82785911422308,1.67637477942243,7.27385255906961));
#137353=CARTESIAN_POINT('',(1.13169592297835,1.58673401368698,7.28664976426088));
#137354=CARTESIAN_POINT('Origin',(-1.58944038486375E-13,1.67745375800067,
-1.02565525517129E-12));
#137355=CARTESIAN_POINT('',(1.82088906321883,1.49654505841717,7.27560052616862));
#137356=CARTESIAN_POINT('Origin',(-0.0489661124338905,1.48214578504932,
-0.186087345027959));
#137357=CARTESIAN_POINT('',(2.36822808233295,1.58673401541125,7.11628384459579));
#137358=CARTESIAN_POINT('Origin',(-0.0202030731975594,1.33942798224484,
-0.183880141435366));
#137359=CARTESIAN_POINT('Origin',(-0.0752306731453836,1.48219934190074,
-0.173029379240938));
#137360=CARTESIAN_POINT('Ctrl Pts',(1.761840242,1.716084912,7.032667983));
#137361=CARTESIAN_POINT('Ctrl Pts',(2.144063713,1.651909459,6.93691247599999));
#137362=CARTESIAN_POINT('Ctrl Pts',(2.513657828,1.586734015,6.8002959));
#137363=CARTESIAN_POINT('Ctrl Pts',(2.52624666878501,1.5845140573375,6.79564256745476));
#137364=CARTESIAN_POINT('Ctrl Pts',(2.53883550957,1.58229409967501,6.79098923490962));
#137365=CARTESIAN_POINT('Ctrl Pts',(1.58265767436727,1.716084912,7.33163858915172));
#137366=CARTESIAN_POINT('Ctrl Pts',(1.98113011132105,1.651909459,7.24562160212943));
#137367=CARTESIAN_POINT('Ctrl Pts',(2.36793293409444,1.586734015,7.1169251321701));
#137368=CARTESIAN_POINT('Ctrl Pts',(2.38110792512774,1.5845140573375,7.11254156840608));
#137369=CARTESIAN_POINT('Ctrl Pts',(2.39428291616108,1.58229409967502,7.10815800464207));
#137370=CARTESIAN_POINT('',(2.44094296070756,1.58673401622024,6.95828986997161));
#137371=CARTESIAN_POINT('Ctrl Pts',(2.513657828,1.586734015,6.8002959));
#137372=CARTESIAN_POINT('Ctrl Pts',(2.572675843,1.596957843,6.778480511));
#137373=CARTESIAN_POINT('Ctrl Pts',(2.631306337,1.607142857,6.755644082));
#137374=CARTESIAN_POINT('Ctrl Pts',(2.942325725,1.661171687,6.634502815));
#137375=CARTESIAN_POINT('Ctrl Pts',(3.240898745,1.716105035,6.48529685700001));
#137376=CARTESIAN_POINT('Ctrl Pts',(2.829645774,1.586734015,6.94572564900001));
#137377=CARTESIAN_POINT('Ctrl Pts',(2.889925936,1.596957843,6.921167883));
#137378=CARTESIAN_POINT('Ctrl Pts',(2.94977079,1.607142857,6.895567583));
#137379=CARTESIAN_POINT('Ctrl Pts',(3.267232039,1.661171687,6.75976470500001));
#137380=CARTESIAN_POINT('Ctrl Pts',(3.57087253,1.716105035,6.59536726600001));
#137381=CARTESIAN_POINT('',(2.82964577863492,1.58673401412041,6.94572564643079));
#137382=CARTESIAN_POINT('',(3.34878806638739,1.67637478036033,6.71085825246303));
#137383=CARTESIAN_POINT('Ctrl Pts',(2.82964577786913,1.58673401434343,6.94572564760425));
#137384=CARTESIAN_POINT('Ctrl Pts',(2.86986881736956,1.59355605125276,6.92933902946382));
#137385=CARTESIAN_POINT('Ctrl Pts',(2.90991319578077,1.60035948085479,6.9126177769304));
#137386=CARTESIAN_POINT('Ctrl Pts',(2.94977078968452,1.60714285723677,6.89556758275372));
#137387=CARTESIAN_POINT('Ctrl Pts',(3.08413814382473,1.63001087929511,6.83808821045067));
#137388=CARTESIAN_POINT('Ctrl Pts',(3.21726747328943,1.65310706412526,6.77648839638024));
#137389=CARTESIAN_POINT('Ctrl Pts',(3.34878806267424,1.67637478135681,6.71085825444783));
#137390=CARTESIAN_POINT('Ctrl Pts',(3.23664946313647,1.71532338696461,6.48741861413624));
#137391=CARTESIAN_POINT('Ctrl Pts',(3.25541488900748,1.70851142691025,6.52455382658057));
#137392=CARTESIAN_POINT('Ctrl Pts',(3.2741497950716,1.70186463296974,6.56176431152001));
#137393=CARTESIAN_POINT('Ctrl Pts',(3.31151972142592,1.68889233604064,6.63623297774042));
#137394=CARTESIAN_POINT('Ctrl Pts',(3.33017692015088,1.68255913650151,6.67353537259707));
#137395=CARTESIAN_POINT('Ctrl Pts',(3.34878807097847,1.67637477938387,6.71085825001188));
#137396=CARTESIAN_POINT('',(2.6716518085261,1.58673401368687,6.87301077157449));
#137397=CARTESIAN_POINT('Origin',(3.76001313417973E-13,1.677453758,7.04297731246584E-13));
#137398=CARTESIAN_POINT('',(3.34235673590871,1.49654505837964,6.71406370599629));
#137399=CARTESIAN_POINT('Origin',(-0.0878244442498344,1.48214574245629,
-0.171210134418975));
#137400=CARTESIAN_POINT('',(3.84265089985349,1.58673401497662,6.44081004656482));
#137401=CARTESIAN_POINT('Origin',(-0.0592595317475542,1.33942796996735,
-0.17523807301288));
#137402=CARTESIAN_POINT('Origin',(-0.11066787247884,1.48219935974344,-0.152811403070521));
#137403=CARTESIAN_POINT('Ctrl Pts',(3.232465128,1.716084912,6.489504542));
#137404=CARTESIAN_POINT('Ctrl Pts',(3.585167823,1.651909459,6.313820997));
#137405=CARTESIAN_POINT('Ctrl Pts',(3.916752508,1.586734015,6.100946631));
#137406=CARTESIAN_POINT('Ctrl Pts',(3.92804669933292,1.5845140574204,6.09369586240833));
#137407=CARTESIAN_POINT('Ctrl Pts',(3.93934089066585,1.58229409984081,6.08644509381663));
#137408=CARTESIAN_POINT('Ctrl Pts',(3.12174159234192,1.716084912,6.82000433698394));
#137409=CARTESIAN_POINT('Ctrl Pts',(3.49240685595113,1.651909459,6.65033858415981));
#137410=CARTESIAN_POINT('Ctrl Pts',(3.84250050620848,1.586734015,6.44149979263774));
#137411=CARTESIAN_POINT('Ctrl Pts',(3.85442513617274,1.5845140574204,6.43438648078746));
#137412=CARTESIAN_POINT('Ctrl Pts',(3.86634976613706,1.58229409984081,6.42727316893712));
#137413=CARTESIAN_POINT('',(3.87970170699552,1.58673401622024,6.27087833698131));
#137414=CARTESIAN_POINT('Ctrl Pts',(3.916752508,1.586734015,6.100946631));
#137415=CARTESIAN_POINT('Ctrl Pts',(3.969701051,1.596957843,6.066954145));
#137416=CARTESIAN_POINT('Ctrl Pts',(4.022051639,1.607142857,6.032047796));
#137417=CARTESIAN_POINT('Ctrl Pts',(4.299757775,1.661171687,5.846878769));
#137418=CARTESIAN_POINT('Ctrl Pts',(4.559275454,1.716105035,5.636976791));
#137419=CARTESIAN_POINT('Ctrl Pts',(4.256615929,1.586734015,6.17504824600001));
#137420=CARTESIAN_POINT('Ctrl Pts',(4.310207581,1.596957843,6.138106173));
#137421=CARTESIAN_POINT('Ctrl Pts',(4.363149987,1.607142857,6.100239519));
#137422=CARTESIAN_POINT('Ctrl Pts',(4.643995564,1.661171687,5.899366853));
#137423=CARTESIAN_POINT('Ctrl Pts',(4.905196519,1.716105035,5.673539205));
#137424=CARTESIAN_POINT('',(4.25661593240845,1.58673401455502,6.17504824276234));
#137425=CARTESIAN_POINT('',(4.71313141536523,1.67637477921302,5.83407167023774));
#137426=CARTESIAN_POINT('Ctrl Pts',(4.2566159320791,1.58673401558741,6.1750482438775));
#137427=CARTESIAN_POINT('Ctrl Pts',(4.2923759412647,1.59355605166272,6.15039797052476));
#137428=CARTESIAN_POINT('Ctrl Pts',(4.32788952943669,1.6003594808548,6.12545929360655));
#137429=CARTESIAN_POINT('Ctrl Pts',(4.36314998703704,1.60714285700713,6.1002395189735));
#137430=CARTESIAN_POINT('Ctrl Pts',(4.48201954105858,1.63001087933828,6.01521897324191));
#137431=CARTESIAN_POINT('Ctrl Pts',(4.59879424145111,1.65310706305078,5.92644045793392));
#137432=CARTESIAN_POINT('Ctrl Pts',(4.71313141195594,1.67637477809031,5.83407167271127));
#137433=CARTESIAN_POINT('Ctrl Pts',(4.55558163244203,1.71532338704987,5.63996241217782));
#137434=CARTESIAN_POINT('Ctrl Pts',(4.58189130563171,1.70851142709471,5.67219541149811));
#137435=CARTESIAN_POINT('Ctrl Pts',(4.60818735396652,1.70186463322795,5.70450848448949));
#137436=CARTESIAN_POINT('Ctrl Pts',(4.66069215498257,1.6888923360782,5.76920268614747));
#137437=CARTESIAN_POINT('Ctrl Pts',(4.68693207092282,1.68255913655261,5.80162222542772));
#137438=CARTESIAN_POINT('Ctrl Pts',(4.71313141882367,1.67637477941883,5.83407166748466));
#137439=CARTESIAN_POINT('',(4.08668422522155,1.5867340136868,6.13799743402479));
#137440=CARTESIAN_POINT('Origin',(-3.35668992601512E-13,1.67745375799922,
-3.29163779566599E-13));
#137441=CARTESIAN_POINT('',(4.70753952324108,1.49654505823086,5.83858472873868));
#137442=CARTESIAN_POINT('Origin',(-0.122576383705985,1.48214561512888,-0.148327772102289));
#137443=CARTESIAN_POINT('',(5.13739562869252,1.58673401497662,5.46417113114493));
#137444=CARTESIAN_POINT('Origin',(-0.0955451243659877,1.33942795239901,
-0.158402113986218));
#137445=CARTESIAN_POINT('Origin',(-0.140930589051371,1.48219934068697,-0.125448596449305));
#137446=CARTESIAN_POINT('Ctrl Pts',(4.551943538,1.716084912,5.64289908));
#137447=CARTESIAN_POINT('Ctrl Pts',(4.858633471,1.651909459,5.395502265));
#137448=CARTESIAN_POINT('Ctrl Pts',(5.136704194,1.586734015,5.11632387800001));
#137449=CARTESIAN_POINT('Ctrl Pts',(5.14617563270623,1.58451405737073,5.10681471086421));
#137450=CARTESIAN_POINT('Ctrl Pts',(5.15564707141259,1.58229409974149,5.09730554372844));
#137451=CARTESIAN_POINT('Ctrl Pts',(4.51485634319875,1.716084912,5.98947426038962));
#137452=CARTESIAN_POINT('Ctrl Pts',(4.84038253734788,1.651909459,5.74409312385766));
#137453=CARTESIAN_POINT('Ctrl Pts',(5.13739702623245,1.586734015,5.46487708159231));
#137454=CARTESIAN_POINT('Ctrl Pts',(5.14751371344061,1.58451405737074,5.45536663187083));
#137455=CARTESIAN_POINT('Ctrl Pts',(5.15763040064876,1.58229409974148,5.44585618214922));
#137456=CARTESIAN_POINT('',(5.13704991397976,1.58673401622024,5.29024750217892));
#137457=CARTESIAN_POINT('Ctrl Pts',(5.136704194,1.586734015,5.116323878));
#137458=CARTESIAN_POINT('Ctrl Pts',(5.18110745,1.596957843,5.071743746));
#137459=CARTESIAN_POINT('Ctrl Pts',(5.224730277,1.607142857,5.026399659));
#137460=CARTESIAN_POINT('Ctrl Pts',(5.45613793,1.661171687,4.785861171));
#137461=CARTESIAN_POINT('Ctrl Pts',(5.664465509,1.716105035,4.525077954));
#137462=CARTESIAN_POINT('Ctrl Pts',(5.48455145300001,1.586734015,5.115632449));
#137463=CARTESIAN_POINT('Ctrl Pts',(5.528948709,1.596957843,5.068033441));
#137464=CARTESIAN_POINT('Ctrl Pts',(5.57251314,1.607142857,5.019671036));
#137465=CARTESIAN_POINT('Ctrl Pts',(5.80361101800001,1.661171687,4.763121164));
#137466=CARTESIAN_POINT('Ctrl Pts',(6.010158971,1.716105035,4.486422756));
#137467=CARTESIAN_POINT('',(5.48455145598238,1.58673401455096,5.1156324447679));
#137468=CARTESIAN_POINT('',(5.85709397744235,1.6763747791622,4.68449038193992));
#137469=CARTESIAN_POINT('Ctrl Pts',(5.48455145555049,1.58673401558733,5.11563244626559));
#137470=CARTESIAN_POINT('Ctrl Pts',(5.51417633597188,1.59355605166269,5.08387113827875));
#137471=CARTESIAN_POINT('Ctrl Pts',(5.54349855818175,1.6003594808548,5.05188114237765));
#137472=CARTESIAN_POINT('Ctrl Pts',(5.57251313993258,1.60714285700702,5.01967103596857));
#137473=CARTESIAN_POINT('Ctrl Pts',(5.67032668528231,1.63001087932259,4.91108478308228));
#137474=CARTESIAN_POINT('Ctrl Pts',(5.7652865019684,1.65310706301201,4.79927875139742));
#137475=CARTESIAN_POINT('Ctrl Pts',(5.85709397459755,1.67637477801778,4.68449038515019));
#137476=CARTESIAN_POINT('Ctrl Pts',(5.66149986807226,1.71532338702862,4.52878783547239));
#137477=CARTESIAN_POINT('Ctrl Pts',(5.69412357879441,1.70851142687279,4.55461144413884));
#137478=CARTESIAN_POINT('Ctrl Pts',(5.72675119652746,1.70186463284792,4.58051618321537));
#137479=CARTESIAN_POINT('Ctrl Pts',(5.79193580377598,1.68889233604302,4.63241088915536));
#137480=CARTESIAN_POINT('Ctrl Pts',(5.82453148777529,1.68255913650028,4.65843167155449));
#137481=CARTESIAN_POINT('Ctrl Pts',(5.85709398027991,1.67637477937176,4.68449037844389));
#137482=CARTESIAN_POINT('',(5.31062782910159,1.58673401368699,5.11597815768528));
#137483=CARTESIAN_POINT('Origin',(1.03302782994419E-12,1.6774537579995,
9.41521166586412E-13));
#137484=CARTESIAN_POINT('',(5.85260299487725,1.49654505844533,4.6901000181293));
#137485=CARTESIAN_POINT('Origin',(-0.151596599578943,1.48214574060145,-0.118509601591543));
#137486=CARTESIAN_POINT('',(6.19192144724154,1.58673401497662,4.2320336470176));
#137487=CARTESIAN_POINT('Origin',(-0.127363302340727,1.33942796605195,-0.134159530787841));
#137488=CARTESIAN_POINT('Origin',(-0.164603305646737,1.48219936907616,-0.0922196613299897));
#137489=CARTESIAN_POINT('Ctrl Pts',(5.658578127,1.716084912,4.532437929));
#137490=CARTESIAN_POINT('Ctrl Pts',(5.904914818,1.651909459,4.224895844));
#137491=CARTESIAN_POINT('Ctrl Pts',(6.116469301,1.586734015,3.892467507));
#137492=CARTESIAN_POINT('Ctrl Pts',(6.12367511279101,1.58451405739759,3.88114457970276));
#137493=CARTESIAN_POINT('Ctrl Pts',(6.13088092458192,1.58229409979519,3.86982165240546));
#137494=CARTESIAN_POINT('Ctrl Pts',(5.69686142934484,1.716084912,4.87888302591572));
#137495=CARTESIAN_POINT('Ctrl Pts',(5.96202731117359,1.651909459,4.56926025478402));
#137496=CARTESIAN_POINT('Ctrl Pts',(6.19207457064325,1.586734015,4.23272279233906));
#137497=CARTESIAN_POINT('Ctrl Pts',(6.1999102696616,1.58451405739759,4.22125990306055));
#137498=CARTESIAN_POINT('Ctrl Pts',(6.20774596868001,1.58229409979519,4.20979701378211));
#137499=CARTESIAN_POINT('',(6.15419537620777,1.58673401622024,4.06225057412534));
#137500=CARTESIAN_POINT('Ctrl Pts',(6.116469301,1.586734015,3.892467507));
#137501=CARTESIAN_POINT('Ctrl Pts',(6.15025102300001,1.596957843,3.839384247));
#137502=CARTESIAN_POINT('Ctrl Pts',(6.183106334,1.607142857,3.785722661));
#137503=CARTESIAN_POINT('Ctrl Pts',(6.35739514,1.661171687,3.501062024));
#137504=CARTESIAN_POINT('Ctrl Pts',(6.504791453,1.716105035,3.201591502));
#137505=CARTESIAN_POINT('Ctrl Pts',(6.456035448,1.586734015,3.817015365));
#137506=CARTESIAN_POINT('Ctrl Pts',(6.48916234,1.596957843,3.760985098));
#137507=CARTESIAN_POINT('Ctrl Pts',(6.521311771,1.607142857,3.704388314));
#137508=CARTESIAN_POINT('Ctrl Pts',(6.691856071,1.661171687,3.404157223));
#137509=CARTESIAN_POINT('Ctrl Pts',(6.834093069,1.716105035,3.089526165));
#137510=CARTESIAN_POINT('',(6.45603544999827,1.5867340141205,3.81701536011187));
#137511=CARTESIAN_POINT('',(6.72718533431618,1.67637478035739,3.31586752983505));
#137512=CARTESIAN_POINT('Ctrl Pts',(6.4560354499492,1.58673401434349,3.81701536137849));
#137513=CARTESIAN_POINT('Ctrl Pts',(6.47813997398216,1.59355605125278,3.77962814198058));
#137514=CARTESIAN_POINT('Ctrl Pts',(6.49989975501628,1.60035948085479,3.74208264361557));
#137515=CARTESIAN_POINT('Ctrl Pts',(6.52131177123809,1.60714285723678,3.70438831419057));
#137516=CARTESIAN_POINT('Ctrl Pts',(6.59349565604718,1.63001087929981,3.57731372649253));
#137517=CARTESIAN_POINT('Ctrl Pts',(6.66220037299145,1.6531070641298,3.44770810410909));
#137518=CARTESIAN_POINT('Ctrl Pts',(6.72718533265722,1.67637478135621,3.31586753355462));
#137519=CARTESIAN_POINT('Ctrl Pts',(6.50269266198306,1.71532338705695,3.20585217351008));
#137520=CARTESIAN_POINT('Ctrl Pts',(6.54010496095514,1.708511426897,3.22405890711588));
#137521=CARTESIAN_POINT('Ctrl Pts',(6.57753851629545,1.70186463285819,3.24234403449837));
#137522=CARTESIAN_POINT('Ctrl Pts',(6.65235497134765,1.68889233604686,3.27901270739335));
#137523=CARTESIAN_POINT('Ctrl Pts',(6.68978228522786,1.68255913652599,3.29741802977717));
#137524=CARTESIAN_POINT('Ctrl Pts',(6.72718533641487,1.67637477939228,3.31586752525681));
#137525=CARTESIAN_POINT('',(6.28625237872066,1.58673401368698,3.85474142911702));
#137526=CARTESIAN_POINT('Origin',(4.28910379435266E-13,1.67745375799939,
2.50233861409654E-13));
#137527=CARTESIAN_POINT('',(6.72400525501397,1.49654505839823,3.32231144352664));
#137528=CARTESIAN_POINT('Origin',(-0.173528731532434,1.48214576180425,-0.0831502913214777));
#137529=CARTESIAN_POINT('',(6.95691990064217,1.58673401497662,2.80201097326936));
#137530=CARTESIAN_POINT('Origin',(-0.153225813866532,1.33942799701563,-0.103643539900192));
#137531=CARTESIAN_POINT('Origin',(-0.180579826077908,1.48219935447444,-0.0546789315472151));
#137532=CARTESIAN_POINT('Ctrl Pts',(6.50062389200001,1.716084912,3.210045018));
#137533=CARTESIAN_POINT('Ctrl Pts',(6.67508891000001,1.651909459,2.85673799));
#137534=CARTESIAN_POINT('Ctrl Pts',(6.81023510100001,1.586734015,2.486603681));
#137535=CARTESIAN_POINT('Ctrl Pts',(6.81483835017594,1.58451405743652,2.47399644108972));
#137536=CARTESIAN_POINT('Ctrl Pts',(6.81944159935196,1.58229409987305,2.46138920117939));
#137537=CARTESIAN_POINT('Ctrl Pts',(6.6124876069262,1.716084912,3.5401606418956));
#137538=CARTESIAN_POINT('Ctrl Pts',(6.80489431324512,1.651909459,3.18077385321148));
#137539=CARTESIAN_POINT('Ctrl Pts',(6.95721758997104,1.586734015,2.80265108974158));
#137540=CARTESIAN_POINT('Ctrl Pts',(6.96240591228245,1.58451405743652,2.78977175302867));
#137541=CARTESIAN_POINT('Ctrl Pts',(6.96759423459393,1.58229409987304,2.77689241631583));
#137542=CARTESIAN_POINT('',(6.88357750223904,1.58673401622024,2.64430732386983));
#137543=CARTESIAN_POINT('Ctrl Pts',(6.810235101,1.586734015,2.486603681));
#137544=CARTESIAN_POINT('Ctrl Pts',(6.831815693,1.596957843,2.427499407));
#137545=CARTESIAN_POINT('Ctrl Pts',(6.852367211,1.607142857,2.368029478));
#137546=CARTESIAN_POINT('Ctrl Pts',(6.961387619,1.661171687,2.052557107));
#137547=CARTESIAN_POINT('Ctrl Pts',(7.040960579,1.716105035,1.72840219));
#137548=CARTESIAN_POINT('Ctrl Pts',(7.1256424,1.586734015,2.339918885));
#137549=CARTESIAN_POINT('Ctrl Pts',(7.145949953,1.596957843,2.278077271));
#137550=CARTESIAN_POINT('Ctrl Pts',(7.165181113,1.607142857,2.215892511));
#137551=CARTESIAN_POINT('Ctrl Pts',(7.267197371,1.661171687,1.886018673));
#137552=CARTESIAN_POINT('Ctrl Pts',(7.338472571,1.716105035,1.548166765));
#137553=CARTESIAN_POINT('',(7.1256424007853,1.58673401455508,2.33991888034589));
#137554=CARTESIAN_POINT('',(7.2827209820599,1.67637477916436,1.79219839630654));
#137555=CARTESIAN_POINT('Ctrl Pts',(7.1256424011666,1.58673401558733,2.33991888144739));
#137556=CARTESIAN_POINT('Ctrl Pts',(7.13919298701102,1.59355605166269,2.29865393432779));
#137557=CARTESIAN_POINT('Ctrl Pts',(7.15237286433238,1.60035948085477,2.25730851863362));
#137558=CARTESIAN_POINT('Ctrl Pts',(7.16518111287102,1.60714285699147,2.21589251110698));
#137559=CARTESIAN_POINT('Ctrl Pts',(7.20836009784246,1.63001087925354,2.0762714558123));
#137560=CARTESIAN_POINT('Ctrl Pts',(7.24759715930115,1.6531070630198,1.9349264571486));
#137561=CARTESIAN_POINT('Ctrl Pts',(7.28272098085021,1.67637477804653,1.79219840031975));
#137562=CARTESIAN_POINT('Ctrl Pts',(7.03982677420651,1.71532338701833,1.73301442804905));
#137563=CARTESIAN_POINT('Ctrl Pts',(7.08027830270189,1.70851142707053,1.74275295944677));
#137564=CARTESIAN_POINT('Ctrl Pts',(7.12076744301577,1.70186463321145,1.75256348237523));
#137565=CARTESIAN_POINT('Ctrl Pts',(7.20171741388181,1.68889233604349,1.77229153604284));
#137566=CARTESIAN_POINT('Ctrl Pts',(7.24222629826762,1.68255913651346,1.78222078597184));
#137567=CARTESIAN_POINT('Ctrl Pts',(7.28272098314211,1.67637477936909,1.79219839204119));
#137568=CARTESIAN_POINT('',(6.96793875314233,1.58673401368699,2.41326127537066));
#137569=CARTESIAN_POINT('Origin',(5.78096598369271E-13,1.67745375800033,
1.52221985016965E-13));
#137570=CARTESIAN_POINT('',(7.28100050215491,1.49654505820162,1.799175278978));
#137571=CARTESIAN_POINT('Origin',(-0.187346444560271,1.48214560241578,-0.0439026723522515));
#137572=CARTESIAN_POINT('',(7.39662051196621,1.5867340154113,1.24096938282043));
#137573=CARTESIAN_POINT('Origin',(-0.171923645285352,1.33942798281817,-0.0682813679420349));
#137574=CARTESIAN_POINT('Origin',(-0.188112242013981,1.48219937988002,-0.0145812322219743));
#137575=CARTESIAN_POINT('Ctrl Pts',(7.038707708,1.716084912,1.73755397));
#137576=CARTESIAN_POINT('Ctrl Pts',(7.133143264,1.651909459,1.355002242));
#137577=CARTESIAN_POINT('Ctrl Pts',(7.185561877,1.586734015,0.964469032));
#137578=CARTESIAN_POINT('Ctrl Pts',(7.18734732086528,1.58451405743156,0.951166979845766));
#137579=CARTESIAN_POINT('Ctrl Pts',(7.18913276473049,1.58229409986314,0.937864927691542));
#137580=CARTESIAN_POINT('Ctrl Pts',(7.21892121263256,1.716084912,2.0359042818088));
#137581=CARTESIAN_POINT('Ctrl Pts',(7.32957202130352,1.651909459,1.64355800234819));
#137582=CARTESIAN_POINT('Ctrl Pts',(7.39704884755691,1.586734015,1.24153053637962));
#137583=CARTESIAN_POINT('Ctrl Pts',(7.39934719309846,1.58451405743156,1.22783697541526));
#137584=CARTESIAN_POINT('Ctrl Pts',(7.40164553863998,1.58229409986314,1.21414341445083));
#137585=CARTESIAN_POINT('',(7.29109119514222,1.58673401622024,1.10271920244772));
#137586=CARTESIAN_POINT('Ctrl Pts',(7.18556187699999,1.586734015,0.964469031999999));
#137587=CARTESIAN_POINT('Ctrl Pts',(7.193932255,1.596957843,0.902107393));
#137588=CARTESIAN_POINT('Ctrl Pts',(7.201219013,1.607142857,0.839609869));
#137589=CARTESIAN_POINT('Ctrl Pts',(7.23987335,1.661171687,0.508076902));
#137590=CARTESIAN_POINT('Ctrl Pts',(7.247902213,1.716105035,0.174394712));
#137591=CARTESIAN_POINT('Ctrl Pts',(7.462062233,1.586734015,0.753410398));
#137592=CARTESIAN_POINT('Ctrl Pts',(7.468600888,1.596957843,0.688649083));
#137593=CARTESIAN_POINT('Ctrl Pts',(7.474014549,1.607142857,0.623784038));
#137594=CARTESIAN_POINT('Ctrl Pts',(7.502732599,1.661171687,0.279691987));
#137595=CARTESIAN_POINT('Ctrl Pts',(7.499713251,1.716105035,-0.065583193));
#137596=CARTESIAN_POINT('Ctrl Pts',(7.24778641104372,1.71532338698279,0.179142852969469));
#137597=CARTESIAN_POINT('Ctrl Pts',(7.28938567962167,1.70851143064064,0.17995781963721));
#137598=CARTESIAN_POINT('Ctrl Pts',(7.33103715327861,1.70186464057295,0.180835009060724));
#137599=CARTESIAN_POINT('Ctrl Pts',(7.41433555438445,1.68889233605274,0.182699982007276));
#137600=CARTESIAN_POINT('Ctrl Pts',(7.45603185895234,1.68255913649846,0.183688878893547));
#137601=CARTESIAN_POINT('Ctrl Pts',(7.49772469090217,1.67637477936472,0.184728053859447));
#137602=CARTESIAN_POINT('',(7.32381205594063,1.58673401368678,0.858939706979712));
#137603=CARTESIAN_POINT('Ctrl Pts',(7.247669375,1.716084912,0.183816829));
#137604=CARTESIAN_POINT('Ctrl Pts',(7.257659767,1.651909459,-0.210091905));
#137605=CARTESIAN_POINT('Ctrl Pts',(7.224899766,1.586734015,-0.602763118000001));
#137606=CARTESIAN_POINT('Ctrl Pts',(7.22439583072087,1.58573144465319,-0.608803437636323));
#137607=CARTESIAN_POINT('Ctrl Pts',(7.22389189544178,1.58472887430638,-0.614843757272649));
#137608=CARTESIAN_POINT('Ctrl Pts',(7.48753937345035,1.716084912,0.436170706964462));
#137609=CARTESIAN_POINT('Ctrl Pts',(7.51124512463293,1.651909459,0.0292251070795899));
#137610=CARTESIAN_POINT('Ctrl Pts',(7.49070676901871,1.586734015,-0.377892639641015));
#137611=CARTESIAN_POINT('Ctrl Pts',(7.49039083490232,1.58573144465319,-0.384155185094818));
#137612=CARTESIAN_POINT('Ctrl Pts',(7.49007490078591,1.58472887430638,-0.390417730548621));
#137613=CARTESIAN_POINT('',(7.357681566992,1.58673401622024,-0.490430843621259));
#137614=CARTESIAN_POINT('Ctrl Pts',(7.224899766,1.586734015,-0.602763118));
#137615=CARTESIAN_POINT('Ctrl Pts',(7.21966854,1.596957843,-0.665466161));
#137616=CARTESIAN_POINT('Ctrl Pts',(7.213349817,1.607142857,-0.728068964));
#137617=CARTESIAN_POINT('Ctrl Pts',(7.17983065,1.661171687,-1.060160415));
#137618=CARTESIAN_POINT('Ctrl Pts',(7.115939995,1.716105035,-1.387767269));
#137619=CARTESIAN_POINT('Ctrl Pts',(7.44956433,1.586734015,-0.868326722));
#137620=CARTESIAN_POINT('Ctrl Pts',(7.44202834600001,1.596957843,-0.93297957));
#137621=CARTESIAN_POINT('Ctrl Pts',(7.433371371,1.607142857,-0.997491884));
#137622=CARTESIAN_POINT('Ctrl Pts',(7.38744839,1.661171687,-1.339712786));
#137623=CARTESIAN_POINT('Ctrl Pts',(7.310275675,1.716105035,-1.676266553));
#137624=CARTESIAN_POINT('',(7.44956432875069,1.58673401455491,-0.868326726545714));
#137625=CARTESIAN_POINT('',(7.36214312592754,1.67637477918984,-1.43137995832493));
#137626=CARTESIAN_POINT('Ctrl Pts',(7.44956432956708,1.58673401558733,-0.868326725714101));
#137627=CARTESIAN_POINT('Ctrl Pts',(7.44453580649953,1.59355605166269,-0.911467520086966));
#137628=CARTESIAN_POINT('Ctrl Pts',(7.43913704964326,1.60035948085477,-0.954525689563659));
#137629=CARTESIAN_POINT('Ctrl Pts',(7.43337137100822,1.6071428569901,-0.997491883937084));
#137630=CARTESIAN_POINT('Ctrl Pts',(7.41393419733618,1.63001087925624,-1.14233890740316));
#137631=CARTESIAN_POINT('Ctrl Pts',(7.39019556503952,1.65310706303524,-1.28709536808967));
#137632=CARTESIAN_POINT('Ctrl Pts',(7.3621431265162,1.67637477806622,-1.43137995415095));
#137633=CARTESIAN_POINT('Ctrl Pts',(7.11684761016369,1.71532338701382,-1.38310524283572));
#137634=CARTESIAN_POINT('Ctrl Pts',(7.15764950362438,1.70851143085927,-1.39125194239245));
#137635=CARTESIAN_POINT('Ctrl Pts',(7.19851575811647,1.70186464089017,-1.39934909660988));
#137636=CARTESIAN_POINT('Ctrl Pts',(7.28026760508993,1.68889233603728,-1.41543442000141));
#137637=CARTESIAN_POINT('Ctrl Pts',(7.32120165656825,1.68255913652326,-1.42343211586704));
#137638=CARTESIAN_POINT('Ctrl Pts',(7.36214312511442,1.67637477939578,-1.43137996267382));
#137639=CARTESIAN_POINT('',(7.33723204719464,1.58673401368699,-0.735544928033687));
#137640=CARTESIAN_POINT('Origin',(1.43418263376383E-12,1.67745375799961,
-2.05998412772246E-13));
#137641=CARTESIAN_POINT('',(7.36351117796384,1.49654505843051,-1.42432549981701));
#137642=CARTESIAN_POINT('Origin',(-0.18846518142437,1.48214575541465,0.0388197040358929));
#137643=CARTESIAN_POINT('',(7.23406048264311,1.58673401497662,-1.97948703581295));
#137644=CARTESIAN_POINT('Origin',(-0.184704478899498,1.33942795330298,0.0102184252568263));
#137645=CARTESIAN_POINT('Origin',(-0.176848317883889,1.48219940476887,0.0657526625594348));
#137646=CARTESIAN_POINT('Ctrl Pts',(7.11773807800001,1.716084912,-1.378515382));
#137647=CARTESIAN_POINT('Ctrl Pts',(7.042816165,1.651909459,-1.765362388));
#137648=CARTESIAN_POINT('Ctrl Pts',(6.92640937100001,1.586734015,-2.141810735));
#137649=CARTESIAN_POINT('Ctrl Pts',(6.92244440913062,1.58451405737209,-2.1546330393549));
#137650=CARTESIAN_POINT('Ctrl Pts',(6.91847944726124,1.5822940997442,-2.16745534370988));
#137651=CARTESIAN_POINT('Ctrl Pts',(7.40656946861343,1.716084912,-1.18340965930295));
#137652=CARTESIAN_POINT('Ctrl Pts',(7.34225149637669,1.651909459,-1.5859545671548));
#137653=CARTESIAN_POINT('Ctrl Pts',(7.2346848528353,1.586734015,-1.97915759736593));
#137654=CARTESIAN_POINT('Ctrl Pts',(7.2310209976134,1.58451405737209,-1.99255058731215));
#137655=CARTESIAN_POINT('Ctrl Pts',(7.22735714239161,1.5822940997442,-2.00594357725841));
#137656=CARTESIAN_POINT('',(7.08023492586553,1.58673401622024,-2.06064888883387));
#137657=CARTESIAN_POINT('Ctrl Pts',(6.926409371,1.586734015,-2.141810735));
#137658=CARTESIAN_POINT('Ctrl Pts',(6.907821148,1.596957843,-2.201923256));
#137659=CARTESIAN_POINT('Ctrl Pts',(6.888192401,1.607142857,-2.261704102));
#137660=CARTESIAN_POINT('Ctrl Pts',(6.784067048,1.661171687,-2.578825809));
#137661=CARTESIAN_POINT('Ctrl Pts',(6.65124433100001,1.716105035,-2.885038794));
#137662=CARTESIAN_POINT('Ctrl Pts',(7.088733078,1.586734015,-2.449461849));
#137663=CARTESIAN_POINT('Ctrl Pts',(7.06747483,1.596957843,-2.510983136));
#137664=CARTESIAN_POINT('Ctrl Pts',(7.04515201,1.607142857,-2.572126194));
#137665=CARTESIAN_POINT('Ctrl Pts',(6.926735305,1.661171687,-2.896474078));
#137666=CARTESIAN_POINT('Ctrl Pts',(6.779017733,1.716105035,-3.208569553));
#137667=CARTESIAN_POINT('',(7.08873307580802,1.5867340145549,-2.44946185318096));
#137668=CARTESIAN_POINT('',(6.88231593134819,1.67637477914804,-2.98055823903319));
#137669=CARTESIAN_POINT('Ctrl Pts',(7.08873307677878,1.58673401558733,-2.44946185253421));
#137670=CARTESIAN_POINT('Ctrl Pts',(7.07454812228038,1.59355605166269,-2.49051305559517));
#137671=CARTESIAN_POINT('Ctrl Pts',(7.06001935183029,1.60035948085483,-2.53140397593767));
#137672=CARTESIAN_POINT('Ctrl Pts',(7.04515200990372,1.60714285702295,-2.57212619404686));
#137673=CARTESIAN_POINT('Ctrl Pts',(6.99503143785801,1.63001087938643,-2.70940835707287));
#137674=CARTESIAN_POINT('Ctrl Pts',(6.94072944202669,1.65310706300655,-2.84567738743838));
#137675=CARTESIAN_POINT('Ctrl Pts',(6.88231593282676,1.6763747780208,-2.98055823507385));
#137676=CARTESIAN_POINT('Ctrl Pts',(6.65313292476228,1.7153233870372,-2.88068087492377));
#137677=CARTESIAN_POINT('Ctrl Pts',(6.69122961548308,1.70851142685965,-2.8974083199357));
#137678=CARTESIAN_POINT('Ctrl Pts',(6.72939981587422,1.70186463283989,-2.91410121463492));
#137679=CARTESIAN_POINT('Ctrl Pts',(6.80578243382259,1.68889233601505,-2.94738468186202));
#137680=CARTESIAN_POINT('Ctrl Pts',(6.84404020187127,1.6825591364863,-2.9639950070758));
#137681=CARTESIAN_POINT('Ctrl Pts',(6.88231592961413,1.67637477935449,-2.98055824311748));
#137682=CARTESIAN_POINT('',(7.00757122198646,1.58673401368699,-2.29563629967273));
#137683=CARTESIAN_POINT('Origin',(-2.16406753628107E-13,1.67745375799956,
1.17961196366423E-13));
#137684=CARTESIAN_POINT('',(6.88516849880378,1.49654505841873,-2.9739628013933));
#137685=CARTESIAN_POINT('Origin',(-0.175713816965931,1.48214581178345,0.0784265254199706));
#137686=CARTESIAN_POINT('',(6.63940096982194,1.58673401497662,-3.48831689502028));
#137687=CARTESIAN_POINT('Origin',(-0.178189687439472,1.33942793954582,0.049685594845269));
#137688=CARTESIAN_POINT('Origin',(-0.158578871248328,1.48219936885196,0.102232585110383));
#137689=CARTESIAN_POINT('Ctrl Pts',(6.65498925800001,1.716084912,-2.876389747));
#137690=CARTESIAN_POINT('Ctrl Pts',(6.498658307,1.651909459,-3.238086488));
#137691=CARTESIAN_POINT('Ctrl Pts',(6.304047773,1.586734015,-3.580709661));
#137692=CARTESIAN_POINT('Ctrl Pts',(6.29741909342054,1.58451405739623,-3.59237983724195));
#137693=CARTESIAN_POINT('Ctrl Pts',(6.29079041384104,1.58229409979248,-3.60405001348384));
#137694=CARTESIAN_POINT('Ctrl Pts',(6.97900989538563,1.716084912,-2.74793569772402));
#137695=CARTESIAN_POINT('Ctrl Pts',(6.8296603852941,1.651909459,-3.12724286712408));
#137696=CARTESIAN_POINT('Ctrl Pts',(6.64008156230396,1.586734015,-3.48812937990261));
#137697=CARTESIAN_POINT('Ctrl Pts',(6.63362426913067,1.58451405739623,-3.50042162846999));
#137698=CARTESIAN_POINT('Ctrl Pts',(6.62716697595724,1.58229409979248,-3.51271387703745));
#137699=CARTESIAN_POINT('',(6.47172436983887,1.58673401622024,-3.53451328120357));
#137700=CARTESIAN_POINT('Ctrl Pts',(6.304047773,1.586734015,-3.580709661));
#137701=CARTESIAN_POINT('Ctrl Pts',(6.27297171700001,1.596957843,-3.635420867));
#137702=CARTESIAN_POINT('Ctrl Pts',(6.240950764,1.607142857,-3.68958447));
#137703=CARTESIAN_POINT('Ctrl Pts',(6.07108801100001,1.661171687,-3.976908175));
#137704=CARTESIAN_POINT('Ctrl Pts',(5.875543876,1.716105035,-4.247409112));
#137705=CARTESIAN_POINT('Ctrl Pts',(6.396440546,1.586734015,-3.916062862));
#137706=CARTESIAN_POINT('Ctrl Pts',(6.362454046,1.596957843,-3.971575921));
#137707=CARTESIAN_POINT('Ctrl Pts',(6.327509171,1.607142857,-4.026490742));
#137708=CARTESIAN_POINT('Ctrl Pts',(6.142135775,1.661171687,-4.317799462));
#137709=CARTESIAN_POINT('Ctrl Pts',(5.930780456,1.716105035,-4.590843406));
#137710=CARTESIAN_POINT('',(6.3964405427229,1.58673401455097,-3.91606286599164));
#137711=CARTESIAN_POINT('',(6.08067929234869,1.67637477917653,-4.39036892940065));
#137712=CARTESIAN_POINT('Ctrl Pts',(6.39644054404754,1.58673401558734,-3.91606286518912));
#137713=CARTESIAN_POINT('Ctrl Pts',(6.3737624307921,1.5935560516627,-3.9531049683109));
#137714=CARTESIAN_POINT('Ctrl Pts',(6.35078299580488,1.60035948085484,-3.98991662567754));
#137715=CARTESIAN_POINT('Ctrl Pts',(6.32750917087876,1.60714285702463,-4.02649074198977));
#137716=CARTESIAN_POINT('Ctrl Pts',(6.24904878270096,1.63001087940218,-4.14978888302909));
#137717=CARTESIAN_POINT('Ctrl Pts',(6.16672252380312,1.65310706302945,-4.2711986954548));
#137718=CARTESIAN_POINT('Ctrl Pts',(6.08067929460951,1.67637477806564,-4.39036892590092));
#137719=CARTESIAN_POINT('Ctrl Pts',(5.87832513927852,1.71532338701635,-4.2435590700475));
#137720=CARTESIAN_POINT('Ctrl Pts',(5.91193524335975,1.70851142698047,-4.26808509887298));
#137721=CARTESIAN_POINT('Ctrl Pts',(5.94562456606603,1.70186463304736,-4.2925931876029));
#137722=CARTESIAN_POINT('Ctrl Pts',(6.01306643993702,1.68889233602917,-4.34151851184358));
#137723=CARTESIAN_POINT('Ctrl Pts',(6.04685903352462,1.68255913651325,-4.36596478612269));
#137724=CARTESIAN_POINT('Ctrl Pts',(6.08067928981379,1.67637477938004,-4.39036893296519));
#137725=CARTESIAN_POINT('',(6.35024415539573,1.58673401368695,-3.74838626845317));
#137726=CARTESIAN_POINT('Origin',(-1.10154940724527E-13,1.67745375800039,
4.33680868994202E-15));
#137727=CARTESIAN_POINT('',(6.08488299311142,1.49654505834991,-4.38454090602216));
#137728=CARTESIAN_POINT('Origin',(-0.154746378784828,1.48214577664056,0.114366264112796));
#137729=CARTESIAN_POINT('',(5.73429044748078,1.58673401540867,-4.83403693234886));
#137730=CARTESIAN_POINT('Origin',(-0.163342471950216,1.33942798155973,0.0868292586961655));
#137731=CARTESIAN_POINT('Origin',(-0.132894531346506,1.4821993605615,0.133932321928627));
#137732=CARTESIAN_POINT('Ctrl Pts',(5.881060538,1.716084912,-4.239767323));
#137733=CARTESIAN_POINT('Ctrl Pts',(5.65063041,1.651909459,-4.559401263));
#137734=CARTESIAN_POINT('Ctrl Pts',(5.386915907,1.586734015,-4.852178584));
#137735=CARTESIAN_POINT('Ctrl Pts',(5.37793345927031,1.58451405738548,-4.86215094787234));
#137736=CARTESIAN_POINT('Ctrl Pts',(5.3689510115405,1.58229409977099,-4.87212331174469));
#137737=CARTESIAN_POINT('Ctrl Pts',(6.22511957529754,1.716084912,-4.18397131818438));
#137738=CARTESIAN_POINT('Ctrl Pts',(5.99772194418561,1.651909459,-4.5223047663597));
#137739=CARTESIAN_POINT('Ctrl Pts',(5.73499543622806,1.586734015,-4.83400011010498));
#137740=CARTESIAN_POINT('Ctrl Pts',(5.72604664085241,1.58451405738548,-4.84461684563125));
#137741=CARTESIAN_POINT('Ctrl Pts',(5.71709784547668,1.58229409977099,-4.8552335811575));
#137742=CARTESIAN_POINT('',(5.56060317398339,1.58673401622024,-4.84310776175981));
#137743=CARTESIAN_POINT('Ctrl Pts',(5.386915907,1.586734015,-4.852178584));
#137744=CARTESIAN_POINT('Ctrl Pts',(5.3448051,1.596957843,-4.898930239));
#137745=CARTESIAN_POINT('Ctrl Pts',(5.301889206,1.607142857,-4.944943968));
#137746=CARTESIAN_POINT('Ctrl Pts',(5.074231646,1.661171687,-5.189034734));
#137747=CARTESIAN_POINT('Ctrl Pts',(4.825109518,1.716105035,-5.411175301));
#137748=CARTESIAN_POINT('Ctrl Pts',(5.405057563,1.586734015,-5.199553129));
#137749=CARTESIAN_POINT('Ctrl Pts',(5.359931982,1.596957843,-5.24646223));
#137750=CARTESIAN_POINT('Ctrl Pts',(5.313999035,1.607142857,-5.292581058));
#137751=CARTESIAN_POINT('Ctrl Pts',(5.070336803,1.661171687,-5.537229341));
#137752=CARTESIAN_POINT('Ctrl Pts',(4.805226477,1.716105035,-5.758454524));
#137753=CARTESIAN_POINT('',(5.40505755925514,1.5867340145549,-5.19955313187524));
#137754=CARTESIAN_POINT('',(4.99471684849644,1.67637477913455,-5.59489084771419));
#137755=CARTESIAN_POINT('Ctrl Pts',(5.40505756040768,1.58673401558733,-5.19955313169478));
#137756=CARTESIAN_POINT('Ctrl Pts',(5.37494669178826,1.59355605166269,-5.23085408659786));
#137757=CARTESIAN_POINT('Ctrl Pts',(5.34459108494202,1.6003594808547,-5.26186520844752));
#137758=CARTESIAN_POINT('Ctrl Pts',(5.31399903520763,1.60714285695396,-5.29258105779153));
#137759=CARTESIAN_POINT('Ctrl Pts',(5.21086755313719,1.63001087907978,-5.39612989179284));
#137760=CARTESIAN_POINT('Ctrl Pts',(5.10436651448534,1.65310706299861,-5.49700349882506));
#137761=CARTESIAN_POINT('Ctrl Pts',(4.99471685148991,1.67637477801125,-5.59489084475157));
#137762=CARTESIAN_POINT('Ctrl Pts',(4.82865340178371,1.71532338709796,-5.40801315987009));
#137763=CARTESIAN_POINT('Ctrl Pts',(4.8562053335994,1.70851143095389,-5.43919094458338));
#137764=CARTESIAN_POINT('Ctrl Pts',(4.88383848635188,1.7018646410062,-5.47036823620498));
#137765=CARTESIAN_POINT('Ctrl Pts',(4.93918614250612,1.68889233601318,-5.53264776102485));
#137766=CARTESIAN_POINT('Ctrl Pts',(4.96693345785353,1.68255913648008,-5.56378690379754));
#137767=CARTESIAN_POINT('Ctrl Pts',(4.9947168452189,1.67637477934025,-5.59489085068274));
#137768=CARTESIAN_POINT('',(5.39598672949708,1.58673401368699,-5.02586586240818));
#137769=CARTESIAN_POINT('Origin',(1.14491749414469E-12,1.67745375800011,
-1.23555679576448E-12));
#137770=CARTESIAN_POINT('',(5.00007512100252,1.49654505843305,-5.59010275254307));
#137771=CARTESIAN_POINT('Origin',(-0.126543208156581,1.48214574783257,0.144958432986629));
#137772=CARTESIAN_POINT('',(4.56105087436642,1.58673401497662,-5.95372277775556));
#137773=CARTESIAN_POINT('Origin',(-0.140857935027798,1.33942800656016,0.119913108632639));
#137774=CARTESIAN_POINT('Origin',(-0.100995901576229,1.48219934910415,0.159369293085917));
#137775=CARTESIAN_POINT('Ctrl Pts',(4.832139962,1.716084912,-5.404898092));
#137776=CARTESIAN_POINT('Ctrl Pts',(4.53838531400001,1.651909459,-5.667523501));
#137777=CARTESIAN_POINT('Ctrl Pts',(4.21789784,1.586734015,-5.896765029));
#137778=CARTESIAN_POINT('Ctrl Pts',(4.20698163327222,1.58451405734799,-5.90457328396551));
#137779=CARTESIAN_POINT('Ctrl Pts',(4.19606542654451,1.58229409969599,-5.91238153893092));
#137780=CARTESIAN_POINT('Ctrl Pts',(5.18014958365216,1.716084912,-5.42436908871552));
#137781=CARTESIAN_POINT('Ctrl Pts',(4.88533669233185,1.651909459,-5.7059087207657));
#137782=CARTESIAN_POINT('Ctrl Pts',(4.56174729883813,1.586734015,-5.95383836687271));
#137783=CARTESIAN_POINT('Ctrl Pts',(4.55072543682834,1.58451405734799,-5.96228316266166));
#137784=CARTESIAN_POINT('Ctrl Pts',(4.53970357481859,1.58229409969599,-5.97072795845062));
#137785=CARTESIAN_POINT('',(4.38947435436249,1.58673401622024,-5.92524390554672));
#137786=CARTESIAN_POINT('Ctrl Pts',(4.21789784,1.586734015,-5.896765029));
#137787=CARTESIAN_POINT('Ctrl Pts',(4.166721337,1.596957843,-5.933371077));
#137788=CARTESIAN_POINT('Ctrl Pts',(4.114917201,1.607142857,-5.969083383));
#137789=CARTESIAN_POINT('Ctrl Pts',(3.840109849,1.661171687,-6.158527796));
#137790=CARTESIAN_POINT('Ctrl Pts',(3.549058402,1.716105035,-6.32192094700001));
#137791=CARTESIAN_POINT('Ctrl Pts',(4.160940096,1.586734015,-6.23991807));
#137792=CARTESIAN_POINT('Ctrl Pts',(4.106785456,1.596957843,-6.276029796));
#137793=CARTESIAN_POINT('Ctrl Pts',(4.052012211,1.607142857,-6.311196166));
#137794=CARTESIAN_POINT('Ctrl Pts',(3.761454517,1.661171687,-6.49774453));
#137795=CARTESIAN_POINT('Ctrl Pts',(3.454985449,1.716105035,-6.656806708));
#137796=CARTESIAN_POINT('',(4.16094009122312,1.58673401412031,-6.23991807225148));
#137797=CARTESIAN_POINT('',(3.6752069964955,1.67637478034391,-6.5378018882331));
#137798=CARTESIAN_POINT('Ctrl Pts',(4.1609400924762,1.58673401434335,-6.23991807212436));
#137799=CARTESIAN_POINT('Ctrl Pts',(4.12480441948581,1.59355605125273,-6.26401428120538));
#137800=CARTESIAN_POINT('Ctrl Pts',(4.08849203547424,1.60035948085479,-6.28777482204739));
#137801=CARTESIAN_POINT('Ctrl Pts',(4.05201221122053,1.60714285723681,-6.31119616555529));
#137802=CARTESIAN_POINT('Ctrl Pts',(3.9290319461485,1.63001087929038,-6.39015386592446));
#137803=CARTESIAN_POINT('Ctrl Pts',(3.80333600022774,1.65310706412051,-6.46577452826259));
#137804=CARTESIAN_POINT('Ctrl Pts',(3.67520700022725,1.67637478135681,-6.5378018863744));
#137805=CARTESIAN_POINT('Ctrl Pts',(3.55319919884997,1.71532338706032,-6.31959456502606));
#137806=CARTESIAN_POINT('Ctrl Pts',(3.57340469129327,1.70851142706105,-6.35596630201538));
#137807=CARTESIAN_POINT('Ctrl Pts',(3.5936896134933,1.70186463310274,-6.39235502044082));
#137808=CARTESIAN_POINT('Ctrl Pts',(3.63435499056764,1.68889233603733,-6.46507655017275));
#137809=CARTESIAN_POINT('Ctrl Pts',(3.65475959393252,1.68255913648579,-6.50145252979146));
#137810=CARTESIAN_POINT('Ctrl Pts',(3.67520699193589,1.67637477935762,-6.53780189063019));
#137811=CARTESIAN_POINT('',(4.18941896135415,1.58673401368669,-6.06834155408811));
#137812=CARTESIAN_POINT('Origin',(3.68411898210574E-13,1.67745375799978,
-6.76975836499949E-13));
#137813=CARTESIAN_POINT('',(3.68146929365968,1.4965450583892,-6.53427760673528));
#137814=CARTESIAN_POINT('Origin',(-0.0924228176382863,1.48214577209747,
0.168772261139138));
#137815=CARTESIAN_POINT('',(3.17454163251369,1.58673401497662,-6.79501916224933));
#137816=CARTESIAN_POINT('Origin',(-0.111786908323656,1.33942794745275,0.147389747057465));
#137817=CARTESIAN_POINT('Origin',(-0.0643749739487942,1.48219938687106,
0.17735442406437));
#137818=CARTESIAN_POINT('Ctrl Pts',(3.557273893,1.716084912,-6.317301833));
#137819=CARTESIAN_POINT('Ctrl Pts',(3.213930366,1.651909459,-6.51063864));
#137820=CARTESIAN_POINT('Ctrl Pts',(2.851655559,1.586734015,-6.665625295));
#137821=CARTESIAN_POINT('Ctrl Pts',(2.83931602349466,1.58451405741593,-6.67090433537289));
#137822=CARTESIAN_POINT('Ctrl Pts',(2.82697648798927,1.58229409983188,-6.67618337574564));
#137823=CARTESIAN_POINT('Ctrl Pts',(3.89296155426518,1.716084912,-6.41112939027493));
#137824=CARTESIAN_POINT('Ctrl Pts',(3.54451852595587,1.651909459,-6.62271072495192));
#137825=CARTESIAN_POINT('Ctrl Pts',(3.1751969266877,1.586734015,-6.79528175959364));
#137826=CARTESIAN_POINT('Ctrl Pts',(3.162617368576,1.58451405741593,-6.80115974605037));
#137827=CARTESIAN_POINT('Ctrl Pts',(3.15003781046428,1.58229409983188,-6.8070377325071));
#137828=CARTESIAN_POINT('',(3.01309859252858,1.58673401622024,-6.73032223012104));
#137829=CARTESIAN_POINT('Ctrl Pts',(2.851655559,1.586734015,-6.665625295));
#137830=CARTESIAN_POINT('Ctrl Pts',(2.793806315,1.596957843,-6.690374079));
#137831=CARTESIAN_POINT('Ctrl Pts',(2.735536241,1.607142857,-6.714115092));
#137832=CARTESIAN_POINT('Ctrl Pts',(2.426428783,1.661171687,-6.840054943));
#137833=CARTESIAN_POINT('Ctrl Pts',(2.10705726,1.716105035,-6.937060595));
#137834=CARTESIAN_POINT('Ctrl Pts',(2.722261695,1.586734015,-6.988511377));
#137835=CARTESIAN_POINT('Ctrl Pts',(2.661610206,1.596957843,-7.012137184));
#137836=CARTESIAN_POINT('Ctrl Pts',(2.600557799,1.607142857,-7.034706755));
#137837=CARTESIAN_POINT('Ctrl Pts',(2.276690798,1.661171687,-7.154432408));
#137838=CARTESIAN_POINT('Ctrl Pts',(1.94319314,1.716105035,-7.243894009));
#137839=CARTESIAN_POINT('',(2.72226169039777,1.5867340145549,-6.9885113780276));
#137840=CARTESIAN_POINT('',(2.1838485481367,1.67637477913636,-7.17501257923925));
#137841=CARTESIAN_POINT('Ctrl Pts',(2.72226169151576,1.58673401558733,-6.98851137835724));
#137842=CARTESIAN_POINT('Ctrl Pts',(2.68179087705114,1.59355605166269,-7.00427612982548));
#137843=CARTESIAN_POINT('Ctrl Pts',(2.64121964210082,1.60035948085471,-7.01967507320326));
#137844=CARTESIAN_POINT('Ctrl Pts',(2.60055779923287,1.60714285696172,-7.03470675490712));
#137845=CARTESIAN_POINT('Ctrl Pts',(2.4634791737446,1.63001087911566,-7.08538134630581));
#137846=CARTESIAN_POINT('Ctrl Pts',(2.32446572072597,1.65310706299496,-7.13221312719443));
#137847=CARTESIAN_POINT('Ctrl Pts',(2.18384855217046,1.67637477799263,-7.17501257778031));
#137848=CARTESIAN_POINT('Ctrl Pts',(2.11160135108966,1.71532338690958,-6.93567875205951));
#137849=CARTESIAN_POINT('Ctrl Pts',(2.12351559544664,1.70851143053091,-6.97554370062043));
#137850=CARTESIAN_POINT('Ctrl Pts',(2.13550376091455,1.70186464041742,-7.01544230514015));
#137851=CARTESIAN_POINT('Ctrl Pts',(2.15958543818596,1.68889233600329,-7.09520554538441));
#137852=CARTESIAN_POINT('Ctrl Pts',(2.17169323280053,1.6825591364667,-7.13511746140698));
#137853=CARTESIAN_POINT('Ctrl Pts',(2.18384854383863,1.67637477934591,-7.17501258058127));
#137854=CARTESIAN_POINT('',(2.7869586195249,1.58673401368699,-6.8270683390515));
#137855=CARTESIAN_POINT('Origin',(4.42679747025831E-13,1.67745375799939,
-1.495765317161E-12));
#137856=CARTESIAN_POINT('',(2.19072205418073,1.49654505837267,-7.17291690205873));
#137857=CARTESIAN_POINT('Origin',(-0.0539810490203899,1.48214576132564,
0.184694844397544));
#137858=CARTESIAN_POINT('',(1.63959435298178,1.58673401497662,-7.31858800252645));
#137859=CARTESIAN_POINT('Origin',(-0.0774889774619666,1.33942798701671,
0.167974844422635));
#137860=CARTESIAN_POINT('Origin',(-0.0247439678196198,1.48219933560951,
0.187046733158217));
#137861=CARTESIAN_POINT('Ctrl Pts',(2.116073651,1.716084912,-6.93431556100001));
#137862=CARTESIAN_POINT('Ctrl Pts',(1.739195605,1.651909459,-7.049323552));
#137863=CARTESIAN_POINT('Ctrl Pts',(1.352073032,1.586734015,-7.122808331));
#137864=CARTESIAN_POINT('Ctrl Pts',(1.33888715021876,1.58451405739596,-7.1253113150061));
#137865=CARTESIAN_POINT('Ctrl Pts',(1.32570126843754,1.58229409979194,-7.12781429901219));
#137866=CARTESIAN_POINT('Ctrl Pts',(2.42374296913084,1.716084912,-7.09811240704809));
#137867=CARTESIAN_POINT('Ctrl Pts',(2.03796261177443,1.651909459,-7.22984213653404));
#137868=CARTESIAN_POINT('Ctrl Pts',(1.64017787609125,1.586734015,-7.3189853294083));
#137869=CARTESIAN_POINT('Ctrl Pts',(1.62662882763753,1.58451405739596,-7.32202165868699));
#137870=CARTESIAN_POINT('Ctrl Pts',(1.61307977918388,1.58229409979194,-7.32505798796576));
#137871=CARTESIAN_POINT('',(1.49583368902063,1.58673401622024,-7.22069816754942));
#137872=CARTESIAN_POINT('Ctrl Pts',(1.352073032,1.586734015,-7.122808331));
#137873=CARTESIAN_POINT('Ctrl Pts',(1.290256015,1.596957843,-7.134542624));
#137874=CARTESIAN_POINT('Ctrl Pts',(1.228244647,1.607142857,-7.145202243));
#137875=CARTESIAN_POINT('Ctrl Pts',(0.899290605,1.661171687,-7.201748723));
#137876=CARTESIAN_POINT('Ctrl Pts',(0.566532463,1.716105035,-7.227831));
#137877=CARTESIAN_POINT('Ctrl Pts',(1.156293362,1.586734015,-7.410329659));
#137878=CARTESIAN_POINT('Ctrl Pts',(1.091981021,1.596957843,-7.42036483100001));
#137879=CARTESIAN_POINT('Ctrl Pts',(1.027504195,1.607142857,-7.429282275));
#137880=CARTESIAN_POINT('Ctrl Pts',(0.685471549000001,1.661171687,-7.476586977));
#137881=CARTESIAN_POINT('Ctrl Pts',(0.340539281,1.716105035,-7.492264878));
#137882=CARTESIAN_POINT('',(1.15629335682412,1.58673401455096,-7.41032965909313));
#137883=CARTESIAN_POINT('',(0.590375770590217,1.67637477916754,-7.47672765614166));
#137884=CARTESIAN_POINT('Ctrl Pts',(1.15629335830546,1.58673401558733,-7.41032965957648));
#137885=CARTESIAN_POINT('Ctrl Pts',(1.11337977344535,1.59355605166269,-7.41702581146744));
#137886=CARTESIAN_POINT('Ctrl Pts',(1.0704467538818,1.60035948085471,-7.42334311999044));
#137887=CARTESIAN_POINT('Ctrl Pts',(1.02750419524604,1.60714285696113,-7.42928227496597));
#137888=CARTESIAN_POINT('Ctrl Pts',(0.882736852912321,1.63001087912203,
-7.44930427014739));
#137889=CARTESIAN_POINT('Ctrl Pts',(0.736906008782792,1.65310706302017,
-7.46515736687437));
#137890=CARTESIAN_POINT('Ctrl Pts',(0.590375774770585,1.6763747780432,-7.47672765559436));
#137891=CARTESIAN_POINT('Ctrl Pts',(0.571267370680839,1.71532338695618,
-7.22745830928171));
#137892=CARTESIAN_POINT('Ctrl Pts',(0.574333282776174,1.70851142694226,
-7.26895247004213));
#137893=CARTESIAN_POINT('Ctrl Pts',(0.577464153095201,1.70186463307537,
-7.31049539372416));
#137894=CARTESIAN_POINT('Ctrl Pts',(0.583836071793672,1.68889233605644,
-7.39357061501269));
#137895=CARTESIAN_POINT('Ctrl Pts',(0.587080910820238,1.68255913651965,
-7.43515223045215));
#137896=CARTESIAN_POINT('Ctrl Pts',(0.590375766180676,1.67637477937349,
-7.47672765652176));
#137897=CARTESIAN_POINT('',(1.25418318904368,1.58673401368699,-7.26656899637323));
#137898=CARTESIAN_POINT('Origin',(1.03483709231952E-13,1.67745375799956,
-1.06902334207071E-12));
#137899=CARTESIAN_POINT('',(0.597539085963974,1.49654505840547,-7.47615857508329));
#137900=CARTESIAN_POINT('Origin',(-0.0130150326916503,1.48214575193959,
0.191980769349778));
#137901=CARTESIAN_POINT('',(0.0279814687171162,1.58673401541125,-7.49994780268285));
#137902=CARTESIAN_POINT('Origin',(-0.0395677149432771,1.33942796522644,
0.180705713823447));
#137903=CARTESIAN_POINT('Origin',(0.0160440422792048,1.48219934306306,0.187993145569987));
#137904=CARTESIAN_POINT('Ctrl Pts',(0.575928156,1.716084912,-7.227088401));
#137905=CARTESIAN_POINT('Ctrl Pts',(0.183137991,1.651909459,-7.25838993));
#137906=CARTESIAN_POINT('Ctrl Pts',(-0.210730926,1.586734015,-7.246936765));
#137907=CARTESIAN_POINT('Ctrl Pts',(-0.224146596640912,1.58451405741299,
-7.24654665579665));
#137908=CARTESIAN_POINT('Ctrl Pts',(-0.237562267281824,1.582294099826,-7.24615654659332));
#137909=CARTESIAN_POINT('Ctrl Pts',(0.841192856648398,1.716084912,-7.45319557669144));
#137910=CARTESIAN_POINT('Ctrl Pts',(0.436113832324383,1.651909459,-7.49891416437837));
#137911=CARTESIAN_POINT('Ctrl Pts',(0.0284659309655903,1.586734015,-7.50046127958347));
#137912=CARTESIAN_POINT('Ctrl Pts',(0.0145809307890254,1.58451405741299,
-7.50051397627298));
#137913=CARTESIAN_POINT('Ctrl Pts',(0.000695930612460646,1.582294099826,
-7.5005666729626));
#137914=CARTESIAN_POINT('',(-0.091374734637584,1.58673401622024,-7.37344228340535));
#137915=CARTESIAN_POINT('Ctrl Pts',(-0.210730926,1.586734015,-7.24693676500001));
#137916=CARTESIAN_POINT('Ctrl Pts',(-0.273625222,1.596957843,-7.245107886));
#137917=CARTESIAN_POINT('Ctrl Pts',(-0.336478302,1.607142857,-7.242187677));
#137918=CARTESIAN_POINT('Ctrl Pts',(-0.669897403,1.661171687,-7.226696737));
#137919=CARTESIAN_POINT('Ctrl Pts',(-1.000482763,1.716105035,-7.18063606100001));
#137920=CARTESIAN_POINT('Ctrl Pts',(-0.463741963,1.586734015,-7.48564916300001));
#137921=CARTESIAN_POINT('Ctrl Pts',(-0.528707983,1.596957843,-7.481624466));
#137922=CARTESIAN_POINT('Ctrl Pts',(-0.593594363,1.607142857,-7.476472814));
#137923=CARTESIAN_POINT('Ctrl Pts',(-0.937799589,1.661171687,-7.449144649));
#137924=CARTESIAN_POINT('Ctrl Pts',(-1.278037818,1.716105035,-7.390305767));
#137925=CARTESIAN_POINT('',(-0.463741967621627,1.58673401455466,-7.48564916200989));
#137926=CARTESIAN_POINT('',(-1.0307023228524,1.67637477913704,-7.42883925771828));
#137927=CARTESIAN_POINT('Ctrl Pts',(-0.463741966734078,1.58673401558764,
-7.48564916276868));
#137928=CARTESIAN_POINT('Ctrl Pts',(-0.507091730847073,1.59355605166279,
-7.48296361012152));
#137929=CARTESIAN_POINT('Ctrl Pts',(-0.550379034849969,1.60035948085491,
-7.47990389355397));
#137930=CARTESIAN_POINT('Ctrl Pts',(-0.593594363123317,1.60714285706055,
-7.47647281373026));
#137931=CARTESIAN_POINT('Ctrl Pts',(-0.739281263995284,1.63001087954842,
-7.4649060051311));
#137932=CARTESIAN_POINT('Ctrl Pts',(-0.885110609776605,1.6531070629954,
-7.44903914546373));
#137933=CARTESIAN_POINT('Ctrl Pts',(-1.03070231858164,1.67637477799372,
-7.42883925808922));
#137934=CARTESIAN_POINT('Ctrl Pts',(-0.995778437805123,1.71532338707607,
-7.18128994846951));
#137935=CARTESIAN_POINT('Ctrl Pts',(-1.00170422311022,1.70851142698573,
-7.22247307939769));
#137936=CARTESIAN_POINT('Ctrl Pts',(-1.00757705150579,1.70186463299444,
-7.26371779773764));
#137937=CARTESIAN_POINT('Ctrl Pts',(-1.01921282155258,1.68889233601896,
-7.34622054014056));
#137938=CARTESIAN_POINT('Ctrl Pts',(-1.0249826632171,1.68255913647026,-7.38752754502936));
#137939=CARTESIAN_POINT('Ctrl Pts',(-1.0307023273142,1.67637477934645,-7.42883925713188));
#137940=CARTESIAN_POINT('',(-0.337236452569776,1.58673401368629,-7.36629296363056));
#137941=CARTESIAN_POINT('Origin',(3.81991530420955E-13,1.67745375799972,
2.79160375371568E-12));
#137942=CARTESIAN_POINT('',(-1.02358414613805,1.49654505839789,-7.42982338246688));
#137943=CARTESIAN_POINT('Origin',(0.0285594814258901,1.4821457438531,0.190290540546657));
#137944=CARTESIAN_POINT('',(-1.58493980789077,1.58673401497662,-7.33061837789233));
#137945=CARTESIAN_POINT('Origin',(0.000203747006136679,1.33942799327937,
0.184986838896626));
#137946=CARTESIAN_POINT('Origin',(0.0560818439985851,1.48219938129434,0.180148667665314));
#137947=CARTESIAN_POINT('Ctrl Pts',(-0.9911471,1.716084912,-7.18193062000001));
#137948=CARTESIAN_POINT('Ctrl Pts',(-1.381482952,1.651909459,-7.128062062));
#137949=CARTESIAN_POINT('Ctrl Pts',(-1.763681341,1.586734015,-7.032206491));
#137950=CARTESIAN_POINT('Ctrl Pts',(-1.77669949876394,1.5845140574158,-7.02894152970832));
#137951=CARTESIAN_POINT('Ctrl Pts',(-1.78971765652795,1.58229409983161,
-7.02567656841653));
#137952=CARTESIAN_POINT('Ctrl Pts',(-0.780690499306596,1.716084912,-7.45977560420975));
#137953=CARTESIAN_POINT('Ctrl Pts',(-1.18612714580241,1.651909459,-7.41734530175765));
#137954=CARTESIAN_POINT('Ctrl Pts',(-1.58457704991799,1.586734015,-7.33122399711957));
#137955=CARTESIAN_POINT('Ctrl Pts',(-1.59814875472392,1.5845140574158,-7.32829059718152));
#137956=CARTESIAN_POINT('Ctrl Pts',(-1.61172045952986,1.58229409983162,
-7.32535719724342));
#137957=CARTESIAN_POINT('',(-1.67431057793867,1.58673401622024,-7.18141243376571));
#137958=CARTESIAN_POINT('Ctrl Pts',(-1.763681341,1.586734015,-7.03220649099999));
#137959=CARTESIAN_POINT('Ctrl Pts',(-1.824712048,1.596957843,-7.01689995500001));
#137960=CARTESIAN_POINT('Ctrl Pts',(-1.885467899,1.607142857,-7.000536465));
#137961=CARTESIAN_POINT('Ctrl Pts',(-2.207761753,1.661171687,-6.913732444));
#137962=CARTESIAN_POINT('Ctrl Pts',(-2.520716527,1.716105035,-6.79768256));
#137963=CARTESIAN_POINT('Ctrl Pts',(-2.06209323,1.586734015,-7.210948031));
#137964=CARTESIAN_POINT('Ctrl Pts',(-2.124675189,1.596957843,-7.193051656));
#137965=CARTESIAN_POINT('Ctrl Pts',(-2.186937109,1.607142857,-7.174071792));
#137966=CARTESIAN_POINT('Ctrl Pts',(-2.51722026,1.661171687,-7.073388596));
#137967=CARTESIAN_POINT('Ctrl Pts',(-2.836855288,1.716105035,-6.94278417300001));
#137968=CARTESIAN_POINT('',(-2.06209323492603,1.58673401411967,-7.21094802900619));
#137969=CARTESIAN_POINT('',(-2.60358592031819,1.6763747803427,-7.03358659236033));
#137970=CARTESIAN_POINT('Ctrl Pts',(-2.06209323404642,1.58673401434289,
-7.21094803018993));
#137971=CARTESIAN_POINT('Ctrl Pts',(-2.10385218957466,1.59355605125258,
-7.19900634661447));
#137972=CARTESIAN_POINT('Ctrl Pts',(-2.14546971161618,1.60035948085479,
-7.1867126736392));
#137973=CARTESIAN_POINT('Ctrl Pts',(-2.18693710880305,1.60714285723704,
-7.17407179237427));
#137974=CARTESIAN_POINT('Ctrl Pts',(-2.32673140886269,1.63001087929119,
-7.1314570331068));
#137975=CARTESIAN_POINT('Ctrl Pts',(-2.46574043981844,1.65310706412132,
-7.0846121322515));
#137976=CARTESIAN_POINT('Ctrl Pts',(-2.60358591652084,1.67637478135681,
-7.03358659399984));
#137977=CARTESIAN_POINT('Ctrl Pts',(-2.51626275262574,1.7153233870309,-6.79933245094728));
#137978=CARTESIAN_POINT('Ctrl Pts',(-2.53090315232834,1.70851142686521,
-6.83827887509107));
#137979=CARTESIAN_POINT('Ctrl Pts',(-2.54550507265091,1.7018646328347,-6.87729683070493));
#137980=CARTESIAN_POINT('Ctrl Pts',(-2.57460445544453,1.68889233602686,
-6.9553693573294));
#137981=CARTESIAN_POINT('Ctrl Pts',(-2.58911918650035,1.6825591364838,-6.99447028196159));
#137982=CARTESIAN_POINT('Ctrl Pts',(-2.60358592505921,1.6763747793587,-7.03358659045134));
#137983=CARTESIAN_POINT('',(-1.91288729330474,1.58673401368578,-7.12157725890361));
#137984=CARTESIAN_POINT('Origin',(2.82326245715225E-13,1.67745375799956,
7.75855074630627E-13));
#137985=CARTESIAN_POINT('',(-2.59684572075915,1.49654505838387,-7.03607790633467));
#137986=CARTESIAN_POINT('Origin',(0.0687986018264219,1.48214576764147,0.179702193597693));
#137987=CARTESIAN_POINT('',(-3.12375105413881,1.58673401540865,-6.81851738676565));
#137988=CARTESIAN_POINT('Origin',(0.0399656944841692,1.33942795304523,0.180618175323255));
#137989=CARTESIAN_POINT('Origin',(0.093497447181683,1.48219938683692,0.163881262855647));
#137990=CARTESIAN_POINT('Ctrl Pts',(-2.511877418,1.716084912,-6.800953745));
#137991=CARTESIAN_POINT('Ctrl Pts',(-2.881507287,1.651909459,-6.664433933));
#137992=CARTESIAN_POINT('Ctrl Pts',(-3.234163976,1.586734015,-6.488658057));
#137993=CARTESIAN_POINT('Ctrl Pts',(-3.24617590589201,1.58451405749336,
-6.48267090982519));
#137994=CARTESIAN_POINT('Ctrl Pts',(-3.25818783578402,1.58229409998675,
-6.47668376265049));
#137995=CARTESIAN_POINT('Ctrl Pts',(-2.36606963523562,1.716084912,-7.11754481583485));
#137996=CARTESIAN_POINT('Ctrl Pts',(-2.75290613680355,1.651909459,-6.98894961499887));
#137997=CARTESIAN_POINT('Ctrl Pts',(-3.12352696960189,1.586734015,-6.81918682764803));
#137998=CARTESIAN_POINT('Ctrl Pts',(-3.13615078080114,1.58451405749337,
-6.81340449382726));
#137999=CARTESIAN_POINT('Ctrl Pts',(-3.14877459200044,1.58229409998674,
-6.80762216000638));
#138000=CARTESIAN_POINT('',(-3.17895751939195,1.58673401622024,-6.65358771970716));
#138001=CARTESIAN_POINT('Ctrl Pts',(-3.234163976,1.586734015,-6.488658057));
#138002=CARTESIAN_POINT('Ctrl Pts',(-3.290477367,1.596957843,-6.460589581));
#138003=CARTESIAN_POINT('Ctrl Pts',(-3.346295113,1.607142857,-6.431547949));
#138004=CARTESIAN_POINT('Ctrl Pts',(-3.642393617,1.661171687,-6.277489706));
#138005=CARTESIAN_POINT('Ctrl Pts',(-3.923084388,1.716105035,-6.09687697800001));
#138006=CARTESIAN_POINT('Ctrl Pts',(-3.564023309,1.586734015,-6.599070984));
#138007=CARTESIAN_POINT('Ctrl Pts',(-3.621294945,1.596957843,-6.568139745));
#138008=CARTESIAN_POINT('Ctrl Pts',(-3.678021106,1.607142857,-6.536219148));
#138009=CARTESIAN_POINT('Ctrl Pts',(-3.978938509,1.661171687,-6.366888754));
#138010=CARTESIAN_POINT('Ctrl Pts',(-4.263024558,1.716105035,-6.170625707));
#138011=CARTESIAN_POINT('',(-3.56402331316047,1.58673401455072,-6.59907098094287));
#138012=CARTESIAN_POINT('',(-4.05472873457929,1.67637477916353,-6.3094512345042));
#138013=CARTESIAN_POINT('Ctrl Pts',(-3.56402331229197,1.58673401558767,
-6.59907098222207));
#138014=CARTESIAN_POINT('Ctrl Pts',(-3.60223885805523,1.5935560516628,-6.57843154770463));
#138015=CARTESIAN_POINT('Ctrl Pts',(-3.64024060934755,1.60035948085481,
-6.55747875709107));
#138016=CARTESIAN_POINT('Ctrl Pts',(-3.67802110594051,1.60714285701092,
-6.53621914792779));
#138017=CARTESIAN_POINT('Ctrl Pts',(-3.80538617878491,1.63001087933882,
-6.46454905554143));
#138018=CARTESIAN_POINT('Ctrl Pts',(-3.93107498717681,1.65310706301777,
-6.38891652970493));
#138019=CARTESIAN_POINT('Ctrl Pts',(-4.0547287309188,1.67637477803959,-6.30945123659626));
#138020=CARTESIAN_POINT('Ctrl Pts',(-3.9190894175443,1.71532338703037,-6.09944572512069));
#138021=CARTESIAN_POINT('Ctrl Pts',(-3.94175986227678,1.70851142704216,
-6.13433434944167));
#138022=CARTESIAN_POINT('Ctrl Pts',(-3.96440810447552,1.70186463314016,
-6.16930110495159));
#138023=CARTESIAN_POINT('Ctrl Pts',(-4.00961044632058,1.68889233604367,
-6.23929283370253));
#138024=CARTESIAN_POINT('Ctrl Pts',(-4.03219137397222,1.68255913650916,
-6.27435936226819));
#138025=CARTESIAN_POINT('Ctrl Pts',(-4.05472873831957,1.67637477936948,
-6.30945123213834));
#138026=CARTESIAN_POINT('',(-3.39909364966914,1.58673401368624,-6.54386451677612));
#138027=CARTESIAN_POINT('Origin',(-1.49619899803E-14,1.67745375800056,1.30104260698261E-14));
#138028=CARTESIAN_POINT('',(-4.04868167575622,1.49654505838002,-6.31333324677893));
#138029=CARTESIAN_POINT('Origin',(0.105820797630874,1.48214573279163,0.160711178895498));
#138030=CARTESIAN_POINT('',(-4.51649917455081,1.58673401540864,-5.98759010069407));
#138031=CARTESIAN_POINT('Origin',(0.077858890967587,1.33942797597349,0.167803995583545));
#138032=CARTESIAN_POINT('Origin',(0.126541175047707,1.48219933721307,0.139950647587942));
#138033=CARTESIAN_POINT('Ctrl Pts',(-3.91515514,1.716084912,-6.101971831));
#138034=CARTESIAN_POINT('Ctrl Pts',(-4.246795545,1.651909459,-5.889184282));
#138035=CARTESIAN_POINT('Ctrl Pts',(-4.553420698,1.586734015,-5.641707183));
#138036=CARTESIAN_POINT('Ctrl Pts',(-4.56386473620058,1.58451405743873,
-5.63327780187965));
#138037=CARTESIAN_POINT('Ctrl Pts',(-4.57430877440114,1.58229409987748,
-5.62484842075922));
#138038=CARTESIAN_POINT('Ctrl Pts',(-3.84081398363992,1.716084912,-6.44250554223807));
#138039=CARTESIAN_POINT('Ctrl Pts',(-4.19096229675586,1.651909459,-6.2337584125284));
#138040=CARTESIAN_POINT('Ctrl Pts',(-4.51642423897335,1.586734015,-5.98829206201134));
#138041=CARTESIAN_POINT('Ctrl Pts',(-4.52750988189632,1.58451405743873,
-5.9799311695122));
#138042=CARTESIAN_POINT('Ctrl Pts',(-4.53859552481923,1.58229409987747,
-5.97157027701318));
#138043=CARTESIAN_POINT('',(-4.53495994002295,1.58673401622024,-5.81464863880259));
#138044=CARTESIAN_POINT('Ctrl Pts',(-4.553420698,1.586734015,-5.641707183));
#138045=CARTESIAN_POINT('Ctrl Pts',(-4.602383621,1.596957843,-5.602189219));
#138046=CARTESIAN_POINT('Ctrl Pts',(-4.650653287,1.607142857,-5.561827398));
#138047=CARTESIAN_POINT('Ctrl Pts',(-4.906711204,1.661171687,-5.347718525));
#138048=CARTESIAN_POINT('Ctrl Pts',(-5.142013183,1.716105035,-5.110988204));
#138049=CARTESIAN_POINT('Ctrl Pts',(-4.899303619,1.586734015,-5.678628712));
#138050=CARTESIAN_POINT('Ctrl Pts',(-4.948586973,1.596957843,-5.636108919));
#138051=CARTESIAN_POINT('Ctrl Pts',(-4.997124924,1.607142857,-5.59274016));
#138052=CARTESIAN_POINT('Ctrl Pts',(-5.254606016,1.661171687,-5.36268027));
#138053=CARTESIAN_POINT('Ctrl Pts',(-5.489859537,1.716105035,-5.109935642));
#138054=CARTESIAN_POINT('',(-4.89930362251769,1.58673401411985,-5.67862870804427));
#138055=CARTESIAN_POINT('',(-5.31627693897885,1.67637478034043,-5.29029295069965));
#138056=CARTESIAN_POINT('Ctrl Pts',(-4.89930362211821,1.58673401434301,
-5.67862870931878));
#138057=CARTESIAN_POINT('Ctrl Pts',(-4.93218884071548,1.59355605125262,
-5.65025660069274));
#138058=CARTESIAN_POINT('Ctrl Pts',(-4.96479790140868,1.60035948085479,
-5.62162442138197));
#138059=CARTESIAN_POINT('Ctrl Pts',(-4.99712492354918,1.60714285723698,
-5.59274016010432));
#138060=CARTESIAN_POINT('Ctrl Pts',(-5.10610532116016,1.6300108792918,-5.49536594898596));
#138061=CARTESIAN_POINT('Ctrl Pts',(-5.21259683738857,1.65310706412193,
-5.39448229136159));
#138062=CARTESIAN_POINT('Ctrl Pts',(-5.31627693626695,1.67637478135681,
-5.29029295378962));
#138063=CARTESIAN_POINT('Ctrl Pts',(-5.13866381750373,1.71532338696521,
-5.11435569607225));
#138064=CARTESIAN_POINT('Ctrl Pts',(-5.16830424634674,1.70851143073915,
-5.14355515230682));
#138065=CARTESIAN_POINT('Ctrl Pts',(-5.19793978547661,1.70186464073664,
-5.17283568354511));
#138066=CARTESIAN_POINT('Ctrl Pts',(-5.2571315092576,1.6888923360179,-5.23147391192988));
#138067=CARTESIAN_POINT('Ctrl Pts',(-5.28672277448894,1.68255913648335,
-5.26086637267337));
#138068=CARTESIAN_POINT('Ctrl Pts',(-5.3162769424568,1.67637477935555,-5.29029294699963));
#138069=CARTESIAN_POINT('',(-4.726362164702,1.58673401368602,-5.6601679423212));
#138070=CARTESIAN_POINT('Origin',(5.96311194867027E-13,1.67745375799967,
5.55111512312578E-13));
#138071=CARTESIAN_POINT('',(-5.31120577464674,1.49654505840871,-5.29538414253195));
#138072=CARTESIAN_POINT('Origin',(0.137894918178038,1.48214572826549,0.134205497018995));
#138073=CARTESIAN_POINT('',(-5.69806081408171,1.58673401497662,-4.87668975361135));
#138074=CARTESIAN_POINT('Origin',(0.112111456014379,1.33942796695583,0.147143430278365));
#138075=CARTESIAN_POINT('Origin',(0.153667784907622,1.48219935481058,0.109475894747609));
#138076=CARTESIAN_POINT('Ctrl Pts',(-5.135364559,1.716084912,-5.11766849700001));
#138077=CARTESIAN_POINT('Ctrl Pts',(-5.413508362,1.651909459,-4.838562918));
#138078=CARTESIAN_POINT('Ctrl Pts',(-5.65976453,1.586734015,-4.530956353));
#138079=CARTESIAN_POINT('Ctrl Pts',(-5.66815232495067,1.58451405736592,
-4.52047888632921));
#138080=CARTESIAN_POINT('Ctrl Pts',(-5.67654011990131,1.58229409973185,
-4.51000141965846));
#138081=CARTESIAN_POINT('Ctrl Pts',(-5.13596613941497,1.716084912,-5.46622186993683));
#138082=CARTESIAN_POINT('Ctrl Pts',(-5.4330537173179,1.651909459,-5.18708359571734));
#138083=CARTESIAN_POINT('Ctrl Pts',(-5.69813853004114,1.586734015,-4.8773914146006));
#138084=CARTESIAN_POINT('Ctrl Pts',(-5.70716765232347,1.58451405736592,
-4.86684290922051));
#138085=CARTESIAN_POINT('Ctrl Pts',(-5.71619677460589,1.58229409973185,
-4.85629440384044));
#138086=CARTESIAN_POINT('',(-5.67891267437233,1.58673401622024,-4.70382305061765));
#138087=CARTESIAN_POINT('Ctrl Pts',(-5.65976453,1.586734015,-4.530956353));
#138088=CARTESIAN_POINT('Ctrl Pts',(-5.699087532,1.596957843,-4.481836715));
#138089=CARTESIAN_POINT('Ctrl Pts',(-5.737552082,1.607142857,-4.43204198));
#138090=CARTESIAN_POINT('Ctrl Pts',(-5.941596428,1.661171687,-4.167893971));
#138091=CARTESIAN_POINT('Ctrl Pts',(-6.120507157,1.716105035,-3.886115303));
#138092=CARTESIAN_POINT('Ctrl Pts',(-6.005497937,1.586734015,-4.492660073));
#138093=CARTESIAN_POINT('Ctrl Pts',(-6.044488575,1.596957843,-4.440539904));
#138094=CARTESIAN_POINT('Ctrl Pts',(-6.082568734,1.607142857,-4.387750858));
#138095=CARTESIAN_POINT('Ctrl Pts',(-6.284573986,1.661171687,-4.107718817));
#138096=CARTESIAN_POINT('Ctrl Pts',(-6.459994786,1.716105035,-3.810310665));
#138097=CARTESIAN_POINT('',(-6.00549793922469,1.5867340145539,-4.49266006883129));
#138098=CARTESIAN_POINT('',(-6.32924194324064,1.67637477916489,-4.023766446818));
#138099=CARTESIAN_POINT('Ctrl Pts',(-6.00549793924492,1.58673401558864,
-4.49266006999914));
#138100=CARTESIAN_POINT('Ctrl Pts',(-6.03151515499356,1.59355605166312,
-4.45788193471596));
#138101=CARTESIAN_POINT('Ctrl Pts',(-6.0572067617763,1.6003594808548,-4.4229091754408));
#138102=CARTESIAN_POINT('Ctrl Pts',(-6.08256873376882,1.60714285700729,
-4.38775085799541));
#138103=CARTESIAN_POINT('Ctrl Pts',(-6.16806865231114,1.63001087932493,
-4.26922563809061));
#138104=CARTESIAN_POINT('Ctrl Pts',(-6.25038345283621,1.65310706301181,
-4.14780805601408));
#138105=CARTESIAN_POINT('Ctrl Pts',(-6.329241940739,1.67637477801304,-4.0237664503399));
#138106=CARTESIAN_POINT('Ctrl Pts',(-6.11796000837387,1.7153233870224,-3.89012407945758));
#138107=CARTESIAN_POINT('Ctrl Pts',(-6.15318448065138,1.7085114307687,-3.91226905256771));
#138108=CARTESIAN_POINT('Ctrl Pts',(-6.18842160622695,1.70186464073718,
-3.93449425635916));
#138109=CARTESIAN_POINT('Ctrl Pts',(-6.25883494579709,1.68889233608524,
-3.97903708417286));
#138110=CARTESIAN_POINT('Ctrl Pts',(-6.29405289406707,1.68255913651809,
-4.00138111820375));
#138111=CARTESIAN_POINT('Ctrl Pts',(-6.32924194570051,1.67637477937598,
-4.02376644300949));
#138112=CARTESIAN_POINT('',(-5.83263123845116,1.58673401368404,-4.51180820659941));
#138113=CARTESIAN_POINT('Origin',(8.00574884163296E-13,1.6774537580005,
5.19549681055054E-13));
#138114=CARTESIAN_POINT('',(-6.32538379609198,1.49654505840891,-4.02982876001943));
#138115=CARTESIAN_POINT('Origin',(0.163521297462732,1.48214578095595,0.101424576443183));
#138116=CARTESIAN_POINT('',(-6.61318746238814,1.58673401497662,-3.53776081556057));
#138117=CARTESIAN_POINT('Origin',(0.141121857032126,1.33942798108242,0.119602660461818));
#138118=CARTESIAN_POINT('Origin',(0.173609169352683,1.48219938729381,0.0738823743943423));
#138119=CARTESIAN_POINT('Ctrl Pts',(-6.115450039,1.716084912,-3.894068671));
#138120=CARTESIAN_POINT('Ctrl Pts',(-6.327091546,1.651909459,-3.56169573));
#138121=CARTESIAN_POINT('Ctrl Pts',(-6.501464062,1.586734015,-3.208343039));
#138122=CARTESIAN_POINT('Ctrl Pts',(-6.50740340903144,1.58451405747043,
-3.1963074022811));
#138123=CARTESIAN_POINT('Ctrl Pts',(-6.51334275606286,1.58229409994087,
-3.18427176556214));
#138124=CARTESIAN_POINT('Ctrl Pts',(-6.19096622721656,1.716084912,-4.23434373838217));
#138125=CARTESIAN_POINT('Ctrl Pts',(-6.42110158486059,1.651909459,-3.8978665147459));
#138126=CARTESIAN_POINT('Ctrl Pts',(-6.61341419795615,1.586734015,-3.53842936554782));
#138127=CARTESIAN_POINT('Ctrl Pts',(-6.61996460724023,1.58451405747043,
-3.52618648453627));
#138128=CARTESIAN_POINT('Ctrl Pts',(-6.62651501652436,1.58229409994087,
-3.51394360352467));
#138129=CARTESIAN_POINT('',(-6.55732576399389,1.58673401622024,-3.37305192420777));
#138130=CARTESIAN_POINT('Ctrl Pts',(-6.501464062,1.586734015,-3.208343039));
#138131=CARTESIAN_POINT('Ctrl Pts',(-6.529308444,1.596957843,-3.151918508));
#138132=CARTESIAN_POINT('Ctrl Pts',(-6.556169318,1.607142857,-3.095019205));
#138133=CARTESIAN_POINT('Ctrl Pts',(-6.698659207,1.661171687,-2.793183326));
#138134=CARTESIAN_POINT('Ctrl Pts',(-6.812813018,1.716105035,-2.479531969));
#138135=CARTESIAN_POINT('Ctrl Pts',(-6.830881846,1.586734015,-3.096619642));
#138136=CARTESIAN_POINT('Ctrl Pts',(-6.85775661,1.596957843,-3.037336179));
#138137=CARTESIAN_POINT('Ctrl Pts',(-6.883598391,1.607142857,-2.977595203));
#138138=CARTESIAN_POINT('Ctrl Pts',(-7.020682261,1.661171687,-2.660684997));
#138139=CARTESIAN_POINT('Ctrl Pts',(-7.128067859,1.716105035,-2.332519796));
#138140=CARTESIAN_POINT('',(-6.83088184728289,1.58673401455455,-3.09661963745425));
#138141=CARTESIAN_POINT('',(-7.04625862555874,1.67637477889898,-2.56909310230143));
#138142=CARTESIAN_POINT('Ctrl Pts',(-6.83088184754511,1.5867340155878,-3.09661963859161));
#138143=CARTESIAN_POINT('Ctrl Pts',(-6.84881452494674,1.59355605166285,
-3.05706166447727));
#138144=CARTESIAN_POINT('Ctrl Pts',(-6.86638736696152,1.60035948085478,
-3.01738361286274));
#138145=CARTESIAN_POINT('Ctrl Pts',(-6.88359839099221,1.60714285699693,
-2.97759520301802));
#138146=CARTESIAN_POINT('Ctrl Pts',(-6.94161994920343,1.63001087863148,
-2.84346108523285));
#138147=CARTESIAN_POINT('Ctrl Pts',(-6.99590908163633,1.65310706174197,
-2.70718693367039));
#138148=CARTESIAN_POINT('Ctrl Pts',(-7.04625862155055,1.67637477616413,
-2.56909311176525));
#138149=CARTESIAN_POINT('Ctrl Pts',(-6.81118718894288,1.71532338700859,
-2.48399458411567));
#138150=CARTESIAN_POINT('Ctrl Pts',(-6.85034866843755,1.70851142705774,
-2.49804960736224));
#138151=CARTESIAN_POINT('Ctrl Pts',(-6.88953975570717,1.70186463317932,
-2.51218026669214));
#138152=CARTESIAN_POINT('Ctrl Pts',(-6.96788221635299,1.6888923360513,-2.54054490485863));
#138153=CARTESIAN_POINT('Ctrl Pts',(-7.00708009495013,1.68255913655582,
-2.55479572977348));
#138154=CARTESIAN_POINT('Ctrl Pts',(-7.0462586293168,1.67637477940267,-2.56909309222123));
#138155=CARTESIAN_POINT('',(-6.6661729574545,1.58673401368593,-3.15248133319519));
#138156=CARTESIAN_POINT('Ctrl Pts',(-6.809583872,1.716084912,-2.488386523));
#138157=CARTESIAN_POINT('Ctrl Pts',(-6.94482696000001,1.651909459,-2.118287608));
#138158=CARTESIAN_POINT('Ctrl Pts',(-7.03916236,1.586734015,-1.73571117));
#138159=CARTESIAN_POINT('Ctrl Pts',(-7.04237554241109,1.58451405737756,
-1.72268013518725));
#138160=CARTESIAN_POINT('Ctrl Pts',(-7.04558872482218,1.58229409975514,
-1.70964910037451));
#138161=CARTESIAN_POINT('Ctrl Pts',(-6.95648361439213,1.716084912,-2.80447239967962));
#138162=CARTESIAN_POINT('Ctrl Pts',(-7.10890587835298,1.651909459,-2.42638952731729));
#138163=CARTESIAN_POINT('Ctrl Pts',(-7.21945396683182,1.586734015,-2.03401429125501));
#138164=CARTESIAN_POINT('Ctrl Pts',(-7.22321937381032,1.58451405737757,
-2.020649497052));
#138165=CARTESIAN_POINT('Ctrl Pts',(-7.22698478078881,1.58229409975514,
-2.00728470284901));
#138166=CARTESIAN_POINT('',(-7.21908881409604,1.58673401498684,-2.03341011390865));
#138167=CARTESIAN_POINT('Origin',(0.185432819398685,1.48219938584591,0.0348342073597357));
#138168=CARTESIAN_POINT('',(-7.12912558795207,1.58673401622024,-1.88456063811549));
#138169=CARTESIAN_POINT('Origin',(9.4542429440736E-13,1.67745375799972,
2.49366499671666E-13));
#138170=CARTESIAN_POINT('',(-7.04379390009598,1.49654505840544,-2.57584306385715));
#138171=CARTESIAN_POINT('Origin',(0.181501620529565,1.48214573542086,0.0639010986816974));
#138172=CARTESIAN_POINT('Origin',(0.163533519886799,1.33942795423984,0.086469386724336));
#138173=CARTESIAN_POINT('Ctrl Pts',(-7.03916236,1.586734015,-1.73571117));
#138174=CARTESIAN_POINT('Ctrl Pts',(-7.05422615,1.596957843,-1.674620094));
#138175=CARTESIAN_POINT('Ctrl Pts',(-7.068227363,1.607142857,-1.613276771));
#138176=CARTESIAN_POINT('Ctrl Pts',(-7.142500127,1.661171687,-1.287866533));
#138177=CARTESIAN_POINT('Ctrl Pts',(-7.186559314,1.716105035,-0.957008476));
#138178=CARTESIAN_POINT('Ctrl Pts',(-7.336861312,1.586734015,-1.555784718));
#138179=CARTESIAN_POINT('Ctrl Pts',(-7.350363566,1.596957843,-1.49210999));
#138180=CARTESIAN_POINT('Ctrl Pts',(-7.362758637,1.607142857,-1.428210506));
#138181=CARTESIAN_POINT('Ctrl Pts',(-7.428511236,1.661171687,-1.089240504));
#138182=CARTESIAN_POINT('Ctrl Pts',(-7.462840401,1.716105035,-0.745662894));
#138183=CARTESIAN_POINT('',(-7.33686131228108,1.58673401455507,-1.55578471328603));
#138184=CARTESIAN_POINT('',(-7.188011837802,1.58673401368697,-1.64574793612957));
#138185=CARTESIAN_POINT('',(-7.43380009082176,1.67637477914435,-0.994291808505194));
#138186=CARTESIAN_POINT('Ctrl Pts',(-7.33686131277568,1.58673401558734,
-1.55578471434202));
#138187=CARTESIAN_POINT('Ctrl Pts',(-7.34587093849314,1.59355605166269,
-1.51329658840759));
#138188=CARTESIAN_POINT('Ctrl Pts',(-7.354503328865,1.60035948085488,-1.47076854621938));
#138189=CARTESIAN_POINT('Ctrl Pts',(-7.36275863686387,1.60714285704628,
-1.42821050583054));
#138190=CARTESIAN_POINT('Ctrl Pts',(-7.39058881335076,1.63001087948788,
-1.28473944435232));
#138191=CARTESIAN_POINT('Ctrl Pts',(-7.41431378314698,1.65310706300321,
-1.13998074464423));
#138192=CARTESIAN_POINT('Ctrl Pts',(-7.43380009004028,1.6763747780124,-0.994291812679242));
#138193=CARTESIAN_POINT('Ctrl Pts',(-7.18593082707723,1.71532338700727,
-0.961716262227243));
#138194=CARTESIAN_POINT('Ctrl Pts',(-7.22719814866542,1.70851142685462,
-0.967024126647668));
#138195=CARTESIAN_POINT('Ctrl Pts',(-7.26851064495947,1.70186463284726,
-0.97239949394857));
#138196=CARTESIAN_POINT('Ctrl Pts',(-7.35111905906606,1.68889233602461,
-0.983259669302536));
#138197=CARTESIAN_POINT('Ctrl Pts',(-7.39246401931295,1.68255913649073,
-0.988750932741153));
#138198=CARTESIAN_POINT('Ctrl Pts',(-7.43380009144446,1.67637477935179,
-0.994291804091257));
#138199=CARTESIAN_POINT('Origin',(3.40439482160448E-13,1.67745375799922,
5.13640779215008E-14));
#138200=CARTESIAN_POINT('',(-7.4874335964436,1.58673401541129,-0.43397941779166));
#138201=CARTESIAN_POINT('Origin',(0.188585854968112,1.48219938148668,-0.00584277830929555));
#138202=CARTESIAN_POINT('',(-7.4328440300674,1.49654505822092,-1.00141380955591));
#138203=CARTESIAN_POINT('Origin',(0.190994941521154,1.48214558438775,0.0233895971421555));
#138204=CARTESIAN_POINT('Origin',(0.178298506284001,1.33942798528867,0.049292893791802));
#138205=CARTESIAN_POINT('Ctrl Pts',(-7.185309132,1.716084912,-0.966350186));
#138206=CARTESIAN_POINT('Ctrl Pts',(-7.23782998500001,1.651909459,-0.575830712));
#138207=CARTESIAN_POINT('Ctrl Pts',(-7.24771725000001,1.586734015,-0.181919376));
#138208=CARTESIAN_POINT('Ctrl Pts',(-7.24805402267975,1.58451405741505,
-0.168502260527041));
#138209=CARTESIAN_POINT('Ctrl Pts',(-7.24839079535963,1.58229409983011,
-0.155085145054078));
#138210=CARTESIAN_POINT('Ctrl Pts',(-7.3967235596348,1.716084912,-1.24346704850373));
#138211=CARTESIAN_POINT('Ctrl Pts',(-7.46430563398088,1.651909459,-0.841457262522982));
#138212=CARTESIAN_POINT('Ctrl Pts',(-7.48792009244461,1.586734015,-0.434490970580043));
#138213=CARTESIAN_POINT('Ctrl Pts',(-7.48872443059658,1.58451405741505,
-0.420629186890223));
#138214=CARTESIAN_POINT('Ctrl Pts',(-7.48952876874859,1.58229409983011,
-0.4067674032004));
#138215=CARTESIAN_POINT('',(-7.36757542331898,1.58673401622022,-0.307949391868585));
#138216=CARTESIAN_POINT('Ctrl Pts',(-7.24771725,1.586734015,-0.181919376));
#138217=CARTESIAN_POINT('Ctrl Pts',(-7.24929608200001,1.596957843,-0.119018306));
#138218=CARTESIAN_POINT('Ctrl Pts',(-7.249782953,1.607142857,-0.056099309));
#138219=CARTESIAN_POINT('Ctrl Pts',(-7.25236567800001,1.661171687,0.277669467));
#138220=CARTESIAN_POINT('Ctrl Pts',(-7.224270084,1.716105035,0.610263670000001));
#138221=CARTESIAN_POINT('Ctrl Pts',(-7.49977729699999,1.586734015,0.05779697));
#138222=CARTESIAN_POINT('Ctrl Pts',(-7.49927569200001,1.596957843,0.122885604));
#138223=CARTESIAN_POINT('Ctrl Pts',(-7.497644473,1.607142857,0.187955727));
#138224=CARTESIAN_POINT('Ctrl Pts',(-7.488991283,1.661171687,0.533135664000001));
#138225=CARTESIAN_POINT('Ctrl Pts',(-7.44865882,1.716105035,0.876060377));
#138226=CARTESIAN_POINT('',(-7.49977729625411,1.58673401455095,0.057796975121696));
#138227=CARTESIAN_POINT('',(-7.47374532379189,1.67637477914009,0.62700145943416));
#138228=CARTESIAN_POINT('Ctrl Pts',(-7.49977729697118,1.58673401558734,
0.0577969737392455));
#138229=CARTESIAN_POINT('Ctrl Pts',(-7.49944259184632,1.59355605166269,
0.101228554286963));
#138230=CARTESIAN_POINT('Ctrl Pts',(-7.49873088997243,1.60035948085494,
0.144618023182082));
#138231=CARTESIAN_POINT('Ctrl Pts',(-7.49764447287025,1.60714285707618,
0.18795572737095));
#138232=CARTESIAN_POINT('Ctrl Pts',(-7.49398195850961,1.63001087961635,
0.334055181280936));
#138233=CARTESIAN_POINT('Ctrl Pts',(-7.48603341016074,1.65310706300346,
0.480529669341363));
#138234=CARTESIAN_POINT('Ctrl Pts',(-7.47374532392755,1.67637477802169,
0.627001455243438));
#138235=CARTESIAN_POINT('Ctrl Pts',(-7.2246683252045,1.71532338708746,0.605530843116696));
#138236=CARTESIAN_POINT('Ctrl Pts',(-7.26611187320349,1.70851142700761,
0.60921832783714));
#138237=CARTESIAN_POINT('Ctrl Pts',(-7.30761405160807,1.70186463296282,
0.612849599107477));
#138238=CARTESIAN_POINT('Ctrl Pts',(-7.39062574460637,1.6888923360062,0.620001695686318));
#138239=CARTESIAN_POINT('Ctrl Pts',(-7.43218454204251,1.68255913648216,
0.623526759146004));
#138240=CARTESIAN_POINT('Ctrl Pts',(-7.47374532345536,1.67637477934486,
0.627001463823824));
#138241=CARTESIAN_POINT('',(-7.37374727356795,1.58673401368695,-0.0620611949261003));
#138242=CARTESIAN_POINT('Origin',(-9.14632952708772E-13,1.67745375800011,
2.80537312130624E-15));
#138243=CARTESIAN_POINT('',(-7.47434263494036,1.49654505840813,0.619840442693668));
#138244=CARTESIAN_POINT('Origin',(0.191557338754434,1.48214579038053,-0.0182154483195574));
#138245=CARTESIAN_POINT('',(-7.40567430550057,1.58673401497661,1.18574367902254));
#138246=CARTESIAN_POINT('Origin',(0.18472656006578,1.33942794290295,0.00981153906990759));
#138247=CARTESIAN_POINT('Origin',(0.182920782974308,1.48219935504351,-0.0462465674927783));
#138248=CARTESIAN_POINT('Ctrl Pts',(-7.225057322,1.716084912,0.600871612));
#138249=CARTESIAN_POINT('Ctrl Pts',(-7.192400124,1.651909459,0.993551388));
#138250=CARTESIAN_POINT('Ctrl Pts',(-7.117376937,1.586734015,1.380378766));
#138251=CARTESIAN_POINT('Ctrl Pts',(-7.1148215528193,1.5845140573412,1.39355459339328));
#138252=CARTESIAN_POINT('Ctrl Pts',(-7.1122661686386,1.58229409968241,1.40673042078652));
#138253=CARTESIAN_POINT('Ctrl Pts',(-7.49110093223557,1.716084912,0.375681439552532));
#138254=CARTESIAN_POINT('Ctrl Pts',(-7.47068275461875,1.651909459,0.782820608983368));
#138255=CARTESIAN_POINT('Ctrl Pts',(-7.4062593970554,1.586734015,1.18534866545931));
#138256=CARTESIAN_POINT('Ctrl Pts',(-7.40406505640728,1.5845140573412,1.19905927772388));
#138257=CARTESIAN_POINT('Ctrl Pts',(-7.40187071575919,1.58229409968241,
1.21276988998847));
#138258=CARTESIAN_POINT('',(-7.261525620671,1.58673401622021,1.28306122602152));
#138259=CARTESIAN_POINT('Ctrl Pts',(-7.117376937,1.586734015,1.380378766));
#138260=CARTESIAN_POINT('Ctrl Pts',(-7.105396986,1.596957843,1.442148645));
#138261=CARTESIAN_POINT('Ctrl Pts',(-7.09234675,1.607142857,1.503701295));
#138262=CARTESIAN_POINT('Ctrl Pts',(-7.023118672,1.661171687,1.830221952));
#138263=CARTESIAN_POINT('Ctrl Pts',(-6.924182015,1.716105035,2.149000565));
#138264=CARTESIAN_POINT('Ctrl Pts',(-7.312012032,1.586734015,1.668676136));
#138265=CARTESIAN_POINT('Ctrl Pts',(-7.297530022,1.596957843,1.732135204));
#138266=CARTESIAN_POINT('Ctrl Pts',(-7.281948786,1.607142857,1.79533336));
#138267=CARTESIAN_POINT('Ctrl Pts',(-7.19929442,1.661171687,2.130583001));
#138268=CARTESIAN_POINT('Ctrl Pts',(-7.086186231,1.716105035,2.456820037));
#138269=CARTESIAN_POINT('',(-7.31201203007812,1.58673401412069,1.66867614091693));
#138270=CARTESIAN_POINT('',(-7.16422653185322,1.67637478035133,2.21897683545438));
#138271=CARTESIAN_POINT('Ctrl Pts',(-7.31201203089279,1.58673401434349,
1.66867613996222));
#138272=CARTESIAN_POINT('Ctrl Pts',(-7.30234864499606,1.59355605125278,
1.71102036257308));
#138273=CARTESIAN_POINT('Ctrl Pts',(-7.29232612896216,1.60035948085479,
1.75324241500101));
#138274=CARTESIAN_POINT('Ctrl Pts',(-7.28194878628072,1.60714285723673,
1.79533336012697));
#138275=CARTESIAN_POINT('Ctrl Pts',(-7.24696483610422,1.6300108792978,1.93722975618628));
#138276=CARTESIAN_POINT('Ctrl Pts',(-7.20771443454255,1.65310706412798,
2.07857105028278));
#138277=CARTESIAN_POINT('Ctrl Pts',(-7.16422653331938,1.67637478135684,
2.21897683162364));
#138278=CARTESIAN_POINT('Ctrl Pts',(-6.92558836329049,1.71532338701588,
2.14446399814966));
#138279=CARTESIAN_POINT('Ctrl Pts',(-6.96527028317949,1.70851142707599,
2.15697440921553));
#138280=CARTESIAN_POINT('Ctrl Pts',(-7.00502154671859,1.70186463319256,
2.1694425247741));
#138281=CARTESIAN_POINT('Ctrl Pts',(-7.08455498415042,1.68889233605714,
2.1942724700893));
#138282=CARTESIAN_POINT('Ctrl Pts',(-7.12438437564887,1.68255913650904,
2.20664903265677));
#138283=CARTESIAN_POINT('Ctrl Pts',(-7.16422653021818,1.67637477937239,
2.21897684024757));
#138284=CARTESIAN_POINT('',(-7.21469448283075,1.58673401368698,1.52452745889956));
#138285=CARTESIAN_POINT('Origin',(4.69676381120721E-13,1.67745375799961,
-1.7499023063916E-13));
#138286=CARTESIAN_POINT('',(-7.16634928489004,1.49654505824553,2.21211164336113));
#138287=CARTESIAN_POINT('Origin',(0.183163363348232,1.48214558960764,-0.058968873837181));
#138288=CARTESIAN_POINT('',(-6.97763391702804,1.58673401540863,2.75002271427369));
#138289=CARTESIAN_POINT('Origin',(0.182516852866949,1.3394279789947,-0.0301285564507109));
#138290=CARTESIAN_POINT('Origin',(0.168702839582741,1.4821993589666,-0.0844879943072543));
#138291=CARTESIAN_POINT('Ctrl Pts',(-6.926969862,1.716084912,2.13999732));
#138292=CARTESIAN_POINT('Ctrl Pts',(-6.810661627,1.651909459,2.516476129));
#138293=CARTESIAN_POINT('Ctrl Pts',(-6.654235988,1.586734015,2.878131931));
#138294=CARTESIAN_POINT('Ctrl Pts',(-6.64890793416401,1.58451405747489,
2.89045038208945));
#138295=CARTESIAN_POINT('Ctrl Pts',(-6.6435798803279,1.5822940999498,2.90276883317886));
#138296=CARTESIAN_POINT('Ctrl Pts',(-7.23520275053982,1.716084912,1.977263481934));
#138297=CARTESIAN_POINT('Ctrl Pts',(-7.12773905188058,1.651909459,2.37049465845346));
#138298=CARTESIAN_POINT('Ctrl Pts',(-6.97829024445302,1.586734015,2.74976271555198));
#138299=CARTESIAN_POINT('Ctrl Pts',(-6.9731998302678,1.58451405747489,2.76268106218245));
#138300=CARTESIAN_POINT('Ctrl Pts',(-6.96810941608252,1.5822940999498,2.77559940881284));
#138301=CARTESIAN_POINT('',(-6.81593495058514,1.58673401622023,2.81407732706006));
#138302=CARTESIAN_POINT('Ctrl Pts',(-6.654235988,1.586734015,2.878131931));
#138303=CARTESIAN_POINT('Ctrl Pts',(-6.629257423,1.596957843,2.935882329));
#138304=CARTESIAN_POINT('Ctrl Pts',(-6.603280295,1.607142857,2.993190497));
#138305=CARTESIAN_POINT('Ctrl Pts',(-6.465478441,1.661171687,3.297195292));
#138306=CARTESIAN_POINT('Ctrl Pts',(-6.30032689000001,1.716105035,3.587252582));
#138307=CARTESIAN_POINT('Ctrl Pts',(-6.78234521,1.586734015,3.201529861));
#138308=CARTESIAN_POINT('Ctrl Pts',(-6.754559958,1.596957843,3.260392086));
#138309=CARTESIAN_POINT('Ctrl Pts',(-6.725757268,1.607142857,3.3187632));
#138310=CARTESIAN_POINT('Ctrl Pts',(-6.572966551,1.661171687,3.628406645));
#138311=CARTESIAN_POINT('Ctrl Pts',(-6.39237145,1.716105035,3.922701524));
#138312=CARTESIAN_POINT('',(-6.78234520716232,1.58673401412049,3.20152986547042));
#138313=CARTESIAN_POINT('',(-6.51971646961656,1.67637478034357,3.70719532168303));
#138314=CARTESIAN_POINT('Ctrl Pts',(-6.78234520833718,1.58673401434349,
3.20152986475931));
#138315=CARTESIAN_POINT('Ctrl Pts',(-6.76380499121345,1.59355605125278,
3.24080675989459));
#138316=CARTESIAN_POINT('Ctrl Pts',(-6.74494030295206,1.60035948085479,
3.27988713929682));
#138317=CARTESIAN_POINT('Ctrl Pts',(-6.72575726772998,1.60714285723673,
3.31876319968409));
#138318=CARTESIAN_POINT('Ctrl Pts',(-6.66108769201959,1.63001087928986,
3.44982162195314));
#138319=CARTESIAN_POINT('Ctrl Pts',(-6.59237074276419,1.65310706411997,
3.57942075914026));
#138320=CARTESIAN_POINT('Ctrl Pts',(-6.51971647182816,1.67637478135681,
3.707195318158));
#138321=CARTESIAN_POINT('Ctrl Pts',(-6.30267558623198,1.7153233870683,3.58312440106051));
#138322=CARTESIAN_POINT('Ctrl Pts',(-6.33874037621333,1.70851143090008,
3.60387275388008));
#138323=CARTESIAN_POINT('Ctrl Pts',(-6.37488197802835,1.70186464092893,
3.62459470539109));
#138324=CARTESIAN_POINT('Ctrl Pts',(-6.44721830671353,1.6888923360433,3.66594150307704));
#138325=CARTESIAN_POINT('Ctrl Pts',(-6.48345591407357,1.68255913648982,
3.68659085031422));
#138326=CARTESIAN_POINT('Ctrl Pts',(-6.51971646694944,1.67637477935982,
3.70719532608147));
#138327=CARTESIAN_POINT('',(-6.71829059567161,1.58673401368698,3.03983090335604));
#138328=CARTESIAN_POINT('Origin',(-2.04697370165263E-13,1.67745375799961,
1.346579098227E-13));
#138329=CARTESIAN_POINT('',(-6.52326540700298,1.49654505841246,3.70094696342879));
#138330=CARTESIAN_POINT('Origin',(0.166204606236854,1.48214575970179,-0.0969649219425217));
#138331=CARTESIAN_POINT('',(-6.22332711995983,1.58673401540865,4.1857137457124));
#138332=CARTESIAN_POINT('Origin',(0.17177301985814,1.33942795617175,-0.068659935349929));
#138333=CARTESIAN_POINT('Origin',(0.146596010498544,1.48219934874745,-0.118778704936435));
#138334=CARTESIAN_POINT('Ctrl Pts',(-6.30498499000001,1.716084912,3.579059133));
#138335=CARTESIAN_POINT('Ctrl Pts',(-6.110464161,1.651909459,3.921733244));
#138336=CARTESIAN_POINT('Ctrl Pts',(-5.87995036100001,1.586734015,4.241306845));
#138337=CARTESIAN_POINT('Ctrl Pts',(-5.87209877115736,1.5845140574352,4.25219192363558));
#138338=CARTESIAN_POINT('Ctrl Pts',(-5.86424718131484,1.58229409987042,
4.26307700227107));
#138339=CARTESIAN_POINT('Ctrl Pts',(-6.64099453017892,1.716084912,3.48639088073289));
#138340=CARTESIAN_POINT('Ctrl Pts',(-6.45151019387323,1.651909459,3.84732701283999));
#138341=CARTESIAN_POINT('Ctrl Pts',(-6.22402399484519,1.586734015,4.18560091662383));
#138342=CARTESIAN_POINT('Ctrl Pts',(-6.21627552889814,1.5845140574352,4.19712295108326));
#138343=CARTESIAN_POINT('Ctrl Pts',(-6.20852706295096,1.58229409987042,
4.20864498554271));
#138344=CARTESIAN_POINT('',(-6.05163873763563,1.58673401622021,4.21351029926832));
#138345=CARTESIAN_POINT('Ctrl Pts',(-5.879950361,1.586734015,4.241306845));
#138346=CARTESIAN_POINT('Ctrl Pts',(-5.843141152,1.596957843,4.292337419));
#138347=CARTESIAN_POINT('Ctrl Pts',(-5.805451792,1.607142857,4.342721438));
#138348=CARTESIAN_POINT('Ctrl Pts',(-5.605519625,1.661171687,4.609995445));
#138349=CARTESIAN_POINT('Ctrl Pts',(-5.381875481,1.716105035,4.857768655));
#138350=CARTESIAN_POINT('Ctrl Pts',(-5.935543465,1.586734015,4.584683607));
#138351=CARTESIAN_POINT('Ctrl Pts',(-5.895754178,1.596957843,4.636196659));
#138352=CARTESIAN_POINT('Ctrl Pts',(-5.855076814,1.607142857,4.687011361));
#138353=CARTESIAN_POINT('Ctrl Pts',(-5.639294072,1.661171687,4.956570027));
#138354=CARTESIAN_POINT('Ctrl Pts',(-5.399656485,1.716105035,5.205161847));
#138355=CARTESIAN_POINT('',(-5.93554346122076,1.58673401412049,4.58468361069456));
#138356=CARTESIAN_POINT('',(-5.57035171146692,1.67637478034078,5.02206947459704));
#138357=CARTESIAN_POINT('Ctrl Pts',(-5.93554346242469,1.58673401434348,
4.58468361020337));
#138358=CARTESIAN_POINT('Ctrl Pts',(-5.908993333447,1.59355605125278,4.61905663523161));
#138359=CARTESIAN_POINT('Ctrl Pts',(-5.88216856458618,1.60035948085479,
4.65316798694213));
#138360=CARTESIAN_POINT('Ctrl Pts',(-5.85507681426963,1.60714285723673,
4.68701136109163));
#138361=CARTESIAN_POINT('Ctrl Pts',(-5.76374549062467,1.63001087929165,
4.80110366304963));
#138362=CARTESIAN_POINT('Ctrl Pts',(-5.6687751219266,1.65310706412178,4.9129007315449));
#138363=CARTESIAN_POINT('Ctrl Pts',(-5.57035171433747,1.67637478135681,
5.02206947169965));
#138364=CARTESIAN_POINT('Ctrl Pts',(-5.38505670288533,1.7153233870728,4.85424188880678));
#138365=CARTESIAN_POINT('Ctrl Pts',(-5.41581803545826,1.70851143101226,
4.88225801990094));
#138366=CARTESIAN_POINT('Ctrl Pts',(-5.44666005950121,1.70186464111915,
4.91026487937284));
#138367=CARTESIAN_POINT('Ctrl Pts',(-5.50841686694514,1.68889233603578,
4.96619518521198));
#138368=CARTESIAN_POINT('Ctrl Pts',(-5.53936825983376,1.68255913650977,
4.99415177652447));
#138369=CARTESIAN_POINT('Ctrl Pts',(-5.57035170798474,1.67637477936395,
5.02206947824522));
#138370=CARTESIAN_POINT('',(-5.90774690816807,1.58673401368697,4.41299523246859));
#138371=CARTESIAN_POINT('Origin',(-2.94902990916057E-13,1.67745375800039,
3.69062419514066E-13));
#138372=CARTESIAN_POINT('',(-5.57516088947637,1.4965450584209,5.01673011568442));
#138373=CARTESIAN_POINT('Origin',(0.141473953944199,1.48214574136492,-0.130426776897208));
#138374=CARTESIAN_POINT('',(-5.17802446096194,1.58673401497661,5.4256854564893));
#138375=CARTESIAN_POINT('Origin',(0.152997134318694,1.33942795405182,-0.103980765192834));
#138376=CARTESIAN_POINT('Origin',(0.11763457126844,1.48219938277928,-0.147515345083278));
#138377=CARTESIAN_POINT('Ctrl Pts',(-5.388186027,1.716084912,4.850768118));
#138378=CARTESIAN_POINT('Ctrl Pts',(-5.124548183,1.651909459,5.14361447));
#138379=CARTESIAN_POINT('Ctrl Pts',(-4.830724789,1.586734015,5.406162966));
#138380=CARTESIAN_POINT('Ctrl Pts',(-4.8207167940839,1.5845140572787,5.41510569849458));
#138381=CARTESIAN_POINT('Ctrl Pts',(-4.81070879916784,1.58229409955743,
5.42404843098929));
#138382=CARTESIAN_POINT('Ctrl Pts',(-5.73626078559967,1.716084912,4.83249851653737));
#138383=CARTESIAN_POINT('Ctrl Pts',(-5.47361588967387,1.651909459,5.14426263175886));
#138384=CARTESIAN_POINT('Ctrl Pts',(-5.17872930032388,1.586734015,5.42572507124403));
#138385=CARTESIAN_POINT('Ctrl Pts',(-5.1686850916349,1.5845140572787,5.43531203647878));
#138386=CARTESIAN_POINT('Ctrl Pts',(-5.15864088294596,1.58229409955742,
5.44489900171361));
#138387=CARTESIAN_POINT('',(-5.00437462239016,1.58673401622021,5.41592421368356));
#138388=CARTESIAN_POINT('Ctrl Pts',(-4.830724789,1.586734015,5.406162966));
#138389=CARTESIAN_POINT('Ctrl Pts',(-4.783806095,1.596957843,5.448087581));
#138390=CARTESIAN_POINT('Ctrl Pts',(-4.736166816,1.607142857,5.489191552));
#138391=CARTESIAN_POINT('Ctrl Pts',(-4.483452941,1.661171687,5.707237335));
#138392=CARTESIAN_POINT('Ctrl Pts',(-4.211773557,1.716105035,5.901140864));
#138393=CARTESIAN_POINT('Ctrl Pts',(-4.811202304,1.586734015,5.753462644));
#138394=CARTESIAN_POINT('Ctrl Pts',(-4.761269485,1.596957843,5.795217828));
#138395=CARTESIAN_POINT('Ctrl Pts',(-4.710619476,1.607142857,5.83610008));
#138396=CARTESIAN_POINT('Ctrl Pts',(-4.44193447,1.661171687,6.052969703));
#138397=CARTESIAN_POINT('Ctrl Pts',(-4.154459583,1.716105035,6.244234587));
#138398=CARTESIAN_POINT('',(-4.81120229945899,1.58673401412069,5.75346264667531));
#138399=CARTESIAN_POINT('',(-4.36052349819178,1.67637478035157,6.10211724071305));
#138400=CARTESIAN_POINT('Ctrl Pts',(-4.81120230059445,1.58673401434349,
5.75346264633348));
#138401=CARTESIAN_POINT('Ctrl Pts',(-4.77788371487983,1.59355605125278,
5.78132455595149));
#138402=CARTESIAN_POINT('Ctrl Pts',(-4.74435316195746,1.60035948085479,
5.80887187081411));
#138403=CARTESIAN_POINT('Ctrl Pts',(-4.71061947665077,1.60714285723673,
5.83610008020754));
#138404=CARTESIAN_POINT('Ctrl Pts',(-4.59689695616064,1.63001087929168,
5.92789143275329));
#138405=CARTESIAN_POINT('Ctrl Pts',(-4.48011387691959,1.65310706412176,
6.01665892591959));
#138406=CARTESIAN_POINT('Ctrl Pts',(-4.36052350170302,1.67637478135664,
6.10211723839322));
#138407=CARTESIAN_POINT('Ctrl Pts',(-4.21563855474019,1.7153233868915,5.89838042160329));
#138408=CARTESIAN_POINT('Ctrl Pts',(-4.2396580786889,1.70851142675315,5.93235434885314));
#138409=CARTESIAN_POINT('Ctrl Pts',(-4.2637584022233,1.70186463282375,5.96633656926233));
#138410=CARTESIAN_POINT('Ctrl Pts',(-4.3120479764043,1.68889233603723,6.03423510042615));
#138411=CARTESIAN_POINT('Ctrl Pts',(-4.33626590225745,1.68255913648983,
6.06819171687066));
#138412=CARTESIAN_POINT('Ctrl Pts',(-4.36052349387761,1.67637477936853,
6.10211724361858));
#138413=CARTESIAN_POINT('',(-4.82096354039051,1.58673401368698,5.5798128102786));
#138414=CARTESIAN_POINT('Origin',(-4.59918561568351E-13,1.67745375799967,
6.99960922556642E-13));
#138415=CARTESIAN_POINT('',(-4.36636804460131,1.49654505819906,6.0979365443449));
#138416=CARTESIAN_POINT('Origin',(0.110128493780438,1.48214560147655,-0.157790257786166));
#138417=CARTESIAN_POINT('',(-3.89060313579184,1.58673401497661,6.41195814384654));
#138418=CARTESIAN_POINT('Origin',(0.127067328912721,1.33942798463397,-0.134439566054244));
#138419=CARTESIAN_POINT('Origin',(0.0831730144276299,1.48219940270008,-0.169354622117295));
#138420=CARTESIAN_POINT('Ctrl Pts',(-4.219441475,1.716084912,5.895660577));
#138421=CARTESIAN_POINT('Ctrl Pts',(-3.899014027,1.651909459,6.124986001));
#138422=CARTESIAN_POINT('Ctrl Pts',(-3.555619896,1.586734015,6.318232914));
#138423=CARTESIAN_POINT('Ctrl Pts',(-3.54392346041923,1.58451405748362,
6.32481514667389));
#138424=CARTESIAN_POINT('Ctrl Pts',(-3.53222702483845,1.58229409996724,
6.33139737934781));
#138425=CARTESIAN_POINT('Ctrl Pts',(-4.56330586303262,1.716084912,5.95264389354036));
#138426=CARTESIAN_POINT('Ctrl Pts',(-4.2397813894512,1.651909459,6.20065824728892));
#138427=CARTESIAN_POINT('Ctrl Pts',(-3.89128298046772,1.586734015,6.4121483522595));
#138428=CARTESIAN_POINT('Ctrl Pts',(-3.87941268676526,1.58451405748362,
6.41935197097467));
#138429=CARTESIAN_POINT('Ctrl Pts',(-3.86754239306272,1.58229409996724,
6.42655558968996));
#138430=CARTESIAN_POINT('',(-3.72311151290708,1.58673401622019,6.36509553085638));
#138431=CARTESIAN_POINT('Ctrl Pts',(-3.555619896,1.586734015,6.318232914));
#138432=CARTESIAN_POINT('Ctrl Pts',(-3.500785581,1.596957843,6.34909122300001));
#138433=CARTESIAN_POINT('Ctrl Pts',(-3.445423944,1.607142857,6.378993169));
#138434=CARTESIAN_POINT('Ctrl Pts',(-3.15174498,1.661171687,6.53761515));
#138435=CARTESIAN_POINT('Ctrl Pts',(-2.844733783,1.716105035,6.668582286));
#138436=CARTESIAN_POINT('Ctrl Pts',(-3.46189467,1.586734015,6.653216162));
#138437=CARTESIAN_POINT('Ctrl Pts',(-3.404153122,1.596957843,6.683261053));
#138438=CARTESIAN_POINT('Ctrl Pts',(-3.345898807,1.607142857,6.712299246));
#138439=CARTESIAN_POINT('Ctrl Pts',(-3.036874949,1.661171687,6.86633924400001));
#138440=CARTESIAN_POINT('Ctrl Pts',(-2.715004769,1.716105035,6.991333857));
#138441=CARTESIAN_POINT('',(-3.46189466553869,1.5867340145549,6.653216163509));
#138442=CARTESIAN_POINT('',(-2.94680205198768,1.67637477917517,6.89683678639208));
#138443=CARTESIAN_POINT('Ctrl Pts',(-3.46189466668291,1.58673401558733,
6.653216163726));
#138444=CARTESIAN_POINT('Ctrl Pts',(-3.42336556352834,1.59355605166269,
6.67326416630461));
#138445=CARTESIAN_POINT('Ctrl Pts',(-3.38469707774585,1.60035948085472,
6.69295936235249));
#138446=CARTESIAN_POINT('Ctrl Pts',(-3.34589880719225,1.60714285696639,
6.71229924590417));
#138447=CARTESIAN_POINT('Ctrl Pts',(-3.21510262968249,1.63001087914796,
6.77749758707386));
#138448=CARTESIAN_POINT('Ctrl Pts',(-3.08196748589179,1.65310706302618,
6.83908483597189));
#138449=CARTESIAN_POINT('Ctrl Pts',(-2.94680205576956,1.67637477805243,
6.89683678453843));
#138450=CARTESIAN_POINT('Ctrl Pts',(-2.8491018325826,1.71532338701036,6.66671724050236));
#138451=CARTESIAN_POINT('Ctrl Pts',(-2.86525640264206,1.70851142706009,
6.70506036268628));
#138452=CARTESIAN_POINT('Ctrl Pts',(-2.881488100747,1.70186463322583,6.74342895411978));
#138453=CARTESIAN_POINT('Ctrl Pts',(-2.91405251523444,1.68889233606425,
6.82012088845218));
#138454=CARTESIAN_POINT('Ctrl Pts',(-2.93040457065015,1.6825591365248,6.85848975614808));
#138455=CARTESIAN_POINT('Ctrl Pts',(-2.94680204793491,1.67637477938092,
6.89683678815825));
#138456=CARTESIAN_POINT('',(-3.50875727589861,1.58673401368698,6.48572454184184));
#138457=CARTESIAN_POINT('Origin',(7.02563007770607E-14,1.67745375799983,
-7.28583859910259E-14));
#138458=CARTESIAN_POINT('',(-2.95340868202948,1.49654505841521,6.89401023776211));
#138459=CARTESIAN_POINT('Origin',(0.0736336045579739,1.4821457425204,-0.177775726754538));
#138460=CARTESIAN_POINT('',(-2.4212615321408,1.58673401497661,7.0984147942295));
#138461=CARTESIAN_POINT('Origin',(0.0951960600761595,1.33942795485371,-0.158612234490675));
#138462=CARTESIAN_POINT('Origin',(0.0448223004672105,1.48219937047135,-0.183275116942858));
#138463=CARTESIAN_POINT('Ctrl Pts',(-2.853400528,1.716084912,6.6648785));
#138464=CARTESIAN_POINT('Ctrl Pts',(-2.491166309,1.651909459,6.819959994));
#138465=CARTESIAN_POINT('Ctrl Pts',(-2.114258167,1.586734015,6.934869314));
#138466=CARTESIAN_POINT('Ctrl Pts',(-2.10142020173575,1.5845140574217,6.93878326993332));
#138467=CARTESIAN_POINT('Ctrl Pts',(-2.08858223647144,1.58229409984341,
6.94269722586663));
#138468=CARTESIAN_POINT('Ctrl Pts',(-3.17697582941391,1.716084912,6.79445025702993));
#138469=CARTESIAN_POINT('Ctrl Pts',(-2.80769942347321,1.651909459,6.96711797440578));
#138470=CARTESIAN_POINT('Ctrl Pts',(-2.42188459325229,1.586734015,7.09874670217079));
#138471=CARTESIAN_POINT('Ctrl Pts',(-2.4087432549874,1.5845140574217,7.10323014215661));
#138472=CARTESIAN_POINT('Ctrl Pts',(-2.39560191672256,1.58229409984341,
7.10771358214244));
#138473=CARTESIAN_POINT('',(-2.26775984623204,1.58673401622023,7.01664205534898));
#138474=CARTESIAN_POINT('Ctrl Pts',(-2.114258167,1.586734015,6.934869314));
#138475=CARTESIAN_POINT('Ctrl Pts',(-2.054072224,1.596957843,6.95321841600001));
#138476=CARTESIAN_POINT('Ctrl Pts',(-1.993576877,1.607142857,6.970520155));
#138477=CARTESIAN_POINT('Ctrl Pts',(-1.672664928,1.661171687,7.06230134600001));
#138478=CARTESIAN_POINT('Ctrl Pts',(-1.344677418,1.716105035,7.124208212));
#138479=CARTESIAN_POINT('Ctrl Pts',(-1.95071269,1.586734015,7.241872686));
#138480=CARTESIAN_POINT('Ctrl Pts',(-1.887862343,1.596957843,7.258802419));
#138481=CARTESIAN_POINT('Ctrl Pts',(-1.824727629,1.607142857,7.274638759));
#138482=CARTESIAN_POINT('Ctrl Pts',(-1.48981453,1.661171687,7.358646393));
#138483=CARTESIAN_POINT('Ctrl Pts',(-1.148599349,1.716105035,7.411526127));
#138484=CARTESIAN_POINT('',(-1.95071268475582,1.58673401412067,7.24187268671358));
#138485=CARTESIAN_POINT('',(-1.39529141789594,1.67637478035405,7.36906790958503));
#138486=CARTESIAN_POINT('Ctrl Pts',(-1.95071268604658,1.58673401434349,
7.24187268712292));
#138487=CARTESIAN_POINT('Ctrl Pts',(-1.90877464357686,1.59355605125278,
7.25316936065035));
#138488=CARTESIAN_POINT('Ctrl Pts',(-1.86677632062753,1.60035948085479,
7.26409151275274));
#138489=CARTESIAN_POINT('Ctrl Pts',(-1.82472762875065,1.60714285723673,
7.27463875947624));
#138490=CARTESIAN_POINT('Ctrl Pts',(-1.68297367624678,1.63001087929739,
7.31019548774422));
#138491=CARTESIAN_POINT('Ctrl Pts',(-1.53971172097606,1.65310706412721,
7.34172274042649));
#138492=CARTESIAN_POINT('Ctrl Pts',(-1.39529142198336,1.67637478135573,
7.3690679090194));
#138493=CARTESIAN_POINT('Ctrl Pts',(-1.349344274309,1.71532338715986,7.12332577116148));
#138494=CARTESIAN_POINT('Ctrl Pts',(-1.35687852187631,1.70851142713905,
7.16424520772288));
#138495=CARTESIAN_POINT('Ctrl Pts',(-1.36448261923405,1.70186463308513,
7.20520609934646));
#138496=CARTESIAN_POINT('Ctrl Pts',(-1.37979919683592,1.68889233604116,
7.28710540449341));
#138497=CARTESIAN_POINT('Ctrl Pts',(-1.38752077788562,1.68255913650202,
7.32809243790103));
#138498=CARTESIAN_POINT('Ctrl Pts',(-1.39529141286165,1.6763747793784,7.36906791039249));
#138499=CARTESIAN_POINT('',(-2.03248542073876,1.58673401368698,7.08837100222542));
#138500=CARTESIAN_POINT('Origin',(2.86988315056913E-13,1.67745375800067,
-1.91426735574041E-12));
#138501=CARTESIAN_POINT('',(-1.40235121259847,1.49654505820771,7.36772767361412));
#138502=CARTESIAN_POINT('Origin',(0.0336955570525715,1.48214561198427,-0.189448532417833));
#138503=CARTESIAN_POINT('',(-0.838704434774169,1.58673401541122,7.45295745902514));
#138504=CARTESIAN_POINT('Origin',(0.058873471499683,1.3394279908441,-0.175368207935244));
#138505=CARTESIAN_POINT('Origin',(0.00437563783938805,1.48219935231658,
-0.18862567772804));
#138506=CARTESIAN_POINT('Ctrl Pts',(-1.353937744,1.716084912,7.122454113));
#138507=CARTESIAN_POINT('Ctrl Pts',(-0.966834423,1.651909459,7.196040237));
#138508=CARTESIAN_POINT('Ctrl Pts',(-0.574036077,1.586734015,7.227238932));
#138509=CARTESIAN_POINT('Ctrl Pts',(-0.560656871444095,1.58451405742799,
7.22830159877987));
#138510=CARTESIAN_POINT('Ctrl Pts',(-0.547277665888199,1.582294099856,7.22936426555975));
#138511=CARTESIAN_POINT('Ctrl Pts',(-1.64209393708288,1.716084912,7.3185556786243));
#138512=CARTESIAN_POINT('Ctrl Pts',(-1.24433255270257,1.651909459,7.40780300915423));
#138513=CARTESIAN_POINT('Ctrl Pts',(-0.839241573735745,1.586734015,7.45341554632637));
#138514=CARTESIAN_POINT('Ctrl Pts',(-0.825443665644656,1.58451405742799,
7.4549691666941));
#138515=CARTESIAN_POINT('Ctrl Pts',(-0.811645757553577,1.582294099856,7.45652278706179));
#138516=CARTESIAN_POINT('',(-0.706370249897001,1.58673401622023,7.34009819573167));
#138517=CARTESIAN_POINT('Origin',(3.25802752831894E-14,1.67745375800039,
5.0263612716428E-13));
#138518=CARTESIAN_POINT('',(0.214278640529097,1.49654505838871,7.49693835249985));
#138519=CARTESIAN_POINT('',(-0.34831754416533,1.58673401414387,7.49190729318426));
#138520=CARTESIAN_POINT('Origin',(-0.00781804144820934,1.48214575524756,
-0.192262944512581));
#138521=CARTESIAN_POINT('Origin',(0.0197980510459872,1.33942797864341,-0.183924310824504));
#138522=CARTESIAN_POINT('Ctrl Pts',(-0.348317544006022,1.5867340149536,
7.49190729310884));
#138523=CARTESIAN_POINT('Ctrl Pts',(-0.304931542030917,1.59355605145578,
7.49392441706153));
#138524=CARTESIAN_POINT('Ctrl Pts',(-0.261567178121288,1.60035948085479,
7.49556281730996));
#138525=CARTESIAN_POINT('Ctrl Pts',(-0.218234214930498,1.60714285723674,
7.49682424946948));
#138526=CARTESIAN_POINT('Ctrl Pts',(-0.0721507453448591,1.63001087927846,
7.501076771636));
#138527=CARTESIAN_POINT('Ctrl Pts',(0.0745392523939352,1.65310706410833,
7.50106984908632));
#138528=CARTESIAN_POINT('Ctrl Pts',(0.221461488025658,1.67637478135631,
7.49672960759033));
#138529=CARTESIAN_POINT('Ctrl Pts',(-0.574036077,1.586734015,7.227238932));
#138530=CARTESIAN_POINT('Ctrl Pts',(-0.511312734,1.596957843,7.23222084300001));
#138531=CARTESIAN_POINT('Ctrl Pts',(-0.448512371,1.607142857,7.236113367));
#138532=CARTESIAN_POINT('Ctrl Pts',(-0.115372922,1.661171687,7.256762181));
#138533=CARTESIAN_POINT('Ctrl Pts',(0.218254568,1.716105035,7.246714079));
#138534=CARTESIAN_POINT('Ctrl Pts',(-0.348317552,1.586734015,7.491907293));
#138535=CARTESIAN_POINT('Ctrl Pts',(-0.28329722,1.596957843,7.494930251));
#138536=CARTESIAN_POINT('Ctrl Pts',(-0.218234215,1.607142857,7.496824249));
#138537=CARTESIAN_POINT('Ctrl Pts',(0.12690796,1.661171687,7.506871415));
#138538=CARTESIAN_POINT('Ctrl Pts',(0.4715133,1.716105035,7.485163673));
#138539=CARTESIAN_POINT('',(-0.461176806441667,1.58673401368695,7.35957311300496));
#138540=CARTESIAN_POINT('Ctrl Pts',(-1.16218918388351,4.30331728230629,
7.40941170763586));
#138541=CARTESIAN_POINT('Ctrl Pts',(-1.15818926544175,4.30267205415314,
7.41003468381793));
#138542=CARTESIAN_POINT('Ctrl Pts',(-1.154189347,4.302026826,7.41065766));
#138543=CARTESIAN_POINT('Ctrl Pts',(-0.752921796,4.237298226,7.473153966));
#138544=CARTESIAN_POINT('Ctrl Pts',(-0.347252113,4.172121859,7.49195675200001));
#138545=CARTESIAN_POINT('Ctrl Pts',(-1.35774016039859,4.30331728230629,
7.12173454350632));
#138546=CARTESIAN_POINT('Ctrl Pts',(-1.35389540219929,4.30267205415314,
7.12246323625316));
#138547=CARTESIAN_POINT('Ctrl Pts',(-1.350050644,4.302026826,7.123191929));
#138548=CARTESIAN_POINT('Ctrl Pts',(-0.964348603,4.237298226,7.196293608));
#138549=CARTESIAN_POINT('Ctrl Pts',(-0.573008275,4.172121859,7.227320494));
#138550=CARTESIAN_POINT('',(-0.596334988833243,4.21216499469303,7.47625471614313));
#138551=CARTESIAN_POINT('Ctrl Pts',(-0.596334996445509,4.21216499507849,
7.47625471552231));
#138552=CARTESIAN_POINT('Ctrl Pts',(-0.593257936526993,4.20594050668202,
7.43465989744348));
#138553=CARTESIAN_POINT('Ctrl Pts',(-0.590163983306183,4.19956141145742,
7.39306522936547));
#138554=CARTESIAN_POINT('Ctrl Pts',(-0.583946887358536,4.18648410045661,
7.30997722747781));
#138555=CARTESIAN_POINT('Ctrl Pts',(-0.58082009119411,4.17977820241928,
7.2684350382799));
#138556=CARTESIAN_POINT('Ctrl Pts',(-0.577677422272544,4.17289950750523,
7.22694879429211));
#138557=CARTESIAN_POINT('',(-1.15418934995013,4.30202682545374,7.41065766134707));
#138558=CARTESIAN_POINT('Origin',(0.00695330665491684,4.16072878976292,
-0.19114668498882));
#138559=CARTESIAN_POINT('',(-1.252120005472,4.30202682438465,7.26692479278178));
#138560=CARTESIAN_POINT('Ctrl Pts',(-2.429504099,4.172114527,7.095597919));
#138561=CARTESIAN_POINT('Ctrl Pts',(-2.089017748,4.22940039,7.212179072));
#138562=CARTESIAN_POINT('Ctrl Pts',(-1.738933089,4.285714286,7.295622778));
#138563=CARTESIAN_POINT('Ctrl Pts',(-1.688306028,4.29385805,7.307689886));
#138564=CARTESIAN_POINT('Ctrl Pts',(-1.637516375,4.302026826,7.319053226));
#138565=CARTESIAN_POINT('Ctrl Pts',(-2.12231099,4.172114527,6.932409109));
#138566=CARTESIAN_POINT('Ctrl Pts',(-1.789655348,4.22940039,7.034249424));
#138567=CARTESIAN_POINT('Ctrl Pts',(-1.448776863,4.285714286,7.103769816));
#138568=CARTESIAN_POINT('Ctrl Pts',(-1.399481142,4.29385805,7.11382342199999));
#138569=CARTESIAN_POINT('Ctrl Pts',(-1.350050644,4.302026826,7.12319192899999));
#138570=CARTESIAN_POINT('',(-1.63751638118266,4.30202682641445,7.31905322493326));
#138571=CARTESIAN_POINT('',(-1.49378351347216,4.30202682665757,7.2211225766783));
#138572=CARTESIAN_POINT('',(-2.18956677646246,4.21216499392671,7.17326964037794));
#138573=CARTESIAN_POINT('Ctrl Pts',(-1.63751638169652,4.30202682552111,
7.31905322426853));
#138574=CARTESIAN_POINT('Ctrl Pts',(-1.67140098825403,4.29657697961046,
7.31147210733645));
#138575=CARTESIAN_POINT('Ctrl Pts',(-1.70520808357999,4.29113922035365,
7.3036612314913));
#138576=CARTESIAN_POINT('Ctrl Pts',(-1.73893308847754,4.28571428571329,
7.29562277765223));
#138577=CARTESIAN_POINT('Ctrl Pts',(-1.88988482580287,4.26143250098634,
7.25964298829109));
#138578=CARTESIAN_POINT('Ctrl Pts',(-2.04024794992858,4.23689343089983,
7.21884767604786));
#138579=CARTESIAN_POINT('Ctrl Pts',(-2.18956676991572,4.21216499285672,
7.17326964222597));
#138580=CARTESIAN_POINT('Ctrl Pts',(-2.11775200805595,4.17289950701588,
6.9338031746523));
#138581=CARTESIAN_POINT('Ctrl Pts',(-2.1297395193464,4.17977820193676,6.97364391235997));
#138582=CARTESIAN_POINT('Ctrl Pts',(-2.14172355644561,4.18648410048624,
7.01354270257986));
#138583=CARTESIAN_POINT('Ctrl Pts',(-2.16565676462317,4.19956141148085,
7.09335166142063));
#138584=CARTESIAN_POINT('Ctrl Pts',(-2.17762000701025,4.20594050665356,
7.13330876057114));
#138585=CARTESIAN_POINT('Ctrl Pts',(-2.18956678338983,4.21216499505426,
7.17326963813129));
#138586=CARTESIAN_POINT('Ctrl Pts',(-2.7278223432099,4.30331728230629,6.98634745883686));
#138587=CARTESIAN_POINT('Ctrl Pts',(-2.72404986210495,4.30267205415314,
6.98781573441843));
#138588=CARTESIAN_POINT('Ctrl Pts',(-2.720277381,4.302026826,6.98928401000001));
#138589=CARTESIAN_POINT('Ctrl Pts',(-2.341826101,4.237298226,7.13657985));
#138590=CARTESIAN_POINT('Ctrl Pts',(-1.949682793,4.172121859,7.242150027));
#138591=CARTESIAN_POINT('Ctrl Pts',(-2.85695935998706,4.30331728230629,
6.66335834764232));
#138592=CARTESIAN_POINT('Ctrl Pts',(-2.85336113749353,4.30267205415314,
6.66489651332116));
#138593=CARTESIAN_POINT('Ctrl Pts',(-2.849762915,4.302026826,6.666434679));
#138594=CARTESIAN_POINT('Ctrl Pts',(-2.488793073,4.237298226,6.820741819));
#138595=CARTESIAN_POINT('Ctrl Pts',(-2.113271928,4.172121859,6.935169916));
#138596=CARTESIAN_POINT('',(-2.72027738416813,4.30202682545393,6.98928401068239));
#138597=CARTESIAN_POINT('Origin',(0.0478815511175334,4.16072878634873,-0.185182782745746));
#138598=CARTESIAN_POINT('',(-2.78502015736614,4.30202682438522,6.82785934067964));
#138599=CARTESIAN_POINT('Origin',(-2.65629532258949E-14,4.39277644300044,
3.06178693509906E-13));
#138600=CARTESIAN_POINT('',(-2.18434923164388,4.39169923735961,7.17486016787817));
#138601=CARTESIAN_POINT('Origin',(0.0183603401161009,4.16082469438197,-0.185324740864866));
#138602=CARTESIAN_POINT('Origin',(0.0286009939169851,4.55341984216358,-0.182407753897521));
#138603=CARTESIAN_POINT('Ctrl Pts',(-3.898047452,4.172114527,6.407435217));
#138604=CARTESIAN_POINT('Ctrl Pts',(-3.590582984,4.22940039,6.594485268));
#138605=CARTESIAN_POINT('Ctrl Pts',(-3.26662104,4.285714286,6.75123596));
#138606=CARTESIAN_POINT('Ctrl Pts',(-3.219771683,4.29385805,6.77390426700001));
#138607=CARTESIAN_POINT('Ctrl Pts',(-3.172612246,4.302026826,6.795920213));
#138608=CARTESIAN_POINT('Ctrl Pts',(-3.562955577,4.172114527,6.31409910900001));
#138609=CARTESIAN_POINT('Ctrl Pts',(-3.259969896,4.22940039,6.485069584));
#138610=CARTESIAN_POINT('Ctrl Pts',(-2.94200579,4.285714286,6.626243425));
#138611=CARTESIAN_POINT('Ctrl Pts',(-2.896023804,4.29385805,6.646659106));
#138612=CARTESIAN_POINT('Ctrl Pts',(-2.849762915,4.302026826,6.666434679));
#138613=CARTESIAN_POINT('',(-3.17261225178721,4.30202682641445,6.79592021059555));
#138614=CARTESIAN_POINT('',(-3.01118758420266,4.30202682665757,6.73117744434362));
#138615=CARTESIAN_POINT('',(-3.68041685431122,4.21216499393234,6.53487044845151));
#138616=CARTESIAN_POINT('Ctrl Pts',(-3.17261225212519,4.30202682552111,
6.79592020977771));
#138617=CARTESIAN_POINT('Ctrl Pts',(-3.20407493953318,4.29657697961046,
6.78123214628165));
#138618=CARTESIAN_POINT('Ctrl Pts',(-3.23541253640356,4.29113922035365,
6.76633635817626));
#138619=CARTESIAN_POINT('Ctrl Pts',(-3.26662103946589,4.28571428571329,
6.75123595977202));
#138620=CARTESIAN_POINT('Ctrl Pts',(-3.40630901782547,4.26143250099806,
6.68364719650128));
#138621=CARTESIAN_POINT('Ctrl Pts',(-3.54438694943116,4.23689343091171,
6.61148202900684));
#138622=CARTESIAN_POINT('Ctrl Pts',(-3.68041684841466,4.21216499285689,
6.5348704518074));
#138623=CARTESIAN_POINT('Ctrl Pts',(-3.55880286439848,4.17289950713874,
6.31644062907105));
#138624=CARTESIAN_POINT('Ctrl Pts',(-3.57907469528383,4.17977820208842,
6.35277295199961));
#138625=CARTESIAN_POINT('Ctrl Pts',(-3.59935561209294,4.18648410044242,
6.38916271579995));
#138626=CARTESIAN_POINT('Ctrl Pts',(-3.63988584216034,4.19956141147502,
6.4619608532525));
#138627=CARTESIAN_POINT('Ctrl Pts',(-3.66015898579949,4.20594050667283,
6.498412034188));
#138628=CARTESIAN_POINT('Ctrl Pts',(-3.6804168605763,4.21216499507368,6.53487044477551));
#138629=CARTESIAN_POINT('Ctrl Pts',(-4.16590556149365,4.30331728230629,
6.23660936793102));
#138630=CARTESIAN_POINT('Ctrl Pts',(-4.16253691474683,4.30267205415314,
6.23885428796551));
#138631=CARTESIAN_POINT('Ctrl Pts',(-4.159168268,4.302026826,6.241099208));
#138632=CARTESIAN_POINT('Ctrl Pts',(-3.82122922,4.237298226,6.466307191));
#138633=CARTESIAN_POINT('Ctrl Pts',(-3.460948472,4.172121859,6.653708415));
#138634=CARTESIAN_POINT('Ctrl Pts',(-4.22259031477876,4.30331728230629,
5.8934109206062));
#138635=CARTESIAN_POINT('Ctrl Pts',(-4.21940687688938,4.30267205415314,
5.8956866363031));
#138636=CARTESIAN_POINT('Ctrl Pts',(-4.216223439,4.302026826,5.897962352));
#138637=CARTESIAN_POINT('Ctrl Pts',(-3.896864346,4.237298226,6.126259723));
#138638=CARTESIAN_POINT('Ctrl Pts',(-3.554721335,4.172121859,6.3187385));
#138639=CARTESIAN_POINT('',(-4.1591682712504,4.30202682545375,6.24109920797393));
#138640=CARTESIAN_POINT('Origin',(0.0865709208982096,4.16072878307092,-0.170560193251753));
#138641=CARTESIAN_POINT('',(-4.18769586182889,4.30202682438465,6.06953077425346));
#138642=CARTESIAN_POINT('Origin',(-2.08166817117217E-14,4.39277644300022,
1.63931368479808E-13));
#138643=CARTESIAN_POINT('',(-3.6756632088494,4.39169923737625,6.53754540854676));
#138644=CARTESIAN_POINT('Origin',(0.0577704175562865,4.16082470835826,-0.177044994129791));
#138645=CARTESIAN_POINT('Origin',(0.0671445342074956,4.55341983699392,-0.171994702565974));
#138646=CARTESIAN_POINT('Ctrl Pts',(-5.18432243800001,4.172114527,5.419667966));
#138647=CARTESIAN_POINT('Ctrl Pts',(-4.92425655,4.22940039,5.668440663));
#138648=CARTESIAN_POINT('Ctrl Pts',(-4.641565421,4.285714286,5.891168852));
#138649=CARTESIAN_POINT('Ctrl Pts',(-4.600684393,4.29385805,5.923378414));
#138650=CARTESIAN_POINT('Ctrl Pts',(-4.55936029400001,4.302026826,5.955017524));
#138651=CARTESIAN_POINT('Ctrl Pts',(-4.83700032,4.172114527,5.400548852));
#138652=CARTESIAN_POINT('Ctrl Pts',(-4.577851874,4.22940039,5.632655097));
#138653=CARTESIAN_POINT('Ctrl Pts',(-4.297669796,4.285714286,5.838881257));
#138654=CARTESIAN_POINT('Ctrl Pts',(-4.25715161,4.29385805,5.868704398));
#138655=CARTESIAN_POINT('Ctrl Pts',(-4.216223439,4.302026826,5.897962352));
#138656=CARTESIAN_POINT('',(-4.55936029919639,4.30202682641445,5.9550175204685));
#138657=CARTESIAN_POINT('',(-4.38779186976002,4.30202682665757,5.92648993558638));
#138658=CARTESIAN_POINT('',(-4.99917473014842,4.21216499393112,5.59090797795424));
#138659=CARTESIAN_POINT('Ctrl Pts',(-4.55936029942192,4.30202682552111,
5.95501751971019));
#138660=CARTESIAN_POINT('Ctrl Pts',(-4.58692990753124,4.29657697961046,
5.93390930696889));
#138661=CARTESIAN_POINT('Ctrl Pts',(-4.61433269467468,4.29113922035365,
5.91262511711567));
#138662=CARTESIAN_POINT('Ctrl Pts',(-4.6415654209329,4.28571428571329,5.89116885203607));
#138663=CARTESIAN_POINT('Ctrl Pts',(-4.76345798551428,4.26143250100584,
5.79513149051414));
#138664=CARTESIAN_POINT('Ctrl Pts',(-4.88279435397564,4.23689343091949,
5.69497083082674));
#138665=CARTESIAN_POINT('Ctrl Pts',(-4.99917472505921,4.21216499285672,
5.59090798245948));
#138666=CARTESIAN_POINT('Ctrl Pts',(-4.83344805250004,4.17289950697198,
5.40372833833061));
#138667=CARTESIAN_POINT('Ctrl Pts',(-4.86105631482581,4.17977820193647,
5.43485338735993));
#138668=CARTESIAN_POINT('Ctrl Pts',(-4.88868579927659,4.18648410044146,
5.46603258182227));
#138669=CARTESIAN_POINT('Ctrl Pts',(-4.94391790281236,4.19956141147817,
5.52841593800416));
#138670=CARTESIAN_POINT('Ctrl Pts',(-4.97155299800196,4.20594050666816,
5.55965678400575));
#138671=CARTESIAN_POINT('Ctrl Pts',(-4.99917473548726,4.2121649950684,5.59090797300892));
#138672=CARTESIAN_POINT('Ctrl Pts',(-5.40919566542744,4.30331728230629,
5.19525435393708));
#138673=CARTESIAN_POINT('Ctrl Pts',(-5.40638836721372,4.30267205415314,
5.19817094846854));
#138674=CARTESIAN_POINT('Ctrl Pts',(-5.403581069,4.302026826,5.201087543));
#138675=CARTESIAN_POINT('Ctrl Pts',(-5.121955907,4.237298226,5.493677195));
#138676=CARTESIAN_POINT('Ctrl Pts',(-4.810384047,4.172121859,5.754146794));
#138677=CARTESIAN_POINT('Ctrl Pts',(-5.39077763956017,4.30331728230629,
4.84789414945679));
#138678=CARTESIAN_POINT('Ctrl Pts',(-5.38815784028008,4.30267205415314,
4.8508010052284));
#138679=CARTESIAN_POINT('Ctrl Pts',(-5.385538041,4.302026826,4.853707861));
#138680=CARTESIAN_POINT('Ctrl Pts',(-5.122722572,4.237298226,5.145320531));
#138681=CARTESIAN_POINT('Ctrl Pts',(-4.829955922,4.172121859,5.406849895));
#138682=CARTESIAN_POINT('',(-5.40358107215755,4.30202682545392,5.2010875422987));
#138683=CARTESIAN_POINT('Origin',(0.121212436242013,4.1607287553436,-0.147962496286492));
#138684=CARTESIAN_POINT('',(-5.39455956189629,4.30202682438524,5.02739769460006));
#138685=CARTESIAN_POINT('Origin',(4.87457296749483E-13,4.39277644300022,
-4.17634676841416E-13));
#138686=CARTESIAN_POINT('',(-4.9951072604849,4.3916992374024,5.59454229148361));
#138687=CARTESIAN_POINT('Origin',(0.0944792292999891,4.16082469009487,-0.160486871840761));
#138688=CARTESIAN_POINT('Origin',(0.102548316312207,4.55341980934995,-0.153539253888896));
#138689=CARTESIAN_POINT('Ctrl Pts',(-6.228184269,4.172114527,4.178483064));
#138690=CARTESIAN_POINT('Ctrl Pts',(-6.027677353,4.22940039,4.477346072));
#138691=CARTESIAN_POINT('Ctrl Pts',(-5.799475362,4.285714286,4.755637236));
#138692=CARTESIAN_POINT('Ctrl Pts',(-5.766474213,4.29385805,4.795881969));
#138693=CARTESIAN_POINT('Ctrl Pts',(-5.73291772300001,4.302026826,4.835664834));
#138694=CARTESIAN_POINT('Ctrl Pts',(-5.884872305,4.172114527,4.234474933));
#138695=CARTESIAN_POINT('Ctrl Pts',(-5.681678587,4.22940039,4.516863918));
#138696=CARTESIAN_POINT('Ctrl Pts',(-5.452379538,4.285714286,4.77849949));
#138697=CARTESIAN_POINT('Ctrl Pts',(-5.419219739,4.29385805,4.81633559500001));
#138698=CARTESIAN_POINT('Ctrl Pts',(-5.385538041,4.302026826,4.853707861));
#138699=CARTESIAN_POINT('',(-5.73291772724476,4.30202682620655,4.83566482943548));
#138700=CARTESIAN_POINT('',(-5.55922788466495,4.30202682665757,4.844686344442));
#138701=CARTESIAN_POINT('',(-6.08417675202275,4.21216499536652,4.38552086333923));
#138702=CARTESIAN_POINT('Ctrl Pts',(-5.73291772722235,4.3020268248974,4.83566482864614));
#138703=CARTESIAN_POINT('Ctrl Pts',(-5.75530513081357,4.29657697940857,
4.80912346338663));
#138704=CARTESIAN_POINT('Ctrl Pts',(-5.77749178408189,4.29113922035363,
4.78244609672125));
#138705=CARTESIAN_POINT('Ctrl Pts',(-5.79947536162674,4.28571428598682,
4.75563723596294));
#138706=CARTESIAN_POINT('Ctrl Pts',(-5.89787295242218,4.26143250093749,
4.63564187593636));
#138707=CARTESIAN_POINT('Ctrl Pts',(-5.9928877215738,4.23689343233045,4.51216912531119));
#138708=CARTESIAN_POINT('Ctrl Pts',(-6.08417674795619,4.21216499709052,
4.38552086837866));
#138709=CARTESIAN_POINT('Ctrl Pts',(-5.88208658344157,4.17289950707543,
4.23834371760513));
#138710=CARTESIAN_POINT('Ctrl Pts',(-5.91574034525287,4.17977820202404,
4.26280611985181));
#138711=CARTESIAN_POINT('Ctrl Pts',(-5.9494264724858,4.18648410047085,4.28731683939213));
#138712=CARTESIAN_POINT('Ctrl Pts',(-6.01677785733755,4.19956141147629,
4.33636843760983));
#138713=CARTESIAN_POINT('Ctrl Pts',(-6.05048271772771,4.20594050667205,
4.36093816143897));
#138714=CARTESIAN_POINT('Ctrl Pts',(-6.08417675605191,4.21216499505843,
4.3855208578947));
#138715=CARTESIAN_POINT('Ctrl Pts',(-6.3995577920639,4.30331728230629,3.91097502038183));
#138716=CARTESIAN_POINT('Ctrl Pts',(-6.39744310853195,4.30267205415314,
3.91442691269092));
#138717=CARTESIAN_POINT('Ctrl Pts',(-6.395328425,4.302026826,3.917878805));
#138718=CARTESIAN_POINT('Ctrl Pts',(-6.18318562899999,4.237298226,4.264168959));
#138719=CARTESIAN_POINT('Ctrl Pts',(-5.93489141,4.172121859,4.585527663));
#138720=CARTESIAN_POINT('Ctrl Pts',(-6.30689819352099,4.30331728230629,
3.57569523599079));
#138721=CARTESIAN_POINT('Ctrl Pts',(-6.30496453176049,4.30267205415314,
3.5790973104954));
#138722=CARTESIAN_POINT('Ctrl Pts',(-6.30303087000001,4.302026826,3.582499385));
#138723=CARTESIAN_POINT('Ctrl Pts',(-6.109047985,4.237298226,3.92379187));
#138724=CARTESIAN_POINT('Ctrl Pts',(-5.879347139,4.172121859,4.242142999));
#138725=CARTESIAN_POINT('',(-6.39532842773336,4.30202682545334,3.91787880426053));
#138726=CARTESIAN_POINT('Origin',(0.150186028649116,4.16072874257247,-0.118446067871733));
#138727=CARTESIAN_POINT('',(-6.34917965264429,4.30202682438524,3.75018908629057));
#138728=CARTESIAN_POINT('Origin',(-3.88578058618805E-13,4.392776443,2.26381413614973E-13));
#138729=CARTESIAN_POINT('',(-6.08098564727151,4.3916992373645,4.38994459505378));
#138730=CARTESIAN_POINT('Origin',(0.12677023788604,4.1608246923527,-0.136424485744108));
#138731=CARTESIAN_POINT('Origin',(0.133157392753959,4.55341981119211,-0.12790486823742));
#138732=CARTESIAN_POINT('Ctrl Pts',(-6.980823125,4.172114527,2.741916938));
#138733=CARTESIAN_POINT('Ctrl Pts',(-6.849250662,4.22940039,3.076895755));
#138734=CARTESIAN_POINT('Ctrl Pts',(-6.686208281,4.285714286,3.397737309));
#138735=CARTESIAN_POINT('Ctrl Pts',(-6.662630109,4.29385805,3.444135414));
#138736=CARTESIAN_POINT('Ctrl Pts',(-6.63841029,4.302026826,3.490201831));
#138737=CARTESIAN_POINT('Ctrl Pts',(-6.657574201,4.172114527,2.870401672));
#138738=CARTESIAN_POINT('Ctrl Pts',(-6.51983632400001,4.22940039,3.189869203));
#138739=CARTESIAN_POINT('Ctrl Pts',(-6.352142073,4.285714286,3.494680397));
#138740=CARTESIAN_POINT('Ctrl Pts',(-6.327891176,4.29385805,3.538760292));
#138741=CARTESIAN_POINT('Ctrl Pts',(-6.30303087,4.302026826,3.582499385));
#138742=CARTESIAN_POINT('',(-6.63841029328694,4.30202682641445,3.49020182563221));
#138743=CARTESIAN_POINT('',(-6.46904368484552,4.30202682665757,3.53681209221154));
#138744=CARTESIAN_POINT('',(-6.88468943140282,4.2121649939256,2.97507166832603));
#138745=CARTESIAN_POINT('Ctrl Pts',(-6.63841029324683,4.30202682552111,
3.49020182489699));
#138746=CARTESIAN_POINT('Ctrl Pts',(-6.65456868331828,4.29657697961046,
3.45946835206243));
#138747=CARTESIAN_POINT('Ctrl Pts',(-6.67050177997155,4.29113922035365,
3.42864521292141));
#138748=CARTESIAN_POINT('Ctrl Pts',(-6.68620828108225,4.28571428571329,
3.39773730914955));
#138749=CARTESIAN_POINT('Ctrl Pts',(-6.75650993520172,4.26143250099124,
3.25939480083334));
#138750=CARTESIAN_POINT('Ctrl Pts',(-6.82276032055342,4.23689343090483,
3.11838340739359));
#138751=CARTESIAN_POINT('Ctrl Pts',(-6.88468942882511,4.21216499285689,
2.97507167453552));
#138752=CARTESIAN_POINT('Ctrl Pts',(-6.65568528196482,4.17289950695789,
2.87477885399687));
#138753=CARTESIAN_POINT('Ctrl Pts',(-6.69381093092921,4.17977820193302,
2.89143477508571));
#138754=CARTESIAN_POINT('Ctrl Pts',(-6.73197857598899,4.18648410048819,
2.90813092634623));
#138755=CARTESIAN_POINT('Ctrl Pts',(-6.80829996668031,4.19956141150126,
2.941557168664));
#138756=CARTESIAN_POINT('Ctrl Pts',(-6.84649859056851,4.20594050668918,
2.95830691729174));
#138757=CARTESIAN_POINT('Ctrl Pts',(-6.88468943413949,4.21216499506285,
2.97507166166953));
#138758=CARTESIAN_POINT('Ctrl Pts',(-7.09068370918432,4.30331728230629,
2.44382284214771));
#138759=CARTESIAN_POINT('Ctrl Pts',(-7.08936052059216,4.30267205415314,
2.44764862557385));
#138760=CARTESIAN_POINT('Ctrl Pts',(-7.088037332,4.302026826,2.451474409));
#138761=CARTESIAN_POINT('Ctrl Pts',(-6.955296464,4.237298226,2.835272921));
#138762=CARTESIAN_POINT('Ctrl Pts',(-6.781889847,4.172121859,3.202494356));
#138763=CARTESIAN_POINT('Ctrl Pts',(-6.92811519775424,4.30331728230629,
2.13630078798455));
#138764=CARTESIAN_POINT('Ctrl Pts',(-6.92695808937712,4.30267205415314,
2.14003900399228));
#138765=CARTESIAN_POINT('Ctrl Pts',(-6.925800981,4.302026826,2.14377722));
#138766=CARTESIAN_POINT('Ctrl Pts',(-6.809721103,4.237298226,2.518791062));
#138767=CARTESIAN_POINT('Ctrl Pts',(-6.653826618,4.172121859,2.87907821));
#138768=CARTESIAN_POINT('',(-7.08803733451121,4.30202682545315,2.45147440767622));
#138769=CARTESIAN_POINT('Origin',(0.172137087639891,4.1607288156607,-0.0833912659878833));
#138770=CARTESIAN_POINT('',(-7.00691915965291,4.30202682438465,2.29762580488479));
#138771=CARTESIAN_POINT('Origin',(1.08333481074752E-12,4.39277644300067,
-5.55545193181572E-13));
#138772=CARTESIAN_POINT('',(-6.88252390416385,4.39169923737767,2.98007796857426));
#138773=CARTESIAN_POINT('Origin',(0.153133619751964,4.16082474247324,-0.105983085249925));
#138774=CARTESIAN_POINT('Origin',(0.1575399643161,4.55341983999308,-0.0962896094476801));
#138775=CARTESIAN_POINT('Ctrl Pts',(-7.407046451,4.172114527,1.177141824));
#138776=CARTESIAN_POINT('Ctrl Pts',(-7.35056062300001,4.22940039,1.532573212));
#138777=CARTESIAN_POINT('Ctrl Pts',(-7.260301532,4.285714286,1.880962961));
#138778=CARTESIAN_POINT('Ctrl Pts',(-7.247248825,4.29385805,1.931344914));
#138779=CARTESIAN_POINT('Ctrl Pts',(-7.233498171,4.302026826,1.981540869));
#138780=CARTESIAN_POINT('Ctrl Pts',(-7.118975327,4.172114527,1.372111619));
#138781=CARTESIAN_POINT('Ctrl Pts',(-7.053133761,4.22940039,1.713719749));
#138782=CARTESIAN_POINT('Ctrl Pts',(-6.954885505,4.285714286,2.047453934));
#138783=CARTESIAN_POINT('Ctrl Pts',(-6.940677455,4.29385805,2.095716491));
#138784=CARTESIAN_POINT('Ctrl Pts',(-6.925800981,4.302026826,2.14377722));
#138785=CARTESIAN_POINT('',(-7.23349817293618,4.30202682620654,1.98154086307485));
#138786=CARTESIAN_POINT('',(-7.07964957713462,4.30202682665757,2.06265904060565));
#138787=CARTESIAN_POINT('',(-7.36328168429495,4.21216499534027,1.4255114278799));
#138788=CARTESIAN_POINT('Ctrl Pts',(-7.23349817258395,4.3020268248974,1.98154086236812));
#138789=CARTESIAN_POINT('Ctrl Pts',(-7.24267199974551,4.29657697940857,
1.94805234476445));
#138790=CARTESIAN_POINT('Ctrl Pts',(-7.25160652540155,4.29113922035358,
1.91452468863712));
#138791=CARTESIAN_POINT('Ctrl Pts',(-7.26030153158397,4.28571428595545,
1.88096296099009));
#138792=CARTESIAN_POINT('Ctrl Pts',(-7.29922002221488,4.2614325007481,1.73074204502813));
#138793=CARTESIAN_POINT('Ctrl Pts',(-7.33360822920324,4.23689343229803,
1.57878554621227));
#138794=CARTESIAN_POINT('Ctrl Pts',(-7.36328168273712,4.21216499704637,
1.42551143409564));
#138795=CARTESIAN_POINT('Ctrl Pts',(-7.11807153505751,4.1728995071105,1.37679252714695));
#138796=CARTESIAN_POINT('Ctrl Pts',(-7.15888635834678,4.17977820204914,
1.38486315444477));
#138797=CARTESIAN_POINT('Ctrl Pts',(-7.19975084304136,4.18648410041248,
1.39296404330249));
#138798=CARTESIAN_POINT('Ctrl Pts',(-7.28147353617586,4.19956141143594,
1.40920195580249));
#138799=CARTESIAN_POINT('Ctrl Pts',(-7.32237979828495,4.2059405066357,1.4173485297049));
#138800=CARTESIAN_POINT('Ctrl Pts',(-7.36328168565133,4.2121649950354,1.42551142131593));
#138801=CARTESIAN_POINT('Ctrl Pts',(-7.45025713667788,4.30331728230629,
0.862400223638416));
#138802=CARTESIAN_POINT('Ctrl Pts',(-7.44978731383894,4.30267205415314,
0.866421008819208));
#138803=CARTESIAN_POINT('Ctrl Pts',(-7.449317491,4.302026826,0.870441794));
#138804=CARTESIAN_POINT('Ctrl Pts',(-7.40218536500001,4.237298226,1.273802674));
#138805=CARTESIAN_POINT('Ctrl Pts',(-7.311774653,4.172121859,1.669715971));
#138806=CARTESIAN_POINT('Ctrl Pts',(-7.22538123576582,4.30331728230629,
0.597015288620854));
#138807=CARTESIAN_POINT('Ctrl Pts',(-7.22505478588291,4.30267205415314,
0.600914851310427));
#138808=CARTESIAN_POINT('Ctrl Pts',(-7.224728336,4.302026826,0.604814414));
#138809=CARTESIAN_POINT('Ctrl Pts',(-7.191979232,4.237298226,0.996014383));
#138810=CARTESIAN_POINT('Ctrl Pts',(-7.117180559,4.172121859,1.381390924));
#138811=CARTESIAN_POINT('',(-7.4493174931666,4.30202682545335,0.870441792165976));
#138812=CARTESIAN_POINT('Origin',(0.186039531007829,4.16072872556647,-0.0444372955112665));
#138813=CARTESIAN_POINT('',(-7.33702291451184,4.30202682438524,0.737628093935509));
#138814=CARTESIAN_POINT('Origin',(-1.12583553590895E-12,4.39277644300022,
2.0046898169257E-13));
#138815=CARTESIAN_POINT('',(-7.36224299305595,4.39169923741706,1.43086620813188));
#138816=CARTESIAN_POINT('Origin',(0.17233670797613,4.16082467495845,-0.0705860755585144));
#138817=CARTESIAN_POINT('Origin',(0.174556151942689,4.55341981959481,-0.0601719639733485));
#138818=CARTESIAN_POINT('Ctrl Pts',(-7.486924517,4.172114527,-0.442675134));
#138819=CARTESIAN_POINT('Ctrl Pts',(-7.50816653800001,4.22940039,-0.0834107510000001));
#138820=CARTESIAN_POINT('Ctrl Pts',(-7.494911153,4.285714286,0.276236876));
#138821=CARTESIAN_POINT('Ctrl Pts',(-7.492994242,4.29385805,0.328246873));
#138822=CARTESIAN_POINT('Ctrl Pts',(-7.490355716,4.302026826,0.380225258));
#138823=CARTESIAN_POINT('Ctrl Pts',(-7.247501079,4.172114527,-0.190336848));
#138824=CARTESIAN_POINT('Ctrl Pts',(-7.256634502,4.22940039,0.157438664));
#138825=CARTESIAN_POINT('Ctrl Pts',(-7.23242622,4.285714286,0.5044908));
#138826=CARTESIAN_POINT('Ctrl Pts',(-7.22892537,4.29385805,0.554679316));
#138827=CARTESIAN_POINT('Ctrl Pts',(-7.224728336,4.302026826,0.604814414));
#138828=CARTESIAN_POINT('',(-7.49035571664362,4.30202682620655,0.380225251774799));
#138829=CARTESIAN_POINT('',(-7.35754202627092,4.30202682665757,0.492519831952797));
#138830=CARTESIAN_POINT('',(-7.49757506976613,4.21216499536516,-0.190704142493896));
#138831=CARTESIAN_POINT('Ctrl Pts',(-7.49035571612153,4.3020268248974,0.380225251182439));
#138832=CARTESIAN_POINT('Ctrl Pts',(-7.4921160237264,4.29657697940857,0.345547575253956));
#138833=CARTESIAN_POINT('Ctrl Pts',(-7.49363421042152,4.29113922035358,
0.310883118420912));
#138834=CARTESIAN_POINT('Ctrl Pts',(-7.49491115271027,4.28571428596,0.276236876004686));
#138835=CARTESIAN_POINT('Ctrl Pts',(-7.50062669436462,4.26143250076421,
0.121161716035054));
#138836=CARTESIAN_POINT('Ctrl Pts',(-7.50154476801792,4.23689343230145,
-0.0346345719932585));
#138837=CARTESIAN_POINT('Ctrl Pts',(-7.49757506958192,4.21216499708899,
-0.190704136023857));
#138838=CARTESIAN_POINT('Ctrl Pts',(-7.24762467296213,4.17289950691553,
-0.185571088361909));
#138839=CARTESIAN_POINT('Ctrl Pts',(-7.28922021464216,4.17977820189018,
-0.186463128323594));
#138840=CARTESIAN_POINT('Ctrl Pts',(-7.33087076318371,4.18648410045675,
-0.187336290073957));
#138841=CARTESIAN_POINT('Ctrl Pts',(-7.41417349632566,4.19956141148362,
-0.189045974414105));
#138842=CARTESIAN_POINT('Ctrl Pts',(-7.45587466532089,4.20594050667357,
-0.189883500166995));
#138843=CARTESIAN_POINT('Ctrl Pts',(-7.49757506967887,4.21216499505722,
-0.190704149263988));
#138844=CARTESIAN_POINT('Ctrl Pts',(-7.46146482034059,4.30331728230629,
-0.759347270947339));
#138845=CARTESIAN_POINT('Ctrl Pts',(-7.46187033167029,4.30267205415314,
-0.75531949147367));
#138846=CARTESIAN_POINT('Ctrl Pts',(-7.462275843,4.302026826,-0.751291712));
#138847=CARTESIAN_POINT('Ctrl Pts',(-7.502956307,4.237298226,-0.347229172));
#138848=CARTESIAN_POINT('Ctrl Pts',(-7.499769002,4.172121859,0.058863524));
#138849=CARTESIAN_POINT('Ctrl Pts',(-7.18479647692406,4.30331728230629,
-0.970185982323433));
#138850=CARTESIAN_POINT('Ctrl Pts',(-7.18531594996203,4.30267205415314,
-0.966307412161716));
#138851=CARTESIAN_POINT('Ctrl Pts',(-7.185835423,4.302026826,-0.962428841999999));
#138852=CARTESIAN_POINT('Ctrl Pts',(-7.23794840400001,4.237298226,-0.573334821));
#138853=CARTESIAN_POINT('Ctrl Pts',(-7.247743048,4.172121859,-0.180888666));
#138854=CARTESIAN_POINT('',(-7.46227584451965,4.30202682545371,-0.751291714841994));
#138855=CARTESIAN_POINT('Origin',(0.19124235071154,4.16072878392355,-0.00340538346760563));
#138856=CARTESIAN_POINT('',(-7.32405563182418,4.30202682438465,-0.856860287050402));
#138857=CARTESIAN_POINT('Origin',(-9.41954847455406E-13,4.39277644300022,
-5.42372136785874E-14));
#138858=CARTESIAN_POINT('',(-7.49771178195657,4.39169923736653,-0.185251266036152));
#138859=CARTESIAN_POINT('Origin',(0.183481501523408,4.16082467772807,-0.0318885222126206));
#138860=CARTESIAN_POINT('Origin',(0.183410145336235,4.5534198137753,-0.0212407675007344));
#138861=CARTESIAN_POINT('Ctrl Pts',(-7.216722314,4.172114527,-2.041793095));
#138862=CARTESIAN_POINT('Ctrl Pts',(-7.314698931,4.22940039,-1.69549452));
#138863=CARTESIAN_POINT('Ctrl Pts',(-7.379067058,4.285714286,-1.341405739));
#138864=CARTESIAN_POINT('Ctrl Pts',(-7.388375575,4.29385805,-1.290199627));
#138865=CARTESIAN_POINT('Ctrl Pts',(-7.39697255300001,4.302026826,-1.238869262));
#138866=CARTESIAN_POINT('Ctrl Pts',(-7.037141735,4.172114527,-1.743885375));
#138867=CARTESIAN_POINT('Ctrl Pts',(-7.120823079,4.22940039,-1.406204078));
#138868=CARTESIAN_POINT('Ctrl Pts',(-7.171786724,4.285714286,-1.062061763));
#138869=CARTESIAN_POINT('Ctrl Pts',(-7.179156768,4.29385805,-1.012294047));
#138870=CARTESIAN_POINT('Ctrl Pts',(-7.185835423,4.302026826,-0.962428842));
#138871=CARTESIAN_POINT('',(-7.39697255240167,4.30202682641445,-1.2388692682728));
#138872=CARTESIAN_POINT('',(-7.29140398739456,4.30202682665757,-1.10064905601082));
#138873=CARTESIAN_POINT('',(-7.2812901778864,4.21216499391656,-1.79800259874241));
#138874=CARTESIAN_POINT('Ctrl Pts',(-7.39697255197888,4.30202682552111,
-1.23886926883788));
#138875=CARTESIAN_POINT('Ctrl Pts',(-7.39123702897011,4.29657697961046,
-1.27311461443996));
#138876=CARTESIAN_POINT('Ctrl Pts',(-7.38526788766412,4.29113922035365,
-1.30729500118857));
#138877=CARTESIAN_POINT('Ctrl Pts',(-7.37906705786746,4.28571428571329,
-1.3414057385799));
#138878=CARTESIAN_POINT('Ctrl Pts',(-7.35131239827258,4.26143250098364,
-1.49408399872788));
#138879=CARTESIAN_POINT('Ctrl Pts',(-7.31871741129183,4.23689343089718,
-1.64643521610912));
#138880=CARTESIAN_POINT('Ctrl Pts',(-7.28129017951097,4.21216499285689,
-1.79800259225534));
#138881=CARTESIAN_POINT('Ctrl Pts',(-7.03828693800445,4.17289950705686,
-1.73925760595926));
#138882=CARTESIAN_POINT('Ctrl Pts',(-7.07871823679367,4.1797782020216,-1.74907060253793));
#138883=CARTESIAN_POINT('Ctrl Pts',(-7.11920731380291,4.18648410043831,
-1.75887698685823));
#138884=CARTESIAN_POINT('Ctrl Pts',(-7.20019494374002,4.19956141146568,
-1.77845432503505));
#138885=CARTESIAN_POINT('Ctrl Pts',(-7.24074111926083,4.20594050665211,
-1.78823678857437));
#138886=CARTESIAN_POINT('Ctrl Pts',(-7.2812901760473,4.21216499504079,-1.79800260566205));
#138887=CARTESIAN_POINT('Ctrl Pts',(-7.12378270255569,4.30331728230629,
-2.34558853055555));
#138888=CARTESIAN_POINT('Ctrl Pts',(-7.12504458677785,4.30267205415314,
-2.34174209127778));
#138889=CARTESIAN_POINT('Ctrl Pts',(-7.126306471,4.302026826,-2.337895652));
#138890=CARTESIAN_POINT('Ctrl Pts',(-7.25289735,4.237298226,-1.952024967));
#138891=CARTESIAN_POINT('Ctrl Pts',(-7.337082488,4.172121859,-1.554741317));
#138892=CARTESIAN_POINT('Ctrl Pts',(-6.80825862002472,4.30331728230629,
-2.4920224339872));
#138893=CARTESIAN_POINT('Ctrl Pts',(-6.80959972601237,4.30267205415314,
-2.4883462139936));
#138894=CARTESIAN_POINT('Ctrl Pts',(-6.81094083199999,4.302026826,-2.484669994));
#138895=CARTESIAN_POINT('Ctrl Pts',(-6.945479154,4.237298226,-2.115875526));
#138896=CARTESIAN_POINT('Ctrl Pts',(-7.039409127,4.172121859,-1.734710103));
#138897=CARTESIAN_POINT('',(-7.12630647186188,4.30202682545374,-2.33789565511669));
#138898=CARTESIAN_POINT('Origin',(0.187503352522165,4.16072876702414,0.0377857023399969));
#138899=CARTESIAN_POINT('',(-6.96862364819113,4.30202682438465,-2.41128283256266));
#138900=CARTESIAN_POINT('Origin',(-7.1730815731641E-13,4.39277644300044,
-1.89843800402212E-13));
#138901=CARTESIAN_POINT('',(-7.28259590084164,4.39169923740603,-1.79270659643726));
#138902=CARTESIAN_POINT('Origin',(0.186046560586159,4.16082471231166,0.00830004912923704));
#138903=CARTESIAN_POINT('Origin',(0.18368817995575,4.55341980852378,0.0186835631696336));
#138904=CARTESIAN_POINT('Ctrl Pts',(-6.609074196,4.172114527,-3.54543908));
#138905=CARTESIAN_POINT('Ctrl Pts',(-6.779204132,4.22940039,-3.22829885));
#138906=CARTESIAN_POINT('Ctrl Pts',(-6.918185988,4.285714286,-2.896325712));
#138907=CARTESIAN_POINT('Ctrl Pts',(-6.938284678,4.29385805,-2.848317827));
#138908=CARTESIAN_POINT('Ctrl Pts',(-6.957715175,4.302026826,-2.800035633));
#138909=CARTESIAN_POINT('Ctrl Pts',(-6.497733465,4.172114527,-3.215891761));
#138910=CARTESIAN_POINT('Ctrl Pts',(-6.652049883,4.22940039,-2.90409428));
#138911=CARTESIAN_POINT('Ctrl Pts',(-6.775802451,4.285714286,-2.578953498));
#138912=CARTESIAN_POINT('Ctrl Pts',(-6.793698776,4.29385805,-2.531933665));
#138913=CARTESIAN_POINT('Ctrl Pts',(-6.81094083200001,4.302026826,-2.484669994));
#138914=CARTESIAN_POINT('',(-6.95771517296804,4.30202682641445,-2.80003563894042));
#138915=CARTESIAN_POINT('',(-6.88432800204651,4.30202682665757,-2.6423528172869));
#138916=CARTESIAN_POINT('',(-6.72454024984592,4.21216499393534,-3.32122845186731));
#138917=CARTESIAN_POINT('Ctrl Pts',(-6.95771517226492,4.30202682552111,
-2.80003563935076));
#138918=CARTESIAN_POINT('Ctrl Pts',(-6.94475200541274,4.29657697961046,
-2.83224738030877));
#138919=CARTESIAN_POINT('Ctrl Pts',(-6.93157464648108,4.29113922035365,
-2.86434545977854));
#138920=CARTESIAN_POINT('Ctrl Pts',(-6.91818598841666,4.28571428571329,
-2.89632571194525));
#138921=CARTESIAN_POINT('Ctrl Pts',(-6.85825890466453,4.26143250101328,
-3.0394680075202));
#138922=CARTESIAN_POINT('Ctrl Pts',(-6.79367496218216,4.23689343092699,
-3.18125037923024));
#138923=CARTESIAN_POINT('Ctrl Pts',(-6.72454025279714,4.21216499285671,
-3.32122844569756));
#138924=CARTESIAN_POINT('Ctrl Pts',(-6.49984672779771,4.1728995071943,-3.21161837090972));
#138925=CARTESIAN_POINT('Ctrl Pts',(-6.53722326117339,4.17977820215861,
-3.22989347930327));
#138926=CARTESIAN_POINT('Ctrl Pts',(-6.57465764293399,4.18648410049424,
-3.24817455038812));
#138927=CARTESIAN_POINT('Ctrl Pts',(-6.64954327818949,4.19956141151884,
-3.28470412787107));
#138928=CARTESIAN_POINT('Ctrl Pts',(-6.68703856609739,4.20594050668611,
-3.30297411204387));
#138929=CARTESIAN_POINT('Ctrl Pts',(-6.72454024648908,4.21216499507469,
-3.3212284583751));
#138930=CARTESIAN_POINT('Ctrl Pts',(-6.45300042338213,4.30331728230629,
-3.82215267771983));
#138931=CARTESIAN_POINT('Ctrl Pts',(-6.45505967619106,4.30267205415314,
-3.81866743385991));
#138932=CARTESIAN_POINT('Ctrl Pts',(-6.457118929,4.302026826,-3.81518219));
#138933=CARTESIAN_POINT('Ctrl Pts',(-6.663700974,4.237298226,-3.465546244));
#138934=CARTESIAN_POINT('Ctrl Pts',(-6.83132215200001,4.172121859,-3.095648181));
#138935=CARTESIAN_POINT('Ctrl Pts',(-6.11337415738809,4.30331728230629,
-3.89733468775749));
#138936=CARTESIAN_POINT('Ctrl Pts',(-6.11547418769404,4.30267205415314,
-3.89403271387874));
#138937=CARTESIAN_POINT('Ctrl Pts',(-6.117574218,4.302026826,-3.89073074));
#138938=CARTESIAN_POINT('Ctrl Pts',(-6.328247018,4.237298226,-3.559480243));
#138939=CARTESIAN_POINT('Ctrl Pts',(-6.501920259,4.172121859,-3.207418423));
#138940=CARTESIAN_POINT('',(-6.45711892914839,4.30202682545394,-3.81518219324713));
#138941=CARTESIAN_POINT('Origin',(0.174996990872773,4.16072877815487,0.0772100619350202));
#138942=CARTESIAN_POINT('',(-6.28734656821467,4.30202682438522,-3.85295647362473));
#138943=CARTESIAN_POINT('Origin',(-5.98479599211998E-14,4.39277644300111,
9.97465998686664E-15));
#138944=CARTESIAN_POINT('',(-6.72695392951752,4.3916992373877,-3.31633695910688));
#138945=CARTESIAN_POINT('Origin',(0.179912927710379,4.16082471999665,0.0481006479497342));
#138946=CARTESIAN_POINT('Origin',(0.175377460269127,4.55341978905206,0.0577343964042454));
#138947=CARTESIAN_POINT('Ctrl Pts',(-5.692393115,4.172114527,-4.883304274));
#138948=CARTESIAN_POINT('Ctrl Pts',(-5.926721282,4.22940039,-4.610151513));
#138949=CARTESIAN_POINT('Ctrl Pts',(-6.133818231,4.285714286,-4.315816714));
#138950=CARTESIAN_POINT('Ctrl Pts',(-6.163767301,4.29385805,-4.27325185));
#138951=CARTESIAN_POINT('Ctrl Pts',(-6.193122768,4.302026826,-4.23027545));
#138952=CARTESIAN_POINT('Ctrl Pts',(-5.6544984,4.172114527,-4.537526622));
#138953=CARTESIAN_POINT('Ctrl Pts',(-5.87223422700001,4.22940039,-4.266192261));
#138954=CARTESIAN_POINT('Ctrl Pts',(-6.062989186,4.285714286,-3.975256234));
#138955=CARTESIAN_POINT('Ctrl Pts',(-6.090574979,4.29385805,-3.93318288));
#138956=CARTESIAN_POINT('Ctrl Pts',(-6.117574218,4.302026826,-3.89073074));
#138957=CARTESIAN_POINT('',(-6.19312276474054,4.30202682641444,-4.2302754553667));
#138958=CARTESIAN_POINT('',(-6.15534849076645,4.30202682665756,-4.06050309838586));
#138959=CARTESIAN_POINT('',(-5.85335829350893,4.21216499391699,-4.6891573537254));
#138960=CARTESIAN_POINT('Ctrl Pts',(-6.1931227639692,4.30202682552109,-4.23027545561829));
#138961=CARTESIAN_POINT('Ctrl Pts',(-6.17353809687833,4.29657697961046,
-4.25894740591034));
#138962=CARTESIAN_POINT('Ctrl Pts',(-6.15376867898852,4.29113922035365,
-4.28746230749566));
#138963=CARTESIAN_POINT('Ctrl Pts',(-6.13381823140102,4.28571428571329,
-4.3158167134544));
#138964=CARTESIAN_POINT('Ctrl Pts',(-6.04452084714403,4.26143250100524,
-4.44272987032328));
#138965=CARTESIAN_POINT('Ctrl Pts',(-5.95096782255411,4.23689343091894,
-4.56731381033318));
#138966=CARTESIAN_POINT('Ctrl Pts',(-5.85335829768833,4.21216499285688,
-4.68915734848842));
#138967=CARTESIAN_POINT('Ctrl Pts',(-5.65748090767041,4.17289950703237,
-4.53380742990244));
#138968=CARTESIAN_POINT('Ctrl Pts',(-5.69005499041686,4.17977820200376,
-4.55969012622329));
#138969=CARTESIAN_POINT('Ctrl Pts',(-5.72268428790545,4.18648410046869,
-4.58559108199846));
#138970=CARTESIAN_POINT('Ctrl Pts',(-5.78796635935612,4.19956141148752,
-4.63736481611499));
#138971=CARTESIAN_POINT('Ctrl Pts',(-5.82065752182051,4.20594050665946,
-4.66326803672648));
#138972=CARTESIAN_POINT('Ctrl Pts',(-5.85335828892578,4.2121649950401,-4.68915735924435));
#138973=CARTESIAN_POINT('Ctrl Pts',(-5.4804830149175,4.30331728230629,-5.1199972136303));
#138974=CARTESIAN_POINT('Ctrl Pts',(-5.48324334795874,4.30267205415314,
-5.11703613131514));
#138975=CARTESIAN_POINT('Ctrl Pts',(-5.486003681,4.302026826,-5.114075049));
#138976=CARTESIAN_POINT('Ctrl Pts',(-5.762917347,4.237298226,-4.81702243));
#138977=CARTESIAN_POINT('Ctrl Pts',(-6.006136784,4.172121859,-4.491805977));
#138978=CARTESIAN_POINT('Ctrl Pts',(-5.13263511291799,4.30331728230629,
-5.12041190225208));
#138979=CARTESIAN_POINT('Ctrl Pts',(-5.135395872459,4.30267205415314,-5.11763857112605));
#138980=CARTESIAN_POINT('Ctrl Pts',(-5.138156632,4.302026826,-5.11486524));
#138981=CARTESIAN_POINT('Ctrl Pts',(-5.415113084,4.237298226,-4.83664762));
#138982=CARTESIAN_POINT('Ctrl Pts',(-5.660408826,4.172121859,-4.530151423));
#138983=CARTESIAN_POINT('',(-5.48600368048579,4.30202682545371,-5.11407505218425));
#138984=CARTESIAN_POINT('Origin',(0.154307684794188,4.16072873661738,0.113024035958856));
#138985=CARTESIAN_POINT('',(-5.31208014948166,4.30202682438463,-5.11447015178951));
#138986=CARTESIAN_POINT('Origin',(-3.62557206479153E-13,4.39277644300067,
-2.0643209364124E-13));
#138987=CARTESIAN_POINT('',(-5.85676706859328,4.39169923740595,-4.68489909144703));
#138988=CARTESIAN_POINT('Origin',(0.165366468826336,4.16082471323804,0.0856520620843465));
#138989=CARTESIAN_POINT('Origin',(0.158866106015709,4.55341982996691,0.0940856226204201));
#138990=CARTESIAN_POINT('Ctrl Pts',(-4.509542057,4.172114527,-5.992831587));
#138991=CARTESIAN_POINT('Ctrl Pts',(-4.79711153099999,4.22940039,-5.776438615));
#138992=CARTESIAN_POINT('Ctrl Pts',(-5.062639951,4.285714286,-5.533504923));
#138993=CARTESIAN_POINT('Ctrl Pts',(-5.101039015,4.29385805,-5.498373367));
#138994=CARTESIAN_POINT('Ctrl Pts',(-5.138946823,4.302026826,-5.462712289));
#138995=CARTESIAN_POINT('Ctrl Pts',(-4.546865274,4.172114527,-5.646991781));
#138996=CARTESIAN_POINT('Ctrl Pts',(-4.817839426,4.22940039,-5.428807833));
#138997=CARTESIAN_POINT('Ctrl Pts',(-5.066677286,4.285714286,-5.185680407));
#138998=CARTESIAN_POINT('Ctrl Pts',(-5.102662666,4.29385805,-5.150520834));
#138999=CARTESIAN_POINT('Ctrl Pts',(-5.138156632,4.302026826,-5.11486524));
#139000=CARTESIAN_POINT('',(-5.13894681866893,4.30202682641444,-5.4627122935483));
#139001=CARTESIAN_POINT('',(-5.1385517245908,4.30202682665756,-5.28878876732656));
#139002=CARTESIAN_POINT('',(-4.70847980829036,4.21216499392856,-5.83782647009015));
#139003=CARTESIAN_POINT('Ctrl Pts',(-5.13894681787326,4.30202682552109,
-5.46271229363858));
#139004=CARTESIAN_POINT('Ctrl Pts',(-5.11365640767574,4.29657697961046,
-5.48650378512141));
#139005=CARTESIAN_POINT('Ctrl Pts',(-5.08821932709154,4.29113922035365,
-5.51010218345383));
#139006=CARTESIAN_POINT('Ctrl Pts',(-5.06263995080817,4.28571428571329,
-5.53350492260383));
#139007=CARTESIAN_POINT('Ctrl Pts',(-4.94814771273062,4.26143250098491,
-5.63825462223473));
#139008=CARTESIAN_POINT('Ctrl Pts',(-4.83000004119946,4.23689343089845,
-5.73981472429379));
#139009=CARTESIAN_POINT('Ctrl Pts',(-4.70847981356072,4.21216499285688,
-5.83782646584249));
#139010=CARTESIAN_POINT('Ctrl Pts',(-4.55057756815832,4.17289950692595,
-5.64400069300954));
#139011=CARTESIAN_POINT('Ctrl Pts',(-4.57682607217492,4.1797782018608,-5.67628073086688));
#139012=CARTESIAN_POINT('Ctrl Pts',(-4.60312457549802,4.1864841004784,-5.70859047178126));
#139013=CARTESIAN_POINT('Ctrl Pts',(-4.65575056577685,4.1995614114796,-5.77318748021941));
#139014=CARTESIAN_POINT('Ctrl Pts',(-4.68210900029073,4.20594050666992,
-5.80551273159959));
#139015=CARTESIAN_POINT('Ctrl Pts',(-4.7084798025698,4.21216499506463,-5.83782647453979));
#139016=CARTESIAN_POINT('Ctrl Pts',(-4.2517043126979,4.30331728230629,-6.178436370691));
#139017=CARTESIAN_POINT('Ctrl Pts',(-4.25503665584895,4.30267205415314,
-6.1761379068455));
#139018=CARTESIAN_POINT('Ctrl Pts',(-4.258368999,4.302026826,-6.173839443));
#139019=CARTESIAN_POINT('Ctrl Pts',(-4.592666109,4.237298226,-5.943260002));
#139020=CARTESIAN_POINT('Ctrl Pts',(-4.900111135,4.172121859,-5.677931918));
#139021=CARTESIAN_POINT('Ctrl Pts',(-3.91189975656577,4.30331728230629,
-6.10406434697834));
#139022=CARTESIAN_POINT('Ctrl Pts',(-3.91519215528289,4.30267205415314,
-6.10194933648917));
#139023=CARTESIAN_POINT('Ctrl Pts',(-3.918484554,4.302026826,-6.099834326));
#139024=CARTESIAN_POINT('Ctrl Pts',(-4.248774481,4.237298226,-5.88765873000001));
#139025=CARTESIAN_POINT('Ctrl Pts',(-4.554222968,4.172121859,-5.64105957800001));
#139026=CARTESIAN_POINT('',(-4.25836899838928,4.30202682545315,-6.17383944577572));
#139027=CARTESIAN_POINT('Origin',(0.126403232601331,4.16072876476957,0.143553190585521));
#139028=CARTESIAN_POINT('',(-4.08842676807871,4.30202682438463,-6.13683689011035));
#139029=CARTESIAN_POINT('Origin',(-1.50053580671994E-13,4.39277644300067,
-3.65592972562112E-13));
#139030=CARTESIAN_POINT('',(-4.71272428942334,4.39169923736879,-5.83440054895474));
#139031=CARTESIAN_POINT('Origin',(0.143087622696539,4.16082468452531,0.11919844841964));
#139032=CARTESIAN_POINT('Origin',(0.134926334767914,4.55341983712944,0.126037539353255));
#139033=CARTESIAN_POINT('Ctrl Pts',(-3.115829826,4.172114527,-6.822140756));
#139034=CARTESIAN_POINT('Ctrl Pts',(-3.443194178,4.22940039,-6.672625868));
#139035=CARTESIAN_POINT('Ctrl Pts',(-3.754738253,4.285714286,-6.492452591));
#139036=CARTESIAN_POINT('Ctrl Pts',(-3.799791815,4.29385805,-6.466397055));
#139037=CARTESIAN_POINT('Ctrl Pts',(-3.844479437,4.302026826,-6.439718772));
#139038=CARTESIAN_POINT('Ctrl Pts',(-3.226625782,4.172114527,-6.492409881));
#139039=CARTESIAN_POINT('Ctrl Pts',(-3.538167808,4.22940039,-6.337578385));
#139040=CARTESIAN_POINT('Ctrl Pts',(-3.833453187,4.285714286,-6.153627927));
#139041=CARTESIAN_POINT('Ctrl Pts',(-3.876155517,4.29385805,-6.127026159));
#139042=CARTESIAN_POINT('Ctrl Pts',(-3.918484554,4.302026826,-6.099834326));
#139043=CARTESIAN_POINT('',(-3.84447943177234,4.30202682641444,-6.4397187754636));
#139044=CARTESIAN_POINT('',(-3.88148199205119,4.30202682665756,-6.26977655113509));
#139045=CARTESIAN_POINT('',(-3.34343804111563,4.21216499391003,-6.71352530840784));
#139046=CARTESIAN_POINT('Ctrl Pts',(-3.84447943092908,4.30202682552109,
-6.43971877531644));
#139047=CARTESIAN_POINT('Ctrl Pts',(-3.81466582933418,4.29657697961046,
-6.45751734418141));
#139048=CARTESIAN_POINT('Ctrl Pts',(-3.78475049544117,4.29113922035365,
-6.47509580469299));
#139049=CARTESIAN_POINT('Ctrl Pts',(-3.7547382535708,4.28571428571329,-6.49245259106079));
#139050=CARTESIAN_POINT('Ctrl Pts',(-3.62040469104493,4.26143250097169,
-6.57014085429876));
#139051=CARTESIAN_POINT('Ctrl Pts',(-3.48318682656126,4.23689343088507,
-6.64392828065515));
#139052=CARTESIAN_POINT('Ctrl Pts',(-3.34343804705431,4.2121649928567,-6.71352530534514));
#139053=CARTESIAN_POINT('Ctrl Pts',(-3.23089428070165,4.17289950706335,
-6.49028675709695));
#139054=CARTESIAN_POINT('Ctrl Pts',(-3.24958985533249,4.17977820200827,
-6.52745475823694));
#139055=CARTESIAN_POINT('Ctrl Pts',(-3.26832787454873,4.18648410044612,
-6.56466251525528));
#139056=CARTESIAN_POINT('Ctrl Pts',(-3.3058370511616,4.19956141145617,-6.63906231389585));
#139057=CARTESIAN_POINT('Ctrl Pts',(-3.32463026659627,4.20594050662904,
-6.67629810299704));
#139058=CARTESIAN_POINT('Ctrl Pts',(-3.34343803465716,4.21216499502219,
-6.71352531148481));
#139059=CARTESIAN_POINT('Ctrl Pts',(-2.82412064279616,4.30331728230629,
-6.94797870952977));
#139060=CARTESIAN_POINT('Ctrl Pts',(-2.82786917939808,4.30267205415314,
-6.94645033776488));
#139061=CARTESIAN_POINT('Ctrl Pts',(-2.831617716,4.302026826,-6.94492196600001));
#139062=CARTESIAN_POINT('Ctrl Pts',(-3.207666909,4.237298226,-6.791597341));
#139063=CARTESIAN_POINT('Ctrl Pts',(-3.564961736,4.172121859,-6.598564073));
#139064=CARTESIAN_POINT('Ctrl Pts',(-2.5082483139853,4.30331728230629,-6.80229752762605));
#139065=CARTESIAN_POINT('Ctrl Pts',(-2.51191840299265,4.30267205415314,
-6.80093973331303));
#139066=CARTESIAN_POINT('Ctrl Pts',(-2.515588492,4.302026826,-6.799581939));
#139067=CARTESIAN_POINT('Ctrl Pts',(-2.883767906,4.237298226,-6.663369462));
#139068=CARTESIAN_POINT('Ctrl Pts',(-3.235086705,4.172121859,-6.488198056));
#139069=CARTESIAN_POINT('',(-2.83161771479313,4.30202682545336,-6.9449219685791));
#139070=CARTESIAN_POINT('Origin',(0.0925883270804578,4.1607287623299,0.167370006069153));
#139071=CARTESIAN_POINT('',(-2.67360309457301,4.30202682438522,-6.87225195616751));
#139072=CARTESIAN_POINT('Origin',(2.81892564846231E-13,4.39277644300022,
5.06539254985228E-13));
#139073=CARTESIAN_POINT('',(-3.3483197599588,4.39169923740935,-6.71109192160016));
#139074=CARTESIAN_POINT('Origin',(0.114118211480692,4.16082470782816,0.147171347731774));
#139075=CARTESIAN_POINT('Origin',(0.104677531084114,4.5534198439215,0.152096115214863));
#139076=CARTESIAN_POINT('Ctrl Pts',(-1.576424854,4.172114527,-7.332454206));
#139077=CARTESIAN_POINT('Ctrl Pts',(-1.928276891,4.22940039,-7.256808551));
#139078=CARTESIAN_POINT('Ctrl Pts',(-2.271269168,4.285714286,-7.147820393));
#139079=CARTESIAN_POINT('Ctrl Pts',(-2.320870572,4.29385805,-7.132059205));
#139080=CARTESIAN_POINT('Ctrl Pts',(-2.370248465,4.302026826,-7.115611162));
#139081=CARTESIAN_POINT('Ctrl Pts',(-1.755512854,4.172114527,-7.034250111));
#139082=CARTESIAN_POINT('Ctrl Pts',(-2.093055395,4.22940039,-6.950010816));
#139083=CARTESIAN_POINT('Ctrl Pts',(-2.420981077,4.285714286,-6.833838645));
#139084=CARTESIAN_POINT('Ctrl Pts',(-2.468403645,4.29385805,-6.81703855));
#139085=CARTESIAN_POINT('Ctrl Pts',(-2.515588492,4.302026826,-6.799581939));
#139086=CARTESIAN_POINT('',(-2.37024845919458,4.30202682641444,-7.11561116450187));
#139087=CARTESIAN_POINT('',(-2.44291847467284,4.30202682665756,-6.95759655184378));
#139088=CARTESIAN_POINT('',(-1.82206082675909,4.21216499392044,-7.27530716467459));
#139089=CARTESIAN_POINT('Ctrl Pts',(-2.37024845855516,4.30202682552109,
-7.11561116452528));
#139090=CARTESIAN_POINT('Ctrl Pts',(-2.33730571565344,4.29657697961046,
-7.12658456986995));
#139091=CARTESIAN_POINT('Ctrl Pts',(-2.30431093621402,4.29113922035365,
-7.1373211432536));
#139092=CARTESIAN_POINT('Ctrl Pts',(-2.27126916793844,4.28571428571329,
-7.14782039273317));
#139093=CARTESIAN_POINT('Ctrl Pts',(-2.12337556972221,4.26143250099285,
-7.19481460233943));
#139094=CARTESIAN_POINT('Ctrl Pts',(-1.97350366708589,4.23689343090646,
-7.2373791349662));
#139095=CARTESIAN_POINT('Ctrl Pts',(-1.82206083326747,4.21216499285688,
-7.27530716326621));
#139096=CARTESIAN_POINT('Ctrl Pts',(-1.76013796653428,4.172899507013,-7.03309422503798));
#139097=CARTESIAN_POINT('Ctrl Pts',(-1.77040642745592,4.1797782019747,-7.07341225479918));
#139098=CARTESIAN_POINT('Ctrl Pts',(-1.78070779428442,4.18648410042518,
-7.11377823530059));
#139099=CARTESIAN_POINT('Ctrl Pts',(-1.80134626972003,4.1995614114513,-7.19450197207154));
#139100=CARTESIAN_POINT('Ctrl Pts',(-1.81169551631347,4.20594050666897,
-7.23490719511896));
#139101=CARTESIAN_POINT('Ctrl Pts',(-1.82206081981772,4.21216499505768,
-7.2753071662803));
#139102=CARTESIAN_POINT('Ctrl Pts',(-1.26448422969873,4.30331728230629,
-7.39264128645948));
#139103=CARTESIAN_POINT('Ctrl Pts',(-1.26847368234936,4.30267205415314,
-7.39195447172974));
#139104=CARTESIAN_POINT('Ctrl Pts',(-1.272463135,4.302026826,-7.391267657));
#139105=CARTESIAN_POINT('Ctrl Pts',(-1.672680769,4.237298226,-7.322367136));
#139106=CARTESIAN_POINT('Ctrl Pts',(-2.063118688,4.172121859,-7.210654705));
#139107=CARTESIAN_POINT('Ctrl Pts',(-0.987313967966847,4.30331728230629,
-7.18246283536846));
#139108=CARTESIAN_POINT('Ctrl Pts',(-0.991190137983424,4.30267205415314,
-7.18192574618423));
#139109=CARTESIAN_POINT('Ctrl Pts',(-0.995066308,4.302026826,-7.181388657));
#139110=CARTESIAN_POINT('Ctrl Pts',(-1.383919549,4.237298226,-7.127508443));
#139111=CARTESIAN_POINT('Ctrl Pts',(-1.764681383,4.172121859,-7.031955604));
#139112=CARTESIAN_POINT('',(-1.27246313325074,4.30202682545318,-7.39126765925747));
#139113=CARTESIAN_POINT('Origin',(0.0544441196529202,4.16072874802149,0.18336095777007));
#139114=CARTESIAN_POINT('',(-1.13376471150132,4.30202682438463,-7.28632815855581));
#139115=CARTESIAN_POINT('Origin',(-1.57209315010398E-13,4.39277644300022,
-4.39318720291126E-13));
#139116=CARTESIAN_POINT('',(-1.82735151989587,4.39169923740219,-7.27398009464001));
#139117=CARTESIAN_POINT('Origin',(0.079812667389377,4.16082472253925,0.168262469875141));
#139118=CARTESIAN_POINT('Origin',(0.0695339680088305,4.55341979676417,0.171042352095149));
#139119=CARTESIAN_POINT('Ctrl Pts',(0.036691991,4.172114527,-7.499910246));
#139120=CARTESIAN_POINT('Ctrl Pts',(-0.32319552,4.22940039,-7.501670932));
#139121=CARTESIAN_POINT('Ctrl Pts',(-0.68159806,4.285714286,-7.468964057));
#139122=CARTESIAN_POINT('Ctrl Pts',(-0.733428001,4.29385805,-7.464234193));
#139123=CARTESIAN_POINT('Ctrl Pts',(-0.785187309,4.302026826,-7.458785484));
#139124=CARTESIAN_POINT('Ctrl Pts',(-0.202314096,4.172114527,-7.247176623));
#139125=CARTESIAN_POINT('Ctrl Pts',(-0.550074039,4.22940039,-7.237468465));
#139126=CARTESIAN_POINT('Ctrl Pts',(-0.895306583,4.285714286,-7.194506663));
#139127=CARTESIAN_POINT('Ctrl Pts',(-0.945231961,4.29385805,-7.188293795));
#139128=CARTESIAN_POINT('Ctrl Pts',(-0.995066308,4.302026826,-7.181388657));
#139129=CARTESIAN_POINT('',(-0.891176199469209,4.30202682665757,-7.31870008685521));
#139130=CARTESIAN_POINT('Ctrl Pts',(-0.207079557734034,4.17289950701476,
-7.24704202304173));
#139131=CARTESIAN_POINT('Ctrl Pts',(-0.208440763114175,4.17977820195709,
-7.28862485543279));
#139132=CARTESIAN_POINT('Ctrl Pts',(-0.209823797074378,4.18648410047151,
-7.33026159173366));
#139133=CARTESIAN_POINT('Ctrl Pts',(-0.212626539052888,4.19956141147973,
-7.41353471477598));
#139134=CARTESIAN_POINT('Ctrl Pts',(-0.214047897339691,4.20594050669437,
-7.45522006833701));
#139135=CARTESIAN_POINT('Ctrl Pts',(-0.215486066129178,4.21216499508158,
-7.49690374451352));
#139136=CARTESIAN_POINT('Ctrl Pts',(0.354278060649863,4.30331728230629,
-7.49163217195819));
#139137=CARTESIAN_POINT('Ctrl Pts',(0.350234234324932,4.30267205415314,
-7.49181902897909));
#139138=CARTESIAN_POINT('Ctrl Pts',(0.346190408,4.302026826,-7.492005886));
#139139=CARTESIAN_POINT('Ctrl Pts',(-0.059481935,4.237298226,-7.510751183));
#139140=CARTESIAN_POINT('Ctrl Pts',(-0.464806504,4.172121859,-7.48558313800001));
#139141=CARTESIAN_POINT('Ctrl Pts',(0.579786081215257,4.30331728230629,
-7.22678416372269));
#139142=CARTESIAN_POINT('Ctrl Pts',(0.575885075607629,4.30267205415314,
-7.22709289336134));
#139143=CARTESIAN_POINT('Ctrl Pts',(0.57198407,4.302026826,-7.227401623));
#139144=CARTESIAN_POINT('Ctrl Pts',(0.180639349,4.237298226,-7.258373051));
#139145=CARTESIAN_POINT('Ctrl Pts',(-0.211761522,4.172121859,-7.246906723));
#139146=CARTESIAN_POINT('',(0.459087249095649,4.30202682438522,-7.35970375387025));
#139147=CARTESIAN_POINT('Ctrl Pts',(1.64809316,4.172114527,-7.316678819));
#139148=CARTESIAN_POINT('Ctrl Pts',(1.296998114,4.22940039,-7.395763518));
#139149=CARTESIAN_POINT('Ctrl Pts',(0.939943815,4.285714286,-7.440867263));
#139150=CARTESIAN_POINT('Ctrl Pts',(0.888308847999999,4.29385805,-7.447389885));
#139151=CARTESIAN_POINT('Ctrl Pts',(0.836588333,4.302026826,-7.453195285));
#139152=CARTESIAN_POINT('Ctrl Pts',(1.360344644,4.172114527,-7.121233211));
#139153=CARTESIAN_POINT('Ctrl Pts',(1.018628168,4.22940039,-7.186510132));
#139154=CARTESIAN_POINT('Ctrl Pts',(0.672231452,4.285714286,-7.218767545));
#139155=CARTESIAN_POINT('Ctrl Pts',(0.622137718,4.29385805,-7.223432411));
#139156=CARTESIAN_POINT('Ctrl Pts',(0.57198407,4.302026826,-7.227401623));
#139157=CARTESIAN_POINT('',(0.83658833931498,4.30202682641444,-7.45319528481644));
#139158=CARTESIAN_POINT('',(0.704286205537671,4.30202682665756,-7.3402984536126));
#139159=CARTESIAN_POINT('',(1.40116456911329,4.21216499392617,-7.36795343699078));
#139160=CARTESIAN_POINT('Ctrl Pts',(0.836588339904591,4.30202682552109,
-7.45319528454309));
#139161=CARTESIAN_POINT('Ctrl Pts',(0.871093976326916,4.29657697961046,
-7.44932217884951));
#139162=CARTESIAN_POINT('Ctrl Pts',(0.90554739726429,4.29113922035365,-7.44521228065406));
#139163=CARTESIAN_POINT('Ctrl Pts',(0.939943814463379,4.28571428571329,
-7.44086726300447));
#139164=CARTESIAN_POINT('Ctrl Pts',(1.09390076555659,4.26143250100661,-7.42141914240793));
#139165=CARTESIAN_POINT('Ctrl Pts',(1.24779320355042,4.23689343092027,-7.39712008746252));
#139166=CARTESIAN_POINT('Ctrl Pts',(1.40116456249542,4.21216499285671,-7.3679534382898));
#139167=CARTESIAN_POINT('Ctrl Pts',(1.35566166214689,4.17289950714709,-7.12212619271643));
#139168=CARTESIAN_POINT('Ctrl Pts',(1.36327136050992,4.17977820208819,-7.16302946035241));
#139169=CARTESIAN_POINT('Ctrl Pts',(1.37087132825782,4.18648410045764,-7.20399006333472));
#139170=CARTESIAN_POINT('Ctrl Pts',(1.38603537237231,4.19956141147093,-7.28591881362589));
#139171=CARTESIAN_POINT('Ctrl Pts',(1.39360836328108,4.20594050666662,-7.32693513667193));
#139172=CARTESIAN_POINT('Ctrl Pts',(1.40116457618158,4.2121649950616,-7.36795343551639));
#139173=CARTESIAN_POINT('Ctrl Pts',(1.95647470236699,4.30331728230629,-7.24032266494494));
#139174=CARTESIAN_POINT('Ctrl Pts',(1.9525655871835,4.30267205415314,-7.24137445647247));
#139175=CARTESIAN_POINT('Ctrl Pts',(1.948656472,4.302026826,-7.242426248));
#139176=CARTESIAN_POINT('Ctrl Pts',(1.556498207,4.237298226,-7.347940852));
#139177=CARTESIAN_POINT('Ctrl Pts',(1.155239516,4.172121859,-7.410494023));
#139178=CARTESIAN_POINT('Ctrl Pts',(2.11977597804828,4.30331728230629,-6.93318909679542));
#139179=CARTESIAN_POINT('Ctrl Pts',(2.11603254352414,4.30267205415314,-6.93432920939771));
#139180=CARTESIAN_POINT('Ctrl Pts',(2.112289109,4.302026826,-6.935469322));
#139181=CARTESIAN_POINT('Ctrl Pts',(1.736751751,4.237298226,-7.049844202));
#139182=CARTESIAN_POINT('Ctrl Pts',(1.351060074,4.172121859,-7.123000539));
#139183=CARTESIAN_POINT('',(1.94865647508094,4.30202682545393,-7.24242624901735));
#139184=CARTESIAN_POINT('Origin',(-0.0275791282628238,4.16072876086824,
0.189274367559337));
#139185=CARTESIAN_POINT('',(2.03047280022433,4.30202682438522,-7.08894778221468));
#139186=CARTESIAN_POINT('Origin',(1.07661275727811E-13,4.39277644300133,
-1.57426155444895E-13));
#139187=CARTESIAN_POINT('',(1.39580564426364,4.39169923738589,-7.36897052498046));
#139188=CARTESIAN_POINT('Origin',(0.00178446840968821,4.16082465943076,
0.186223212668429));
#139189=CARTESIAN_POINT('Origin',(-0.00871151387813629,4.55341982448314,
0.184430458010395));
#139190=CARTESIAN_POINT('Ctrl Pts',(3.182431324,4.172114527,-6.791327622));
#139191=CARTESIAN_POINT('Ctrl Pts',(2.856545558,4.22940039,-6.944038421));
#139192=CARTESIAN_POINT('Ctrl Pts',(2.517534962,4.285714286,-7.064843786));
#139193=CARTESIAN_POINT('Ctrl Pts',(2.468509363,4.29385805,-7.082313904));
#139194=CARTESIAN_POINT('Ctrl Pts',(2.419246034,4.302026826,-7.099101959));
#139195=CARTESIAN_POINT('Ctrl Pts',(2.85939518,4.172114527,-6.66230884900001));
#139196=CARTESIAN_POINT('Ctrl Pts',(2.539700455,4.22940039,-6.799518573));
#139197=CARTESIAN_POINT('Ctrl Pts',(2.208336691,4.285714286,-6.905486881));
#139198=CARTESIAN_POINT('Ctrl Pts',(2.16041693,4.29385805,-6.920811357));
#139199=CARTESIAN_POINT('Ctrl Pts',(2.112289109,4.302026826,-6.93546932199999));
#139200=CARTESIAN_POINT('',(2.41924604010374,4.30202682641444,-7.09910195741508));
#139201=CARTESIAN_POINT('',(2.26576757536,4.30202682665756,-7.01728563925367));
#139202=CARTESIAN_POINT('',(2.95229831432839,4.21216499391278,-6.89448581575544));
#139203=CARTESIAN_POINT('Ctrl Pts',(2.41924604060121,4.30202682552109,-7.09910195694042));
#139204=CARTESIAN_POINT('Ctrl Pts',(2.45211235138791,4.29657697961046,-7.08790171038499));
#139205=CARTESIAN_POINT('Ctrl Pts',(2.4848767638631,4.29113922035365,-7.07648143225898));
#139206=CARTESIAN_POINT('Ctrl Pts',(2.51753496156321,4.28571428571329,-7.06484378576816));
#139207=CARTESIAN_POINT('Ctrl Pts',(2.66371171372217,4.26143250097783,-7.01275415784613));
#139208=CARTESIAN_POINT('Ctrl Pts',(2.80878265369269,4.23689343089126,-6.95594087607972));
#139209=CARTESIAN_POINT('Ctrl Pts',(2.95229830817655,4.21216499285671,-6.89448581835788));
#139210=CARTESIAN_POINT('Ctrl Pts',(2.85501364803054,4.17289950713964,-6.66418765580658));
#139211=CARTESIAN_POINT('Ctrl Pts',(2.87123842958936,4.17977820207062,-6.70249876752659));
#139212=CARTESIAN_POINT('Ctrl Pts',(2.88746603344633,4.18648410046127,-6.74086796610841));
#139213=CARTESIAN_POINT('Ctrl Pts',(2.91988781046986,4.19956141145946,-6.81762144647725));
#139214=CARTESIAN_POINT('Ctrl Pts',(2.93610104616866,4.20594050663945,-6.85605086142833));
#139215=CARTESIAN_POINT('Ctrl Pts',(2.95229832085231,4.21216499503082,-6.89448581282505));
#139216=CARTESIAN_POINT('Ctrl Pts',(3.46718876129397,4.30331728230629,-6.65046371610525));
#139217=CARTESIAN_POINT('Ctrl Pts',(3.46359714314698,4.30267205415314,-6.65233126155262));
#139218=CARTESIAN_POINT('Ctrl Pts',(3.460005525,4.302026826,-6.654198807));
#139219=CARTESIAN_POINT('Ctrl Pts',(3.099698224,4.237298226,-6.841548974));
#139220=CARTESIAN_POINT('Ctrl Pts',(2.721267821,4.172121859,-6.988898443));
#139221=CARTESIAN_POINT('Ctrl Pts',(3.56064750517537,4.30331728230629,-6.31540581365904));
#139222=CARTESIAN_POINT('Ctrl Pts',(3.55723668058768,4.30267205415314,-6.31732399882952));
#139223=CARTESIAN_POINT('Ctrl Pts',(3.553825856,4.302026826,-6.319242184));
#139224=CARTESIAN_POINT('Ctrl Pts',(3.211655572,4.237298226,-6.511672474));
#139225=CARTESIAN_POINT('Ctrl Pts',(2.850707601,4.172121859,-6.666030766));
#139226=CARTESIAN_POINT('',(3.46000552820812,4.30202682545392,-6.65419880735245));
#139227=CARTESIAN_POINT('Origin',(-0.0676225796773755,4.16072876375072,
0.1789201855255));
#139228=CARTESIAN_POINT('',(3.50691569939822,4.30202682438522,-6.48672049068936));
#139229=CARTESIAN_POINT('Origin',(1.59160878920872E-13,4.39277644299978,
-3.81639164714898E-13));
#139230=CARTESIAN_POINT('',(2.94728332132454,4.39169923738473,-6.89663113553976));
#139231=CARTESIAN_POINT('Origin',(-0.038289672908362,4.16082472551501,0.182252826938747));
#139232=CARTESIAN_POINT('Origin',(-0.048155027945111,4.55341983599227,0.178246030496119));
#139233=CARTESIAN_POINT('Ctrl Pts',(4.567962537,4.172114527,-5.948421493));
#139234=CARTESIAN_POINT('Ctrl Pts',(4.282524107,4.22940039,-6.167617806));
#139235=CARTESIAN_POINT('Ctrl Pts',(3.977408972,4.285714286,-6.358476065));
#139236=CARTESIAN_POINT('Ctrl Pts',(3.933285124,4.29385805,-6.38607679600001));
#139237=CARTESIAN_POINT('Ctrl Pts',(3.88878248,4.302026826,-6.413062515));
#139238=CARTESIAN_POINT('Ctrl Pts',(4.224743576,4.172114527,-5.89186233000001));
#139239=CARTESIAN_POINT('Ctrl Pts',(3.94201917,4.22940039,-6.094589083));
#139240=CARTESIAN_POINT('Ctrl Pts',(3.641182561,4.285714286,-6.269313324));
#139241=CARTESIAN_POINT('Ctrl Pts',(3.597677446,4.29385805,-6.294580855));
#139242=CARTESIAN_POINT('Ctrl Pts',(3.553825856,4.302026826,-6.319242184));
#139243=CARTESIAN_POINT('',(3.88878248551807,4.30202682620654,-6.41306251204045));
#139244=CARTESIAN_POINT('',(3.72130417150183,4.30202682665756,-6.36615234745303));
#139245=CARTESIAN_POINT('',(4.36538587107081,4.21216499538059,-6.09863970011031));
#139246=CARTESIAN_POINT('Ctrl Pts',(3.88878248571021,4.3020268248974,-6.41306251127443));
#139247=CARTESIAN_POINT('Ctrl Pts',(3.91847267837001,4.29657697940857,-6.39505883492328));
#139248=CARTESIAN_POINT('Ctrl Pts',(3.94801605464148,4.29113922035353,-6.37686217649245));
#139249=CARTESIAN_POINT('Ctrl Pts',(3.97740897183812,4.2857142859281,-6.35847606461008));
#139250=CARTESIAN_POINT('Ctrl Pts',(4.10897046367738,4.26143250061917,-6.27618058148517));
#139251=CARTESIAN_POINT('Ctrl Pts',(4.23843654813059,4.23689343234178,-6.18950960024396));
#139252=CARTESIAN_POINT('Ctrl Pts',(4.36538586557831,4.21216499711468,-6.09863970360881));
#139253=CARTESIAN_POINT('Ctrl Pts',(4.22086836923851,4.17289950698576,-5.8946391104573));
#139254=CARTESIAN_POINT('Ctrl Pts',(4.24494958093159,4.17977820193852,-5.92856668125073));
#139255=CARTESIAN_POINT('Ctrl Pts',(4.26904603628066,4.18648410046027,-5.96255037473311));
#139256=CARTESIAN_POINT('Ctrl Pts',(4.31720953947562,4.19956141148043,-6.03053967769934));
#139257=CARTESIAN_POINT('Ctrl Pts',(4.34130490693522,4.20594050667908,-6.06458526792232));
#139258=CARTESIAN_POINT('Ctrl Pts',(4.36538587665905,4.21216499507077,-6.09863969621531));
#139259=CARTESIAN_POINT('Ctrl Pts',(4.81578092811415,4.30331728230629,-5.74963647599278));
#139260=CARTESIAN_POINT('Ctrl Pts',(4.81267474705707,4.30267205415314,-5.75223245099639));
#139261=CARTESIAN_POINT('Ctrl Pts',(4.809568566,4.302026826,-5.75482842600001));
#139262=CARTESIAN_POINT('Ctrl Pts',(4.497959796,4.237298226,-6.015253869));
#139263=CARTESIAN_POINT('Ctrl Pts',(4.160052666,4.172121859,-6.24050974));
#139264=CARTESIAN_POINT('Ctrl Pts',(4.83502711359236,4.30331728230629,-5.40232117394616));
#139265=CARTESIAN_POINT('Ctrl Pts',(4.83210838529618,4.30267205415314,-5.40492773947309));
#139266=CARTESIAN_POINT('Ctrl Pts',(4.829189657,4.302026826,-5.407534305));
#139267=CARTESIAN_POINT('Ctrl Pts',(4.536385948,4.237298226,-5.669022178));
#139268=CARTESIAN_POINT('Ctrl Pts',(4.21705921,4.172121859,-5.897364803));
#139269=CARTESIAN_POINT('',(4.80956856922516,4.30202682545373,-5.75482842562856));
#139270=CARTESIAN_POINT('Origin',(-0.104504317360521,4.16072873536559,0.16020051259355));
#139271=CARTESIAN_POINT('',(4.81937911915879,4.30202682438463,-5.5811813588866));
#139272=CARTESIAN_POINT('Origin',(-9.54097911787244E-14,4.39277644299978,
-5.76795555762288E-14));
#139273=CARTESIAN_POINT('',(4.36094930658773,4.39169923740455,-6.10181293897598));
#139274=CARTESIAN_POINT('Origin',(-0.0765736298748837,4.16082464507458,
0.169761002488217));
#139275=CARTESIAN_POINT('Origin',(-0.0853466643918449,4.55341982008006,
0.163726636932791));
#139276=CARTESIAN_POINT('Ctrl Pts',(5.739900898,4.172114527,-4.827373787));
#139277=CARTESIAN_POINT('Ctrl Pts',(5.50825658799999,4.22940039,-5.102806236));
#139278=CARTESIAN_POINT('Ctrl Pts',(5.251303759,4.285714286,-5.35479307));
#139279=CARTESIAN_POINT('Ctrl Pts',(5.214144843,4.29385805,-5.391233835));
#139280=CARTESIAN_POINT('Ctrl Pts',(5.176483778,4.302026826,-5.427155396));
#139281=CARTESIAN_POINT('Ctrl Pts',(5.392547658,4.172114527,-4.845918877));
#139282=CARTESIAN_POINT('Ctrl Pts',(5.160013451,4.22940039,-5.10468338));
#139283=CARTESIAN_POINT('Ctrl Pts',(4.903770781,4.285714286,-5.339993645));
#139284=CARTESIAN_POINT('Ctrl Pts',(4.866714564,4.29385805,-5.374022748));
#139285=CARTESIAN_POINT('Ctrl Pts',(4.829189657,4.302026826,-5.40753430500001));
#139286=CARTESIAN_POINT('',(5.17648378289629,4.30202682641444,-5.42715539201625));
#139287=CARTESIAN_POINT('',(5.00110024987486,4.30202682665756,-5.41724674229405));
#139288=CARTESIAN_POINT('',(5.57435283649055,4.21216499393313,-5.01762797091983));
#139289=CARTESIAN_POINT('Ctrl Pts',(5.17648378317564,4.30202682552109,-5.42715539141083));
#139290=CARTESIAN_POINT('Ctrl Pts',(5.20160957745646,4.29657697961046,-5.40319011729322));
#139291=CARTESIAN_POINT('Ctrl Pts',(5.22655050253311,4.29113922035365,-5.37906793386813));
#139292=CARTESIAN_POINT('Ctrl Pts',(5.2513037591335,4.28571428571329,-5.35479307063405));
#139293=CARTESIAN_POINT('Ctrl Pts',(5.36209831934726,4.26143250100229,-5.24613977948583));
#139294=CARTESIAN_POINT('Ctrl Pts',(5.46990586068578,4.23689343091578,-5.1336637348362));
#139295=CARTESIAN_POINT('Ctrl Pts',(5.57435283192434,4.21216499285632,-5.01762797596803));
#139296=CARTESIAN_POINT('Ctrl Pts',(5.38935997722701,4.17289950705447,-4.84946379305138));
#139297=CARTESIAN_POINT('Ctrl Pts',(5.42017160857531,4.17977820204229,-4.87742140740549));
#139298=CARTESIAN_POINT('Ctrl Pts',(5.45101019120633,4.18648410043973,-4.90543055477744));
#139299=CARTESIAN_POINT('Ctrl Pts',(5.51266334906687,4.19956141148847,-4.9614765760749));
#139300=CARTESIAN_POINT('Ctrl Pts',(5.54351417574768,4.20594050667875,-4.98954640745752));
#139301=CARTESIAN_POINT('Ctrl Pts',(5.5743528412703,4.21216499507376,-5.01762796541796));
#139302=CARTESIAN_POINT('Ctrl Pts',(5.93919252974169,4.30331728230629,-4.57996262468676));
#139303=CARTESIAN_POINT('Ctrl Pts',(5.93671702737085,4.30267205415314,-4.58316564434338));
#139304=CARTESIAN_POINT('Ctrl Pts',(5.934241525,4.302026826,-4.586368664));
#139305=CARTESIAN_POINT('Ctrl Pts',(5.685901768,4.237298226,-4.907692179));
#139306=CARTESIAN_POINT('Ctrl Pts',(5.404318073,4.172121859,-5.20032173700001));
#139307=CARTESIAN_POINT('Ctrl Pts',(5.88332622702706,4.30331728230629,-4.23662999944104));
#139308=CARTESIAN_POINT('Ctrl Pts',(5.88103607151352,4.30267205415314,-4.23980306522052));
#139309=CARTESIAN_POINT('Ctrl Pts',(5.878745916,4.302026826,-4.242976131));
#139310=CARTESIAN_POINT('Ctrl Pts',(5.648999958,4.237298226,-4.561294705));
#139311=CARTESIAN_POINT('Ctrl Pts',(5.386225817,4.172121859,-4.852944616));
#139312=CARTESIAN_POINT('',(5.93424152780051,4.3020268254538,-4.58636866354332));
#139313=CARTESIAN_POINT('Origin',(-0.13649934832537,4.16072874717212,0.1339896869126));
#139314=CARTESIAN_POINT('',(5.90649372655079,4.30202682438657,-4.4146723894045));
#139315=CARTESIAN_POINT('Origin',(1.14925430283463E-13,4.39277644300022,
-2.97071395261028E-13));
#139316=CARTESIAN_POINT('',(5.57070214838826,4.39169923734753,-5.02168075129061));
#139317=CARTESIAN_POINT('Origin',(-0.111276857686425,4.16082467415457,0.149330892505302));
#139318=CARTESIAN_POINT('Origin',(-0.118547837337244,4.55341981857088,0.141551906684535));
#139319=CARTESIAN_POINT('Ctrl Pts',(6.643447873,4.172114527,-3.480603448));
#139320=CARTESIAN_POINT('Ctrl Pts',(6.476429113,4.22940039,-3.799393119));
#139321=CARTESIAN_POINT('Ctrl Pts',(6.279653419,4.285714286,-4.100725903));
#139322=CARTESIAN_POINT('Ctrl Pts',(6.25119694500001,4.29385805,-4.144302772));
#139323=CARTESIAN_POINT('Ctrl Pts',(6.222138449,4.302026826,-4.187480522));
#139324=CARTESIAN_POINT('Ctrl Pts',(6.308202204,4.172114527,-3.573385642));
#139325=CARTESIAN_POINT('Ctrl Pts',(6.136731237,4.22940039,-3.876088357));
#139326=CARTESIAN_POINT('Ctrl Pts',(5.93706413,4.285714286,-4.160981797));
#139327=CARTESIAN_POINT('Ctrl Pts',(5.908189518,4.29385805,-4.20218131));
#139328=CARTESIAN_POINT('Ctrl Pts',(5.878745916,4.302026826,-4.242976131));
#139329=CARTESIAN_POINT('',(6.22213845282046,4.30202682641444,-4.18748051700569));
#139330=CARTESIAN_POINT('',(6.05044218481867,4.30202682665756,-4.21522832317184));
#139331=CARTESIAN_POINT('',(6.52266925847057,4.21216499391789,-3.70199753443422));
#139332=CARTESIAN_POINT('Ctrl Pts',(6.22213845282351,4.30202682552109,-4.18748051624066));
#139333=CARTESIAN_POINT('Ctrl Pts',(6.24152499419235,4.29657697961046,-4.15867423426502));
#139334=CARTESIAN_POINT('Ctrl Pts',(6.26069725783376,4.29113922035365,-4.12975445256131));
#139335=CARTESIAN_POINT('Ctrl Pts',(6.27965341901304,4.28571428571329,-4.10072590367582));
#139336=CARTESIAN_POINT('Ctrl Pts',(6.36450041815192,4.26143250099931,-3.97079531071474));
#139337=CARTESIAN_POINT('Ctrl Pts',(6.44560845419607,4.23689343091297,-3.83777345896538));
#139338=CARTESIAN_POINT('Ctrl Pts',(6.5226692551384,4.21216499285688,-3.70199754025746));
#139339=CARTESIAN_POINT('Ctrl Pts',(6.30585110167865,4.17289950699659,-3.57753293676332));
#139340=CARTESIAN_POINT('Ctrl Pts',(6.34195243458989,4.17977820193396,-3.59821332791846));
#139341=CARTESIAN_POINT('Ctrl Pts',(6.37809116773949,4.18648410045907,-3.61893825397248));
#139342=CARTESIAN_POINT('Ctrl Pts',(6.45035114673858,4.19956141146249,-3.66042034419561));
#139343=CARTESIAN_POINT('Ctrl Pts',(6.48651488228287,4.20594050664729,-3.68120190282239));
#139344=CARTESIAN_POINT('Ctrl Pts',(6.52266926190589,4.21216499504144,-3.70199752812543));
#139345=CARTESIAN_POINT('Ctrl Pts',(6.78489409091065,4.30331728230629,-3.19613481065053));
#139346=CARTESIAN_POINT('Ctrl Pts',(6.78316501895532,4.30267205415314,-3.19979510532527));
#139347=CARTESIAN_POINT('Ctrl Pts',(6.781435947,4.302026826,-3.2034554));
#139348=CARTESIAN_POINT('Ctrl Pts',(6.60797729300001,4.237298226,-3.570652257));
#139349=CARTESIAN_POINT('Ctrl Pts',(6.395883572,4.172121859,-3.91697247));
#139350=CARTESIAN_POINT('Ctrl Pts',(6.65652754520183,4.30331728230629,-2.87283871599968));
#139351=CARTESIAN_POINT('Ctrl Pts',(6.65497304760091,4.30267205415314,-2.87642991299984));
#139352=CARTESIAN_POINT('Ctrl Pts',(6.65341854999999,4.302026826,-2.88002111));
#139353=CARTESIAN_POINT('Ctrl Pts',(6.497473009,4.237298226,-3.240286162));
#139354=CARTESIAN_POINT('Ctrl Pts',(6.303538491,4.172121859,-3.581606133));
#139355=CARTESIAN_POINT('',(6.78143594964156,4.30202682545316,-3.20345539893517));
#139356=CARTESIAN_POINT('Origin',(-0.162111758480733,4.16072877310877,0.101513687625245));
#139357=CARTESIAN_POINT('',(6.71742725267403,4.30202682438463,-3.041738245782));
#139358=CARTESIAN_POINT('Origin',(-1.1666015375944E-13,4.392776443,2.42861286636753E-14));
#139359=CARTESIAN_POINT('',(6.51997514986713,4.39169923735663,-3.70674035236029));
#139360=CARTESIAN_POINT('Origin',(-0.140777006050024,4.16082471773229,0.121918379360347));
#139361=CARTESIAN_POINT('Origin',(-0.146205751230233,4.55341981097136,0.112758233578279));
#139362=CARTESIAN_POINT('Ctrl Pts',(7.236354609,4.172114527,-1.971083959));
#139363=CARTESIAN_POINT('Ctrl Pts',(7.14177101,4.22940039,-2.318324601));
#139364=CARTESIAN_POINT('Ctrl Pts',(7.014373465,4.285714286,-2.65491335));
#139365=CARTESIAN_POINT('Ctrl Pts',(6.995950026,4.29385805,-2.703588717));
#139366=CARTESIAN_POINT('Ctrl Pts',(6.97685284100001,4.302026826,-2.752003713));
#139367=CARTESIAN_POINT('Ctrl Pts',(6.928892227,4.172114527,-2.133764867));
#139368=CARTESIAN_POINT('Ctrl Pts',(6.826502291,4.22940039,-2.466251749));
#139369=CARTESIAN_POINT('Ctrl Pts',(6.692746959,4.285714286,-2.787407065));
#139370=CARTESIAN_POINT('Ctrl Pts',(6.673404096,4.29385805,-2.833850545));
#139371=CARTESIAN_POINT('Ctrl Pts',(6.65341855,4.302026826,-2.88002111));
#139372=CARTESIAN_POINT('',(6.97685284363954,4.30202682641444,-2.75200370729722));
#139373=CARTESIAN_POINT('',(6.81513569704902,4.30202682665757,-2.81601240775116));
#139374=CARTESIAN_POINT('',(7.16599291560661,4.21216499395295,-2.21326580715179));
#139375=CARTESIAN_POINT('Ctrl Pts',(6.97685284345356,4.30202682552109,-2.75200370653707));
#139376=CARTESIAN_POINT('Ctrl Pts',(6.98959363920653,4.29657697961046,-2.71970336592859));
#139377=CARTESIAN_POINT('Ctrl Pts',(7.00210076784173,4.29113922035365,-2.68733824251606));
#139378=CARTESIAN_POINT('Ctrl Pts',(7.01437346458369,4.28571428571329,-2.65491335062824));
#139379=CARTESIAN_POINT('Ctrl Pts',(7.06930555124679,4.26143250102719,-2.50978086600207));
#139380=CARTESIAN_POINT('Ctrl Pts',(7.1199215604026,4.23689343094102,-2.36243316113239));
#139381=CARTESIAN_POINT('Ctrl Pts',(7.16599291358868,4.21216499285673,-2.21326581376853));
#139382=CARTESIAN_POINT('Ctrl Pts',(6.92748763804898,4.17289950710276,-2.13832061824829));
#139383=CARTESIAN_POINT('Ctrl Pts',(6.96719061483953,4.17977820206479,-2.1507567935532));
#139384=CARTESIAN_POINT('Ctrl Pts',(7.00693969037473,4.18648410049305,-2.16322842251709));
#139385=CARTESIAN_POINT('Ctrl Pts',(7.08642769447389,4.1995614115264,-2.18820692471099));
#139386=CARTESIAN_POINT('Ctrl Pts',(7.12621336273325,4.20594050671967,-2.20072848782133));
#139387=CARTESIAN_POINT('Ctrl Pts',(7.16599291766674,4.21216499511605,-2.21326580003777));
#139388=CARTESIAN_POINT('Ctrl Pts',(7.31334154411131,4.30331728230629,-1.66285928523758));
#139389=CARTESIAN_POINT('Ctrl Pts',(7.31243975205566,4.30267205415314,-1.66680570361879));
#139390=CARTESIAN_POINT('Ctrl Pts',(7.31153796000001,4.302026826,-1.670752122));
#139391=CARTESIAN_POINT('Ctrl Pts',(7.221071143,4.237298226,-2.066652604));
#139392=CARTESIAN_POINT('Ctrl Pts',(7.088384665,4.172121859,-2.450469923));
#139393=CARTESIAN_POINT('Ctrl Pts',(7.11847703421988,4.30331728230629,-1.37471668631063));
#139394=CARTESIAN_POINT('Ctrl Pts',(7.11773088110994,4.30267205415314,-1.37855809415531));
#139395=CARTESIAN_POINT('Ctrl Pts',(7.116984728,4.302026826,-1.382399502));
#139396=CARTESIAN_POINT('Ctrl Pts',(7.042131444,4.237298226,-1.767765439));
#139397=CARTESIAN_POINT('Ctrl Pts',(6.926104711,4.172121859,-2.142795728));
#139398=CARTESIAN_POINT('',(7.31153796235453,4.30202682545332,-1.67075212042859));
#139399=CARTESIAN_POINT('Origin',(-0.180144240362469,4.16072874364623,0.0642911481372335));
#139400=CARTESIAN_POINT('',(7.21426134609414,4.30202682438518,-1.52657580210354));
#139401=CARTESIAN_POINT('Origin',(1.90819582357449E-14,4.39277644300067,
-5.85469173142172E-15));
#139402=CARTESIAN_POINT('',(7.16438135929105,4.39169923736879,-2.21847689478551));
#139403=CARTESIAN_POINT('Origin',(-0.163694659822479,4.16082469767973,0.0888051356908687));
#139404=CARTESIAN_POINT('Origin',(-0.167027008642707,4.5534198132657,0.0786920270273214));
#139405=CARTESIAN_POINT('Ctrl Pts',(7.490897446,4.172114527,-0.369398776));
#139406=CARTESIAN_POINT('Ctrl Pts',(7.473171633,4.22940039,-0.728853803));
#139407=CARTESIAN_POINT('Ctrl Pts',(7.421109203,4.285714286,-1.08496));
#139408=CARTESIAN_POINT('Ctrl Pts',(7.413580259,4.29385805,-1.136457858));
#139409=CARTESIAN_POINT('Ctrl Pts',(7.405337348,4.302026826,-1.187846269));
#139410=CARTESIAN_POINT('Ctrl Pts',(7.22559495,4.172114527,-0.594371618));
#139411=CARTESIAN_POINT('Ctrl Pts',(7.197073686,4.22940039,-0.941095951));
#139412=CARTESIAN_POINT('Ctrl Pts',(7.135484378,4.285714286,-1.283496277));
#139413=CARTESIAN_POINT('Ctrl Pts',(7.126577716,4.29385805,-1.333012078));
#139414=CARTESIAN_POINT('Ctrl Pts',(7.116984728,4.302026826,-1.382399502));
#139415=CARTESIAN_POINT('',(7.40533734948122,4.30202682641445,-1.18784626286505));
#139416=CARTESIAN_POINT('',(7.26116103870691,4.30202682665756,-1.28512288150586));
#139417=CARTESIAN_POINT('',(7.47424270827965,4.21216499391622,-0.621044231009006));
#139418=CARTESIAN_POINT('Ctrl Pts',(7.40533734932785,4.30202682552109,-1.18784626221161));
#139419=CARTESIAN_POINT('Ctrl Pts',(7.41083665397239,4.29657697961046,-1.15356219080014));
#139420=CARTESIAN_POINT('Ctrl Pts',(7.41609382804621,4.29113922035365,-1.1192650831263));
#139421=CARTESIAN_POINT('Ctrl Pts',(7.42110920265718,4.28571428571329,-1.08496000029361));
#139422=CARTESIAN_POINT('Ctrl Pts',(7.44355781350102,4.26143250099309,-0.931411857988833));
#139423=CARTESIAN_POINT('Ctrl Pts',(7.46131504754232,4.2368934309067,-0.776628114674704));
#139424=CARTESIAN_POINT('Ctrl Pts',(7.474242707784,4.21216499285688,-0.621044237665823));
#139425=CARTESIAN_POINT('Ctrl Pts',(7.22520255128188,4.17289950705358,-0.599122803260408));
#139426=CARTESIAN_POINT('Ctrl Pts',(7.26665070451171,4.17977820198768,-0.602733261370328));
#139427=CARTESIAN_POINT('Ctrl Pts',(7.30815150059235,4.18648410045454,-0.60636843442612));
#139428=CARTESIAN_POINT('Ctrl Pts',(7.39115075880867,4.1995614114589,-0.613675382042574));
#139429=CARTESIAN_POINT('Ctrl Pts',(7.43269802619587,4.20594050665111,-0.617351455425911));
#139430=CARTESIAN_POINT('Ctrl Pts',(7.47424270874489,4.21216499504173,-0.621044223877748));
#139431=CARTESIAN_POINT('Ctrl Pts',(7.49982527573975,4.30331728230629,-0.0518303081088053));
#139432=CARTESIAN_POINT('Ctrl Pts',(7.49979293036987,4.30267205415314,-0.0558783200544026));
#139433=CARTESIAN_POINT('Ctrl Pts',(7.499760585,4.302026826,-0.059926332));
#139434=CARTESIAN_POINT('Ctrl Pts',(7.496515732,4.237298226,-0.466018572));
#139435=CARTESIAN_POINT('Ctrl Pts',(7.449440769,4.172121859,-0.869386126));
#139436=CARTESIAN_POINT('Ctrl Pts',(7.24757444764504,4.30331728230629,0.187685567453841));
#139437=CARTESIAN_POINT('Ctrl Pts',(7.24767152832252,4.30267205415314,0.18377356872692));
#139438=CARTESIAN_POINT('Ctrl Pts',(7.247768609,4.302026826,0.17986157));
#139439=CARTESIAN_POINT('Ctrl Pts',(7.25750763900001,4.237298226,-0.212585969));
#139440=CARTESIAN_POINT('Ctrl Pts',(7.224813973,4.172121859,-0.603790576));
#139441=CARTESIAN_POINT('',(7.49976058695747,4.30202682545315,-0.0599263299449481));
#139442=CARTESIAN_POINT('Origin',(-0.189753551632893,4.16072874191932,0.0240623880134643));
#139443=CARTESIAN_POINT('',(7.37376459691771,4.30202682438463,0.0599676291186608));
#139444=CARTESIAN_POINT('Origin',(2.31932528738099E-12,4.39277644299933,
-2.63183301107278E-13));
#139445=CARTESIAN_POINT('',(7.47378905921352,4.39169923737642,-0.626479923766734));
#139446=CARTESIAN_POINT('Origin',(-0.178957929415752,4.16082468300723,0.0515394024429872));
#139447=CARTESIAN_POINT('Origin',(-0.180038598006461,4.55341981446118,0.0409463889791393));
#139448=CARTESIAN_POINT('Ctrl Pts',(7.395174244,4.172114527,1.249559084));
#139449=CARTESIAN_POINT('Ctrl Pts',(7.455135056,4.22940039,0.894697389999999));
#139450=CARTESIAN_POINT('Ctrl Pts',(7.480842122,4.285714286,0.535724874));
#139451=CARTESIAN_POINT('Ctrl Pts',(7.484559718,4.29385805,0.483812507));
#139452=CARTESIAN_POINT('Ctrl Pts',(7.487556512,4.302026826,0.431853546));
#139453=CARTESIAN_POINT('Ctrl Pts',(7.18443688400001,4.172114527,0.972813787));
#139454=CARTESIAN_POINT('Ctrl Pts',(7.231117913,4.22940039,0.628064447));
#139455=CARTESIAN_POINT('Ctrl Pts',(7.244574478,4.285714286,0.28042937));
#139456=CARTESIAN_POINT('Ctrl Pts',(7.246520483,4.29385805,0.230156553));
#139457=CARTESIAN_POINT('Ctrl Pts',(7.247768609,4.302026826,0.17986157));
#139458=CARTESIAN_POINT('',(7.48755651189106,4.30202682641444,0.431853552262134));
#139459=CARTESIAN_POINT('',(7.36766256033176,4.30202682665756,0.305857562052724));
#139460=CARTESIAN_POINT('',(7.43300521886331,4.21216499391146,1.00021668358226));
#139461=CARTESIAN_POINT('Ctrl Pts',(7.48755651123017,4.30202682552109,0.431853552879705));
#139462=CARTESIAN_POINT('Ctrl Pts',(7.48555718325308,4.29657697961046,0.466518269918783));
#139463=CARTESIAN_POINT('Ctrl Pts',(7.48331858317738,4.29113922035365,0.501143667389628));
#139464=CARTESIAN_POINT('Ctrl Pts',(7.48084212235687,4.28571428571329,0.535724873765609));
#139465=CARTESIAN_POINT('Ctrl Pts',(7.46975758539743,4.26143250098825,0.69050893374431));
#139466=CARTESIAN_POINT('Ctrl Pts',(7.45382573571466,4.23689343090182,0.845491199722909));
#139467=CARTESIAN_POINT('Ctrl Pts',(7.43300521989358,4.21216499285686,1.00021667704294));
#139468=CARTESIAN_POINT('Ctrl Pts',(7.18507502302376,4.17289950688029,0.968089327989833));
#139469=CARTESIAN_POINT('Ctrl Pts',(7.22633028323422,4.17977820185,0.973473408110541));
#139470=CARTESIAN_POINT('Ctrl Pts',(7.26764226897952,4.18648410041496,0.978844667865212));
#139471=CARTESIAN_POINT('Ctrl Pts',(7.35027182833364,4.19956141144009,0.989550939784512));
#139472=CARTESIAN_POINT('Ctrl Pts',(7.39163799084773,4.20594050664826,0.994892245391633));
#139473=CARTESIAN_POINT('Ctrl Pts',(7.4330052177926,4.21216499503617,1.00021669058607));
#139474=CARTESIAN_POINT('Ctrl Pts',(7.33562551247557,4.30331728230629,1.56162219693697));
#139475=CARTESIAN_POINT('Ctrl Pts',(7.33646412623779,4.30267205415314,1.55766187196849));
#139476=CARTESIAN_POINT('Ctrl Pts',(7.33730274,4.302026826,1.553701547));
#139477=CARTESIAN_POINT('Ctrl Pts',(7.42143157800001,4.237298226,1.156405971));
#139478=CARTESIAN_POINT('Ctrl Pts',(7.462169301,4.172121859,0.7523492));
#139479=CARTESIAN_POINT('Ctrl Pts',(7.03778333585493,4.30331728230629,1.74131185278812));
#139480=CARTESIAN_POINT('Ctrl Pts',(7.03871911092747,4.30267205415314,1.73751218389406));
#139481=CARTESIAN_POINT('Ctrl Pts',(7.039654886,4.302026826,1.733712515));
#139482=CARTESIAN_POINT('Ctrl Pts',(7.133530843,4.237298226,1.352533785));
#139483=CARTESIAN_POINT('Ctrl Pts',(7.185698963,4.172121859,0.963447153));
#139484=CARTESIAN_POINT('',(7.33730274119938,4.30202682545375,1.55370154999587));
#139485=CARTESIAN_POINT('Origin',(-0.190489594696511,4.16072877780515,-0.0172915305091799));
#139486=CARTESIAN_POINT('',(7.18847881074456,4.30202682438474,1.64370704086378));
#139487=CARTESIAN_POINT('Origin',(-8.23559970219989E-13,4.39277644299978,
-1.08094956596805E-13));
#139488=CARTESIAN_POINT('',(7.43373068909092,4.39169923741036,0.994810553290058));
#139489=CARTESIAN_POINT('Origin',(-0.185853746422783,4.16082470961366,0.0118637316186057));
#139490=CARTESIAN_POINT('Origin',(-0.184631640022924,4.55341981006142,0.00128611064958345));
#139491=CARTESIAN_POINT('Ctrl Pts',(6.953660913,4.172114527,2.810088949));
#139492=CARTESIAN_POINT('Ctrl Pts',(7.088504649,4.22940039,2.476413527));
#139493=CARTESIAN_POINT('Ctrl Pts',(7.190779179,4.285714286,2.131359848));
#139494=CARTESIAN_POINT('Ctrl Pts',(7.20556948400001,4.29385805,2.081460337));
#139495=CARTESIAN_POINT('Ctrl Pts',(7.219665854,4.302026826,2.031360369));
#139496=CARTESIAN_POINT('Ctrl Pts',(6.80734253400001,4.172114527,2.494511501));
#139497=CARTESIAN_POINT('Ctrl Pts',(6.927043104,4.22940039,2.167857251));
#139498=CARTESIAN_POINT('Ctrl Pts',(7.014916327,4.285714286,1.831242452));
#139499=CARTESIAN_POINT('Ctrl Pts',(7.02762400500001,4.29385805,1.782563319));
#139500=CARTESIAN_POINT('Ctrl Pts',(7.039654886,4.302026826,1.733712515));
#139501=CARTESIAN_POINT('',(7.21966585287234,4.30202682641444,2.03136037523548));
#139502=CARTESIAN_POINT('',(7.12966036896448,4.30202682665756,1.88253644592181));
#139503=CARTESIAN_POINT('',(7.04420866668809,4.21216499392905,2.57470857710942));
#139504=CARTESIAN_POINT('Ctrl Pts',(7.21966585263097,4.30202682552109,2.03136037579604));
#139505=CARTESIAN_POINT('Ctrl Pts',(7.21026137828318,4.29657697961046,2.06478485483961));
#139506=CARTESIAN_POINT('Ctrl Pts',(7.20063167850688,4.29113922035365,2.09811949687687));
#139507=CARTESIAN_POINT('Ctrl Pts',(7.1907791788114,4.28571428571329,2.13135984797792));
#139508=CARTESIAN_POINT('Ctrl Pts',(7.14667979468729,4.26143250099391,2.28014229476132));
#139509=CARTESIAN_POINT('Ctrl Pts',(7.09780381684114,4.23689343090752,2.42807628479987));
#139510=CARTESIAN_POINT('Ctrl Pts',(7.04420866918739,4.21216499285688,2.57470857087657));
#139511=CARTESIAN_POINT('Ctrl Pts',(6.80898137272616,4.17289950689835,2.49003467807449));
#139512=CARTESIAN_POINT('Ctrl Pts',(6.84811468974111,4.17977820186027,2.50416154280778));
#139513=CARTESIAN_POINT('Ctrl Pts',(6.88730616221774,4.18648410044305,2.51828808128039));
#139514=CARTESIAN_POINT('Ctrl Pts',(6.96570235636468,4.19956141146743,2.54650695922136));
#139515=CARTESIAN_POINT('Ctrl Pts',(7.00495317822537,4.20594050668545,2.56061589023492));
#139516=CARTESIAN_POINT('Ctrl Pts',(7.04420866410003,4.21216499507508,2.57470858381234));
#139517=CARTESIAN_POINT('Ctrl Pts',(6.82842005352701,4.30331728230629,3.10205498320627));
#139518=CARTESIAN_POINT('Ctrl Pts',(6.83009041376351,4.30267205415314,3.09836752560313));
#139519=CARTESIAN_POINT('Ctrl Pts',(6.831760774,4.302026826,3.094680068));
#139520=CARTESIAN_POINT('Ctrl Pts',(6.999329531,4.237298226,2.724758255));
#139521=CARTESIAN_POINT('Ctrl Pts',(7.125975091,4.172121859,2.338905513));
#139522=CARTESIAN_POINT('Ctrl Pts',(6.49891329666129,4.30331728230629,3.21351633154874));
#139523=CARTESIAN_POINT('Ctrl Pts',(6.50064401033065,4.30267205415314,3.21000666077437));
#139524=CARTESIAN_POINT('Ctrl Pts',(6.502374724,4.302026826,3.20649699));
#139525=CARTESIAN_POINT('Ctrl Pts',(6.675998073,4.237298226,2.854410562));
#139526=CARTESIAN_POINT('Ctrl Pts',(6.810588656,4.172121859,2.485635163));
#139527=CARTESIAN_POINT('',(6.83176077452481,4.30202682545371,3.09468007118652));
#139528=CARTESIAN_POINT('Origin',(-0.182319011662516,4.16072878009169,-0.0578369453895083));
#139529=CARTESIAN_POINT('',(6.66706774467661,4.30202682438463,3.1505885381489));
#139530=CARTESIAN_POINT('Origin',(1.34484437475102E-12,4.39277644299978,
4.93962509784396E-13));
#139531=CARTESIAN_POINT('',(7.04607933373822,4.39169923741341,2.56958479416804));
#139532=CARTESIAN_POINT('Origin',(-0.184058831711233,4.16082468518637,-0.0283666495870066));
#139533=CARTESIAN_POINT('Origin',(-0.180591247415827,4.55341982673589,-0.0384341815324341));
#139534=CARTESIAN_POINT('Ctrl Pts',(6.187002127,4.172114527,4.239222179));
#139535=CARTESIAN_POINT('Ctrl Pts',(6.390423644,4.22940039,3.94233532));
#139536=CARTESIAN_POINT('Ctrl Pts',(6.564483393,4.285714286,3.627334805));
#139537=CARTESIAN_POINT('Ctrl Pts',(6.589654828,4.29385805,3.581781394));
#139538=CARTESIAN_POINT('Ctrl Pts',(6.61419164600001,4.302026826,3.53588304));
#139539=CARTESIAN_POINT('Ctrl Pts',(6.11194441300001,4.172114527,3.89956863));
#139540=CARTESIAN_POINT('Ctrl Pts',(6.299067458,4.22940039,3.606283458));
#139541=CARTESIAN_POINT('Ctrl Pts',(6.457248486,4.285714286,3.296428672));
#139542=CARTESIAN_POINT('Ctrl Pts',(6.48012364,4.29385805,3.251619405));
#139543=CARTESIAN_POINT('Ctrl Pts',(6.50237472400001,4.302026826,3.20649699));
#139544=CARTESIAN_POINT('',(6.61419164333589,4.30202682641444,3.53588304568432));
#139545=CARTESIAN_POINT('',(6.55772409853652,4.30202682665757,3.36954308835721));
#139546=CARTESIAN_POINT('',(6.32603274655909,4.21216499392067,4.02880995941814));
#139547=CARTESIAN_POINT('Ctrl Pts',(6.6141916425897,4.30202682552109,3.53588304601502));
#139548=CARTESIAN_POINT('Ctrl Pts',(6.59782176496394,4.29657697961046,3.56650439473428));
#139549=CARTESIAN_POINT('Ctrl Pts',(6.58125123958368,4.29113922035365,3.59698959050121));
#139550=CARTESIAN_POINT('Ctrl Pts',(6.56448339291723,4.28571428571329,3.62733480452437));
#139551=CARTESIAN_POINT('Ctrl Pts',(6.48943119969881,4.26143250100208,3.76315873656664));
#139552=CARTESIAN_POINT('Ctrl Pts',(6.40989648014607,4.23689343091575,3.897127221554));
#139553=CARTESIAN_POINT('Ctrl Pts',(6.32603275018521,4.21216499285683,4.02880995376847));
#139554=CARTESIAN_POINT('Ctrl Pts',(6.11450732205272,4.17289950712114,3.89554877408609));
#139555=CARTESIAN_POINT('Ctrl Pts',(6.14968886578877,4.1797782021083,3.91775786726618));
#139556=CARTESIAN_POINT('Ctrl Pts',(6.18492727408787,4.18648410045048,3.93997914259056));
#139557=CARTESIAN_POINT('Ctrl Pts',(6.25542438446169,4.19956141148895,3.98439114355122));
#139558=CARTESIAN_POINT('Ctrl Pts',(6.29072454069049,4.20594050666881,4.00660798203398));
#139559=CARTESIAN_POINT('Ctrl Pts',(6.32603274259154,4.21216499504938,4.02880996541136));
#139560=CARTESIAN_POINT('Ctrl Pts',(6.00192526193812,4.30331728230629,4.4974391266339));
#139561=CARTESIAN_POINT('Ctrl Pts',(6.00434926446906,4.30267205415315,4.49419695781695));
#139562=CARTESIAN_POINT('Ctrl Pts',(6.006773267,4.302026826,4.490954789));
#139563=CARTESIAN_POINT('Ctrl Pts',(6.249946615,4.237298226,4.165703872));
#139564=CARTESIAN_POINT('Ctrl Pts',(6.456578206,4.172121859,3.816097204));
#139565=CARTESIAN_POINT('Ctrl Pts',(5.65616129496628,4.30331728230629,4.53546035768119));
#139566=CARTESIAN_POINT('Ctrl Pts',(5.65860602098314,4.30267205415315,4.5324047933406));
#139567=CARTESIAN_POINT('Ctrl Pts',(5.661050747,4.302026826,4.529349229));
#139568=CARTESIAN_POINT('Ctrl Pts',(5.906303053,4.237298226,4.222818274));
#139569=CARTESIAN_POINT('Ctrl Pts',(6.117022792,4.172121859,3.891597635));
#139570=CARTESIAN_POINT('',(6.00677326682245,4.30202682545379,4.49095479222783));
#139571=CARTESIAN_POINT('Origin',(-0.165623166175317,4.16072878917566,-0.0956778885946874));
#139572=CARTESIAN_POINT('',(5.83391200081167,4.30202682438483,4.51015201700465));
#139573=CARTESIAN_POINT('Origin',(-5.31692745386891E-13,4.39277644300067,
-3.68411898210574E-13));
#139574=CARTESIAN_POINT('',(6.32896114034785,4.39169923739958,4.02420810597715));
#139575=CARTESIAN_POINT('Origin',(-0.173657580569582,4.1608246493853,-0.0672706206153839));
#139576=CARTESIAN_POINT('Origin',(-0.168107033907274,4.55341982151689,-0.076357479274628));
#139577=CARTESIAN_POINT('Ctrl Pts',(5.131045997,4.172114527,5.470134091));
#139578=CARTESIAN_POINT('Ctrl Pts',(5.393533531,4.22940039,5.223917895));
#139579=CARTESIAN_POINT('Ctrl Pts',(5.631239659,4.285714286,4.953699618));
#139580=CARTESIAN_POINT('Ctrl Pts',(5.66561523700001,4.29385805,4.914622335));
#139581=CARTESIAN_POINT('Ctrl Pts',(5.69944518700001,4.302026826,4.875071749));
#139582=CARTESIAN_POINT('Ctrl Pts',(5.130758564,4.172114527,5.122286263));
#139583=CARTESIAN_POINT('Ctrl Pts',(5.376554419,4.22940039,4.87608386));
#139584=CARTESIAN_POINT('Ctrl Pts',(5.597646882,4.285714286,4.607477551));
#139585=CARTESIAN_POINT('Ctrl Pts',(5.629619895,4.29385805,4.568633382));
#139586=CARTESIAN_POINT('Ctrl Pts',(5.661050747,4.302026826,4.529349229));
#139587=CARTESIAN_POINT('',(5.69944518326463,4.30202682641445,4.8750717540797));
#139588=CARTESIAN_POINT('',(5.68005599221441,4.30202682665756,4.70048187952442));
#139589=CARTESIAN_POINT('',(5.3120585659177,4.21216499394814,5.29452866556222));
#139590=CARTESIAN_POINT('Ctrl Pts',(5.69944518263236,4.30202682552109,4.87507175436104));
#139591=CARTESIAN_POINT('Ctrl Pts',(5.67687533869791,4.29657697961046,4.90145815332426));
#139592=CARTESIAN_POINT('Ctrl Pts',(5.65413880693874,4.29113922035365,4.92766844913144));
#139593=CARTESIAN_POINT('Ctrl Pts',(5.63123965919007,4.28571428571329,4.95369961753485));
#139594=CARTESIAN_POINT('Ctrl Pts',(5.52874401419247,4.26143250103135,5.07021405837047));
#139595=CARTESIAN_POINT('Ctrl Pts',(5.42226950816182,4.23689343094526,5.18395282076903));
#139596=CARTESIAN_POINT('Ctrl Pts',(5.3120585708442,4.21216499285688,5.29452866078942));
#139597=CARTESIAN_POINT('Ctrl Pts',(5.13412570350878,4.17289950703851,5.11891133959974));
#139598=CARTESIAN_POINT('Ctrl Pts',(5.16371042366419,4.17977820201081,5.14816418808481));
#139599=CARTESIAN_POINT('Ctrl Pts',(5.19334806060398,4.1864841004508,5.17744115868062));
#139600=CARTESIAN_POINT('Ctrl Pts',(5.25264972022252,4.19956141149291,5.23596962626228));
#139601=CARTESIAN_POINT('Ctrl Pts',(5.28234861498335,4.20594050671005,5.26525553759414));
#139602=CARTESIAN_POINT('Ctrl Pts',(5.31205856064242,4.21216499511036,5.29452867066908));
#139603=CARTESIAN_POINT('Ctrl Pts',(4.89478711568802,4.30331728230629,5.68252801464834));
#139604=CARTESIAN_POINT('Ctrl Pts',(4.89785141684401,4.30267205415314,5.67988273482417));
#139605=CARTESIAN_POINT('Ctrl Pts',(4.90091571800001,4.302026826,5.67723745499999));
#139606=CARTESIAN_POINT('Ctrl Pts',(5.208323141,4.237298226,5.41186580500001));
#139607=CARTESIAN_POINT('Ctrl Pts',(5.4852789,4.172121859,5.114852431));
#139608=CARTESIAN_POINT('Ctrl Pts',(4.54893347762908,4.30331728230629,5.64533129824391));
#139609=CARTESIAN_POINT('Ctrl Pts',(4.55197790331453,4.30267205415314,5.64287271512195));
#139610=CARTESIAN_POINT('Ctrl Pts',(4.555022329,4.302026826,5.640414132));
#139611=CARTESIAN_POINT('Ctrl Pts',(4.860435866,4.237298226,5.39377169600001));
#139612=CARTESIAN_POINT('Ctrl Pts',(5.137431742,4.172121859,5.115593328));
#139613=CARTESIAN_POINT('',(4.90091571714228,4.30202682545372,5.67723745811082));
#139614=CARTESIAN_POINT('Origin',(-0.141183175810484,4.16072878338812,-0.129045188906731));
#139615=CARTESIAN_POINT('',(4.72796901573467,4.30202682438463,5.65882579998796));
#139616=CARTESIAN_POINT('Origin',(7.01695646032618E-13,4.39277644300044,
6.59628601740181E-13));
#139617=CARTESIAN_POINT('',(5.31590775787188,4.39169923738042,5.29066391891839));
#139618=CARTESIAN_POINT('Origin',(-0.15513626692275,4.16082473539166,-0.103029040356922));
#139619=CARTESIAN_POINT('Origin',(-0.14776242244722,4.55341983644703,-0.110710578795594));
#139620=CARTESIAN_POINT('Ctrl Pts',(3.83516786,4.172114527,6.445268612));
#139621=CARTESIAN_POINT('Ctrl Pts',(4.144447785,4.22940039,6.261235875));
#139622=CARTESIAN_POINT('Ctrl Pts',(4.434685418,4.285714286,6.048434942));
#139623=CARTESIAN_POINT('Ctrl Pts',(4.476657775,4.29385805,6.01766099800001));
#139624=CARTESIAN_POINT('Ctrl Pts',(4.518199006,4.302026826,5.986307521));
#139625=CARTESIAN_POINT('Ctrl Pts',(3.909664147,4.172114527,6.105491484));
#139626=CARTESIAN_POINT('Ctrl Pts',(4.202639671,4.22940039,5.917883999));
#139627=CARTESIAN_POINT('Ctrl Pts',(4.476305531,4.285714286,5.703085901));
#139628=CARTESIAN_POINT('Ctrl Pts',(4.51588138100001,4.29385805,5.67202313900001));
#139629=CARTESIAN_POINT('Ctrl Pts',(4.555022329,4.302026826,5.640414132));
#139630=CARTESIAN_POINT('',(4.51819900130735,4.30202682641451,5.98630752524338));
#139631=CARTESIAN_POINT('',(4.53661066430174,4.30202682665767,5.81336082899585));
#139632=CARTESIAN_POINT('',(4.04969843050623,4.21216499391419,6.31268109603982));
#139633=CARTESIAN_POINT('Ctrl Pts',(4.51819900073126,4.30202682552109,5.98630752549441));
#139634=CARTESIAN_POINT('Ctrl Pts',(4.49048453128782,4.29657697961046,6.00722517591779));
#139635=CARTESIAN_POINT('Ctrl Pts',(4.46264512820145,4.29113922035365,6.02793500731677));
#139636=CARTESIAN_POINT('Ctrl Pts',(4.43468541808248,4.28571428571326,6.04843494158998));
#139637=CARTESIAN_POINT('Ctrl Pts',(4.30953890349148,4.2614325009866,6.14019180576064));
#139638=CARTESIAN_POINT('Ctrl Pts',(4.18110324017952,4.23689343090015,6.22838254783057));
#139639=CARTESIAN_POINT('Ctrl Pts',(4.04969843616027,4.21216499285689,6.31268109254388));
#139640=CARTESIAN_POINT('Ctrl Pts',(3.91367807290479,4.17289950687043,6.10291929893263));
#139641=CARTESIAN_POINT('Ctrl Pts',(3.93628262107007,4.17977820182286,6.13784807241261));
#139642=CARTESIAN_POINT('Ctrl Pts',(3.9589336638548,4.18648410041305,6.17281178040934));
#139643=CARTESIAN_POINT('Ctrl Pts',(4.00426699324573,4.1995614114377,6.24271998879621));
#139644=CARTESIAN_POINT('Ctrl Pts',(4.02697593910242,4.20594050664488,6.27770559622218));
#139645=CARTESIAN_POINT('Ctrl Pts',(4.04969842444934,4.21216499503999,6.31268109977444));
#139646=CARTESIAN_POINT('Ctrl Pts',(3.5587741640618,4.30331728230629,6.60190820898191));
#139647=CARTESIAN_POINT('Ctrl Pts',(3.5623354805309,4.30267205415314,6.59998350849095));
#139648=CARTESIAN_POINT('Ctrl Pts',(3.565896797,4.302026826,6.598058808));
#139649=CARTESIAN_POINT('Ctrl Pts',(3.923164266,4.237298226,6.404974908));
#139650=CARTESIAN_POINT('Ctrl Pts',(4.257494048,4.172121859,6.174442844));
#139651=CARTESIAN_POINT('Ctrl Pts',(3.22900258618386,4.30331728230629,6.49123282156182));
#139652=CARTESIAN_POINT('Ctrl Pts',(3.23250435759193,4.30267205415314,6.48948618028091));
#139653=CARTESIAN_POINT('Ctrl Pts',(3.236006129,4.302026826,6.487739539));
#139654=CARTESIAN_POINT('Ctrl Pts',(3.587300101,4.237298226,6.312518349));
#139655=CARTESIAN_POINT('Ctrl Pts',(3.917620093,4.172121859,6.100389562));
#139656=CARTESIAN_POINT('',(3.56589679608909,4.30202682545316,6.59805881069389));
#139657=CARTESIAN_POINT('Origin',(-0.110141570649285,4.16072872614212,-0.156378502227356));
#139658=CARTESIAN_POINT('',(3.40095145402154,4.30202682438465,6.54289917816694));
#139659=CARTESIAN_POINT('Origin',(-8.72565908416334E-13,4.392776443,-1.20823490101785E-12));
#139660=CARTESIAN_POINT('',(4.05428843735919,4.3916992373681,6.30973416716977));
#139661=CARTESIAN_POINT('Origin',(-0.129361106999302,4.16082469154354,-0.13397002573184));
#139662=CARTESIAN_POINT('Origin',(-0.120508300879558,4.55341982873688,-0.139886746186956));
#139663=CARTESIAN_POINT('Ctrl Pts',(2.359961536,4.172114527,7.119029537));
#139664=CARTESIAN_POINT('Ctrl Pts',(2.701572267,4.22940039,7.005785424));
#139665=CARTESIAN_POINT('Ctrl Pts',(3.030770215,4.285714286,6.86035217));
#139666=CARTESIAN_POINT('Ctrl Pts',(3.07837677,4.29385805,6.83932052));
#139667=CARTESIAN_POINT('Ctrl Pts',(3.125686861,4.302026826,6.817630208));
#139668=CARTESIAN_POINT('Ctrl Pts',(2.50575818,4.172114527,6.803210709));
#139669=CARTESIAN_POINT('Ctrl Pts',(2.832214162,4.22940039,6.68297046));
#139670=CARTESIAN_POINT('Ctrl Pts',(3.145657109,4.285714286,6.532024292));
#139671=CARTESIAN_POINT('Ctrl Pts',(3.190985273,4.29385805,6.510195399));
#139672=CARTESIAN_POINT('Ctrl Pts',(3.236006129,4.302026826,6.487739539));
#139673=CARTESIAN_POINT('',(3.1256868554126,4.30202682641445,6.81763021082508));
#139674=CARTESIAN_POINT('',(3.18084649134053,4.30202682665757,6.65268487524971));
#139675=CARTESIAN_POINT('',(2.59797889752575,4.21216499390815,7.03565957449181));
#139676=CARTESIAN_POINT('Ctrl Pts',(3.12568685454772,4.30202682552111,6.81763021051357));
#139677=CARTESIAN_POINT('Ctrl Pts',(3.0941236577602,4.29657697961046,6.83210102606678));
#139678=CARTESIAN_POINT('Ctrl Pts',(3.06248312301008,4.29113922035365,6.84634202432006));
#139679=CARTESIAN_POINT('Ctrl Pts',(3.03077021551498,4.28571428571329,6.8603521703151));
#139680=CARTESIAN_POINT('Ctrl Pts',(2.88882454346608,4.26143250097105,6.92306100863517));
#139681=CARTESIAN_POINT('Ctrl Pts',(2.74443323190568,4.23689343088443,6.98158002910692));
#139682=CARTESIAN_POINT('Ctrl Pts',(2.59797890375575,4.21216499285672,7.03565957218225));
#139683=CARTESIAN_POINT('Ctrl Pts',(2.51023120678092,4.17289950702997,6.80156153618877));
#139684=CARTESIAN_POINT('Ctrl Pts',(2.52479861929105,4.17977820199321,6.84053300412659));
#139685=CARTESIAN_POINT('Ctrl Pts',(2.53940392922748,4.18648410044078,6.8795485839286));
#139686=CARTESIAN_POINT('Ctrl Pts',(2.56864919216302,4.19956141145792,6.95756770310241));
#139687=CARTESIAN_POINT('Ctrl Pts',(2.58330634398361,4.20594050663845,6.99661711845852));
#139688=CARTESIAN_POINT('Ctrl Pts',(2.59797889080986,4.21216499502226,7.03565957683809));
#139689=CARTESIAN_POINT('Ctrl Pts',(2.05635688783999,4.30331728230629,7.21259051257531));
#139690=CARTESIAN_POINT('Ctrl Pts',(2.06024869641999,4.30267205415314,7.21147638828766));
#139691=CARTESIAN_POINT('Ctrl Pts',(2.064140505,4.302026826,7.210362264));
#139692=CARTESIAN_POINT('Ctrl Pts',(2.45456259,4.237298226,7.098594504));
#139693=CARTESIAN_POINT('Ctrl Pts',(2.830633507,4.172121859,6.945323171));
#139694=CARTESIAN_POINT('Ctrl Pts',(1.75808712366278,4.30331728230629,7.03361151287165));
#139695=CARTESIAN_POINT('Ctrl Pts',(1.76188250183139,4.30267205415314,7.03265848443582));
#139696=CARTESIAN_POINT('Ctrl Pts',(1.76567788,4.302026826,7.031705456));
#139697=CARTESIAN_POINT('Ctrl Pts',(2.146426169,4.237298226,6.93609866000001));
#139698=CARTESIAN_POINT('Ctrl Pts',(2.514624883,4.172121859,6.79993836));
#139699=CARTESIAN_POINT('',(2.06414050352516,4.30202682545337,7.2103622664337));
#139700=CARTESIAN_POINT('Origin',(-0.073949683909128,4.16072875403252,-0.176399408683935));
#139701=CARTESIAN_POINT('',(1.91490918273179,4.30202682438524,7.12103386262676));
#139702=CARTESIAN_POINT('Origin',(5.20417042793042E-15,4.39277644300089,
1.95156391047391E-14));
#139703=CARTESIAN_POINT('',(2.60309509487783,4.39169923735874,7.03376825908966));
#139704=CARTESIAN_POINT('Origin',(-0.0975371601152519,4.16082466558289,
-0.158646804130117));
#139705=CARTESIAN_POINT('Origin',(-0.0876193823186891,4.55341984404931,
-0.162522029489007));
#139706=CARTESIAN_POINT('Ctrl Pts',(0.774406033,4.172114527,7.45991255300001));
#139707=CARTESIAN_POINT('Ctrl Pts',(1.132374232,4.22940039,7.422752234));
#139708=CARTESIAN_POINT('Ctrl Pts',(1.485139566,4.285714286,7.351486956));
#139709=CARTESIAN_POINT('Ctrl Pts',(1.536154289,4.29385805,7.341181016));
#139710=CARTESIAN_POINT('Ctrl Pts',(1.587021072,4.302026826,7.330168082));
#139711=CARTESIAN_POINT('Ctrl Pts',(0.984685745,4.172114527,7.182819362));
#139712=CARTESIAN_POINT('Ctrl Pts',(1.329357467,4.22940039,7.135568649));
#139713=CARTESIAN_POINT('Ctrl Pts',(1.667921256,4.285714286,7.055532488));
#139714=CARTESIAN_POINT('Ctrl Pts',(1.71688224,4.29385805,7.043958157));
#139715=CARTESIAN_POINT('Ctrl Pts',(1.76567788,4.302026826,7.031705456));
#139716=CARTESIAN_POINT('',(1.58702106594486,4.30202682620655,7.33016808366913));
#139717=CARTESIAN_POINT('',(1.67634947204994,4.30202682665757,7.18093676992212));
#139718=CARTESIAN_POINT('',(1.02478075832104,4.21216499529598,7.42965843030395));
#139719=CARTESIAN_POINT('Ctrl Pts',(1.58702106529163,4.3020268248974,7.33016808322337));
#139720=CARTESIAN_POINT('Ctrl Pts',(1.55308500096568,4.29657697940857,7.33751542487662));
#139721=CARTESIAN_POINT('Ctrl Pts',(1.51912281074809,4.29113922035362,7.34462169677195));
#139722=CARTESIAN_POINT('Ctrl Pts',(1.48513956610293,4.28571428598436,7.35148695569453));
#139723=CARTESIAN_POINT('Ctrl Pts',(1.33303195779561,4.26143250089043,7.38221557329729));
#139724=CARTESIAN_POINT('Ctrl Pts',(1.1794365756078,4.23689343225755,7.40832658749199));
#139725=CARTESIAN_POINT('Ctrl Pts',(1.02478076449991,4.21216499697171,7.42965842910681));
#139726=CARTESIAN_POINT('Ctrl Pts',(0.989408718343246,4.17289950709276,
7.18217031486416));
#139727=CARTESIAN_POINT('Ctrl Pts',(0.995257839240748,4.17977820203178,
7.22336221448962));
#139728=CARTESIAN_POINT('Ctrl Pts',(1.00113448880787,4.18648410043884,7.26460534140605));
#139729=CARTESIAN_POINT('Ctrl Pts',(1.01292420948285,4.19956141142547,7.34708728384108));
#139730=CARTESIAN_POINT('Ctrl Pts',(1.01884421533533,4.20594050661628,7.38837460004229));
#139731=CARTESIAN_POINT('Ctrl Pts',(1.02478075181138,4.21216499499655,7.42965843128517));
#139732=CARTESIAN_POINT('Ctrl Pts',(0.457786649930205,4.30331728230629,
7.4860200997665));
#139733=CARTESIAN_POINT('Ctrl Pts',(0.461826973965103,4.30267205415314,
7.48576864688325));
#139734=CARTESIAN_POINT('Ctrl Pts',(0.465867298,4.302026826,7.485517194));
#139735=CARTESIAN_POINT('Ctrl Pts',(0.871188295,4.237298226,7.460291709));
#139736=CARTESIAN_POINT('Ctrl Pts',(1.271415689,4.172121859,7.391447906));
#139737=CARTESIAN_POINT('Ctrl Pts',(0.20496545941525,4.30331728230629,7.24710634709099));
#139738=CARTESIAN_POINT('Ctrl Pts',(0.208876976707625,4.30267205415314,
7.24699149404549));
#139739=CARTESIAN_POINT('Ctrl Pts',(0.212788494,4.302026826,7.246876641));
#139740=CARTESIAN_POINT('Ctrl Pts',(0.605187736,4.237298226,7.235354706));
#139741=CARTESIAN_POINT('Ctrl Pts',(0.994048608,4.172121859,7.181529598));
#139742=CARTESIAN_POINT('',(0.465867296042565,4.30202682545335,7.48551719606147));
#139743=CARTESIAN_POINT('Origin',(-0.0343001461811986,4.16072877971437,
-0.188172529920452));
#139744=CARTESIAN_POINT('',(0.33932788589549,4.30202682438524,7.36619691796547));
#139745=CARTESIAN_POINT('Origin',(-7.7005459300783E-14,4.392776443,-7.73686670285656E-13));
#139746=CARTESIAN_POINT('',(1.03018391903457,4.39169923738309,7.42891116439695));
#139747=CARTESIAN_POINT('Origin',(-0.0611523990539982,4.16082467447941,
-0.175905147910012));
#139748=CARTESIAN_POINT('Origin',(-0.0506334197676744,4.55341979579773,
-0.177557643365398));
#139749=CARTESIAN_POINT('Origin',(-8.63194335887912E-14,4.39277644299978,
1.0547118733939E-12));
#139750=CARTESIAN_POINT('',(-0.0258520642580682,4.30202682641445,7.49995544522258));
#139751=CARTESIAN_POINT('Ctrl Pts',(-0.0258520649115978,4.30202682552111,
7.49995544458365));
#139752=CARTESIAN_POINT('Ctrl Pts',(-0.0605741846835186,4.29657697961046,
7.49983575874007));
#139753=CARTESIAN_POINT('Ctrl Pts',(-0.0952699962294244,4.29113922035365,
7.49947502299388));
#139754=CARTESIAN_POINT('Ctrl Pts',(-0.129934559142506,4.28571428571329,
7.49887438288844));
#139755=CARTESIAN_POINT('Ctrl Pts',(-0.28509171907091,4.26143250106465,
7.49618594244476));
#139756=CARTESIAN_POINT('Ctrl Pts',(-0.440709222886184,4.23689343175884,
7.48866802895951));
#139757=CARTESIAN_POINT('Ctrl Pts',(-0.596334981605774,4.21216499520884,
7.47625471674912));
#139758=CARTESIAN_POINT('',(-0.590897510512571,4.39169923729323,7.47668644066963));
#139759=CARTESIAN_POINT('Origin',(-0.0219082601953907,4.1608246528612,-0.18493894311418));
#139760=CARTESIAN_POINT('Origin',(-0.0112799649723951,4.55341977946789,
-0.184291312800935));
#139761=CARTESIAN_POINT('Ctrl Pts',(-0.847359835,4.172114527,7.451978349));
#139762=CARTESIAN_POINT('Ctrl Pts',(-0.489772364,4.22940039,7.492639398));
#139763=CARTESIAN_POINT('Ctrl Pts',(-0.129934559,4.285714286,7.498874383));
#139764=CARTESIAN_POINT('Ctrl Pts',(-0.07789706,4.29385805,7.499776047));
#139765=CARTESIAN_POINT('Ctrl Pts',(-0.025852058,4.302026826,7.499955445));
#139766=CARTESIAN_POINT('Ctrl Pts',(-0.582429501,4.172114527,7.226567365));
#139767=CARTESIAN_POINT('Ctrl Pts',(-0.235658505,4.22940039,7.25451558));
#139768=CARTESIAN_POINT('Ctrl Pts',(0.112195259,4.285714286,7.249131826));
#139769=CARTESIAN_POINT('Ctrl Pts',(0.162499702,4.29385805,7.248353261));
#139770=CARTESIAN_POINT('Ctrl Pts',(0.212788494,4.302026826,7.246876641));
#139771=CARTESIAN_POINT('',(0.0946614167047613,4.30202682665757,7.37215064903207));
#139772=CARTESIAN_POINT('Ctrl Pts',(-0.0379316651699341,1.456406735,7.50043718252163));
#139773=CARTESIAN_POINT('Ctrl Pts',(0.373468759383251,1.522118786,7.50251774175917));
#139774=CARTESIAN_POINT('Ctrl Pts',(0.782628730039567,1.586734015,7.45959040487358));
#139775=CARTESIAN_POINT('Ctrl Pts',(0.796789298954691,1.58897027579979,
7.4581047377607));
#139776=CARTESIAN_POINT('Ctrl Pts',(0.810949867869816,1.59120653659958,
7.45661907064781));
#139777=CARTESIAN_POINT('Ctrl Pts',(0.201601146,1.456406735,7.247196491));
#139778=CARTESIAN_POINT('Ctrl Pts',(0.59911127,1.522118786,7.236138629));
#139779=CARTESIAN_POINT('Ctrl Pts',(0.993027301999999,1.586734015,7.18167089));
#139780=CARTESIAN_POINT('Ctrl Pts',(1.00666029524947,1.58897027579979,7.17978582247854));
#139781=CARTESIAN_POINT('Ctrl Pts',(1.02029328849892,1.59120653659958,7.17790075495718));
#139782=CARTESIAN_POINT('',(0.206355417658743,1.45719264060538,7.24706267593716));
#139783=CARTESIAN_POINT('Origin',(0.0140775383922631,1.3393957313777,-0.192312383039513));
#139784=CARTESIAN_POINT('Ctrl Pts',(0.206355413361966,1.45719264074914,
7.24706267701225));
#139785=CARTESIAN_POINT('Ctrl Pts',(0.207635378906658,1.46408307495124,
7.28864821236279));
#139786=CARTESIAN_POINT('Ctrl Pts',(0.208937534794803,1.47080219913258,
7.33028717574197));
#139787=CARTESIAN_POINT('Ctrl Pts',(0.211579281208753,1.48390865064158,
7.41356511687401));
#139788=CARTESIAN_POINT('Ctrl Pts',(0.212920408593059,1.49030358392773,
7.45525246629562));
#139789=CARTESIAN_POINT('Ctrl Pts',(0.21427864176539,1.49654505838725,7.49693835245978));
#139790=CARTESIAN_POINT('Ctrl Pts',(1.270364528,1.586734015,7.391628641));
#139791=CARTESIAN_POINT('Ctrl Pts',(1.67128584,1.521690237,7.322724176));
#139792=CARTESIAN_POINT('Ctrl Pts',(2.062402258,1.456414446,7.210859652));
#139793=CARTESIAN_POINT('Ctrl Pts',(0.993027302,1.586734015,7.18167089));
#139794=CARTESIAN_POINT('Ctrl Pts',(1.382560524,1.521690237,7.127809173));
#139795=CARTESIAN_POINT('Ctrl Pts',(1.763982709,1.456414446,7.032130901));
#139796=CARTESIAN_POINT('',(1.7594351956975,1.45719264061351,7.03327006337353));
#139797=CARTESIAN_POINT('Origin',(-0.0443700637135178,1.48214301195865,
-0.194387020949511));
#139798=CARTESIAN_POINT('Ctrl Pts',(1.82088906445054,1.49654505841197,7.27560052582954));
#139799=CARTESIAN_POINT('Ctrl Pts',(1.81060137241627,1.49030359595976,7.23518129027469));
#139800=CARTESIAN_POINT('Ctrl Pts',(1.80033004124374,1.48390865652201,7.19475682903767));
#139801=CARTESIAN_POINT('Ctrl Pts',(1.77984774251394,1.47080219290275,7.11399370280525));
#139802=CARTESIAN_POINT('Ctrl Pts',(1.76962488919469,1.4640830719819,7.07360818143262));
#139803=CARTESIAN_POINT('Ctrl Pts',(1.75943519192526,1.45719264079878,7.03327006541419));
#139804=CARTESIAN_POINT('Ctrl Pts',(1.57532743863952,1.456406735,7.33323531634185));
#139805=CARTESIAN_POINT('Ctrl Pts',(1.97755680933516,1.522118786,7.24682830281802));
#139806=CARTESIAN_POINT('Ctrl Pts',(2.36792273908022,1.586734015,7.11694728376987));
#139807=CARTESIAN_POINT('Ctrl Pts',(2.38143286751847,1.58897027584229,7.11245224689466));
#139808=CARTESIAN_POINT('Ctrl Pts',(2.39494299595673,1.59120653668464,7.10795721001934));
#139809=CARTESIAN_POINT('Ctrl Pts',(1.754820843,1.456406735,7.034422777));
#139810=CARTESIAN_POINT('Ctrl Pts',(2.140660288,1.522118786,6.938170516));
#139811=CARTESIAN_POINT('Ctrl Pts',(2.513657828,1.586734015,6.8002959));
#139812=CARTESIAN_POINT('Ctrl Pts',(2.5265668558853,1.58897027584229,6.79552421367031));
#139813=CARTESIAN_POINT('Ctrl Pts',(2.53947588377066,1.59120653668465,6.79075252734073));
#139814=CARTESIAN_POINT('Origin',(-0.0275930671526198,1.3393957380865,-0.190842484788214));
#139815=CARTESIAN_POINT('Ctrl Pts',(2.829645774,1.586734015,6.94572564900001));
#139816=CARTESIAN_POINT('Ctrl Pts',(3.206381346,1.521690237,6.792245902));
#139817=CARTESIAN_POINT('Ctrl Pts',(3.564306113,1.456414446,6.59891824));
#139818=CARTESIAN_POINT('Ctrl Pts',(2.513657828,1.586734015,6.80029590000001));
#139819=CARTESIAN_POINT('Ctrl Pts',(2.882505303,1.521690237,6.663955312));
#139820=CARTESIAN_POINT('Ctrl Pts',(3.234442049,1.456414446,6.488519448));
#139821=CARTESIAN_POINT('',(3.23024574016728,1.45719264061225,6.4906095589037));
#139822=CARTESIAN_POINT('Origin',(-0.0851200586044626,1.4821430323664,-0.180303803708292));
#139823=CARTESIAN_POINT('Ctrl Pts',(3.34235673751931,1.49654505837742,6.71406370518684));
#139824=CARTESIAN_POINT('Ctrl Pts',(3.32362058915717,1.49030358391892,6.67680092687681));
#139825=CARTESIAN_POINT('Ctrl Pts',(3.30489935139105,1.48390865070044,6.63952963836113));
#139826=CARTESIAN_POINT('Ctrl Pts',(3.26753424118067,1.47080218999584,6.56505781410445));
#139827=CARTESIAN_POINT('Ctrl Pts',(3.248868703834,1.46408307057618,6.52781410369618));
#139828=CARTESIAN_POINT('Ctrl Pts',(3.23024573750669,1.45719264080038,6.49060956132151));
#139829=CARTESIAN_POINT('Ctrl Pts',(3.11492598304595,1.456406735,6.82313951611896));
#139830=CARTESIAN_POINT('Ctrl Pts',(3.48917650019526,1.522118786,6.65228522632019));
#139831=CARTESIAN_POINT('Ctrl Pts',(3.84249531148225,1.586734015,6.4415236179946));
#139832=CARTESIAN_POINT('Ctrl Pts',(3.85472328050915,1.58897027583195,6.43422939437467));
#139833=CARTESIAN_POINT('Ctrl Pts',(3.86695124953596,1.59120653666397,6.4269351707547));
#139834=CARTESIAN_POINT('Ctrl Pts',(3.225987068,1.456406735,6.492727273));
#139835=CARTESIAN_POINT('Ctrl Pts',(3.58211441,1.522118786,6.31578126));
#139836=CARTESIAN_POINT('Ctrl Pts',(3.916752508,1.586734015,6.100946631));
#139837=CARTESIAN_POINT('Ctrl Pts',(3.92833395842618,1.58897027583195,6.09351144468842));
#139838=CARTESIAN_POINT('Ctrl Pts',(3.93991540885235,1.59120653666397,6.08607625837668));
#139839=CARTESIAN_POINT('Origin',(-0.0679733892134116,1.33939578365377,
-0.18044889177114));
#139840=CARTESIAN_POINT('Ctrl Pts',(4.256615929,1.586734015,6.175048246));
#139841=CARTESIAN_POINT('Ctrl Pts',(4.591550023,1.521690237,5.94416975800001));
#139842=CARTESIAN_POINT('Ctrl Pts',(4.899546976,1.456414446,5.678418744));
#139843=CARTESIAN_POINT('Ctrl Pts',(3.916752508,1.586734015,6.10094663100001));
#139844=CARTESIAN_POINT('Ctrl Pts',(4.247667337,1.521690237,5.888502306));
#139845=CARTESIAN_POINT('Ctrl Pts',(4.553662473,1.456414446,5.641512038));
#139846=CARTESIAN_POINT('',(4.55001358390391,1.45719264061043,5.64445536527957));
#139847=CARTESIAN_POINT('Origin',(-0.121890082462435,1.48214305403045,-0.157790240855409));
#139848=CARTESIAN_POINT('Ctrl Pts',(4.70753952467976,1.49654505838546,5.83858472753936));
#139849=CARTESIAN_POINT('Ctrl Pts',(4.68123102122198,1.49030358392642,5.80622085031352));
#139850=CARTESIAN_POINT('Ctrl Pts',(4.65493525026563,1.4839086506962,5.77384545647786));
#139851=CARTESIAN_POINT('Ctrl Pts',(4.60243447779945,1.47080219076287,5.70914714015477));
#139852=CARTESIAN_POINT('Ctrl Pts',(4.57619903173408,1.46408307092509,5.67678670369149));
#139853=CARTESIAN_POINT('Ctrl Pts',(4.55001358156978,1.45719264075695,5.64445536838016));
#139854=CARTESIAN_POINT('Ctrl Pts',(4.50887404986767,1.456406735,5.99400129611256));
#139855=CARTESIAN_POINT('Ctrl Pts',(4.8376461759817,1.522118786,5.74668868624035));
#139856=CARTESIAN_POINT('Ctrl Pts',(5.13739707470347,1.586734015,5.46490146661415));
#139857=CARTESIAN_POINT('Ctrl Pts',(5.14777111805187,1.58897027580677,5.45514912610781));
#139858=CARTESIAN_POINT('Ctrl Pts',(5.15814516140012,1.59120653661362,5.44539678560135));
#139859=CARTESIAN_POINT('Ctrl Pts',(4.546309723,1.456406735,5.647439057));
#139860=CARTESIAN_POINT('Ctrl Pts',(4.856072844,1.522118786,5.39807309299999));
#139861=CARTESIAN_POINT('Ctrl Pts',(5.136704194,1.586734015,5.116323878));
#139862=CARTESIAN_POINT('Ctrl Pts',(5.14641653115139,1.58897027580677,5.10657285279125));
#139863=CARTESIAN_POINT('Ctrl Pts',(5.15612886830264,1.59120653661362,5.0968218275825));
#139864=CARTESIAN_POINT('Origin',(-0.105175429545894,1.33939576646129,-0.161617879589773));
#139865=CARTESIAN_POINT('Ctrl Pts',(5.484551453,1.586734015,5.115632449));
#139866=CARTESIAN_POINT('Ctrl Pts',(5.762022925,1.521690237,4.818150842));
#139867=CARTESIAN_POINT('Ctrl Pts',(6.005690467,1.456414446,4.492402699));
#139868=CARTESIAN_POINT('Ctrl Pts',(5.136704194,1.586734015,5.11632387800001));
#139869=CARTESIAN_POINT('Ctrl Pts',(5.414213168,1.521690237,4.837709477));
#139870=CARTESIAN_POINT('Ctrl Pts',(5.659958701,1.456414446,4.530713796));
#139871=CARTESIAN_POINT('',(5.65702784900627,1.4571926405954,4.53437271261321));
#139872=CARTESIAN_POINT('Origin',(-0.152960641359311,1.48214303826057,-0.127898470071886));
#139873=CARTESIAN_POINT('Ctrl Pts',(5.85260299563806,1.49654505844387,4.69010001717245));
#139874=CARTESIAN_POINT('Ctrl Pts',(5.81995229347557,1.49030358399253,4.66414834014743));
#139875=CARTESIAN_POINT('Ctrl Pts',(5.7873115502117,1.48390865073091,4.6381826785139));
#139876=CARTESIAN_POINT('Ctrl Pts',(5.72213000906081,1.47080219440202,4.58628310167367));
#139877=CARTESIAN_POINT('Ctrl Pts',(5.68955138599843,1.46408307265874,4.56031907194432));
#139878=CARTESIAN_POINT('Ctrl Pts',(5.65702784741049,1.45719264071491,4.53437271658464));
#139879=CARTESIAN_POINT('Ctrl Pts',(5.69199217717728,1.456406735,4.88459023813095));
#139880=CARTESIAN_POINT('Ctrl Pts',(5.95991289298511,1.522118786,4.57238337002368));
#139881=CARTESIAN_POINT('Ctrl Pts',(6.192079860037,1.586734015,4.23274659681978));
#139882=CARTESIAN_POINT('Ctrl Pts',(6.2001148988587,1.58897027573975,4.22099214831824));
#139883=CARTESIAN_POINT('Ctrl Pts',(6.20814993768041,1.59120653647956,4.20923769981674));
#139884=CARTESIAN_POINT('Ctrl Pts',(5.654051988,1.456406735,4.538082868));
#139885=CARTESIAN_POINT('Ctrl Pts',(5.902966708,1.522118786,4.227957027));
#139886=CARTESIAN_POINT('Ctrl Pts',(6.116469301,1.586734015,3.892467507));
#139887=CARTESIAN_POINT('Ctrl Pts',(6.12385838673028,1.58897027573975,3.88085659028905));
#139888=CARTESIAN_POINT('Ctrl Pts',(6.13124747246068,1.59120653647956,3.86924567357812));
#139889=CARTESIAN_POINT('Origin',(-0.13745956902366,1.33939578570686,-0.135229751280372));
#139890=CARTESIAN_POINT('Ctrl Pts',(6.456035448,1.586734015,3.817015365));
#139891=CARTESIAN_POINT('Ctrl Pts',(6.663070038,1.521690237,3.466840548));
#139892=CARTESIAN_POINT('Ctrl Pts',(6.831014547,1.456414446,3.096326897));
#139893=CARTESIAN_POINT('Ctrl Pts',(6.116469301,1.586734015,3.892467507));
#139894=CARTESIAN_POINT('Ctrl Pts',(6.32759640899999,1.521690237,3.560710729));
#139895=CARTESIAN_POINT('Ctrl Pts',(6.501601551,1.456414446,3.208064411));
#139896=CARTESIAN_POINT('',(6.49952578032314,1.45719264059455,3.21226783095441));
#139897=CARTESIAN_POINT('Origin',(-0.176878902021876,1.48214302079141,-0.0920262527007942));
#139898=CARTESIAN_POINT('Ctrl Pts',(6.72400525554584,1.4965450583912,3.32231144235511));
#139899=CARTESIAN_POINT('Ctrl Pts',(6.68653913777695,1.49030359603181,3.30398547236691));
#139900=CARTESIAN_POINT('Ctrl Pts',(6.64907962791025,1.48390865650943,3.28564364915465));
#139901=CARTESIAN_POINT('Ctrl Pts',(6.57426505880495,1.4708021894492,3.24896952995088));
#139902=CARTESIAN_POINT('Ctrl Pts',(6.5368666223405,1.46408307028397,3.23061597316369));
#139903=CARTESIAN_POINT('Ctrl Pts',(6.49952577957866,1.45719264073368,3.21226783479966));
#139904=CARTESIAN_POINT('Ctrl Pts',(6.60895907756974,1.456406735,3.54678116859748));
#139905=CARTESIAN_POINT('Ctrl Pts',(6.80350070809704,1.522118786,3.1842784891296));
#139906=CARTESIAN_POINT('Ctrl Pts',(6.95722787297183,1.586734015,2.80267320064594));
#139907=CARTESIAN_POINT('Ctrl Pts',(6.96254819814243,1.58897027577753,2.78946626859066));
#139908=CARTESIAN_POINT('Ctrl Pts',(6.96786852331302,1.59120653655514,2.77625933653536));
#139909=CARTESIAN_POINT('Ctrl Pts',(6.497417067,1.456406735,3.216530967));
#139910=CARTESIAN_POINT('Ctrl Pts',(6.67384440999999,1.522118786,2.860146389));
#139911=CARTESIAN_POINT('Ctrl Pts',(6.810235101,1.586734015,2.486603681));
#139912=CARTESIAN_POINT('Ctrl Pts',(6.81495543020762,1.58897027577753,2.47367578583401));
#139913=CARTESIAN_POINT('Ctrl Pts',(6.81967575941525,1.59120653655514,2.46074789066802));
#139914=CARTESIAN_POINT('Origin',(-0.163316158578842,1.33939575347006,-0.102518366935395));
#139915=CARTESIAN_POINT('Ctrl Pts',(7.12564240000001,1.586734015,2.339918885));
#139916=CARTESIAN_POINT('Ctrl Pts',(7.252559402,1.521690237,1.953424644));
#139917=CARTESIAN_POINT('Ctrl Pts',(7.336927979,1.456414446,1.555470291));
#139918=CARTESIAN_POINT('Ctrl Pts',(6.81023510100001,1.586734015,2.486603681));
#139919=CARTESIAN_POINT('Ctrl Pts',(6.945108274,1.521690237,2.117217106));
#139920=CARTESIAN_POINT('Ctrl Pts',(7.039236739,1.456414446,1.7354095));
#139921=CARTESIAN_POINT('',(7.03811310899877,1.45719264060774,1.73996087620211));
#139922=CARTESIAN_POINT('Origin',(-0.192526489986935,1.48214308462136,-0.0518510129485178));
#139923=CARTESIAN_POINT('Ctrl Pts',(7.28100050240532,1.49654505835033,1.79917527769442));
#139924=CARTESIAN_POINT('Ctrl Pts',(7.24047070142308,1.4903035839255,1.78933184746777));
#139925=CARTESIAN_POINT('Ctrl Pts',(7.1999440667875,1.48390865067248,1.77947154348188));
#139926=CARTESIAN_POINT('Ctrl Pts',(7.11899482593458,1.47080219282059,1.75973777943903));
#139927=CARTESIAN_POINT('Ctrl Pts',(7.07852526065664,1.46408307191996,1.74985287418798));
#139928=CARTESIAN_POINT('Ctrl Pts',(7.03811310915023,1.45719264076508,1.73996088015336));
#139929=CARTESIAN_POINT('Ctrl Pts',(7.21689839543718,1.456406735,2.04312855315931));
#139930=CARTESIAN_POINT('Ctrl Pts',(7.32896439106467,1.522118786,1.6472802857093));
#139931=CARTESIAN_POINT('Ctrl Pts',(7.39706364334694,1.586734015,1.24154991981414));
#139932=CARTESIAN_POINT('Ctrl Pts',(7.39942048232618,1.58897027582894,1.22750804550049));
#139933=CARTESIAN_POINT('Ctrl Pts',(7.40177732130554,1.59120653665793,1.21346617118682));
#139934=CARTESIAN_POINT('Ctrl Pts',(7.036970144,1.456406735,1.744577653));
#139935=CARTESIAN_POINT('Ctrl Pts',(7.132660565,1.522118786,1.358598485));
#139936=CARTESIAN_POINT('Ctrl Pts',(7.185561877,1.586734015,0.964469032));
#139937=CARTESIAN_POINT('Ctrl Pts',(7.187392732259,1.58897027582894,0.950828652310581));
#139938=CARTESIAN_POINT('Ctrl Pts',(7.18922358751792,1.59120653665794,0.937188272621161));
#139939=CARTESIAN_POINT('Origin',(-0.181536210942589,1.33939575825133,-0.0650133800666799));
#139940=CARTESIAN_POINT('Ctrl Pts',(7.462062233,1.586734015,0.753410398000001));
#139941=CARTESIAN_POINT('Ctrl Pts',(7.502927149,1.521690237,0.348668774));
#139942=CARTESIAN_POINT('Ctrl Pts',(7.49977481399999,1.456414446,-0.058118378));
#139943=CARTESIAN_POINT('Ctrl Pts',(7.18556187700001,1.586734015,0.964469032000001));
#139944=CARTESIAN_POINT('Ctrl Pts',(7.237874596,1.521690237,0.574724763));
#139945=CARTESIAN_POINT('Ctrl Pts',(7.24772504,1.456414446,0.18160877));
#139946=CARTESIAN_POINT('',(7.24760609128638,1.45719264059485,0.186295284537503));
#139947=CARTESIAN_POINT('Origin',(-0.199171610313214,1.48214301715221,-0.00925123469859398));
#139948=CARTESIAN_POINT('Ctrl Pts',(7.49754425842133,1.49654505839625,0.191911676403582));
#139949=CARTESIAN_POINT('Ctrl Pts',(7.45584597507916,1.49030358395697,0.191011089299526));
#139950=CARTESIAN_POINT('Ctrl Pts',(7.41414715678101,1.48390865070444,0.19009334226442));
#139951=CARTESIAN_POINT('Ctrl Pts',(7.33084828706449,1.47080219265943,0.188222636638891));
#139952=CARTESIAN_POINT('Ctrl Pts',(7.28919991587746,1.46408307184296,0.187268595286479));
#139953=CARTESIAN_POINT('Ctrl Pts',(7.247606092197,1.4571926407666,0.18629528861405));
#139954=CARTESIAN_POINT('Ctrl Pts',(7.48710214575945,1.456406735,0.443644859291493));
#139955=CARTESIAN_POINT('Ctrl Pts',(7.51143615240203,1.522118786,0.0329758636742104));
#139956=CARTESIAN_POINT('Ctrl Pts',(7.49070876024206,1.586734015,-0.377890955082889));
#139957=CARTESIAN_POINT('Ctrl Pts',(7.49039304717479,1.58771821368654,-0.384149148230609));
#139958=CARTESIAN_POINT('Ctrl Pts',(7.49007733410756,1.58870241237309,-0.390407341378328));
#139959=CARTESIAN_POINT('Ctrl Pts',(7.247482319,1.456406735,0.191049828));
#139960=CARTESIAN_POINT('Ctrl Pts',(7.257961439,1.522118786,-0.206475974));
#139961=CARTESIAN_POINT('Ctrl Pts',(7.224899766,1.586734015,-0.602763118));
#139962=CARTESIAN_POINT('Ctrl Pts',(7.22439618107668,1.58771821368654,-0.60879923816325));
#139963=CARTESIAN_POINT('Ctrl Pts',(7.22389259615334,1.58870241237309,-0.6148353583265));
#139964=CARTESIAN_POINT('Origin',(-0.191268234113869,1.33939575786211,-0.0244684761353829));
#139965=CARTESIAN_POINT('Ctrl Pts',(7.44956433,1.586734015,-0.868326722));
#139966=CARTESIAN_POINT('Ctrl Pts',(7.402466362,1.521690237,-1.272390461));
#139967=CARTESIAN_POINT('Ctrl Pts',(7.311940513,1.456414446,-1.668989496));
#139968=CARTESIAN_POINT('Ctrl Pts',(7.224899766,1.586734015,-0.602763118000001));
#139969=CARTESIAN_POINT('Ctrl Pts',(7.192205945,1.521690237,-0.994641069999999));
#139970=CARTESIAN_POINT('Ctrl Pts',(7.117317773,1.456414446,-1.380683784));
#139971=CARTESIAN_POINT('',(7.11820906753265,1.4571926405863,-1.37608126762224));
#139972=CARTESIAN_POINT('Origin',(-0.19650394698959,1.48214304210119,0.0337810818111164));
#139973=CARTESIAN_POINT('Ctrl Pts',(7.36351117761109,1.49654505842827,-1.4243255016041));
#139974=CARTESIAN_POINT('Ctrl Pts',(7.32259417719388,1.490303583954,-1.41624113518447));
#139975=CARTESIAN_POINT('Ctrl Pts',(7.28167296572904,1.48390865070893,-1.40817341256504));
#139976=CARTESIAN_POINT('Ctrl Pts',(7.19991942750816,1.47080219210175,-1.39209358688636));
#139977=CARTESIAN_POINT('Ctrl Pts',(7.15903968301798,1.46408307152146,-1.38407215495896));
#139978=CARTESIAN_POINT('Ctrl Pts',(7.11820906898563,1.45719264066128,-1.37608126395452));
#139979=CARTESIAN_POINT('Ctrl Pts',(7.40776700316167,1.456406735,-1.17600372880381));
#139980=CARTESIAN_POINT('Ctrl Pts',(7.34326297149683,1.522118786,-1.58232117638735));
#139981=CARTESIAN_POINT('Ctrl Pts',(7.23470641998929,1.586734015,-1.97914621804622));
#139982=CARTESIAN_POINT('Ctrl Pts',(7.23094939922131,1.58897027576831,-1.99287988867284));
#139983=CARTESIAN_POINT('Ctrl Pts',(7.22719237845333,1.59120653653669,-2.00661355929947));
#139984=CARTESIAN_POINT('Ctrl Pts',(7.119110275,1.456406735,-1.371411276));
#139985=CARTESIAN_POINT('Ctrl Pts',(7.043888103,1.522118786,-1.761895846));
#139986=CARTESIAN_POINT('Ctrl Pts',(6.926409371,1.586734015,-2.141810735));
#139987=CARTESIAN_POINT('Ctrl Pts',(6.92234356354949,1.58897027576831,-2.15495916416633));
#139988=CARTESIAN_POINT('Ctrl Pts',(6.91827775609913,1.59120653653669,-2.16810759333264));
#139989=CARTESIAN_POINT('Origin',(-0.192056303861984,1.33939579070899,0.0172205636933778));
#139990=CARTESIAN_POINT('Ctrl Pts',(7.088733078,1.586734015,-2.449461849));
#139991=CARTESIAN_POINT('Ctrl Pts',(6.955874475,1.521690237,-2.833954131));
#139992=CARTESIAN_POINT('Ctrl Pts',(6.782208,1.456414446,-3.20182052));
#139993=CARTESIAN_POINT('Ctrl Pts',(6.92640937100001,1.586734015,-2.141810735));
#139994=CARTESIAN_POINT('Ctrl Pts',(6.810237738,1.521690237,-2.517498593));
#139995=CARTESIAN_POINT('Ctrl Pts',(6.654112638,1.456414446,-2.8784171));
#139996=CARTESIAN_POINT('',(6.65597249932013,1.45719264060419,-2.8741137892278));
#139997=CARTESIAN_POINT('Origin',(-0.184647872090671,1.48214305780332,0.0752338312691325));
#139998=CARTESIAN_POINT('Ctrl Pts',(6.88516849829515,1.4965450584155,-2.97396280252883));
#139999=CARTESIAN_POINT('Ctrl Pts',(6.84694601453562,1.49030358397952,-2.95727149861205));
#140000=CARTESIAN_POINT('Ctrl Pts',(6.80871583992957,1.48390865071542,-2.94059554396094));
#140001=CARTESIAN_POINT('Ctrl Pts',(6.73233034632222,1.47080219300501,-2.90731706378751));
#140002=CARTESIAN_POINT('Ctrl Pts',(6.69413071574009,1.46408307201041,-2.8906952306549));
#140003=CARTESIAN_POINT('Ctrl Pts',(6.65597250201484,1.457192640761,-2.87411378614891));
#140004=CARTESIAN_POINT('Ctrl Pts',(6.98177148812184,1.456406735,-2.74096034957496));
#140005=CARTESIAN_POINT('Ctrl Pts',(6.83142928431654,1.522118786,-3.12391186004801));
#140006=CARTESIAN_POINT('Ctrl Pts',(6.64010507143633,1.586734015,-3.48812290292871));
#140007=CARTESIAN_POINT('Ctrl Pts',(6.63348355470157,1.58897027571003,-3.50072783922566));
#140008=CARTESIAN_POINT('Ctrl Pts',(6.62686203796677,1.59120653642013,-3.51333277552261));
#140009=CARTESIAN_POINT('Ctrl Pts',(6.657856548,1.456406735,-2.869746712));
#140010=CARTESIAN_POINT('Ctrl Pts',(6.500450388,1.522118786,-3.234931426));
#140011=CARTESIAN_POINT('Ctrl Pts',(6.304047773,1.586734015,-3.580709661));
#140012=CARTESIAN_POINT('Ctrl Pts',(6.29725049845539,1.58897027571003,-3.59267665845998));
#140013=CARTESIAN_POINT('Ctrl Pts',(6.29045322391093,1.59120653642013,-3.60464365591992));
#140014=CARTESIAN_POINT('Origin',(-0.183864365343379,1.33939572752096,0.0581044355765459));
#140015=CARTESIAN_POINT('Ctrl Pts',(6.396440546,1.586734015,-3.916062862));
#140016=CARTESIAN_POINT('Ctrl Pts',(6.184033628,1.521690237,-4.263005256));
#140017=CARTESIAN_POINT('Ctrl Pts',(5.93534698,1.456414446,-4.584937975));
#140018=CARTESIAN_POINT('Ctrl Pts',(6.304047773,1.586734015,-3.580709661));
#140019=CARTESIAN_POINT('Ctrl Pts',(6.109830384,1.521690237,-3.922640679));
#140020=CARTESIAN_POINT('Ctrl Pts',(5.879768591,1.456414446,-4.24155883));
#140021=CARTESIAN_POINT('',(5.88251005465644,1.45719264060703,-4.23775594375922));
#140022=CARTESIAN_POINT('Origin',(-0.16415770266568,1.48214305229595,0.113168649877636));
#140023=CARTESIAN_POINT('Ctrl Pts',(6.08488299206125,1.49654505834768,-4.38454090746793));
#140024=CARTESIAN_POINT('Ctrl Pts',(6.05114226559013,1.4903035838881,-4.36002313261337));
#140025=CARTESIAN_POINT('Ctrl Pts',(6.01739072882777,1.4839086506801,-4.3355186951666));
#140026=CARTESIAN_POINT('Ctrl Pts',(5.94994497315982,1.47080219260878,-4.28659762264575));
#140027=CARTESIAN_POINT('Ctrl Pts',(5.91621163238358,1.46408307180186,-4.26215260797914));
#140028=CARTESIAN_POINT('Ctrl Pts',(5.88251005761056,1.45719264073823,-4.23775594102181));
#140029=CARTESIAN_POINT('Ctrl Pts',(6.22931609688172,1.456406735,-4.17775270925097));
#140030=CARTESIAN_POINT('Ctrl Pts',(6.00016555589557,1.522118786,-4.51943189804365));
#140031=CARTESIAN_POINT('Ctrl Pts',(5.73501978812084,1.586734015,-4.83399883832595));
#140032=CARTESIAN_POINT('Ctrl Pts',(5.72584338958945,1.58897027582164,-4.84488564837412));
#140033=CARTESIAN_POINT('Ctrl Pts',(5.71666699105796,1.59120653664335,-4.85577245842213));
#140034=CARTESIAN_POINT('Ctrl Pts',(5.885288847,1.456406735,-4.233895981));
#140035=CARTESIAN_POINT('Ctrl Pts',(5.65305883699999,1.522118786,-4.556705209));
#140036=CARTESIAN_POINT('Ctrl Pts',(5.386915907,1.586734015,-4.852178584));
#140037=CARTESIAN_POINT('Ctrl Pts',(5.37770499779902,1.58897027582164,-4.86240458710454));
#140038=CARTESIAN_POINT('Ctrl Pts',(5.36849408859803,1.59120653664335,-4.87263059020909));
#140039=CARTESIAN_POINT('Origin',(-0.167074862435231,1.33939576027358,0.0962713050185793));
#140040=CARTESIAN_POINT('Ctrl Pts',(5.405057563,1.586734015,-5.199553129));
#140041=CARTESIAN_POINT('Ctrl Pts',(5.123034241,1.521690237,-5.492722994));
#140042=CARTESIAN_POINT('Ctrl Pts',(4.810955731,1.456414446,-5.753668826));
#140043=CARTESIAN_POINT('Ctrl Pts',(5.386915907,1.586734015,-4.852178584));
#140044=CARTESIAN_POINT('Ctrl Pts',(5.123734151,1.521690237,-5.14436444699999));
#140045=CARTESIAN_POINT('Ctrl Pts',(4.8304931,1.456414446,-5.406369984));
#140046=CARTESIAN_POINT('',(4.83398797806342,1.45719264060821,-5.40324534124832));
#140047=CARTESIAN_POINT('Origin',(-0.135991943969288,1.48214304425118,0.145811955775491));
#140048=CARTESIAN_POINT('Ctrl Pts',(5.00007512009465,1.49654505843161,-5.59010275334889));
#140049=CARTESIAN_POINT('Ctrl Pts',(4.97239382994859,1.49030358396498,-5.5589049316866));
#140050=CARTESIAN_POINT('Ctrl Pts',(4.94469911487078,1.48390865069507,-5.52771781147434));
#140051=CARTESIAN_POINT('Ctrl Pts',(4.88934677262698,1.47080218895167,-5.4654416255449));
#140052=CARTESIAN_POINT('Ctrl Pts',(4.86165706264628,1.46408307004702,-5.43431646029439));
#140053=CARTESIAN_POINT('Ctrl Pts',(4.83398798131907,1.4571926407418,-5.40324533969528));
#140054=CARTESIAN_POINT('Ctrl Pts',(5.18558480998957,1.456406735,-5.41919799617496));
#140055=CARTESIAN_POINT('Ctrl Pts',(4.88834075513256,1.522118786,-5.70362832263702));
#140056=CARTESIAN_POINT('Ctrl Pts',(4.56177135477614,1.586734015,-5.95384235976158));
#140057=CARTESIAN_POINT('Ctrl Pts',(4.55046915307313,1.5889702758084,-5.96250198774084));
#140058=CARTESIAN_POINT('Ctrl Pts',(4.53916695137025,1.59120653661686,-5.97116161572024));
#140059=CARTESIAN_POINT('Ctrl Pts',(4.837531582,1.456406735,-5.400072981));
#140060=CARTESIAN_POINT('Ctrl Pts',(4.541336538,1.522118786,-5.66541252));
#140061=CARTESIAN_POINT('Ctrl Pts',(4.21789784,1.586734015,-5.896765029));
#140062=CARTESIAN_POINT('Ctrl Pts',(4.20670398840411,1.5889702758084,-5.90477188058608));
#140063=CARTESIAN_POINT('Ctrl Pts',(4.19551013680818,1.59120653661686,-5.91277873217229));
#140064=CARTESIAN_POINT('Origin',(-0.142473359438439,1.33939579211148,0.129936838327164));
#140065=CARTESIAN_POINT('Ctrl Pts',(4.160940096,1.586734015,-6.23991807));
#140066=CARTESIAN_POINT('Ctrl Pts',(3.822487468,1.521690237,-6.465607109));
#140067=CARTESIAN_POINT('Ctrl Pts',(3.461609539,1.456414446,-6.653364517));
#140068=CARTESIAN_POINT('Ctrl Pts',(4.21789784,1.586734015,-5.896765029));
#140069=CARTESIAN_POINT('Ctrl Pts',(3.898057804,1.521690237,-6.125543451));
#140070=CARTESIAN_POINT('Ctrl Pts',(3.55534912,1.456414446,-6.318385287));
#140071=CARTESIAN_POINT('',(3.55943399578583,1.45719264062358,-6.31608499155558));
#140072=CARTESIAN_POINT('Origin',(-0.101467299577748,1.48214306600203,0.171637231264682));
#140073=CARTESIAN_POINT('Ctrl Pts',(3.68146929256206,1.49654505838464,-6.53427760732435));
#140074=CARTESIAN_POINT('Ctrl Pts',(3.66114178509383,1.49030358395292,-6.49785851436745));
#140075=CARTESIAN_POINT('Ctrl Pts',(3.6407988659998,1.48390865069154,-6.46144698653651));
#140076=CARTESIAN_POINT('Ctrl Pts',(3.60012817905484,1.47080219192019,-6.38872768207194));
#140077=CARTESIAN_POINT('Ctrl Pts',(3.57977682462906,1.46408307147985,-6.35237772768102));
#140078=CARTESIAN_POINT('Ctrl Pts',(3.55943399940581,1.45719264075089,-6.31608499035852));
#140079=CARTESIAN_POINT('Ctrl Pts',(3.89938133908589,1.456406735,-6.40724760846988));
#140080=CARTESIAN_POINT('Ctrl Pts',(3.54794257412965,1.522118786,-6.62112942631615));
#140081=CARTESIAN_POINT('Ctrl Pts',(3.17521956189425,1.586734015,-6.79529083046107));
#140082=CARTESIAN_POINT('Ctrl Pts',(3.16232003499673,1.58897027586157,-6.80131836201544));
#140083=CARTESIAN_POINT('Ctrl Pts',(3.14942050809924,1.59120653672322,-6.8073458935697));
#140084=CARTESIAN_POINT('Ctrl Pts',(3.563576716,1.456406735,-6.313748569));
#140085=CARTESIAN_POINT('Ctrl Pts',(3.21726639,1.522118786,-6.509211438));
#140086=CARTESIAN_POINT('Ctrl Pts',(2.851655559,1.586734015,-6.665625295));
#140087=CARTESIAN_POINT('Ctrl Pts',(2.83900217674645,1.58897027586157,-6.67103860378233));
#140088=CARTESIAN_POINT('Ctrl Pts',(2.82634879449291,1.59120653672321,-6.6764519125648));
#140089=CARTESIAN_POINT('Origin',(-0.111209903498641,1.33939578981825,0.157526672287099));
#140090=CARTESIAN_POINT('Ctrl Pts',(2.722261695,1.586734015,-6.988511377));
#140091=CARTESIAN_POINT('Ctrl Pts',(2.343205429,1.521690237,-7.136166621));
#140092=CARTESIAN_POINT('Ctrl Pts',(1.950402333,1.456414446,-7.241956279));
#140093=CARTESIAN_POINT('Ctrl Pts',(2.851655559,1.586734015,-6.665625295));
#140094=CARTESIAN_POINT('Ctrl Pts',(2.490112606,1.521690237,-6.820298851));
#140095=CARTESIAN_POINT('Ctrl Pts',(2.113960967,1.456414446,-6.934959915));
#140096=CARTESIAN_POINT('',(2.11844483589611,1.45719264061025,-6.93359152692528));
#140097=CARTESIAN_POINT('Origin',(-0.0621981411917949,1.48214301209216,
0.189437027024965));
#140098=CARTESIAN_POINT('Ctrl Pts',(2.19072205301252,1.49654505837123,-7.17291690241065));
#140099=CARTESIAN_POINT('Ctrl Pts',(2.17869881975251,1.49030358392898,-7.13297945426369));
#140100=CARTESIAN_POINT('Ctrl Pts',(2.16665890893221,1.48390865067593,-7.09304608144557));
#140101=CARTESIAN_POINT('Ctrl Pts',(2.14257158065369,1.47080219181767,-7.01328391782613));
#140102=CARTESIAN_POINT('Ctrl Pts',(2.13051019526033,1.4640830714041,-6.97340886569849));
#140103=CARTESIAN_POINT('Ctrl Pts',(2.11844483965137,1.45719264069612,-6.93359152644189));
#140104=CARTESIAN_POINT('Ctrl Pts',(2.43084713209955,1.456406735,-7.09570144285708));
#140105=CARTESIAN_POINT('Ctrl Pts',(2.04164654045883,1.522118786,-7.22903387662134));
#140106=CARTESIAN_POINT('Ctrl Pts',(1.64019803211863,1.586734015,-7.3189990540958));
#140107=CARTESIAN_POINT('Ctrl Pts',(1.62630434806752,1.58897027583535,-7.32211264830641));
#140108=CARTESIAN_POINT('Ctrl Pts',(1.61241066401639,1.59120653667077,-7.32522624251717));
#140109=CARTESIAN_POINT('Ctrl Pts',(2.122992963,1.456406735,-6.932200291));
#140110=CARTESIAN_POINT('Ctrl Pts',(1.742760442,1.522118786,-7.048646864));
#140111=CARTESIAN_POINT('Ctrl Pts',(1.352073032,1.586734015,-7.122808331));
#140112=CARTESIAN_POINT('Ctrl Pts',(1.33855177753145,1.58897027583535,-7.12537497645977));
#140113=CARTESIAN_POINT('Ctrl Pts',(1.32503052306288,1.59120653667077,-7.1279416219196));
#140114=CARTESIAN_POINT('Origin',(-0.0747462306198937,1.33939577632165,
0.177750342394769));
#140115=CARTESIAN_POINT('Ctrl Pts',(1.156293362,1.586734015,-7.410329659));
#140116=CARTESIAN_POINT('Ctrl Pts',(0.754357708,1.521690237,-7.473046914));
#140117=CARTESIAN_POINT('Ctrl Pts',(0.347996481,1.456414446,-7.491922213));
#140118=CARTESIAN_POINT('Ctrl Pts',(1.352073032,1.586734015,-7.122808331));
#140119=CARTESIAN_POINT('Ctrl Pts',(0.965732511,1.521690237,-7.19614465799999));
#140120=CARTESIAN_POINT('Ctrl Pts',(0.573726349,1.456414446,-7.227263526));
#140121=CARTESIAN_POINT('',(0.578399550200102,1.45719264058788,-7.22689102927039));
#140122=CARTESIAN_POINT('Origin',(-0.0200205943984027,1.48214303746773,
0.198378610296187));
#140123=CARTESIAN_POINT('Ctrl Pts',(0.597539084743176,1.49654505840402,
-7.47615857517617));
#140124=CARTESIAN_POINT('Ctrl Pts',(0.594382318797104,1.49030358394784,
-7.43457020272796));
#140125=CARTESIAN_POINT('Ctrl Pts',(0.591208389122253,1.48390865067692,
-7.39298222514298));
#140126=CARTESIAN_POINT('Ctrl Pts',(0.584830715843341,1.4708021902267,-7.3099067833631));
#140127=CARTESIAN_POINT('Ctrl Pts',(0.581623276858751,1.46408307062406,
-7.26837115206612));
#140128=CARTESIAN_POINT('Ctrl Pts',(0.578399553874345,1.45719264066649,
-7.22689102998411));
#140129=CARTESIAN_POINT('Ctrl Pts',(0.848649214287756,1.456406735,-7.45236816437262));
#140130=CARTESIAN_POINT('Ctrl Pts',(0.439885384551297,1.522118786,-7.49891673678234));
#140131=CARTESIAN_POINT('Ctrl Pts',(0.0284826653430106,1.586734015,-7.50047901633372));
#140132=CARTESIAN_POINT('Ctrl Pts',(0.0142444776038436,1.58897027576919,
-7.50053308508075));
#140133=CARTESIAN_POINT('Ctrl Pts',(6.28986467648867E-6,1.59120653653846,
-7.50058715382782));
#140134=CARTESIAN_POINT('Ctrl Pts',(0.583140419,1.456406735,-7.226510033));
#140135=CARTESIAN_POINT('Ctrl Pts',(0.186764952,1.522118786,-7.258495397));
#140136=CARTESIAN_POINT('Ctrl Pts',(-0.210730926,1.586734015,-7.246936765));
#140137=CARTESIAN_POINT('Ctrl Pts',(-0.224487813527143,1.58897027576919,
-7.24653673368094));
#140138=CARTESIAN_POINT('Ctrl Pts',(-0.238244701054285,1.59120653653846,
-7.246136702362));
#140139=CARTESIAN_POINT('Origin',(-0.0347876382410184,1.33939576438634,
0.189663017003805));
#140140=CARTESIAN_POINT('Ctrl Pts',(-0.463741963,1.586734015,-7.485649163));
#140141=CARTESIAN_POINT('Ctrl Pts',(-0.869762941,1.521690237,-7.460495838));
#140142=CARTESIAN_POINT('Ctrl Pts',(-1.2706813,1.456414446,-7.391574192));
#140143=CARTESIAN_POINT('Ctrl Pts',(-0.210730926,1.586734015,-7.246936765));
#140144=CARTESIAN_POINT('Ctrl Pts',(-0.603804163,1.521690237,-7.235506737));
#140145=CARTESIAN_POINT('Ctrl Pts',(-0.993335076,1.456414446,-7.181628327));
#140146=CARTESIAN_POINT('',(-0.988691055730179,1.45719264059555,-7.18226913885259));
#140147=CARTESIAN_POINT('Origin',(0.0230930328052294,1.48214303776053,0.198044760086257));
#140148=CARTESIAN_POINT('Ctrl Pts',(-1.02358414735161,1.49654505839643,
-7.42982338229497));
#140149=CARTESIAN_POINT('Ctrl Pts',(-1.01772683905243,1.49030358395369,
-7.38852871155802));
#140150=CARTESIAN_POINT('Ctrl Pts',(-1.01188637805703,1.48390865069583,
-7.34723073675153));
#140151=CARTESIAN_POINT('Ctrl Pts',(-1.00025618222517,1.470802192435,-7.26472655507432));
#140152=CARTESIAN_POINT('Ctrl Pts',(-0.994459698903287,1.46408307172406,
-7.2234724918208));
#140153=CARTESIAN_POINT('Ctrl Pts',(-0.988691051854014,1.45719264074061,
-7.18226914059731));
#140154=CARTESIAN_POINT('Ctrl Pts',(-0.773230597839086,1.456406735,-7.46057043305704));
#140155=CARTESIAN_POINT('Ctrl Pts',(-1.18244432400898,1.522118786,-7.41815858538821));
#140156=CARTESIAN_POINT('Ctrl Pts',(-1.58456451966023,1.586734015,-7.33124491658723));
#140157=CARTESIAN_POINT('Ctrl Pts',(-1.59848144954698,1.5889702757532,-7.32823693179069));
#140158=CARTESIAN_POINT('Ctrl Pts',(-1.61239837943374,1.59120653650647,
-7.32522894699414));
#140159=CARTESIAN_POINT('Ctrl Pts',(-0.983979122,1.456406735,-7.182916197));
#140160=CARTESIAN_POINT('Ctrl Pts',(-1.37796346,1.522118786,-7.128944752));
#140161=CARTESIAN_POINT('Ctrl Pts',(-1.763681341,1.586734015,-7.032206491));
#140162=CARTESIAN_POINT('Ctrl Pts',(-1.77703060513542,1.5889702757532,-7.02885848806392));
#140163=CARTESIAN_POINT('Ctrl Pts',(-1.79037986927085,1.59120653650647,
-7.02551048512773));
#140164=CARTESIAN_POINT('Origin',(0.00679763605717421,1.33939574081864,
0.19270726971784));
#140165=CARTESIAN_POINT('Ctrl Pts',(-2.06209323,1.586734015,-7.21094803100001));
#140166=CARTESIAN_POINT('Ctrl Pts',(-2.453214441,1.521690237,-7.099100269));
#140167=CARTESIAN_POINT('Ctrl Pts',(-2.829943435,1.456414446,-6.945604377));
#140168=CARTESIAN_POINT('Ctrl Pts',(-1.763681341,1.586734015,-7.032206491));
#140169=CARTESIAN_POINT('Ctrl Pts',(-2.145107626,1.521690237,-6.936544564));
#140170=CARTESIAN_POINT('Ctrl Pts',(-2.513949257,1.456414446,-6.800188169));
#140171=CARTESIAN_POINT('',(-2.50955156696889,1.45719264059073,-6.80181232626542));
#140172=CARTESIAN_POINT('Origin',(0.0651268731420246,1.48214303842256,0.188450166502925));
#140173=CARTESIAN_POINT('Ctrl Pts',(-2.59684572190938,1.49654505838242,
-7.03607790590515));
#140174=CARTESIAN_POINT('Ctrl Pts',(-2.58224822063562,1.49030358394116,
-6.99700782975637));
#140175=CARTESIAN_POINT('Ctrl Pts',(-2.56766646253126,1.48390865068695,
-6.9579309050984));
#140176=CARTESIAN_POINT('Ctrl Pts',(-2.53857221501543,1.47080219291372,
-6.87985577640133));
#140177=CARTESIAN_POINT('Ctrl Pts',(-2.52404284554602,1.46408307195932,
-6.84081228116058));
#140178=CARTESIAN_POINT('Ctrl Pts',(-2.50955156324783,1.45719264075521,
-6.80181232858497));
#140179=CARTESIAN_POINT('Ctrl Pts',(-2.35895500654193,1.456406735,-7.11992472055498));
#140180=CARTESIAN_POINT('Ctrl Pts',(-2.74948424915749,1.522118786,-6.99053558333553));
#140181=CARTESIAN_POINT('Ctrl Pts',(-3.12351922935449,1.586734015,-6.81920995168709));
#140182=CARTESIAN_POINT('Ctrl Pts',(-3.13646416134242,1.58897027574851,
-6.81328056334937));
#140183=CARTESIAN_POINT('Ctrl Pts',(-3.14940909333042,1.5912065364971,-6.80735117501149));
#140184=CARTESIAN_POINT('Ctrl Pts',(-2.505088894,1.456406735,-6.803457182));
#140185=CARTESIAN_POINT('Ctrl Pts',(-2.878259831,1.522118786,-6.666052574));
#140186=CARTESIAN_POINT('Ctrl Pts',(-3.234163976,1.586734015,-6.488658057));
#140187=CARTESIAN_POINT('Ctrl Pts',(-3.24648142007655,1.58897027574851,
-6.48251863133349));
#140188=CARTESIAN_POINT('Ctrl Pts',(-3.25879886415312,1.59120653649709,
-6.47637920566687));
#140189=CARTESIAN_POINT('Origin',(0.0480650262539523,1.33939571431161,0.186740464814124));
#140190=CARTESIAN_POINT('Ctrl Pts',(-3.564023309,1.586734015,-6.599070984));
#140191=CARTESIAN_POINT('Ctrl Pts',(-3.921956361,1.521690237,-6.405758661));
#140192=CARTESIAN_POINT('Ctrl Pts',(-4.25688056,1.456414446,-6.17486582));
#140193=CARTESIAN_POINT('Ctrl Pts',(-3.234163976,1.586734015,-6.48865805700001));
#140194=CARTESIAN_POINT('Ctrl Pts',(-3.58610824,1.521690237,-6.313237276));
#140195=CARTESIAN_POINT('Ctrl Pts',(-3.917013965,1.456414446,-6.10077877));
#140196=CARTESIAN_POINT('',(-3.91306823593771,1.45719264060545,-6.10331032877246));
#140197=CARTESIAN_POINT('Origin',(0.104115509672377,1.4821430441907,0.170044049113139));
#140198=CARTESIAN_POINT('Ctrl Pts',(-4.04868167678958,1.49654505837857,
-6.31333324611067));
#140199=CARTESIAN_POINT('Ctrl Pts',(-4.02602654552554,1.49030358394781,
-6.27831463799634));
#140200=CARTESIAN_POINT('Ctrl Pts',(-4.00338531713499,1.48390865070025,
-6.24328595714916));
#140201=CARTESIAN_POINT('Ctrl Pts',(-3.9581874309852,1.47080219258203,-6.17329058298485));
#140202=CARTESIAN_POINT('Ctrl Pts',(-3.93560455346299,1.46408307182328,
-6.13828328903141));
#140203=CARTESIAN_POINT('Ctrl Pts',(-3.91306823295187,1.45719264080112,
-6.10331033194857));
#140204=CARTESIAN_POINT('Ctrl Pts',(-3.83437730066977,1.456406735,-6.44635924039643));
#140205=CARTESIAN_POINT('Ctrl Pts',(-4.1879613471737,1.522118786,-6.23604290637256));
#140206=CARTESIAN_POINT('Ctrl Pts',(-4.51642165067597,1.586734015,-5.98831630932468));
#140207=CARTESIAN_POINT('Ctrl Pts',(-4.5277892940278,1.58897027573085,-5.97974276916175));
#140208=CARTESIAN_POINT('Ctrl Pts',(-4.53915693737959,1.59120653646176,
-5.97116922899881));
#140209=CARTESIAN_POINT('Ctrl Pts',(-3.909063493,1.456406735,-6.105876072));
#140210=CARTESIAN_POINT('Ctrl Pts',(-4.243971972,1.522118786,-5.891463186));
#140211=CARTESIAN_POINT('Ctrl Pts',(-4.553420698,1.586734015,-5.64170718300001));
#140212=CARTESIAN_POINT('Ctrl Pts',(-4.56413037194033,1.58897027573085,
-5.63306340736922));
#140213=CARTESIAN_POINT('Ctrl Pts',(-4.57484004588063,1.59120653646176,
-5.62441963173858));
#140214=CARTESIAN_POINT('Origin',(0.087084894057271,1.33939575604422,0.172041892552222));
#140215=CARTESIAN_POINT('Ctrl Pts',(-4.899303619,1.586734015,-5.678628712));
#140216=CARTESIAN_POINT('Ctrl Pts',(-5.20731196,1.521690237,-5.412890898));
#140217=CARTESIAN_POINT('Ctrl Pts',(-5.484770682,1.456414446,-5.115397401));
#140218=CARTESIAN_POINT('Ctrl Pts',(-4.553420698,1.586734015,-5.641707183));
#140219=CARTESIAN_POINT('Ctrl Pts',(-4.859426419,1.521690237,-5.39473003));
#140220=CARTESIAN_POINT('Ctrl Pts',(-5.136923453,1.456414446,-5.116103736));
#140221=CARTESIAN_POINT('',(-5.13361418323162,1.45719264060118,-5.11942432355012));
#140222=CARTESIAN_POINT('Origin',(0.138235559677372,1.48214304625789,0.143686509911358));
#140223=CARTESIAN_POINT('Ctrl Pts',(-5.31120577594162,1.49654505840647,
-5.29538414122325));
#140224=CARTESIAN_POINT('Ctrl Pts',(-5.28155234347734,1.49030358394726,
-5.26605443207318));
#140225=CARTESIAN_POINT('Ctrl Pts',(-5.25191032365658,1.48390865070959,
-5.23671189715127));
#140226=CARTESIAN_POINT('Ctrl Pts',(-5.19272219896809,1.4708021917559,-5.17806918153808));
#140227=CARTESIAN_POINT('Ctrl Pts',(-5.16314176519753,1.46408307141407,
-5.1487349916414));
#140228=CARTESIAN_POINT('Ctrl Pts',(-5.13361418103969,1.45719264078779,
-5.11942432714059));
#140229=CARTESIAN_POINT('Ctrl Pts',(-5.13050837364047,1.456406735,-5.47136916785226));
#140230=CARTESIAN_POINT('Ctrl Pts',(-5.43061402642661,1.522118786,-5.18995979468923));
#140231=CARTESIAN_POINT('Ctrl Pts',(-5.69814121471094,1.586734015,-4.87741565142108));
#140232=CARTESIAN_POINT('Ctrl Pts',(-5.70740003131374,1.58897027576622,
-4.86659884838373));
#140233=CARTESIAN_POINT('Ctrl Pts',(-5.71665884791666,1.5912065365325,-4.8557820453464));
#140234=CARTESIAN_POINT('Ctrl Pts',(-5.130254628,1.456406735,-5.122790982));
#140235=CARTESIAN_POINT('Ctrl Pts',(-5.411240701,1.522118786,-4.841395528));
#140236=CARTESIAN_POINT('Ctrl Pts',(-5.65976453,1.586734015,-4.530956353));
#140237=CARTESIAN_POINT('Ctrl Pts',(-5.66836566160424,1.58897027576622,
-4.52021240055879));
#140238=CARTESIAN_POINT('Ctrl Pts',(-5.67696679320846,1.5912065365325,-4.50946844811759));
#140239=CARTESIAN_POINT('Origin',(0.122032764432546,1.3393957688585,0.149298916293734));
#140240=CARTESIAN_POINT('Ctrl Pts',(-6.005497937,1.586734015,-4.492660073));
#140241=CARTESIAN_POINT('Ctrl Pts',(-6.249179439,1.521690237,-4.166922373));
#140242=CARTESIAN_POINT('Ctrl Pts',(-6.456199023,1.456414446,-3.816738684));
#140243=CARTESIAN_POINT('Ctrl Pts',(-5.65976453000001,1.586734015,-4.530956353));
#140244=CARTESIAN_POINT('Ctrl Pts',(-5.905523219,1.521690237,-4.223971203));
#140245=CARTESIAN_POINT('Ctrl Pts',(-6.116636109,1.456414446,-3.892205378));
#140246=CARTESIAN_POINT('',(-6.11411803681458,1.45719264058743,-3.89615972708495));
#140247=CARTESIAN_POINT('Origin',(0.165892242204772,1.48214301587359,0.110610760436994));
#140248=CARTESIAN_POINT('Ctrl Pts',(-6.32538379675321,1.49654505840746,
-4.02982875897274));
#140249=CARTESIAN_POINT('Ctrl Pts',(-6.29011862453828,1.49030358395683,
-4.00755937353871));
#140250=CARTESIAN_POINT('Ctrl Pts',(-6.2548618407542,1.48390865067755,-3.98527500864475));
#140251=CARTESIAN_POINT('Ctrl Pts',(-6.1844510440732,1.47080219039292,-3.94072701982678));
#140252=CARTESIAN_POINT('Ctrl Pts',(-6.14925620457091,1.46408307071962,
-3.91843756826649));
#140253=CARTESIAN_POINT('Ctrl Pts',(-6.1141180357621,1.45719264069513,-3.89615973061763));
#140254=CARTESIAN_POINT('Ctrl Pts',(-6.18674257775374,1.456406735,-4.2405439538314));
#140255=CARTESIAN_POINT('Ctrl Pts',(-6.41933723072151,1.522118786,-3.90119993089596));
#140256=CARTESIAN_POINT('Ctrl Pts',(-6.61342203006909,1.586734015,-3.53845245862732));
#140257=CARTESIAN_POINT('Ctrl Pts',(-6.62013908773575,1.58897027575197,
-3.52589817463466));
#140258=CARTESIAN_POINT('Ctrl Pts',(-6.62685614540246,1.59120653650401,
-3.51334389064201));
#140259=CARTESIAN_POINT('Ctrl Pts',(-6.111560759,1.456406735,-3.90016988));
#140260=CARTESIAN_POINT('Ctrl Pts',(-6.325485828,1.522118786,-3.564949595));
#140261=CARTESIAN_POINT('Ctrl Pts',(-6.501464062,1.586734015,-3.208343039));
#140262=CARTESIAN_POINT('Ctrl Pts',(-6.50755447170662,1.58897027575197,
-3.19600128524589));
#140263=CARTESIAN_POINT('Ctrl Pts',(-6.51364488141335,1.59120653650401,
-3.18365953149176));
#140264=CARTESIAN_POINT('Origin',(0.151274700206816,1.33939575620768,0.119575041319626));
#140265=CARTESIAN_POINT('Ctrl Pts',(-6.830881846,1.586734015,-3.096619642));
#140266=CARTESIAN_POINT('Ctrl Pts',(-6.99884223300001,1.521690237,-2.726113188));
#140267=CARTESIAN_POINT('Ctrl Pts',(-7.125742672,1.456414446,-2.339613509));
#140268=CARTESIAN_POINT('Ctrl Pts',(-6.501464062,1.586734015,-3.208343039));
#140269=CARTESIAN_POINT('Ctrl Pts',(-6.675484317,1.521690237,-2.855704178));
#140270=CARTESIAN_POINT('Ctrl Pts',(-6.81034166,1.456414446,-2.486311822));
#140271=CARTESIAN_POINT('',(-6.8087325263123,1.4571926406148,-2.49071503215939));
#140272=CARTESIAN_POINT('Origin',(0.185791769945721,1.48214304416343,0.0723628059213374));
#140273=CARTESIAN_POINT('Ctrl Pts',(-7.04379390051593,1.49654505840368,
-2.575843062689));
#140274=CARTESIAN_POINT('Ctrl Pts',(-7.00456594895746,1.49030358396683,
-2.56167529283628));
#140275=CARTESIAN_POINT('Ctrl Pts',(-6.96534296957004,1.48390865070459,
-2.54749109047069));
#140276=CARTESIAN_POINT('Ctrl Pts',(-6.88700185505409,1.4708021933808,-2.51912085537668));
#140277=CARTESIAN_POINT('Ctrl Pts',(-6.84783826862204,1.46408307220057,
-2.50491836558355));
#140278=CARTESIAN_POINT('Ctrl Pts',(-6.80873252610584,1.45719264079019,
-2.4907150361556));
#140279=CARTESIAN_POINT('Ctrl Pts',(-6.95369157446804,1.456406735,-2.8114356170973));
#140280=CARTESIAN_POINT('Ctrl Pts',(-7.10789935959439,1.522118786,-2.43002429438231));
#140281=CARTESIAN_POINT('Ctrl Pts',(-7.21946658014416,1.586734015,-2.03403516072589));
#140282=CARTESIAN_POINT('Ctrl Pts',(-7.2233277967278,1.58897027572729,-2.02033042019118));
#140283=CARTESIAN_POINT('Ctrl Pts',(-7.22718901331137,1.59120653645465,
-2.00662567965648));
#140284=CARTESIAN_POINT('Ctrl Pts',(-6.8070971,1.456406735,-2.495181169));
#140285=CARTESIAN_POINT('Ctrl Pts',(-6.943958268,1.522118786,-2.121810582));
#140286=CARTESIAN_POINT('Ctrl Pts',(-7.03916236,1.586734015,-1.73571117));
#140287=CARTESIAN_POINT('Ctrl Pts',(-7.04245726702598,1.58897027572729,
-1.72234870165851));
#140288=CARTESIAN_POINT('Ctrl Pts',(-7.045752174052,1.59120653645465,-1.70898623331697));
#140289=CARTESIAN_POINT('Origin',(0.173442981648092,1.33939574964305,0.0842598250749746));
#140290=CARTESIAN_POINT('Ctrl Pts',(-7.33686131200001,1.586734015,-1.555784718));
#140291=CARTESIAN_POINT('Ctrl Pts',(-7.421246943,1.521690237,-1.157833981));
#140292=CARTESIAN_POINT('Ctrl Pts',(-7.462094514,1.456414446,-0.753090606));
#140293=CARTESIAN_POINT('Ctrl Pts',(-7.03916236,1.586734015,-1.73571117));
#140294=CARTESIAN_POINT('Ctrl Pts',(-7.133307187,1.521690237,-1.353907599));
#140295=CARTESIAN_POINT('Ctrl Pts',(-7.185603203,1.456414446,-0.964161089));
#140296=CARTESIAN_POINT('',(-7.18497825045877,1.45719264059852,-0.968807270208435));
#140297=CARTESIAN_POINT('Origin',(0.197003933959137,1.48214303945679,0.0307312683202327));
#140298=CARTESIAN_POINT('Ctrl Pts',(-7.4328440302926,1.49654505837467,-1.00141380765487));
#140299=CARTESIAN_POINT('Ctrl Pts',(-7.39148755465633,1.49030358392794,
-0.996010122351639));
#140300=CARTESIAN_POINT('Ctrl Pts',(-7.35013240261102,1.48390865068228,
-0.990589319895403));
#140301=CARTESIAN_POINT('Ctrl Pts',(-7.26752408917957,1.47080219197549,
-0.979723387895179));
#140302=CARTESIAN_POINT('Ctrl Pts',(-7.22622301479003,1.46408307149698,
-0.97427195849633));
#140303=CARTESIAN_POINT('Ctrl Pts',(-7.18497825071308,1.45719264073434,
-0.96880727432235));
#140304=CARTESIAN_POINT('Ctrl Pts',(-7.39549368163616,1.456406735,-1.25086767559283));
#140305=CARTESIAN_POINT('Ctrl Pts',(-7.46410401451051,1.522118786,-0.845223421831543));
#140306=CARTESIAN_POINT('Ctrl Pts',(-7.48793689720321,1.586734015,-0.434508640665181));
#140307=CARTESIAN_POINT('Ctrl Pts',(-7.48876172660557,1.58897027577494,
-0.42029426165538));
#140308=CARTESIAN_POINT('Ctrl Pts',(-7.48958655600797,1.59120653654989,
-0.40607988264558));
#140309=CARTESIAN_POINT('Ctrl Pts',(-7.184341147,1.456406735,-0.97352056));
#140310=CARTESIAN_POINT('Ctrl Pts',(-7.237738938,1.522118786,-0.579458064));
#140311=CARTESIAN_POINT('Ctrl Pts',(-7.24771725,1.586734015,-0.181919376));
#140312=CARTESIAN_POINT('Ctrl Pts',(-7.24806258821318,1.58897027577494,
-0.168161006831391));
#140313=CARTESIAN_POINT('Ctrl Pts',(-7.24840792642632,1.59120653654989,
-0.154402637662788));
#140314=CARTESIAN_POINT('Origin',(0.187501581422369,1.33939575027433,0.0450047815784362));
#140315=CARTESIAN_POINT('Ctrl Pts',(-7.499777297,1.586734015,0.05779697));
#140316=CARTESIAN_POINT('Ctrl Pts',(-7.496642395,1.521690237,0.464584256));
#140317=CARTESIAN_POINT('Ctrl Pts',(-7.44952710999999,1.456414446,0.868645977));
#140318=CARTESIAN_POINT('Ctrl Pts',(-7.24771725,1.586734015,-0.181919376));
#140319=CARTESIAN_POINT('Ctrl Pts',(-7.257584542,1.521690237,0.211196195));
#140320=CARTESIAN_POINT('Ctrl Pts',(-7.224873927,1.456414446,0.603072745000001));
#140321=CARTESIAN_POINT('',(-7.22526237690475,1.45719264059895,0.598400842763318));
#140322=CARTESIAN_POINT('Origin',(0.199004244131034,1.48214300852825,-0.0123372337775944));
#140323=CARTESIAN_POINT('Ctrl Pts',(-7.47434263483393,1.49654505840668,
0.619840443920158));
#140324=CARTESIAN_POINT('Ctrl Pts',(-7.43279141797426,1.49030358396172,
0.616227374350938));
#140325=CARTESIAN_POINT('Ctrl Pts',(-7.39123781394946,1.48390865069529,
0.612631306257495));
#140326=CARTESIAN_POINT('Ctrl Pts',(-7.30822498460246,1.47080219226751,
0.605484853522584));
#140327=CARTESIAN_POINT('Ctrl Pts',(-7.26671760915856,1.46408307162048,
0.601930321309041));
#140328=CARTESIAN_POINT('Ctrl Pts',(-7.22526237832533,1.45719264069052,
0.598400839016716));
#140329=CARTESIAN_POINT('Ctrl Pts',(-7.49149072463768,1.456406735,0.368189448021402));
#140330=CARTESIAN_POINT('Ctrl Pts',(-7.47129546192193,1.522118786,0.779099157187545));
#140331=CARTESIAN_POINT('Ctrl Pts',(-7.40627960745038,1.586734015,1.18533502103326));
#140332=CARTESIAN_POINT('Ctrl Pts',(-7.40402948149176,1.58897027575943,
1.19939438962868));
#140333=CARTESIAN_POINT('Ctrl Pts',(-7.40177935553306,1.59120653651885,
1.21345375822411));
#140334=CARTESIAN_POINT('Ctrl Pts',(-7.225653387,1.456406735,0.593660789));
#140335=CARTESIAN_POINT('Ctrl Pts',(-7.193090978,1.522118786,0.989989269));
#140336=CARTESIAN_POINT('Ctrl Pts',(-7.117376937,1.586734015,1.380378766));
#140337=CARTESIAN_POINT('Ctrl Pts',(-7.11475655877887,1.58897027575943,
1.39388970957387));
#140338=CARTESIAN_POINT('Ctrl Pts',(-7.11213618055764,1.59120653651885,
1.40740065314777));
#140339=CARTESIAN_POINT('Origin',(0.192792530964795,1.33939579133204,0.00364529811479691));
#140340=CARTESIAN_POINT('Ctrl Pts',(-7.312012032,1.586734015,1.668676136));
#140341=CARTESIAN_POINT('Ctrl Pts',(-7.221503179,1.521690237,2.06527905));
#140342=CARTESIAN_POINT('Ctrl Pts',(-7.088628098,1.456414446,2.449765639));
#140343=CARTESIAN_POINT('Ctrl Pts',(-7.117376937,1.586734015,1.380378766));
#140344=CARTESIAN_POINT('Ctrl Pts',(-7.042505309,1.521690237,1.766424689));
#140345=CARTESIAN_POINT('Ctrl Pts',(-6.926317576,1.456414446,2.142107568));
#140346=CARTESIAN_POINT('',(-6.92770126528305,1.45719264059855,2.13762839733776));
#140347=CARTESIAN_POINT('Origin',(0.191699739143811,1.48214301911425,-0.0548288895523261));
#140348=CARTESIAN_POINT('Ctrl Pts',(-7.16634928428777,1.49654505841316,
2.21211164520096));
#140349=CARTESIAN_POINT('Ctrl Pts',(-7.12654621497199,1.49030358397192,
2.19965076379803));
#140350=CARTESIAN_POINT('Ctrl Pts',(-7.08673715953174,1.48390865071391,
2.18720597323833));
#140351=CARTESIAN_POINT('Ctrl Pts',(-7.00720139359456,1.47080219120606,
2.1623812941064));
#140352=CARTESIAN_POINT('Ctrl Pts',(-6.96742856043393,1.46408307111354,
2.14998700724187));
#140353=CARTESIAN_POINT('Ctrl Pts',(-6.92770126721526,1.45719264069766,
2.13762839403927));
#140354=CARTESIAN_POINT('Ctrl Pts',(-7.23719398613241,1.456406735,1.97003044157164));
#140355=CARTESIAN_POINT('Ctrl Pts',(-7.12913743724507,1.522118786,2.3669919266526));
#140356=CARTESIAN_POINT('Ctrl Pts',(-6.97831291553588,1.586734015,2.74975373474379));
#140357=CARTESIAN_POINT('Ctrl Pts',(-6.97309304757981,1.5889702757851,2.76300069269339));
#140358=CARTESIAN_POINT('Ctrl Pts',(-6.96787317962392,1.5912065365702,2.77624765064298));
#140359=CARTESIAN_POINT('Ctrl Pts',(-6.929102105,1.456406735,2.133083219));
#140360=CARTESIAN_POINT('Ctrl Pts',(-6.812102079,1.522118786,2.513145805));
#140361=CARTESIAN_POINT('Ctrl Pts',(-6.654235988,1.586734015,2.878131931));
#140362=CARTESIAN_POINT('Ctrl Pts',(-6.64877241920881,1.5889702757851,2.8907636924796));
#140363=CARTESIAN_POINT('Ctrl Pts',(-6.64330885041767,1.5912065365702,2.90339545395922));
#140364=CARTESIAN_POINT('Origin',(0.189068793117005,1.33939575948771,-0.0378846249694881));
#140365=CARTESIAN_POINT('Ctrl Pts',(-6.78234521,1.586734015,3.201529861));
#140366=CARTESIAN_POINT('Ctrl Pts',(-6.608694501,1.521690237,3.569403691));
#140367=CARTESIAN_POINT('Ctrl Pts',(-6.396272715,1.456414446,3.916336982));
#140368=CARTESIAN_POINT('Ctrl Pts',(-6.654235988,1.586734015,2.878131931));
#140369=CARTESIAN_POINT('Ctrl Pts',(-6.498126356,1.521690237,3.239057128));
#140370=CARTESIAN_POINT('Ctrl Pts',(-6.303894313,1.456414446,3.580979822));
#140371=CARTESIAN_POINT('',(-6.3062085417898,1.45719264061766,3.57690282398186));
#140372=CARTESIAN_POINT('Origin',(0.17543108332008,1.48214304481658,-0.094756675136119));
#140373=CARTESIAN_POINT('Ctrl Pts',(-6.52326540639353,1.49654505841099,
3.70094696449352));
#140374=CARTESIAN_POINT('Ctrl Pts',(-6.48707163187202,1.4903035839601,3.6802209282024));
#140375=CARTESIAN_POINT('Ctrl Pts',(-6.45086855211468,1.48390865069852,
3.65950931972571));
#140376=CARTESIAN_POINT('Ctrl Pts',(-6.37852886526687,1.47080219210092,
3.61816719197017));
#140377=CARTESIAN_POINT('Ctrl Pts',(-6.34235030148423,1.46408307157444,
3.59751269169146));
#140378=CARTESIAN_POINT('Ctrl Pts',(-6.30620854453905,1.45719264077253,
3.57690282104796));
#140379=CARTESIAN_POINT('Ctrl Pts',(-6.64449410151412,1.456406735,3.47975500206342));
#140380=CARTESIAN_POINT('Ctrl Pts',(-6.45362886927911,1.522118786,3.84420678350785));
#140381=CARTESIAN_POINT('Ctrl Pts',(-6.22404806648052,1.586734015,4.18559701939759));
#140382=CARTESIAN_POINT('Ctrl Pts',(-6.2161025318132,1.58897027576657,4.19741215342132));
#140383=CARTESIAN_POINT('Ctrl Pts',(-6.20815699714588,1.59120653653314,
4.2092272874451));
#140384=CARTESIAN_POINT('Ctrl Pts',(-6.30855371000001,1.456406735,3.572765048));
#140385=CARTESIAN_POINT('Ctrl Pts',(-6.11258685800001,1.522118786,3.918790435));
#140386=CARTESIAN_POINT('Ctrl Pts',(-5.879950361,1.586734015,4.241306845));
#140387=CARTESIAN_POINT('Ctrl Pts',(-5.87189907217594,1.58897027576657,
4.25246877703087));
#140388=CARTESIAN_POINT('Ctrl Pts',(-5.86384778335191,1.59120653653313,
4.26363070906172));
#140389=CARTESIAN_POINT('Origin',(0.176504357918514,1.33939572459492,-0.0776430649301657));
#140390=CARTESIAN_POINT('Ctrl Pts',(-5.935543465,1.586734015,4.584683607));
#140391=CARTESIAN_POINT('Ctrl Pts',(-5.686870614,1.521690237,4.906626983));
#140392=CARTESIAN_POINT('Ctrl Pts',(-5.404834728,1.456414446,5.199784761));
#140393=CARTESIAN_POINT('Ctrl Pts',(-5.87995036100001,1.586734015,4.241306845));
#140394=CARTESIAN_POINT('Ctrl Pts',(-5.649902236,1.521690237,4.560234855));
#140395=CARTESIAN_POINT('Ctrl Pts',(-5.386707959,1.456414446,4.852409439));
#140396=CARTESIAN_POINT('',(-5.389844515688,1.45719264057876,4.8489252501941));
#140397=CARTESIAN_POINT('Origin',(0.150959951003083,1.48214302133659,-0.130254007742108));
#140398=CARTESIAN_POINT('Ctrl Pts',(-5.57516088824712,1.49654505841865,
5.01673011704007));
#140399=CARTESIAN_POINT('Ctrl Pts',(-5.5442687891568,1.49030358396378,4.98870805233087));
#140400=CARTESIAN_POINT('Ctrl Pts',(-5.51336450100249,1.4839086507277,4.96069807790661));
#140401=CARTESIAN_POINT('Ctrl Pts',(-5.45160341771219,1.47080219347429,
4.90477161763631));
#140402=CARTESIAN_POINT('Ctrl Pts',(-5.42071079214679,1.46408307220416,
4.87682268306431));
#140403=CARTESIAN_POINT('Ctrl Pts',(-5.38984451945149,1.45719264069583,
4.8489252475705));
#140404=CARTESIAN_POINT('Ctrl Pts',(-5.74110505755524,1.456406735,4.82677008554393));
#140405=CARTESIAN_POINT('Ctrl Pts',(-5.47635578817438,1.522118786,5.14167080416162));
#140406=CARTESIAN_POINT('Ctrl Pts',(-5.17875364692979,1.586734015,5.42572643982073));
#140407=CARTESIAN_POINT('Ctrl Pts',(-5.16845396967177,1.58897027580737,
5.4355572876714));
#140408=CARTESIAN_POINT('Ctrl Pts',(-5.15815429241373,1.59120653661473,
5.44538813552219));
#140409=CARTESIAN_POINT('Ctrl Pts',(-5.393024354,1.456406735,4.845388355));
#140410=CARTESIAN_POINT('Ctrl Pts',(-5.12725387,1.522118786,5.14119678));
#140411=CARTESIAN_POINT('Ctrl Pts',(-4.830724789,1.586734015,5.406162966));
#140412=CARTESIAN_POINT('Ctrl Pts',(-4.82046224915688,1.58897027580737,
5.4153331493484));
#140413=CARTESIAN_POINT('Ctrl Pts',(-4.81019970931389,1.59120653661473,
5.42450333269675));
#140414=CARTESIAN_POINT('Origin',(0.155686880664996,1.33939574493368,-0.113771102637439));
#140415=CARTESIAN_POINT('Ctrl Pts',(-4.811202304,1.586734015,5.753462644));
#140416=CARTESIAN_POINT('Ctrl Pts',(-4.499134977,1.521690237,6.01442185));
#140417=CARTESIAN_POINT('Ctrl Pts',(-4.160672677,1.456414446,6.240096384));
#140418=CARTESIAN_POINT('Ctrl Pts',(-4.830724789,1.586734015,5.406162966));
#140419=CARTESIAN_POINT('Ctrl Pts',(-4.537494967,1.521690237,5.66818106999999));
#140420=CARTESIAN_POINT('Ctrl Pts',(-4.217645127,1.456414446,5.89694578400001));
#140421=CARTESIAN_POINT('',(-4.22145735081421,1.45719264057815,5.8942173209189));
#140422=CARTESIAN_POINT('Origin',(0.119429677617468,1.48214300882117,-0.15966048512369));
#140423=CARTESIAN_POINT('Ctrl Pts',(-4.36636804309702,1.49654505833465,
6.09793654538808));
#140424=CARTESIAN_POINT('Ctrl Pts',(-4.34222209965503,1.49030358387838,
6.06392873275962));
#140425=CARTESIAN_POINT('Ctrl Pts',(-4.31806165314823,1.48390865066516,
6.02993010761874));
#140426=CARTESIAN_POINT('Ctrl Pts',(-4.26976703323237,1.47080219014011,
5.9620343526714));
#140427=CARTESIAN_POINT('Ctrl Pts',(-4.245604861298,1.4640830705707,5.92809785658239));
#140428=CARTESIAN_POINT('Ctrl Pts',(-4.22145735427668,1.45719264064155,
5.89421731921874));
#140429=CARTESIAN_POINT('Ctrl Pts',(-4.56926832085666,1.456406735,5.94809076502081));
#140430=CARTESIAN_POINT('Ctrl Pts',(-4.24301439628944,1.522118786,6.19871601337983));
#140431=CARTESIAN_POINT('Ctrl Pts',(-3.89130646372213,1.586734015,6.41215492265771));
#140432=CARTESIAN_POINT('Ctrl Pts',(-3.87913424555063,1.58897027580551,
6.41954180458288));
#140433=CARTESIAN_POINT('Ctrl Pts',(-3.86696202737906,1.59120653661107,
6.42692868650803));
#140434=CARTESIAN_POINT('Ctrl Pts',(-4.225323174,1.456406735,5.891446688));
#140435=CARTESIAN_POINT('Ctrl Pts',(-3.902176188,1.522118786,6.12320647800001));
#140436=CARTESIAN_POINT('Ctrl Pts',(-3.555619896,1.586734015,6.318232914));
#140437=CARTESIAN_POINT('Ctrl Pts',(-3.54362597034658,1.58897027580551,
6.32498256081882));
#140438=CARTESIAN_POINT('Ctrl Pts',(-3.5316320446931,1.59120653661108,6.33173220763764));
#140439=CARTESIAN_POINT('Origin',(0.127589615055193,1.33939577602722,-0.144579345888991));
#140440=CARTESIAN_POINT('Ctrl Pts',(-3.46189467,1.586734015,6.653216162));
#140441=CARTESIAN_POINT('Ctrl Pts',(-3.101024788,1.521690237,6.840989036));
#140442=CARTESIAN_POINT('Ctrl Pts',(-2.721962195,1.456414446,6.988628035));
#140443=CARTESIAN_POINT('Ctrl Pts',(-3.555619896,1.586734015,6.318232914));
#140444=CARTESIAN_POINT('Ctrl Pts',(-3.212919477,1.521690237,6.511089437));
#140445=CARTESIAN_POINT('Ctrl Pts',(-2.851369896,1.456414446,6.665747499));
#140446=CARTESIAN_POINT('',(-2.85567953178776,1.45719264062456,6.66390234040533));
#140447=CARTESIAN_POINT('Origin',(0.0823151945383094,1.48214303903916,-0.181601539638054));
#140448=CARTESIAN_POINT('Ctrl Pts',(-2.95340868090108,1.49654505841376,
6.89401023824042));
#140449=CARTESIAN_POINT('Ctrl Pts',(-2.93713793078994,1.49030358397024,
6.85560684540494));
#140450=CARTESIAN_POINT('Ctrl Pts',(-2.92085104149715,1.48390865071599,
6.81720930716423));
#140451=CARTESIAN_POINT('Ctrl Pts',(-2.88828110970201,1.47080219272414,
6.74051901626872));
#140452=CARTESIAN_POINT('Ctrl Pts',(-2.87197917614153,1.46408307188037,
6.70218177595652));
#140453=CARTESIAN_POINT('Ctrl Pts',(-2.8556795356562,1.45719264078122,6.66390233986534));
#140454=CARTESIAN_POINT('Ctrl Pts',(-3.18377767658021,1.456406735,6.79128533119686));
#140455=CARTESIAN_POINT('Ctrl Pts',(-2.81127436820566,1.522118786,6.96591615008536));
#140456=CARTESIAN_POINT('Ctrl Pts',(-2.42190611501465,1.586734015,7.09875816714877));
#140457=CARTESIAN_POINT('Ctrl Pts',(-2.4084305154338,1.58897027577805,7.10335568072313));
#140458=CARTESIAN_POINT('Ctrl Pts',(-2.39495491585294,1.59120653655611,
7.10795319429734));
#140459=CARTESIAN_POINT('Ctrl Pts',(-2.860050579,1.456406735,6.662027521));
#140460=CARTESIAN_POINT('Ctrl Pts',(-2.494637086,1.522118786,6.818901846));
#140461=CARTESIAN_POINT('Ctrl Pts',(-2.114258167,1.586734015,6.934869314));
#140462=CARTESIAN_POINT('Ctrl Pts',(-2.10109367821737,1.58897027577805,
6.93888281831208));
#140463=CARTESIAN_POINT('Ctrl Pts',(-2.08792918943474,1.59120653655611,
6.9428963226243));
#140464=CARTESIAN_POINT('Origin',(0.0935262382739294,1.33939574779353,-0.168626831068447));
#140465=CARTESIAN_POINT('Ctrl Pts',(-1.95071269,1.586734015,7.241872686));
#140466=CARTESIAN_POINT('Ctrl Pts',(-1.557914128,1.521690237,7.347679177));
#140467=CARTESIAN_POINT('Ctrl Pts',(-1.155975786,1.456414446,7.410379206));
#140468=CARTESIAN_POINT('Ctrl Pts',(-2.114258167,1.586734015,6.934869314));
#140469=CARTESIAN_POINT('Ctrl Pts',(-1.738111442,1.521690237,7.049546498));
#140470=CARTESIAN_POINT('Ctrl Pts',(-1.351767779,1.456414446,7.122866268));
#140471=CARTESIAN_POINT('',(-1.35637331164624,1.45719264058601,7.12199069254741));
#140472=CARTESIAN_POINT('Origin',(0.0413517804108662,1.48214301341937,-0.195051286303984));
#140473=CARTESIAN_POINT('Ctrl Pts',(-1.4023512112938,1.49654505835954,7.36772767377926));
#140474=CARTESIAN_POINT('Ctrl Pts',(-1.39471645654411,1.49030358393859,
7.32672440067643));
#140475=CARTESIAN_POINT('Ctrl Pts',(-1.38706468140528,1.48390865068783,
7.28572337574005));
#140476=CARTESIAN_POINT('Ctrl Pts',(-1.37174236273163,1.47080219302608,
7.20382449064787));
#140477=CARTESIAN_POINT('Ctrl Pts',(-1.36406293274997,1.46408307201767,
7.16287911879417));
#140478=CARTESIAN_POINT('Ctrl Pts',(-1.35637331617947,1.45719264075502,
7.12199069281731));
#140479=CARTESIAN_POINT('Ctrl Pts',(-1.64941712647212,1.456406735,7.31692694226868));
#140480=CARTESIAN_POINT('Ctrl Pts',(-1.24808227386318,1.522118786,7.40739779012271));
#140481=CARTESIAN_POINT('Ctrl Pts',(-0.839260127710371,1.586734015,7.45343136981124));
#140482=CARTESIAN_POINT('Ctrl Pts',(-0.82511125043235,1.58897027581419,
7.45502454052325));
#140483=CARTESIAN_POINT('Ctrl Pts',(-0.810962373154327,1.59120653662838,
7.45661771123534));
#140484=CARTESIAN_POINT('Ctrl Pts',(-1.361045197,1.456406735,7.121099351));
#140485=CARTESIAN_POINT('Ctrl Pts',(-0.970451525,1.522118786,7.195752943));
#140486=CARTESIAN_POINT('Ctrl Pts',(-0.574036077000001,1.586734015,7.227238932));
#140487=CARTESIAN_POINT('Ctrl Pts',(-0.560316581670197,1.58897027581419,
7.22832862686738));
#140488=CARTESIAN_POINT('Ctrl Pts',(-0.546597086340393,1.59120653662838,
7.22941832173478));
#140489=CARTESIAN_POINT('Origin',(0.0550898964041995,1.33939576732543,-0.184790043833353));
#140490=CARTESIAN_POINT('Ctrl Pts',(-0.348317552,1.586734015,7.491907293));
#140491=CARTESIAN_POINT('Ctrl Pts',(0.0580428659999999,1.521690237,7.510800007));
#140492=CARTESIAN_POINT('Ctrl Pts',(0.464062765,1.456414446,7.485629282));
#140493=CARTESIAN_POINT('Ctrl Pts',(-0.574036077,1.586734015,7.227238932));
#140494=CARTESIAN_POINT('Ctrl Pts',(-0.182031249,1.521690237,7.2583746));
#140495=CARTESIAN_POINT('Ctrl Pts',(0.211041498,1.456414446,7.246927727));
#140496=CARTESIAN_POINT('Origin',(-0.00154525971137284,1.48214304894328,
-0.19938049318742));
#140497=CARTESIAN_POINT('Ctrl Pts',(-1.35776704393169,4.30075163058632,
7.12172944830897));
#140498=CARTESIAN_POINT('Ctrl Pts',(-1.35390884396585,4.30138922829316,
7.12246068865448));
#140499=CARTESIAN_POINT('Ctrl Pts',(-1.350050644,4.302026826,7.12319192899999));
#140500=CARTESIAN_POINT('Ctrl Pts',(-0.962010097,4.36615356,7.196736822));
#140501=CARTESIAN_POINT('Ctrl Pts',(-0.568276727,4.431389364,7.227694069));
#140502=CARTESIAN_POINT('Ctrl Pts',(-1.16221715234734,4.30075163058632,
7.4094073516114));
#140503=CARTESIAN_POINT('Ctrl Pts',(-1.15820324967367,4.30138922829316,
7.4100325058057));
#140504=CARTESIAN_POINT('Ctrl Pts',(-1.154189347,4.302026826,7.41065766));
#140505=CARTESIAN_POINT('Ctrl Pts',(-0.750488916,4.36615356,7.473532881));
#140506=CARTESIAN_POINT('Ctrl Pts',(-0.342347366,4.431389364,7.492182478));
#140507=CARTESIAN_POINT('',(-0.572986203456379,4.43060907981178,7.22732224112228));
#140508=CARTESIAN_POINT('Ctrl Pts',(-0.572986202613025,4.43060907940012,
7.22732224306242));
#140509=CARTESIAN_POINT('Ctrl Pts',(-0.575775813424748,4.42401550332526,
7.26754705881263));
#140510=CARTESIAN_POINT('Ctrl Pts',(-0.57866334130313,4.41742229674867,
7.30876626432251));
#140511=CARTESIAN_POINT('Ctrl Pts',(-0.584752497706469,4.40420945810707,
7.39349824679339));
#140512=CARTESIAN_POINT('Ctrl Pts',(-0.587799206996747,4.39788077308853,
7.43509547553819));
#140513=CARTESIAN_POINT('Ctrl Pts',(-0.590897510188735,4.39169923734407,
7.47668644070131));
#140514=CARTESIAN_POINT('Origin',(-0.0051813612548729,4.55345288605838,
-0.19241258054202));
#140515=CARTESIAN_POINT('Ctrl Pts',(-2.117742488,4.431369595,6.93380608));
#140516=CARTESIAN_POINT('Ctrl Pts',(-2.10947844,4.429970133,6.936330109));
#140517=CARTESIAN_POINT('Ctrl Pts',(-2.1012084,4.428571429,6.938834431));
#140518=CARTESIAN_POINT('Ctrl Pts',(-1.730553477,4.365882895,7.05107565));
#140519=CARTESIAN_POINT('Ctrl Pts',(-1.350050644,4.302026826,7.123191929));
#140520=CARTESIAN_POINT('Ctrl Pts',(-2.424827999,4.431369595,7.097197276));
#140521=CARTESIAN_POINT('Ctrl Pts',(-2.416369214,4.429970133,7.100087304));
#140522=CARTESIAN_POINT('Ctrl Pts',(-2.407903564,4.428571429,7.102957161));
#140523=CARTESIAN_POINT('Ctrl Pts',(-2.028481621,4.365882895,7.231581257));
#140524=CARTESIAN_POINT('Ctrl Pts',(-1.637516375,4.302026826,7.319053226));
#140525=CARTESIAN_POINT('',(-2.11325074782748,4.43060907981219,6.93517636705374));
#140526=CARTESIAN_POINT('Origin',(0.0123907588393973,4.16114693626522,-0.190611787166877));
#140527=CARTESIAN_POINT('Ctrl Pts',(-2.18434923030009,4.39169923736146,
7.17486016828095));
#140528=CARTESIAN_POINT('Ctrl Pts',(-2.17238253565825,4.39788077311386,
7.1349076203884));
#140529=CARTESIAN_POINT('Ctrl Pts',(-2.16046488222165,4.4042094581219,7.09493786428154));
#140530=CARTESIAN_POINT('Ctrl Pts',(-2.13630354384551,4.41742211712242,
7.01349696440219));
#140531=CARTESIAN_POINT('Ctrl Pts',(-2.12462260024002,4.42401532021671,
6.97386214323707));
#140532=CARTESIAN_POINT('Ctrl Pts',(-2.11325074774409,4.4306090792906,6.9351763699027));
#140533=CARTESIAN_POINT('Ctrl Pts',(-2.85698451967887,4.30075163058632,
6.66334759239431));
#140534=CARTESIAN_POINT('Ctrl Pts',(-2.85337371733943,4.30138922829316,
6.66489113569716));
#140535=CARTESIAN_POINT('Ctrl Pts',(-2.849762915,4.302026826,6.666434679));
#140536=CARTESIAN_POINT('Ctrl Pts',(-2.486604518,4.36615356,6.821677381));
#140537=CARTESIAN_POINT('Ctrl Pts',(-2.108731308,4.431389364,6.93655190100001));
#140538=CARTESIAN_POINT('Ctrl Pts',(-2.72784872138814,4.30075163058632,
6.98633719228998));
#140539=CARTESIAN_POINT('Ctrl Pts',(-2.72406305119407,4.30138922829316,
6.98781060114499));
#140540=CARTESIAN_POINT('Ctrl Pts',(-2.720277381,4.302026826,6.98928401000001));
#140541=CARTESIAN_POINT('Ctrl Pts',(-2.339531555,4.36615356,7.137472902));
#140542=CARTESIAN_POINT('Ctrl Pts',(-1.944941241,4.431389364,7.243424851));
#140543=CARTESIAN_POINT('Origin',(0.0363027951225431,4.55345288672837,-0.189027909640508));
#140544=CARTESIAN_POINT('Ctrl Pts',(-3.558794191,4.431369595,6.316445512));
#140545=CARTESIAN_POINT('Ctrl Pts',(-3.551265944,4.429970133,6.320687056));
#140546=CARTESIAN_POINT('Ctrl Pts',(-3.543727607,4.428571429,6.324910643));
#140547=CARTESIAN_POINT('Ctrl Pts',(-3.205866935,4.365882895,6.514207577));
#140548=CARTESIAN_POINT('Ctrl Pts',(-2.849762915,4.302026826,6.666434679));
#140549=CARTESIAN_POINT('Ctrl Pts',(-3.89382449,4.431369595,6.410002406));
#140550=CARTESIAN_POINT('Ctrl Pts',(-3.886184737,4.429970133,6.414643255));
#140551=CARTESIAN_POINT('Ctrl Pts',(-3.878533944,4.428571429,6.419265881));
#140552=CARTESIAN_POINT('Ctrl Pts',(-3.535633054,4.365882895,6.626447319));
#140553=CARTESIAN_POINT('Ctrl Pts',(-3.172612246,4.302026826,6.795920213));
#140554=CARTESIAN_POINT('',(-3.55470203688038,4.43060907982634,6.3187493536364));
#140555=CARTESIAN_POINT('Origin',(0.053076451612849,4.16114717394356,-0.183490596981692));
#140556=CARTESIAN_POINT('Ctrl Pts',(-3.67566320760579,4.39169923737812,
6.53754540923891));
#140557=CARTESIAN_POINT('Ctrl Pts',(-3.65538767083827,4.39788077313931,
6.50109941524975));
#140558=CARTESIAN_POINT('Ctrl Pts',(-3.63515632942581,4.40420945817687,
6.46462607283171));
#140559=CARTESIAN_POINT('Ctrl Pts',(-3.5940520600491,4.417422253397,6.39028242292873));
#140560=CARTESIAN_POINT('Ctrl Pts',(-3.57412391075028,4.42401545916239,
6.35408531972618));
#140561=CARTESIAN_POINT('Ctrl Pts',(-3.55470203703904,4.43060907932611,
6.31874935621956));
#140562=CARTESIAN_POINT('Ctrl Pts',(-4.22261257419804,4.30075163058632,
5.89339500821418));
#140563=CARTESIAN_POINT('Ctrl Pts',(-4.21941800659903,4.30138922829316,
5.89567868010709));
#140564=CARTESIAN_POINT('Ctrl Pts',(-4.216223439,4.302026826,5.897962352));
#140565=CARTESIAN_POINT('Ctrl Pts',(-3.894928076,4.36615356,6.127643887));
#140566=CARTESIAN_POINT('Ctrl Pts',(-3.550583958,4.431389364,6.321064274));
#140567=CARTESIAN_POINT('Ctrl Pts',(-4.16592911596048,4.30075163058632,
6.23659367087182));
#140568=CARTESIAN_POINT('Ctrl Pts',(-4.16254869198024,4.30138922829316,
6.23884643943591));
#140569=CARTESIAN_POINT('Ctrl Pts',(-4.159168268,4.302026826,6.241099208));
#140570=CARTESIAN_POINT('Ctrl Pts',(-3.819180299,4.36615356,6.46767262400001));
#140571=CARTESIAN_POINT('Ctrl Pts',(-3.456591824,4.431389364,6.655972728));
#140572=CARTESIAN_POINT('Origin',(0.0760893310981942,4.55345288953098,-0.176804295814729));
#140573=CARTESIAN_POINT('Ctrl Pts',(-4.833440632,4.431369595,5.403734972));
#140574=CARTESIAN_POINT('Ctrl Pts',(-4.827000198,4.429970133,5.409495702));
#140575=CARTESIAN_POINT('Ctrl Pts',(-4.82054605,4.428571429,5.415241063));
#140576=CARTESIAN_POINT('Ctrl Pts',(-4.531277618,4.365882895,5.672742398));
#140577=CARTESIAN_POINT('Ctrl Pts',(-4.216223439,4.302026826,5.897962352));
#140578=CARTESIAN_POINT('Ctrl Pts',(-5.18075007600001,4.431369595,5.42308294700001));
#140579=CARTESIAN_POINT('Ctrl Pts',(-5.174286582,4.429970133,5.429257617));
#140580=CARTESIAN_POINT('Ctrl Pts',(-5.167808388,4.428571429,5.435416862));
#140581=CARTESIAN_POINT('Ctrl Pts',(-4.877462215,4.365882895,5.711468069));
#140582=CARTESIAN_POINT('Ctrl Pts',(-4.559360294,4.302026826,5.955017524));
#140583=CARTESIAN_POINT('',(-4.82993940821837,4.43060907984581,5.40686464364233));
#140584=CARTESIAN_POINT('Origin',(0.0912803947604635,4.16114721112737,-0.1677905457368));
#140585=CARTESIAN_POINT('Ctrl Pts',(-4.99510725948457,4.39169923740419,
5.59454229236904));
#140586=CARTESIAN_POINT('Ctrl Pts',(-4.96747094198499,4.3978807731843,5.56330702642334));
#140587=CARTESIAN_POINT('Ctrl Pts',(-4.93987190779603,4.40420945816489,
5.53203555112992));
#140588=CARTESIAN_POINT('Ctrl Pts',(-4.88374728278851,4.41742217412659,
5.46826659984238));
#140589=CARTESIAN_POINT('Ctrl Pts',(-4.8565037268247,4.42401537766957,5.43719972099938));
#140590=CARTESIAN_POINT('Ctrl Pts',(-4.82993941000097,4.43060907926912,
5.40686464621053));
#140591=CARTESIAN_POINT('Ctrl Pts',(-5.39079595785797,4.30075163058632,
4.84787382396709));
#140592=CARTESIAN_POINT('Ctrl Pts',(-5.38816699942899,4.30138922829316,
4.85079084248355));
#140593=CARTESIAN_POINT('Ctrl Pts',(-5.38553804100001,4.302026826,4.853707861));
#140594=CARTESIAN_POINT('Ctrl Pts',(-5.121129126,4.36615356,5.147088575));
#140595=CARTESIAN_POINT('Ctrl Pts',(-4.826415248,4.431389364,5.410010708));
#140596=CARTESIAN_POINT('Ctrl Pts',(-5.40921529476771,4.30075163058632,
5.19523396035998));
#140597=CARTESIAN_POINT('Ctrl Pts',(-5.40639818188385,4.30138922829316,
5.19816075168));
#140598=CARTESIAN_POINT('Ctrl Pts',(-5.403581069,4.302026826,5.201087543));
#140599=CARTESIAN_POINT('Ctrl Pts',(-5.12024841800001,4.36615356,5.495451162));
#140600=CARTESIAN_POINT('Ctrl Pts',(-4.806616016,4.431389364,5.757294719));
#140601=CARTESIAN_POINT('Origin',(0.112318141206794,4.55345288046685,-0.156313780444495));
#140602=CARTESIAN_POINT('Ctrl Pts',(-5.882080762,4.431369595,4.238351791));
#140603=CARTESIAN_POINT('Ctrl Pts',(-5.87702928800001,4.429970133,4.245362341));
#140604=CARTESIAN_POINT('Ctrl Pts',(-5.871961118,4.428571429,4.25236083));
#140605=CARTESIAN_POINT('Ctrl Pts',(-5.64481079600001,4.365882895,4.566026089));
#140606=CARTESIAN_POINT('Ctrl Pts',(-5.38553804100001,4.302026826,4.853707861));
#140607=CARTESIAN_POINT('Ctrl Pts',(-6.225429547,4.431369595,4.182586157));
#140608=CARTESIAN_POINT('Ctrl Pts',(-6.220444537,4.429970133,4.190005926));
#140609=CARTESIAN_POINT('Ctrl Pts',(-6.215441855,4.428571429,4.197413792));
#140610=CARTESIAN_POINT('Ctrl Pts',(-5.991226664,4.365882895,4.52942692));
#140611=CARTESIAN_POINT('Ctrl Pts',(-5.732917723,4.302026826,4.835664834));
#140612=CARTESIAN_POINT('',(-5.87933418163029,4.43060907985417,4.2421609519141));
#140613=CARTESIAN_POINT('Origin',(0.125218936516226,4.16114644057551,-0.144247389551539));
#140614=CARTESIAN_POINT('Ctrl Pts',(-6.08098564645014,4.39169923736635,
4.38994459618127));
#140615=CARTESIAN_POINT('Ctrl Pts',(-6.04728079196535,4.39788077313033,
4.36538058482446));
#140616=CARTESIAN_POINT('Ctrl Pts',(-6.01360456489737,4.40420945815512,
4.34077319563697));
#140617=CARTESIAN_POINT('Ctrl Pts',(-5.94508333958322,4.41742223651246,
4.29056002530658));
#140618=CARTESIAN_POINT('Ctrl Pts',(-5.91179827121222,4.42401544155975,
4.26607603671574));
#140619=CARTESIAN_POINT('Ctrl Pts',(-5.87933418351883,4.43060907933619,
4.2421609540683));
#140620=CARTESIAN_POINT('Ctrl Pts',(-6.30691171418917,4.30075163058632,
3.57567144780525));
#140621=CARTESIAN_POINT('Ctrl Pts',(-6.30497129209458,4.30138922829316,
3.57908541640262));
#140622=CARTESIAN_POINT('Ctrl Pts',(-6.30303087,4.302026826,3.582499385));
#140623=CARTESIAN_POINT('Ctrl Pts',(-6.107871869,4.36615356,3.925861122));
#140624=CARTESIAN_POINT('Ctrl Pts',(-5.876568725,4.431389364,4.245991053));
#140625=CARTESIAN_POINT('Ctrl Pts',(-6.399572578477,4.30075163058632,3.91095088387329));
#140626=CARTESIAN_POINT('Ctrl Pts',(-6.3974505017385,4.30138922829316,3.91441484443665));
#140627=CARTESIAN_POINT('Ctrl Pts',(-6.39532842500001,4.302026826,3.917878805));
#140628=CARTESIAN_POINT('Ctrl Pts',(-6.18189941,4.36615356,4.266268511));
#140629=CARTESIAN_POINT('Ctrl Pts',(-5.931888184,4.431389364,4.589412007));
#140630=CARTESIAN_POINT('Origin',(0.143295128420577,4.55345292751047,-0.128514236351981));
#140631=CARTESIAN_POINT('Ctrl Pts',(-6.65244799782001,4.431369595,2.87607070805));
#140632=CARTESIAN_POINT('Ctrl Pts',(-6.64902015702,4.429970133,2.8839994194));
#140633=CARTESIAN_POINT('Ctrl Pts',(-6.64557342641,4.428571429,2.89191993712));
#140634=CARTESIAN_POINT('Ctrl Pts',(-6.49109440281,4.365882895,3.24690960173));
#140635=CARTESIAN_POINT('Ctrl Pts',(-6.2996770758,4.302026826,3.58342236054));
#140636=CARTESIAN_POINT('Ctrl Pts',(-6.655681333,4.431369595,2.874787991));
#140637=CARTESIAN_POINT('Ctrl Pts',(-6.652255021,4.429970133,2.882720556));
#140638=CARTESIAN_POINT('Ctrl Pts',(-6.64880981,4.428571429,2.890644931));
#140639=CARTESIAN_POINT('Ctrl Pts',(-6.494398894,4.365882895,3.245807475));
#140640=CARTESIAN_POINT('Ctrl Pts',(-6.30303087,4.302026826,3.582499385));
#140641=CARTESIAN_POINT('Ctrl Pts',(-6.979014851,4.431369595,2.746516286));
#140642=CARTESIAN_POINT('Ctrl Pts',(-6.975741419,4.429970133,2.754834216));
#140643=CARTESIAN_POINT('Ctrl Pts',(-6.972448169,4.428571429,2.763144319));
#140644=CARTESIAN_POINT('Ctrl Pts',(-6.824848013,4.365882895,3.135594802));
#140645=CARTESIAN_POINT('Ctrl Pts',(-6.63841029,4.302026826,3.490201831));
#140646=CARTESIAN_POINT('',(-6.65381782292298,4.43060907982855,2.87909852931941));
#140647=CARTESIAN_POINT('Origin',(0.153300462456629,4.16114644726734,-0.113956670212826));
#140648=CARTESIAN_POINT('Ctrl Pts',(-6.88252390360049,4.39169923737952,
2.98007796986011));
#140649=CARTESIAN_POINT('Ctrl Pts',(-6.84432651354025,4.3978807731492,2.96333379889397));
#140650=CARTESIAN_POINT('Ctrl Pts',(-6.80614775662989,4.40420945817943,
2.94654111021513));
#140651=CARTESIAN_POINT('Ctrl Pts',(-6.7284342824622,4.41742221776468,2.91223198283376));
#140652=CARTESIAN_POINT('Ctrl Pts',(-6.69066405869933,4.42401542328448,
2.89547571962815));
#140653=CARTESIAN_POINT('Ctrl Pts',(-6.6538178243887,4.43060907942241,2.87909853129467));
#140654=CARTESIAN_POINT('Ctrl Pts',(-6.92812328853911,4.30075163058632,
2.13627464941378));
#140655=CARTESIAN_POINT('Ctrl Pts',(-6.92696213476955,4.30138922829316,
2.14002593470689));
#140656=CARTESIAN_POINT('Ctrl Pts',(-6.925800981,4.302026826,2.14377722));
#140657=CARTESIAN_POINT('Ctrl Pts',(-6.809017313,4.36615356,2.521064766));
#140658=CARTESIAN_POINT('Ctrl Pts',(-6.651940379,4.431389364,2.883433576));
#140659=CARTESIAN_POINT('Ctrl Pts',(-7.09069296127744,4.30075163058632,
2.44379609126981));
#140660=CARTESIAN_POINT('Ctrl Pts',(-7.08936514663872,4.30138922829316,
2.44763525013491));
#140661=CARTESIAN_POINT('Ctrl Pts',(-7.088037332,4.302026826,2.451474409));
#140662=CARTESIAN_POINT('Ctrl Pts',(-6.954491657,4.36615356,2.837599887));
#140663=CARTESIAN_POINT('Ctrl Pts',(-6.779791854,4.431389364,3.20693349));
#140664=CARTESIAN_POINT('Origin',(0.167571566098508,4.55345287895314,-0.0947053690531868));
#140665=CARTESIAN_POINT('Ctrl Pts',(-7.118069642,4.431369595,1.376802299));
#140666=CARTESIAN_POINT('Ctrl Pts',(-7.116428702,4.429970133,1.385285961));
#140667=CARTESIAN_POINT('Ctrl Pts',(-7.114767544,4.428571429,1.393765687));
#140668=CARTESIAN_POINT('Ctrl Pts',(-7.040316119,4.365882895,1.77381851));
#140669=CARTESIAN_POINT('Ctrl Pts',(-6.925800981,4.302026826,2.14377722));
#140670=CARTESIAN_POINT('Ctrl Pts',(-7.406269177,4.431369595,1.182022367));
#140671=CARTESIAN_POINT('Ctrl Pts',(-7.404860385,4.429970133,1.190849519));
#140672=CARTESIAN_POINT('Ctrl Pts',(-7.403430556,4.428571429,1.199673288));
#140673=CARTESIAN_POINT('Ctrl Pts',(-7.339347054,4.365882895,1.595145757));
#140674=CARTESIAN_POINT('Ctrl Pts',(-7.233498171,4.302026826,1.981540869));
#140675=CARTESIAN_POINT('',(-7.11717633793565,4.43060907981108,1.38141265923023));
#140676=CARTESIAN_POINT('Origin',(0.174211298471878,4.16114702584248,-0.0783366564974439));
#140677=CARTESIAN_POINT('Ctrl Pts',(-7.36224299279149,4.39169923741886,
1.43086620946198));
#140678=CARTESIAN_POINT('Ctrl Pts',(-7.32133913467307,4.39788077316404,
1.42272481765021));
#140679=CARTESIAN_POINT('Ctrl Pts',(-7.28044304443845,4.40420945813066,
1.41453203690386));
#140680=CARTESIAN_POINT('Ctrl Pts',(-7.19717121000547,4.41742218750417,
1.39773117588273));
#140681=CARTESIAN_POINT('Ctrl Pts',(-7.15668193244824,4.4240153913157,1.38948614686132));
#140682=CARTESIAN_POINT('Ctrl Pts',(-7.11717634035813,4.4306090793536,1.38141266056319));
#140683=CARTESIAN_POINT('Ctrl Pts',(-7.2253835183998,4.30075163058632,0.596988021858047));
#140684=CARTESIAN_POINT('Ctrl Pts',(-7.22505592719991,4.30138922829316,
0.600901217929024));
#140685=CARTESIAN_POINT('Ctrl Pts',(-7.224728336,4.302026826,0.604814414));
#140686=CARTESIAN_POINT('Ctrl Pts',(-7.191780674,4.36615356,0.998386223999999));
#140687=CARTESIAN_POINT('Ctrl Pts',(-7.116274695,4.431389364,1.38604995));
#140688=CARTESIAN_POINT('Ctrl Pts',(-7.45026042179122,4.30075163058632,
0.862372109285386));
#140689=CARTESIAN_POINT('Ctrl Pts',(-7.44978895639561,4.30138922829316,
0.866406951642693));
#140690=CARTESIAN_POINT('Ctrl Pts',(-7.449317491,4.302026826,0.870441794));
#140691=CARTESIAN_POINT('Ctrl Pts',(-7.401899604,4.36615356,1.276248245));
#140692=CARTESIAN_POINT('Ctrl Pts',(-7.310679993,4.431389364,1.674502328));
#140693=CARTESIAN_POINT('Origin',(0.184013027002503,4.55345292796302,-0.0564683324674287));
#140694=CARTESIAN_POINT('Ctrl Pts',(-7.247624926,4.431369595,-0.185561138));
#140695=CARTESIAN_POINT('Ctrl Pts',(-7.247846087,4.429970133,-0.176923066));
#140696=CARTESIAN_POINT('Ctrl Pts',(-7.248046656,4.428571429,-0.168284491));
#140697=CARTESIAN_POINT('Ctrl Pts',(-7.257035987,4.365882895,0.218887764));
#140698=CARTESIAN_POINT('Ctrl Pts',(-7.224728336,4.302026826,0.604814414));
#140699=CARTESIAN_POINT('Ctrl Pts',(-7.487214588,4.431369595,-0.437741604));
#140700=CARTESIAN_POINT('Ctrl Pts',(-7.48773631,4.429970133,-0.428817978));
#140701=CARTESIAN_POINT('Ctrl Pts',(-7.488236759,4.428571429,-0.419893133));
#140702=CARTESIAN_POINT('Ctrl Pts',(-7.510666384,4.365882895,-0.019890532));
#140703=CARTESIAN_POINT('Ctrl Pts',(-7.490355716,4.302026826,0.380225258));
#140704=CARTESIAN_POINT('',(-7.24774359797091,4.43060907983566,-0.180866531823111));
#140705=CARTESIAN_POINT('Origin',(0.186975432915708,4.16114763470212,-0.0390547221848561));
#140706=CARTESIAN_POINT('Ctrl Pts',(-7.49771178198432,4.39169923736833,
-0.185251264675212));
#140707=CARTESIAN_POINT('Ctrl Pts',(-7.45601407454653,4.39788077315963,
-0.184409194783559));
#140708=CARTESIAN_POINT('Ctrl Pts',(-7.41431290627343,4.40420945817067,
-0.183618982244392));
#140709=CARTESIAN_POINT('Ctrl Pts',(-7.32937619817061,4.41742219290252,
-0.182126064751352));
#140710=CARTESIAN_POINT('Ctrl Pts',(-7.28806110256997,4.42401539652318,
-0.181474331916151));
#140711=CARTESIAN_POINT('Ctrl Pts',(-7.24774360024735,4.43060907935805,
-0.180866530270858));
#140712=CARTESIAN_POINT('Ctrl Pts',(-7.18479284462103,4.30075163058632,
-0.970213102287846));
#140713=CARTESIAN_POINT('Ctrl Pts',(-7.18531413381051,4.30138922829316,
-0.966320972143922));
#140714=CARTESIAN_POINT('Ctrl Pts',(-7.185835423,4.302026826,-0.962428842));
#140715=CARTESIAN_POINT('Ctrl Pts',(-7.238264365,4.36615356,-0.570975749));
#140716=CARTESIAN_POINT('Ctrl Pts',(-7.24785991500001,4.431389364,-0.176143831));
#140717=CARTESIAN_POINT('Ctrl Pts',(-7.46146198490312,4.30075163058632,
-0.759375434223065));
#140718=CARTESIAN_POINT('Ctrl Pts',(-7.46186891395157,4.30138922829316,
-0.755333573111533));
#140719=CARTESIAN_POINT('Ctrl Pts',(-7.462275843,4.302026826,-0.751291712));
#140720=CARTESIAN_POINT('Ctrl Pts',(-7.503202952,4.36615356,-0.344779346));
#140721=CARTESIAN_POINT('Ctrl Pts',(-7.49972886,4.431389364,0.063773298));
#140722=CARTESIAN_POINT('Origin',(0.191849688360268,4.55345288722648,-0.0155907848465334));
#140723=CARTESIAN_POINT('Ctrl Pts',(-7.038289323,4.431369595,-1.739247943));
#140724=CARTESIAN_POINT('Ctrl Pts',(-7.040362243,4.429970133,-1.730859367));
#140725=CARTESIAN_POINT('Ctrl Pts',(-7.042415162,4.428571429,-1.722465874));
#140726=CARTESIAN_POINT('Ctrl Pts',(-7.134424917,4.365882895,-1.346277931));
#140727=CARTESIAN_POINT('Ctrl Pts',(-7.185835423,4.302026826,-0.962428842));
#140728=CARTESIAN_POINT('Ctrl Pts',(-7.218066166,4.431369595,-2.037037265));
#140729=CARTESIAN_POINT('Ctrl Pts',(-7.220494006,4.429970133,-2.028434422));
#140730=CARTESIAN_POINT('Ctrl Pts',(-7.222901333,4.428571429,-2.019825817));
#140731=CARTESIAN_POINT('Ctrl Pts',(-7.330795302,4.365882895,-1.633996761));
#140732=CARTESIAN_POINT('Ctrl Pts',(-7.396972553,4.302026826,-1.238869262));
#140733=CARTESIAN_POINT('',(-7.03941442235693,4.4306090798324,-1.73468860429048));
#140734=CARTESIAN_POINT('Origin',(0.191005240678206,4.16114639188231,0.00205339969632512));
#140735=CARTESIAN_POINT('Ctrl Pts',(-7.28259590116914,4.39169923740785,
-1.79270659508165));
#140736=CARTESIAN_POINT('Ctrl Pts',(-7.24205408327968,4.39788077315036,
-1.7829204379314));
#140737=CARTESIAN_POINT('Ctrl Pts',(-7.20149773745199,4.40420945814961,
-1.773184181719));
#140738=CARTESIAN_POINT('Ctrl Pts',(-7.1188672875784,4.41742226448833,-1.75346717962484));
#140739=CARTESIAN_POINT('Ctrl Pts',(-7.07865822430606,4.42401547082464,
-1.74394916249829));
#140740=CARTESIAN_POINT('Ctrl Pts',(-7.03941442481537,4.43060907931634,
-1.73468860419115));
#140741=CARTESIAN_POINT('Ctrl Pts',(-6.80824924266725,4.30075163058632,
-2.49204813906551));
#140742=CARTESIAN_POINT('Ctrl Pts',(-6.80959503733362,4.30138922829316,
-2.48835906653276));
#140743=CARTESIAN_POINT('Ctrl Pts',(-6.81094083200001,4.302026826,-2.484669994));
#140744=CARTESIAN_POINT('Ctrl Pts',(-6.946294858,4.36615356,-2.11363953));
#140745=CARTESIAN_POINT('Ctrl Pts',(-7.040543261,4.431389364,-1.730101323));
#140746=CARTESIAN_POINT('Ctrl Pts',(-7.12377387913241,4.30075163058632,
-2.3456154258534));
#140747=CARTESIAN_POINT('Ctrl Pts',(-7.12504017506621,4.30138922829316,
-2.3417555389267));
#140748=CARTESIAN_POINT('Ctrl Pts',(-7.126306471,4.302026826,-2.337895652));
#140749=CARTESIAN_POINT('Ctrl Pts',(-7.253664869,4.36615356,-1.949685438));
#140750=CARTESIAN_POINT('Ctrl Pts',(-7.33809874,4.431389364,-1.549937701));
#140751=CARTESIAN_POINT('Origin',(0.190715988738417,4.55345289011465,0.0260157603670164));
#140752=CARTESIAN_POINT('Ctrl Pts',(-6.499851134,4.431369595,-3.211609446));
#140753=CARTESIAN_POINT('Ctrl Pts',(-6.503678886,4.429970133,-3.203862607));
#140754=CARTESIAN_POINT('Ctrl Pts',(-6.507488162,4.428571429,-3.196106666));
#140755=CARTESIAN_POINT('Ctrl Pts',(-6.678216068,4.365882895,-2.848493166));
#140756=CARTESIAN_POINT('Ctrl Pts',(-6.810940832,4.302026826,-2.484669994));
#140757=CARTESIAN_POINT('Ctrl Pts',(-6.611408993,4.431369595,-3.541083327));
#140758=CARTESIAN_POINT('Ctrl Pts',(-6.615629428,4.429970133,-3.533203528));
#140759=CARTESIAN_POINT('Ctrl Pts',(-6.619831069,4.428571429,-3.525313691));
#140760=CARTESIAN_POINT('Ctrl Pts',(-6.80814437800001,4.365882895,-3.171699118));
#140761=CARTESIAN_POINT('Ctrl Pts',(-6.957715175,4.302026826,-2.800035633));
#140762=CARTESIAN_POINT('',(-6.50193005203167,4.43060907982022,-3.2073985659925));
#140763=CARTESIAN_POINT('Origin',(0.186097995353229,4.16114642092722,0.043065778632051));
#140764=CARTESIAN_POINT('Ctrl Pts',(-6.72695393012471,4.39169923738952,
-3.31633695786171));
#140765=CARTESIAN_POINT('Ctrl Pts',(-6.68946369205208,4.39788077312887,
-3.29806430321486));
#140766=CARTESIAN_POINT('Ctrl Pts',(-6.65194853850495,4.40420945811866,
-3.27983725979241));
#140767=CARTESIAN_POINT('Ctrl Pts',(-6.57548829283599,4.41742230292223,
-3.24281801837052));
#140768=CARTESIAN_POINT('Ctrl Pts',(-6.53826539478635,4.42401550976215,
-3.22487877186494));
#140769=CARTESIAN_POINT('Ctrl Pts',(-6.50193005463137,4.43060907935782,
-3.20739856646714));
#140770=CARTESIAN_POINT('Ctrl Pts',(-6.11335947344275,4.30075163058632,
-3.89735777600252));
#140771=CARTESIAN_POINT('Ctrl Pts',(-6.11546684572138,4.30138922829316,
-3.89404425800126));
#140772=CARTESIAN_POINT('Ctrl Pts',(-6.117574218,4.30202682600001,-3.89073074));
#140773=CARTESIAN_POINT('Ctrl Pts',(-6.329524324,4.36615356,-3.557471876));
#140774=CARTESIAN_POINT('Ctrl Pts',(-6.504018629,4.431389364,-3.2031612));
#140775=CARTESIAN_POINT('Ctrl Pts',(-6.45298602455971,4.30075163058632,
-3.8221770474411));
#140776=CARTESIAN_POINT('Ctrl Pts',(-6.45505247677986,4.30138922829316,
-3.81867961872055));
#140777=CARTESIAN_POINT('Ctrl Pts',(-6.457118929,4.30202682600001,-3.81518219));
#140778=CARTESIAN_POINT('Ctrl Pts',(-6.664953478,4.36615356,-3.463426406));
#140779=CARTESIAN_POINT('Ctrl Pts',(-6.83334728,4.431389364,-3.091175335));
#140780=CARTESIAN_POINT('Origin',(0.180664648443238,4.55345290995932,0.0664058816356417));
#140781=CARTESIAN_POINT('Ctrl Pts',(-5.65748713,4.431369595,-4.533799662));
#140782=CARTESIAN_POINT('Ctrl Pts',(-5.662890733,4.429970133,-4.527056793));
#140783=CARTESIAN_POINT('Ctrl Pts',(-5.668278248,4.428571429,-4.520301063));
#140784=CARTESIAN_POINT('Ctrl Pts',(-5.90974125700001,4.365882895,-4.217516027));
#140785=CARTESIAN_POINT('Ctrl Pts',(-6.11757421800001,4.302026826,-3.89073074));
#140786=CARTESIAN_POINT('Ctrl Pts',(-5.695609683,4.431369595,-4.879552268));
#140787=CARTESIAN_POINT('Ctrl Pts',(-5.701425371,4.429970133,-4.872763963));
#140788=CARTESIAN_POINT('Ctrl Pts',(-5.707224861,4.428571429,-4.865961815));
#140789=CARTESIAN_POINT('Ctrl Pts',(-5.96715219,4.365882895,-4.561096349));
#140790=CARTESIAN_POINT('Ctrl Pts',(-6.193122768,4.302026826,-4.23027545));
#140791=CARTESIAN_POINT('',(-5.66042265901053,4.43060907979696,-4.53013413550827));
#140792=CARTESIAN_POINT('Origin',(0.172489379695488,4.16114643978824,0.0820645868625702));
#140793=CARTESIAN_POINT('Ctrl Pts',(-5.85676706945755,4.39169923740779,
-4.68489909035697));
#140794=CARTESIAN_POINT('Ctrl Pts',(-5.82408141295841,4.39788077313851,
-4.65899434735462));
#140795=CARTESIAN_POINT('Ctrl Pts',(-5.79136161844954,4.40420945811769,
-4.63312879310501));
#140796=CARTESIAN_POINT('Ctrl Pts',(-5.72464727543306,4.41742225104424,
-4.58053855480103));
#140797=CARTESIAN_POINT('Ctrl Pts',(-5.69215102468486,4.42401545785814,
-4.55501688435888));
#140798=CARTESIAN_POINT('Ctrl Pts',(-5.66042266160367,4.43060907930436,
-4.5301341366984));
#140799=CARTESIAN_POINT('Ctrl Pts',(-5.13261580896174,4.30075163058632,
-5.12043129408338));
#140800=CARTESIAN_POINT('Ctrl Pts',(-5.13538622048087,4.30138922829316,
-5.11764826704169));
#140801=CARTESIAN_POINT('Ctrl Pts',(-5.138156632,4.302026826,-5.11486524));
#140802=CARTESIAN_POINT('Ctrl Pts',(-5.416792268,4.36615356,-4.834960791));
#140803=CARTESIAN_POINT('Ctrl Pts',(-5.663373315,4.431389364,-4.526444819));
#140804=CARTESIAN_POINT('Ctrl Pts',(-5.48046371397504,4.30075163058632,
-5.12001791827923));
#140805=CARTESIAN_POINT('Ctrl Pts',(-5.48323369748752,4.30138922829316,
-5.11704648363962));
#140806=CARTESIAN_POINT('Ctrl Pts',(-5.486003681,4.302026826,-5.114075049));
#140807=CARTESIAN_POINT('Ctrl Pts',(-5.76459627,4.36615356,-4.815221404));
#140808=CARTESIAN_POINT('Ctrl Pts',(-6.009076095,4.431389364,-4.487873047));
#140809=CARTESIAN_POINT('Origin',(0.162165348725356,4.55345290765384,0.103690775807935));
#140810=CARTESIAN_POINT('Ctrl Pts',(-4.550585316,4.431369595,-5.643994444));
#140811=CARTESIAN_POINT('Ctrl Pts',(-4.557312103,4.429970133,-5.638570835));
#140812=CARTESIAN_POINT('Ctrl Pts',(-4.564025943,4.428571429,-5.633131207));
#140813=CARTESIAN_POINT('Ctrl Pts',(-4.864933514,4.365882895,-5.389332525));
#140814=CARTESIAN_POINT('Ctrl Pts',(-5.138156632,4.302026826,-5.11486524));
#140815=CARTESIAN_POINT('Ctrl Pts',(-4.513489995,4.431369595,-5.989858769));
#140816=CARTESIAN_POINT('Ctrl Pts',(-4.520629,4.429970133,-5.984479372));
#140817=CARTESIAN_POINT('Ctrl Pts',(-4.527755162,4.428571429,-5.979082973));
#140818=CARTESIAN_POINT('Ctrl Pts',(-4.847142598,4.365882895,-5.737221784));
#140819=CARTESIAN_POINT('Ctrl Pts',(-5.138946823,4.302026826,-5.462712289));
#140820=CARTESIAN_POINT('',(-4.55424019369446,4.4306090798157,-5.64104566757866));
#140821=CARTESIAN_POINT('Origin',(0.150815320472325,4.16114637789378,0.117226175772075));
#140822=CARTESIAN_POINT('Ctrl Pts',(-4.71272429052055,4.39169923737066,
-5.83440054806061));
#140823=CARTESIAN_POINT('Ctrl Pts',(-4.68637156050115,4.39788077310936,
-5.80207499348842));
#140824=CARTESIAN_POINT('Ctrl Pts',(-4.65997706604305,4.40420945812496,
-5.76978037268453));
#140825=CARTESIAN_POINT('Ctrl Pts',(-4.60612778558633,4.41742225800792,
-5.70407801870093));
#140826=CARTESIAN_POINT('Ctrl Pts',(-4.57987769065069,4.4240154632115,-5.67216730675844));
#140827=CARTESIAN_POINT('Ctrl Pts',(-4.55424019597839,4.43060907930317,
-5.64104566923627));
#140828=CARTESIAN_POINT('Ctrl Pts',(-3.91187673525438,4.30075163058632,
-6.10407913568028));
#140829=CARTESIAN_POINT('Ctrl Pts',(-3.91518064462719,4.30138922829316,
-6.10195673084014));
#140830=CARTESIAN_POINT('Ctrl Pts',(-3.918484554,4.302026826,-6.099834326));
#140831=CARTESIAN_POINT('Ctrl Pts',(-4.250777025,4.36615356,-5.886372312));
#140832=CARTESIAN_POINT('Ctrl Pts',(-4.557914959,4.431389364,-5.638076909));
#140833=CARTESIAN_POINT('Ctrl Pts',(-4.25168101209463,4.30075163058632,
-6.17845244216063));
#140834=CARTESIAN_POINT('Ctrl Pts',(-4.25502500554731,4.30138922829316,
-6.17614594258032));
#140835=CARTESIAN_POINT('Ctrl Pts',(-4.258368999,4.302026826,-6.17383944300001));
#140836=CARTESIAN_POINT('Ctrl Pts',(-4.594692948,4.36615356,-5.941862001));
#140837=CARTESIAN_POINT('Ctrl Pts',(-4.903827191,4.431389364,-5.674722802));
#140838=CARTESIAN_POINT('Origin',(0.136083798206303,4.55345291224455,0.136127620145613));
#140839=CARTESIAN_POINT('Ctrl Pts',(-3.23090319,4.431369595,-6.490282319));
#140840=CARTESIAN_POINT('Ctrl Pts',(-3.238638624,4.429970133,-6.486431571));
#140841=CARTESIAN_POINT('Ctrl Pts',(-3.246364857,4.428571429,-6.482562396));
#140842=CARTESIAN_POINT('Ctrl Pts',(-3.592646886,4.365882895,-6.30914982500001));
#140843=CARTESIAN_POINT('Ctrl Pts',(-3.918484554,4.302026826,-6.099834326));
#140844=CARTESIAN_POINT('Ctrl Pts',(-3.120324531,4.431369595,-6.82008613));
#140845=CARTESIAN_POINT('Ctrl Pts',(-3.128453041,4.429970133,-6.816367176));
#140846=CARTESIAN_POINT('Ctrl Pts',(-3.136572664,4.428571429,-6.812628856));
#140847=CARTESIAN_POINT('Ctrl Pts',(-3.500486005,4.365882895,-6.64508110500001));
#140848=CARTESIAN_POINT('Ctrl Pts',(-3.844479437,4.302026826,-6.43971877199999));
#140849=CARTESIAN_POINT('',(-3.23510651809109,4.43060907984298,-6.48818817439076));
#140850=CARTESIAN_POINT('Origin',(0.122089187039252,4.16114645729476,0.146906377531372));
#140851=CARTESIAN_POINT('Ctrl Pts',(-3.34831976121393,4.3916992374112,-6.71109192096717));
#140852=CARTESIAN_POINT('Ctrl Pts',(-3.32953218197703,4.39788077316559,
-6.67385706182384));
#140853=CARTESIAN_POINT('Ctrl Pts',(-3.31069716493212,4.4042094581807,-6.63664343517182));
#140854=CARTESIAN_POINT('Ctrl Pts',(-3.27223093014627,4.41742225272145,
-6.56090119261109));
#140855=CARTESIAN_POINT('Ctrl Pts',(-3.25345441215866,4.42401545580878,
-6.52409355054411));
#140856=CARTESIAN_POINT('Ctrl Pts',(-3.23510652026311,4.43060907931498,
-6.48818817582034));
#140857=CARTESIAN_POINT('Ctrl Pts',(-2.50822265177515,4.30075163058632,
-6.80230702168494));
#140858=CARTESIAN_POINT('Ctrl Pts',(-2.51190557188757,4.30138922829316,
-6.80094448034247));
#140859=CARTESIAN_POINT('Ctrl Pts',(-2.515588492,4.302026826,-6.799581939));
#140860=CARTESIAN_POINT('Ctrl Pts',(-2.886000173,4.36615356,-6.66254360700001));
#140861=CARTESIAN_POINT('Ctrl Pts',(-3.239333565,4.431389364,-6.486078789));
#140862=CARTESIAN_POINT('Ctrl Pts',(-2.82409443206748,4.30075163058632,
-6.94798939631561));
#140863=CARTESIAN_POINT('Ctrl Pts',(-2.82785607403374,4.30138922829316,
-6.9464556811578));
#140864=CARTESIAN_POINT('Ctrl Pts',(-2.831617716,4.302026826,-6.944921966));
#140865=CARTESIAN_POINT('Ctrl Pts',(-3.20994689,4.36615356,-6.79066773500001));
#140866=CARTESIAN_POINT('Ctrl Pts',(-3.569280777,4.431389364,-6.596228827));
#140867=CARTESIAN_POINT('Origin',(0.103638799473347,4.5534529061386,0.162198973411815));
#140868=CARTESIAN_POINT('Ctrl Pts',(-1.760147622,4.431369595,-7.033091806));
#140869=CARTESIAN_POINT('Ctrl Pts',(-1.768530003,4.429970133,-7.030993976));
#140870=CARTESIAN_POINT('Ctrl Pts',(-1.776907359,4.428571429,-7.028876172));
#140871=CARTESIAN_POINT('Ctrl Pts',(-2.152372083,4.365882895,-6.933958291));
#140872=CARTESIAN_POINT('Ctrl Pts',(-2.515588492,4.302026826,-6.799581939));
#140873=CARTESIAN_POINT('Ctrl Pts',(-1.581256159,4.431369595,-7.331413844));
#140874=CARTESIAN_POINT('Ctrl Pts',(-1.589994095,4.429970133,-7.329529226));
#140875=CARTESIAN_POINT('Ctrl Pts',(-1.598727514,4.428571429,-7.327623785));
#140876=CARTESIAN_POINT('Ctrl Pts',(-1.990150577,4.365882895,-7.242223819));
#140877=CARTESIAN_POINT('Ctrl Pts',(-2.370248465,4.302026826,-7.115611162));
#140878=CARTESIAN_POINT('',(-1.7647028575926,4.43060907985456,-7.03195021221419));
#140879=CARTESIAN_POINT('Origin',(0.087654253277924,4.16114647010977,0.169717275906408));
#140880=CARTESIAN_POINT('Ctrl Pts',(-1.82735152120739,4.39169923740398,
-7.27398009430452));
#140881=CARTESIAN_POINT('Ctrl Pts',(-1.81700757923929,4.39788077317501,
-7.23357699113929));
#140882=CARTESIAN_POINT('Ctrl Pts',(-1.80661274423284,4.40420945816821,
-7.1931844266176));
#140883=CARTESIAN_POINT('Ctrl Pts',(-1.78532820116453,4.41742223458717,
-7.11094400505928));
#140884=CARTESIAN_POINT('Ctrl Pts',(-1.774903222269,4.42401543741975,-7.07096050504536));
#140885=CARTESIAN_POINT('Ctrl Pts',(-1.76470285943447,4.43060907931923,
-7.03195021485679));
#140886=CARTESIAN_POINT('Ctrl Pts',(-0.987286864787932,4.30075163058632,
-7.182466590834));
#140887=CARTESIAN_POINT('Ctrl Pts',(-0.991176586393966,4.30138922829316,
-7.181927623917));
#140888=CARTESIAN_POINT('Ctrl Pts',(-0.995066308,4.302026826,-7.181388657));
#140889=CARTESIAN_POINT('Ctrl Pts',(-1.386277161,4.36615356,-7.127181768));
#140890=CARTESIAN_POINT('Ctrl Pts',(-1.769284534,4.431389364,-7.030798834));
#140891=CARTESIAN_POINT('Ctrl Pts',(-1.2644563344217,4.30075163058632,-7.39264608882629));
#140892=CARTESIAN_POINT('Ctrl Pts',(-1.26845973471085,4.30138922829316,
-7.39195687291315));
#140893=CARTESIAN_POINT('Ctrl Pts',(-1.272463135,4.302026826,-7.391267657));
#140894=CARTESIAN_POINT('Ctrl Pts',(-1.675107283,4.36615356,-7.321949394));
#140895=CARTESIAN_POINT('Ctrl Pts',(-2.067838762,4.431389364,-7.209302522));
#140896=CARTESIAN_POINT('Origin',(0.0663477542198945,4.55345291749259,0.180685933335134));
#140897=CARTESIAN_POINT('Ctrl Pts',(-0.20947790199,4.431369595,-7.24451282641));
#140898=CARTESIAN_POINT('Ctrl Pts',(-0.21811226492,4.429970133,-7.24426316081));
#140899=CARTESIAN_POINT('Ctrl Pts',(-0.22674600806,4.428571429,-7.24399291339));
#140900=CARTESIAN_POINT('Ctrl Pts',(-0.61370172234,4.365882895,-7.23188071676));
#140901=CARTESIAN_POINT('Ctrl Pts',(-0.997165097989999,4.302026826,-7.17861468873));
#140902=CARTESIAN_POINT('Ctrl Pts',(-0.207089507,4.431369595,-7.247041737));
#140903=CARTESIAN_POINT('Ctrl Pts',(-0.215726884,4.429970133,-7.246794918));
#140904=CARTESIAN_POINT('Ctrl Pts',(-0.224363648,4.428571429,-7.24652751));
#140905=CARTESIAN_POINT('Ctrl Pts',(-0.611454754,4.365882895,-7.234542573));
#140906=CARTESIAN_POINT('Ctrl Pts',(-0.995066308,4.302026826,-7.181388657));
#140907=CARTESIAN_POINT('Ctrl Pts',(0.031749992,4.431369595,-7.499932796));
#140908=CARTESIAN_POINT('Ctrl Pts',(0.022811208,4.429970133,-7.499970637));
#140909=CARTESIAN_POINT('Ctrl Pts',(0.013872358,4.428571429,-7.499987171));
#140910=CARTESIAN_POINT('Ctrl Pts',(-0.38675792,4.365882895,-7.500728197));
#140911=CARTESIAN_POINT('Ctrl Pts',(-0.785187309,4.302026826,-7.458785484));
#140912=CARTESIAN_POINT('',(-0.211783652922208,4.43060907981772,-7.2469060743844));
#140913=CARTESIAN_POINT('Origin',(0.0491207418811837,4.16114636362922,0.18459210558284));
#140914=CARTESIAN_POINT('Ctrl Pts',(-0.22093835562386,4.39169923735867,
-7.4967450430742));
#140915=CARTESIAN_POINT('Ctrl Pts',(-0.219521722060892,4.39788077308784,
-7.45506290053831));
#140916=CARTESIAN_POINT('Ctrl Pts',(-0.218053119813242,4.40420945810867,
-7.41338010930172));
#140917=CARTESIAN_POINT('Ctrl Pts',(-0.214945473836398,4.41742216317101,
-7.32848733401049));
#140918=CARTESIAN_POINT('Ctrl Pts',(-0.213359497213433,4.42401536555907,
-7.2871975450429));
#140919=CARTESIAN_POINT('Ctrl Pts',(-0.211783654082422,4.43060907940009,
-7.24690607660022));
#140920=CARTESIAN_POINT('Ctrl Pts',(0.579813358054801,4.30075163058632,
-7.22678200501259));
#140921=CARTESIAN_POINT('Ctrl Pts',(0.5758987140274,4.30138922829316,-7.22709181400629));
#140922=CARTESIAN_POINT('Ctrl Pts',(0.57198407,4.302026826,-7.227401623));
#140923=CARTESIAN_POINT('Ctrl Pts',(0.178266631,4.36615356,-7.25856083));
#140924=CARTESIAN_POINT('Ctrl Pts',(-0.216505724,4.431389364,-7.246766539));
#140925=CARTESIAN_POINT('Ctrl Pts',(0.354306336144935,4.30075163058632,
-7.49163086539554));
#140926=CARTESIAN_POINT('Ctrl Pts',(0.350248372072468,4.30138922829316,
-7.49181837569778));
#140927=CARTESIAN_POINT('Ctrl Pts',(0.346190408,4.302026826,-7.49200588600001));
#140928=CARTESIAN_POINT('Ctrl Pts',(-0.061941522,4.36615356,-7.510864836));
#140929=CARTESIAN_POINT('Ctrl Pts',(-0.469706904,4.431389364,-7.48527724400001));
#140930=CARTESIAN_POINT('Origin',(0.0259544467066953,4.55345291197526,0.190724426768116));
#140931=CARTESIAN_POINT('Ctrl Pts',(1.355651883,4.431369595,-7.12212805100001));
#140932=CARTESIAN_POINT('Ctrl Pts',(1.347163385,4.429970133,-7.12374378300001));
#140933=CARTESIAN_POINT('Ctrl Pts',(1.338671059,4.428571429,-7.125339276));
#140934=CARTESIAN_POINT('Ctrl Pts',(0.95805352,4.365882895,-7.196847686));
#140935=CARTESIAN_POINT('Ctrl Pts',(0.57198407,4.302026826,-7.227401623));
#140936=CARTESIAN_POINT('Ctrl Pts',(1.64327155,4.431369595,-7.317763225));
#140937=CARTESIAN_POINT('Ctrl Pts',(1.634549884,4.429970133,-7.319721756));
#140938=CARTESIAN_POINT('Ctrl Pts',(1.625823574,4.428571429,-7.321659491));
#140939=CARTESIAN_POINT('Ctrl Pts',(1.234719107,4.365882895,-7.40850686));
#140940=CARTESIAN_POINT('Ctrl Pts',(0.836588333,4.302026826,-7.453195285));
#140941=CARTESIAN_POINT('',(1.35103832001141,4.4306090798317,-7.12300466238332));
#140942=CARTESIAN_POINT('Origin',(0.00829069334600696,4.16114701816254,
0.190833578894729));
#140943=CARTESIAN_POINT('Ctrl Pts',(1.39580564292763,4.39169923738768,-7.36897052522756));
#140944=CARTESIAN_POINT('Ctrl Pts',(1.38822872775217,4.39788077315009,-7.32795835342677));
#140945=CARTESIAN_POINT('Ctrl Pts',(1.38070242688303,4.40420945812951,-7.2869343768277));
#140946=CARTESIAN_POINT('Ctrl Pts',(1.36548790457561,4.41742222896235,-7.20335787923211));
#140947=CARTESIAN_POINT('Ctrl Pts',(1.35816072347522,4.42401543119208,-7.16269250411706));
#140948=CARTESIAN_POINT('Ctrl Pts',(1.35103831922291,4.43060907936442,-7.12300466481012));
#140949=CARTESIAN_POINT('Ctrl Pts',(2.11980215310686,4.30075163058632,-6.93318112482194));
#140950=CARTESIAN_POINT('Ctrl Pts',(2.11604563105343,4.30138922829316,-6.93432522341097));
#140951=CARTESIAN_POINT('Ctrl Pts',(2.112289109,4.302026826,-6.935469322));
#140952=CARTESIAN_POINT('Ctrl Pts',(1.734474873,4.36615356,-7.05053765600001));
#140953=CARTESIAN_POINT('Ctrl Pts',(1.346396652,4.431389364,-7.123883495));
#140954=CARTESIAN_POINT('Ctrl Pts',(1.95650203590071,4.30075163058632,-7.24031531054044));
#140955=CARTESIAN_POINT('Ctrl Pts',(1.95257925395036,4.30138922829316,-7.24137077927022));
#140956=CARTESIAN_POINT('Ctrl Pts',(1.948656472,4.302026826,-7.242426248));
#140957=CARTESIAN_POINT('Ctrl Pts',(1.554120557,4.36615356,-7.348580586));
#140958=CARTESIAN_POINT('Ctrl Pts',(1.150387927,4.431389364,-7.411248722));
#140959=CARTESIAN_POINT('Origin',(-0.0156524015817822,4.55345290941761,
0.191844575301596));
#140960=CARTESIAN_POINT('Ctrl Pts',(2.855004498,4.431369595,-6.664191573));
#140961=CARTESIAN_POINT('Ctrl Pts',(2.84706179,4.429970133,-6.667594306));
#140962=CARTESIAN_POINT('Ctrl Pts',(2.839110994,4.428571429,-6.670978097));
#140963=CARTESIAN_POINT('Ctrl Pts',(2.482764276,4.365882895,-6.8226362));
#140964=CARTESIAN_POINT('Ctrl Pts',(2.112289109,4.302026826,-6.935469322));
#140965=CARTESIAN_POINT('Ctrl Pts',(3.177955556,4.431369595,-6.793423179));
#140966=CARTESIAN_POINT('Ctrl Pts',(3.169858824,4.429970133,-6.797210821));
#140967=CARTESIAN_POINT('Ctrl Pts',(3.161753086,4.428571429,-6.800979152));
#140968=CARTESIAN_POINT('Ctrl Pts',(2.798462042,4.365882895,-6.969871977));
#140969=CARTESIAN_POINT('Ctrl Pts',(2.419246034,4.302026826,-7.099101959));
#140970=CARTESIAN_POINT('',(2.85068724288564,4.43060907986153,-6.66603946941678));
#140971=CARTESIAN_POINT('Origin',(-0.0329275039884303,4.16114638744478,
0.188156706573089));
#140972=CARTESIAN_POINT('Ctrl Pts',(2.94728332000655,4.39169923738661,-6.8966311360963));
#140973=CARTESIAN_POINT('Ctrl Pts',(2.93106714437857,4.39788077313744,-6.8582066190441));
#140974=CARTESIAN_POINT('Ctrl Pts',(2.91489786188011,4.40420945817505,-6.81975969218555));
#140975=CARTESIAN_POINT('Ctrl Pts',(2.88207248593745,4.41742226301248,-6.7414076377763));
#140976=CARTESIAN_POINT('Ctrl Pts',(2.86617475262101,4.42401546888816,-6.70326811363609));
#140977=CARTESIAN_POINT('Ctrl Pts',(2.85068724309641,4.43060907936564,-6.66603947211694));
#140978=CARTESIAN_POINT('Ctrl Pts',(3.56067135454208,4.30075163058632,-6.31539240121984));
#140979=CARTESIAN_POINT('Ctrl Pts',(3.55724860527104,4.30138922829316,-6.31731729260992));
#140980=CARTESIAN_POINT('Ctrl Pts',(3.553825856,4.30202682600001,-6.319242184));
#140981=CARTESIAN_POINT('Ctrl Pts',(3.209580998,4.36615356,-6.51283917600001));
#140982=CARTESIAN_POINT('Ctrl Pts',(2.846343018,4.431389364,-6.66789557700001));
#140983=CARTESIAN_POINT('Ctrl Pts',(3.46721387482592,4.30075163058632,-6.65045065775765));
#140984=CARTESIAN_POINT('Ctrl Pts',(3.46360969991296,4.30138922829316,-6.65232473237882));
#140985=CARTESIAN_POINT('Ctrl Pts',(3.460005525,4.30202682600001,-6.654198807));
#140986=CARTESIAN_POINT('Ctrl Pts',(3.097513685,4.36615356,-6.842684875));
#140987=CARTESIAN_POINT('Ctrl Pts',(2.716691897,4.431389364,-6.990678446));
#140988=CARTESIAN_POINT('Origin',(-0.0565274918812825,4.55345289725118,
0.183994782434824));
#140989=CARTESIAN_POINT('Ctrl Pts',(4.220860275,4.431369595,-5.894644903));
#140990=CARTESIAN_POINT('Ctrl Pts',(4.213834751,4.429970133,-5.89967553000001));
#140991=CARTESIAN_POINT('Ctrl Pts',(4.206797255,4.428571429,-5.904689396));
#140992=CARTESIAN_POINT('Ctrl Pts',(3.891383734,4.365882895,-6.129405827));
#140993=CARTESIAN_POINT('Ctrl Pts',(3.553825856,4.302026826,-6.319242184));
#140994=CARTESIAN_POINT('Ctrl Pts',(4.564041892,4.431369595,-5.951430215));
#140995=CARTESIAN_POINT('Ctrl Pts',(4.55694868800001,4.429970133,-5.956869862));
#140996=CARTESIAN_POINT('Ctrl Pts',(4.549842538,4.428571429,-5.962292586));
#140997=CARTESIAN_POINT('Ctrl Pts',(4.231352001,4.365882895,-6.205333626));
#140998=CARTESIAN_POINT('Ctrl Pts',(3.88878248,4.302026826,-6.413062515));
#140999=CARTESIAN_POINT('',(4.21704119835812,4.43060907984144,-5.89737767934635));
#141000=CARTESIAN_POINT('Origin',(-0.0726058677300551,4.16114640939035,
0.176679351281246));
#141001=CARTESIAN_POINT('Ctrl Pts',(4.36094930547041,4.39169923740635,-6.10181293976727));
#141002=CARTESIAN_POINT('Ctrl Pts',(4.33685211954446,4.39788077316035,-6.0677727649374));
#141003=CARTESIAN_POINT('Ctrl Pts',(4.31279591317222,4.40420945814279,-6.03370062390091));
#141004=CARTESIAN_POINT('Ctrl Pts',(4.26389471364212,4.41742223236811,-5.96423704339406));
#141005=CARTESIAN_POINT('Ctrl Pts',(4.24016977758101,4.42401544004617,-5.93040672751236));
#141006=CARTESIAN_POINT('Ctrl Pts',(4.2170411989522,4.43060907934584,-5.89737768176648));
#141007=CARTESIAN_POINT('Ctrl Pts',(4.83504752209277,4.30075163058632,-5.40230294817827));
#141008=CARTESIAN_POINT('Ctrl Pts',(4.83211858954639,4.30138922829316,-5.40491862658914));
#141009=CARTESIAN_POINT('Ctrl Pts',(4.829189657,4.302026826,-5.40753430500001));
#141010=CARTESIAN_POINT('Ctrl Pts',(4.53461068300001,4.36615356,-5.670607575));
#141011=CARTESIAN_POINT('Ctrl Pts',(4.213197547,4.431389364,-5.900124272));
#141012=CARTESIAN_POINT('Ctrl Pts',(4.81580264731597,4.30075163058632,-5.74961832426662));
#141013=CARTESIAN_POINT('Ctrl Pts',(4.81268560665798,4.30138922829316,-5.75222337513331));
#141014=CARTESIAN_POINT('Ctrl Pts',(4.809568566,4.302026826,-5.754828426));
#141015=CARTESIAN_POINT('Ctrl Pts',(4.496070517,4.36615356,-6.01683282500001));
#141016=CARTESIAN_POINT('Ctrl Pts',(4.155966373,4.431389364,-6.243231816));
#141017=CARTESIAN_POINT('Origin',(-0.0947593468897162,4.55345286736327,
0.1675413508447));
#141018=CARTESIAN_POINT('Ctrl Pts',(5.38587966315001,4.431369595,-4.84965435201));
#141019=CARTESIAN_POINT('Ctrl Pts',(5.38009960985,4.429970133,-4.85607350493001));
#141020=CARTESIAN_POINT('Ctrl Pts',(5.37430427041,4.428571429,-4.86247886236));
#141021=CARTESIAN_POINT('Ctrl Pts',(5.1145629917,4.365882895,-5.14956055579));
#141022=CARTESIAN_POINT('Ctrl Pts',(4.82571671579,4.302026826,-5.40733809408999));
#141023=CARTESIAN_POINT('Ctrl Pts',(5.38935331700001,4.431369595,-4.84947119));
#141024=CARTESIAN_POINT('Ctrl Pts',(5.383573482,4.429970133,-4.855894483));
#141025=CARTESIAN_POINT('Ctrl Pts',(5.377778351,4.428571429,-4.862303981));
#141026=CARTESIAN_POINT('Ctrl Pts',(5.118046414,4.365882895,-5.149571251));
#141027=CARTESIAN_POINT('Ctrl Pts',(4.829189657,4.302026826,-5.407534305));
#141028=CARTESIAN_POINT('Ctrl Pts',(5.736718702,4.431369595,-4.831154989));
#141029=CARTESIAN_POINT('Ctrl Pts',(5.730960697,4.429970133,-4.83799229));
#141030=CARTESIAN_POINT('Ctrl Pts',(5.72518641,4.428571429,-4.844815845));
#141031=CARTESIAN_POINT('Ctrl Pts',(5.46638864400001,4.365882895,-5.150640772));
#141032=CARTESIAN_POINT('Ctrl Pts',(5.176483778,4.302026826,-5.427155396));
#141033=CARTESIAN_POINT('',(5.38621099464683,4.43060907978048,-4.85296106368865));
#141034=CARTESIAN_POINT('Origin',(-0.108889318602821,4.16114639848255,0.156940670217498));
#141035=CARTESIAN_POINT('Ctrl Pts',(5.57070214744086,4.39169923734938,-5.02168075233251));
#141036=CARTESIAN_POINT('Ctrl Pts',(5.53985070913859,4.39788077309921,-4.99361660052216));
#141037=CARTESIAN_POINT('Ctrl Pts',(5.50903242037404,4.4042094581094,-4.96551242031131));
#141038=CARTESIAN_POINT('Ctrl Pts',(5.44634166948302,4.4174222782979,-4.90818497253391));
#141039=CARTESIAN_POINT('Ctrl Pts',(5.41589892139967,4.42401548178228,-4.88024577479643));
#141040=CARTESIAN_POINT('Ctrl Pts',(5.38621099577858,4.43060907934932,-4.85296106598922));
#141041=CARTESIAN_POINT('Ctrl Pts',(5.8833422403708,4.30075163058632,-4.23660781253323));
#141042=CARTESIAN_POINT('Ctrl Pts',(5.88104407818541,4.30138922829316,-4.23979197176662));
#141043=CARTESIAN_POINT('Ctrl Pts',(5.878745916,4.302026826,-4.242976131));
#141044=CARTESIAN_POINT('Ctrl Pts',(5.647607012,4.36615356,-4.563224667));
#141045=CARTESIAN_POINT('Ctrl Pts',(5.383047642,4.431389364,-4.856469714));
#141046=CARTESIAN_POINT('Ctrl Pts',(5.93920983909918,4.30075163058632,-4.57994022835198));
#141047=CARTESIAN_POINT('Ctrl Pts',(5.93672568204959,4.30138922829316,-4.58315444617599));
#141048=CARTESIAN_POINT('Ctrl Pts',(5.93424152499999,4.302026826,-4.58636866399999));
#141049=CARTESIAN_POINT('Ctrl Pts',(5.684396087,4.36615356,-4.909640359));
#141050=CARTESIAN_POINT('Ctrl Pts',(5.40091248,4.431389364,-5.20385860500001));
#141051=CARTESIAN_POINT('Origin',(-0.128560173577943,4.55345288250795,0.143253706416722));
#141052=CARTESIAN_POINT('Ctrl Pts',(6.30584618800001,4.431369595,-3.577541593));
#141053=CARTESIAN_POINT('Ctrl Pts',(6.3015823,4.429970133,-3.585057207));
#141054=CARTESIAN_POINT('Ctrl Pts',(6.297300509,4.428571429,-3.592562637));
#141055=CARTESIAN_POINT('Ctrl Pts',(6.105394932,4.365882895,-3.928948446));
#141056=CARTESIAN_POINT('Ctrl Pts',(5.878745916,4.302026826,-4.242976131));
#141057=CARTESIAN_POINT('Ctrl Pts',(6.641152922,4.431369595,-3.484980325));
#141058=CARTESIAN_POINT('Ctrl Pts',(6.636999353,4.429970133,-3.492895575));
#141059=CARTESIAN_POINT('Ctrl Pts',(6.632826928,4.428571429,-3.5008009));
#141060=CARTESIAN_POINT('Ctrl Pts',(6.44582303,4.365882895,-3.855109679));
#141061=CARTESIAN_POINT('Ctrl Pts',(6.222138449,4.302026826,-4.187480522));
#141062=CARTESIAN_POINT('',(6.30352755149585,4.43060907983456,-3.58162538195155));
#141063=CARTESIAN_POINT('Origin',(-0.140080817418023,4.16114641568227,0.129863282877415));
#141064=CARTESIAN_POINT('Ctrl Pts',(6.51997514917063,4.39169923735847,-3.70674035357318));
#141065=CARTESIAN_POINT('Ctrl Pts',(6.48381203713831,4.39788077312318,-3.6859644733829));
#141066=CARTESIAN_POINT('Ctrl Pts',(6.4476726947445,4.40420945814442,-3.66514237449988));
#141067=CARTESIAN_POINT('Ctrl Pts',(6.37412364237302,4.41742232677805,-3.62263171337457));
#141068=CARTESIAN_POINT('Ctrl Pts',(6.33838650801649,4.42401553650283,-3.6018899985056));
#141069=CARTESIAN_POINT('Ctrl Pts',(6.30352755295668,4.43060907926899,-3.58162538425232));
#141070=CARTESIAN_POINT('Ctrl Pts',(6.65653841463485,4.30075163058632,-2.87281360540941));
#141071=CARTESIAN_POINT('Ctrl Pts',(6.65497848231742,4.30138922829316,-2.87641735770471));
#141072=CARTESIAN_POINT('Ctrl Pts',(6.65341855,4.302026826,-2.88002111));
#141073=CARTESIAN_POINT('Ctrl Pts',(6.49652751400001,4.36615356,-3.242470445));
#141074=CARTESIAN_POINT('Ctrl Pts',(6.301192412,4.431389364,-3.58573203));
#141075=CARTESIAN_POINT('Ctrl Pts',(6.78490618103697,4.30075163058632,-3.1961092169402));
#141076=CARTESIAN_POINT('Ctrl Pts',(6.78317106401849,4.30138922829316,-3.1997823084701));
#141077=CARTESIAN_POINT('Ctrl Pts',(6.781435947,4.302026826,-3.2034554));
#141078=CARTESIAN_POINT('Ctrl Pts',(6.606925615,4.36615356,-3.572878566));
#141079=CARTESIAN_POINT('Ctrl Pts',(6.393317923,4.431389364,-3.921158749));
#141080=CARTESIAN_POINT('Origin',(-0.156349827180969,4.55345287947972,0.112267878198957));
#141081=CARTESIAN_POINT('Ctrl Pts',(6.9274847,4.431369595,-2.138330128));
#141082=CARTESIAN_POINT('Ctrl Pts',(6.924936134,4.429970133,-2.146586641));
#141083=CARTESIAN_POINT('Ctrl Pts',(6.922367894,4.428571429,-2.154837056));
#141084=CARTESIAN_POINT('Ctrl Pts',(6.807261968,4.365882895,-2.524612378));
#141085=CARTESIAN_POINT('Ctrl Pts',(6.65341854999999,4.302026826,-2.88002111));
#141086=CARTESIAN_POINT('Ctrl Pts',(7.235054212,4.431369595,-1.975851855));
#141087=CARTESIAN_POINT('Ctrl Pts',(7.232699295,4.429970133,-1.984474945));
#141088=CARTESIAN_POINT('Ctrl Pts',(7.230323831,4.428571429,-1.993092396));
#141089=CARTESIAN_POINT('Ctrl Pts',(7.123857894,4.365882895,-2.379317943));
#141090=CARTESIAN_POINT('Ctrl Pts',(6.976852841,4.302026826,-2.752003713));
#141091=CARTESIAN_POINT('',(6.92609816488622,4.43060907984139,-2.14281687848));
#141092=CARTESIAN_POINT('Origin',(-0.164720287169465,4.16114706774232,0.0967129603737812));
#141093=CARTESIAN_POINT('Ctrl Pts',(7.16438135887083,4.39169923737064,-2.21847689612214));
#141094=CARTESIAN_POINT('Ctrl Pts',(7.12459752024601,4.39788077311949,-2.20596074454318));
#141095=CARTESIAN_POINT('Ctrl Pts',(7.08482695982538,4.40420945813223,-2.19339434504391));
#141096=CARTESIAN_POINT('Ctrl Pts',(7.00385935975969,4.41742225301334,-2.16768857502343));
#141097=CARTESIAN_POINT('Ctrl Pts',(6.96449889674919,4.42401545667019,-2.15511422210393));
#141098=CARTESIAN_POINT('Ctrl Pts',(6.92609816709728,4.43060907932906,-2.14281688041309));
#141099=CARTESIAN_POINT('Ctrl Pts',(7.11848225152532,4.30075163058632,-1.37468982618827));
#141100=CARTESIAN_POINT('Ctrl Pts',(7.11773348976266,4.30138922829316,-1.37854466409414));
#141101=CARTESIAN_POINT('Ctrl Pts',(7.116984728,4.302026826,-1.382399502));
#141102=CARTESIAN_POINT('Ctrl Pts',(7.041677609,4.36615356,-1.770101908));
#141103=CARTESIAN_POINT('Ctrl Pts',(6.92470042800001,4.431389364,-2.147329501));
#141104=CARTESIAN_POINT('Ctrl Pts',(7.31334784967157,4.30075163058632,-1.66283169087053));
#141105=CARTESIAN_POINT('Ctrl Pts',(7.31244290483579,4.30138922829316,-1.66679190643526));
#141106=CARTESIAN_POINT('Ctrl Pts',(7.31153796,4.302026826,-1.670752122));
#141107=CARTESIAN_POINT('Ctrl Pts',(7.220522644,4.36615356,-2.069052943));
#141108=CARTESIAN_POINT('Ctrl Pts',(7.086778925,4.431389364,-2.455109868));
#141109=CARTESIAN_POINT('Origin',(-0.176829096811765,4.55345290497252,0.0760326273964132));
#141110=CARTESIAN_POINT('Ctrl Pts',(7.225201726,4.431369595,-0.599132722));
#141111=CARTESIAN_POINT('Ctrl Pts',(7.22448765,4.429970133,-0.607744069));
#141112=CARTESIAN_POINT('Ctrl Pts',(7.22375305,4.428571429,-0.616353689));
#141113=CARTESIAN_POINT('Ctrl Pts',(7.190829,4.365882895,-1.002228242));
#141114=CARTESIAN_POINT('Ctrl Pts',(7.116984728,4.302026826,-1.382399502));
#141115=CARTESIAN_POINT('Ctrl Pts',(7.490652408,4.431369595,-0.374334748));
#141116=CARTESIAN_POINT('Ctrl Pts',(7.490206258,4.429970133,-0.383262472));
#141117=CARTESIAN_POINT('Ctrl Pts',(7.489738828,4.428571429,-0.392189107));
#141118=CARTESIAN_POINT('Ctrl Pts',(7.468789081,4.365882895,-0.792271945));
#141119=CARTESIAN_POINT('Ctrl Pts',(7.405337348,4.302026826,-1.187846269));
#141120=CARTESIAN_POINT('',(7.22481212632807,4.430609079793,-0.6038126392582));
#141121=CARTESIAN_POINT('Origin',(-0.181662538350398,4.16114641014556,0.0590423734243478));
#141122=CARTESIAN_POINT('Ctrl Pts',(7.47378905908835,4.39169923737829,-0.626479925186403));
#141123=CARTESIAN_POINT('Ctrl Pts',(7.43224474213264,4.39788077308007,-0.622808743525736));
#141124=CARTESIAN_POINT('Ctrl Pts',(7.390702590998,4.4042094580625,-0.619085634240142));
#141125=CARTESIAN_POINT('Ctrl Pts',(7.30610202033978,4.41742224782026,-0.61138649412038));
#141126=CARTESIAN_POINT('Ctrl Pts',(7.26495866855288,4.42401545126193,-0.607567458551672));
#141127=CARTESIAN_POINT('Ctrl Pts',(7.22481212871226,4.43060907931025,-0.603812640279783));
#141128=CARTESIAN_POINT('Ctrl Pts',(7.24757376884405,4.30075163058632,0.187712921172618));
#141129=CARTESIAN_POINT('Ctrl Pts',(7.24767118892203,4.30138922829316,0.183787245586309));
#141130=CARTESIAN_POINT('Ctrl Pts',(7.247768609,4.302026826,0.17986157));
#141131=CARTESIAN_POINT('Ctrl Pts',(7.257566686,4.36615356,-0.214965374));
#141132=CARTESIAN_POINT('Ctrl Pts',(7.224417148,4.431389364,-0.608520231));
#141133=CARTESIAN_POINT('Ctrl Pts',(7.49982550189696,4.30075163058632,-0.051802003363299));
#141134=CARTESIAN_POINT('Ctrl Pts',(7.49979304344848,4.30138922829316,-0.0558641676816495));
#141135=CARTESIAN_POINT('Ctrl Pts',(7.499760585,4.302026826,-0.059926332));
#141136=CARTESIAN_POINT('Ctrl Pts',(7.496496059,4.36615356,-0.468480704));
#141137=CARTESIAN_POINT('Ctrl Pts',(7.448870021,4.431389364,-0.874262779));
#141138=CARTESIAN_POINT('Origin',(-0.189039560576475,4.55345292231119,0.0362419940865541));
#141139=CARTESIAN_POINT('Ctrl Pts',(7.18507635,4.431369595,0.968079464000001));
#141140=CARTESIAN_POINT('Ctrl Pts',(7.186230154,4.429970133,0.959515940000001));
#141141=CARTESIAN_POINT('Ctrl Pts',(7.187363542,4.428571429,0.95094969));
#141142=CARTESIAN_POINT('Ctrl Pts',(7.238160861,4.365882895,0.567018973000001));
#141143=CARTESIAN_POINT('Ctrl Pts',(7.247768609,4.302026826,0.17986157));
#141144=CARTESIAN_POINT('Ctrl Pts',(7.395996023,4.431369595,1.244685836));
#141145=CARTESIAN_POINT('Ctrl Pts',(7.3974795,4.429970133,1.235870928));
#141146=CARTESIAN_POINT('Ctrl Pts',(7.398941961,4.428571429,1.227052509));
#141147=CARTESIAN_POINT('Ctrl Pts',(7.464487991,4.365882895,0.83181981));
#141148=CARTESIAN_POINT('Ctrl Pts',(7.487556512,4.302026826,0.431853546));
#141149=CARTESIAN_POINT('',(7.18570190260038,4.43060907983529,0.96342520766656));
#141150=CARTESIAN_POINT('Origin',(-0.190105587267123,4.16114681587434,0.0186100314583489));
#141151=CARTESIAN_POINT('Ctrl Pts',(7.43373068926963,4.39169923741219,0.994810551909341));
#141152=CARTESIAN_POINT('Ctrl Pts',(7.39236845954255,4.39788077317017,0.989465103128073));
#141153=CARTESIAN_POINT('Ctrl Pts',(7.35099718228765,4.40420945818285,0.984170833502881));
#141154=CARTESIAN_POINT('Ctrl Pts',(7.2667195205937,4.41742223508709,0.973503360110972));
#141155=CARTESIAN_POINT('Ctrl Pts',(7.22571707860693,4.4240154411964,0.96838850065241));
#141156=CARTESIAN_POINT('Ctrl Pts',(7.18570190540487,4.43060907928109,0.96342520723106));
#141157=CARTESIAN_POINT('Ctrl Pts',(7.03777679268802,4.30075163058632,1.74133842106059));
#141158=CARTESIAN_POINT('Ctrl Pts',(7.03871583934401,4.30138922829316,1.73752546803029));
#141159=CARTESIAN_POINT('Ctrl Pts',(7.03965488600001,4.302026826,1.733712515));
#141160=CARTESIAN_POINT('Ctrl Pts',(7.134100011,4.36615356,1.350222703));
#141161=CARTESIAN_POINT('Ctrl Pts',(7.186328152,4.431389364,0.958742768));
#141162=CARTESIAN_POINT('Ctrl Pts',(7.33561964867258,4.30075163058632,1.56164988855367));
#141163=CARTESIAN_POINT('Ctrl Pts',(7.33646119433629,4.30138922829316,1.55767571777684));
#141164=CARTESIAN_POINT('Ctrl Pts',(7.33730274,4.302026826,1.553701547));
#141165=CARTESIAN_POINT('Ctrl Pts',(7.42194165,4.36615356,1.153997173));
#141166=CARTESIAN_POINT('Ctrl Pts',(7.462660234,4.431389364,0.747463866999999));
#141167=CARTESIAN_POINT('Origin',(-0.192410959441722,4.5534528786585,-0.00524326309890105));
#141168=CARTESIAN_POINT('Ctrl Pts',(6.808984789,4.431369595,2.49002533));
#141169=CARTESIAN_POINT('Ctrl Pts',(6.811952522,4.429970133,2.48191005));
#141170=CARTESIAN_POINT('Ctrl Pts',(6.814900903,4.428571429,2.47378772));
#141171=CARTESIAN_POINT('Ctrl Pts',(6.947044364,4.365882895,2.109753011));
#141172=CARTESIAN_POINT('Ctrl Pts',(7.039654886,4.302026826,1.733712515));
#141173=CARTESIAN_POINT('Ctrl Pts',(6.955511084,4.431369595,2.805506294));
#141174=CARTESIAN_POINT('Ctrl Pts',(6.958854823,4.429970133,2.797216377));
#141175=CARTESIAN_POINT('Ctrl Pts',(6.962178791,4.428571429,2.788918514));
#141176=CARTESIAN_POINT('Ctrl Pts',(7.11115573900001,4.365882895,2.417016594));
#141177=CARTESIAN_POINT('Ctrl Pts',(7.219665854,4.302026826,2.031360369));
#141178=CARTESIAN_POINT('',(6.81059624420884,4.43060907983355,2.48561436300287));
#141179=CARTESIAN_POINT('Origin',(-0.189663453657438,4.16114641601856,-0.0226926354563547));
#141180=CARTESIAN_POINT('Ctrl Pts',(7.04607933419032,4.3916992374152,2.56958479291152));
#141181=CARTESIAN_POINT('Ctrl Pts',(7.00683324387289,4.39788077317029,2.55547266099481));
#141182=CARTESIAN_POINT('Ctrl Pts',(6.96756731588636,4.40420945812354,2.54140856685183));
#141183=CARTESIAN_POINT('Ctrl Pts',(6.88755313080646,4.41742224818086,2.51287325847989));
#141184=CARTESIAN_POINT('Ctrl Pts',(6.8486088500697,4.42401545432448,2.49906367011868));
#141185=CARTESIAN_POINT('Ctrl Pts',(6.81059624670237,4.43060907928598,2.48561436286732));
#141186=CARTESIAN_POINT('Ctrl Pts',(6.4989011950665,4.30075163058632,3.21354087208441));
#141187=CARTESIAN_POINT('Ctrl Pts',(6.50063795953325,4.30138922829316,3.2100189310422));
#141188=CARTESIAN_POINT('Ctrl Pts',(6.50237472400001,4.302026826,3.20649699));
#141189=CARTESIAN_POINT('Ctrl Pts',(6.677050749,4.36615356,2.852275866));
#141190=CARTESIAN_POINT('Ctrl Pts',(6.812214438,4.431389364,2.481176021));
#141191=CARTESIAN_POINT('Ctrl Pts',(6.82840837392086,4.30075163058632,3.10208076685929));
#141192=CARTESIAN_POINT('Ctrl Pts',(6.83008457396043,4.30138922829316,3.09838041742964));
#141193=CARTESIAN_POINT('Ctrl Pts',(6.83176077400001,4.302026826,3.094680068));
#141194=CARTESIAN_POINT('Ctrl Pts',(7.000345499,4.36615356,2.722515424));
#141195=CARTESIAN_POINT('Ctrl Pts',(7.127504748,4.431389364,2.334239933));
#141196=CARTESIAN_POINT('Origin',(-0.186785148316219,4.55345291235534,-0.0464832497892625));
#141197=CARTESIAN_POINT('Ctrl Pts',(6.1137598519,4.431369595,3.89214433884));
#141198=CARTESIAN_POINT('Ctrl Pts',(6.11839869934,4.429970133,3.88485766207));
#141199=CARTESIAN_POINT('Ctrl Pts',(6.12302016393,4.428571429,3.87755994896));
#141200=CARTESIAN_POINT('Ctrl Pts',(6.33014957445,4.365882895,3.55048375274));
#141201=CARTESIAN_POINT('Ctrl Pts',(6.50125655478,4.302026826,3.2032031295));
#141202=CARTESIAN_POINT('Ctrl Pts',(6.114512667,4.431369595,3.895540379));
#141203=CARTESIAN_POINT('Ctrl Pts',(6.119155562,4.429970133,3.888252805));
#141204=CARTESIAN_POINT('Ctrl Pts',(6.123781072,4.428571429,3.880954185));
#141205=CARTESIAN_POINT('Ctrl Pts',(6.331091794,4.365882895,3.553837343));
#141206=CARTESIAN_POINT('Ctrl Pts',(6.502374724,4.302026826,3.20649699));
#141207=CARTESIAN_POINT('Ctrl Pts',(6.189794177,4.431369595,4.235144395));
#141208=CARTESIAN_POINT('Ctrl Pts',(6.194841828,4.429970133,4.227767098));
#141209=CARTESIAN_POINT('Ctrl Pts',(6.199871879,4.428571429,4.220377789));
#141210=CARTESIAN_POINT('Ctrl Pts',(6.425313749,4.365882895,3.889196369));
#141211=CARTESIAN_POINT('Ctrl Pts',(6.614191646,4.302026826,3.53588304));
#141212=CARTESIAN_POINT('',(6.11703467512379,4.43060907974158,3.89157895330898));
#141213=CARTESIAN_POINT('Origin',(-0.180351123952476,4.16114643519017,-0.0629342094358598));
#141214=CARTESIAN_POINT('Ctrl Pts',(6.3289611410797,4.39169923740138,4.02420810481511));
#141215=CARTESIAN_POINT('Ctrl Pts',(6.29366629386744,4.3978807731276,4.00198915746816));
#141216=CARTESIAN_POINT('Ctrl Pts',(6.25834174588008,4.40420945808978,3.97981286015401));
#141217=CARTESIAN_POINT('Ctrl Pts',(6.18633291490832,4.41742217123992,3.93474426914271));
#141218=CARTESIAN_POINT('Ctrl Pts',(6.15126776957677,4.42401537644418,3.91288566100586));
#141219=CARTESIAN_POINT('Ctrl Pts',(6.11703467769023,4.43060907925216,3.89157895377656));
#141220=CARTESIAN_POINT('Ctrl Pts',(5.65614420082141,4.30075163058632,4.53548172299218));
#141221=CARTESIAN_POINT('Ctrl Pts',(5.6585974739107,4.30138922829316,4.53241547599609));
#141222=CARTESIAN_POINT('Ctrl Pts',(5.661050747,4.302026826,4.529349229));
#141223=CARTESIAN_POINT('Ctrl Pts',(5.907790014,4.36615356,4.22095978));
#141224=CARTESIAN_POINT('Ctrl Pts',(6.119569149,4.431389364,3.887592241));
#141225=CARTESIAN_POINT('Ctrl Pts',(6.00190831268338,4.30075163058632,4.49746179671396));
#141226=CARTESIAN_POINT('Ctrl Pts',(6.00434078984169,4.30138922829316,4.49420829285698));
#141227=CARTESIAN_POINT('Ctrl Pts',(6.00677326700001,4.302026826,4.490954789));
#141228=CARTESIAN_POINT('Ctrl Pts',(6.251420972,4.36615356,4.16373188));
#141229=CARTESIAN_POINT('Ctrl Pts',(6.45907506200001,4.431389364,3.811869534));
#141230=CARTESIAN_POINT('Origin',(-0.172425869120202,4.55345290385811,-0.0855499160282613));
#141231=CARTESIAN_POINT('Ctrl Pts',(5.13412756255,4.431369595,5.11542581336999));
#141232=CARTESIAN_POINT('Ctrl Pts',(5.14022437574001,4.429970133,5.10930671053));
#141233=CARTESIAN_POINT('Ctrl Pts',(5.14630658595,4.428571429,5.10317309157));
#141234=CARTESIAN_POINT('Ctrl Pts',(5.4189051398,4.365882895,4.82827045646));
#141235=CARTESIAN_POINT('Ctrl Pts',(5.6606668026,4.302026826,4.5258920038));
#141236=CARTESIAN_POINT('Ctrl Pts',(5.134132729,4.431369595,5.118904289));
#141237=CARTESIAN_POINT('Ctrl Pts',(5.140233688,4.429970133,5.11278518));
#141238=CARTESIAN_POINT('Ctrl Pts',(5.146320044,4.428571429,5.106651545));
#141239=CARTESIAN_POINT('Ctrl Pts',(5.419104408,4.365882895,4.831748191));
#141240=CARTESIAN_POINT('Ctrl Pts',(5.661050747,4.302026826,4.529349229));
#141241=CARTESIAN_POINT('Ctrl Pts',(5.134649374,4.431369595,5.46675185200001));
#141242=CARTESIAN_POINT('Ctrl Pts',(5.141164914,4.429970133,5.460632127));
#141243=CARTESIAN_POINT('Ctrl Pts',(5.147665849,4.428571429,5.454496888));
#141244=CARTESIAN_POINT('Ctrl Pts',(5.439031228,4.365882895,5.179521645));
#141245=CARTESIAN_POINT('Ctrl Pts',(5.69944518700001,4.302026826,4.875071749));
#141246=CARTESIAN_POINT('',(5.13744736268223,4.43060907978605,5.11557763715302));
#141247=CARTESIAN_POINT('Origin',(-0.162605461209986,4.16114639537215,-0.100232851895971));
#141248=CARTESIAN_POINT('Ctrl Pts',(5.3159077588462,4.39169923738225,5.29066391793093));
#141249=CARTESIAN_POINT('Ctrl Pts',(5.28621450234274,4.39788077314604,5.26137708832544));
#141250=CARTESIAN_POINT('Ctrl Pts',(5.2564830708976,4.40420945815575,5.23212552680058));
#141251=CARTESIAN_POINT('Ctrl Pts',(5.19584578481867,4.41742225769839,5.17263045556358));
#141252=CARTESIAN_POINT('Ctrl Pts',(5.16629941639326,4.42401546239431,5.14374494205272));
#141253=CARTESIAN_POINT('Ctrl Pts',(5.13744736516035,4.43060907933145,5.11557763789017));
#141254=CARTESIAN_POINT('Ctrl Pts',(4.54891219022449,4.30075163058632,5.64534848929436));
#141255=CARTESIAN_POINT('Ctrl Pts',(4.55196725961225,4.30138922829316,5.64288131064718));
#141256=CARTESIAN_POINT('Ctrl Pts',(4.555022329,4.302026826,5.640414132));
#141257=CARTESIAN_POINT('Ctrl Pts',(4.862287584,4.36615356,5.392276306));
#141258=CARTESIAN_POINT('Ctrl Pts',(5.14077960699999,4.431389364,5.112228969));
#141259=CARTESIAN_POINT('Ctrl Pts',(4.89476568930713,4.30075163058632,5.68254651113073));
#141260=CARTESIAN_POINT('Ctrl Pts',(4.89784070365356,4.30138922829316,5.67989198306536));
#141261=CARTESIAN_POINT('Ctrl Pts',(4.900915718,4.302026826,5.677237455));
#141262=CARTESIAN_POINT('Ctrl Pts',(5.210186948,4.36615356,5.41025686));
#141263=CARTESIAN_POINT('Ctrl Pts',(5.488626205,4.431389364,5.111260352));
#141264=CARTESIAN_POINT('Origin',(-0.150003984782877,4.55345289786449,-0.120616314865278));
#141265=CARTESIAN_POINT('Ctrl Pts',(3.91368645,4.431369595,6.102913924));
#141266=CARTESIAN_POINT('Ctrl Pts',(3.9209602,4.429970133,6.098249402));
#141267=CARTESIAN_POINT('Ctrl Pts',(3.928222811,4.428571429,6.093567555));
#141268=CARTESIAN_POINT('Ctrl Pts',(4.253725723,4.365882895,5.883731863));
#141269=CARTESIAN_POINT('Ctrl Pts',(4.55502232900001,4.302026826,5.640414132));
#141270=CARTESIAN_POINT('Ctrl Pts',(3.839414072,4.431369595,6.442740068));
#141271=CARTESIAN_POINT('Ctrl Pts',(3.847092844,4.429970133,6.438164067));
#141272=CARTESIAN_POINT('Ctrl Pts',(3.854760685,4.428571429,6.433569776));
#141273=CARTESIAN_POINT('Ctrl Pts',(4.198425653,4.365882895,6.227658244));
#141274=CARTESIAN_POINT('Ctrl Pts',(4.518199006,4.302026826,5.986307521));
#141275=CARTESIAN_POINT('',(3.91763872170725,4.43060907983154,6.10037759560077));
#141276=CARTESIAN_POINT('Origin',(-0.137256717281262,4.16114637760005,-0.132844812216939));
#141277=CARTESIAN_POINT('Ctrl Pts',(4.05428843853699,4.39169923736995,6.30973416640578));
#141278=CARTESIAN_POINT('Ctrl Pts',(4.0315851965443,4.39788077312087,6.27474887425655));
#141279=CARTESIAN_POINT('Ctrl Pts',(4.0088370904528,4.40420945813757,6.23978981908078));
#141280=CARTESIAN_POINT('Ctrl Pts',(3.96240709071846,4.41742227513582,6.16865039165864));
#141281=CARTESIAN_POINT('Ctrl Pts',(3.93976101701759,4.42401548541367,6.1340885862235));
#141282=CARTESIAN_POINT('Ctrl Pts',(3.91763872389686,4.43060907925384,6.1003775976299));
#141283=CARTESIAN_POINT('Ctrl Pts',(3.22897810090943,4.30075163058632,6.49124503453277));
#141284=CARTESIAN_POINT('Ctrl Pts',(3.23249211495472,4.30138922829316,6.48949228676638));
#141285=CARTESIAN_POINT('Ctrl Pts',(3.236006129,4.302026826,6.487739539));
#141286=CARTESIAN_POINT('Ctrl Pts',(3.589429991,4.36615356,6.311455985));
#141287=CARTESIAN_POINT('Ctrl Pts',(3.921612925,4.431389364,6.097823552));
#141288=CARTESIAN_POINT('Ctrl Pts',(3.55874926241771,4.30075163058632,6.60192166698133));
#141289=CARTESIAN_POINT('Ctrl Pts',(3.56232302970886,4.30138922829316,6.59999023749066));
#141290=CARTESIAN_POINT('Ctrl Pts',(3.565896797,4.302026826,6.598058808));
#141291=CARTESIAN_POINT('Ctrl Pts',(3.925330374,4.36615356,6.403804243));
#141292=CARTESIAN_POINT('Ctrl Pts',(4.261535287,4.431389364,6.171654316));
#141293=CARTESIAN_POINT('Origin',(-0.120568015468438,4.55345288918264,-0.150042782148404));
#141294=CARTESIAN_POINT('Ctrl Pts',(2.510240543,4.431369595,6.801558087));
#141295=CARTESIAN_POINT('Ctrl Pts',(2.518346971,4.429970133,6.79856626));
#141296=CARTESIAN_POINT('Ctrl Pts',(2.526446244,4.428571429,6.795555119));
#141297=CARTESIAN_POINT('Ctrl Pts',(2.88944755,4.365882895,6.660598773));
#141298=CARTESIAN_POINT('Ctrl Pts',(3.236006129,4.302026826,6.487739539));
#141299=CARTESIAN_POINT('Ctrl Pts',(2.364652037,4.431369595,7.117472919));
#141300=CARTESIAN_POINT('Ctrl Pts',(2.373134987,4.429970133,7.114654611));
#141301=CARTESIAN_POINT('Ctrl Pts',(2.381611195,4.428571429,7.111816091));
#141302=CARTESIAN_POINT('Ctrl Pts',(2.76150636,4.365882895,6.984596466));
#141303=CARTESIAN_POINT('Ctrl Pts',(3.125686861,4.302026826,6.817630208));
#141304=CARTESIAN_POINT('',(2.51464564830737,4.43060907980155,6.79993067800396));
#141305=CARTESIAN_POINT('Origin',(-0.105490043542784,4.16114643440491,-0.159245170787863));
#141306=CARTESIAN_POINT('Ctrl Pts',(2.6030950961635,4.39169923736054,7.03376825860753));
#141307=CARTESIAN_POINT('Ctrl Pts',(2.58844344688307,4.39788077312132,6.99472037711179));
#141308=CARTESIAN_POINT('Ctrl Pts',(2.57374234231555,4.40420945811645,6.95568847492197));
#141309=CARTESIAN_POINT('Ctrl Pts',(2.54369085516498,4.41742221748141,6.87623151675625));
#141310=CARTESIAN_POINT('Ctrl Pts',(2.5290040057849,4.42401542249756,6.83760952313001));
#141311=CARTESIAN_POINT('Ctrl Pts',(2.51464565003509,4.43060907922589,6.79993068076175));
#141312=CARTESIAN_POINT('Ctrl Pts',(1.75806058539698,4.30075163058632,7.03361817669735));
#141313=CARTESIAN_POINT('Ctrl Pts',(1.76186923269849,4.30138922829316,7.03266181634867));
#141314=CARTESIAN_POINT('Ctrl Pts',(1.76567788,4.302026826,7.031705456));
#141315=CARTESIAN_POINT('Ctrl Pts',(2.148734641,4.36615356,6.935518997));
#141316=CARTESIAN_POINT('Ctrl Pts',(2.519075981,4.431389364,6.798290683));
#141317=CARTESIAN_POINT('Ctrl Pts',(2.05632967530983,4.30075163058632,7.21259830283048));
#141318=CARTESIAN_POINT('Ctrl Pts',(2.06023509015492,4.30138922829316,7.21148028341524));
#141319=CARTESIAN_POINT('Ctrl Pts',(2.064140505,4.302026826,7.210362264));
#141320=CARTESIAN_POINT('Ctrl Pts',(2.456929714,4.36615356,7.097916857));
#141321=CARTESIAN_POINT('Ctrl Pts',(2.835179715,4.431389364,6.94346858500001));
#141322=CARTESIAN_POINT('Origin',(-0.0854944270200353,4.55345285995928,
-0.172453402573198));
#141323=CARTESIAN_POINT('Ctrl Pts',(0.989418577999999,4.431369595,7.182168954));
#141324=CARTESIAN_POINT('Ctrl Pts',(0.997978637,4.429970133,7.180989716));
#141325=CARTESIAN_POINT('Ctrl Pts',(1.00653586,4.428571429,7.179790078));
#141326=CARTESIAN_POINT('Ctrl Pts',(1.390062022,4.365882895,7.126023487));
#141327=CARTESIAN_POINT('Ctrl Pts',(1.76567788,4.302026826,7.031705456));
#141328=CARTESIAN_POINT('Ctrl Pts',(0.779321499,4.431369595,7.459400646));
#141329=CARTESIAN_POINT('Ctrl Pts',(0.788211976,4.429970133,7.458471813));
#141330=CARTESIAN_POINT('Ctrl Pts',(0.797100213,4.428571429,7.45752179));
#141331=CARTESIAN_POINT('Ctrl Pts',(1.195462099,4.365882895,7.41494272));
#141332=CARTESIAN_POINT('Ctrl Pts',(1.587021072,4.302026826,7.330168082));
#141333=CARTESIAN_POINT('',(0.994070539475338,4.43060907984242,7.18152655971494));
#141334=CARTESIAN_POINT('Origin',(-0.0687907678335942,4.16114642128525,
-0.178199462025521));
#141335=CARTESIAN_POINT('Ctrl Pts',(1.03018392039923,4.3916992373849,7.42891116420171));
#141336=CARTESIAN_POINT('Ctrl Pts',(1.02426895890848,4.3978807731304,7.38762652911978));
#141337=CARTESIAN_POINT('Ctrl Pts',(1.01830226328049,4.40420945811811,7.34634686826014));
#141338=CARTESIAN_POINT('Ctrl Pts',(1.006034236914,4.41742224301326,7.2622872258476));
#141339=CARTESIAN_POINT('Ctrl Pts',(0.999993344785503,4.42401544886382,
7.22141095734852));
#141340=CARTESIAN_POINT('Ctrl Pts',(0.994070540471638,4.43060907935679,
7.18152656222649));
#141341=CARTESIAN_POINT('Ctrl Pts',(0.204938109066286,4.30075163058632,
7.24710715016635));
#141342=CARTESIAN_POINT('Ctrl Pts',(0.208863301533143,4.30138922829316,
7.24699189558317));
#141343=CARTESIAN_POINT('Ctrl Pts',(0.212788494,4.302026826,7.246876641));
#141344=CARTESIAN_POINT('Ctrl Pts',(0.607566848,4.36615356,7.235284849));
#141345=CARTESIAN_POINT('Ctrl Pts',(0.998749843,4.431389364,7.180877297));
#141346=CARTESIAN_POINT('Ctrl Pts',(0.457758398939834,4.30075163058632,
7.48602185797434));
#141347=CARTESIAN_POINT('Ctrl Pts',(0.461812848469918,4.30138922829316,
7.48576952598717));
#141348=CARTESIAN_POINT('Ctrl Pts',(0.465867298,4.302026826,7.485517194));
#141349=CARTESIAN_POINT('Ctrl Pts',(0.873645751,4.36615356,7.460138768));
#141350=CARTESIAN_POINT('Ctrl Pts',(1.27625429,4.431389364,7.390613979));
#141351=CARTESIAN_POINT('Origin',(-0.0464232246340045,4.55345293116766,
-0.186800079926107));
#141352=CARTESIAN_POINT('Ctrl Pts',(-0.57501968255,4.431369595,7.22469372692));
#141353=CARTESIAN_POINT('Ctrl Pts',(-0.56640894119,4.429970133,7.22537906312));
#141354=CARTESIAN_POINT('Ctrl Pts',(-0.55779659034,4.428571429,7.22604387274));
#141355=CARTESIAN_POINT('Ctrl Pts',(-0.17179966821,4.365882895,7.2558399507));
#141356=CARTESIAN_POINT('Ctrl Pts',(0.21517489952,4.302026826,7.24434585296));
#141357=CARTESIAN_POINT('Ctrl Pts',(-0.5776675,4.431369595,7.226949582));
#141358=CARTESIAN_POINT('Ctrl Pts',(-0.56905407,4.429970133,7.22763807400001));
#141359=CARTESIAN_POINT('Ctrl Pts',(-0.560439023,4.428571429,7.228306033));
#141360=CARTESIAN_POINT('Ctrl Pts',(-0.174321262,4.365882895,7.25824326300001));
#141361=CARTESIAN_POINT('Ctrl Pts',(0.212788494,4.302026826,7.246876641));
#141362=CARTESIAN_POINT('Ctrl Pts',(-0.842449245,4.431369595,7.45253509));
#141363=CARTESIAN_POINT('Ctrl Pts',(-0.833566951,4.429970133,7.453539162));
#141364=CARTESIAN_POINT('Ctrl Pts',(-0.824682289,4.428571429,7.454522059));
#141365=CARTESIAN_POINT('Ctrl Pts',(-0.426480641,4.365882895,7.498574493));
#141366=CARTESIAN_POINT('Ctrl Pts',(-0.025852058,4.302026826,7.499955445));
#141367=CARTESIAN_POINT('Origin',(-0.0288748555719586,4.16114642761327,
-0.188821302368569));
#141368=CARTESIAN_POINT('Ctrl Pts',(0.206355414,1.457192641,7.247062677));
#141369=CARTESIAN_POINT('Ctrl Pts',(0.603838305,1.522897175,7.235744609));
#141370=CARTESIAN_POINT('Ctrl Pts',(0.997699109,1.587500328,7.181023359));
#141371=CARTESIAN_POINT('Ctrl Pts',(0.459222278,1.457192641,7.485927791));
#141372=CARTESIAN_POINT('Ctrl Pts',(0.869806311,1.522897175,7.460740622));
#141373=CARTESIAN_POINT('Ctrl Pts',(1.275172863,1.587500328,7.390800645));
#141374=CARTESIAN_POINT('',(0.459222295417621,1.45719263974394,7.48592778870736));
#141375=CARTESIAN_POINT('',(1.02534975045092,1.54766053442819,7.429579834804));
#141376=CARTESIAN_POINT('Origin',(0.00737832284867054,1.3393599161851,-0.18767758211871));
#141377=CARTESIAN_POINT('Ctrl Pts',(0.993027301226868,1.58673401519535,
7.18167089033084));
#141378=CARTESIAN_POINT('Ctrl Pts',(0.998359708366294,1.57991285715115,
7.22293886439134));
#141379=CARTESIAN_POINT('Ctrl Pts',(1.00372395719946,1.57325083217545,7.26425318543439));
#141380=CARTESIAN_POINT('Ctrl Pts',(1.01449798875009,1.56023624973537,7.34687598194897));
#141381=CARTESIAN_POINT('Ctrl Pts',(1.019913657707,1.55387659346546,7.38822956347221));
#141382=CARTESIAN_POINT('Ctrl Pts',(1.02534975010316,1.54766054355296,7.42957983622142));
#141383=CARTESIAN_POINT('',(0.332788868614406,1.45719263730543,7.36649523297837));
#141384=CARTESIAN_POINT('Origin',(-1.07932326270932E-13,1.54874775200011,
-8.50014503228635E-13));
#141385=CARTESIAN_POINT('',(1.02275296019507,1.36645689999125,7.42993784473413));
#141386=CARTESIAN_POINT('Origin',(-0.00775337357056385,1.48213729927608,
-0.191983098392322));
#141387=CARTESIAN_POINT('',(1.58051349599227,1.45719264185526,7.33157405540269));
#141388=CARTESIAN_POINT('Origin',(-0.021854084256511,1.33929189546777,-0.190828900708343));
#141389=CARTESIAN_POINT('Origin',(-0.0367451552969436,1.48214297993429,
-0.189449351628988));
#141390=CARTESIAN_POINT('Ctrl Pts',(0.988391585,1.587508025,7.182310358));
#141391=CARTESIAN_POINT('Ctrl Pts',(1.377955312,1.52246862,7.128700657));
#141392=CARTESIAN_POINT('Ctrl Pts',(1.759435193,1.457192641,7.033270065));
#141393=CARTESIAN_POINT('Ctrl Pts',(1.77256190375125,1.45494649660808,7.02998630131967));
#141394=CARTESIAN_POINT('Ctrl Pts',(1.78568861450254,1.45270035221617,7.02670253763929));
#141395=CARTESIAN_POINT('Ctrl Pts',(0.777825679513265,1.587508025,7.4600781682574));
#141396=CARTESIAN_POINT('Ctrl Pts',(1.18245534777751,1.52246862,7.41788942109954));
#141397=CARTESIAN_POINT('Ctrl Pts',(1.58014807973878,1.457192641,7.33218324295674));
#141398=CARTESIAN_POINT('Ctrl Pts',(1.59383267418357,1.45494649660808,7.32923409605251));
#141399=CARTESIAN_POINT('Ctrl Pts',(1.60751726862837,1.45270035221618,7.32628494914832));
#141400=CARTESIAN_POINT('',(1.66997436233271,1.4571926425566,7.18242202083007));
#141401=CARTESIAN_POINT('Ctrl Pts',(1.759435193,1.457192641,7.033270065));
#141402=CARTESIAN_POINT('Ctrl Pts',(2.145192105,1.522897175,6.93676953500001));
#141403=CARTESIAN_POINT('Ctrl Pts',(2.518081211,1.587500328,6.798659207));
#141404=CARTESIAN_POINT('Ctrl Pts',(2.057739109,1.457192641,7.212191744));
#141405=CARTESIAN_POINT('Ctrl Pts',(2.453309419,1.522897175,7.099330006));
#141406=CARTESIAN_POINT('Ctrl Pts',(2.834163698,1.587500328,6.94388336100001));
#141407=CARTESIAN_POINT('',(2.05773912551659,1.45719263974394,7.21219173801661));
#141408=CARTESIAN_POINT('',(2.59851769117755,1.54766053444267,7.03546049931711));
#141409=CARTESIAN_POINT('Origin',(-0.0331393637470409,1.33935993853076,
-0.1848760404687));
#141410=CARTESIAN_POINT('Ctrl Pts',(2.51365782782729,1.58673401524756,6.80029589983965));
#141411=CARTESIAN_POINT('Ctrl Pts',(2.52773696267109,1.57991285627922,6.83945274689865));
#141412=CARTESIAN_POINT('Ctrl Pts',(2.54185715832421,1.57325083034138,6.87864801308967));
#141413=CARTESIAN_POINT('Ctrl Pts',(2.57014083739803,1.56023621136334,6.95702325605497));
#141414=CARTESIAN_POINT('Ctrl Pts',(2.58431978334036,1.55387651552159,6.99624606562961));
#141415=CARTESIAN_POINT('Ctrl Pts',(2.59851769119417,1.54766054358843,7.0354605007608));
#141416=CARTESIAN_POINT('',(1.90858717286608,1.45719263730543,7.12273089864083));
#141417=CARTESIAN_POINT('Origin',(-1.39211558947139E-13,1.54874775199994,
-1.9819215713035E-13));
#141418=CARTESIAN_POINT('',(2.59605857345536,1.36645689997628,7.03636837262591));
#141419=CARTESIAN_POINT('Origin',(-0.0488428478450981,1.48213730590088,
-0.185828051894329));
#141420=CARTESIAN_POINT('',(3.1196336713731,1.45719264185526,6.82040224533446));
#141421=CARTESIAN_POINT('Origin',(-0.0623657656572568,1.33929186513119,
-0.181669549898223));
#141422=CARTESIAN_POINT('Origin',(-0.0766119206329151,1.48214301573756,
-0.177120609940757));
#141423=CARTESIAN_POINT('Ctrl Pts',(2.509267959,1.587508025,6.801916959));
#141424=CARTESIAN_POINT('Ctrl Pts',(2.878199401,1.52246862,6.665815937));
#141425=CARTESIAN_POINT('Ctrl Pts',(3.230245738,1.457192641,6.490609561));
#141426=CARTESIAN_POINT('Ctrl Pts',(3.24235964108627,1.4549464966708,6.48458071526042));
#141427=CARTESIAN_POINT('Ctrl Pts',(3.2544735441726,1.45270035234162,6.47855186952078));
#141428=CARTESIAN_POINT('Ctrl Pts',(2.36333683583635,1.587508025,7.11845615730253));
#141429=CARTESIAN_POINT('Ctrl Pts',(2.74943715342077,1.52246862,6.99027034253071));
#141430=CARTESIAN_POINT('Ctrl Pts',(3.11940775568363,1.457192641,6.82107574407964));
#141431=CARTESIAN_POINT('Ctrl Pts',(3.1321384321587,1.4549464966708,6.81525376341134));
#141432=CARTESIAN_POINT('Ctrl Pts',(3.14486910863384,1.45270035234162,6.80943178274304));
#141433=CARTESIAN_POINT('',(3.17493971364809,1.4571926425566,6.65550586087452));
#141434=CARTESIAN_POINT('Ctrl Pts',(3.230245738,1.457192641,6.490609561));
#141435=CARTESIAN_POINT('Ctrl Pts',(3.586239107,1.522897175,6.313438827));
#141436=CARTESIAN_POINT('Ctrl Pts',(3.920720634,1.587500328,6.098397307));
#141437=CARTESIAN_POINT('Ctrl Pts',(3.560038347,1.457192641,6.601221627));
#141438=CARTESIAN_POINT('Ctrl Pts',(3.922098505,1.522897175,6.40596261));
#141439=CARTESIAN_POINT('Ctrl Pts',(4.26063218900001,1.587500328,6.172277809));
#141440=CARTESIAN_POINT('',(3.56003836181377,1.45719263974395,6.60122161761045));
#141441=CARTESIAN_POINT('',(4.05018183213464,1.54766053440617,6.31237085077319));
#141442=CARTESIAN_POINT('Origin',(-0.0721074795453386,1.33935992231088,
-0.173429776045458));
#141443=CARTESIAN_POINT('Ctrl Pts',(3.91675250729274,1.58673401518852,6.10094663167512));
#141444=CARTESIAN_POINT('Ctrl Pts',(3.93892001923704,1.57991286402647,6.13616137513056));
#141445=CARTESIAN_POINT('Ctrl Pts',(3.9611358874709,1.57325084614049,6.17140480742286));
#141446=CARTESIAN_POINT('Ctrl Pts',(4.00560673407309,1.56023620854231,6.24186762645686));
#141447=CARTESIAN_POINT('Ctrl Pts',(4.02788593933092,1.55387650989478,6.27712539084905));
#141448=CARTESIAN_POINT('Ctrl Pts',(4.05018183241762,1.54766054352542,6.31237085220247));
#141449=CARTESIAN_POINT('',(3.39514206259527,1.45719263730544,6.54591558357728));
#141450=CARTESIAN_POINT('Origin',(6.46184494801361E-13,1.54874775199939,
9.74480912629971E-13));
#141451=CARTESIAN_POINT('',(4.04797537329225,1.36645690002083,6.31378613588496));
#141452=CARTESIAN_POINT('Origin',(-0.0876483475473111,1.48213729582552,
-0.170983506854183));
#141453=CARTESIAN_POINT('',(4.5128832428005,1.45719264185525,5.99031600768223));
#141454=CARTESIAN_POINT('Origin',(-0.0999613416881162,1.33929187558694,
-0.164015522851519));
#141455=CARTESIAN_POINT('Origin',(-0.112896555986552,1.48214303935283,-0.156510462046193));
#141456=CARTESIAN_POINT('Ctrl Pts',(3.912813751,1.587508025,6.10347348200001));
#141457=CARTESIAN_POINT('Ctrl Pts',(4.243862085,1.52246862,5.891245072));
#141458=CARTESIAN_POINT('Ctrl Pts',(4.550013582,1.457192641,5.644455368));
#141459=CARTESIAN_POINT('Ctrl Pts',(4.56054824525312,1.45494649664329,5.63596334215186));
#141460=CARTESIAN_POINT('Ctrl Pts',(4.57108290850628,1.45270035228661,5.62747131630359));
#141461=CARTESIAN_POINT('Ctrl Pts',(3.83834098735086,1.587508025,6.44398304808587));
#141462=CARTESIAN_POINT('Ctrl Pts',(4.18785833294733,1.52246862,6.23579399132682));
#141463=CARTESIAN_POINT('Ctrl Pts',(4.51280739121253,1.457192641,5.99102232560795));
#141464=CARTESIAN_POINT('Ctrl Pts',(4.52398887794962,1.45494649664329,5.98259974039272));
#141465=CARTESIAN_POINT('Ctrl Pts',(4.53517036468666,1.45270035228661,5.97417715517737));
#141466=CARTESIAN_POINT('',(4.53144841205905,1.4571926425566,5.81738564461188));
#141467=CARTESIAN_POINT('Ctrl Pts',(4.550013582,1.457192641,5.644455368));
#141468=CARTESIAN_POINT('Ctrl Pts',(4.859597553,1.522897175,5.394898736));
#141469=CARTESIAN_POINT('Ctrl Pts',(5.14003151800001,1.587500328,5.112981126));
#141470=CARTESIAN_POINT('Ctrl Pts',(4.895874148,1.457192641,5.681585723));
#141471=CARTESIAN_POINT('Ctrl Pts',(5.207494623,1.522897175,5.413059522));
#141472=CARTESIAN_POINT('Ctrl Pts',(5.487878254,1.587500328,5.112063406));
#141473=CARTESIAN_POINT('',(4.89587416044907,1.45719263974395,5.68158571064541));
#141474=CARTESIAN_POINT('',(5.31246397217837,1.54766053441173,5.29412175647425));
#141475=CARTESIAN_POINT('Origin',(-0.107703978192127,1.33935986531226,-0.153874175233379));
#141476=CARTESIAN_POINT('Ctrl Pts',(5.13670419329786,1.5867340151723,5.11632387889823));
#141477=CARTESIAN_POINT('Ctrl Pts',(5.16592358955562,1.57991285945224,5.14594998118021));
#141478=CARTESIAN_POINT('Ctrl Pts',(5.19519638141006,1.57325083687793,5.17559370893319));
#141479=CARTESIAN_POINT('Ctrl Pts',(5.25377489534235,1.56023621089933,5.23484917606375));
#141480=CARTESIAN_POINT('Ctrl Pts',(5.28311259043306,1.55387651466602,5.26449325097607));
#141481=CARTESIAN_POINT('Ctrl Pts',(5.3124639727899,1.54766054354084,5.2941217577837));
#141482=CARTESIAN_POINT('',(4.72294388238488,1.45719263730544,5.66302053100106));
#141483=CARTESIAN_POINT('Origin',(-5.89805981832114E-13,1.54874775200067,
-4.53630188967935E-13));
#141484=CARTESIAN_POINT('',(5.31061334361147,1.36645689999454,5.29597827676676));
#141485=CARTESIAN_POINT('Origin',(-0.122355703598187,1.48213731350686,-0.14814434441156));
#141486=CARTESIAN_POINT('',(5.69511540948564,1.45719264185527,4.88012925152646));
#141487=CARTESIAN_POINT('Origin',(-0.132882732145188,1.33929190568236,-0.13869214103061));
#141488=CARTESIAN_POINT('Origin',(-0.143902244688174,1.48214299053564,-0.128581930462383));
#141489=CARTESIAN_POINT('Ctrl Pts',(5.133400721,1.587508025,5.11963837));
#141490=CARTESIAN_POINT('Ctrl Pts',(5.411086494,1.52246862,4.841206136));
#141491=CARTESIAN_POINT('Ctrl Pts',(5.657027848,1.457192641,4.534372715));
#141492=CARTESIAN_POINT('Ctrl Pts',(5.66549068205718,1.45494649666838,4.52381458688173));
#141493=CARTESIAN_POINT('Ctrl Pts',(5.67395351611424,1.45270035233679,4.51325645876339));
#141494=CARTESIAN_POINT('Ctrl Pts',(5.13386858061824,1.587508025,5.4681964540282));
#141495=CARTESIAN_POINT('Ctrl Pts',(5.43045991200896,1.52246862,5.18973884330391));
#141496=CARTESIAN_POINT('Ctrl Pts',(5.6951931687402,1.457192641,4.88083536198855));
#141497=CARTESIAN_POINT('Ctrl Pts',(5.70430263156415,1.45494649666838,4.87020600316158));
#141498=CARTESIAN_POINT('Ctrl Pts',(5.713412094388,1.45270035233679,4.85957664433463));
#141499=CARTESIAN_POINT('',(5.67607161911655,1.4571926425566,4.70725094112458));
#141500=CARTESIAN_POINT('Ctrl Pts',(5.657027848,1.457192641,4.534372715));
#141501=CARTESIAN_POINT('Ctrl Pts',(5.905726619,1.522897175,4.224099176));
#141502=CARTESIAN_POINT('Ctrl Pts',(6.119000241,1.587500328,3.888487631));
#141503=CARTESIAN_POINT('Ctrl Pts',(6.002784315,1.457192641,4.496285186));
#141504=CARTESIAN_POINT('Ctrl Pts',(6.249394081,1.522897175,4.167047787));
#141505=CARTESIAN_POINT('Ctrl Pts',(6.45851723100001,1.587500328,3.812814601));
#141506=CARTESIAN_POINT('',(6.00278432448469,1.45719263974395,4.49628517126952));
#141507=CARTESIAN_POINT('',(6.32634120131154,1.54766053441944,4.02832541346193));
#141508=CARTESIAN_POINT('Origin',(-0.138264419467786,1.33935989120299,-0.127123575016829));
#141509=CARTESIAN_POINT('Ctrl Pts',(6.1164693003912,1.5867340151904,3.89246750855191));
#141510=CARTESIAN_POINT('Ctrl Pts',(6.15137427891944,1.57991286352367,3.91511964903068));
#141511=CARTESIAN_POINT('Ctrl Pts',(6.18633519089036,1.57325084512343,3.93777752274988));
#141512=CARTESIAN_POINT('Ctrl Pts',(6.25628239279515,1.56023621035438,3.98305501161561));
#141513=CARTESIAN_POINT('Ctrl Pts',(6.29130679201329,1.55387651355754,4.00569928945281));
#141514=CARTESIAN_POINT('Ctrl Pts',(6.3263412021866,1.5476605435511,4.02832541461568));
#141515=CARTESIAN_POINT('',(5.82990609536158,1.45719263730544,4.51532893260281));
#141516=CARTESIAN_POINT('Origin',(3.81205483845903E-13,1.54874775199939,
2.8948198005363E-13));
#141517=CARTESIAN_POINT('',(6.32493293650937,1.36645689998581,4.03053635942365));
#141518=CARTESIAN_POINT('Origin',(-0.151342008501366,1.4821373052914,-0.118378126660252));
#141519=CARTESIAN_POINT('',(6.61105030969859,1.45719264185525,3.54175307414458));
#141520=CARTESIAN_POINT('Origin',(-0.159590726309623,1.33929188180681,-0.10688373894521));
#141521=CARTESIAN_POINT('Origin',(-0.168179198710835,1.48214303405179,-0.0946410250360736));
#141522=CARTESIAN_POINT('Ctrl Pts',(6.113955579,1.587508025,3.896414657));
#141523=CARTESIAN_POINT('Ctrl Pts',(6.325294513,1.52246862,3.564797781));
#141524=CARTESIAN_POINT('Ctrl Pts',(6.49952578,1.457192641,3.212267834));
#141525=CARTESIAN_POINT('Ctrl Pts',(6.50552107216591,1.45494649670994,3.20013729012063));
#141526=CARTESIAN_POINT('Ctrl Pts',(6.51151636433198,1.45270035241989,3.18800674624118));
#141527=CARTESIAN_POINT('Ctrl Pts',(6.18934218529096,1.587508025,4.23672307106577));
#141528=CARTESIAN_POINT('Ctrl Pts',(6.41913922064845,1.52246862,3.90101727579674));
#141529=CARTESIAN_POINT('Ctrl Pts',(6.61127804385332,1.457192641,3.54242596016866));
#141530=CARTESIAN_POINT('Ctrl Pts',(6.61788953443919,1.45494649670994,3.53008684479417));
#141531=CARTESIAN_POINT('Ctrl Pts',(6.62450102502494,1.45270035241989,3.51774772941973));
#141532=CARTESIAN_POINT('',(6.55528802638805,1.4571926425566,3.37701041498213));
#141533=CARTESIAN_POINT('Ctrl Pts',(6.49952578000001,1.457192641,3.212267834));
#141534=CARTESIAN_POINT('Ctrl Pts',(6.675710472,1.522897175,2.855785434));
#141535=CARTESIAN_POINT('Ctrl Pts',(6.81185131300001,1.587500328,2.482172775));
#141536=CARTESIAN_POINT('Ctrl Pts',(6.829010959,1.457192641,3.10074335));
#141537=CARTESIAN_POINT('Ctrl Pts',(6.999078818,1.522897175,2.726189529));
#141538=CARTESIAN_POINT('Ctrl Pts',(7.12716312,1.587500328,2.335282822));
#141539=CARTESIAN_POINT('',(6.82901096511129,1.45719263974395,3.10074333355966));
#141540=CARTESIAN_POINT('',(7.04440574696063,1.54766053442346,2.57416905094527));
#141541=CARTESIAN_POINT('Origin',(-0.162359327312468,1.33935990693384,-0.094428589318758));
#141542=CARTESIAN_POINT('Ctrl Pts',(6.81023510049718,1.58673401520783,2.48660368253255));
#141543=CARTESIAN_POINT('Ctrl Pts',(6.84919357949377,1.57991286024168,2.50122269723687));
#141544=CARTESIAN_POINT('Ctrl Pts',(6.88820791919594,1.57325083844524,2.51583528792782));
#141545=CARTESIAN_POINT('Ctrl Pts',(6.96625284006547,1.56023624971961,2.54501753047916));
#141546=CARTESIAN_POINT('Ctrl Pts',(7.00532597248801,1.55387659345106,2.55960308829892));
#141547=CARTESIAN_POINT('Ctrl Pts',(7.0444057480503,1.54766054354709,2.57416905191524));
#141548=CARTESIAN_POINT('',(6.66426837919014,1.45719263730544,3.15650557154141));
#141549=CARTESIAN_POINT('Origin',(7.84962372879505E-13,1.548747752,3.46944695195361E-13));
#141550=CARTESIAN_POINT('',(7.04350569482777,1.36645690003436,2.57663104150567));
#141551=CARTESIAN_POINT('Origin',(-0.173251244287309,1.48213728690228,-0.0830763464165341));
#141552=CARTESIAN_POINT('',(7.21785984476966,1.45719264185526,2.03776846088087));
#141553=CARTESIAN_POINT('Origin',(-0.178836261220207,1.33929187072181,-0.0700775177607763));
#141554=CARTESIAN_POINT('Origin',(-0.184592117991271,1.48214298945751,-0.0562747580030781));
#141555=CARTESIAN_POINT('Ctrl Pts',(6.80862866900001,1.587508025,2.490998925));
#141556=CARTESIAN_POINT('Ctrl Pts',(6.943738791,1.52246862,2.121703444));
#141557=CARTESIAN_POINT('Ctrl Pts',(7.038113109,1.457192641,1.739960879));
#141558=CARTESIAN_POINT('Ctrl Pts',(7.04136052648581,1.45494649649692,1.72682512865051));
#141559=CARTESIAN_POINT('Ctrl Pts',(7.04460794397148,1.45270035199387,1.71368937830096));
#141560=CARTESIAN_POINT('Ctrl Pts',(6.95540902714619,1.587508025,2.80714522552581));
#141561=CARTESIAN_POINT('Ctrl Pts',(7.10766671429717,1.52246862,2.42988847541039));
#141562=CARTESIAN_POINT('Ctrl Pts',(7.21822690527199,1.457192641,2.03837665916208));
#141563=CARTESIAN_POINT('Ctrl Pts',(7.22203127816718,1.45494649649693,2.02490474916662));
#141564=CARTESIAN_POINT('Ctrl Pts',(7.22583565106249,1.45270035199386,2.01143283917115));
#141565=CARTESIAN_POINT('',(7.12798645045437,1.4571926425566,1.88886463573798));
#141566=CARTESIAN_POINT('Ctrl Pts',(7.038113109,1.457192641,1.739960879));
#141567=CARTESIAN_POINT('Ctrl Pts',(7.133545523,1.522897175,1.353938339));
#141568=CARTESIAN_POINT('Ctrl Pts',(7.18618778900001,1.587500328,0.95979428));
#141569=CARTESIAN_POINT('Ctrl Pts',(7.335920641,1.457192641,1.560214201));
#141570=CARTESIAN_POINT('Ctrl Pts',(7.421494407,1.522897175,1.157857678));
#141571=CARTESIAN_POINT('Ctrl Pts',(7.462550783,1.587500328,0.748555814));
#141572=CARTESIAN_POINT('',(7.3359206434274,1.45719263974395,1.56021418364124));
#141573=CARTESIAN_POINT('',(7.43308170912172,1.54766053441375,0.999647404332543));
#141574=CARTESIAN_POINT('Origin',(-0.17886312272908,1.3393598776417,-0.057318495887754));
#141575=CARTESIAN_POINT('Ctrl Pts',(7.18556187684235,1.5867340152581,0.964469032973011));
#141576=CARTESIAN_POINT('Ctrl Pts',(7.22675217653307,1.57991286155787,0.970371340689533));
#141577=CARTESIAN_POINT('Ctrl Pts',(7.26799564895476,1.57325084106422,0.97625536603543));
#141578=CARTESIAN_POINT('Ctrl Pts',(7.35048949777617,1.56023621202256,0.987978029095562));
#141579=CARTESIAN_POINT('Ctrl Pts',(7.39178485552251,1.55387651687792,0.993823053896906));
#141580=CARTESIAN_POINT('Ctrl Pts',(7.43308171040408,1.54766054354744,0.999647404987986));
#141581=CARTESIAN_POINT('',(7.18701688006559,1.45719263730544,1.65008751793662));
#141582=CARTESIAN_POINT('Origin',(3.56485674313234E-13,1.54874775200056,
-3.28784308806229E-14));
#141583=CARTESIAN_POINT('',(7.43273195491697,1.36645690001638,1.002245319997));
#141584=CARTESIAN_POINT('Origin',(-0.187059724892573,1.48213730249397,-0.043890175824452));
#141585=CARTESIAN_POINT('',(7.48717027514498,1.45719264185527,0.438500058308726));
#141586=CARTESIAN_POINT('Origin',(-0.189719945583939,1.33929187097265,-0.0299946459976366));
#141587=CARTESIAN_POINT('Origin',(-0.192373778352274,1.48214300277812,-0.0152772230601544));
#141588=CARTESIAN_POINT('Ctrl Pts',(7.18493785,1.587508025,0.969106852));
#141589=CARTESIAN_POINT('Ctrl Pts',(7.23750156,1.52246862,0.579400611999999));
#141590=CARTESIAN_POINT('Ctrl Pts',(7.247606092,1.457192641,0.186295287));
#141591=CARTESIAN_POINT('Ctrl Pts',(7.24795378862651,1.4549464966273,0.172768545200744));
#141592=CARTESIAN_POINT('Ctrl Pts',(7.24830148525303,1.45270035225462,0.159241803401487));
#141593=CARTESIAN_POINT('Ctrl Pts',(7.39624867482026,1.587508025,1.24630839004406));
#141594=CARTESIAN_POINT('Ctrl Pts',(7.46384761147997,1.52246862,0.845140790845598));
#141595=CARTESIAN_POINT('Ctrl Pts',(7.48765949859589,1.457192641,0.439015130051796));
#141596=CARTESIAN_POINT('Ctrl Pts',(7.48847886487837,1.4549464966273,0.42504035890971));
#141597=CARTESIAN_POINT('Ctrl Pts',(7.48929823116085,1.45270035225462,0.411065587767622));
#141598=CARTESIAN_POINT('',(7.36738815040593,1.4571926425566,0.312397644926896));
#141599=CARTESIAN_POINT('Ctrl Pts',(7.247606092,1.457192641,0.186295287));
#141600=CARTESIAN_POINT('Ctrl Pts',(7.257823913,1.522897175,-0.211217409));
#141601=CARTESIAN_POINT('Ctrl Pts',(7.224506111,1.587500328,-0.60746313));
#141602=CARTESIAN_POINT('Ctrl Pts',(7.499810826,1.457192641,-0.053268829));
#141603=CARTESIAN_POINT('Ctrl Pts',(7.496889167,1.522897175,-0.464614311000001));
#141604=CARTESIAN_POINT('Ctrl Pts',(7.448997866,1.587500328,-0.873172832));
#141605=CARTESIAN_POINT('',(7.49981082465209,1.45719263974394,-0.0532688465116229));
#141606=CARTESIAN_POINT('',(7.47419503211715,1.54766053441069,-0.621616643533504));
#141607=CARTESIAN_POINT('Origin',(-0.1870030549888,1.33935990731118,-0.0175281510573762));
#141608=CARTESIAN_POINT('Ctrl Pts',(7.22489976603804,1.58673401514931,-0.602763116835093));
#141609=CARTESIAN_POINT('Ctrl Pts',(7.26639587926554,1.57991286177347,-0.605853498624341));
#141610=CARTESIAN_POINT('Ctrl Pts',(7.30793999166598,1.57325084160804,-0.6089731658026));
#141611=CARTESIAN_POINT('Ctrl Pts',(7.39102522824991,1.56023620913844,-0.615258312705757));
#141612=CARTESIAN_POINT('Ctrl Pts',(7.43261165127053,1.55387651110979,-0.61842722407249));
#141613=CARTESIAN_POINT('Ctrl Pts',(7.47419503351237,1.54766054353441,-0.621616643124316));
#141614=CARTESIAN_POINT('',(7.37370845920419,1.45719263730544,0.0665132063634968));
#141615=CARTESIAN_POINT('Origin',(-1.13971332371676E-12,1.54874775200017,
1.87861743305637E-13));
#141616=CARTESIAN_POINT('',(7.47441192966151,1.36645689996761,-0.619004279255739));
#141617=CARTESIAN_POINT('Origin',(-0.192121367400876,1.48213734012576,-0.00265175309706843));
#141618=CARTESIAN_POINT('',(7.4063889453873,1.45719264185525,-1.18127211997309));
#141619=CARTESIAN_POINT('Origin',(-0.19173213102862,1.33929187347829,0.0114907606312091));
#141620=CARTESIAN_POINT('Origin',(-0.191160650925758,1.48214304788297,0.0264346549692207));
#141621=CARTESIAN_POINT('Ctrl Pts',(7.225287322,1.587508025,-0.59809958));
#141622=CARTESIAN_POINT('Ctrl Pts',(7.19284679999999,1.52246862,-0.989994349));
#141623=CARTESIAN_POINT('Ctrl Pts',(7.118209069,1.457192641,-1.376081265));
#141624=CARTESIAN_POINT('Ctrl Pts',(7.11564078712196,1.45494649670151,-1.38936650312861));
#141625=CARTESIAN_POINT('Ctrl Pts',(7.11307250524391,1.45270035240304,-1.40265174125726));
#141626=CARTESIAN_POINT('Ctrl Pts',(7.49124795416804,1.587508025,-0.372804441566535));
#141627=CARTESIAN_POINT('Ctrl Pts',(7.47102728937974,1.52246862,-0.779124737500378));
#141628=CARTESIAN_POINT('Ctrl Pts',(7.40697745623856,1.457192641,-1.18087425891832));
#141629=CARTESIAN_POINT('Ctrl Pts',(7.40477350357891,1.45494649670151,-1.19469844678615));
#141630=CARTESIAN_POINT('Ctrl Pts',(7.40256955091918,1.45270035240304,-1.20852263465398));
#141631=CARTESIAN_POINT('',(7.2622989688385,1.4571926425566,-1.27867671243655));
#141632=CARTESIAN_POINT('Ctrl Pts',(7.118209069,1.457192641,-1.376081265));
#141633=CARTESIAN_POINT('Ctrl Pts',(7.042734524,1.522897175,-1.766496865));
#141634=CARTESIAN_POINT('Ctrl Pts',(6.925014556,1.587500328,-2.146316238));
#141635=CARTESIAN_POINT('Ctrl Pts',(7.313018193,1.457192641,-1.664261068));
#141636=CARTESIAN_POINT('Ctrl Pts',(7.221737721,1.522897175,-2.065361451));
#141637=CARTESIAN_POINT('Ctrl Pts',(7.087138087,1.587500328,-2.454072887));
#141638=CARTESIAN_POINT('',(7.31301818791927,1.45719263974395,-1.66426108481367));
#141639=CARTESIAN_POINT('',(7.16582330191368,1.54766053442354,-2.21381458832635));
#141640=CARTESIAN_POINT('Origin',(-0.186399158114623,1.33935990274223,0.0230818051578077));
#141641=CARTESIAN_POINT('Ctrl Pts',(6.92640937124286,1.58673401530334,-2.14181073366906));
#141642=CARTESIAN_POINT('Ctrl Pts',(6.96627100042353,1.57991285972098,-2.15374930543162));
#141643=CARTESIAN_POINT('Ctrl Pts',(7.00617321276576,1.57325083728514,-2.16572679693239));
#141644=CARTESIAN_POINT('Ctrl Pts',(7.08596481245988,1.56023620958924,-2.1897258615654));
#141645=CARTESIAN_POINT('Ctrl Pts',(7.12589774304569,1.55387651195406,-2.20176053641058));
#141646=CARTESIAN_POINT('Ctrl Pts',(7.16582330336277,1.54766054355409,-2.21381458823503));
#141647=CARTESIAN_POINT('',(7.21561362633324,1.45719263730544,-1.52017118865117));
#141648=CARTESIAN_POINT('Origin',(7.45931094670027E-14,1.54874775199967,
-2.84060969191202E-14));
#141649=CARTESIAN_POINT('',(7.16659671021182,1.36645689998289,-2.21130992592685));
#141650=CARTESIAN_POINT('Origin',(-0.188199584662476,1.48213731844567,0.0387106208168392));
#141651=CARTESIAN_POINT('',(6.97929310018135,1.45719264185527,-2.7458093262454));
#141652=CARTESIAN_POINT('Origin',(-0.184779512962319,1.33929189526918,0.0524389094193656));
#141653=CARTESIAN_POINT('Origin',(-0.181008753759127,1.48214299350174,0.066910520889546));
#141654=CARTESIAN_POINT('Ctrl Pts',(6.92779039,1.587508025,-2.137339541));
#141655=CARTESIAN_POINT('Ctrl Pts',(6.811862518,1.52246862,-2.513098274));
#141656=CARTESIAN_POINT('Ctrl Pts',(6.655972501,1.457192641,-2.874113787));
#141657=CARTESIAN_POINT('Ctrl Pts',(6.65060833047937,1.45494649664132,-2.88653631930577));
#141658=CARTESIAN_POINT('Ctrl Pts',(6.64524415995863,1.45270035228267,-2.89895885161157));
#141659=CARTESIAN_POINT('Ctrl Pts',(7.23596480473053,1.587508025,-1.9744853512695));
#141660=CARTESIAN_POINT('Ctrl Pts',(7.12887003486487,1.52246862,-2.36695926009757));
#141661=CARTESIAN_POINT('Ctrl Pts',(6.97995338037145,1.457192641,-2.74554727938565));
#141662=CARTESIAN_POINT('Ctrl Pts',(6.97482916303261,1.45494649664132,-2.75857448107319));
#141663=CARTESIAN_POINT('Ctrl Pts',(6.96970494569362,1.45270035228266,-2.77160168276073));
#141664=CARTESIAN_POINT('',(6.81763275884877,1.4571926425566,-2.80996156785876));
#141665=CARTESIAN_POINT('Ctrl Pts',(6.655972501,1.457192641,-2.874113787));
#141666=CARTESIAN_POINT('Ctrl Pts',(6.498334696,1.522897175,-3.23917689));
#141667=CARTESIAN_POINT('Ctrl Pts',(6.30171701800001,1.587500328,-3.584809985));
#141668=CARTESIAN_POINT('Ctrl Pts',(6.784276957,1.457192641,-3.19743431));
#141669=CARTESIAN_POINT('Ctrl Pts',(6.608905846,1.522897175,-3.569534585));
#141670=CARTESIAN_POINT('Ctrl Pts',(6.393891608,1.587500328,-3.920223221));
#141671=CARTESIAN_POINT('',(6.78427694842449,1.45719263974394,-3.19743432531899));
#141672=CARTESIAN_POINT('',(6.52238563870992,1.54766053439312,-3.70249702286805));
#141673=CARTESIAN_POINT('Origin',(-0.177079318188234,1.33935988613101,0.0626124614222701));
#141674=CARTESIAN_POINT('Ctrl Pts',(6.30404777361277,1.58673401525752,-3.58070966061121));
#141675=CARTESIAN_POINT('Ctrl Pts',(6.34041100652666,1.57991286218685,-3.60093817965368));
#141676=CARTESIAN_POINT('Ctrl Pts',(6.37680550545298,1.57325084234179,-3.62121343167707));
#141677=CARTESIAN_POINT('Ctrl Pts',(6.44957233621988,1.56023624969758,-3.66180413737314));
#141678=CARTESIAN_POINT('Ctrl Pts',(6.48598430483409,1.55387659341557,-3.68214170613826));
#141679=CARTESIAN_POINT('Ctrl Pts',(6.52238564015445,1.54766054350425,-3.70249702306713));
#141680=CARTESIAN_POINT('',(6.72012471968049,1.45719263730544,-3.03577406913007));
#141681=CARTESIAN_POINT('Origin',(8.23993651088983E-13,1.54874775200056,
-4.59051199830363E-13));
#141682=CARTESIAN_POINT('',(6.52367939340938,1.36645690002423,-3.70021717832745));
#141683=CARTESIAN_POINT('Origin',(-0.175478228337718,1.48213730287669,0.0782630889140629));
#141684=CARTESIAN_POINT('',(6.225853266432,1.45719264185525,-4.18195553973064));
#141685=CARTESIAN_POINT('Origin',(-0.169186457812871,1.33929186673091,0.0909349252721464));
#141686=CARTESIAN_POINT('Origin',(-0.1623930351778,1.48214304712937,0.104257681158234));
#141687=CARTESIAN_POINT('Ctrl Pts',(6.30635767900001,1.587508025,-3.57663988));
#141688=CARTESIAN_POINT('Ctrl Pts',(6.112363115,1.52246862,-3.918692517));
#141689=CARTESIAN_POINT('Ctrl Pts',(5.882510057,1.457192641,-4.237755942));
#141690=CARTESIAN_POINT('Ctrl Pts',(5.87460082057932,1.45494649663718,-4.24873490431392));
#141691=CARTESIAN_POINT('Ctrl Pts',(5.86669158415865,1.45270035227438,-4.25971386662783));
#141692=CARTESIAN_POINT('Ctrl Pts',(6.64233598321045,1.587508025,-3.48384152007118));
#141693=CARTESIAN_POINT('Ctrl Pts',(6.45337474141586,1.52246862,-3.8441173967213));
#141694=CARTESIAN_POINT('Ctrl Pts',(6.22655444195791,1.457192641,-4.18184156010638));
#141695=CARTESIAN_POINT('Ctrl Pts',(6.21874956266229,1.45494649663718,-4.19346263783506));
#141696=CARTESIAN_POINT('Ctrl Pts',(6.21094468336658,1.45270035227438,-4.20508371556375));
#141697=CARTESIAN_POINT('',(6.05418161852976,1.4571926425566,-4.20985574286674));
#141698=CARTESIAN_POINT('Ctrl Pts',(5.882510057,1.457192641,-4.237755942));
#141699=CARTESIAN_POINT('Ctrl Pts',(5.65007996,1.522897175,-4.560396605));
#141700=CARTESIAN_POINT('Ctrl Pts',(5.383758195,1.587500328,-4.855682001));
#141701=CARTESIAN_POINT('Ctrl Pts',(5.938310471,1.457192641,-4.58109907600001));
#141702=CARTESIAN_POINT('Ctrl Pts',(5.687048879,1.522897175,-4.906800249));
#141703=CARTESIAN_POINT('Ctrl Pts',(5.401673864,1.587500328,-5.203068274));
#141704=CARTESIAN_POINT('',(5.93831045932958,1.45719263974394,-4.58109908912447));
#141705=CARTESIAN_POINT('',(5.57396847218265,1.54766053441674,-5.01805481222604));
#141706=CARTESIAN_POINT('Origin',(-0.159479453596245,1.3393599059375,0.0992154203879853));
#141707=CARTESIAN_POINT('Ctrl Pts',(5.38691590761031,1.58673401520329,-4.85217858324993));
#141708=CARTESIAN_POINT('Ctrl Pts',(5.41808046339618,1.5799128602683,-4.87975119871157));
#141709=CARTESIAN_POINT('Ctrl Pts',(5.44926550910829,1.57325083849597,-4.90737617685212));
#141710=CARTESIAN_POINT('Ctrl Pts',(5.51160545057504,1.56023621236661,-4.96266075465083));
#141711=CARTESIAN_POINT('Ctrl Pts',(5.54279435303737,1.55387651759433,-4.99035051879934));
#141712=CARTESIAN_POINT('Ctrl Pts',(5.57396847350867,1.54766054355305,-5.01805481278384));
#141713=CARTESIAN_POINT('',(5.91041025046353,1.45719263730544,-4.40942752714433));
#141714=CARTESIAN_POINT('Origin',(-4.93528828915402E-13,1.5487477519995,
2.74953670942324E-13));
#141715=CARTESIAN_POINT('',(5.57572207888938,1.36645689999383,-5.01610638785686));
#141716=CARTESIAN_POINT('Origin',(-0.154551226723378,1.48213732987919,0.114155825250313));
#141717=CARTESIAN_POINT('',(5.18129945413096,1.45719264185526,-5.42255816067617));
#141718=CARTESIAN_POINT('Origin',(-0.145682930593092,1.33929190911084,0.125179275449958));
#141719=CARTESIAN_POINT('Origin',(-0.13618400097974,1.48214300333004,0.136729849610384));
#141720=CARTESIAN_POINT('Ctrl Pts',(5.390046691,1.587508025,-4.848700513));
#141721=CARTESIAN_POINT('Ctrl Pts',(5.127056407,1.52246862,-5.141053053));
#141722=CARTESIAN_POINT('Ctrl Pts',(4.833987981,1.457192641,-5.40324534));
#141723=CARTESIAN_POINT('Ctrl Pts',(4.82390350610173,1.45494649670983,-5.41226736797098));
#141724=CARTESIAN_POINT('Ctrl Pts',(4.81381903120335,1.45270035241968,-5.42128939594183));
#141725=CARTESIAN_POINT('Ctrl Pts',(5.73811891470674,1.587508025,-4.83029713217703));
#141726=CARTESIAN_POINT('Ctrl Pts',(5.47612681726766,1.52246862,-5.14152887785342));
#141727=CARTESIAN_POINT('Ctrl Pts',(5.18200873880599,1.457192641,-5.42259757783759));
#141728=CARTESIAN_POINT('Ctrl Pts',(5.17188814540104,1.45494649670983,-5.4322691425584));
#141729=CARTESIAN_POINT('Ctrl Pts',(5.16176755199595,1.45270035241968,-5.44194070727923));
#141730=CARTESIAN_POINT('',(5.00764367496653,1.4571926425566,-5.41290174300688));
#141731=CARTESIAN_POINT('Ctrl Pts',(4.833987981,1.457192641,-5.40324534));
#141732=CARTESIAN_POINT('Ctrl Pts',(4.537633764,1.522897175,-5.668377243));
#141733=CARTESIAN_POINT('Ctrl Pts',(4.214060823,1.587500328,-5.899507723));
#141734=CARTESIAN_POINT('Ctrl Pts',(4.814675187,1.457192641,-5.750556742));
#141735=CARTESIAN_POINT('Ctrl Pts',(4.499271827,1.522897175,-6.014629387));
#141736=CARTESIAN_POINT('Ctrl Pts',(4.156879854,1.587500328,-6.242623638));
#141737=CARTESIAN_POINT('',(4.81467517279107,1.45719263974395,-5.75055675229159));
#141738=CARTESIAN_POINT('',(4.36491873502114,1.54766053442457,-6.09897393559969));
#141739=CARTESIAN_POINT('Origin',(-0.134422621474323,1.3393598918314,0.131179301547834));
#141740=CARTESIAN_POINT('Ctrl Pts',(4.21789784076114,1.58673401530912,-5.89676502847127));
#141741=CARTESIAN_POINT('Ctrl Pts',(4.24240649244411,1.57991285950272,-5.93039247395833));
#141742=CARTESIAN_POINT('Ctrl Pts',(4.26692389901355,1.57325083682591,-5.96407546325322));
#141743=CARTESIAN_POINT('Ctrl Pts',(4.31592182297214,1.56023620921133,-6.03146877052655));
#141744=CARTESIAN_POINT('Ctrl Pts',(4.34042907888917,1.55387651117993,-6.06521587390367));
#141745=CARTESIAN_POINT('Ctrl Pts',(4.3649187362348,1.54766054355502,-6.09897393640046));
#141746=CARTESIAN_POINT('',(4.8243315668795,1.45719263730544,-5.57690105581019));
#141747=CARTESIAN_POINT('Origin',(-1.10350097115575E-12,1.54874775199972,
1.61632859874139E-12));
#141748=CARTESIAN_POINT('',(4.36705019674112,1.36645689997257,-6.09744803763054));
#141749=CARTESIAN_POINT('Origin',(-0.126397840611546,1.48213731061574,0.144710969876972));
#141750=CARTESIAN_POINT('',(3.894473836524,1.45719264185525,-6.40960798932386));
#141751=CARTESIAN_POINT('Origin',(-0.115367111514261,1.33929186087925,0.153570173473314));
#141752=CARTESIAN_POINT('Origin',(-0.103607175345854,1.48214303893616,0.162808640033903));
#141753=CARTESIAN_POINT('Ctrl Pts',(4.221703111,1.587508025,-5.8940413));
#141754=CARTESIAN_POINT('Ctrl Pts',(3.902014239,1.52246862,-6.123023663));
#141755=CARTESIAN_POINT('Ctrl Pts',(3.559433999,1.457192641,-6.316084991));
#141756=CARTESIAN_POINT('Ctrl Pts',(3.54764582377339,1.45494649662652,-6.32272822519221));
#141757=CARTESIAN_POINT('Ctrl Pts',(3.53585764854677,1.45270035225306,-6.32937145938454));
#141758=CARTESIAN_POINT('Ctrl Pts',(4.56559378165187,1.587508025,-5.95089341824206));
#141759=CARTESIAN_POINT('Ctrl Pts',(4.24282128944063,1.52246862,-6.19852818263438));
#141760=CARTESIAN_POINT('Ctrl Pts',(3.89515806501077,1.457192641,-6.40979896017689));
#141761=CARTESIAN_POINT('Ctrl Pts',(3.88319498445065,1.45494649662652,-6.41706878095212));
#141762=CARTESIAN_POINT('Ctrl Pts',(3.87123190389051,1.45270035225306,-6.4243386017273));
#141763=CARTESIAN_POINT('',(3.72695387773219,1.4571926425566,-6.36284647384276));
#141764=CARTESIAN_POINT('Ctrl Pts',(3.559433999,1.457192641,-6.316084991));
#141765=CARTESIAN_POINT('Ctrl Pts',(3.213012857,1.522897175,-6.511310861));
#141766=CARTESIAN_POINT('Ctrl Pts',(2.847318651,1.587500328,-6.667479022));
#141767=CARTESIAN_POINT('Ctrl Pts',(3.465911043,1.457192641,-6.651124765));
#141768=CARTESIAN_POINT('Ctrl Pts',(3.101113825,1.522897175,-6.84122114));
#141769=CARTESIAN_POINT('Ctrl Pts',(2.717714761,1.587500328,-6.99028085800001));
#141770=CARTESIAN_POINT('',(3.46591102690645,1.45719263974395,-6.65112477200129));
#141771=CARTESIAN_POINT('',(2.95177024883936,1.54766053440804,-6.89471181599442));
#141772=CARTESIAN_POINT('Origin',(-0.103080109074172,1.3393599228025,0.157009065809987));
#141773=CARTESIAN_POINT('Ctrl Pts',(2.85165556024229,1.58673401520964,-6.6656252952509));
#141774=CARTESIAN_POINT('Ctrl Pts',(2.8683622922353,1.57991286510536,-6.70373515343773));
#141775=CARTESIAN_POINT('Ctrl Pts',(2.88506563246328,1.57325084832053,-6.7419011346062));
#141776=CARTESIAN_POINT('Ctrl Pts',(2.91843047321997,1.56023620891076,-6.8182519981467));
#141777=CARTESIAN_POINT('Ctrl Pts',(2.93511013399784,1.55387651065815,-6.85647844996434));
#141778=CARTESIAN_POINT('Ctrl Pts',(2.95177024985786,1.54766054352959,-6.89471181703358));
#141779=CARTESIAN_POINT('',(3.51267250109602,1.45719263730544,-6.48360488878353));
#141780=CARTESIAN_POINT('Origin',(2.16623594062604E-13,1.54874775200028,
-3.87277016011822E-13));
#141781=CARTESIAN_POINT('',(2.95417990117129,1.36645689997214,-6.89367979427387));
#141782=CARTESIAN_POINT('Origin',(-0.0923341930573607,1.48213729937307,
0.168499597711493));
#141783=CARTESIAN_POINT('',(2.42554695194354,1.45719264185525,-7.09695167098787));
#141784=CARTESIAN_POINT('Origin',(-0.079656774793801,1.33929190696925,0.174780160197634));
#141785=CARTESIAN_POINT('Origin',(-0.0661858565428452,1.48214303095805,
0.181274761702213));
#141786=CARTESIAN_POINT('Ctrl Pts',(2.855957386,1.587508025,-6.663783266));
#141787=CARTESIAN_POINT('Ctrl Pts',(2.494518222,1.52246862,-6.818688491));
#141788=CARTESIAN_POINT('Ctrl Pts',(2.118444839,1.457192641,-6.933591527));
#141789=CARTESIAN_POINT('Ctrl Pts',(2.10550416565715,1.45494649660489,-6.93754533687381));
#141790=CARTESIAN_POINT('Ctrl Pts',(2.09256349231424,1.4527003522098,-6.94149914674754));
#141791=CARTESIAN_POINT('Ctrl Pts',(3.17958655851289,1.587508025,-6.79323254192744));
#141792=CARTESIAN_POINT('Ctrl Pts',(2.8111261534172,1.52246862,-6.96569119833659));
#141793=CARTESIAN_POINT('Ctrl Pts',(2.42617413046479,1.457192641,-7.09728526595308));
#141794=CARTESIAN_POINT('Ctrl Pts',(2.41292794339896,1.45494649660489,-7.10181341370261));
#141795=CARTESIAN_POINT('Ctrl Pts',(2.39968175633314,1.4527003522098,-7.10634156145212));
#141796=CARTESIAN_POINT('',(2.27199585988443,1.4571926425566,-7.01527157445221));
#141797=CARTESIAN_POINT('Ctrl Pts',(2.118444839,1.457192641,-6.933591527));
#141798=CARTESIAN_POINT('Ctrl Pts',(1.73815504,1.522897175,-7.04978282));
#141799=CARTESIAN_POINT('Ctrl Pts',(1.347439022,1.587500328,-7.123686411));
#141800=CARTESIAN_POINT('Ctrl Pts',(1.95508475,1.457192641,-7.24069358700001));
#141801=CARTESIAN_POINT('Ctrl Pts',(1.557951187,1.522897175,-7.347924996));
#141802=CARTESIAN_POINT('Ctrl Pts',(1.151472347,1.587500328,-7.411080315));
#141803=CARTESIAN_POINT('',(1.95508473278689,1.45719263974395,-7.2406935903715));
#141804=CARTESIAN_POINT('',(1.4006002665678,1.54766053440241,-7.3680606353879));
#141805=CARTESIAN_POINT('Origin',(-0.0669178377820953,1.33935992498632,
0.175497415683959));
#141806=CARTESIAN_POINT('Ctrl Pts',(1.35207303364076,1.58673401511228,-7.12280833072784));
#141807=CARTESIAN_POINT('Ctrl Pts',(1.36019668439255,1.57991286020301,-7.16361868427083));
#141808=CARTESIAN_POINT('Ctrl Pts',(1.36830495851984,1.57325083847865,-7.20448312315888));
#141809=CARTESIAN_POINT('Ctrl Pts',(1.38447655624212,1.56023620952076,-7.28622133522495));
#141810=CARTESIAN_POINT('Ctrl Pts',(1.3925486978465,1.55387651188962,-7.32713970373119));
#141811=CARTESIAN_POINT('Ctrl Pts',(1.40060026733081,1.54766054352305,-7.36806063662321));
#141812=CARTESIAN_POINT('',(2.03676477274322,1.45719263730544,-7.08714256325266));
#141813=CARTESIAN_POINT('Origin',(2.57064335096313E-13,1.548747752,-1.34397701301303E-12));
#141814=CARTESIAN_POINT('',(1.40317543654935,1.36645689995696,-7.36757074550127));
#141815=CARTESIAN_POINT('Origin',(-0.0539530301924446,1.48213733479762,
0.184409239511821));
#141816=CARTESIAN_POINT('',(0.843204186877448,1.45719264185526,-7.45244978108034));
#141817=CARTESIAN_POINT('Origin',(-0.040221868221116,1.33929184342171,0.18781761646123));
#141818=CARTESIAN_POINT('Origin',(-0.025669781634416,1.48214301518814,0.191264884919913));
#141819=CARTESIAN_POINT('Ctrl Pts',(1.356670267,1.587508025,-7.121934132));
#141820=CARTESIAN_POINT('Ctrl Pts',(0.970381306,1.52246862,-7.195519024));
#141821=CARTESIAN_POINT('Ctrl Pts',(0.578399553,1.457192641,-7.22689103));
#141822=CARTESIAN_POINT('Ctrl Pts',(0.5649114735089,1.45494649666579,-7.22797053971566));
#141823=CARTESIAN_POINT('Ctrl Pts',(0.551423394017799,1.45270035233161,
-7.22905004943133));
#141824=CARTESIAN_POINT('Ctrl Pts',(1.64490540234363,1.587508025,-7.31792766322871));
#141825=CARTESIAN_POINT('Ctrl Pts',(1.24798588253044,1.52246862,-7.40714623569068));
#141826=CARTESIAN_POINT('Ctrl Pts',(0.843744989249345,1.457192641,-7.45291040161445));
#141827=CARTESIAN_POINT('Ctrl Pts',(0.829835073136161,1.45494649666579,
-7.45448514508938));
#141828=CARTESIAN_POINT('Ctrl Pts',(0.815925157022971,1.45270035233161,
-7.4560598885642));
#141829=CARTESIAN_POINT('',(0.710801840462912,1.4571926425566,-7.33967037392361));
#141830=CARTESIAN_POINT('Ctrl Pts',(0.578399553,1.457192641,-7.22689103));
#141831=CARTESIAN_POINT('Ctrl Pts',(0.182023025,1.522897175,-7.258614769));
#141832=CARTESIAN_POINT('Ctrl Pts',(-0.215445357,1.587500328,-7.246798141));
#141833=CARTESIAN_POINT('Ctrl Pts',(0.352840867,1.457192641,-7.491695624));
#141834=CARTESIAN_POINT('Ctrl Pts',(-0.058059517,1.522897175,-7.511048045));
#141835=CARTESIAN_POINT('Ctrl Pts',(-0.468611634,1.587500328,-7.48534589300001));
#141836=CARTESIAN_POINT('Ctrl Pts',(-0.210730925521493,1.58673401525584,
-7.24693676521558));
#141837=CARTESIAN_POINT('Ctrl Pts',(-0.211570220744212,1.5799128597931,
-7.28853934333384));
#141838=CARTESIAN_POINT('Ctrl Pts',(-0.212436159925911,1.57325083749109,
-7.33019143731403));
#141839=CARTESIAN_POINT('Ctrl Pts',(-0.214213944260977,1.5602362096519,
-7.41349506349758));
#141840=CARTESIAN_POINT('Ctrl Pts',(-0.2151267644695,1.55387651209001,-7.45519205454709));
#141841=CARTESIAN_POINT('Ctrl Pts',(-0.216060227165612,1.54766054354964,
-7.49688712930759));
#141842=CARTESIAN_POINT('',(0.46562018740775,1.45719263730544,-7.35929332842941));
#141843=CARTESIAN_POINT('Ctrl Pts',(-0.206053246,1.587508025,-7.247071275));
#141844=CARTESIAN_POINT('Ctrl Pts',(-0.599129562,1.52246862,-7.235895084));
#141845=CARTESIAN_POINT('Ctrl Pts',(-0.988691053,1.457192641,-7.18226914));
#141846=CARTESIAN_POINT('Ctrl Pts',(-1.00209585148419,1.45494649664392,
-7.1804238729768));
#141847=CARTESIAN_POINT('Ctrl Pts',(-1.01550064996838,1.45270035228786,
-7.17857860595374));
#141848=CARTESIAN_POINT('Ctrl Pts',(0.0333102964716851,1.587508025,-7.50044461905109));
#141849=CARTESIAN_POINT('Ctrl Pts',(-0.373508820892593,1.52246862,-7.50225134758072));
#141850=CARTESIAN_POINT('Ctrl Pts',(-0.77813672912649,1.457192641,-7.46004573014393));
#141851=CARTESIAN_POINT('Ctrl Pts',(-0.79205996254731,1.45494649664392,
-7.45859343619367));
#141852=CARTESIAN_POINT('Ctrl Pts',(-0.80598319596813,1.45270035228786,
-7.45714114224333));
#141853=CARTESIAN_POINT('',(-0.883628482512665,1.4571926425566,-7.32087434385182));
#141854=CARTESIAN_POINT('Ctrl Pts',(-0.988691053000001,1.457192641,-7.18226914));
#141855=CARTESIAN_POINT('Ctrl Pts',(-1.382620184,1.522897175,-7.128041959));
#141856=CARTESIAN_POINT('Ctrl Pts',(-1.768255751,1.587500328,-7.031057645));
#141857=CARTESIAN_POINT('Ctrl Pts',(-1.265901463,1.457192641,-7.3923943));
#141858=CARTESIAN_POINT('Ctrl Pts',(-1.671355422,1.522897175,-7.322962836));
#141859=CARTESIAN_POINT('Ctrl Pts',(-2.066783856,1.587500328,-7.209605016));
#141860=CARTESIAN_POINT('',(-1.26590148003712,1.45719263974395,-7.39239429583215));
#141861=CARTESIAN_POINT('',(-1.82261798538781,1.54766053442901,-7.27516751052101));
#141862=CARTESIAN_POINT('Origin',(0.0129564616365227,1.3393598983656,0.187375177902643));
#141863=CARTESIAN_POINT('Ctrl Pts',(-1.76368133957537,1.58673401513823,
-7.03220649175476));
#141864=CARTESIAN_POINT('Ctrl Pts',(-1.77344433386828,1.57991286204784,
-7.07265598690311));
#141865=CARTESIAN_POINT('Ctrl Pts',(-1.78324399311111,1.57325084218189,
-7.11314811086283));
#141866=CARTESIAN_POINT('Ctrl Pts',(-1.8028879778074,1.56023624969878,-7.19412175345604));
#141867=CARTESIAN_POINT('Ctrl Pts',(-1.81274300853095,1.5538765934469,-7.23464738147635));
#141868=CARTESIAN_POINT('Ctrl Pts',(-1.82261798519599,1.54766054355515,
-7.27516751196777));
#141869=CARTESIAN_POINT('',(-1.12729628037134,1.45719263730544,-7.28733171653932));
#141870=CARTESIAN_POINT('Origin',(-6.00648003556969E-14,1.54874775200072,
-2.22044604925031E-13));
#141871=CARTESIAN_POINT('',(-1.82007512541694,1.36645689996024,-7.27580418490887));
#141872=CARTESIAN_POINT('Origin',(0.0284649540105197,1.4821373527878,0.190019460791293));
#141873=CARTESIAN_POINT('',(-2.36393104912784,1.45719264185525,-7.11771248581866));
#141874=CARTESIAN_POINT('Origin',(0.0423581924463326,1.33929188429066,0.187347329950757));
#141875=CARTESIAN_POINT('Origin',(0.0570127905286599,1.48214303509046,0.184365834749383));
#141876=CARTESIAN_POINT('Ctrl Pts',(-1.759141937,1.587508025,-7.033343419));
#141877=CARTESIAN_POINT('Ctrl Pts',(-2.140625797,1.52246862,-6.937928732));
#141878=CARTESIAN_POINT('Ctrl Pts',(-2.509551565,1.457192641,-6.801812328));
#141879=CARTESIAN_POINT('Ctrl Pts',(-2.5222462887854,1.45494649666663,-6.79712856692576));
#141880=CARTESIAN_POINT('Ctrl Pts',(-2.53494101257083,1.45270035233327,
-6.79244480585149));
#141881=CARTESIAN_POINT('Ctrl Pts',(-1.57984236134693,1.587508025,-7.33224912070202));
#141882=CARTESIAN_POINT('Ctrl Pts',(-1.97753866648013,1.52246862,-7.24655952393732));
#141883=CARTESIAN_POINT('Ctrl Pts',(-2.36363363973656,1.457192641,-7.1183576107052));
#141884=CARTESIAN_POINT('Ctrl Pts',(-2.37691915532143,1.45494649666663,
-7.11394618700318));
#141885=CARTESIAN_POINT('Ctrl Pts',(-2.39020467090635,1.45270035233327,
-7.10953476330116));
#141886=CARTESIAN_POINT('',(-2.43674132054344,1.4571926425566,-6.95976236583373));
#141887=CARTESIAN_POINT('Ctrl Pts',(-2.509551565,1.457192641,-6.801812328));
#141888=CARTESIAN_POINT('Ctrl Pts',(-2.88261361,1.522897175,-6.66416983));
#141889=CARTESIAN_POINT('Ctrl Pts',(-3.238384471,1.587500328,-6.486552707));
#141890=CARTESIAN_POINT('Ctrl Pts',(-2.825451647,1.457192641,-6.947432835));
#141891=CARTESIAN_POINT('Ctrl Pts',(-3.206500606,1.522897175,-6.792464023));
#141892=CARTESIAN_POINT('Ctrl Pts',(-3.568315562,1.587500328,-6.596751022));
#141893=CARTESIAN_POINT('',(-2.82545166272092,1.45719263974396,-6.94743282726797));
#141894=CARTESIAN_POINT('',(-3.34395215211899,1.54766053439511,-6.71326914643272));
#141895=CARTESIAN_POINT('Origin',(0.0529337710475369,1.33935993033793,0.180209392100278));
#141896=CARTESIAN_POINT('Ctrl Pts',(-3.23416397491896,1.58673401514799,
-6.48865805757573));
#141897=CARTESIAN_POINT('Ctrl Pts',(-3.25239416131963,1.57991286216089,
-6.5260631103915));
#141898=CARTESIAN_POINT('Ctrl Pts',(-3.27066931941682,1.57325084239135,
-6.56350191339419));
#141899=CARTESIAN_POINT('Ctrl Pts',(-3.3072610931085,1.56023620907719,-6.63835979603121));
#141900=CARTESIAN_POINT('Ctrl Pts',(-3.32559766007564,1.55387651099262,
-6.67581968015788));
#141901=CARTESIAN_POINT('Ctrl Pts',(-3.34395215225177,1.54766054351071,
-6.71326914788068));
#141902=CARTESIAN_POINT('',(-2.66750162710437,1.45719263730544,-6.87462257331105));
#141903=CARTESIAN_POINT('Origin',(6.51388665229291E-13,1.54874775200017,
1.46887710328336E-12));
#141904=CARTESIAN_POINT('',(-3.34160560871151,1.36645689996004,-6.7144375749348));
#141905=CARTESIAN_POINT('Origin',(0.0686481189057614,1.48213732606978,0.179457952751823));
#141906=CARTESIAN_POINT('',(-3.83876144062859,1.45719264185526,-6.44312902495316));
#141907=CARTESIAN_POINT('Origin',(0.0816420330951445,1.33929190588146,0.173861516083871));
#141908=CARTESIAN_POINT('Origin',(0.095313027403887,1.48214302028424,0.167799306102822));
#141909=CARTESIAN_POINT('Ctrl Pts',(-3.229975107,1.587508025,-6.490744241));
#141910=CARTESIAN_POINT('Ctrl Pts',(-3.582028749,1.52246862,-6.315552544));
#141911=CARTESIAN_POINT('Ctrl Pts',(-3.913068234,1.457192641,-6.103310331));
#141912=CARTESIAN_POINT('Ctrl Pts',(-3.92445929216235,1.4549464966363,-6.0960070831932));
#141913=CARTESIAN_POINT('Ctrl Pts',(-3.93585035032469,1.45270035227262,
-6.08870383538653));
#141914=CARTESIAN_POINT('Ctrl Pts',(-3.1191233455948,1.587508025,-6.8212058036725));
#141915=CARTESIAN_POINT('Ctrl Pts',(-3.48910100234763,1.52246862,-6.65202663174526));
#141916=CARTESIAN_POINT('Ctrl Pts',(-3.83860966728736,1.457192641,-6.44382300141562));
#141917=CARTESIAN_POINT('Ctrl Pts',(-3.85063624934469,1.4549464966363,-6.43665872111024));
#141918=CARTESIAN_POINT('Ctrl Pts',(-3.86266283140208,1.45270035227263,
-6.42949444080476));
#141919=CARTESIAN_POINT('',(-3.87591484165136,1.4571926425566,-6.27321963496368));
#141920=CARTESIAN_POINT('Ctrl Pts',(-3.913068234,1.457192641,-6.103310331));
#141921=CARTESIAN_POINT('Ctrl Pts',(-4.247819228,1.522897175,-5.888688526));
#141922=CARTESIAN_POINT('Ctrl Pts',(-4.557089932,1.587500328,-5.638743774));
#141923=CARTESIAN_POINT('Ctrl Pts',(-4.252886852,1.457192641,-6.177617131));
#141924=CARTESIAN_POINT('Ctrl Pts',(-4.591713385,1.522897175,-5.944357142));
#141925=CARTESIAN_POINT('Ctrl Pts',(-4.902996799,1.587500328,-5.675440282));
#141926=CARTESIAN_POINT('',(-4.2528868657407,1.45719263974395,-6.17761712005628));
#141927=CARTESIAN_POINT('',(-4.70892683314116,1.54766053440519,-5.83746577820715));
#141928=CARTESIAN_POINT('Origin',(0.0904358410859302,1.33935992808476,0.164616946156038));
#141929=CARTESIAN_POINT('Ctrl Pts',(-4.55342069736999,1.58673401524537,
-5.64170718417167));
#141930=CARTESIAN_POINT('Ctrl Pts',(-4.57926564391121,1.57991286459559,
-5.67431876527237));
#141931=CARTESIAN_POINT('Ctrl Pts',(-4.60516176487816,1.57325084723576,
-5.706953638461));
#141932=CARTESIAN_POINT('Ctrl Pts',(-4.65699029618465,1.56023620867294,
-5.77219526201295));
#141933=CARTESIAN_POINT('Ctrl Pts',(-4.68295093425734,1.55387651012817,
-5.8048375375051));
#141934=CARTESIAN_POINT('Ctrl Pts',(-4.70892683357838,1.54766054352409,
-5.8374657795963));
#141935=CARTESIAN_POINT('',(-4.08297756185057,1.45719263730544,-6.14046371846569));
#141936=CARTESIAN_POINT('Origin',(2.7148422399037E-13,1.54874775199939,
3.90312782094782E-13));
#141937=CARTESIAN_POINT('',(-4.7068863277423,1.36645689996666,-5.8391113271748));
#141938=CARTESIAN_POINT('Origin',(0.105621170002923,1.48213731632719,0.16050482919108));
#141939=CARTESIAN_POINT('',(-5.13409561478569,1.45719264185526,-5.46727201252331));
#141940=CARTESIAN_POINT('Origin',(0.117108542340334,1.33929187422864,0.15224631969547));
#141941=CARTESIAN_POINT('Origin',(0.129156500169967,1.48214300490656,0.143386714287882));
#141942=CARTESIAN_POINT('Ctrl Pts',(-4.549778231,1.587508025,-5.64464507700001));
#141943=CARTESIAN_POINT('Ctrl Pts',(-4.855940018,1.52246862,-5.397868138));
#141944=CARTESIAN_POINT('Ctrl Pts',(-5.133614182,1.457192641,-5.119424326));
#141945=CARTESIAN_POINT('Ctrl Pts',(-5.14316894137441,1.45494649658638,
-5.10984308306178));
#141946=CARTESIAN_POINT('Ctrl Pts',(-5.15272370074882,1.45270035217278,
-5.10026184012343));
#141947=CARTESIAN_POINT('Ctrl Pts',(-4.51255758975684,1.587508025,-5.99121048346444));
#141948=CARTESIAN_POINT('Ctrl Pts',(-4.83751685385146,1.52246862,-5.74645236734487));
#141949=CARTESIAN_POINT('Ctrl Pts',(-5.13409657423949,1.457192641,-5.46798239101524));
#141950=CARTESIAN_POINT('Ctrl Pts',(-5.14430187322309,1.45494649658638,
-5.45840024776324));
#141951=CARTESIAN_POINT('Ctrl Pts',(-5.1545071722067,1.45270035217278,-5.44881810451121));
#141952=CARTESIAN_POINT('',(-5.13385489337812,1.4571926425566,-5.29334812632913));
#141953=CARTESIAN_POINT('Ctrl Pts',(-5.133614182,1.457192641,-5.119424326));
#141954=CARTESIAN_POINT('Ctrl Pts',(-5.41440154,1.522897175,-4.837858691));
#141955=CARTESIAN_POINT('Ctrl Pts',(-5.662710933,1.587500328,-4.527273449));
#141956=CARTESIAN_POINT('Ctrl Pts',(-5.481461795,1.457192641,-5.118942917));
#141957=CARTESIAN_POINT('Ctrl Pts',(-5.762222749,1.522897175,-4.818298728));
#141958=CARTESIAN_POINT('Ctrl Pts',(-6.008419354,1.587500328,-4.488752262));
#141959=CARTESIAN_POINT('',(-5.48146180605169,1.45719263974395,-5.11894290336604));
#141960=CARTESIAN_POINT('',(-5.85371732860827,1.54766053443418,-4.68870899802457));
#141961=CARTESIAN_POINT('Origin',(0.123709297947897,1.33935991377548,0.14132727420044));
#141962=CARTESIAN_POINT('Ctrl Pts',(-5.65976452885599,1.58673401514067,
-4.53095635370605));
#141963=CARTESIAN_POINT('Ctrl Pts',(-5.69201580749368,1.57991285466834,
-4.557249632553));
#141964=CARTESIAN_POINT('Ctrl Pts',(-5.72432207704209,1.57325082725242,
-4.58355466254332));
#141965=CARTESIAN_POINT('Ctrl Pts',(-5.78896380224465,1.560236209744,-4.63612928610754));
#141966=CARTESIAN_POINT('Ctrl Pts',(-5.82133461356332,1.55387651227514,
-4.66242762888687));
#141967=CARTESIAN_POINT('Ctrl Pts',(-5.85371732934915,1.54766054357026,
-4.68870899927252));
#141968=CARTESIAN_POINT('',(-5.30753800421536,1.45719263730544,-5.11918360520642));
#141969=CARTESIAN_POINT('Origin',(9.69710423071035E-13,1.54874775199978,
7.9580439460436E-13));
#141970=CARTESIAN_POINT('',(-5.85207827353352,1.36645689999347,-4.69075472315437));
#141971=CARTESIAN_POINT('Origin',(0.137655674484553,1.48213726869552,0.134046934225625));
#141972=CARTESIAN_POINT('',(-6.18936518382049,1.45719264185526,-4.2357714367106));
#141973=CARTESIAN_POINT('Origin',(0.147099097618275,1.33929186443815,0.123512037903616));
#141974=CARTESIAN_POINT('Origin',(0.156960848221607,1.482142982868,0.112269617512034));
#141975=CARTESIAN_POINT('Ctrl Pts',(-5.65683878100001,1.587508025,-4.534608583));
#141976=CARTESIAN_POINT('Ctrl Pts',(-5.902792929,1.52246862,-4.227785417));
#141977=CARTESIAN_POINT('Ctrl Pts',(-6.11411803600001,1.457192641,-3.89615973));
#141978=CARTESIAN_POINT('Ctrl Pts',(-6.12138972626193,1.45494649662288,
-3.88474850057724));
#141979=CARTESIAN_POINT('Ctrl Pts',(-6.12866141652386,1.45270035224577,
-3.87333727115454));
#141980=CARTESIAN_POINT('Ctrl Pts',(-5.69498965629825,1.587508025,-4.88107282024414));
#141981=CARTESIAN_POINT('Ctrl Pts',(-5.95973579320592,1.52246862,-4.57218037652381));
#141982=CARTESIAN_POINT('Ctrl Pts',(-6.18951883121766,1.457192641,-4.23646500068588));
#141983=CARTESIAN_POINT('Ctrl Pts',(-6.19742565830312,1.45494649662288,
-4.2249130451993));
#141984=CARTESIAN_POINT('Ctrl Pts',(-6.20533248538868,1.45270035224577,
-4.2133610897127));
#141985=CARTESIAN_POINT('',(-6.15174159578327,1.4571926425566,-4.0659655425065));
#141986=CARTESIAN_POINT('Ctrl Pts',(-6.11411803599999,1.457192641,-3.89615973));
#141987=CARTESIAN_POINT('Ctrl Pts',(-6.327812453,1.522897175,-3.560815961));
#141988=CARTESIAN_POINT('Ctrl Pts',(-6.503549865,1.587500328,-3.20411285));
#141989=CARTESIAN_POINT('Ctrl Pts',(-6.45372967700001,1.457192641,-3.820912621));
#141990=CARTESIAN_POINT('Ctrl Pts',(-6.663296982,1.522897175,-3.46694202));
#141991=CARTESIAN_POINT('Ctrl Pts',(-6.83289489800001,1.587500328,-3.092175175));
#141992=CARTESIAN_POINT('',(-6.4537296848518,1.45719263974395,-3.82091260531775));
#141993=CARTESIAN_POINT('',(-6.72479450781096,1.54766053411122,-3.32071339617971));
#141994=CARTESIAN_POINT('Origin',(0.151198256987238,1.33935992429777,0.111429286576262));
#141995=CARTESIAN_POINT('Ctrl Pts',(-6.50146406158762,1.58673401527825,
-3.20834303966898));
#141996=CARTESIAN_POINT('Ctrl Pts',(-6.53861356713749,1.579912860971,-3.2270885076737));
#141997=CARTESIAN_POINT('Ctrl Pts',(-6.57581930002437,1.57325083984644,
-3.24583362870954));
#141998=CARTESIAN_POINT('Ctrl Pts',(-6.65025181673889,1.56023620668024,
-3.28328307158585));
#141999=CARTESIAN_POINT('Ctrl Pts',(-6.68751920262667,1.55387650601835,
-3.30200781611423));
#142000=CARTESIAN_POINT('Ctrl Pts',(-6.72479450885229,1.54766054352925,
-3.32071339723427));
#142001=CARTESIAN_POINT('',(-6.2839238683453,1.45719263730544,-3.85853615620902));
#142002=CARTESIAN_POINT('Ctrl Pts',(-6.499391838,1.587508025,-3.212538831));
#142003=CARTESIAN_POINT('Ctrl Pts',(-6.673637803,1.52246862,-2.860016149));
#142004=CARTESIAN_POINT('Ctrl Pts',(-6.808732526,1.457192641,-2.490715035));
#142005=CARTESIAN_POINT('Ctrl Pts',(-6.81338107273537,1.45494652485023,
-2.47800755502054));
#142006=CARTESIAN_POINT('Ctrl Pts',(-6.81802961947073,1.45270040870047,
-2.46530007504108));
#142007=CARTESIAN_POINT('Ctrl Pts',(-6.61113033294257,1.587508025,-3.54270160823892));
#142008=CARTESIAN_POINT('Ctrl Pts',(-6.8032841072071,1.52246862,-3.18411830528917));
#142009=CARTESIAN_POINT('Ctrl Pts',(-6.955526062239,1.457192641,-2.80685520692023));
#142010=CARTESIAN_POINT('Ctrl Pts',(-6.96076463727239,1.45494652485023,
-2.79387375875293));
#142011=CARTESIAN_POINT('Ctrl Pts',(-6.96600321230576,1.45270040870047,
-2.78089231058564));
#142012=CARTESIAN_POINT('',(-6.95522691796392,1.45719264137165,-2.80621090518347));
#142013=CARTESIAN_POINT('Origin',(0.177429031347391,1.48214211412438,0.0759042936399814));
#142014=CARTESIAN_POINT('',(-6.88197969794138,1.4571926425566,-2.64846292855763));
#142015=CARTESIAN_POINT('Origin',(2.9316826744008E-13,1.54874775200017,
1.08637057683048E-13));
#142016=CARTESIAN_POINT('',(-6.72363354338728,1.36645689999664,-3.32306364210357));
#142017=CARTESIAN_POINT('Origin',(0.163253390778436,1.48213728905676,0.101321039931211));
#142018=CARTESIAN_POINT('Origin',(0.170211330103566,1.33929193126131,0.0890023750191199));
#142019=CARTESIAN_POINT('Ctrl Pts',(-6.808732526,1.457192641,-2.490715035));
#142020=CARTESIAN_POINT('Ctrl Pts',(-6.94534188900001,1.522897175,-2.117273434));
#142021=CARTESIAN_POINT('Ctrl Pts',(-7.040290033,1.587500328,-1.731131494));
#142022=CARTESIAN_POINT('Ctrl Pts',(-7.124228332,1.457192641,-2.344220698));
#142023=CARTESIAN_POINT('Ctrl Pts',(-7.252802854,1.522897175,-1.953474957));
#142024=CARTESIAN_POINT('Ctrl Pts',(-7.337871871,1.587500328,-1.551011413));
#142025=CARTESIAN_POINT('',(-7.12422833628606,1.45719263974321,-2.34422068100311));
#142026=CARTESIAN_POINT('',(-6.96648043642576,1.45719263730326,-2.41746784510099));
#142027=CARTESIAN_POINT('',(-7.28142776962645,1.54766053439865,-1.79744492686919));
#142028=CARTESIAN_POINT('Origin',(0.171617199416872,1.33935992031392,0.0763209337251755));
#142029=CARTESIAN_POINT('Ctrl Pts',(-7.03916236014505,1.58673401520612,
-1.73571117070114));
#142030=CARTESIAN_POINT('Ctrl Pts',(-7.07947305391297,1.57991286063993,
-1.74603233503983));
#142031=CARTESIAN_POINT('Ctrl Pts',(-7.11983858607961,1.57325083925278,
-1.75634107332856));
#142032=CARTESIAN_POINT('Ctrl Pts',(-7.20058116476357,1.5602362496801,-1.77691410944693));
#142033=CARTESIAN_POINT('Ctrl Pts',(-7.2410022248956,1.55387659341529,-1.78718961737455));
#142034=CARTESIAN_POINT('Ctrl Pts',(-7.28142777080766,1.54766054350339,
-1.79744492773161));
#142035=CARTESIAN_POINT('Origin',(2.97071395261028E-13,1.54874775199939,
9.81202966099382E-14));
#142036=CARTESIAN_POINT('',(-7.39586996682369,1.45719264185526,-1.24543505334299));
#142037=CARTESIAN_POINT('Origin',(0.189594667274074,1.48214300128502,0.0359870116380092));
#142038=CARTESIAN_POINT('',(-7.28079918149878,1.36645690001541,-1.79998979818328));
#142039=CARTESIAN_POINT('Origin',(0.181217841331761,1.48213730043766,0.0638576089250154));
#142040=CARTESIAN_POINT('Origin',(0.185364917278654,1.33929188297289,0.050331179048184));
#142041=CARTESIAN_POINT('Ctrl Pts',(-7.03804055500001,1.587508025,-1.740254334));
#142042=CARTESIAN_POINT('Ctrl Pts',(-7.13243079,1.52246862,-1.358515705));
#142043=CARTESIAN_POINT('Ctrl Pts',(-7.184978251,1.457192641,-0.968807273));
#142044=CARTESIAN_POINT('Ctrl Pts',(-7.18678640753855,1.4549464965433,-0.955397417679967));
#142045=CARTESIAN_POINT('Ctrl Pts',(-7.18859456407698,1.45270035208663,
-0.941987562359948));
#142046=CARTESIAN_POINT('Ctrl Pts',(-7.21814190790164,1.587508025,-2.03867762345543));
#142047=CARTESIAN_POINT('Ctrl Pts',(-7.32871842370705,1.52246862,-1.64717041658003));
#142048=CARTESIAN_POINT('Ctrl Pts',(-7.39630063339368,1.457192641,-1.24600000010623));
#142049=CARTESIAN_POINT('Ctrl Pts',(-7.3986261351783,1.4549464965433,-1.23219573824825));
#142050=CARTESIAN_POINT('Ctrl Pts',(-7.40095163696292,1.45270035208663,
-1.2183914763903));
#142051=CARTESIAN_POINT('',(-7.29042407893858,1.4571926425566,-1.10712113202695));
#142052=CARTESIAN_POINT('Ctrl Pts',(-7.18497825100001,1.457192641,-0.968807273));
#142053=CARTESIAN_POINT('Ctrl Pts',(-7.238114857,1.522897175,-0.574729554));
#142054=CARTESIAN_POINT('Ctrl Pts',(-7.247834064,1.587500328,-0.177204354));
#142055=CARTESIAN_POINT('Ctrl Pts',(-7.461605988,1.457192641,-0.757915620000001));
#142056=CARTESIAN_POINT('Ctrl Pts',(-7.50317572500001,1.522897175,-0.348665576));
#142057=CARTESIAN_POINT('Ctrl Pts',(-7.499738111,1.587500328,0.062675918));
#142058=CARTESIAN_POINT('',(-7.46160598853109,1.45719263974396,-0.757915602491484));
#142059=CARTESIAN_POINT('',(-7.49758956218103,1.54766053442178,-0.190129930142415));
#142060=CARTESIAN_POINT('Origin',(0.184011793195198,1.33935989717502,0.0376439855327804));
#142061=CARTESIAN_POINT('Ctrl Pts',(-7.24771725059273,1.58673401519803,
-0.181919376803811));
#142062=CARTESIAN_POINT('Ctrl Pts',(-7.28930422196723,1.57991286491238,
-0.18333362947525));
#142063=CARTESIAN_POINT('Ctrl Pts',(-7.33094207499939,1.57325084793404,
-0.184723957980302));
#142064=CARTESIAN_POINT('Ctrl Pts',(-7.41421984954447,1.56023620870582,
-0.187458750645032));
#142065=CARTESIAN_POINT('Ctrl Pts',(-7.45590511399854,1.55387651022022,
-0.18880469894532));
#142066=CARTESIAN_POINT('Ctrl Pts',(-7.4975895635242,1.54766054354907,-0.190129930705154));
#142067=CARTESIAN_POINT('',(-7.32329212215043,1.45719263730543,-0.863361424018223));
#142068=CARTESIAN_POINT('Origin',(-2.48412401759879E-12,1.54874775199939,
-1.02673945734377E-13));
#142069=CARTESIAN_POINT('',(-7.49752274173799,1.36645690002332,-0.192750431785836));
#142070=CARTESIAN_POINT('Origin',(0.190708686305372,1.48213731107654,0.0234081809724727));
#142071=CARTESIAN_POINT('',(-7.4906903586766,1.45719264185525,0.373575949174442));
#142072=CARTESIAN_POINT('Origin',(0.191850856540546,1.33929189026274,0.00930648937180201));
#142073=CARTESIAN_POINT('Origin',(0.192898202986575,1.48214301628634,-0.0056115938680452));
#142074=CARTESIAN_POINT('Ctrl Pts',(-7.24759831800001,1.587508025,-0.186597478));
#142075=CARTESIAN_POINT('Ctrl Pts',(-7.257719241,1.52246862,0.206507424));
#142076=CARTESIAN_POINT('Ctrl Pts',(-7.225262378,1.457192641,0.59840084));
#142077=CARTESIAN_POINT('Ctrl Pts',(-7.22414553838937,1.45494649666465,
0.611885879824641));
#142078=CARTESIAN_POINT('Ctrl Pts',(-7.22302869877862,1.45270035232932,
0.625370919649284));
#142079=CARTESIAN_POINT('Ctrl Pts',(-7.48764118811158,1.587508025,-0.439327329442798));
#142080=CARTESIAN_POINT('Ctrl Pts',(-7.51147000933402,1.52246862,-0.0332026618115801));
#142081=CARTESIAN_POINT('Ctrl Pts',(-7.49123240332272,1.457192641,0.373116791162346));
#142082=CARTESIAN_POINT('Ctrl Pts',(-7.49053602795158,1.45494649666465,
0.387098230454708));
#142083=CARTESIAN_POINT('Ctrl Pts',(-7.48983965258032,1.45270035232932,
0.401079669747064));
#142084=CARTESIAN_POINT('',(-7.35797633236851,1.4571926425566,0.485988418560827));
#142085=CARTESIAN_POINT('Ctrl Pts',(-7.225262378,1.457192641,0.59840084));
#142086=CARTESIAN_POINT('Ctrl Pts',(-7.192441619,1.522897175,0.994688041));
#142087=CARTESIAN_POINT('Ctrl Pts',(-7.116477429,1.587500328,1.385008664));
#142088=CARTESIAN_POINT('Ctrl Pts',(-7.450087241,1.457192641,0.86382875));
#142089=CARTESIAN_POINT('Ctrl Pts',(-7.402708438,1.522897175,1.27244702));
#142090=CARTESIAN_POINT('Ctrl Pts',(-7.310924932,1.587500328,1.673432593));
#142091=CARTESIAN_POINT('',(-7.45008723775429,1.45719263974396,0.863828767210929));
#142092=CARTESIAN_POINT('',(-7.36317239925506,1.54766053442505,1.42607533061921));
#142093=CARTESIAN_POINT('Origin',(0.187802206685309,1.33935989621408,-0.00279323486872568));
#142094=CARTESIAN_POINT('Ctrl Pts',(-7.11737693722939,1.58673401523545,
1.38037876479302));
#142095=CARTESIAN_POINT('Ctrl Pts',(-7.15829567894936,1.57991286024203,
1.38793755122839));
#142096=CARTESIAN_POINT('Ctrl Pts',(-7.19925897331848,1.57325083844015,
1.39553064135406));
#142097=CARTESIAN_POINT('Ctrl Pts',(-7.2811773413793,1.56023624971792,1.41076198743301));
#142098=CARTESIAN_POINT('Ctrl Pts',(-7.32217707587334,1.55387659344704,
1.4184085517289));
#142099=CARTESIAN_POINT('Ctrl Pts',(-7.36317240068876,1.54766054355037,
1.42607533035161));
#142100=CARTESIAN_POINT('',(-7.33767480725555,1.45719263730543,0.73111481752593));
#142101=CARTESIAN_POINT('Origin',(-3.37837396946483E-13,1.54874775200022,
4.32054565735474E-14));
#142102=CARTESIAN_POINT('',(-7.36367047181139,1.36645689998334,1.42350173056156));
#142103=CARTESIAN_POINT('Origin',(0.191281723351053,1.48213728127495,-0.0181357654416722));
#142104=CARTESIAN_POINT('',(-7.23525439421974,1.45719264185526,1.97511895503844));
#142105=CARTESIAN_POINT('Origin',(0.189366035974033,1.33929190661057,-0.0321533450512154));
#142106=CARTESIAN_POINT('Origin',(0.187181716114306,1.48214299980185,-0.0469477408946925));
#142107=CARTESIAN_POINT('Ctrl Pts',(-7.118266439,1.587508025,1.375784468));
#142108=CARTESIAN_POINT('Ctrl Pts',(-7.043644806,1.52246862,1.761874495));
#142109=CARTESIAN_POINT('Ctrl Pts',(-6.927701267,1.457192641,2.137628395));
#142110=CARTESIAN_POINT('Ctrl Pts',(-6.92371165326549,1.45494649650072,
2.15055807554245));
#142111=CARTESIAN_POINT('Ctrl Pts',(-6.91972203953099,1.45270035200146,
2.16348775608497));
#142112=CARTESIAN_POINT('Ctrl Pts',(-7.40702668670085,1.587508025,1.18056542134086));
#142113=CARTESIAN_POINT('Ctrl Pts',(-7.34299360589532,1.52246862,1.58231761286301));
#142114=CARTESIAN_POINT('Ctrl Pts',(-7.23588247160926,1.457192641,1.97478705544074));
#142115=CARTESIAN_POINT('Ctrl Pts',(-7.2321967806587,1.45494649650072,1.988291917307));
#142116=CARTESIAN_POINT('Ctrl Pts',(-7.22851108970826,1.45270035200146,
2.00179677917319));
#142117=CARTESIAN_POINT('',(-7.08147779032799,1.4571926425566,2.05637369070155));
#142118=CARTESIAN_POINT('Ctrl Pts',(-6.927701267,1.457192641,2.137628395));
#142119=CARTESIAN_POINT('Ctrl Pts',(-6.810457805,1.522897175,2.517595128));
#142120=CARTESIAN_POINT('Ctrl Pts',(-6.65236221900001,1.587500328,2.882460217));
#142121=CARTESIAN_POINT('Ctrl Pts',(-7.090210694,1.457192641,2.445181447));
#142122=CARTESIAN_POINT('Ctrl Pts',(-6.956098733,1.522897175,2.834061408));
#142123=CARTESIAN_POINT('Ctrl Pts',(-6.78026102800001,1.587500328,3.20594142));
#142124=CARTESIAN_POINT('',(-7.09021068713113,1.45719263974395,2.44518146316404));
#142125=CARTESIAN_POINT('',(-6.88446147870823,1.54766053440234,2.97559889400155));
#142126=CARTESIAN_POINT('Origin',(0.182810596389243,1.33935993317304,-0.0430996776829071));
#142127=CARTESIAN_POINT('Ctrl Pts',(-6.65423598875174,1.58673401519076,
2.8781319295331));
#142128=CARTESIAN_POINT('Ctrl Pts',(-6.69257316710717,1.57991285848942,
2.89431032002908));
#142129=CARTESIAN_POINT('Ctrl Pts',(-6.73094648358784,1.57325083489832,
2.9105317901649));
#142130=CARTESIAN_POINT('Ctrl Pts',(-6.8076755759705,1.56023620896865,2.94301715641383));
#142131=CARTESIAN_POINT('Ctrl Pts',(-6.84607324461083,1.55387651075103,
2.95929879432475));
#142132=CARTESIAN_POINT('Ctrl Pts',(-6.884461480162,1.54766054352115,2.9755988940552));
#142133=CARTESIAN_POINT('',(-7.00895597346562,1.45719263730543,2.29140494251679));
#142134=CARTESIAN_POINT('Origin',(9.87925019568792E-13,1.54874775199989,
-3.72531866466019E-13));
#142135=CARTESIAN_POINT('',(-6.88550115471298,1.36645690001127,2.97319253421908));
#142136=CARTESIAN_POINT('Origin',(0.182911044278466,1.48213728633115,-0.0588316746106976));
#142137=CARTESIAN_POINT('',(-6.64150597624838,1.45719264185525,3.48430759351434));
#142138=CARTESIAN_POINT('Origin',(0.178026527221111,1.3392919067952,-0.0721096143840466));
#142139=CARTESIAN_POINT('Origin',(0.172713603740644,1.4821430259791,-0.0860888809879978));
#142140=CARTESIAN_POINT('Ctrl Pts',(-6.656092333,1.587508025,2.873836261));
#142141=CARTESIAN_POINT('Ctrl Pts',(-6.500217369,1.52246862,3.234858274));
#142142=CARTESIAN_POINT('Ctrl Pts',(-6.306208544,1.457192641,3.576902822));
#142143=CARTESIAN_POINT('Ctrl Pts',(-6.29953270679689,1.45494649673786,
3.58867256349837));
#142144=CARTESIAN_POINT('Ctrl Pts',(-6.29285686959388,1.45270035247575,
3.6004423049968));
#142145=CARTESIAN_POINT('Ctrl Pts',(-6.98006785141597,1.587508025,2.74525624586515));
#142146=CARTESIAN_POINT('Ctrl Pts',(-6.8311669814129,1.52246862,3.12385047355734));
#142147=CARTESIAN_POINT('Ctrl Pts',(-6.64219071806767,1.457192641,3.48411847163471));
#142148=CARTESIAN_POINT('Ctrl Pts',(-6.63568805114341,1.45494649673787,
3.49651528144297));
#142149=CARTESIAN_POINT('Ctrl Pts',(-6.62918538421904,1.45270035247575,
3.50891209125129));
#142150=CARTESIAN_POINT('',(-6.47385721741239,1.4571926425566,3.53060521441202));
#142151=CARTESIAN_POINT('Ctrl Pts',(-6.306208544,1.457192641,3.576902822));
#142152=CARTESIAN_POINT('Ctrl Pts',(-6.110024554,1.522897175,3.922782265));
#142153=CARTESIAN_POINT('Ctrl Pts',(-5.877189946,1.587500328,4.245131134));
#142154=CARTESIAN_POINT('Ctrl Pts',(-6.398803776,1.457192641,3.912200178));
#142155=CARTESIAN_POINT('Ctrl Pts',(-6.184229582,1.522897175,4.263158233));
#142156=CARTESIAN_POINT('Ctrl Pts',(-5.932559655,1.587500328,4.58854398900001));
#142157=CARTESIAN_POINT('',(-6.39880376581881,1.45719263974394,3.91220019230033));
#142158=CARTESIAN_POINT('',(-6.08384079107012,1.54766053443313,4.38598675995203));
#142159=CARTESIAN_POINT('Origin',(0.169271559227505,1.3393598742129,-0.0813909837261839));
#142160=CARTESIAN_POINT('Ctrl Pts',(-5.87995036175847,1.5867340152341,4.24130684477094));
#142161=CARTESIAN_POINT('Ctrl Pts',(-5.91391334078849,1.57991286287284,
4.26534833798605));
#142162=CARTESIAN_POINT('Ctrl Pts',(-5.9479023493887,1.57325084375826,4.28943967034669));
#142163=CARTESIAN_POINT('Ctrl Pts',(-6.01585420760897,1.56023620959703,
4.33766006384379));
#142164=CARTESIAN_POINT('Ctrl Pts',(-6.04985408564389,1.55387651199764,
4.36181540730131));
#142165=CARTESIAN_POINT('Ctrl Pts',(-6.08384079247201,1.54766054356863,
4.38598676033019));
#142166=CARTESIAN_POINT('',(-6.3525061485046,1.45719263730543,3.74455151950157));
#142167=CARTESIAN_POINT('Origin',(9.04224611852911E-13,1.54874775199961,
-6.71771666072019E-13));
#142168=CARTESIAN_POINT('',(-6.08537345586261,1.3664568999914,4.38386015927589));
#142169=CARTESIAN_POINT('Origin',(0.1659877218699,1.48213730823444,-0.0967767643559736));
#142170=CARTESIAN_POINT('',(-5.73720811971245,1.45719264185525,4.83057388182145));
#142171=CARTESIAN_POINT('Origin',(0.158363050588438,1.33929187171589,-0.108694257324458));
#142172=CARTESIAN_POINT('Origin',(0.150168911388342,1.48214300824914,-0.121204356352433));
#142173=CARTESIAN_POINT('Ctrl Pts',(-5.882686747,1.587508025,4.237510666));
#142174=CARTESIAN_POINT('Ctrl Pts',(-5.652846992,1.52246862,4.556583674));
#142175=CARTESIAN_POINT('Ctrl Pts',(-5.389844518,1.457192641,4.848925249));
#142176=CARTESIAN_POINT('Ctrl Pts',(-5.38079461137339,1.45494649667319,
4.85898471314341));
#142177=CARTESIAN_POINT('Ctrl Pts',(-5.3717447047468,1.4527003523464,4.86904417728667));
#142178=CARTESIAN_POINT('Ctrl Pts',(-6.22672880019407,1.587508025,4.18158193886891));
#142179=CARTESIAN_POINT('Ctrl Pts',(-5.99992258232298,1.52246862,4.51931555899604));
#142180=CARTESIAN_POINT('Ctrl Pts',(-5.73791750828063,1.457192641,4.83053638075679));
#142181=CARTESIAN_POINT('Ctrl Pts',(-5.72890192215432,1.45494649667319,
4.84124547917079));
#142182=CARTESIAN_POINT('Ctrl Pts',(-5.71988633602798,1.4527003523464,4.85195457758482));
#142183=CARTESIAN_POINT('',(-5.56352627571132,1.4571926425566,4.83974956272915));
#142184=CARTESIAN_POINT('Ctrl Pts',(-5.389844518,1.457192641,4.848925249));
#142185=CARTESIAN_POINT('Ctrl Pts',(-5.12389334400001,1.522897175,5.144544464));
#142186=CARTESIAN_POINT('Ctrl Pts',(-4.827206802,1.587500328,5.409304437));
#142187=CARTESIAN_POINT('Ctrl Pts',(-5.408195905,1.457192641,5.19628877700001));
#142188=CARTESIAN_POINT('Ctrl Pts',(-5.123192728,1.522897175,5.492914519));
#142189=CARTESIAN_POINT('Ctrl Pts',(-4.807458386,1.587500328,5.756591341));
#142190=CARTESIAN_POINT('',(-5.40819589198951,1.45719263974395,5.19628878876201));
#142191=CARTESIAN_POINT('',(-4.99874646949496,1.54766053441164,5.59129076007773));
#142192=CARTESIAN_POINT('Origin',(0.147817494022358,1.33935992725899,-0.1158765739251));
#142193=CARTESIAN_POINT('Ctrl Pts',(-4.83072478992621,1.58673401522937,
5.406162965312));
#142194=CARTESIAN_POINT('Ctrl Pts',(-4.85872552726679,1.57991286184182,
5.43694342298225));
#142195=CARTESIAN_POINT('Ctrl Pts',(-4.88674097219751,1.57325084166877,
5.46777815078991));
#142196=CARTESIAN_POINT('Ctrl Pts',(-4.9427381876837,1.56023620910422,5.52947881162374));
#142197=CARTESIAN_POINT('Ctrl Pts',(-4.97075048493763,1.55387651101871,
5.56037838786652));
#142198=CARTESIAN_POINT('Ctrl Pts',(-4.99874647078971,1.54766054353552,
5.5912907607398));
#142199=CARTESIAN_POINT('',(-5.3990201960811,1.45719263730543,5.02260702957445));
#142200=CARTESIAN_POINT('Origin',(3.33934269125535E-13,1.5487477520005,
-3.63424568217141E-13));
#142201=CARTESIAN_POINT('',(-5.00070045811103,1.36645689998942,5.58954335527285));
#142202=CARTESIAN_POINT('Origin',(0.141302887539335,1.48213731600747,-0.130196646736684));
#142203=CARTESIAN_POINT('',(-4.56464478872102,1.45719264185524,5.95096790420931));
#142204=CARTESIAN_POINT('Origin',(0.131294734058009,1.33929188265673,-0.140196623232732));
#142205=CARTESIAN_POINT('Origin',(0.120602720415548,1.48214303576771,-0.150652559824696));
#142206=CARTESIAN_POINT('Ctrl Pts',(-4.834213266,1.587508025,5.403043781));
#142207=CARTESIAN_POINT('Ctrl Pts',(-4.541155773,1.52246862,5.665248286));
#142208=CARTESIAN_POINT('Ctrl Pts',(-4.221457354,1.457192641,5.89421732));
#142209=CARTESIAN_POINT('Ctrl Pts',(-4.21045654185964,1.4549464966978,5.90209613697032));
#142210=CARTESIAN_POINT('Ctrl Pts',(-4.19945572971929,1.45270035239562,
5.90997495394052));
#142211=CARTESIAN_POINT('Ctrl Pts',(-5.18223483045369,1.587508025,5.4223815082615));
#142212=CARTESIAN_POINT('Ctrl Pts',(-4.88812847159532,1.52246862,5.70346247133777));
#142213=CARTESIAN_POINT('Ctrl Pts',(-4.56534565379732,1.457192641,5.95108377746541));
#142214=CARTESIAN_POINT('Ctrl Pts',(-4.55423870759519,1.4549464966978,5.95960441850951));
#142215=CARTESIAN_POINT('Ctrl Pts',(-4.54313176139316,1.45270035239562,
5.96812505955364));
#142216=CARTESIAN_POINT('',(-4.39305102980428,1.4571926425566,5.92259260020826));
#142217=CARTESIAN_POINT('Ctrl Pts',(-4.221457354,1.457192641,5.89421732));
#142218=CARTESIAN_POINT('Ctrl Pts',(-3.898174577,1.522897175,6.125753481));
#142219=CARTESIAN_POINT('Ctrl Pts',(-3.551508834,1.587500328,6.320544676));
#142220=CARTESIAN_POINT('Ctrl Pts',(-4.164706805,1.457192641,6.237404687));
#142221=CARTESIAN_POINT('Ctrl Pts',(-3.822601077,1.522897175,6.465828226));
#142222=CARTESIAN_POINT('Ctrl Pts',(-3.457565706,1.587500328,6.65546688));
#142223=CARTESIAN_POINT('',(-4.16470678976563,1.45719263974395,6.23740469568957));
#142224=CARTESIAN_POINT('',(-3.67991631912743,1.54766053440482,6.53515221826147));
#142225=CARTESIAN_POINT('Origin',(0.119451572345765,1.33935994579391,-0.144943851805711));
#142226=CARTESIAN_POINT('Ctrl Pts',(-3.55561989709399,1.58673401518731,
6.31823291346998));
#142227=CARTESIAN_POINT('Ctrl Pts',(-3.57634910582028,1.57991286122881,
6.35431307522638));
#142228=CARTESIAN_POINT('Ctrl Pts',(-3.59708101208162,1.57325084046458,
6.39044940037043));
#142229=CARTESIAN_POINT('Ctrl Pts',(-3.63850521952105,1.56023620976,6.46274527001499));
#142230=CARTESIAN_POINT('Ctrl Pts',(-3.65922010693531,1.55387651235248,
6.49894424315467));
#142231=CARTESIAN_POINT('Ctrl Pts',(-3.67991632024148,1.54766054352706,
6.53515221919074));
#142232=CARTESIAN_POINT('',(-4.19308206087856,1.45719263730543,6.06581101637234));
#142233=CARTESIAN_POINT('Origin',(-2.08166817117217E-13,1.54874775199961,
4.32813507256213E-13));
#142234=CARTESIAN_POINT('',(-3.68220026482123,1.36645690002958,6.53386571702019));
#142235=CARTESIAN_POINT('Origin',(0.110010924704643,1.48213728422803,-0.157528746971618));
#142236=CARTESIAN_POINT('',(-3.17864374056536,1.45719264185526,6.79310128094016));
#142237=CARTESIAN_POINT('Origin',(0.0980868957313646,1.33929187957912,-0.165143190374958));
#142238=CARTESIAN_POINT('Origin',(0.0853972507623617,1.48214300224995,-0.173056429922132));
#142239=CARTESIAN_POINT('Ctrl Pts',(-3.559697347,1.587508025,6.315936573));
#142240=CARTESIAN_POINT('Ctrl Pts',(-3.217125156,1.52246862,6.509012185));
#142241=CARTESIAN_POINT('Ctrl Pts',(-2.855679535,1.457192641,6.66390234));
#142242=CARTESIAN_POINT('Ctrl Pts',(-2.84324220287946,1.45494649667524,
6.66923210522061));
#142243=CARTESIAN_POINT('Ctrl Pts',(-2.83080487075887,1.4527003523505,6.67456187044107));
#142244=CARTESIAN_POINT('Ctrl Pts',(-3.89542532096169,1.587508025,6.40963654464227));
#142245=CARTESIAN_POINT('Ctrl Pts',(-3.54777090608225,1.52246862,6.62092181761493));
#142246=CARTESIAN_POINT('Ctrl Pts',(-3.17930331049195,1.457192641,6.79336511042453));
#142247=CARTESIAN_POINT('Ctrl Pts',(-3.16662435245302,1.45494649667524,
6.79929887854907));
#142248=CARTESIAN_POINT('Ctrl Pts',(-3.153945394414,1.4527003523505,6.80523264667356));
#142249=CARTESIAN_POINT('',(-3.01716159975711,1.4571926425566,6.72850178992045));
#142250=CARTESIAN_POINT('Ctrl Pts',(-2.855679535,1.457192641,6.66390234));
#142251=CARTESIAN_POINT('Ctrl Pts',(-2.4901815,1.522897175,6.820529074));
#142252=CARTESIAN_POINT('Ctrl Pts',(-2.109746259,1.587500328,6.936243271));
#142253=CARTESIAN_POINT('Ctrl Pts',(-2.726480643,1.457192641,6.986866487));
#142254=CARTESIAN_POINT('Ctrl Pts',(-2.343268848,1.522897175,7.136406991));
#142255=CARTESIAN_POINT('Ctrl Pts',(-1.946001096,1.587500328,7.243140185));
#142256=CARTESIAN_POINT('',(-2.72648062626192,1.45719263974396,6.98686649220436));
#142257=CARTESIAN_POINT('',(-2.18901737115193,1.54766053442488,7.1734372219873));
#142258=CARTESIAN_POINT('Origin',(0.0855002844435065,1.33935992351952,-0.167233897191608));
#142259=CARTESIAN_POINT('Ctrl Pts',(-2.11425816793634,1.58673401521377,
6.93486931377602));
#142260=CARTESIAN_POINT('Ctrl Pts',(-2.12674657914192,1.57991285703008,
6.974562133025));
#142261=CARTESIAN_POINT('Ctrl Pts',(-2.13922555206339,1.57325083195643,
7.01431038546371));
#142262=CARTESIAN_POINT('Ctrl Pts',(-2.16413971704552,1.56023624975565,
7.09382070150504));
#142263=CARTESIAN_POINT('Ctrl Pts',(-2.17658850712719,1.55387659347072,
7.13362617601876));
#142264=CARTESIAN_POINT('Ctrl Pts',(-2.18901737205927,1.54766054355077,
7.17343722312894));
#142265=CARTESIAN_POINT('',(-2.79108006804675,1.45719263730543,6.82538442206834));
#142266=CARTESIAN_POINT('Origin',(1.88868018446975E-13,1.54874775200011,
-8.56086035394554E-13));
#142267=CARTESIAN_POINT('',(-2.19152447924759,1.36645689997044,7.17267177913987));
#142268=CARTESIAN_POINT('Origin',(0.0735749316633463,1.48213731777391,-0.177494984800044));
#142269=CARTESIAN_POINT('',(-1.64401284267834,1.45719264185524,7.31759679238916));
#142270=CARTESIAN_POINT('Origin',(0.0602927793857641,1.33929186759675,-0.182368014253653));
#142271=CARTESIAN_POINT('Origin',(0.046198706450094,1.48214301892206,-0.187368375610238));
#142272=CARTESIAN_POINT('Ctrl Pts',(-2.118733935,1.587508025,6.933503192));
#142273=CARTESIAN_POINT('Ctrl Pts',(-1.742665343,1.52246862,7.048421908));
#142274=CARTESIAN_POINT('Ctrl Pts',(-1.356373314,1.457192641,7.121990693));
#142275=CARTESIAN_POINT('Ctrl Pts',(-1.34308101774021,1.45494649666779,
7.12452219251923));
#142276=CARTESIAN_POINT('Ctrl Pts',(-1.32978872148043,1.4527003523356,7.12705369203845));
#142277=CARTESIAN_POINT('Ctrl Pts',(-2.42647005135815,1.587508025,7.09718409979056));
#142278=CARTESIAN_POINT('Ctrl Pts',(-2.04152351582573,1.52246862,7.22879421816179));
#142279=CARTESIAN_POINT('Ctrl Pts',(-1.64460027668501,1.457192641,7.31799624172302));
#142280=CARTESIAN_POINT('Ctrl Pts',(-1.63094216082715,1.45494649666779,
7.32106568047695));
#142281=CARTESIAN_POINT('Ctrl Pts',(-1.61728404496923,1.45270035233559,
7.32413511923084));
#142282=CARTESIAN_POINT('',(-1.50019304561873,1.4571926425566,7.21979371444933));
#142283=CARTESIAN_POINT('Ctrl Pts',(-1.356373314,1.457192641,7.121990693));
#142284=CARTESIAN_POINT('Ctrl Pts',(-0.965750302,1.522897175,7.196384307));
#142285=CARTESIAN_POINT('Ctrl Pts',(-0.569334295,1.587500328,7.22761084000001));
#142286=CARTESIAN_POINT('Ctrl Pts',(-1.160767276,1.457192641,7.409630175));
#142287=CARTESIAN_POINT('Ctrl Pts',(-0.754367972,1.522897175,7.473295298));
#142288=CARTESIAN_POINT('Ctrl Pts',(-0.343443638,1.587500328,7.49213230400001));
#142289=CARTESIAN_POINT('',(-1.16076725851918,1.45719263974395,7.4096301764929));
#142290=CARTESIAN_POINT('',(-0.59576240422708,1.54766053440468,7.47630027399342));
#142291=CARTESIAN_POINT('Origin',(0.0475509340222015,1.33935995780179,-0.181703625814522));
#142292=CARTESIAN_POINT('Ctrl Pts',(-0.574036078207936,1.58673401524647,
7.22723893192767));
#142293=CARTESIAN_POINT('Ctrl Pts',(-0.577699733054604,1.57991285914198,
7.26868838164303));
#142294=CARTESIAN_POINT('Ctrl Pts',(-0.581342253842358,1.5732508361904,
7.31018993810145));
#142295=CARTESIAN_POINT('Ctrl Pts',(-0.5885815969205,1.56023620877839,7.39319744444684));
#142296=CARTESIAN_POINT('Ctrl Pts',(-0.592182365966404,1.55387651034652,
7.434748705256));
#142297=CARTESIAN_POINT('Ctrl Pts',(-0.595762404863382,1.54766054352378,
7.47630027530278));
#142298=CARTESIAN_POINT('',(-1.25857027269469,1.45719263730543,7.26581043786369));
#142299=CARTESIAN_POINT('Origin',(6.04950930929021E-14,1.54874775200061,
7.50267903359969E-14));
#142300=CARTESIAN_POINT('',(-0.598375444936869,1.36645689998177,7.47609168110421));
#142301=CARTESIAN_POINT('Origin',(0.0336986056209087,1.48213727193679,-0.189161605056248));
#142302=CARTESIAN_POINT('',(-0.0325097326105792,1.45719264185525,7.49992961001097));
#142303=CARTESIAN_POINT('Origin',(0.0196794318992366,1.33929185017855,-0.191065540471456));
#142304=CARTESIAN_POINT('Origin',(0.00483994282569893,1.48214301066781,
-0.192919282835899));
#142305=CARTESIAN_POINT('Ctrl Pts',(-0.57870088,1.587508025,7.226866907));
#142306=CARTESIAN_POINT('Ctrl Pts',(-0.186720435,1.52246862,7.258255257));
#142307=CARTESIAN_POINT('Ctrl Pts',(0.206355414,1.457192641,7.247062677));
#142308=CARTESIAN_POINT('Ctrl Pts',(0.21988114116028,1.45494649668887,7.24667754068678));
#142309=CARTESIAN_POINT('Ctrl Pts',(0.23340686832056,1.45270035237775,7.24629240437358));
#142310=CARTESIAN_POINT('Ctrl Pts',(-0.844055740452744,1.587508025,7.45287521505935));
#142311=CARTESIAN_POINT('Ctrl Pts',(-0.439816755395308,1.52246862,7.49865623502241));
#142312=CARTESIAN_POINT('Ctrl Pts',(-0.0329975629266414,1.457192641,7.50044600138326));
#142313=CARTESIAN_POINT('Ctrl Pts',(-0.0189989277652717,1.45494649668887,
7.50050758718543));
#142314=CARTESIAN_POINT('Ctrl Pts',(-0.00500029260390189,1.45270035237775,
7.5005691729876));
#142315=CARTESIAN_POINT('',(0.0869228665809933,1.4571926425566,7.37349610888705));
#142316=CARTESIAN_POINT('Ctrl Pts',(-1.642244642,4.301266351,7.317993751));
#142317=CARTESIAN_POINT('Ctrl Pts',(-1.243612454,4.365380951,7.407451544));
#142318=CARTESIAN_POINT('Ctrl Pts',(-0.837621771000001,4.430609079,7.453079214));
#142319=CARTESIAN_POINT('Ctrl Pts',(-0.833550507349874,4.43126318491329,
7.45353676704762));
#142320=CARTESIAN_POINT('Ctrl Pts',(-0.829479243699748,4.43191729082659,
7.45399432009524));
#142321=CARTESIAN_POINT('Ctrl Pts',(-1.354652431,4.301266351,7.122318217));
#142322=CARTESIAN_POINT('Ctrl Pts',(-0.966679253,4.365380951,7.196110035));
#142323=CARTESIAN_POINT('Ctrl Pts',(-0.572986203,4.430609079,7.22732224400001));
#142324=CARTESIAN_POINT('Ctrl Pts',(-0.569038259682857,4.43126318491329,
7.22763523919241));
#142325=CARTESIAN_POINT('Ctrl Pts',(-0.565090316365713,4.43191729082659,
7.22794823438482));
#142326=CARTESIAN_POINT('',(-0.837621778443153,4.43060908007271,7.45307921003498));
#142327=CARTESIAN_POINT('',(-0.705304006274358,4.43060908208283,7.34020072714797));
#142328=CARTESIAN_POINT('',(-1.39540249029647,4.34096089506028,7.36904687802678));
#142329=CARTESIAN_POINT('Origin',(0.00129585974664434,4.55349066438059,
-0.187514887673611));
#142330=CARTESIAN_POINT('Ctrl Pts',(-1.35005064267087,4.30202682666956,
7.12319192941445));
#142331=CARTESIAN_POINT('Ctrl Pts',(-1.35748387767582,4.30883434438056,
7.16413036593558));
#142332=CARTESIAN_POINT('Ctrl Pts',(-1.36498789722174,4.31547777947418,
7.20511000407318));
#142333=CARTESIAN_POINT('Ctrl Pts',(-1.38010626519058,4.32844538542126,
7.28704728890771));
#142334=CARTESIAN_POINT('Ctrl Pts',(-1.38772947470995,4.33477714733287,
7.32805291775489));
#142335=CARTESIAN_POINT('Ctrl Pts',(-1.39540248946664,4.3409608950497,7.3690468781837));
#142336=CARTESIAN_POINT('Ctrl Pts',(-1.95752567888767,4.43188407004788,
7.24003864400306));
#142337=CARTESIAN_POINT('Ctrl Pts',(-1.95359317694383,4.43124657452394,
7.24109731250152));
#142338=CARTESIAN_POINT('Ctrl Pts',(-1.949660675,4.430609079,7.242155981));
#142339=CARTESIAN_POINT('Ctrl Pts',(-1.943374636,4.429590053,7.243848245));
#142340=CARTESIAN_POINT('Ctrl Pts',(-1.93708567,4.428571429,7.245529595));
#142341=CARTESIAN_POINT('Ctrl Pts',(-1.547673393,4.365498301,7.349638609));
#142342=CARTESIAN_POINT('Ctrl Pts',(-1.149345823,4.301245526,7.411410404));
#142343=CARTESIAN_POINT('Ctrl Pts',(-2.12078237088003,4.43188407004788,
6.93288137335172));
#142344=CARTESIAN_POINT('Ctrl Pts',(-2.11701655944001,4.43124657452394,
6.93402887167586));
#142345=CARTESIAN_POINT('Ctrl Pts',(-2.113250748,4.430609079,6.93517637));
#142346=CARTESIAN_POINT('Ctrl Pts',(-2.107231161,4.429590053,6.937010627));
#142347=CARTESIAN_POINT('Ctrl Pts',(-2.1012084,4.428571429,6.938834431));
#142348=CARTESIAN_POINT('Ctrl Pts',(-1.728279509,4.365498301,7.05176425));
#142349=CARTESIAN_POINT('Ctrl Pts',(-1.345394953,4.301245526,7.124072741));
#142350=CARTESIAN_POINT('',(-1.94966066672091,4.43060908088842,7.2421559806126));
#142351=CARTESIAN_POINT('Origin',(0.00564046052463463,4.16161686280091,
-0.183011846437567));
#142352=CARTESIAN_POINT('',(-2.03145569497605,4.43060908179129,7.0886661802354));
#142353=CARTESIAN_POINT('Origin',(3.81747584932146E-13,4.52171036999889,
-1.76074432811646E-12));
#142354=CARTESIAN_POINT('',(-1.40181135465044,4.52063234085899,7.36783040844133));
#142355=CARTESIAN_POINT('Origin',(0.0613272168278398,4.69624338552546,-0.17289401675978));
#142356=CARTESIAN_POINT('Origin',(0.0306516469109547,4.5535636689927,-0.189451099243872));
#142357=CARTESIAN_POINT('Ctrl Pts',(-3.177002213,4.301266351,6.79386907));
#142358=CARTESIAN_POINT('Ctrl Pts',(-2.806920605,4.365380951,6.966929527));
#142359=CARTESIAN_POINT('Ctrl Pts',(-2.420230359,4.430609079,7.098766443));
#142360=CARTESIAN_POINT('Ctrl Pts',(-2.41635263961303,4.43126318491329,
7.10008850004794));
#142361=CARTESIAN_POINT('Ctrl Pts',(-2.41247492022606,4.43191729082659,
7.10141055709587));
#142362=CARTESIAN_POINT('Ctrl Pts',(-2.854069293,4.301266351,6.66459214600001));
#142363=CARTESIAN_POINT('Ctrl Pts',(-2.491029771,4.365380951,6.820061517));
#142364=CARTESIAN_POINT('Ctrl Pts',(-2.113250748,4.430609079,6.93517637));
#142365=CARTESIAN_POINT('Ctrl Pts',(-2.10946239011761,4.43126318491329,
6.93633073864991));
#142366=CARTESIAN_POINT('Ctrl Pts',(-2.10567403223522,4.43191729082659,
6.93748510729981));
#142367=CARTESIAN_POINT('',(-2.42023036541207,4.43060908007271,7.09876643752801));
#142368=CARTESIAN_POINT('',(-2.26674057192561,4.43060908208283,7.01697140054785));
#142369=CARTESIAN_POINT('',(-2.94690600724563,4.34096089499786,6.89679236925532));
#142370=CARTESIAN_POINT('Origin',(0.0415756784798843,4.55349067515581,-0.182852214336201));
#142371=CARTESIAN_POINT('Ctrl Pts',(-2.84976291363964,4.30202682662798,
6.66643467952211));
#142372=CARTESIAN_POINT('Ctrl Pts',(-2.86582299171485,4.30883437576907,
6.70481824956525));
#142373=CARTESIAN_POINT('Ctrl Pts',(-2.88196106599946,4.31547784262711,
6.74322686106965));
#142374=CARTESIAN_POINT('Ctrl Pts',(-2.91433991142714,4.32844538539627,
6.81999812150008));
#142375=CARTESIAN_POINT('Ctrl Pts',(-2.93059989259798,4.33477714729532,
6.85840629676247));
#142376=CARTESIAN_POINT('Ctrl Pts',(-2.94690600618894,4.34096089499144,
6.896792369698));
#142377=CARTESIAN_POINT('Ctrl Pts',(-3.46815410914429,4.43188407004788,
6.64996040604056));
#142378=CARTESIAN_POINT('Ctrl Pts',(-3.46454113007215,4.43124657452394,
6.65183969552028));
#142379=CARTESIAN_POINT('Ctrl Pts',(-3.460928151,4.430609079,6.65371898500001));
#142380=CARTESIAN_POINT('Ctrl Pts',(-3.455152864,4.429590053,6.656722998));
#142381=CARTESIAN_POINT('Ctrl Pts',(-3.44937237,4.428571429,6.65971698));
#142382=CARTESIAN_POINT('Ctrl Pts',(-3.091444697,4.365498301,6.845104111));
#142383=CARTESIAN_POINT('Ctrl Pts',(-2.715708914,4.301245526,6.99106037));
#142384=CARTESIAN_POINT('Ctrl Pts',(-3.56156421782437,4.43188407004788,
6.31488893800863));
#142385=CARTESIAN_POINT('Ctrl Pts',(-3.55813312741219,4.43124657452394,
6.31681914700431));
#142386=CARTESIAN_POINT('Ctrl Pts',(-3.554702037,4.430609079,6.318749356));
#142387=CARTESIAN_POINT('Ctrl Pts',(-3.549217496,4.429590053,6.321834763));
#142388=CARTESIAN_POINT('Ctrl Pts',(-3.543727607,4.428571429,6.324910643));
#142389=CARTESIAN_POINT('Ctrl Pts',(-3.20379416,4.365498301,6.515368914));
#142390=CARTESIAN_POINT('Ctrl Pts',(-2.84540542,4.301245526,6.668295734));
#142391=CARTESIAN_POINT('',(-3.46092814283634,4.43060908088845,6.6537189864983));
#142392=CARTESIAN_POINT('Origin',(0.0448507385774199,4.16161693133534,-0.17752059842843));
#142393=CARTESIAN_POINT('',(-3.50781507888034,4.43060908179129,6.48623417867685));
#142394=CARTESIAN_POINT('Origin',(1.97324795392362E-13,4.52171037000089,
-4.11129463806503E-13));
#142395=CARTESIAN_POINT('',(-2.95290353040656,4.52063234086375,6.89422662374213));
#142396=CARTESIAN_POINT('Origin',(0.0970604625450294,4.69624336322254,-0.155668159305726));
#142397=CARTESIAN_POINT('Origin',(0.0706614301360553,4.55356366994914,-0.178432672195805));
#142398=CARTESIAN_POINT('Ctrl Pts',(-4.563206691,4.301266351,5.95207062200001));
#142399=CARTESIAN_POINT('Ctrl Pts',(-4.238980268,4.365380951,6.200641628));
#142400=CARTESIAN_POINT('Ctrl Pts',(-3.889671666,4.430609079,6.412523242));
#142401=CARTESIAN_POINT('Ctrl Pts',(-3.8861688087337,4.43126318491329,6.4146479851267));
#142402=CARTESIAN_POINT('Ctrl Pts',(-3.88266595146739,4.43191729082659,
6.4167727282534));
#142403=CARTESIAN_POINT('Ctrl Pts',(-4.220033046,4.301266351,5.895237153));
#142404=CARTESIAN_POINT('Ctrl Pts',(-3.898902506,4.365380951,6.125114502));
#142405=CARTESIAN_POINT('Ctrl Pts',(-3.554702037,4.430609079,6.318749356));
#142406=CARTESIAN_POINT('Ctrl Pts',(-3.55125040395404,4.43126318491329,
6.32069112110816));
#142407=CARTESIAN_POINT('Ctrl Pts',(-3.54779877090807,4.43191729082659,
6.32263288621632));
#142408=CARTESIAN_POINT('',(-3.88967167115354,4.43060908007263,6.41252323525665));
#142409=CARTESIAN_POINT('',(-3.72218686821525,4.43060908208281,6.36563628922607));
#142410=CARTESIAN_POINT('',(-4.36061547382111,4.34096089500174,6.10205151464986));
#142411=CARTESIAN_POINT('Origin',(0.0799114620200347,4.55349070799973,-0.169639663486321));
#142412=CARTESIAN_POINT('Ctrl Pts',(-4.21622343834095,4.30202682667494,
5.89796235369777));
#142413=CARTESIAN_POINT('Ctrl Pts',(-4.24015925232632,4.30883434132914,
5.93199592261722));
#142414=CARTESIAN_POINT('Ctrl Pts',(-4.26417660738963,4.31547777332414,
5.96603716179003));
#142415=CARTESIAN_POINT('Ctrl Pts',(-4.31230226225936,4.32844538539751,
6.03405342154499));
#142416=CARTESIAN_POINT('Ctrl Pts',(-4.33643871635989,4.33477714726343,
6.06806821949402));
#142417=CARTESIAN_POINT('Ctrl Pts',(-4.36061547322445,4.34096089498421,
6.10205151507753));
#142418=CARTESIAN_POINT('Ctrl Pts',(-4.81661550888204,4.43188407004788,
5.74893741316841));
#142419=CARTESIAN_POINT('Ctrl Pts',(-4.81349099094102,4.43124657452394,
5.7515494490842));
#142420=CARTESIAN_POINT('Ctrl Pts',(-4.81036647300001,4.430609079,5.75416148500001));
#142421=CARTESIAN_POINT('Ctrl Pts',(-4.805371983,4.429590053,5.758336781));
#142422=CARTESIAN_POINT('Ctrl Pts',(-4.800370252,4.428571429,5.762503401));
#142423=CARTESIAN_POINT('Ctrl Pts',(-4.490663482,4.365498301,6.020500154));
#142424=CARTESIAN_POINT('Ctrl Pts',(-4.155088474,4.301245526,6.243816123));
#142425=CARTESIAN_POINT('Ctrl Pts',(-4.8358112798721,4.43188407004788,5.40161931776974));
#142426=CARTESIAN_POINT('Ctrl Pts',(-4.83287534443605,4.43124657452394,
5.40424198188487));
#142427=CARTESIAN_POINT('Ctrl Pts',(-4.829939409,4.430609079,5.406864646));
#142428=CARTESIAN_POINT('Ctrl Pts',(-4.825246365,4.429590053,5.411056931));
#142429=CARTESIAN_POINT('Ctrl Pts',(-4.82054605,4.428571429,5.415241063));
#142430=CARTESIAN_POINT('Ctrl Pts',(-4.529502956,4.365498301,5.674322168));
#142431=CARTESIAN_POINT('Ctrl Pts',(-4.212367892,4.301245526,5.90071663));
#142432=CARTESIAN_POINT('',(-4.81036646532986,4.43060908088843,5.75416148814806));
#142433=CARTESIAN_POINT('Origin',(0.0819638448501125,4.16161699509913,-0.163728679574764));
#142434=CARTESIAN_POINT('',(-4.82015292799161,4.43060908179129,5.58051307673596));
#142435=CARTESIAN_POINT('Origin',(-4.33680868994202E-14,4.52171037,1.34441069388203E-13));
#142436=CARTESIAN_POINT('',(-4.3659212187363,4.52063234082487,6.09825646507154));
#142437=CARTESIAN_POINT('Origin',(0.128255209085647,4.69624332240152,-0.131163488074278));
#142438=CARTESIAN_POINT('Origin',(0.107367251794376,4.55356365553789,-0.159071021084871));
#142439=CARTESIAN_POINT('Ctrl Pts',(-5.73604069600001,4.301266351,4.831959968));
#142440=CARTESIAN_POINT('Ctrl Pts',(-5.47282992599999,4.365380951,5.144418618));
#142441=CARTESIAN_POINT('Ctrl Pts',(-5.17723624800001,4.430609079,5.426437582));
#142442=CARTESIAN_POINT('Ctrl Pts',(-5.17427204254692,4.43126318491329,
5.42926566058618));
#142443=CARTESIAN_POINT('Ctrl Pts',(-5.17130783709384,4.43191729082659,
5.43209373917236));
#142444=CARTESIAN_POINT('Ctrl Pts',(-5.388672745,4.301266351,4.850227423));
#142445=CARTESIAN_POINT('Ctrl Pts',(-5.124466893,4.365380951,5.143763941));
#142446=CARTESIAN_POINT('Ctrl Pts',(-4.829939409,4.430609079,5.40686464600001));
#142447=CARTESIAN_POINT('Ctrl Pts',(-4.82698589531168,4.43126318491329,
5.40950301279372));
#142448=CARTESIAN_POINT('Ctrl Pts',(-4.82403238162336,4.43191729082659,
5.41214137958745));
#142449=CARTESIAN_POINT('',(-5.17723625158181,4.43060908007265,5.42643757430715));
#142450=CARTESIAN_POINT('',(-5.00358784272338,4.43060908208283,5.41665110086127));
#142451=CARTESIAN_POINT('',(-5.57042740767327,4.34096089499433,5.02198551318363));
#142452=CARTESIAN_POINT('Origin',(0.114510668632672,4.55349064898209,-0.148494951778445));
#142453=CARTESIAN_POINT('Ctrl Pts',(-5.38553804049223,4.30202682659519,
4.85370786275825));
#142454=CARTESIAN_POINT('Ctrl Pts',(-5.41623061531528,4.30883437574001,
4.88180039567836));
#142455=CARTESIAN_POINT('Ctrl Pts',(-5.44700449218597,4.31547784259929,
4.90988290582544));
#142456=CARTESIAN_POINT('Ctrl Pts',(-5.50862617915739,4.32844539111283,
4.96596311513484));
#142457=CARTESIAN_POINT('Ctrl Pts',(-5.53951054287518,4.33477715879874,
4.99399406931061));
#142458=CARTESIAN_POINT('Ctrl Pts',(-5.57042740683775,4.34096089498869,
5.02198551401675));
#142459=CARTESIAN_POINT('Ctrl Pts',(-5.93985732264998,4.43188407004788,
4.57910049458699));
#142460=CARTESIAN_POINT('Ctrl Pts',(-5.93736736432499,4.43124657452394,
4.58232314179349));
#142461=CARTESIAN_POINT('Ctrl Pts',(-5.934877406,4.430609079,4.585545789));
#142462=CARTESIAN_POINT('Ctrl Pts',(-5.930897249,4.429590053,4.590697137));
#142463=CARTESIAN_POINT('Ctrl Pts',(-5.926908156,4.428571429,4.595841568));
#142464=CARTESIAN_POINT('Ctrl Pts',(-5.679903833,4.365498301,4.9143843));
#142465=CARTESIAN_POINT('Ctrl Pts',(-5.400180715,4.301245526,5.204617973));
#142466=CARTESIAN_POINT('Ctrl Pts',(-5.88394118241646,4.43188407004788,
4.23577597926324));
#142467=CARTESIAN_POINT('Ctrl Pts',(-5.88163768270823,4.43124657452394,
4.23896846663162));
#142468=CARTESIAN_POINT('Ctrl Pts',(-5.879334183,4.430609079,4.242160954));
#142469=CARTESIAN_POINT('Ctrl Pts',(-5.875652077,4.429590053,4.247264092));
#142470=CARTESIAN_POINT('Ctrl Pts',(-5.871961118,4.428571429,4.25236083));
#142471=CARTESIAN_POINT('Ctrl Pts',(-5.643417229,4.365498301,4.567950425));
#142472=CARTESIAN_POINT('Ctrl Pts',(-5.382364723,4.301245526,4.857226574));
#142473=CARTESIAN_POINT('',(-5.93487739907786,4.43060908088836,4.58554579351896));
#142474=CARTESIAN_POINT('Origin',(0.115244392964607,4.16161693384168,-0.142280995222945));
#142475=CARTESIAN_POINT('',(-5.90710578421114,4.43060908179129,4.41385338526969));
#142476=CARTESIAN_POINT('Origin',(1.12366713156398E-12,4.52171036999933,
-1.00397121172158E-12));
#142477=CARTESIAN_POINT('',(-5.57479328396169,4.52063234083233,5.01713861086988));
#142478=CARTESIAN_POINT('Origin',(0.153452966462989,4.69624336495175,-0.100525882028337));
#142479=CARTESIAN_POINT('Origin',(0.139052551697806,4.55356366360523,-0.132271185767189));
#142480=CARTESIAN_POINT('Ctrl Pts',(-6.640663814,4.301266351,3.485912235));
#142481=CARTESIAN_POINT('Ctrl Pts',(-6.450776138,4.365380951,3.847648312));
#142482=CARTESIAN_POINT('Ctrl Pts',(-6.222719017,4.430609079,4.186617732));
#142483=CARTESIAN_POINT('Ctrl Pts',(-6.22043206632414,4.43126318491329,
4.19001690822728));
#142484=CARTESIAN_POINT('Ctrl Pts',(-6.21814511564828,4.43191729082659,
4.19341608445456));
#142485=CARTESIAN_POINT('Ctrl Pts',(-6.305344095,4.301266351,3.578426449));
#142486=CARTESIAN_POINT('Ctrl Pts',(-6.110416904,4.365380951,3.921896695));
#142487=CARTESIAN_POINT('Ctrl Pts',(-5.879334183,4.430609079,4.242160954));
#142488=CARTESIAN_POINT('Ctrl Pts',(-5.87701689168871,4.43126318491329,
4.24537255537584));
#142489=CARTESIAN_POINT('Ctrl Pts',(-5.87469960037743,4.43191729082659,
4.24858415675168));
#142490=CARTESIAN_POINT('',(-6.2227190188456,4.43060908007265,4.18661772371591));
#142491=CARTESIAN_POINT('',(-6.05102661106641,4.43060908208283,4.21438932711084));
#142492=CARTESIAN_POINT('',(-6.51977234665285,4.34096089500476,3.7070970509502));
#142493=CARTESIAN_POINT('Origin',(0.143755514817397,4.55349071186133,-0.120406833930994));
#142494=CARTESIAN_POINT('Ctrl Pts',(-6.30303086914785,4.30202682657719,
3.58249938692523));
#142495=CARTESIAN_POINT('Ctrl Pts',(-6.33904493287761,4.30883437572862,
3.6033371356933));
#142496=CARTESIAN_POINT('Ctrl Pts',(-6.375136243243,4.31547784259418,3.62414761850538));
#142497=CARTESIAN_POINT('Ctrl Pts',(-6.44737283600404,4.32844539096959,
3.66566986209409));
#142498=CARTESIAN_POINT('Ctrl Pts',(-6.48356096590171,4.33477715846729,
3.68640624225615));
#142499=CARTESIAN_POINT('Ctrl Pts',(-6.51977234599395,4.34096089499908,
3.70709705188124));
#142500=CARTESIAN_POINT('Ctrl Pts',(-6.78535800869693,4.43188407004788,
3.19514992667573));
#142501=CARTESIAN_POINT('Ctrl Pts',(-6.78361903784846,4.43124657452394,
3.19883249733787));
#142502=CARTESIAN_POINT('Ctrl Pts',(-6.78188006700001,4.430609079,3.202515068));
#142503=CARTESIAN_POINT('Ctrl Pts',(-6.779100351,4.429590053,3.208401596));
#142504=CARTESIAN_POINT('Ctrl Pts',(-6.776310422,4.428571429,3.21428329));
#142505=CARTESIAN_POINT('Ctrl Pts',(-6.603558194,4.365498301,3.578477299));
#142506=CARTESIAN_POINT('Ctrl Pts',(-6.392766507,4.301245526,3.922057672));
#142507=CARTESIAN_POINT('Ctrl Pts',(-6.65694453501887,4.43188407004788,
2.87187246525371));
#142508=CARTESIAN_POINT('Ctrl Pts',(-6.65538118000943,4.43124657452394,
2.87548549812686));
#142509=CARTESIAN_POINT('Ctrl Pts',(-6.653817825,4.430609079,2.879098531));
#142510=CARTESIAN_POINT('Ctrl Pts',(-6.651318828,4.429590053,2.884873904));
#142511=CARTESIAN_POINT('Ctrl Pts',(-6.64880981,4.428571429,2.890644931));
#142512=CARTESIAN_POINT('Ctrl Pts',(-6.49345158400001,4.365498301,3.247986396));
#142513=CARTESIAN_POINT('Ctrl Pts',(-6.300688161,4.301245526,3.586618002));
#142514=CARTESIAN_POINT('',(-6.78188006127967,4.43060908088839,3.20251507398212));
#142515=CARTESIAN_POINT('Origin',(0.143136257140021,4.16161698237671,-0.114180401131374));
#142516=CARTESIAN_POINT('',(-6.71784893891177,4.43060908179129,3.04080681515956));
#142517=CARTESIAN_POINT('Origin',(8.00574884163296E-13,4.52171036999978,
-5.12393946716649E-13));
#142518=CARTESIAN_POINT('',(-6.52299421048894,4.52063234083094,3.7014249322747));
#142519=CARTESIAN_POINT('Origin',(0.171475441869195,4.69624338813449,-0.0651878064923755));
#142520=CARTESIAN_POINT('Origin',(0.164236088590776,4.55356368309189,-0.0992866306841322));
#142521=CARTESIAN_POINT('Ctrl Pts',(-7.234776872,4.301266351,1.976867121));
#142522=CARTESIAN_POINT('Ctrl Pts',(-7.127091228,4.365380951,2.370966246));
#142523=CARTESIAN_POINT('Ctrl Pts',(-6.977234361,4.430609079,2.751036289));
#142524=CARTESIAN_POINT('Ctrl Pts',(-6.97573160036808,4.43126318491329,
2.75484762116933));
#142525=CARTESIAN_POINT('Ctrl Pts',(-6.97422883973616,4.43191729082659,
2.75865895333867));
#142526=CARTESIAN_POINT('Ctrl Pts',(-6.927184563,4.301266351,2.139302231));
#142527=CARTESIAN_POINT('Ctrl Pts',(-6.810650611,4.365380951,2.516645918));
#142528=CARTESIAN_POINT('Ctrl Pts',(-6.653817825,4.430609079,2.879098531));
#142529=CARTESIAN_POINT('Ctrl Pts',(-6.65224511003996,4.43126318491329,
2.88273319605511));
#142530=CARTESIAN_POINT('Ctrl Pts',(-6.65067239507992,4.43191729082659,
2.88636786111022));
#142531=CARTESIAN_POINT('',(-6.97723436100188,4.43060908007269,2.75103628054129));
#142532=CARTESIAN_POINT('',(-6.81552610039196,4.43060908208281,2.8150673921034));
#142533=CARTESIAN_POINT('',(-7.16425997738659,4.34096089501395,2.21886885033756));
#142534=CARTESIAN_POINT('Origin',(0.166278515907661,4.55349069049514,-0.0866886118381799));
#142535=CARTESIAN_POINT('Ctrl Pts',(-6.92580098057473,4.30202682665899,
2.14377722136203));
#142536=CARTESIAN_POINT('Ctrl Pts',(-6.96545255544565,4.308834375779,2.15638583604463));
#142537=CARTESIAN_POINT('Ctrl Pts',(-7.00517370965433,4.31547784262409,
2.16895121645212));
#142538=CARTESIAN_POINT('Ctrl Pts',(-7.08464747199278,4.32844538542488,
2.19397395014918));
#142539=CARTESIAN_POINT('Ctrl Pts',(-7.1244472145633,4.33477714731917,2.20644613531202));
#142540=CARTESIAN_POINT('Ctrl Pts',(-7.16425997706287,4.34096089501268,
2.21886885134477));
#142541=CARTESIAN_POINT('Ctrl Pts',(-7.31358289534331,4.43188407004788,
1.66179769895285));
#142542=CARTESIAN_POINT('Ctrl Pts',(-7.31267622467166,4.43124657452394,
1.66576800047642));
#142543=CARTESIAN_POINT('Ctrl Pts',(-7.311769554,4.430609079,1.669738302));
#142544=CARTESIAN_POINT('Ctrl Pts',(-7.310320256,4.429590053,1.676084763));
#142545=CARTESIAN_POINT('Ctrl Pts',(-7.308859943,4.428571429,1.682428699));
#142546=CARTESIAN_POINT('Ctrl Pts',(-7.218437514,4.365498301,2.075244676));
#142547=CARTESIAN_POINT('Ctrl Pts',(-7.086433643,4.301245526,2.456106313));
#142548=CARTESIAN_POINT('Ctrl Pts',(-7.11867655828793,4.43188407004788,
1.37368338701899));
#142549=CARTESIAN_POINT('Ctrl Pts',(-7.11792644914396,4.43124657452394,
1.3775480240095));
#142550=CARTESIAN_POINT('Ctrl Pts',(-7.11717634,4.430609079,1.381412661));
#142551=CARTESIAN_POINT('Ctrl Pts',(-7.115977303,4.429590053,1.387590219));
#142552=CARTESIAN_POINT('Ctrl Pts',(-7.114767544,4.428571429,1.393765687));
#142553=CARTESIAN_POINT('Ctrl Pts',(-7.03985936,4.365498301,1.776150134));
#142554=CARTESIAN_POINT('Ctrl Pts',(-6.92439842400001,4.301245526,2.148303159));
#142555=CARTESIAN_POINT('',(-7.3117695495973,4.43060908088835,1.66973830899428));
#142556=CARTESIAN_POINT('Origin',(0.164335220526527,4.16161696526441,-0.0807408649835453));
#142557=CARTESIAN_POINT('',(-7.21447294344383,4.43060908179129,1.52557549831721));
#142558=CARTESIAN_POINT('Origin',(9.12898229232795E-13,4.52171037000067,
-3.59304599961696E-13));
#142559=CARTESIAN_POINT('',(-7.16618717794668,4.52063234083,2.21263673771566));
#142560=CARTESIAN_POINT('Origin',(0.181479818420224,4.69624337504075,-0.0268015869758415));
#142561=CARTESIAN_POINT('Origin',(0.181740147018993,4.55356363980172,-0.0616594868090475));
#142562=CARTESIAN_POINT('Ctrl Pts',(-7.490599804,4.301266351,0.375385897));
#142563=CARTESIAN_POINT('Ctrl Pts',(-7.470151454,4.365380951,0.783420434));
#142564=CARTESIAN_POINT('Ctrl Pts',(-7.405501982,4.430609079,1.186819448));
#142565=CARTESIAN_POINT('Ctrl Pts',(-7.40485367883351,4.43126318491329,
1.1908647224631));
#142566=CARTESIAN_POINT('Ctrl Pts',(-7.40420537566703,4.43191729082659,
1.19490999692619));
#142567=CARTESIAN_POINT('Ctrl Pts',(-7.225117579,4.301266351,0.600146619));
#142568=CARTESIAN_POINT('Ctrl Pts',(-7.192425865,4.365380951,0.993719575));
#142569=CARTESIAN_POINT('Ctrl Pts',(-7.11717634000001,4.430609079,1.381412661));
#142570=CARTESIAN_POINT('Ctrl Pts',(-7.11642173978711,4.43126318491329,
1.38530043683952));
#142571=CARTESIAN_POINT('Ctrl Pts',(-7.11566713957423,4.43191729082659,
1.38918821267904));
#142572=CARTESIAN_POINT('',(-7.40550198018438,4.43060908007269,1.18681943973392));
#142573=CARTESIAN_POINT('',(-7.26133916437191,4.43060908208281,1.28411603543277));
#142574=CARTESIAN_POINT('',(-7.47375477405679,4.34096089500807,0.62688880836363));
#142575=CARTESIAN_POINT('Origin',(0.181026394718455,4.55349067138657,-0.0489168858748047));
#142576=CARTESIAN_POINT('Ctrl Pts',(-7.22472833593329,4.30202682669847,
0.604814415005951));
#142577=CARTESIAN_POINT('Ctrl Pts',(-7.26616317342456,4.30883434543173,
0.608604313929139));
#142578=CARTESIAN_POINT('Ctrl Pts',(-7.30765664832846,4.31547778156078,
0.612337031069097));
#142579=CARTESIAN_POINT('Ctrl Pts',(-7.39065189691945,4.32844538539013,
0.619690272258531));
#142580=CARTESIAN_POINT('Ctrl Pts',(-7.43220229482626,4.33477714728864,
0.623315096574982));
#142581=CARTESIAN_POINT('Ctrl Pts',(-7.47375477396737,4.34096089499539,
0.62688880942525));
#142582=CARTESIAN_POINT('Ctrl Pts',(-7.49983277261798,4.43188407004788,
0.050741656424082));
#142583=CARTESIAN_POINT('Ctrl Pts',(-7.49980079730899,4.43124657452394,
0.0548140422120409));
#142584=CARTESIAN_POINT('Ctrl Pts',(-7.49976882200001,4.430609079,0.058886428));
#142585=CARTESIAN_POINT('Ctrl Pts',(-7.49971771,4.429590053,0.065396069));
#142586=CARTESIAN_POINT('Ctrl Pts',(-7.499655298,4.428571429,0.071905611));
#142587=CARTESIAN_POINT('Ctrl Pts',(-7.495790718,4.365498301,0.474975919));
#142588=CARTESIAN_POINT('Ctrl Pts',(-7.44874701800001,4.301245526,0.875310152000001));
#142589=CARTESIAN_POINT('Ctrl Pts',(-7.24754717756366,4.43188407004788,
-0.1887376018885));
#142590=CARTESIAN_POINT('Ctrl Pts',(-7.24764538878184,4.43124657452394,
-0.18480206644425));
#142591=CARTESIAN_POINT('Ctrl Pts',(-7.2477436,4.430609079,-0.180866531));
#142592=CARTESIAN_POINT('Ctrl Pts',(-7.247900589,4.429590053,-0.174575643));
#142593=CARTESIAN_POINT('Ctrl Pts',(-7.248046656,4.428571429,-0.168284491));
#142594=CARTESIAN_POINT('Ctrl Pts',(-7.257091136,4.365498301,0.221263065));
#142595=CARTESIAN_POINT('Ctrl Pts',(-7.224331513,4.301245526,0.609536047));
#142596=CARTESIAN_POINT('',(-7.49976881958266,4.43060908088848,0.0588864359526545));
#142597=CARTESIAN_POINT('Origin',(0.177850049580502,4.1616169083973,-0.0435259824795542));
#142598=CARTESIAN_POINT('',(-7.37375621114217,4.43060908179128,-0.0609900343115401));
#142599=CARTESIAN_POINT('Origin',(6.74807432154978E-13,4.52171036999867,
-9.36242457259123E-14));
#142600=CARTESIAN_POINT('',(-7.47429719740143,4.52063234084568,0.620388107456563));
#142601=CARTESIAN_POINT('Origin',(0.182998526927772,4.69624334770116,0.0128378233019234));
#142602=CARTESIAN_POINT('Origin',(0.190745673159929,4.55356367069499,-0.0211491355950279));
#142603=CARTESIAN_POINT('Ctrl Pts',(-7.396170615,4.301266351,-1.243647954));
#142604=CARTESIAN_POINT('Ctrl Pts',(-7.4639157,4.365380951,-0.840757247));
#142605=CARTESIAN_POINT('Ctrl Pts',(-7.48749656,4.430609079,-0.432891753));
#142606=CARTESIAN_POINT('Ctrl Pts',(-7.48773302822988,4.43126318491329,
-0.428801688795589));
#142607=CARTESIAN_POINT('Ctrl Pts',(-7.48796949645976,4.43191729082659,
-0.424711624591177));
#142608=CARTESIAN_POINT('Ctrl Pts',(-7.185212128,4.301266351,-0.967071182));
#142609=CARTESIAN_POINT('Ctrl Pts',(-7.23789128,4.365380951,-0.575671991));
#142610=CARTESIAN_POINT('Ctrl Pts',(-7.2477436,4.430609079,-0.180866531));
#142611=CARTESIAN_POINT('Ctrl Pts',(-7.24784239879999,4.43126318491329,
-0.176907432465295));
#142612=CARTESIAN_POINT('Ctrl Pts',(-7.24794119759997,4.43191729082659,
-0.172948333930589));
#142613=CARTESIAN_POINT('',(-7.48749655645112,4.43060908007267,-0.43289176068817));
#142614=CARTESIAN_POINT('',(-7.36762007919418,4.43060908208281,-0.306879161346311));
#142615=CARTESIAN_POINT('',(-7.4337851039095,4.34096089504206,-0.994403857097817));
#142616=CARTESIAN_POINT('Origin',(0.187309731765656,4.55349068566599,-0.0088579242423243));
#142617=CARTESIAN_POINT('Ctrl Pts',(-7.18583542313158,4.30202682672418,
-0.962428840202224));
#142618=CARTESIAN_POINT('Ctrl Pts',(-7.22711623438974,4.30883434230733,
-0.967634809921265));
#142619=CARTESIAN_POINT('Ctrl Pts',(-7.26844201754806,4.31547777524972,
-0.972909229457909));
#142620=CARTESIAN_POINT('Ctrl Pts',(-7.3510776533894,4.32844538542671,-0.983569433400221));
#142621=CARTESIAN_POINT('Ctrl Pts',(-7.39243585617379,4.33477714732437,
-0.988961462826314));
#142622=CARTESIAN_POINT('Ctrl Pts',(-7.43378510403677,4.34096089502777,
-0.994403856147091));
#142623=CARTESIAN_POINT('Ctrl Pts',(-7.33539880555815,4.43188407004788,
-1.56268700811032));
#142624=CARTESIAN_POINT('Ctrl Pts',(-7.33624302077908,4.43124657452394,
-1.55870295855516));
#142625=CARTESIAN_POINT('Ctrl Pts',(-7.33708723600001,4.430609079,-1.554718909));
#142626=CARTESIAN_POINT('Ctrl Pts',(-7.3384367,4.429590053,-1.548350472));
#142627=CARTESIAN_POINT('Ctrl Pts',(-7.339775105,4.428571429,-1.541979703));
#142628=CARTESIAN_POINT('Ctrl Pts',(-7.422649079,4.365498301,-1.147502184));
#142629=CARTESIAN_POINT('Ctrl Pts',(-7.462765261,4.301245526,-0.746414538));
#142630=CARTESIAN_POINT('Ctrl Pts',(-7.03753054804688,4.43188407004788,
-1.74233342918306));
#142631=CARTESIAN_POINT('Ctrl Pts',(-7.03847248652344,4.43124657452394,
-1.73851101659153));
#142632=CARTESIAN_POINT('Ctrl Pts',(-7.039414425,4.430609079,-1.734688604));
#142633=CARTESIAN_POINT('Ctrl Pts',(-7.040920098,4.429590053,-1.728578541));
#142634=CARTESIAN_POINT('Ctrl Pts',(-7.042415162,4.428571429,-1.722465874));
#142635=CARTESIAN_POINT('Ctrl Pts',(-7.134989397,4.365498301,-1.343970018));
#142636=CARTESIAN_POINT('Ctrl Pts',(-7.186462889,4.301245526,-0.957732292));
#142637=CARTESIAN_POINT('',(-7.3370872353543,4.43060908088849,-1.5547189007123));
#142638=CARTESIAN_POINT('Origin',(0.183048813547394,4.16161690417072,-0.0042758664672185));
#142639=CARTESIAN_POINT('',(-7.18825083433387,4.43060908179129,-1.64470373974391));
#142640=CARTESIAN_POINT('Origin',(-1.4658413372004E-13,4.52171037000022,
-7.2478915230656E-14));
#142641=CARTESIAN_POINT('',(-7.43291738723039,4.52063234080555,-1.00086918069252));
#142642=CARTESIAN_POINT('Origin',(0.175960374723824,4.69624334626897,0.0518769504692056));
#142643=CARTESIAN_POINT('Origin',(0.190832825460228,4.55356370548195,0.0203500376732782));
#142644=CARTESIAN_POINT('Ctrl Pts',(-6.955904708,4.301266351,-2.804530209));
#142645=CARTESIAN_POINT('Ctrl Pts',(-7.10867554300001,4.365380951,-2.425622053));
#142646=CARTESIAN_POINT('Ctrl Pts',(-7.21938412,4.430609079,-2.032361415));
#142647=CARTESIAN_POINT('Ctrl Pts',(-7.22049430263268,4.43126318491329,
-2.02841780789876));
#142648=CARTESIAN_POINT('Ctrl Pts',(-7.22160448526537,4.43191729082659,
-2.02447420079753));
#142649=CARTESIAN_POINT('Ctrl Pts',(-6.809334144,4.301266351,-2.489069809));
#142650=CARTESIAN_POINT('Ctrl Pts',(-6.944920943,4.365380951,-2.118145774));
#142651=CARTESIAN_POINT('Ctrl Pts',(-7.039414425,4.430609079,-1.734688604));
#142652=CARTESIAN_POINT('Ctrl Pts',(-7.04036200309613,4.43126318491329,
-1.73084330581221));
#142653=CARTESIAN_POINT('Ctrl Pts',(-7.04130958119224,4.43191729082659,
-1.72699800762441));
#142654=CARTESIAN_POINT('',(-7.21938411488067,4.43060908007265,-2.03236142178627));
#142655=CARTESIAN_POINT('',(-7.12939926755412,4.43060908208283,-1.88352502822083));
#142656=CARTESIAN_POINT('',(-7.0462199040165,4.34096089499886,-2.56919930375094));
#142657=CARTESIAN_POINT('Origin',(0.184834718843788,4.55349068833185,0.0316152152728183));
#142658=CARTESIAN_POINT('Ctrl Pts',(-6.81094083279843,4.30202682665829,
-2.48466999264095));
#142659=CARTESIAN_POINT('Ctrl Pts',(-6.85013758511489,4.30883437579503,
-2.49862847264263));
#142660=CARTESIAN_POINT('Ctrl Pts',(-6.88936356481079,4.31547784265374,
-2.51266347876292));
#142661=CARTESIAN_POINT('Ctrl Pts',(-6.96777522301014,4.32844539106519,
-2.54083853787839));
#142662=CARTESIAN_POINT('Ctrl Pts',(-7.00700740500025,4.33477715869623,
-2.55499530959718));
#142663=CARTESIAN_POINT('Ctrl Pts',(-7.04621990433313,4.34096089499308,
-2.56919930263159));
#142664=CARTESIAN_POINT('Ctrl Pts',(-6.82796974558505,4.43188407004788,
-3.10304616523142));
#142665=CARTESIAN_POINT('Ctrl Pts',(-6.82965067579253,4.43124657452394,
-3.09933674161571));
#142666=CARTESIAN_POINT('Ctrl Pts',(-6.831331606,4.430609079,-3.095627318));
#142667=CARTESIAN_POINT('Ctrl Pts',(-6.834018545,4.429590053,-3.089697866));
#142668=CARTESIAN_POINT('Ctrl Pts',(-6.836695187,4.428571429,-3.08376376));
#142669=CARTESIAN_POINT('Ctrl Pts',(-7.002432618,4.365498301,-2.716324361));
#142670=CARTESIAN_POINT('Ctrl Pts',(-7.127832894,4.301245526,-2.333237714));
#142671=CARTESIAN_POINT('Ctrl Pts',(-6.49844681077687,4.43188407004788,
-3.21445968164217));
#142672=CARTESIAN_POINT('Ctrl Pts',(-6.50018843288844,4.43124657452394,
-3.21092912382109));
#142673=CARTESIAN_POINT('Ctrl Pts',(-6.501930055,4.430609079,-3.207398566));
#142674=CARTESIAN_POINT('Ctrl Pts',(-6.504714009,4.429590053,-3.201755028));
#142675=CARTESIAN_POINT('Ctrl Pts',(-6.507488162,4.428571429,-3.196106666));
#142676=CARTESIAN_POINT('Ctrl Pts',(-6.679263483,4.365498301,-2.846360558));
#142677=CARTESIAN_POINT('Ctrl Pts',(-6.81256324800001,4.301245526,-2.480218134));
#142678=CARTESIAN_POINT('',(-6.83133160688307,4.4306090808884,-3.09562730976748));
#142679=CARTESIAN_POINT('Origin',(0.179688418953942,4.16161694203418,0.0351741913904707));
#142680=CARTESIAN_POINT('',(-6.6666308378463,4.43060908179129,-3.15151292645983));
#142681=CARTESIAN_POINT('Origin',(3.08347097854877E-13,4.52171036999956,
1.82579645846559E-13));
#142682=CARTESIAN_POINT('',(-7.0439826208049,4.52063234083322,-2.57532693793605));
#142683=CARTESIAN_POINT('Origin',(0.160694476196667,4.69624331874441,0.0884903518980124));
#142684=CARTESIAN_POINT('Origin',(0.181996628585891,4.55356368147533,0.0608976860971794));
#142685=CARTESIAN_POINT('Ctrl Pts',(-6.19038842800001,4.301266351,-4.234275748));
#142686=CARTESIAN_POINT('Ctrl Pts',(-6.421041618,4.365380951,-3.897067468));
#142687=CARTESIAN_POINT('Ctrl Pts',(-6.61370130300001,4.430609079,-3.536800117));
#142688=CARTESIAN_POINT('Ctrl Pts',(-6.61563328913966,4.43126318491329,
-3.53318736569346));
#142689=CARTESIAN_POINT('Ctrl Pts',(-6.61756527527932,4.43191729082659,
-3.52957461438691));
#142690=CARTESIAN_POINT('Ctrl Pts',(-6.115059263,4.301266351,-3.894682299));
#142691=CARTESIAN_POINT('Ctrl Pts',(-6.327213821,4.365380951,-3.561577415));
#142692=CARTESIAN_POINT('Ctrl Pts',(-6.501930055,4.430609079,-3.207398566));
#142693=CARTESIAN_POINT('Ctrl Pts',(-6.50368210469561,4.43126318491329,
-3.20384687002776));
#142694=CARTESIAN_POINT('Ctrl Pts',(-6.50543415439122,4.43191729082659,
-3.20029517405553));
#142695=CARTESIAN_POINT('',(-6.61370129655518,4.4306090800727,-3.53680012247357));
#142696=CARTESIAN_POINT('',(-6.55781567014535,4.43060908208281,-3.37209935871988));
#142697=CARTESIAN_POINT('',(-6.32918129308567,4.34096089502838,-4.02386184619341));
#142698=CARTESIAN_POINT('Origin',(0.173717228485566,4.55349068084526,0.0706101777306029));
#142699=CARTESIAN_POINT('Ctrl Pts',(-6.11757421903206,4.30202682671395,
-3.89073073857304));
#142700=CARTESIAN_POINT('Ctrl Pts',(-6.15285373557848,4.30883434169922,
-3.91278890945845));
#142701=CARTESIAN_POINT('Ctrl Pts',(-6.1881453258119,4.31547777403924,-3.93492808668518));
#142702=CARTESIAN_POINT('Ctrl Pts',(-6.25866730050807,4.32844538540129,
-3.97930083251753));
#142703=CARTESIAN_POINT('Ctrl Pts',(-6.29393893432853,4.3347771473131,-4.00156036445915));
#142704=CARTESIAN_POINT('Ctrl Pts',(-6.32918129360728,4.34096089502917,
-4.0238618453689));
#142705=CARTESIAN_POINT('Ctrl Pts',(-6.00127240686538,4.43188407004787,
-4.49831033178264));
#142706=CARTESIAN_POINT('Ctrl Pts',(-6.00371145443269,4.43124657452394,
-4.49504898289132));
#142707=CARTESIAN_POINT('Ctrl Pts',(-6.006150502,4.430609079,-4.491787634));
#142708=CARTESIAN_POINT('Ctrl Pts',(-6.010049279,4.429590053,-4.486574422));
#142709=CARTESIAN_POINT('Ctrl Pts',(-6.013939,4.428571429,-4.48135445));
#142710=CARTESIAN_POINT('Ctrl Pts',(-6.254790191,4.365498301,-4.158134229));
#142711=CARTESIAN_POINT('Ctrl Pts',(-6.459610984,4.301245526,-3.810961288));
#142712=CARTESIAN_POINT('Ctrl Pts',(-5.6555029236423,4.43188407004787,-4.53628137163683));
#142713=CARTESIAN_POINT('Ctrl Pts',(-5.65796279282115,4.43124657452394,
-4.53320775381842));
#142714=CARTESIAN_POINT('Ctrl Pts',(-5.660422662,4.430609079,-4.530134136));
#142715=CARTESIAN_POINT('Ctrl Pts',(-5.664354722,4.429590053,-4.525221009));
#142716=CARTESIAN_POINT('Ctrl Pts',(-5.668278248,4.428571429,-4.520301063));
#142717=CARTESIAN_POINT('Ctrl Pts',(-5.911222633,4.365498301,-4.215658441));
#142718=CARTESIAN_POINT('Ctrl Pts',(-6.120115721,4.301245526,-3.886731733));
#142719=CARTESIAN_POINT('',(-6.00615050467743,4.43060908088841,-4.49178762615972));
#142720=CARTESIAN_POINT('Origin',(0.16792599438362,4.16161688467452,0.0729795274135941));
#142721=CARTESIAN_POINT('',(-5.83328659251519,4.43060908179128,-4.51096087140242));
#142722=CARTESIAN_POINT('Origin',(-3.89445420356793E-13,4.52171037000067,
-2.85795692667179E-13));
#142723=CARTESIAN_POINT('',(-6.3256790556746,4.52063234084172,-4.02936527022594));
#142724=CARTESIAN_POINT('Origin',(0.137914834917369,4.69624337037489,0.120966140177844));
#142725=CARTESIAN_POINT('Origin',(0.164650191390726,4.55356366224679,0.0985976551418527));
#142726=CARTESIAN_POINT('Ctrl Pts',(-5.135416465,4.301266351,-5.46603126));
#142727=CARTESIAN_POINT('Ctrl Pts',(-5.433166924,4.365380951,-5.18629034));
#142728=CARTESIAN_POINT('Ctrl Pts',(-5.698769164,4.430609079,-4.87586197700001));
#142729=CARTESIAN_POINT('Ctrl Pts',(-5.70143261611943,4.43126318491329,
-4.87274900972471));
#142730=CARTESIAN_POINT('Ctrl Pts',(-5.70409606823886,4.43191729082659,
-4.86963604244942));
#142731=CARTESIAN_POINT('Ctrl Pts',(-5.134851007,4.301266351,-5.118183773));
#142732=CARTESIAN_POINT('Ctrl Pts',(-5.413653213,4.365380951,-4.838473655));
#142733=CARTESIAN_POINT('Ctrl Pts',(-5.660422662,4.430609079,-4.530134136));
#142734=CARTESIAN_POINT('Ctrl Pts',(-5.66289725939779,4.43126318491329,
-4.52704211559617));
#142735=CARTESIAN_POINT('Ctrl Pts',(-5.66537185679557,4.43191729082659,
-4.52395009519234));
#142736=CARTESIAN_POINT('',(-5.69876915651853,4.43060908007267,-4.87586198098007));
#142737=CARTESIAN_POINT('',(-5.67959590065063,4.43060908208281,-4.70299807141377));
#142738=CARTESIAN_POINT('',(-5.31619719916678,4.34096089504047,-5.29037308150137));
#142739=CARTESIAN_POINT('Origin',(0.15447676254813,4.55349068328005,0.106303469704071));
#142740=CARTESIAN_POINT('Ctrl Pts',(-5.13815663368765,4.30202682676978,
-5.11486523948491));
#142741=CARTESIAN_POINT('Ctrl Pts',(-5.16786948420241,4.30883434269612,
-5.1439917597904));
#142742=CARTESIAN_POINT('Ctrl Pts',(-5.197576712673,4.31547777600314,-5.17319998864913));
#142743=CARTESIAN_POINT('Ctrl Pts',(-5.25691108520785,4.32844538540515,
-5.23169545552141));
#142744=CARTESIAN_POINT('Ctrl Pts',(-5.28657294641733,4.33477714730095,
-5.2610169306122));
#142745=CARTESIAN_POINT('Ctrl Pts',(-5.31619719980772,4.34096089502036,
-5.29037308085881));
#142746=CARTESIAN_POINT('Ctrl Pts',(-4.89396224110399,4.43188407004788,
-5.68323850498272));
#142747=CARTESIAN_POINT('Ctrl Pts',(-4.897045358552,4.43124657452394,-5.68057772849136));
#142748=CARTESIAN_POINT('Ctrl Pts',(-4.900128476,4.430609079,-5.677916952));
#142749=CARTESIAN_POINT('Ctrl Pts',(-4.905056788,4.429590053,-5.673663745));
#142750=CARTESIAN_POINT('Ctrl Pts',(-4.909977709,4.428571429,-5.669401988));
#142751=CARTESIAN_POINT('Ctrl Pts',(-5.214680727,4.365498301,-5.405514363));
#142752=CARTESIAN_POINT('Ctrl Pts',(-5.489344843,4.301245526,-5.110488548));
#142753=CARTESIAN_POINT('Ctrl Pts',(-4.5481140040602,4.43188407004788,-5.64599158717323));
#142754=CARTESIAN_POINT('Ctrl Pts',(-4.5511771000301,4.43124657452394,-5.64351862808662));
#142755=CARTESIAN_POINT('Ctrl Pts',(-4.554240196,4.430609079,-5.64104566900001));
#142756=CARTESIAN_POINT('Ctrl Pts',(-4.559136504,4.429590053,-5.637092685));
#142757=CARTESIAN_POINT('Ctrl Pts',(-4.564025943,4.428571429,-5.633131207));
#142758=CARTESIAN_POINT('Ctrl Pts',(-4.866779581,4.365498301,-5.387836821));
#142759=CARTESIAN_POINT('Ctrl Pts',(-5.141498385,4.301245526,-5.111506076));
#142760=CARTESIAN_POINT('',(-4.90012848048857,4.43060908088848,-5.67791694500558));
#142761=CARTESIAN_POINT('Origin',(0.148311530019222,4.1616169810395,0.107372446471978));
#142762=CARTESIAN_POINT('',(-4.72718434919243,4.43060908179128,-5.65948129948078));
#142763=CARTESIAN_POINT('Origin',(9.66240976119082E-13,4.52171037000022,
9.49327422228308E-13));
#142764=CARTESIAN_POINT('',(-5.31159376899682,4.52063234084897,-5.2949949607014));
#142765=CARTESIAN_POINT('Origin',(0.10868640088724,4.69624337596615,0.147785719463314));
#142766=CARTESIAN_POINT('Origin',(0.139605180238045,4.55356367210724,0.131687433562332));
#142767=CARTESIAN_POINT('Ctrl Pts',(-3.840318136,4.301266351,-6.44220122400001));
#142768=CARTESIAN_POINT('Ctrl Pts',(-4.191243384,4.365380951,-6.233008039));
#142769=CARTESIAN_POINT('Ctrl Pts',(-4.517368912,4.430609079,-5.98693394900001));
#142770=CARTESIAN_POINT('Ctrl Pts',(-4.52063929002373,4.43126318491329,
-5.98446632464357));
#142771=CARTESIAN_POINT('Ctrl Pts',(-4.52390966804747,4.43191729082659,
-5.98199870028714));
#142772=CARTESIAN_POINT('Ctrl Pts',(-3.914542826,4.301266351,-6.102364662));
#142773=CARTESIAN_POINT('Ctrl Pts',(-4.246956198,4.365380951,-5.889128244));
#142774=CARTESIAN_POINT('Ctrl Pts',(-4.554240196,4.430609079,-5.641045669));
#142775=CARTESIAN_POINT('Ctrl Pts',(-4.55732163166763,4.43126318491329,
-5.63855790361001));
#142776=CARTESIAN_POINT('Ctrl Pts',(-4.56040306733527,4.43191729082659,
-5.63607013822001));
#142777=CARTESIAN_POINT('',(-4.51736890386037,4.43060908007272,-5.98693395125152));
#142778=CARTESIAN_POINT('',(-4.53580453873334,4.43060908208281,-5.81398982091035));
#142779=CARTESIAN_POINT('',(-4.05463363269045,4.34096089497448,-6.30951235068825));
#142780=CARTESIAN_POINT('Origin',(0.128012933467711,4.55349069865086,0.137025874071772));
#142781=CARTESIAN_POINT('Ctrl Pts',(-3.91848455494606,4.30202682656254,
-6.09983432463177));
#142782=CARTESIAN_POINT('Ctrl Pts',(-3.94124150545646,4.30883437570018,
-6.13466743762631));
#142783=CARTESIAN_POINT('Ctrl Pts',(-3.96397541205488,4.31547784255736,
-6.16957916015969));
#142784=CARTESIAN_POINT('Ctrl Pts',(-4.00934755056748,4.32844538537555,
-6.23946181292879));
#142785=CARTESIAN_POINT('Ctrl Pts',(-4.03201268352545,4.33477714727357,
-6.27447419159833));
#142786=CARTESIAN_POINT('Ctrl Pts',(-4.05463363371516,4.34096089497142,
-6.3095123500129));
#142787=CARTESIAN_POINT('Ctrl Pts',(-3.55781583914299,4.43188407004788,
-6.6024247660727));
#142788=CARTESIAN_POINT('Ctrl Pts',(-3.5613988635715,4.43124657452394,-6.60048897553635));
#142789=CARTESIAN_POINT('Ctrl Pts',(-3.564981888,4.430609079,-6.598553185));
#142790=CARTESIAN_POINT('Ctrl Pts',(-3.570709293,4.429590053,-6.595458856));
#142791=CARTESIAN_POINT('Ctrl Pts',(-3.576431317,4.428571429,-6.592354589));
#142792=CARTESIAN_POINT('Ctrl Pts',(-3.930738587,4.365498301,-6.400138652));
#142793=CARTESIAN_POINT('Ctrl Pts',(-4.262403038,4.301245526,-6.171055043));
#142794=CARTESIAN_POINT('Ctrl Pts',(-3.22806032850427,4.43188407004788,
-6.49170151124601));
#142795=CARTESIAN_POINT('Ctrl Pts',(-3.23158342425213,4.43124657452394,
-6.48994484362301));
#142796=CARTESIAN_POINT('Ctrl Pts',(-3.23510652,4.430609079,-6.488188176));
#142797=CARTESIAN_POINT('Ctrl Pts',(-3.24073813,4.429590053,-6.485380172));
#142798=CARTESIAN_POINT('Ctrl Pts',(-3.246364857,4.428571429,-6.482562396));
#142799=CARTESIAN_POINT('Ctrl Pts',(-3.594771326,4.365498301,-6.308085939));
#142800=CARTESIAN_POINT('Ctrl Pts',(-3.922470298,4.301245526,-6.09727207499999));
#142801=CARTESIAN_POINT('',(-3.56498189383822,4.43060908088846,-6.59855317909686));
#142802=CARTESIAN_POINT('Origin',(0.121762194606682,4.16161690396173,0.136744722697717));
#142803=CARTESIAN_POINT('',(-3.40004421925281,4.43060908179128,-6.54337067257439));
#142804=CARTESIAN_POINT('Origin',(-1.6154612370034E-13,4.52171037000156,
-3.25260651745651E-13));
#142805=CARTESIAN_POINT('',(-4.04914426134536,4.52063234081332,-6.31303657114383));
#142806=CARTESIAN_POINT('Origin',(0.0743757746014689,4.69624335400154,0.167694862273235));
#142807=CARTESIAN_POINT('Origin',(0.108032464906547,4.55356370820857,0.158619752400417));
#142808=CARTESIAN_POINT('Ctrl Pts',(-2.365650799,4.301266351,-7.11714102000001));
#142809=CARTESIAN_POINT('Ctrl Pts',(-2.75334196,4.365380951,-6.98827721));
#142810=CARTESIAN_POINT('Ctrl Pts',(-3.124741511,4.430609079,-6.818063544));
#142811=CARTESIAN_POINT('Ctrl Pts',(-3.12846589570875,4.43126318491329,
-6.8163566459352));
#142812=CARTESIAN_POINT('Ctrl Pts',(-3.1321902804175,4.43191729082659,-6.81464974787039));
#142813=CARTESIAN_POINT('Ctrl Pts',(-2.511194972,4.301266351,-6.801205762));
#142814=CARTESIAN_POINT('Ctrl Pts',(-2.881676231,4.365380951,-6.66441374200001));
#142815=CARTESIAN_POINT('Ctrl Pts',(-3.23510652,4.430609079,-6.488188176));
#142816=CARTESIAN_POINT('Ctrl Pts',(-3.23865070943269,4.43126318491329,
-6.48642099076369));
#142817=CARTESIAN_POINT('Ctrl Pts',(-3.24219489886538,4.43191729082659,
-6.48465380552737));
#142818=CARTESIAN_POINT('',(-3.12474150257614,4.43060908007272,-6.81806354444139));
#142819=CARTESIAN_POINT('',(-3.17992399802989,4.43060908208281,-6.65312586835001));
#142820=CARTESIAN_POINT('',(-2.60347990415908,4.34096089503555,-7.03362583523939));
#142821=CARTESIAN_POINT('Origin',(0.0955636390403675,4.55349066841947,0.161341518445375));
#142822=CARTESIAN_POINT('Ctrl Pts',(-2.51558849342807,4.30202682662507,
-6.79958193799661));
#142823=CARTESIAN_POINT('Ctrl Pts',(-2.53032530952334,4.30883437575032,
-6.83849274378294));
#142824=CARTESIAN_POINT('Ctrl Pts',(-2.54502272159871,4.31547784256747,
-6.87747536732137));
#142825=CARTESIAN_POINT('Ctrl Pts',(-2.57431138013896,4.32844538540733,
-6.95547787121539));
#142826=CARTESIAN_POINT('Ctrl Pts',(-2.58891998835045,4.33477714728761,
-6.99454401342095));
#142827=CARTESIAN_POINT('Ctrl Pts',(-2.60347990497689,4.34096089501081,
-7.03362583493863));
#142828=CARTESIAN_POINT('Ctrl Pts',(-2.05530992479785,4.43188407004787,
-7.21288898031392));
#142829=CARTESIAN_POINT('Ctrl Pts',(-2.05922531739893,4.43124657452394,
-7.21176869215696));
#142830=CARTESIAN_POINT('Ctrl Pts',(-2.06314071,4.430609079,-7.210648404));
#142831=CARTESIAN_POINT('Ctrl Pts',(-2.0693994,4.429590053,-7.208857642));
#142832=CARTESIAN_POINT('Ctrl Pts',(-2.075654973,4.428571429,-7.207056017));
#142833=CARTESIAN_POINT('Ctrl Pts',(-2.46299948,4.365498301,-7.095499572));
#142834=CARTESIAN_POINT('Ctrl Pts',(-2.836156005,4.301245526,-6.943069863));
#142835=CARTESIAN_POINT('Ctrl Pts',(-1.75706614025099,4.43188407004787,
-7.03386668559917));
#142836=CARTESIAN_POINT('Ctrl Pts',(-1.7608844996255,4.43124657452394,-7.03290844979958));
#142837=CARTESIAN_POINT('Ctrl Pts',(-1.764702859,4.430609079,-7.031950214));
#142838=CARTESIAN_POINT('Ctrl Pts',(-1.770806443,4.429590053,-7.03041849));
#142839=CARTESIAN_POINT('Ctrl Pts',(-1.776907359,4.428571429,-7.028876172));
#142840=CARTESIAN_POINT('Ctrl Pts',(-2.154675559,4.365498301,-6.93337597));
#142841=CARTESIAN_POINT('Ctrl Pts',(-2.52003186,4.301245526,-6.79793640900001));
#142842=CARTESIAN_POINT('',(-2.06314071700553,4.43060908088848,-7.21064839953072));
#142843=CARTESIAN_POINT('Origin',(0.0895193861963639,4.16161692514811,0.159722981985705));
#142844=CARTESIAN_POINT('',(-1.91392180109997,4.43060908179128,-7.12129930453859));
#142845=CARTESIAN_POINT('Origin',(2.83844128756705E-13,4.52171036999956,
6.29270940910587E-13));
#142846=CARTESIAN_POINT('',(-2.59736126722513,4.52063234085742,-7.03588760899641));
#142847=CARTESIAN_POINT('Origin',(0.0365874470749949,4.69624336608352,0.179762794924447));
#142848=CARTESIAN_POINT('Origin',(0.0714082026967897,4.55356366313828,0.178135238051541));
#142849=CARTESIAN_POINT('Ctrl Pts',(-0.780368259,4.301266351,-7.459291212));
#142850=CARTESIAN_POINT('Ctrl Pts',(-1.186697327,4.365380951,-7.416782306));
#142851=CARTESIAN_POINT('Ctrl Pts',(-1.586004669,4.430609079,-7.330388065));
#142852=CARTESIAN_POINT('Ctrl Pts',(-1.59000891228632,4.43126318491329,
-7.3295217058748));
#142853=CARTESIAN_POINT('Ctrl Pts',(-1.59401315557265,4.43191729082659,
-7.3286553467496));
#142854=CARTESIAN_POINT('Ctrl Pts',(-0.990426433,4.301266351,-7.182030039));
#142855=CARTESIAN_POINT('Ctrl Pts',(-1.381652286,4.365380951,-7.12807866));
#142856=CARTESIAN_POINT('Ctrl Pts',(-1.764702859,4.430609079,-7.03195021400001));
#142857=CARTESIAN_POINT('Ctrl Pts',(-1.76854407984401,4.43126318491329,
-7.03098624052886));
#142858=CARTESIAN_POINT('Ctrl Pts',(-1.77238530068803,4.43191729082659,
-7.03002226705771));
#142859=CARTESIAN_POINT('',(-1.58600466065801,4.43060908007271,-7.33038806363038));
#142860=CARTESIAN_POINT('',(-1.67535374514333,4.43060908208281,-7.18116914389923));
#142861=CARTESIAN_POINT('',(-1.03059034903994,4.34096089506838,-7.42885479274644));
#142862=CARTESIAN_POINT('Origin',(0.0586457274098809,4.55349069186996,0.178112571906096));
#142863=CARTESIAN_POINT('Ctrl Pts',(-0.995066310316856,4.30202682665611,
-7.18138865679072));
#142864=CARTESIAN_POINT('Ctrl Pts',(-1.00109391475538,4.30883437581194,
-7.22255772940696));
#142865=CARTESIAN_POINT('Ctrl Pts',(-1.00706759779501,4.31547784268671,
-7.26378847026125));
#142866=CARTESIAN_POINT('Ctrl Pts',(-1.01890327495275,4.32844538967593,
-7.34626354102029));
#142867=CARTESIAN_POINT('Ctrl Pts',(-1.02477228040847,4.334777155855,-7.38755678749405));
#142868=CARTESIAN_POINT('Ctrl Pts',(-1.03059034988965,4.34096089506402,
-7.42885479258455));
#142869=CARTESIAN_POINT('Ctrl Pts',(-0.45670000052831,4.43188407004788,
-7.48608652399922));
#142870=CARTESIAN_POINT('Ctrl Pts',(-0.460764682764155,4.43124657452394,
-7.48583412099961));
#142871=CARTESIAN_POINT('Ctrl Pts',(-0.464829365,4.430609079,-7.485581718));
#142872=CARTESIAN_POINT('Ctrl Pts',(-0.471326692,4.429590053,-7.485178256));
#142873=CARTESIAN_POINT('Ctrl Pts',(-0.477823308,4.428571429,-7.484763516));
#142874=CARTESIAN_POINT('Ctrl Pts',(-0.880093255,4.365498301,-7.459082817));
#142875=CARTESIAN_POINT('Ctrl Pts',(-1.277293469,4.301245526,-7.39043445200001));
#142876=CARTESIAN_POINT('Ctrl Pts',(-0.203913492723738,4.43188407004788,
-7.24713607501221));
#142877=CARTESIAN_POINT('Ctrl Pts',(-0.207848573361869,4.43124657452394,
-7.24702107600611));
#142878=CARTESIAN_POINT('Ctrl Pts',(-0.211783654,4.430609079,-7.246906077));
#142879=CARTESIAN_POINT('Ctrl Pts',(-0.218073815,4.429590053,-7.246722253));
#142880=CARTESIAN_POINT('Ctrl Pts',(-0.224363648,4.428571429,-7.24652751));
#142881=CARTESIAN_POINT('Ctrl Pts',(-0.613829558,4.365498301,-7.234469046));
#142882=CARTESIAN_POINT('Ctrl Pts',(-0.999759533999999,4.301245526,-7.180736792));
#142883=CARTESIAN_POINT('',(-0.464829372801399,4.43060908088847,-7.48558171513932));
#142884=CARTESIAN_POINT('Origin',(0.0530907540069721,4.16161691772973,0.175232768417251));
#142885=CARTESIAN_POINT('',(-0.338306526670948,4.43060908179128,-7.3662438967114));
#142886=CARTESIAN_POINT('Origin',(2.08058396899968E-13,4.52171036999933,
1.10935566288717E-12));
#142887=CARTESIAN_POINT('',(-1.02412854774876,4.52063234084464,-7.42974836164533));
#142888=CARTESIAN_POINT('Origin',(-0.00291160711715602,4.69624333806754,
0.183425348602292));
#142889=CARTESIAN_POINT('Origin',(0.0314449105638315,4.55356367649074,0.189321198648889));
#142890=CARTESIAN_POINT('Ctrl Pts',(0.841403432,4.301266351,-7.452653237));
#142891=CARTESIAN_POINT('Ctrl Pts',(0.435435954,4.365380951,-7.498486904));
#142892=CARTESIAN_POINT('Ctrl Pts',(0.026891988,4.430609079,-7.499951788));
#142893=CARTESIAN_POINT('Ctrl Pts',(0.0227951200966196,4.43126318491329,
-7.49996647781735));
#142894=CARTESIAN_POINT('Ctrl Pts',(0.0186982521932392,4.43191729082659,
-7.49998116763471));
#142895=CARTESIAN_POINT('Ctrl Pts',(0.576653346,4.301266351,-7.22703057400001));
#142896=CARTESIAN_POINT('Ctrl Pts',(0.182976184,4.365380951,-7.258442542));
#142897=CARTESIAN_POINT('Ctrl Pts',(-0.211783654,4.430609079,-7.246906077));
#142898=CARTESIAN_POINT('Ctrl Pts',(-0.215742295038517,4.43126318491329,
-7.24679038963925));
#142899=CARTESIAN_POINT('Ctrl Pts',(-0.219700936077033,4.43191729082659,
-7.24667470227851));
#142900=CARTESIAN_POINT('',(0.0268919958281766,4.43060908007272,-7.49995178486281));
#142901=CARTESIAN_POINT('',(-0.0924458136384814,4.43060908208281,-7.37342893274275));
#142902=CARTESIAN_POINT('',(0.590488465954577,4.3409608949906,-7.47671875698683));
#142903=CARTESIAN_POINT('Origin',(0.0189856734592331,4.55349069303058,0.186555619209687));
#142904=CARTESIAN_POINT('Ctrl Pts',(0.571984068188108,4.30202682662381,
-7.22740162320937));
#142905=CARTESIAN_POINT('Ctrl Pts',(0.574947519445653,4.30883437575215,
-7.26890394261364));
#142906=CARTESIAN_POINT('Ctrl Pts',(0.577976888267639,4.31547784260444,
-7.31045489694304));
#142907=CARTESIAN_POINT('Ctrl Pts',(0.584147625599597,4.32844539120785,
-7.39354607766314));
#142908=CARTESIAN_POINT('Ctrl Pts',(0.587292662433661,4.33477715900784,
-7.43513558513006));
#142909=CARTESIAN_POINT('Ctrl Pts',(0.590488464761412,4.34096089498466,
-7.47671875703932));
#142910=CARTESIAN_POINT('Ctrl Pts',(1.16326470617875,4.43188407004787,-7.40924298180975));
#142911=CARTESIAN_POINT('Ctrl Pts',(1.15924079508937,4.43124657452393,-7.40987026640487));
#142912=CARTESIAN_POINT('Ctrl Pts',(1.155216884,4.430609079,-7.410497551));
#142913=CARTESIAN_POINT('Ctrl Pts',(1.148784729,4.429590053,-7.411500255));
#142914=CARTESIAN_POINT('Ctrl Pts',(1.142350843,4.428571429,-7.412491791));
#142915=CARTESIAN_POINT('Ctrl Pts',(0.743965153,4.365498301,-7.47388764));
#142916=CARTESIAN_POINT('Ctrl Pts',(0.341293891,4.301245526,-7.492230541));
#142917=CARTESIAN_POINT('Ctrl Pts',(1.35877392498202,4.43188407004787,-7.12153743297934));
#142918=CARTESIAN_POINT('Ctrl Pts',(1.35490612249101,4.43124657452393,-7.12227104898968));
#142919=CARTESIAN_POINT('Ctrl Pts',(1.35103832,4.430609079,-7.123004665));
#142920=CARTESIAN_POINT('Ctrl Pts',(1.344855702,4.429590053,-7.12417733800001));
#142921=CARTESIAN_POINT('Ctrl Pts',(1.338671059,4.428571429,-7.125339276));
#142922=CARTESIAN_POINT('Ctrl Pts',(0.955718432,4.365498301,-7.19728639000001));
#142923=CARTESIAN_POINT('Ctrl Pts',(0.567260438,4.301245526,-7.227773903));
#142924=CARTESIAN_POINT('',(1.15521687582595,4.4306090808884,-7.41049754966774));
#142925=CARTESIAN_POINT('Origin',(0.0141796548106751,4.16161692684402,0.182548867422564));
#142926=CARTESIAN_POINT('',(1.25312758506097,4.43060908179128,-7.26675111092108));
#142927=CARTESIAN_POINT('Origin',(4.85976683157682E-14,4.52171036999889,
4.54931231574918E-13));
#142928=CARTESIAN_POINT('',(0.59699128478794,4.52063234082281,-7.47620233853116));
#142929=CARTESIAN_POINT('Origin',(-0.0422745649116112,4.6962433242186,0.178510930585105));
#142930=CARTESIAN_POINT('Origin',(-0.00998869204440783,4.55356365368728,
0.191654495980108));
#142931=CARTESIAN_POINT('Ctrl Pts',(2.423832035,4.301266351,-7.097537479));
#142932=CARTESIAN_POINT('Ctrl Pts',(2.037208734,4.365380951,-7.229570588));
#142933=CARTESIAN_POINT('Ctrl Pts',(1.638531205,4.430609079,-7.3188261));
#142934=CARTESIAN_POINT('Ctrl Pts',(1.6345332774615,4.43126318491329,-7.31972115187383));
#142935=CARTESIAN_POINT('Ctrl Pts',(1.630535349923,4.43191729082659,-7.32061620374768));
#142936=CARTESIAN_POINT('Ctrl Pts',(2.116769455,4.301266351,-6.934103192));
#142937=CARTESIAN_POINT('Ctrl Pts',(1.739048891,4.365380951,-7.049409718));
#142938=CARTESIAN_POINT('Ctrl Pts',(1.35103832,4.430609079,-7.123004665));
#142939=CARTESIAN_POINT('Ctrl Pts',(1.34714736042944,4.43126318491329,-7.12374267314921));
#142940=CARTESIAN_POINT('Ctrl Pts',(1.34325640085888,4.43191729082659,-7.1244806812984));
#142941=CARTESIAN_POINT('',(1.63853121200172,4.43060908007271,-7.31882609525449));
#142942=CARTESIAN_POINT('',(1.49478478146104,4.43060908208281,-7.22091537857492));
#142943=CARTESIAN_POINT('',(2.18395669669526,4.34096089502823,-7.1749796617874));
#142944=CARTESIAN_POINT('Origin',(-0.021562133991038,4.55349069234491,0.186275393138425));
#142945=CARTESIAN_POINT('Ctrl Pts',(2.11228910713819,4.30202682661483,-6.93546932305721));
#142946=CARTESIAN_POINT('Ctrl Pts',(2.12410504656257,4.30883437576042,-6.97536428675135));
#142947=CARTESIAN_POINT('Ctrl Pts',(2.13599581749022,4.31547784262358,-7.01529257801128));
#142948=CARTESIAN_POINT('Ctrl Pts',(2.15988442355864,4.32844538540125,-7.09511457087793));
#142949=CARTESIAN_POINT('Ctrl Pts',(2.17189643383093,4.33477714729008,-7.13505560883328));
#142950=CARTESIAN_POINT('Ctrl Pts',(2.1839566958225,4.34096089501118,-7.17497966205368));
#142951=CARTESIAN_POINT('Ctrl Pts',(2.72883644918952,4.43188407004788,-6.98595147272629));
#142952=CARTESIAN_POINT('Ctrl Pts',(2.72504146259476,4.43124657452394,-6.98742911336314));
#142953=CARTESIAN_POINT('Ctrl Pts',(2.721246476,4.430609079,-6.988906754));
#142954=CARTESIAN_POINT('Ctrl Pts',(2.715180253,4.429590053,-6.991268738));
#142955=CARTESIAN_POINT('Ctrl Pts',(2.709109939,4.428571429,-6.993620188));
#142956=CARTESIAN_POINT('Ctrl Pts',(2.333236578,4.365498301,-7.139221784));
#142957=CARTESIAN_POINT('Ctrl Pts',(1.943922727,4.301245526,-7.243698257));
#142958=CARTESIAN_POINT('Ctrl Pts',(2.85792658132718,4.43188407004788,-6.66294361747869));
#142959=CARTESIAN_POINT('Ctrl Pts',(2.85430691216359,4.43124657452394,-6.66449154473935));
#142960=CARTESIAN_POINT('Ctrl Pts',(2.850687243,4.430609079,-6.666039472));
#142961=CARTESIAN_POINT('Ctrl Pts',(2.844901262,4.429590053,-6.66851380800001));
#142962=CARTESIAN_POINT('Ctrl Pts',(2.839110994,4.428571429,-6.670978097));
#142963=CARTESIAN_POINT('Ctrl Pts',(2.48057809,4.365498301,-6.823566622));
#142964=CARTESIAN_POINT('Ctrl Pts',(2.107755942,4.301245526,-6.93684834));
#142965=CARTESIAN_POINT('',(2.72124646772514,4.43060908088843,-6.98890675455777));
#142966=CARTESIAN_POINT('Origin',(-0.0253944807870607,4.16161700236696,
0.181329183444667));
#142967=CARTESIAN_POINT('',(2.78596684358495,4.43060908179128,-6.82747311949418));
#142968=CARTESIAN_POINT('Origin',(-9.20379224222945E-13,4.52171036999956,
2.86532950144469E-12));
#142969=CARTESIAN_POINT('',(2.19019646746151,4.52063234082816,-7.1730774032274));
#142970=CARTESIAN_POINT('Origin',(-0.0796607088715576,4.69624335133068,
0.165249406375639));
#142971=CARTESIAN_POINT('Origin',(-0.0509551821821491,4.55356366255728,
0.185026366182512));
#142972=CARTESIAN_POINT('Ctrl Pts',(3.892924945,4.301266351,-6.410548758));
#142973=CARTESIAN_POINT('Ctrl Pts',(3.543723898,4.365380951,-6.622607587));
#142974=CARTESIAN_POINT('Ctrl Pts',(3.173554525,4.430609079,-6.795480239));
#142975=CARTESIAN_POINT('Ctrl Pts',(3.16984247648315,4.43126318491329,-6.7972138013049));
#142976=CARTESIAN_POINT('Ctrl Pts',(3.1661304279663,4.43191729082659,-6.79894736360979));
#142977=CARTESIAN_POINT('Ctrl Pts',(3.557907777,4.301266351,-6.31694485100001));
#142978=CARTESIAN_POINT('Ctrl Pts',(3.213805605,4.365380951,-6.510754331));
#142979=CARTESIAN_POINT('Ctrl Pts',(2.850687243,4.430609079,-6.666039472));
#142980=CARTESIAN_POINT('Ctrl Pts',(2.84704590183182,4.43126318491329,-6.6675966672176));
#142981=CARTESIAN_POINT('Ctrl Pts',(2.84340456066365,4.43191729082659,-6.6691538624352));
#142982=CARTESIAN_POINT('',(3.17355453084134,4.43060908007268,-6.7954802328551));
#142983=CARTESIAN_POINT('',(3.01212090167401,4.43060908208281,-6.73075984759061));
#142984=CARTESIAN_POINT('',(3.67530553870476,4.34096089505283,-6.53774649241647));
#142985=CARTESIAN_POINT('Origin',(-0.0611017768781913,4.55349067999031,
0.177285242002856));
#142986=CARTESIAN_POINT('Ctrl Pts',(3.55382585549295,4.30202682665132,-6.31924218533956));
#142987=CARTESIAN_POINT('Ctrl Pts',(3.57394168121668,4.30883434154526,-6.35566416610688));
#142988=CARTESIAN_POINT('Ctrl Pts',(3.59413774087051,4.31547777379272,-6.39210258844027));
#142989=CARTESIAN_POINT('Ctrl Pts',(3.63462742824362,4.32844538541138,-6.46492342997811));
#142990=CARTESIAN_POINT('Ctrl Pts',(3.65494474691591,4.33477714732342,-6.50134844167838));
#142991=CARTESIAN_POINT('Ctrl Pts',(3.67530553792546,4.34096089503749,-6.53774649285502));
#142992=CARTESIAN_POINT('Ctrl Pts',(4.16681083229605,4.43188407004787,-6.23600463637641));
#142993=CARTESIAN_POINT('Ctrl Pts',(4.16342221964803,4.43124657452394,-6.2382635406882));
#142994=CARTESIAN_POINT('Ctrl Pts',(4.160033607,4.430609079,-6.240522445));
#142995=CARTESIAN_POINT('Ctrl Pts',(4.154616966,4.429590053,-6.244133266));
#142996=CARTESIAN_POINT('Ctrl Pts',(4.149194064,4.428571429,-6.247734679));
#142997=CARTESIAN_POINT('Ctrl Pts',(3.813408453,4.365498301,-6.470733852));
#142998=CARTESIAN_POINT('Ctrl Pts',(3.455655896,4.301245526,-6.656458693));
#142999=CARTESIAN_POINT('Ctrl Pts',(4.2234457685604,4.43188407004787,-5.89279796219158));
#143000=CARTESIAN_POINT('Ctrl Pts',(4.2202434837802,4.43124657452394,-5.89508782209579));
#143001=CARTESIAN_POINT('Ctrl Pts',(4.217041199,4.430609079,-5.897377682));
#143002=CARTESIAN_POINT('Ctrl Pts',(4.2119224,4.429590053,-5.90103798500001));
#143003=CARTESIAN_POINT('Ctrl Pts',(4.206797255,4.428571429,-5.904689396));
#143004=CARTESIAN_POINT('Ctrl Pts',(3.889448673,4.365498301,-6.130784462));
#143005=CARTESIAN_POINT('Ctrl Pts',(3.549695121,4.301245526,-6.321563458));
#143006=CARTESIAN_POINT('',(4.16003359904532,4.43060908088844,-6.24052244736554));
#143007=CARTESIAN_POINT('Origin',(-0.0637811806429589,4.16161696907178,
0.171630745914088));
#143008=CARTESIAN_POINT('',(4.18853738885309,4.43060908179128,-6.06895007326361));
#143009=CARTESIAN_POINT('Origin',(-2.25730892311482E-13,4.52171037000022,
4.59701721133854E-13));
#143010=CARTESIAN_POINT('',(3.68099049779537,4.52063234084953,-6.53454734113602));
#143011=CARTESIAN_POINT('Origin',(-0.113322216422975,4.6962433515151,0.144261627847397));
#143012=CARTESIAN_POINT('Origin',(-0.089539248214478,4.55356366861275,0.169746975297933));
#143013=CARTESIAN_POINT('Ctrl Pts',(5.179989011,4.301266351,-5.423809901));
#143014=CARTESIAN_POINT('Ctrl Pts',(4.884538471,4.365380951,-5.705978816));
#143015=CARTESIAN_POINT('Ctrl Pts',(4.560185962,4.430609079,-5.954385274));
#143016=CARTESIAN_POINT('Ctrl Pts',(4.55693336376311,4.43126318491329,-5.95687628728));
#143017=CARTESIAN_POINT('Ctrl Pts',(4.55368076552623,4.43191729082659,-5.95936730056002));
#143018=CARTESIAN_POINT('Ctrl Pts',(4.832682286,4.301266351,-5.404413189));
#143019=CARTESIAN_POINT('Ctrl Pts',(4.53828834,4.365380951,-5.66766330700001));
#143020=CARTESIAN_POINT('Ctrl Pts',(4.217041199,4.430609079,-5.897377682));
#143021=CARTESIAN_POINT('Ctrl Pts',(4.2138197413099,4.43126318491329,-5.89968125157441));
#143022=CARTESIAN_POINT('Ctrl Pts',(4.2105982836198,4.43191729082659,-5.90198482114881));
#143023=CARTESIAN_POINT('',(4.5601859663393,4.43060908007276,-5.95438526676242));
#143024=CARTESIAN_POINT('',(4.38861359606048,4.43060908208281,-5.92588146647616));
#143025=CARTESIAN_POINT('',(4.99480117906598,4.34096089499077,-5.59481556261796));
#143026=CARTESIAN_POINT('Origin',(-0.0977841513231226,4.55349066656064,
0.160005103683161));
#143027=CARTESIAN_POINT('Ctrl Pts',(4.82918965631123,4.30202682667343,-5.40753430549404));
#143028=CARTESIAN_POINT('Ctrl Pts',(4.85666484375131,4.3088343438705,-5.43878046339275));
#143029=CARTESIAN_POINT('Ctrl Pts',(4.88422192483148,4.31547777844033,-5.47002543166698));
#143030=CARTESIAN_POINT('Ctrl Pts',(4.93941931908904,4.32844539121672,-5.5324396823216));
#143031=CARTESIAN_POINT('Ctrl Pts',(4.96709195863958,4.33477715901929,-5.56364550569783));
#143032=CARTESIAN_POINT('Ctrl Pts',(4.99480117811663,4.34096089498488,-5.59481556334787));
#143033=CARTESIAN_POINT('Ctrl Pts',(5.40994977202152,4.43188407004788,-5.19446915376555));
#143034=CARTESIAN_POINT('Ctrl Pts',(5.40712598101076,4.43124657452394,-5.19740369788278));
#143035=CARTESIAN_POINT('Ctrl Pts',(5.40430219,4.430609079,-5.200338242));
#143036=CARTESIAN_POINT('Ctrl Pts',(5.399788407,4.429590053,-5.205029062));
#143037=CARTESIAN_POINT('Ctrl Pts',(5.395266487,4.428571429,-5.209712039));
#143038=CARTESIAN_POINT('Ctrl Pts',(5.115269587,4.365498301,-5.499681596));
#143039=CARTESIAN_POINT('Ctrl Pts',(4.805806437,4.301245526,-5.757970518));
#143040=CARTESIAN_POINT('Ctrl Pts',(5.39148132667975,4.43188407004788,-4.84711162513905));
#143041=CARTESIAN_POINT('Ctrl Pts',(5.38884616133987,4.43124657452394,-4.85003634556952));
#143042=CARTESIAN_POINT('Ctrl Pts',(5.38621099600001,4.430609079,-4.852961066));
#143043=CARTESIAN_POINT('Ctrl Pts',(5.381998728,4.429590053,-4.857636183));
#143044=CARTESIAN_POINT('Ctrl Pts',(5.377778351,4.428571429,-4.862303981));
#143045=CARTESIAN_POINT('Ctrl Pts',(5.116452959,4.365498301,-5.15133363500001));
#143046=CARTESIAN_POINT('Ctrl Pts',(4.825654501,4.301245526,-5.410689294));
#143047=CARTESIAN_POINT('',(5.40430218280887,4.4306090808885,-5.20033824619336));
#143048=CARTESIAN_POINT('Origin',(-0.0991855536857289,4.16161699807092,
0.153907044168407));
#143049=CARTESIAN_POINT('',(5.39525658128275,4.43060908179127,-5.02664966657648));
#143050=CARTESIAN_POINT('Origin',(-1.36175792864179E-13,4.52171037000067,
1.70870262383715E-13));
#143051=CARTESIAN_POINT('',(4.99966550416853,4.52063234088266,-5.59046910769365));
#143052=CARTESIAN_POINT('Origin',(-0.141684595591913,4.69624335486042,0.116527713020292));
#143053=CARTESIAN_POINT('Origin',(-0.123936256214732,4.55356364505988,0.146529879876864));
#143054=CARTESIAN_POINT('Ctrl Pts',(6.22484254900001,4.301266351,-4.183459721));
#143055=CARTESIAN_POINT('Ctrl Pts',(5.996957454,4.365380951,-4.522544817));
#143056=CARTESIAN_POINT('Ctrl Pts',(5.733588172,4.430609079,-4.834869871));
#143057=CARTESIAN_POINT('Ctrl Pts',(5.73094711192334,4.43126318491329,-4.83800185824163));
#143058=CARTESIAN_POINT('Ctrl Pts',(5.72830605184669,4.43191729082659,-4.84113384548325));
#143059=CARTESIAN_POINT('Ctrl Pts',(5.881485942,4.301266351,-4.239177174));
#143060=CARTESIAN_POINT('Ctrl Pts',(5.650565757,4.365380951,-4.559558646));
#143061=CARTESIAN_POINT('Ctrl Pts',(5.386210996,4.430609079,-4.852961066));
#143062=CARTESIAN_POINT('Ctrl Pts',(5.38356005356643,4.43126318491329,-4.85590329757679));
#143063=CARTESIAN_POINT('Ctrl Pts',(5.38090911113287,4.43191729082659,-4.85884552915358));
#143064=CARTESIAN_POINT('',(5.73358817469224,4.4306090800727,-4.83486986299197));
#143065=CARTESIAN_POINT('',(5.5598995967194,4.43060908208281,-4.84391545390054));
#143066=CARTESIAN_POINT('',(6.0807454673922,4.34096089504328,-4.39027727584636));
#143067=CARTESIAN_POINT('Origin',(-0.129894276797609,4.55349069609996,0.135243500745896));
#143068=CARTESIAN_POINT('Ctrl Pts',(5.87874591497346,4.30202682664127,-4.24297613265704));
#143069=CARTESIAN_POINT('Ctrl Pts',(5.91229590573509,4.30883437579162,-4.26758553485663));
#143070=CARTESIAN_POINT('Ctrl Pts',(5.9459256381493,4.31547784262217,-4.29217618267673));
#143071=CARTESIAN_POINT('Ctrl Pts',(6.01324942856366,4.32844539019364,-4.34126516762885));
#143072=CARTESIAN_POINT('Ctrl Pts',(6.04698342047828,4.33477715688986,-4.36579261205998));
#143073=CARTESIAN_POINT('Ctrl Pts',(6.08074546675362,4.34096089503838,-4.39027727658286));
#143074=CARTESIAN_POINT('Ctrl Pts',(6.40012547593568,4.43188407004788,-3.91004606778592));
#143075=CARTESIAN_POINT('Ctrl Pts',(6.39799854296784,4.43124657452394,-3.91351903539296));
#143076=CARTESIAN_POINT('Ctrl Pts',(6.39587161,4.430609079,-3.916992003));
#143077=CARTESIAN_POINT('Ctrl Pts',(6.392471743,4.429590053,-3.922543484));
#143078=CARTESIAN_POINT('Ctrl Pts',(6.389062245,4.428571429,-3.928089055));
#143079=CARTESIAN_POINT('Ctrl Pts',(6.1779464,4.365498301,-4.271470342));
#143080=CARTESIAN_POINT('Ctrl Pts',(5.93124281,4.301245526,-4.590246042));
#143081=CARTESIAN_POINT('Ctrl Pts',(6.30741720870541,4.43188407004788,-3.57477973384486));
#143082=CARTESIAN_POINT('Ctrl Pts',(6.30547238085271,4.43124657452394,-3.57820255892243));
#143083=CARTESIAN_POINT('Ctrl Pts',(6.303527553,4.430609079,-3.581625384));
#143084=CARTESIAN_POINT('Ctrl Pts',(6.300418778,4.429590053,-3.587096713));
#143085=CARTESIAN_POINT('Ctrl Pts',(6.297300509,4.428571429,-3.592562637));
#143086=CARTESIAN_POINT('Ctrl Pts',(6.104217591,4.365498301,-3.931012172));
#143087=CARTESIAN_POINT('Ctrl Pts',(5.875971639,4.301245526,-4.246817313));
#143088=CARTESIAN_POINT('',(6.39587160368013,4.43060908088839,-3.91699200834876));
#143089=CARTESIAN_POINT('Origin',(-0.129952104088461,4.16161691724407,0.128986828453043));
#143090=CARTESIAN_POINT('',(6.34969957276025,4.43060908179128,-3.74930870830136));
#143091=CARTESIAN_POINT('Origin',(7.65446733774766E-13,4.52171036999978,
-5.46871575801688E-13));
#143092=CARTESIAN_POINT('',(6.08456170863532,4.52063234083347,-4.38498675147079));
#143093=CARTESIAN_POINT('Origin',(-0.163422130634084,4.69624337618487,0.0833453740582352));
#143094=CARTESIAN_POINT('Origin',(-0.152538369419406,4.55356363696838,0.116461520178344));
#143095=CARTESIAN_POINT('Ctrl Pts',(6.97862936700001,4.301266351,-2.747495615));
#143096=CARTESIAN_POINT('Ctrl Pts',(6.828965371,4.365380951,-3.127641648));
#143097=CARTESIAN_POINT('Ctrl Pts',(6.638894171,4.430609079,-3.489281327));
#143098=CARTESIAN_POINT('Ctrl Pts',(6.63698814211831,4.43126318491329,-3.49290783997482));
#143099=CARTESIAN_POINT('Ctrl Pts',(6.63508211323662,4.43191729082659,-3.49653435294964));
#143100=CARTESIAN_POINT('Ctrl Pts',(6.65527785200001,4.301266351,-2.875721945));
#143101=CARTESIAN_POINT('Ctrl Pts',(6.498628999,4.365380951,-3.238254091));
#143102=CARTESIAN_POINT('Ctrl Pts',(6.303527553,4.430609079,-3.581625384));
#143103=CARTESIAN_POINT('Ctrl Pts',(6.30157108094671,4.43126318491329,-3.58506870209134));
#143104=CARTESIAN_POINT('Ctrl Pts',(6.29961460889341,4.43191729082659,-3.58851202018267));
#143105=CARTESIAN_POINT('',(6.63889417191426,4.43060908007269,-3.48928131859345));
#143106=CARTESIAN_POINT('',(6.47121087128357,4.43060908208281,-3.53545333850757));
#143107=CARTESIAN_POINT('',(6.88236085627095,4.34096089503935,-2.98045450270494));
#143108=CARTESIAN_POINT('Origin',(-0.155930962172045,4.55349066752806,0.104158239654767));
#143109=CARTESIAN_POINT('Ctrl Pts',(6.65341855005723,4.30202682672195,-2.88002111094166));
#143110=CARTESIAN_POINT('Ctrl Pts',(6.69147429397009,4.30883434710691,-2.89684283187069));
#143111=CARTESIAN_POINT('Ctrl Pts',(6.72960386510242,4.31547778490924,-2.91362908767087));
#143112=CARTESIAN_POINT('Ctrl Pts',(6.80590665479749,4.3284453854024,-2.94709791124446));
#143113=CARTESIAN_POINT('Ctrl Pts',(6.84412460925024,4.33477714731954,-2.96380009312779));
#143114=CARTESIAN_POINT('Ctrl Pts',(6.88236085589657,4.34096089503806,-2.98045450356496));
#143115=CARTESIAN_POINT('Ctrl Pts',(7.09103842230695,4.43188407004788,-2.44279357166386));
#143116=CARTESIAN_POINT('Ctrl Pts',(7.08970780165348,4.43124657452394,-2.44664257133193));
#143117=CARTESIAN_POINT('Ctrl Pts',(7.08837718100001,4.430609079,-2.450491571));
#143118=CARTESIAN_POINT('Ctrl Pts',(7.086250206,4.429590053,-2.456644133));
#143119=CARTESIAN_POINT('Ctrl Pts',(7.084112554,4.428571429,-2.462792993));
#143120=CARTESIAN_POINT('Ctrl Pts',(6.951749306,4.365498301,-2.843529882));
#143121=CARTESIAN_POINT('Ctrl Pts',(6.779340862,4.301245526,-3.207886762));
#143122=CARTESIAN_POINT('Ctrl Pts',(6.92842527283416,4.43188407004788,-2.13529511646555));
#143123=CARTESIAN_POINT('Ctrl Pts',(6.92726171991709,4.43124657452394,-2.13905599823277));
#143124=CARTESIAN_POINT('Ctrl Pts',(6.926098167,4.430609079,-2.14281688));
#143125=CARTESIAN_POINT('Ctrl Pts',(6.924238247,4.429590053,-2.148828587));
#143126=CARTESIAN_POINT('Ctrl Pts',(6.922367894,4.428571429,-2.154837056));
#143127=CARTESIAN_POINT('Ctrl Pts',(6.806555793,4.365498301,-2.52688095));
#143128=CARTESIAN_POINT('Ctrl Pts',(6.651534875,4.301245526,-2.884368874));
#143129=CARTESIAN_POINT('',(7.08837717605875,4.43060908088843,-2.45049157765917));
#143130=CARTESIAN_POINT('Origin',(-0.154642244386126,4.16161685423742,0.0980353349978125));
#143131=CARTESIAN_POINT('',(7.00723766864643,4.43060908179128,-2.29665424183409));
#143132=CARTESIAN_POINT('Origin',(1.25333771139324E-13,4.52171037000133,
-1.06902334207071E-13));
#143133=CARTESIAN_POINT('',(6.88495056955131,4.52063234088447,-2.9744672892662));
#143134=CARTESIAN_POINT('Origin',(-0.177518215075657,4.69624335632667,0.0462658936315824));
#143135=CARTESIAN_POINT('Origin',(-0.174007811928394,4.55356365656574,0.080947440733857));
#143136=CARTESIAN_POINT('Ctrl Pts',(7.406103233,4.301266351,-1.183061667));
#143137=CARTESIAN_POINT('Ctrl Pts',(7.341658458,4.365380951,-1.586493433));
#143138=CARTESIAN_POINT('Ctrl Pts',(7.233772858,4.430609079,-1.980537866));
#143139=CARTESIAN_POINT('Ctrl Pts',(7.23269098410475,4.43126318491329,-1.98448933297642));
#143140=CARTESIAN_POINT('Ctrl Pts',(7.2316091102095,4.43191729082659,-1.98844079995283));
#143141=CARTESIAN_POINT('Ctrl Pts',(7.117876367,4.301266351,-1.377801155));
#143142=CARTESIAN_POINT('Ctrl Pts',(7.042823572,4.365380951,-1.765532373));
#143143=CARTESIAN_POINT('Ctrl Pts',(6.926098167,4.430609079,-2.14281688));
#143144=CARTESIAN_POINT('Ctrl Pts',(6.92492764777796,4.43126318491329,-2.14660027888924));
#143145=CARTESIAN_POINT('Ctrl Pts',(6.92375712855592,4.43191729082659,-2.15038367777849));
#143146=CARTESIAN_POINT('',(7.23377285707386,4.43060908007274,-1.98053785761356));
#143147=CARTESIAN_POINT('',(7.07993551791367,4.43060908208281,-2.06167735440911));
#143148=CARTESIAN_POINT('',(7.36216470049487,4.34096089500721,-1.43126898997882));
#143149=CARTESIAN_POINT('Origin',(-0.174676265156352,4.5534907088828,0.0682025180186771));
#143150=CARTESIAN_POINT('Ctrl Pts',(7.11698472797653,4.30202682668443,-1.38239950366295));
#143151=CARTESIAN_POINT('Ctrl Pts',(7.15776689795272,4.30883434300015,-1.39064707707501));
#143152=CARTESIAN_POINT('Ctrl Pts',(7.19861354231777,4.3154777766733,-1.39884414345425));
#143153=CARTESIAN_POINT('Ctrl Pts',(7.28032730928822,4.32844539088522,-1.41512765746602));
#143154=CARTESIAN_POINT('Ctrl Pts',(7.32124226296971,4.33477715833814,-1.42322362860611));
#143155=CARTESIAN_POINT('Ctrl Pts',(7.36216470022103,4.34096089500162,-1.43126899106953));
#143156=CARTESIAN_POINT('Ctrl Pts',(7.45038229297625,4.43188407004787,-0.861318764735012));
#143157=CARTESIAN_POINT('Ctrl Pts',(7.44991020298812,4.43124657452393,-0.865363820867506));
#143158=CARTESIAN_POINT('Ctrl Pts',(7.449438113,4.430609079,-0.869408877000001));
#143159=CARTESIAN_POINT('Ctrl Pts',(7.448683485,4.429590053,-0.875874832));
#143160=CARTESIAN_POINT('Ctrl Pts',(7.447917633,4.428571429,-0.882339467));
#143161=CARTESIAN_POINT('Ctrl Pts',(7.400496141,4.365498301,-1.282629125));
#143162=CARTESIAN_POINT('Ctrl Pts',(7.310444469,4.301245526,-1.675530263));
#143163=CARTESIAN_POINT('Ctrl Pts',(7.22546787182032,4.43188407004787,-0.595966473717372));
#143164=CARTESIAN_POINT('Ctrl Pts',(7.22514000041016,4.43124657452393,-0.599889557358686));
#143165=CARTESIAN_POINT('Ctrl Pts',(7.224812129,4.430609079,-0.603812641));
#143166=CARTESIAN_POINT('Ctrl Pts',(7.224288032,4.429590053,-0.610083625));
#143167=CARTESIAN_POINT('Ctrl Pts',(7.22375305,4.428571429,-0.616353689));
#143168=CARTESIAN_POINT('Ctrl Pts',(7.190627011,4.365498301,-1.004595582));
#143169=CARTESIAN_POINT('Ctrl Pts',(7.116079733,4.301245526,-1.387050553));
#143170=CARTESIAN_POINT('',(7.44943810973751,4.43060908088848,-0.869408884644942));
#143171=CARTESIAN_POINT('Origin',(-0.172101497542194,4.16161689916212,0.0624998054184125));
#143172=CARTESIAN_POINT('',(7.33712511928294,4.43060908179128,-0.736610776103072));
#143173=CARTESIAN_POINT('Origin',(-2.99673480474993E-13,4.52171037000022,
6.90094682787024E-14));
#143174=CARTESIAN_POINT('',(7.36340679369017,4.52063234083055,-1.42486504209282));
#143175=CARTESIAN_POINT('Origin',(-0.183313845500021,4.69624335980962,0.00702306773572942));
#143176=CARTESIAN_POINT('Origin',(-0.1873408563391,4.55356370368071,0.041648395163872));
#143177=CARTESIAN_POINT('Ctrl Pts',(7.487275942,4.301266351,0.436690929));
#143178=CARTESIAN_POINT('Ctrl Pts',(7.511063754,4.365380951,0.028837453));
#143179=CARTESIAN_POINT('Ctrl Pts',(7.490408365,4.430609079,-0.379186656));
#143180=CARTESIAN_POINT('Ctrl Pts',(7.49020123331463,4.43126318491329,-0.383278310791366));
#143181=CARTESIAN_POINT('Ctrl Pts',(7.48999410162926,4.43191729082659,-0.387369965582731));
#143182=CARTESIAN_POINT('Ctrl Pts',(7.247650894,4.301266351,0.184544087));
#143183=CARTESIAN_POINT('Ctrl Pts',(7.257703542,4.365380951,-0.210256324));
#143184=CARTESIAN_POINT('Ctrl Pts',(7.224812129,4.430609079,-0.603812641));
#143185=CARTESIAN_POINT('Ctrl Pts',(7.22448229479504,4.43126318491329,-0.607759213162297));
#143186=CARTESIAN_POINT('Ctrl Pts',(7.22415246059009,4.43191729082659,-0.611705785324594));
#143187=CARTESIAN_POINT('',(7.35761024829061,4.43060908208281,-0.491499629179973));
#143188=CARTESIAN_POINT('Ctrl Pts',(7.24776860954439,4.30202682668585,0.179861568603662));
#143189=CARTESIAN_POINT('Ctrl Pts',(7.2893702940003,4.30883434207202,0.180573779782587));
#143190=CARTESIAN_POINT('Ctrl Pts',(7.33102408727948,4.31547777481083,0.181349177265882));
#143191=CARTESIAN_POINT('Ctrl Pts',(7.41432788288339,4.32844538541458,0.183012406880999));
#143192=CARTESIAN_POINT('Ctrl Pts',(7.45602662296787,4.33477714731221,0.183901219773324));
#143193=CARTESIAN_POINT('Ctrl Pts',(7.49772190592654,4.34096089501742,0.184841069557451));
#143194=CARTESIAN_POINT('Ctrl Pts',(7.46135457079931,4.43188407004788,0.760430350372509));
#143195=CARTESIAN_POINT('Ctrl Pts',(7.46176308489966,4.43124657452394,0.756378380186254));
#143196=CARTESIAN_POINT('Ctrl Pts',(7.462171599,4.430609079,0.75232641));
#143197=CARTESIAN_POINT('Ctrl Pts',(7.46282460200001,4.429590053,0.745849403));
#143198=CARTESIAN_POINT('Ctrl Pts',(7.463466361,4.428571429,0.739371272));
#143199=CARTESIAN_POINT('Ctrl Pts',(7.503204002,4.365498301,0.338245945));
#143200=CARTESIAN_POINT('Ctrl Pts',(7.499719818,4.301245526,-0.064827831));
#143201=CARTESIAN_POINT('Ctrl Pts',(7.18465562199158,4.43188407004788,0.971228900272083));
#143202=CARTESIAN_POINT('Ctrl Pts',(7.1851787634958,4.43124657452394,0.967327053636041));
#143203=CARTESIAN_POINT('Ctrl Pts',(7.18570190500001,4.430609079,0.963425207));
#143204=CARTESIAN_POINT('Ctrl Pts',(7.186538138,4.429590053,0.95718817));
#143205=CARTESIAN_POINT('Ctrl Pts',(7.187363542,4.428571429,0.95094969));
#143206=CARTESIAN_POINT('Ctrl Pts',(7.238472502,4.365498301,0.564663559));
#143207=CARTESIAN_POINT('Ctrl Pts',(7.247884611,4.301245526,0.175124711));
#143208=CARTESIAN_POINT('',(7.32393675399974,4.43060908179128,0.857875791427671));
#143209=CARTESIAN_POINT('Ctrl Pts',(7.21835195,4.301266351,2.036024343));
#143210=CARTESIAN_POINT('Ctrl Pts',(7.329260058,4.365380951,1.642819931));
#143211=CARTESIAN_POINT('Ctrl Pts',(7.396800703,4.430609079,1.239894901));
#143212=CARTESIAN_POINT('Ctrl Pts',(7.39747799877158,4.43126318491329,1.23585437963571));
#143213=CARTESIAN_POINT('Ctrl Pts',(7.39815529454315,4.43191729082659,1.23181385827142));
#143214=CARTESIAN_POINT('Ctrl Pts',(7.03853332,4.301266351,1.738260252));
#143215=CARTESIAN_POINT('Ctrl Pts',(7.13322136,4.365380951,1.354851078));
#143216=CARTESIAN_POINT('Ctrl Pts',(7.185701905,4.430609079,0.963425207));
#143217=CARTESIAN_POINT('Ctrl Pts',(7.18622817849381,4.43126318491329,0.959499998892894));
#143218=CARTESIAN_POINT('Ctrl Pts',(7.18675445198762,4.43191729082659,0.955574790785788));
#143219=CARTESIAN_POINT('',(7.39680069863646,4.43060908007275,1.23989490820429));
#143220=CARTESIAN_POINT('',(7.29125130110721,4.43060908208281,1.10166007314573));
#143221=CARTESIAN_POINT('',(7.28269396809365,4.340960895,1.79230816784698));
#143222=CARTESIAN_POINT('Origin',(-0.187169460194456,4.55349066545353,-0.0114457567602202));
#143223=CARTESIAN_POINT('Ctrl Pts',(7.03965488667234,4.30202682673479,1.73371251360448));
#143224=CARTESIAN_POINT('Ctrl Pts',(7.08013084537838,4.30883434259959,1.74335120698511));
#143225=CARTESIAN_POINT('Ctrl Pts',(7.12064411130631,4.3154777757409,1.75306281112323));
#143226=CARTESIAN_POINT('Ctrl Pts',(7.2016427944238,4.32844539098669,1.77259501597001));
#143227=CARTESIAN_POINT('Ctrl Pts',(7.24217561132369,4.33477715851113,1.78242705484932));
#143228=CARTESIAN_POINT('Ctrl Pts',(7.28269396836801,4.34096089499022,1.79230816672803));
#143229=CARTESIAN_POINT('Ctrl Pts',(7.12344219883282,4.43188407004788,2.34662258804663));
#143230=CARTESIAN_POINT('Ctrl Pts',(7.12471221641641,4.43124657452394,2.34275316902332));
#143231=CARTESIAN_POINT('Ctrl Pts',(7.125982234,4.430609079,2.33888375));
#143232=CARTESIAN_POINT('Ctrl Pts',(7.128012336,4.429590053,2.332698548));
#143233=CARTESIAN_POINT('Ctrl Pts',(7.130031697,4.428571429,2.326509831));
#143234=CARTESIAN_POINT('Ctrl Pts',(7.255070382,4.365498301,1.94330501));
#143235=CARTESIAN_POINT('Ctrl Pts',(7.338316604,4.301245526,1.548905879));
#143236=CARTESIAN_POINT('Ctrl Pts',(6.80789686203716,4.43188407004788,2.49301069013488));
#143237=CARTESIAN_POINT('Ctrl Pts',(6.80924655451859,4.43124657452394,2.48931252656744));
#143238=CARTESIAN_POINT('Ctrl Pts',(6.810596247,4.430609079,2.485614363));
#143239=CARTESIAN_POINT('Ctrl Pts',(6.81275370800001,4.429590053,2.47970291));
#143240=CARTESIAN_POINT('Ctrl Pts',(6.814900903,4.428571429,2.47378772));
#143241=CARTESIAN_POINT('Ctrl Pts',(6.947855064,4.365498301,2.107519659));
#143242=CARTESIAN_POINT('Ctrl Pts',(7.04078646,4.301245526,1.729111338));
#143243=CARTESIAN_POINT('',(7.12598223423435,4.43060908088847,2.33888374169329));
#143244=CARTESIAN_POINT('Origin',(-0.182438076329164,4.16161690204204,-0.0155402565911994));
#143245=CARTESIAN_POINT('',(6.96828924612303,4.43060908179128,2.4122490402567));
#143246=CARTESIAN_POINT('Origin',(-3.29163779566599E-13,4.52171036999978,
-1.60245081093358E-13));
#143247=CARTESIAN_POINT('',(7.28113231366844,4.52063234086887,1.79864177448102));
#143248=CARTESIAN_POINT('Origin',(-0.169320101021773,4.69624337824747,-0.0705975350664123));
#143249=CARTESIAN_POINT('Origin',(-0.18751371703438,4.55356369516498,-0.0408633449075055));
#143250=CARTESIAN_POINT('Ctrl Pts',(6.611905843,4.301266351,3.540155522));
#143251=CARTESIAN_POINT('Ctrl Pts',(6.804748307,4.365380951,3.179985975));
#143252=CARTESIAN_POINT('Ctrl Pts',(6.95732686,4.430609079,2.80100035));
#143253=CARTESIAN_POINT('Ctrl Pts',(6.95885691362593,4.43126318491329,2.79719989234521));
#143254=CARTESIAN_POINT('Ctrl Pts',(6.96038696725186,4.43191729082659,2.79339943469041));
#143255=CARTESIAN_POINT('Ctrl Pts',(6.500301751,4.301266351,3.210697299));
#143256=CARTESIAN_POINT('Ctrl Pts',(6.675197676,4.365380951,2.856607148));
#143257=CARTESIAN_POINT('Ctrl Pts',(6.810596247,4.430609079,2.485614363));
#143258=CARTESIAN_POINT('Ctrl Pts',(6.81195402022849,4.43126318491329,2.48189405732976));
#143259=CARTESIAN_POINT('Ctrl Pts',(6.81331179345697,4.43191729082659,2.47817375165952));
#143260=CARTESIAN_POINT('',(6.95732685418665,4.43060908007271,2.8010003561233));
#143261=CARTESIAN_POINT('',(6.88396154655906,4.43060908208281,2.6433073745763));
#143262=CARTESIAN_POINT('',(6.7271353543509,4.34096089503984,3.3159689269679));
#143263=CARTESIAN_POINT('Origin',(-0.180332952993478,4.55349066696634,-0.0514140168539484));
#143264=CARTESIAN_POINT('Ctrl Pts',(6.50237472517852,4.30202682664099,3.20649698852999));
#143265=CARTESIAN_POINT('Ctrl Pts',(6.53983233913287,4.30883434160489,3.22461146676558));
#143266=CARTESIAN_POINT('Ctrl Pts',(6.57731071430891,4.31547777390474,3.24280517099429));
#143267=CARTESIAN_POINT('Ctrl Pts',(6.65221682469093,4.32844538541513,3.27929303563529));
#143268=CARTESIAN_POINT('Ctrl Pts',(6.68968837343744,4.33477714732117,3.29760854678755));
#143269=CARTESIAN_POINT('Ctrl Pts',(6.72713535476946,4.34096089503156,3.315968926117));
#143270=CARTESIAN_POINT('Ctrl Pts',(6.45244558794698,4.43188407004788,3.82308936021777));
#143271=CARTESIAN_POINT('Ctrl Pts',(6.45451772397349,4.43124657452394,3.81958342260888));
#143272=CARTESIAN_POINT('Ctrl Pts',(6.45658986000001,4.430609079,3.816077485));
#143273=CARTESIAN_POINT('Ctrl Pts',(6.459902135,4.429590053,3.810473302));
#143274=CARTESIAN_POINT('Ctrl Pts',(6.463204676,4.428571429,3.804863377));
#143275=CARTESIAN_POINT('Ctrl Pts',(6.667697735,4.365498301,3.457497292));
#143276=CARTESIAN_POINT('Ctrl Pts',(6.833781861,4.301245526,3.090214471));
#143277=CARTESIAN_POINT('Ctrl Pts',(6.11280841197593,4.43188407004788,3.89822207217764));
#143278=CARTESIAN_POINT('Ctrl Pts',(6.11492154498796,4.43124657452394,3.89490051308882));
#143279=CARTESIAN_POINT('Ctrl Pts',(6.117034678,4.430609079,3.891578954));
#143280=CARTESIAN_POINT('Ctrl Pts',(6.120412486,4.429590053,3.886269497));
#143281=CARTESIAN_POINT('Ctrl Pts',(6.123781072,4.428571429,3.880954185));
#143282=CARTESIAN_POINT('Ctrl Pts',(6.332363645,4.365498301,3.551830482));
#143283=CARTESIAN_POINT('Ctrl Pts',(6.50446896,4.301245526,3.202246641));
#143284=CARTESIAN_POINT('',(6.45658986212607,4.43060908088851,3.81607747694991));
#143285=CARTESIAN_POINT('Origin',(-0.174832079332926,4.16161692141043,-0.0543957308709359));
#143286=CARTESIAN_POINT('',(6.2868122779834,4.43060908179128,3.85382820484524));
#143287=CARTESIAN_POINT('Origin',(1.20519913493489E-12,4.52171036999911,
5.35595873207839E-13));
#143288=CARTESIAN_POINT('',(6.72424867213751,4.52063234084617,3.32181874799288));
#143289=CARTESIAN_POINT('Origin',(-0.150185083091728,4.69624336268068,-0.105345803530265));
#143290=CARTESIAN_POINT('Origin',(-0.174345382848101,4.55356368596386,-0.0802179147523208));
#143291=CARTESIAN_POINT('Ctrl Pts',(5.696294368,4.301266351,4.878752963));
#143292=CARTESIAN_POINT('Ctrl Pts',(5.962054088,4.365380951,4.568459409));
#143293=CARTESIAN_POINT('Ctrl Pts',(6.192536146,4.430609079,4.231134137));
#143294=CARTESIAN_POINT('Ctrl Pts',(6.19484741387888,4.43126318491329,4.22775144824465));
#143295=CARTESIAN_POINT('Ctrl Pts',(6.19715868175776,4.43191729082659,4.22436875948929));
#143296=CARTESIAN_POINT('Ctrl Pts',(5.658123296,4.301266351,4.53300571));
#143297=CARTESIAN_POINT('Ctrl Pts',(5.905049168,4.365380951,4.224791444));
#143298=CARTESIAN_POINT('Ctrl Pts',(6.117034678,4.430609079,3.891578954));
#143299=CARTESIAN_POINT('Ctrl Pts',(6.11916046299299,4.43126318491329,3.88823750811193));
#143300=CARTESIAN_POINT('Ctrl Pts',(6.12128624798599,4.43191729082659,3.88489606222386));
#143301=CARTESIAN_POINT('',(6.19253613901402,4.43060908007276,4.23113414170784));
#143302=CARTESIAN_POINT('',(6.15478540133549,4.43060908208281,4.06135656166154));
#143303=CARTESIAN_POINT('',(5.85702336818681,4.34096089503826,4.68457866470363));
#143304=CARTESIAN_POINT('Origin',(-0.165064523379462,4.55349069367169,-0.0889783509120712));
#143305=CARTESIAN_POINT('Ctrl Pts',(5.66105074783569,4.30202682668129,4.52934922739746));
#143306=CARTESIAN_POINT('Ctrl Pts',(5.69373871051027,4.30883437580268,4.55509260828656));
#143307=CARTESIAN_POINT('Ctrl Pts',(5.72642993561914,4.31547784263449,4.58091784164831));
#143308=CARTESIAN_POINT('Ctrl Pts',(5.79174062469475,4.32844538544317,4.63265496595597));
#143309=CARTESIAN_POINT('Ctrl Pts',(5.8243988159226,4.33477714732765,4.65859754598103));
#143310=CARTESIAN_POINT('Ctrl Pts',(5.8570233687867,4.3409608950263,4.6845786639532));
#143311=CARTESIAN_POINT('Ctrl Pts',(5.47973979224387,4.43188407004788,5.12079272560908));
#143312=CARTESIAN_POINT('Ctrl Pts',(5.48251715612193,4.43124657452394,5.11781420230454));
#143313=CARTESIAN_POINT('Ctrl Pts',(5.48529452,4.430609079,5.11483567900001));
#143314=CARTESIAN_POINT('Ctrl Pts',(5.48973409,4.429590053,5.110074559));
#143315=CARTESIAN_POINT('Ctrl Pts',(5.494165387,4.428571429,5.10530574));
#143316=CARTESIAN_POINT('Ctrl Pts',(5.768550952,4.365498301,4.810020844));
#143317=CARTESIAN_POINT('Ctrl Pts',(6.009707074,4.301245526,4.487028069));
#143318=CARTESIAN_POINT('Ctrl Pts',(5.13189183273128,4.43188407004788,5.12115692153224));
#143319=CARTESIAN_POINT('Ctrl Pts',(5.13466959886564,4.43124657452394,5.11836727976612));
#143320=CARTESIAN_POINT('Ctrl Pts',(5.137447365,4.430609079,5.11557763800001));
#143321=CARTESIAN_POINT('Ctrl Pts',(5.141887578,4.429590053,5.111118442));
#143322=CARTESIAN_POINT('Ctrl Pts',(5.146320044,4.428571429,5.106651545));
#143323=CARTESIAN_POINT('Ctrl Pts',(5.42077793999999,4.365498301,4.830061659));
#143324=CARTESIAN_POINT('Ctrl Pts',(5.66400972,4.301245526,4.525648449));
#143325=CARTESIAN_POINT('',(5.48529452372975,4.43060908088849,5.11483567156938));
#143326=CARTESIAN_POINT('Origin',(-0.159051130077427,4.16161688519082,-0.0907077120393646));
#143327=CARTESIAN_POINT('',(5.31137095442371,4.43060908179128,5.11520664611903));
#143328=CARTESIAN_POINT('Origin',(7.09501901674514E-13,4.52171036999911,
6.53557069574262E-13));
#143329=CARTESIAN_POINT('',(5.85294663643186,4.52063234086129,4.68967116858934));
#143330=CARTESIAN_POINT('Origin',(-0.124027660144729,4.69624335798661,-0.135168275660474));
#143331=CARTESIAN_POINT('Origin',(-0.15302475186547,4.55356366957091,-0.115821519450654));
#143332=CARTESIAN_POINT('Ctrl Pts',(4.514330499,4.30126635099999,5.989225338));
#143333=CARTESIAN_POINT('Ctrl Pts',(4.840580846,4.365380951,5.743316758));
#143334=CARTESIAN_POINT('Ctrl Pts',(5.138189324,4.43060907900001,5.463424793));
#143335=CARTESIAN_POINT('Ctrl Pts',(5.1411737338133,4.43126318491329,5.4606180439026));
#143336=CARTESIAN_POINT('Ctrl Pts',(5.14415814362659,4.43191729082658,5.45781129480519));
#143337=CARTESIAN_POINT('Ctrl Pts',(4.551377285,4.30126635099999,5.643355811));
#143338=CARTESIAN_POINT('Ctrl Pts',(4.858787124,4.365380951,5.39542918700001));
#143339=CARTESIAN_POINT('Ctrl Pts',(5.13744736500001,4.43060907900001,5.115577638));
#143340=CARTESIAN_POINT('Ctrl Pts',(5.14024176240226,4.43126318491329,5.11277129419316));
#143341=CARTESIAN_POINT('Ctrl Pts',(5.14303615980453,4.43191729082658,5.1099649503863));
#143342=CARTESIAN_POINT('',(5.13818931615188,4.43060908007285,5.46342479611677));
#143343=CARTESIAN_POINT('',(5.13781833060832,4.4306090820833,5.28950122899332));
#143344=CARTESIAN_POINT('',(4.71304347885007,4.34096089504838,5.83414271038548));
#143345=CARTESIAN_POINT('Origin',(-0.142077824150623,4.55349070797828,-0.122382224788236));
#143346=CARTESIAN_POINT('Ctrl Pts',(4.55502233006115,4.30202682664792,5.64041413156312));
#143347=CARTESIAN_POINT('Ctrl Pts',(4.58141200045756,4.30883437577953,5.67258259200198));
#143348=CARTESIAN_POINT('Ctrl Pts',(4.60778726118877,4.31547784264405,5.70483169273335));
#143349=CARTESIAN_POINT('Ctrl Pts',(4.66044906993919,4.3284453854127,5.76939909879075));
#143350=CARTESIAN_POINT('Ctrl Pts',(4.68676684300026,4.33477714733193,5.80175570146899));
#143351=CARTESIAN_POINT('Ctrl Pts',(4.71304347955343,4.34096089504684,5.83414270979538));
#143352=CARTESIAN_POINT('Ctrl Pts',(4.25080745523902,4.43188407004788,6.17905351246968));
#143353=CARTESIAN_POINT('Ctrl Pts',(4.25416018011951,4.43124657452394,6.17674167673485));
#143354=CARTESIAN_POINT('Ctrl Pts',(4.257512905,4.430609079,6.174429841));
#143355=CARTESIAN_POINT('Ctrl Pts',(4.26287218,4.429590053,6.17073441));
#143356=CARTESIAN_POINT('Ctrl Pts',(4.268225031,4.428571429,6.167029681));
#143357=CARTESIAN_POINT('Ctrl Pts',(4.599673138,4.365498301,5.937633167));
#143358=CARTESIAN_POINT('Ctrl Pts',(4.904625063,4.301245526,5.674033221));
#143359=CARTESIAN_POINT('Ctrl Pts',(3.91101369546929,4.43188407004788,6.10463216359984));
#143360=CARTESIAN_POINT('Ctrl Pts',(3.91432620973464,4.43124657452394,6.10250488029992));
#143361=CARTESIAN_POINT('Ctrl Pts',(3.917638724,4.430609079,6.100377597));
#143362=CARTESIAN_POINT('Ctrl Pts',(3.922933723,4.429590053,6.09697717));
#143363=CARTESIAN_POINT('Ctrl Pts',(3.928222811,4.428571429,6.093567555));
#143364=CARTESIAN_POINT('Ctrl Pts',(4.255722683,4.365498301,5.882444522));
#143365=CARTESIAN_POINT('Ctrl Pts',(4.558707681,4.301245526,5.637435967));
#143366=CARTESIAN_POINT('',(4.25751291014934,4.43060908088846,6.17442983449011));
#143367=CARTESIAN_POINT('Origin',(-0.135833122815991,4.16161692292354,-0.122778312928644));
#143368=CARTESIAN_POINT('',(4.08757582880652,4.43060908179129,6.13740370947171));
#143369=CARTESIAN_POINT('Origin',(3.38704758684472E-13,4.52171036999933,
4.64038529823796E-13));
#143370=CARTESIAN_POINT('',(4.70796732118483,4.5206323408538,5.8382397777685));
#143371=CARTESIAN_POINT('Origin',(-0.0920707914317653,4.69624335804417,
-0.158670405151131));
#143372=CARTESIAN_POINT('Origin',(-0.124548980264571,4.55356367804712,-0.146009561469306));
#143373=CARTESIAN_POINT('Ctrl Pts',(3.121281553,4.301266351,6.819648192));
#143374=CARTESIAN_POINT('Ctrl Pts',(3.492767424,4.365380951,6.649623));
#143375=CARTESIAN_POINT('Ctrl Pts',(3.84358648,4.430609079,6.440251778));
#143376=CARTESIAN_POINT('Ctrl Pts',(3.84710448405839,4.43126318491329,6.43815220901676));
#143377=CARTESIAN_POINT('Ctrl Pts',(3.85062248811679,4.43191729082659,6.43605264003352));
#143378=CARTESIAN_POINT('Ctrl Pts',(3.231813931,4.301266351,6.489828867));
#143379=CARTESIAN_POINT('Ctrl Pts',(3.585333593,4.365380951,6.313782657));
#143380=CARTESIAN_POINT('Ctrl Pts',(3.917638724,4.430609079,6.100377597));
#143381=CARTESIAN_POINT('Ctrl Pts',(3.92097107091642,4.43126318491329,6.09823757679779));
#143382=CARTESIAN_POINT('Ctrl Pts',(3.92430341783284,4.43191729082659,6.09609755659558));
#143383=CARTESIAN_POINT('',(3.84358647165648,4.43060908007268,6.44025177936701));
#143384=CARTESIAN_POINT('',(3.88061258553502,4.43060908208283,6.27031469768996));
#143385=CARTESIAN_POINT('',(3.34868691448851,4.34096089503725,6.71090872740062));
#143386=CARTESIAN_POINT('Origin',(-0.112447375425123,4.5534906635389,-0.150063190805616));
#143387=CARTESIAN_POINT('Ctrl Pts',(3.23600613130859,4.30202682662047,6.48773953814593));
#143388=CARTESIAN_POINT('Ctrl Pts',(3.25486355746509,4.30883437577991,6.524828917158));
#143389=CARTESIAN_POINT('Ctrl Pts',(3.27368957563181,4.3154778426473,6.561993953406));
#143390=CARTESIAN_POINT('Ctrl Pts',(3.31124009666575,4.32844538546329,6.63637254221788));
#143391=CARTESIAN_POINT('Ctrl Pts',(3.32998686152247,4.33477714735077,6.67363020876695));
#143392=CARTESIAN_POINT('Ctrl Pts',(3.34868691534333,4.34096089503295,6.71090872692928));
#143393=CARTESIAN_POINT('Ctrl Pts',(2.8231120869345,4.43188407004788,6.94838862489945));
#143394=CARTESIAN_POINT('Ctrl Pts',(2.82688340296725,4.43124657452394,6.94685157544973));
#143395=CARTESIAN_POINT('Ctrl Pts',(2.830654719,4.430609079,6.945314526));
#143396=CARTESIAN_POINT('Ctrl Pts',(2.836683105,4.429590053,6.942857578));
#143397=CARTESIAN_POINT('Ctrl Pts',(2.842707217,4.428571429,6.940390168));
#143398=CARTESIAN_POINT('Ctrl Pts',(3.21571972,4.365498301,6.787608363));
#143399=CARTESIAN_POINT('Ctrl Pts',(3.570208235,4.301245526,6.595726886));
#143400=CARTESIAN_POINT('Ctrl Pts',(2.50726090509375,4.43188407004788,6.80266159234725));
#143401=CARTESIAN_POINT('Ctrl Pts',(2.51095327754687,4.43124657452394,6.80129613617363));
#143402=CARTESIAN_POINT('Ctrl Pts',(2.51464565,4.430609079,6.79993068000001));
#143403=CARTESIAN_POINT('Ctrl Pts',(2.520547846,4.429590053,6.797748021));
#143404=CARTESIAN_POINT('Ctrl Pts',(2.526446244,4.428571429,6.795555119));
#143405=CARTESIAN_POINT('Ctrl Pts',(2.891674563,4.365498301,6.659770816));
#143406=CARTESIAN_POINT('Ctrl Pts',(3.240245538,4.301245526,6.485623243));
#143407=CARTESIAN_POINT('',(2.83065472529914,4.4306090808884,6.94531452062695));
#143408=CARTESIAN_POINT('Origin',(-0.106263705412877,4.16161698010819,-0.149107937770643));
#143409=CARTESIAN_POINT('',(2.67265020052035,4.43060908179129,6.87262259676995));
#143410=CARTESIAN_POINT('Origin',(1.00830802041152E-13,4.52171037000067,
1.05384451165591E-13));
#143411=CARTESIAN_POINT('',(3.34284868628253,4.52063234082776,6.71381878362209));
#143412=CARTESIAN_POINT('Origin',(-0.0558087578785244,4.69624333376681,
-0.174753222616125));
#143413=CARTESIAN_POINT('Origin',(-0.0902493206332439,4.55356364651545,
-0.1693702105606));
#143414=CARTESIAN_POINT('Ctrl Pts',(1.582284951,4.301266351,7.331191877));
#143415=CARTESIAN_POINT('Ctrl Pts',(1.981636079,4.365380951,7.24500026));
#143416=CARTESIAN_POINT('Ctrl Pts',(2.369261804,4.430609079,7.115939748));
#143417=CARTESIAN_POINT('Ctrl Pts',(2.37314890434522,4.43126318491329,7.1146455326567));
#143418=CARTESIAN_POINT('Ctrl Pts',(2.37703600469045,4.43191729082659,7.11335131731341));
#143419=CARTESIAN_POINT('Ctrl Pts',(1.761134548,4.301266351,7.032844738));
#143420=CARTESIAN_POINT('Ctrl Pts',(2.144233849,4.365380951,6.936910668));
#143421=CARTESIAN_POINT('Ctrl Pts',(2.51464565,4.430609079,6.79993068));
#143422=CARTESIAN_POINT('Ctrl Pts',(2.51836012957832,4.43126318491329,6.79855704836437));
#143423=CARTESIAN_POINT('Ctrl Pts',(2.52207460915663,4.43191729082659,6.79718341672875));
#143424=CARTESIAN_POINT('',(2.36926179550939,4.43060908007261,7.11593974757192));
#143425=CARTESIAN_POINT('',(2.44195370872942,4.43060908208283,6.95793522041224));
#143426=CARTESIAN_POINT('',(1.82774947215013,4.34096089505207,7.27388011084953));
#143427=CARTESIAN_POINT('Origin',(-0.0775593168197178,4.55349067875258,
-0.170727809510166));
#143428=CARTESIAN_POINT('Ctrl Pts',(1.76567788092872,4.30202682669698,7.0317054563247));
#143429=CARTESIAN_POINT('Ctrl Pts',(1.77612131104473,4.30883437583179,7.07198149539299));
#143430=CARTESIAN_POINT('Ctrl Pts',(1.7865178033652,4.31547784268845,7.11232467109287));
#143431=CARTESIAN_POINT('Ctrl Pts',(1.80720122363574,4.32844539001279,7.19303660981282));
#143432=CARTESIAN_POINT('Ctrl Pts',(1.81750041065261,4.33477715653016,7.23345324471115));
#143433=CARTESIAN_POINT('Ctrl Pts',(1.82774947305039,4.34096089504731,7.27388011060104));
#143434=CARTESIAN_POINT('Ctrl Pts',(1.26341113293498,4.43188407004788,7.39282480932989));
#143435=CARTESIAN_POINT('Ctrl Pts',(1.26742469796749,4.43124657452394,7.39213441616495));
#143436=CARTESIAN_POINT('Ctrl Pts',(1.271438263,4.430609079,7.391444023));
#143437=CARTESIAN_POINT('Ctrl Pts',(1.27785388,4.429590053,7.39034044099999));
#143438=CARTESIAN_POINT('Ctrl Pts',(1.284267572,4.428571429,7.389225724));
#143439=CARTESIAN_POINT('Ctrl Pts',(1.681402823,4.365498301,7.320202535));
#143440=CARTESIAN_POINT('Ctrl Pts',(2.068852438,4.301245526,7.209011693));
#143441=CARTESIAN_POINT('Ctrl Pts',(0.986271382025895,4.43188407004788,
7.18260612530439));
#143442=CARTESIAN_POINT('Ctrl Pts',(0.990170961512947,4.43124657452394,
7.18206634365219));
#143443=CARTESIAN_POINT('Ctrl Pts',(0.994070541000001,4.430609079,7.18152656200001));
#143444=CARTESIAN_POINT('Ctrl Pts',(1.000303954,4.429590053,7.18066373));
#143445=CARTESIAN_POINT('Ctrl Pts',(1.00653586,4.428571429,7.179790078));
#143446=CARTESIAN_POINT('Ctrl Pts',(1.392414954,4.365498301,7.125693629));
#143447=CARTESIAN_POINT('Ctrl Pts',(1.770273114,4.301245526,7.030549986));
#143448=CARTESIAN_POINT('',(1.27143827033362,4.43060908088841,7.39144401914613));
#143449=CARTESIAN_POINT('Origin',(-0.0717255340483477,4.16161688001676,
-0.168465422945171));
#143450=CARTESIAN_POINT('',(1.13275441898507,4.43060908179129,7.28648528985951));
#143451=CARTESIAN_POINT('Origin',(-6.66784336078585E-13,4.52171037000022,
-2.37527011948124E-12));
#143452=CARTESIAN_POINT('',(1.82142216213809,4.5206323408504,7.2754670852764));
#143453=CARTESIAN_POINT('Origin',(-0.0169371445773164,4.69624335525984,
-0.182664612581106));
#143454=CARTESIAN_POINT('Origin',(-0.0517297821939336,4.55356365816114,
-0.184811503839296));
#143455=CARTESIAN_POINT('Ctrl Pts',(-0.030697537,4.301266351,7.499937177));
#143456=CARTESIAN_POINT('Ctrl Pts',(0.377845634,4.365380951,7.50160936));
#143457=CARTESIAN_POINT('Ctrl Pts',(0.784153080000001,4.430609079,7.458894285));
#143458=CARTESIAN_POINT('Ctrl Pts',(0.788227520140971,4.43126318491329,
7.45846593937671));
#143459=CARTESIAN_POINT('Ctrl Pts',(0.792301960281942,4.43191729082659,
7.45803759375342));
#143460=CARTESIAN_POINT('Ctrl Pts',(0.208106472,4.301266351,7.247012605));
#143461=CARTESIAN_POINT('Ctrl Pts',(0.602872113,4.365380951,7.235676446));
#143462=CARTESIAN_POINT('Ctrl Pts',(0.994070541,4.430609079,7.181526562));
#143463=CARTESIAN_POINT('Ctrl Pts',(0.99799346831482,4.43126318491329,7.1809835484196));
#143464=CARTESIAN_POINT('Ctrl Pts',(1.00191639562964,4.43191729082659,7.18044053483919));
#143465=CARTESIAN_POINT('',(0.784153071844491,4.43060908007267,7.45889428273967));
#143466=CARTESIAN_POINT('',(0.88911179127818,4.43060908208281,7.32021042583468));
#143467=CARTESIAN_POINT('',(0.221348495881175,4.34096089505548,7.49673294460434));
#143468=CARTESIAN_POINT('Origin',(-0.0390445919689369,4.55349070825684,
-0.183409434825865));
#143469=CARTESIAN_POINT('Ctrl Pts',(0.21278849589644,4.30202682676222,7.24687664212485));
#143470=CARTESIAN_POINT('Ctrl Pts',(0.214329606545709,4.30883437589522,
7.28845607848061));
#143471=CARTESIAN_POINT('Ctrl Pts',(0.215810444399962,4.31547784270417,
7.33009099135692));
#143472=CARTESIAN_POINT('Ctrl Pts',(0.218659615826445,4.32844538543538,
7.41336222423957));
#143473=CARTESIAN_POINT('Ctrl Pts',(0.220029630859861,4.33477714733755,
7.4550479288828));
#143474=CARTESIAN_POINT('Ctrl Pts',(0.221348496731302,4.34096089504884,
7.49673294457843));
#143475=CARTESIAN_POINT('Ctrl Pts',(-0.355365520534916,4.43188407004788,
7.49158071955885));
#143476=CARTESIAN_POINT('Ctrl Pts',(-0.351297376267458,4.43124657452394,
7.49176926577943));
#143477=CARTESIAN_POINT('Ctrl Pts',(-0.347229232,4.430609079,7.491957812));
#143478=CARTESIAN_POINT('Ctrl Pts',(-0.340726371,4.429590053,7.4922592));
#143479=CARTESIAN_POINT('Ctrl Pts',(-0.334222997,4.428571429,7.492549298));
#143480=CARTESIAN_POINT('Ctrl Pts',(0.0684653979999999,4.365498301,7.510512173));
#143481=CARTESIAN_POINT('Ctrl Pts',(0.470759401,4.301245526,7.485211125));
#143482=CARTESIAN_POINT('Ctrl Pts',(-0.580835096616911,4.43188407004788,
7.22669998041423));
#143483=CARTESIAN_POINT('Ctrl Pts',(-0.576910649808455,4.43124657452394,
7.22701111220711));
#143484=CARTESIAN_POINT('Ctrl Pts',(-0.572986203,4.430609079,7.227322244));
#143485=CARTESIAN_POINT('Ctrl Pts',(-0.56671304,4.429590053,7.227819583));
#143486=CARTESIAN_POINT('Ctrl Pts',(-0.560439023,4.428571429,7.228306033));
#143487=CARTESIAN_POINT('Ctrl Pts',(-0.17195243,4.365498301,7.258426928));
#143488=CARTESIAN_POINT('Ctrl Pts',(0.217524687,4.301245526,7.246736025));
#143489=CARTESIAN_POINT('',(-0.347229223945432,4.43060908088847,7.49195780997297));
#143490=CARTESIAN_POINT('Origin',(-0.033833535587145,4.16161693833491,-0.179945668173186));
#143491=CARTESIAN_POINT('',(-0.460107700344399,4.43060908179129,7.35964002907253));
#143492=CARTESIAN_POINT('Origin',(-7.78999260930835E-14,4.52171037,-6.21464685268691E-13));
#143493=CARTESIAN_POINT('',(0.214827962322351,4.52063234084998,7.49692263181169));
#143494=CARTESIAN_POINT('Origin',(0.0227263342201872,4.69624336296937,-0.182035181962907));
#143495=CARTESIAN_POINT('Origin',(-0.0107913587415697,4.5535636867977,-0.191610899041212));
#143496=CARTESIAN_POINT('Ctrl Pts',(0.459222278,1.457192641,7.485927791));
#143497=CARTESIAN_POINT('Ctrl Pts',(0.867908719,1.391489877,7.460857029));
#143498=CARTESIAN_POINT('Ctrl Pts',(1.271436929,1.326325889,7.39144425200001));
#143499=CARTESIAN_POINT('Ctrl Pts',(0.206355414,1.457192641,7.247062677));
#143500=CARTESIAN_POINT('Ctrl Pts',(0.602001262,1.391489877,7.235796918));
#143501=CARTESIAN_POINT('Ctrl Pts',(0.994069244,1.326325889,7.181526741));
#143502=CARTESIAN_POINT('',(0.989408722995935,1.327100493755,7.18217031262266));
#143503=CARTESIAN_POINT('Origin',(-0.00146137519289088,1.48213100741133,
-0.19802956343801));
#143504=CARTESIAN_POINT('Ctrl Pts',(1.02275296161726,1.36645689999221,7.42993784454118));
#143505=CARTESIAN_POINT('Ctrl Pts',(1.01715038410679,1.3602037253843,7.38860919103333));
#143506=CARTESIAN_POINT('Ctrl Pts',(1.01156636885775,1.35380222444785,7.34727742039455));
#143507=CARTESIAN_POINT('Ctrl Pts',(1.00045203418451,1.3406937976234,7.26470168845419));
#143508=CARTESIAN_POINT('Ctrl Pts',(0.99491552916717,1.33397958626036,7.22341179540039));
#143509=CARTESIAN_POINT('Ctrl Pts',(0.989408718103665,1.32710049397599,
7.18217031323905));
#143510=CARTESIAN_POINT('Ctrl Pts',(0.774029191421309,1.326318298,7.4604791102964));
#143511=CARTESIAN_POINT('Ctrl Pts',(1.18058200259849,1.391911284,7.41829901202036));
#143512=CARTESIAN_POINT('Ctrl Pts',(1.58014381986716,1.457192641,7.33219034515019));
#143513=CARTESIAN_POINT('Ctrl Pts',(1.59395607906417,1.45944932065418,7.32921369629509));
#143514=CARTESIAN_POINT('Ctrl Pts',(1.60776833826125,1.46170600030836,7.32623704743983));
#143515=CARTESIAN_POINT('Ctrl Pts',(0.984741244,1.326318298,7.182811753));
#143516=CARTESIAN_POINT('Ctrl Pts',(1.376162796,1.391911284,7.129149071));
#143517=CARTESIAN_POINT('Ctrl Pts',(1.759435193,1.457192641,7.033270065));
#143518=CARTESIAN_POINT('Ctrl Pts',(1.77268435110679,1.45944932065418,7.02995567001732));
#143519=CARTESIAN_POINT('Ctrl Pts',(1.78593350921352,1.46170600030836,7.02664127503467));
#143520=CARTESIAN_POINT('Origin',(-0.0291612959423751,1.3392876514148,-0.196987598544058));
#143521=CARTESIAN_POINT('Ctrl Pts',(2.057739109,1.457192641,7.212191744));
#143522=CARTESIAN_POINT('Ctrl Pts',(2.451481215,1.391489877,7.099851618));
#143523=CARTESIAN_POINT('Ctrl Pts',(2.830653465,1.326325889,6.945315037));
#143524=CARTESIAN_POINT('Ctrl Pts',(1.759435193,1.457192641,7.033270065));
#143525=CARTESIAN_POINT('Ctrl Pts',(2.143409256,1.391489877,6.93721553));
#143526=CARTESIAN_POINT('Ctrl Pts',(2.514644423,1.326325889,6.799931134));
#143527=CARTESIAN_POINT('',(2.51023121227607,1.32710049351293,6.80156153103146));
#143528=CARTESIAN_POINT('Origin',(-0.0439977657526675,1.4821309558917,-0.193085713929088));
#143529=CARTESIAN_POINT('Ctrl Pts',(2.59605857473254,1.36645689997716,7.03636837215754));
#143530=CARTESIAN_POINT('Ctrl Pts',(2.58170254353218,1.36020372535455,6.99721034804451));
#143531=CARTESIAN_POINT('Ctrl Pts',(2.56736397060224,1.35380222442514,6.95804528949166));
#143532=CARTESIAN_POINT('Ctrl Pts',(2.53875794295237,1.34069370655608,6.8797888422382));
#143533=CARTESIAN_POINT('Ctrl Pts',(2.52447487737159,1.33397954118742,6.84065475640743));
#143534=CARTESIAN_POINT('Ctrl Pts',(2.51023120578947,1.32710049367512,6.80156153336633));
#143535=CARTESIAN_POINT('Ctrl Pts',(2.35971529781516,1.326318298,7.11966385829024));
#143536=CARTESIAN_POINT('Ctrl Pts',(2.74769565534651,1.391911284,6.99107307035004));
#143537=CARTESIAN_POINT('Ctrl Pts',(3.11940512216234,1.457192641,6.82108359598844));
#143538=CARTESIAN_POINT('Ctrl Pts',(3.13225456683688,1.45944932063809,6.81520731211336));
#143539=CARTESIAN_POINT('Ctrl Pts',(3.14510401151136,1.46170600027619,6.80933102823831));
#143540=CARTESIAN_POINT('Ctrl Pts',(2.505810746,1.326318298,6.803191347));
#143541=CARTESIAN_POINT('Ctrl Pts',(2.876545188,1.391911284,6.66663920500001));
#143542=CARTESIAN_POINT('Ctrl Pts',(3.230245738,1.457192641,6.490609561));
#143543=CARTESIAN_POINT('Ctrl Pts',(3.24247264114429,1.45944932063809,6.48452447742378));
#143544=CARTESIAN_POINT('Ctrl Pts',(3.25469954428865,1.46170600027619,6.47843939384745));
#143545=CARTESIAN_POINT('Origin',(-0.070826101358471,1.33928759921943,-0.186113500958953));
#143546=CARTESIAN_POINT('Ctrl Pts',(3.560038347,1.457192641,6.601221627));
#143547=CARTESIAN_POINT('Ctrl Pts',(3.920425175,1.391489877,6.406865037));
#143548=CARTESIAN_POINT('Ctrl Pts',(4.25751179100001,1.326325889,6.174430609));
#143549=CARTESIAN_POINT('Ctrl Pts',(3.230245738,1.457192641,6.490609561));
#143550=CARTESIAN_POINT('Ctrl Pts',(3.584593815,1.391489877,6.314257655));
#143551=CARTESIAN_POINT('Ctrl Pts',(3.917637623,1.326325889,6.100378304));
#143552=CARTESIAN_POINT('',(3.91367807781615,1.32710049352139,6.10291929359378));
#143553=CARTESIAN_POINT('Origin',(-0.0844767839124982,1.48213098853565,
-0.179113172646292));
#143554=CARTESIAN_POINT('Ctrl Pts',(4.04797537440471,1.3664569000217,6.31378613517479));
#143555=CARTESIAN_POINT('Ctrl Pts',(4.02553716157696,1.36020372539197,6.2786297262122));
#143556=CARTESIAN_POINT('Ctrl Pts',(4.00311448672758,1.35380222447382,6.24346269436484));
#143557=CARTESIAN_POINT('Ctrl Pts',(3.95835474007353,1.34069379762387,6.17318577769116));
#143558=CARTESIAN_POINT('Ctrl Pts',(3.93599276743408,1.33397958600384,6.13803680249688));
#143559=CARTESIAN_POINT('Ctrl Pts',(3.91367807236571,1.32710049371077,6.10291929702005));
#143560=CARTESIAN_POINT('Ctrl Pts',(3.83506373905256,1.326318298,6.44594103746665));
#143561=CARTESIAN_POINT('Ctrl Pts',(4.18633011316466,1.391911284,6.23695232226448));
#143562=CARTESIAN_POINT('Ctrl Pts',(4.51280650719234,1.457192641,5.99103056004904));
#143563=CARTESIAN_POINT('Ctrl Pts',(4.52409231142524,1.45944932059043,5.98252940984112));
#143564=CARTESIAN_POINT('Ctrl Pts',(4.53537811565822,1.46170600018087,5.97402825963307));
#143565=CARTESIAN_POINT('Ctrl Pts',(3.909711322,1.326318298,6.105461275));
#143566=CARTESIAN_POINT('Ctrl Pts',(4.242423525,1.391911284,5.8924047));
#143567=CARTESIAN_POINT('Ctrl Pts',(4.550013582,1.457192641,5.644455368));
#143568=CARTESIAN_POINT('Ctrl Pts',(4.56064651360178,1.45944932059043,5.63588412771487));
#143569=CARTESIAN_POINT('Ctrl Pts',(4.57127944520359,1.46170600018087,5.62731288742987));
#143570=CARTESIAN_POINT('Origin',(-0.109179050594557,1.33928761673774,-0.166536633005492));
#143571=CARTESIAN_POINT('Ctrl Pts',(4.895874148,1.457192641,5.681585723));
#143572=CARTESIAN_POINT('Ctrl Pts',(5.20605441,1.391489877,5.414300567));
#143573=CARTESIAN_POINT('Ctrl Pts',(5.485293597,1.326325889,5.114836669));
#143574=CARTESIAN_POINT('Ctrl Pts',(4.550013582,1.457192641,5.644455368));
#143575=CARTESIAN_POINT('Ctrl Pts',(4.858166752,1.391489877,5.396052109));
#143576=CARTESIAN_POINT('Ctrl Pts',(5.137446442,1.326325889,5.115578565));
#143577=CARTESIAN_POINT('',(5.1341257059355,1.32710049403695,5.11891133457276));
#143578=CARTESIAN_POINT('Origin',(-0.121005727499927,1.48213091705073,-0.156765495076171));
#143579=CARTESIAN_POINT('Ctrl Pts',(5.3106133446011,1.36645689999546,5.29597827577827));
#143580=CARTESIAN_POINT('Ctrl Pts',(5.2811421360205,1.3602037253731,5.26646735662183));
#143581=CARTESIAN_POINT('Ctrl Pts',(5.25168381839431,1.35380222443046,5.23694272258867));
#143582=CARTESIAN_POINT('Ctrl Pts',(5.19286307008215,1.34069379760127,5.17793086369866));
#143583=CARTESIAN_POINT('Ctrl Pts',(5.1634679179709,1.33397958614789,5.14841081584665));
#143584=CARTESIAN_POINT('Ctrl Pts',(5.13412570249903,1.3271004938692,5.11891133803002));
#143585=CARTESIAN_POINT('Ctrl Pts',(5.13108886245636,1.326318298,5.47081317818938));
#143586=CARTESIAN_POINT('Ctrl Pts',(5.42921642824446,1.391911284,5.19119861552024));
#143587=CARTESIAN_POINT('Ctrl Pts',(5.69519407555067,1.457192641,4.88084359396323));
#143588=CARTESIAN_POINT('Ctrl Pts',(5.70438852798741,1.45944932060455,4.87011508157465));
#143589=CARTESIAN_POINT('Ctrl Pts',(5.71358298042421,1.46170600020911,4.85938656918593));
#143590=CARTESIAN_POINT('Ctrl Pts',(5.13079814199999,1.326318298,5.122246619));
#143591=CARTESIAN_POINT('Ctrl Pts',(5.409930853,1.391911284,4.8426479));
#143592=CARTESIAN_POINT('Ctrl Pts',(5.657027848,1.457192641,4.534372715));
#143593=CARTESIAN_POINT('Ctrl Pts',(5.66556962431392,1.45944932060455,4.52371609947377));
#143594=CARTESIAN_POINT('Ctrl Pts',(5.67411140062787,1.46170600020911,4.51305948394751));
#143595=CARTESIAN_POINT('Origin',(-0.142426822481519,1.33928760589289,-0.139172707724181));
#143596=CARTESIAN_POINT('Ctrl Pts',(6.002784315,1.457192641,4.496285186));
#143597=CARTESIAN_POINT('Ctrl Pts',(6.24825432699999,1.391489877,4.16856942));
#143598=CARTESIAN_POINT('Ctrl Pts',(6.456589172,1.326325889,3.816078651));
#143599=CARTESIAN_POINT('Ctrl Pts',(5.657027848,1.457192641,4.534372715));
#143600=CARTESIAN_POINT('Ctrl Pts',(5.90457721,1.391489877,4.225533165));
#143601=CARTESIAN_POINT('Ctrl Pts',(6.117033975,1.326325889,3.891580058));
#143602=CARTESIAN_POINT('',(6.114507322733,1.32710049408698,3.89554876943617));
#143603=CARTESIAN_POINT('Origin',(-0.151876474541786,1.48213096602352,-0.12708765510772));
#143604=CARTESIAN_POINT('Ctrl Pts',(6.3249329372562,1.36645689998677,4.03053635825672));
#143605=CARTESIAN_POINT('Ctrl Pts',(6.28980677379601,1.36020372535361,4.00805082670748));
#143606=CARTESIAN_POINT('Ctrl Pts',(6.25469025164565,1.35380222441028,3.98554912980152));
#143607=CARTESIAN_POINT('Ctrl Pts',(6.18455889429005,1.34069379758154,3.94056165765489));
#143608=CARTESIAN_POINT('Ctrl Pts',(6.14950504670855,1.33397958613157,3.91805086095089));
#143609=CARTESIAN_POINT('Ctrl Pts',(6.11450732013077,1.32710049387763,3.89554877354745));
#143610=CARTESIAN_POINT('Ctrl Pts',(6.18718997383337,1.326318298,4.23987617474291));
#143611=CARTESIAN_POINT('Ctrl Pts',(6.41823861689965,1.391911284,3.90271023113778));
#143612=CARTESIAN_POINT('Ctrl Pts',(6.61128069909955,1.457192641,3.54243380476249));
#143613=CARTESIAN_POINT('Ctrl Pts',(6.61795387734748,1.45944932061391,3.52997958346355));
#143614=CARTESIAN_POINT('Ctrl Pts',(6.62462705559532,1.46170600022782,3.51752536216457));
#143615=CARTESIAN_POINT('Ctrl Pts',(6.111974543,1.326318298,3.899521405));
#143616=CARTESIAN_POINT('Ctrl Pts',(6.324475827,1.391911284,3.566454266));
#143617=CARTESIAN_POINT('Ctrl Pts',(6.49952578000001,1.457192641,3.212267834));
#143618=CARTESIAN_POINT('Ctrl Pts',(6.50557699704731,1.45944932061391,3.20002413476719));
#143619=CARTESIAN_POINT('Ctrl Pts',(6.51162821409463,1.46170600022782,3.1877804355344));
#143620=CARTESIAN_POINT('Origin',(-0.169015122135372,1.33928762967766,-0.105301451691872));
#143621=CARTESIAN_POINT('Ctrl Pts',(6.829010959,1.457192641,3.10074335));
#143622=CARTESIAN_POINT('Ctrl Pts',(6.998292817,1.391489877,2.7279206));
#143623=CARTESIAN_POINT('Ctrl Pts',(7.125981812,1.326325889,2.338885036));
#143624=CARTESIAN_POINT('Ctrl Pts',(6.49952578,1.457192641,3.212267834));
#143625=CARTESIAN_POINT('Ctrl Pts',(6.674896201,1.391489877,2.857432985));
#143626=CARTESIAN_POINT('Ctrl Pts',(6.81059579800001,1.326325889,2.485615592));
#143627=CARTESIAN_POINT('',(6.80898137381432,1.3271004938241,2.49003467323014));
#143628=CARTESIAN_POINT('Origin',(-0.1756460283872,1.48213098434334,-0.0914675728584302));
#143629=CARTESIAN_POINT('Ctrl Pts',(7.04350569533385,1.3664569000354,2.57663104013053));
#143630=CARTESIAN_POINT('Ctrl Pts',(7.00436703759397,1.36020372542726,2.56222229464034));
#143631=CARTESIAN_POINT('Ctrl Pts',(6.96523432048731,1.35380222447523,2.54779568903774));
#143632=CARTESIAN_POINT('Ctrl Pts',(6.88707161862786,1.34069379763287,2.51893616756175));
#143633=CARTESIAN_POINT('Ctrl Pts',(6.84799815522327,1.33397958626634,2.50448720190976));
#143634=CARTESIAN_POINT('Ctrl Pts',(6.80898137228227,1.32710049396137,2.4900346773008));
#143635=CARTESIAN_POINT('Ctrl Pts',(6.95398495829248,1.326318298,2.8106872738861));
#143636=CARTESIAN_POINT('Ctrl Pts',(7.10715110139082,1.391911284,2.43173545452953));
#143637=CARTESIAN_POINT('Ctrl Pts',(7.21823118476806,1.457192641,2.03838374950821));
#143638=CARTESIAN_POINT('Ctrl Pts',(7.22207105844789,1.45944932065765,2.02478616465678));
#143639=CARTESIAN_POINT('Ctrl Pts',(7.22591093212768,1.4617060003153,2.01118857980531));
#143640=CARTESIAN_POINT('Ctrl Pts',(6.807361808,1.326318298,2.494458903));
#143641=CARTESIAN_POINT('Ctrl Pts',(6.94329534,1.391911284,2.123497195));
#143642=CARTESIAN_POINT('Ctrl Pts',(7.038113109,1.457192641,1.739960879));
#143643=CARTESIAN_POINT('Ctrl Pts',(7.04139081859919,1.45944932065765,1.72670259758457));
#143644=CARTESIAN_POINT('Ctrl Pts',(7.04466852819825,1.4617060003153,1.71344431616913));
#143645=CARTESIAN_POINT('Origin',(-0.187700324234343,1.33928758702522,-0.0665063034962282));
#143646=CARTESIAN_POINT('Ctrl Pts',(7.335920641,1.457192641,1.560214201));
#143647=CARTESIAN_POINT('Ctrl Pts',(7.421098912,1.391489877,1.159717245));
#143648=CARTESIAN_POINT('Ctrl Pts',(7.462171463,1.326325889,0.752327757));
#143649=CARTESIAN_POINT('Ctrl Pts',(7.038113109,1.457192641,1.739960879));
#143650=CARTESIAN_POINT('Ctrl Pts',(7.133104463,1.391489877,1.355722415));
#143651=CARTESIAN_POINT('Ctrl Pts',(7.18570173100001,1.326325889,0.963426504000001));
#143652=CARTESIAN_POINT('',(7.18507502296379,1.3271004938514,0.968089323470228));
#143653=CARTESIAN_POINT('Origin',(-0.19120240727187,1.48213096794108,-0.0515704215217526));
#143654=CARTESIAN_POINT('Ctrl Pts',(7.43273195510903,1.36645690001734,1.00224531859331));
#143655=CARTESIAN_POINT('Ctrl Pts',(7.39141088307187,1.36020372540559,0.996587095984889));
#143656=CARTESIAN_POINT('Ctrl Pts',(7.35009177350989,1.35380222447435,0.990910153806536));
#143657=CARTESIAN_POINT('Ctrl Pts',(7.26755252815035,1.34069379764965,0.979528022357111));
#143658=CARTESIAN_POINT('Ctrl Pts',(7.22628648016009,1.33397958630851,0.973816505192048));
#143659=CARTESIAN_POINT('Ctrl Pts',(7.18507502234315,1.32710049402831,0.968089327723748));
#143660=CARTESIAN_POINT('Ctrl Pts',(7.39561933502153,1.326318298,1.25007375973625));
#143661=CARTESIAN_POINT('Ctrl Pts',(7.46374109865892,1.391911284,0.847055430001511));
#143662=CARTESIAN_POINT('Ctrl Pts',(7.48766520227525,1.457192641,0.439021134686234));
#143663=CARTESIAN_POINT('Ctrl Pts',(7.48849222302968,1.45944932062251,0.424915994691601));
#143664=CARTESIAN_POINT('Ctrl Pts',(7.48931924378424,1.46170600024503,0.410810854696974));
#143665=CARTESIAN_POINT('Ctrl Pts',(7.1844444,1.326318298,0.972758276));
#143666=CARTESIAN_POINT('Ctrl Pts',(7.23745408,1.391911284,0.581247754));
#143667=CARTESIAN_POINT('Ctrl Pts',(7.247606092,1.457192641,0.186295287));
#143668=CARTESIAN_POINT('Ctrl Pts',(7.24795703198746,1.45944932062251,0.172642366394501));
#143669=CARTESIAN_POINT('Ctrl Pts',(7.24830797197507,1.46170600024503,0.158989445789));
#143670=CARTESIAN_POINT('Origin',(-0.197608983519719,1.33928764106773,-0.0246014040886011));
#143671=CARTESIAN_POINT('Ctrl Pts',(7.49981082600001,1.457192641,-0.053268829));
#143672=CARTESIAN_POINT('Ctrl Pts',(7.49690267000001,1.391489877,-0.462713199));
#143673=CARTESIAN_POINT('Ctrl Pts',(7.44943827,1.326325889,-0.869407533));
#143674=CARTESIAN_POINT('Ctrl Pts',(7.247606092,1.457192641,0.186295287));
#143675=CARTESIAN_POINT('Ctrl Pts',(7.25777669,1.391489877,-0.209380228));
#143676=CARTESIAN_POINT('Ctrl Pts',(7.224812238,1.326325889,-0.603811336));
#143677=CARTESIAN_POINT('',(7.22520254927648,1.32710049375089,-0.599122808396091));
#143678=CARTESIAN_POINT('Origin',(-0.197818010397776,1.48213094674485,-0.00926186906210269));
#143679=CARTESIAN_POINT('Ctrl Pts',(7.47441192954955,1.3664568999685,-0.619004280640579));
#143680=CARTESIAN_POINT('Ctrl Pts',(7.43284057059421,1.36020372535515,-0.615647407941441));
#143681=CARTESIAN_POINT('Ctrl Pts',(7.39126710412496,1.35380222442509,-0.612309239020518));
#143682=CARTESIAN_POINT('Ctrl Pts',(7.3082107589293,1.340693797625,-0.605681764288891));
#143683=CARTESIAN_POINT('Ctrl Pts',(7.26668168012318,1.33397958614964,-0.60238876858733));
#143684=CARTESIAN_POINT('Ctrl Pts',(7.22520254972496,1.32710049389312,-0.599122802400566));
#143685=CARTESIAN_POINT('Ctrl Pts',(7.49144277026383,1.326318298,-0.36899181485995));
#143686=CARTESIAN_POINT('Ctrl Pts',(7.47133485840931,1.391911284,-0.77723196544628));
#143687=CARTESIAN_POINT('Ctrl Pts',(7.40698431742458,1.457192641,-1.18086962076664));
#143688=CARTESIAN_POINT('Ctrl Pts',(7.4047598146672,1.45944932068645,-1.19482277583736));
#143689=CARTESIAN_POINT('Ctrl Pts',(7.4025353119098,1.4617060003729,-1.20877593090805));
#143690=CARTESIAN_POINT('Ctrl Pts',(7.225590357,1.326318298,-0.594427447));
#143691=CARTESIAN_POINT('Ctrl Pts',(7.193197511,1.391911284,-0.988180185000001));
#143692=CARTESIAN_POINT('Ctrl Pts',(7.118209069,1.457192641,-1.376081265));
#143693=CARTESIAN_POINT('Ctrl Pts',(7.11561682978261,1.45944932068645,-1.38949043000231));
#143694=CARTESIAN_POINT('Ctrl Pts',(7.11302459056518,1.4617060003729,-1.40289959500463));
#143695=CARTESIAN_POINT('Origin',(-0.198277551705002,1.33928765473254,0.0184538507370688));
#143696=CARTESIAN_POINT('Ctrl Pts',(7.313018193,1.457192641,-1.664261068));
#143697=CARTESIAN_POINT('Ctrl Pts',(7.222159592,1.391489877,-2.063507689));
#143698=CARTESIAN_POINT('Ctrl Pts',(7.088377623,1.326325889,-2.450490292));
#143699=CARTESIAN_POINT('Ctrl Pts',(7.118209069,1.457192641,-1.376081265));
#143700=CARTESIAN_POINT('Ctrl Pts',(7.043083344,1.391489877,-1.764692484));
#143701=CARTESIAN_POINT('Ctrl Pts',(6.926098554,1.326325889,-2.14281563));
#143702=CARTESIAN_POINT('',(6.92748763502108,1.32710049371206,-2.13832062223762));
#143703=CARTESIAN_POINT('Origin',(-0.195184343043897,1.48213097566634,0.0334797327397524));
#143704=CARTESIAN_POINT('Ctrl Pts',(7.16659670980258,1.36645689998385,-2.21130992726238));
#143705=CARTESIAN_POINT('Ctrl Pts',(7.12671889445975,1.36020372536164,-2.19909492311465));
#143706=CARTESIAN_POINT('Ctrl Pts',(7.08683500011182,1.35380222442229,-2.18689773242826));
#143707=CARTESIAN_POINT('Ctrl Pts',(7.00714461066936,1.34069370442274,-2.16257037256327));
#143708=CARTESIAN_POINT('Ctrl Pts',(6.96729465666842,1.33397954030356,-2.15042693333813));
#143709=CARTESIAN_POINT('Ctrl Pts',(6.92748763645859,1.32710049384016,-2.13832061743811));
#143710=CARTESIAN_POINT('Ctrl Pts',(7.23697466922751,1.326318298,-1.97080374093117));
#143711=CARTESIAN_POINT('Ctrl Pts',(7.12957730341818,1.391911284,-2.36517685756174));
#143712=CARTESIAN_POINT('Ctrl Pts',(6.97996107817798,1.457192641,-2.74554422463716));
#143713=CARTESIAN_POINT('Ctrl Pts',(6.97478906730758,1.45944932063149,-2.75869296003741));
#143714=CARTESIAN_POINT('Ctrl Pts',(6.96961705643702,1.46170600026299,-2.77184169543771));
#143715=CARTESIAN_POINT('Ctrl Pts',(6.92887574,1.326318298,-2.133818404));
#143716=CARTESIAN_POINT('Ctrl Pts',(6.812595022,1.391911284,-2.511401917));
#143717=CARTESIAN_POINT('Ctrl Pts',(6.655972501,1.457192641,-2.874113787));
#143718=CARTESIAN_POINT('Ctrl Pts',(6.65055829288275,1.45944932063149,-2.88665219806779));
#143719=CARTESIAN_POINT('Ctrl Pts',(6.64514408476563,1.46170600026299,-2.89919060913559));
#143720=CARTESIAN_POINT('Origin',(-0.189674642281049,1.33928762627356,0.060646127450637));
#143721=CARTESIAN_POINT('Ctrl Pts',(6.784276957,1.457192641,-3.19743431));
#143722=CARTESIAN_POINT('Ctrl Pts',(6.609716357,1.391489877,-3.567814853));
#143723=CARTESIAN_POINT('Ctrl Pts',(6.395872317,1.326325889,-3.916990849));
#143724=CARTESIAN_POINT('Ctrl Pts',(6.655972501,1.457192641,-2.874113787));
#143725=CARTESIAN_POINT('Ctrl Pts',(6.499063249,1.391489877,-3.237489682));
#143726=CARTESIAN_POINT('Ctrl Pts',(6.303528199,1.326325889,-3.581624247));
#143727=CARTESIAN_POINT('',(6.30585109648612,1.32710049348248,-3.57753294181973));
#143728=CARTESIAN_POINT('Origin',(-0.183423798973755,1.48213096027346,0.0746558163728089));
#143729=CARTESIAN_POINT('Ctrl Pts',(6.5236793927374,1.36645690002517,-3.7002171795176));
#143730=CARTESIAN_POINT('Ctrl Pts',(6.48735976337419,1.36020372540054,-3.67971520379541));
#143731=CARTESIAN_POINT('Ctrl Pts',(6.45103036781519,1.35380222447272,-3.65922931830479));
#143732=CARTESIAN_POINT('Ctrl Pts',(6.37843277317963,1.34069370711926,-3.61833964867325));
#143733=CARTESIAN_POINT('Ctrl Pts',(6.34212496075972,1.33397954151097,-3.59791354930418));
#143734=CARTESIAN_POINT('Ctrl Pts',(6.30585109973058,1.32710049377457,-3.57753293594657));
#143735=CARTESIAN_POINT('Ctrl Pts',(6.64411367475974,1.326318298,-3.48046307510353));
#143736=CARTESIAN_POINT('Ctrl Pts',(6.45444863851167,1.391911284,-3.8425287080016));
#143737=CARTESIAN_POINT('Ctrl Pts',(6.22656261649628,1.457192641,-4.18184023157355));
#143738=CARTESIAN_POINT('Ctrl Pts',(6.21868493465476,1.45944932070366,-4.19356972776744));
#143739=CARTESIAN_POINT('Ctrl Pts',(6.21080725281313,1.46170600040732,-4.20529922396129));
#143740=CARTESIAN_POINT('Ctrl Pts',(6.30817459400001,1.326318298,-3.573434383));
#143741=CARTESIAN_POINT('Ctrl Pts',(6.11344316000001,1.391911284,-3.917193286));
#143742=CARTESIAN_POINT('Ctrl Pts',(5.882510057,1.457192641,-4.237755942));
#143743=CARTESIAN_POINT('Ctrl Pts',(5.87452704208746,1.45944932070366,-4.24883731764522));
#143744=CARTESIAN_POINT('Ctrl Pts',(5.86654402717481,1.46170600040732,-4.25991869329037));
#143745=CARTESIAN_POINT('Origin',(-0.172203235305617,1.33928763528297,0.100002826680549));
#143746=CARTESIAN_POINT('Ctrl Pts',(5.938310471,1.457192641,-4.581099076));
#143747=CARTESIAN_POINT('Ctrl Pts',(5.688210133,1.391489877,-4.905294959));
#143748=CARTESIAN_POINT('Ctrl Pts',(5.404303129,1.326325889,-5.200337267));
#143749=CARTESIAN_POINT('Ctrl Pts',(5.882510057,1.457192641,-4.237755942));
#143750=CARTESIAN_POINT('Ctrl Pts',(5.65115418,1.391489877,-4.55890546));
#143751=CARTESIAN_POINT('Ctrl Pts',(5.386211872,1.326325889,-4.852960094));
#143752=CARTESIAN_POINT('',(5.38935997065952,1.32710049350691,-4.84946379609861));
#143753=CARTESIAN_POINT('Origin',(-0.163086630338602,1.48213094494524,0.112341076983529));
#143754=CARTESIAN_POINT('Ctrl Pts',(5.57572207796247,1.36645689999479,-5.01610638889124));
#143755=CARTESIAN_POINT('Ctrl Pts',(5.54465890009331,1.36020372537892,-4.98827609134551));
#143756=CARTESIAN_POINT('Ctrl Pts',(5.51358272538254,1.35380222444491,-4.96045940835782));
#143757=CARTESIAN_POINT('Ctrl Pts',(5.45147292145161,1.34069379762287,-4.90491976336936));
#143758=CARTESIAN_POINT('Ctrl Pts',(5.42040474501485,1.33397958598093,-4.87716590416787));
#143759=CARTESIAN_POINT('Ctrl Pts',(5.38935997523652,1.32710049369691,-4.84946379111753));
#143760=CARTESIAN_POINT('Ctrl Pts',(5.74058131055227,1.326318298,-4.82737982414743));
#143761=CARTESIAN_POINT('Ctrl Pts',(5.47751712737932,1.391911284,-5.14020818726269));
#143762=CARTESIAN_POINT('Ctrl Pts',(5.18201700780785,1.457192641,-5.42259803764836));
#143763=CARTESIAN_POINT('Ctrl Pts',(5.17180200742665,1.4594493205831,-5.43235983548967));
#143764=CARTESIAN_POINT('Ctrl Pts',(5.16158700704535,1.46170600016621,-5.442121633331));
#143765=CARTESIAN_POINT('Ctrl Pts',(5.392510215,1.326318298,-4.845960543));
#143766=CARTESIAN_POINT('Ctrl Pts',(5.12843349100001,1.391911284,-5.139821051));
#143767=CARTESIAN_POINT('Ctrl Pts',(4.833987981,1.457192641,-5.40324534));
#143768=CARTESIAN_POINT('Ctrl Pts',(4.82380943690582,1.4594493205831,-5.41235152654387));
#143769=CARTESIAN_POINT('Ctrl Pts',(4.81363089281152,1.46170600016621,-5.42145771308775));
#143770=CARTESIAN_POINT('Origin',(-0.146679738616158,1.33928761876399,0.134683584452131));
#143771=CARTESIAN_POINT('Ctrl Pts',(4.814675187,1.457192641,-5.750556742));
#143772=CARTESIAN_POINT('Ctrl Pts',(4.500729524,1.391489877,-6.013408925));
#143773=CARTESIAN_POINT('Ctrl Pts',(4.160034734,1.326325889,-6.240521694));
#143774=CARTESIAN_POINT('Ctrl Pts',(4.833987981,1.457192641,-5.40324534));
#143775=CARTESIAN_POINT('Ctrl Pts',(4.539003422,1.391489877,-5.667151885));
#143776=CARTESIAN_POINT('Ctrl Pts',(4.217042264,1.326325889,-5.897376921));
#143777=CARTESIAN_POINT('',(4.22086836503791,1.32710049374625,-5.89463911253408));
#143778=CARTESIAN_POINT('Origin',(-0.135123900040557,1.48213095657849,0.144773612127819));
#143779=CARTESIAN_POINT('Ctrl Pts',(4.36705019565857,1.36645689997344,-6.09744803840908));
#143780=CARTESIAN_POINT('Ctrl Pts',(4.34269594892901,1.3602037253429,-6.06359073269705));
#143781=CARTESIAN_POINT('Ctrl Pts',(4.31832608257802,1.35380222442097,-6.02974392943819));
#143782=CARTESIAN_POINT('Ctrl Pts',(4.2696074112792,1.34069370556785,-5.96215052401912));
#143783=CARTESIAN_POINT('Ctrl Pts',(4.24523203343021,1.33397954092168,-5.92836704876963));
#143784=CARTESIAN_POINT('Ctrl Pts',(4.22086836888483,1.32710049390968,-5.89463910972189));
#143785=CARTESIAN_POINT('Ctrl Pts',(4.56862574298837,1.326318298,-5.94857365764973));
#143786=CARTESIAN_POINT('Ctrl Pts',(4.24446300427209,1.391911284,-6.19753724418813));
#143787=CARTESIAN_POINT('Ctrl Pts',(3.89516604182185,1.457192641,-6.40980118682283));
#143788=CARTESIAN_POINT('Ctrl Pts',(3.88309136437659,1.45944932059846,-6.41713883620456));
#143789=CARTESIAN_POINT('Ctrl Pts',(3.87101668693131,1.46170600019692,-6.42447648558641));
#143790=CARTESIAN_POINT('Ctrl Pts',(4.224698052,1.326318298,-5.891894973));
#143791=CARTESIAN_POINT('Ctrl Pts',(3.903623972,1.391911284,-6.122116497));
#143792=CARTESIAN_POINT('Ctrl Pts',(3.559433999,1.457192641,-6.316084991));
#143793=CARTESIAN_POINT('Ctrl Pts',(3.54753586259849,1.45944932059845,-6.32279019388286));
#143794=CARTESIAN_POINT('Ctrl Pts',(3.53563772619695,1.46170600019692,-6.32949539676568));
#143795=CARTESIAN_POINT('Origin',(-0.114297347719498,1.33928765193469,0.163066399485854));
#143796=CARTESIAN_POINT('Ctrl Pts',(3.465911043,1.457192641,-6.651124765));
#143797=CARTESIAN_POINT('Ctrl Pts',(3.102799805,1.391489877,-6.840342573));
#143798=CARTESIAN_POINT('Ctrl Pts',(2.721247738,1.326325889,-6.988906263));
#143799=CARTESIAN_POINT('Ctrl Pts',(3.559433999,1.457192641,-6.316084991));
#143800=CARTESIAN_POINT('Ctrl Pts',(3.214613909,1.391489877,-6.510408587));
#143801=CARTESIAN_POINT('Ctrl Pts',(2.850688446,1.326325889,-6.66603895700001));
#143802=CARTESIAN_POINT('',(2.85501364068508,1.32710049349123,-6.66418765582323));
#143803=CARTESIAN_POINT('Origin',(-0.100842727121628,1.48213099008862,0.170436515317088));
#143804=CARTESIAN_POINT('Ctrl Pts',(2.95417989991179,1.36645689997307,-6.89367979481652));
#143805=CARTESIAN_POINT('Ctrl Pts',(2.93767336182599,1.36020372535119,-6.85537861096055));
#143806=CARTESIAN_POINT('Ctrl Pts',(2.92114931151543,1.35380222442209,-6.81708432616746));
#143807=CARTESIAN_POINT('Ctrl Pts',(2.88810047152572,1.34069379757943,-6.74059867960663));
#143808=CARTESIAN_POINT('Ctrl Pts',(2.87155730126059,1.3339795860005,-6.70236477081003));
#143809=CARTESIAN_POINT('Ctrl Pts',(2.85501364640299,1.32710049370827,-6.66418765330632));
#143810=CARTESIAN_POINT('Ctrl Pts',(3.18304631452933,1.326318298,-6.79161879846183));
#143811=CARTESIAN_POINT('Ctrl Pts',(2.81294250805842,1.391911284,-6.96507634840551));
#143812=CARTESIAN_POINT('Ctrl Pts',(2.42618144212585,1.457192641,-7.09728915532328));
#143813=CARTESIAN_POINT('Ctrl Pts',(2.41281168597534,1.45944932064318,-7.10185955587329));
#143814=CARTESIAN_POINT('Ctrl Pts',(2.39944192982491,1.46170600028635,-7.10642995642344));
#143815=CARTESIAN_POINT('Ctrl Pts',(2.859343703,1.326318298,-6.662330943));
#143816=CARTESIAN_POINT('Ctrl Pts',(2.496285335,1.391911284,-6.818148579));
#143817=CARTESIAN_POINT('Ctrl Pts',(2.118444839,1.457192641,-6.933591527));
#143818=CARTESIAN_POINT('Ctrl Pts',(2.10538345371521,1.45944932064317,-6.93758221841136));
#143819=CARTESIAN_POINT('Ctrl Pts',(2.09232206843043,1.46170600028635,-6.94157290982255));
#143820=CARTESIAN_POINT('Origin',(-0.0765706498909213,1.33928761153607,
0.183824456529189));
#143821=CARTESIAN_POINT('Ctrl Pts',(1.95508475,1.457192641,-7.240693587));
#143822=CARTESIAN_POINT('Ctrl Pts',(1.559786616,1.391489877,-7.347429405));
#143823=CARTESIAN_POINT('Ctrl Pts',(1.155218222,1.326325889,-7.41049734200001));
#143824=CARTESIAN_POINT('Ctrl Pts',(2.118444839,1.457192641,-6.933591527));
#143825=CARTESIAN_POINT('Ctrl Pts',(1.739912622,1.391489877,-7.049245819));
#143826=CARTESIAN_POINT('Ctrl Pts',(1.351039605,1.326325889,-7.12300442100001));
#143827=CARTESIAN_POINT('',(1.35566165652867,1.3271004937223,-7.12212619180199));
#143828=CARTESIAN_POINT('Origin',(-0.0618462780225851,1.4821309815227,0.18813004085965));
#143829=CARTESIAN_POINT('Ctrl Pts',(1.40317543510778,1.36645689995796,-7.36757074577874));
#143830=CARTESIAN_POINT('Ctrl Pts',(1.39528843307492,1.36020372535873,-7.32661660460976));
#143831=CARTESIAN_POINT('Ctrl Pts',(1.38738284513841,1.35380222441668,-7.28566543635231));
#143832=CARTESIAN_POINT('Ctrl Pts',(1.37154882199612,1.34069379762891,-7.20386345811269));
#143833=CARTESIAN_POINT('Ctrl Pts',(1.36361158243823,1.33397958625016,-7.16296714532754));
#143834=CARTESIAN_POINT('Ctrl Pts',(1.35566166106545,1.32710049399294,-7.1221261908733));
#143835=CARTESIAN_POINT('Ctrl Pts',(1.64863117716275,1.326318298,-7.31709539294675));
#143836=CARTESIAN_POINT('Ctrl Pts',(1.24989194723245,1.391911284,-7.40693622353499));
#143837=CARTESIAN_POINT('Ctrl Pts',(0.843751293891287,1.457192641,-7.452915771864));
#143838=CARTESIAN_POINT('Ctrl Pts',(0.829711613941566,1.45944932067839,
-7.45450521664739));
#143839=CARTESIAN_POINT('Ctrl Pts',(0.81567193399185,1.46170600035678,-7.45609466143078));
#143840=CARTESIAN_POINT('Ctrl Pts',(1.360289621,1.326318298,-7.121243722));
#143841=CARTESIAN_POINT('Ctrl Pts',(0.972223169,1.391911284,-7.195371611));
#143842=CARTESIAN_POINT('Ctrl Pts',(0.578399553,1.457192641,-7.22689103));
#143843=CARTESIAN_POINT('Ctrl Pts',(0.564785654761062,1.45944932067839,
-7.22798060956149));
#143844=CARTESIAN_POINT('Ctrl Pts',(0.55117175652214,1.46170600035678,-7.22907018912286));
#143845=CARTESIAN_POINT('Origin',(-0.0352636698467937,1.33928765144172,
0.195987353699291));
#143846=CARTESIAN_POINT('Ctrl Pts',(0.352840867,1.457192641,-7.491695624));
#143847=CARTESIAN_POINT('Ctrl Pts',(-0.056160462,1.391489877,-7.510958604));
#143848=CARTESIAN_POINT('Ctrl Pts',(-0.464828014,1.326325889,-7.485581802));
#143849=CARTESIAN_POINT('Ctrl Pts',(0.578399553,1.457192641,-7.22689103));
#143850=CARTESIAN_POINT('Ctrl Pts',(0.183854955,1.391489877,-7.258468152));
#143851=CARTESIAN_POINT('Ctrl Pts',(-0.211782346,1.326325889,-7.246906115));
#143852=CARTESIAN_POINT('',(-0.207079563753079,1.32710049360996,-7.24704202119074));
#143853=CARTESIAN_POINT('Origin',(-0.019957948281468,1.48213098225561,0.197026683410473));
#143854=CARTESIAN_POINT('Ctrl Pts',(-0.213439952651145,1.36645689674192,
-7.49696225529675));
#143855=CARTESIAN_POINT('Ctrl Pts',(-0.212338631177845,1.36020372208674,
-7.45527012694911));
#143856=CARTESIAN_POINT('Ctrl Pts',(-0.211256100755129,1.35380222443176,
-7.41357692822774));
#143857=CARTESIAN_POINT('Ctrl Pts',(-0.209134926056559,1.34069379761266,
-7.33028358799617));
#143858=CARTESIAN_POINT('Ctrl Pts',(-0.208095099061949,1.33397958596669,
-7.28863713496509));
#143859=CARTESIAN_POINT('Ctrl Pts',(-0.207079557909248,1.32710049367483,
-7.24704202132269));
#143860=CARTESIAN_POINT('Ctrl Pts',(0.0371278792293957,1.326318298,-7.5004327383073));
#143861=CARTESIAN_POINT('Ctrl Pts',(-0.371602173148636,1.391911284,-7.50245599257178));
#143862=CARTESIAN_POINT('Ctrl Pts',(-0.778131726340747,1.457192641,-7.46005233013552));
#143863=CARTESIAN_POINT('Ctrl Pts',(-0.792184849719485,1.45944932063632,
-7.4585864984506));
#143864=CARTESIAN_POINT('Ctrl Pts',(-0.806237973098223,1.46170600027265,
-7.45712066676558));
#143865=CARTESIAN_POINT('Ctrl Pts',(-0.202370093,1.326318298,-7.24717506));
#143866=CARTESIAN_POINT('Ctrl Pts',(-0.597299071,1.391911284,-7.236147064));
#143867=CARTESIAN_POINT('Ctrl Pts',(-0.988691053000001,1.457192641,-7.18226914));
#143868=CARTESIAN_POINT('Ctrl Pts',(-1.00222089300623,1.45944932063632,
-7.18040666012023));
#143869=CARTESIAN_POINT('Ctrl Pts',(-1.01575073301247,1.46170600027265,
-7.17854418024035));
#143870=CARTESIAN_POINT('Origin',(0.00769225992611006,1.33928762690979,
0.198985872132881));
#143871=CARTESIAN_POINT('Ctrl Pts',(-1.265901463,1.457192641,-7.3923943));
#143872=CARTESIAN_POINT('Ctrl Pts',(-1.669481539,1.391489877,-7.323283727));
#143873=CARTESIAN_POINT('Ctrl Pts',(-2.063139409,1.326325889,-7.210648777));
#143874=CARTESIAN_POINT('Ctrl Pts',(-0.988691053,1.457192641,-7.18226914));
#143875=CARTESIAN_POINT('Ctrl Pts',(-1.380799566,1.391489877,-7.128292581));
#143876=CARTESIAN_POINT('Ctrl Pts',(-1.76470159,1.326325889,-7.031950533));
#143877=CARTESIAN_POINT('',(-1.76013797088958,1.32710049375817,-7.03309422218891));
#143878=CARTESIAN_POINT('Origin',(0.0228635298486249,1.48213092814597,0.196710412613236));
#143879=CARTESIAN_POINT('Ctrl Pts',(-1.82007512674902,1.36645689996125,
-7.27580418457839));
#143880=CARTESIAN_POINT('Ctrl Pts',(-1.81003697829886,1.36020372534332,
-7.23532354641029));
#143881=CARTESIAN_POINT('Ctrl Pts',(-1.80001694630848,1.35380222441891,
-7.19483780259815));
#143882=CARTESIAN_POINT('Ctrl Pts',(-1.78003962021609,1.34069370770243,
-7.11394724922861));
#143883=CARTESIAN_POINT('Ctrl Pts',(-1.77007142075049,1.33397954195139,
-7.07349829535953));
#143884=CARTESIAN_POINT('Ctrl Pts',(-1.76013796613543,1.32710049389721,
-7.03309422333406));
#143885=CARTESIAN_POINT('Ctrl Pts',(-1.57611147796712,1.326318298,-7.33305818576935));
#143886=CARTESIAN_POINT('Ctrl Pts',(-1.97572058815322,1.391911284,-7.24716925836755));
#143887=CARTESIAN_POINT('Ctrl Pts',(-2.36363017270464,1.457192641,-7.11836513186888));
#143888=CARTESIAN_POINT('Ctrl Pts',(-2.37703963177751,1.45944932070005,
-7.1139125642307));
#143889=CARTESIAN_POINT('Ctrl Pts',(-2.39044909085038,1.46170600040011,
-7.10945999659266));
#143890=CARTESIAN_POINT('Ctrl Pts',(-1.755567205,1.326318298,-7.034236546));
#143891=CARTESIAN_POINT('Ctrl Pts',(-2.13889227,1.391911284,-6.93856832300001));
#143892=CARTESIAN_POINT('Ctrl Pts',(-2.509551565,1.457192641,-6.801812328));
#143893=CARTESIAN_POINT('Ctrl Pts',(-2.52236470714504,1.45944932070005,
-6.7970848760603));
#143894=CARTESIAN_POINT('Ctrl Pts',(-2.53517784929007,1.46170600040011,
-6.79235742412048));
#143895=CARTESIAN_POINT('Origin',(0.050288452313495,1.33928759751438,0.192679977206598));
#143896=CARTESIAN_POINT('Ctrl Pts',(-2.825451647,1.457192641,-6.947432835));
#143897=CARTESIAN_POINT('Ctrl Pts',(-3.204739515,1.391489877,-6.793180241));
#143898=CARTESIAN_POINT('Ctrl Pts',(-3.564980697,1.326325889,-6.598553828));
#143899=CARTESIAN_POINT('Ctrl Pts',(-2.509551565,1.457192641,-6.801812328));
#143900=CARTESIAN_POINT('Ctrl Pts',(-2.880889433,1.391489877,-6.66480597100001));
#143901=CARTESIAN_POINT('Ctrl Pts',(-3.235105349,1.326325889,-6.48818876000001));
#143902=CARTESIAN_POINT('',(-3.23089428594815,1.32710049348572,-6.49028675121906));
#143903=CARTESIAN_POINT('Origin',(0.0646160045864197,1.48213096720064,0.187196666467568));
#143904=CARTESIAN_POINT('Ctrl Pts',(-3.34160561001,1.36645689996097,-6.71443757429174));
#143905=CARTESIAN_POINT('Ctrl Pts',(-3.32310000733223,1.36020372536039,
-6.67706125633319));
#143906=CARTESIAN_POINT('Ctrl Pts',(-3.30461099988384,1.35380222441652,
-6.63967605740425));
#143907=CARTESIAN_POINT('Ctrl Pts',(-3.26771162001808,1.34069369538312,
-6.56497114488844));
#143908=CARTESIAN_POINT('Ctrl Pts',(-3.2492811600615,1.33397953570377,-6.52761076976344));
#143909=CARTESIAN_POINT('Ctrl Pts',(-3.23089427915016,1.3271004937052,-6.49028675464853));
#143910=CARTESIAN_POINT('Ctrl Pts',(-3.11565361346418,1.326318298,-6.82279798221481));
#143911=CARTESIAN_POINT('Ctrl Pts',(-3.48745650442699,1.391911284,-6.65301294327397));
#143912=CARTESIAN_POINT('Ctrl Pts',(-3.83860789814415,1.457192641,-6.44383109203171));
#143913=CARTESIAN_POINT('Ctrl Pts',(-3.85074668095551,1.45944932067843,
-6.43659998571765));
#143914=CARTESIAN_POINT('Ctrl Pts',(-3.8628854637669,1.46170600035686,-6.42936887940343));
#143915=CARTESIAN_POINT('Ctrl Pts',(-3.226675946,1.326318298,-6.49238495));
#143916=CARTESIAN_POINT('Ctrl Pts',(-3.580473244,1.391911284,-6.316549838));
#143917=CARTESIAN_POINT('Ctrl Pts',(-3.913068234,1.457192641,-6.10331033100001));
#143918=CARTESIAN_POINT('Ctrl Pts',(-3.92456554945993,1.45944932067843,
-6.09593895754517));
#143919=CARTESIAN_POINT('Ctrl Pts',(-3.93606286491986,1.46170600035686,
-6.0885675840903));
#143920=CARTESIAN_POINT('Origin',(0.0905333490495397,1.33928762116643,0.177364880444342));
#143921=CARTESIAN_POINT('Ctrl Pts',(-4.252886852,1.457192641,-6.177617131));
#143922=CARTESIAN_POINT('Ctrl Pts',(-4.590147433,1.391489877,-5.945435198));
#143923=CARTESIAN_POINT('Ctrl Pts',(-4.900127451,1.326325889,-5.67791783700001));
#143924=CARTESIAN_POINT('Ctrl Pts',(-3.913068234,1.457192641,-6.103310331));
#143925=CARTESIAN_POINT('Ctrl Pts',(-4.246272112,1.391489877,-5.889680441));
#143926=CARTESIAN_POINT('Ctrl Pts',(-4.554239178,1.326325889,-5.641046491));
#143927=CARTESIAN_POINT('',(-4.55057757322335,1.32710049349811,-5.64400068666468));
#143928=CARTESIAN_POINT('Origin',(0.103347140030356,1.48213096708157,0.168929683164989));
#143929=CARTESIAN_POINT('Ctrl Pts',(-4.70688632880667,1.36645689996756,
-5.83911132632025));
#143930=CARTESIAN_POINT('Ctrl Pts',(-4.68077857330409,1.36020372535252,
-5.80658700333002));
#143931=CARTESIAN_POINT('Ctrl Pts',(-4.65468511606554,1.35380222443658,
-5.77405043970525));
#143932=CARTESIAN_POINT('Ctrl Pts',(-4.60258908000211,1.34069369659121,
-5.70902436814684));
#143933=CARTESIAN_POINT('Ctrl Pts',(-4.57655813520577,1.33397953632925,
-5.67649945876565));
#143934=CARTESIAN_POINT('Ctrl Pts',(-4.55057756715233,1.32710049376822,
-5.64400069147785));
#143935=CARTESIAN_POINT('Ctrl Pts',(-4.50951124921828,1.326318298,-5.99351132775202));
#143936=CARTESIAN_POINT('Ctrl Pts',(-4.83612282993803,1.391911284,-5.74776913795098));
#143937=CARTESIAN_POINT('Ctrl Pts',(-5.13409658570113,1.457192641,-5.4679906727476));
#143938=CARTESIAN_POINT('Ctrl Pts',(-5.14439709605691,1.45944932059279,
-5.45831914657319));
#143939=CARTESIAN_POINT('Ctrl Pts',(-5.15469760641271,1.46170600018559,
-5.44864762039864));
#143940=CARTESIAN_POINT('Ctrl Pts',(-4.546908906,1.326318298,-5.646956649));
#143941=CARTESIAN_POINT('Ctrl Pts',(-4.854635269,1.391911284,-5.399176504));
#143942=CARTESIAN_POINT('Ctrl Pts',(-5.133614182,1.457192641,-5.119424326));
#143943=CARTESIAN_POINT('Ctrl Pts',(-5.14325806884177,1.45944932059279,
-5.10975370853518));
#143944=CARTESIAN_POINT('Ctrl Pts',(-5.15290195568366,1.46170600018559,
-5.10008309107027));
#143945=CARTESIAN_POINT('Origin',(0.126544741838824,1.3392876175325,0.153755982148334));
#143946=CARTESIAN_POINT('Ctrl Pts',(-5.481461795,1.457192641,-5.118942917));
#143947=CARTESIAN_POINT('Ctrl Pts',(-5.760925159,1.391489877,-4.819688212));
#143948=CARTESIAN_POINT('Ctrl Pts',(-6.006149691,1.326325889,-4.491788718));
#143949=CARTESIAN_POINT('Ctrl Pts',(-5.133614182,1.457192641,-5.119424326));
#143950=CARTESIAN_POINT('Ctrl Pts',(-5.413103827,1.391489877,-4.83916));
#143951=CARTESIAN_POINT('Ctrl Pts',(-5.660421844,1.326325889,-4.530135158));
#143952=CARTESIAN_POINT('',(-5.65748091030866,1.32710049348203,-4.53380742346978));
#143953=CARTESIAN_POINT('Origin',(0.137245870428021,1.48213098361316,0.142763663710617));
#143954=CARTESIAN_POINT('Ctrl Pts',(-5.85207827439091,1.36645689999436,
-4.69075472208899));
#143955=CARTESIAN_POINT('Ctrl Pts',(-5.81958913571005,1.36020372537183,
-4.66460319540688));
#143956=CARTESIAN_POINT('Ctrl Pts',(-5.78711132963947,1.35380222444224,
-4.63843664054921));
#143957=CARTESIAN_POINT('Ctrl Pts',(-5.72225508680042,1.34069379760831,
-4.5861303533718));
#143958=CARTESIAN_POINT('Ctrl Pts',(-5.68984057087204,1.33397958597717,
-4.55996152766193));
#143959=CARTESIAN_POINT('Ctrl Pts',(-5.65748090610616,1.32710049369622,
-4.53380742861306));
#143960=CARTESIAN_POINT('Ctrl Pts',(-5.69250915066891,1.326318298,-4.88397474512399));
#143961=CARTESIAN_POINT('Ctrl Pts',(-5.95865742732611,1.391911284,-4.57376603597315));
#143962=CARTESIAN_POINT('Ctrl Pts',(-6.18952062274078,1.457192641,-4.23647308634013));
#143963=CARTESIAN_POINT('Ctrl Pts',(-6.19750122062436,1.4594493205828,-4.22481336987838));
#143964=CARTESIAN_POINT('Ctrl Pts',(-6.20548181850794,1.46170600016559,
-4.21315365341668));
#143965=CARTESIAN_POINT('Ctrl Pts',(-5.65453346,1.326318298,-4.537482931));
#143966=CARTESIAN_POINT('Ctrl Pts',(-5.901799944,1.391911284,-4.229343677));
#143967=CARTESIAN_POINT('Ctrl Pts',(-6.114118036,1.457192641,-3.89615973));
#143968=CARTESIAN_POINT('Ctrl Pts',(-6.12145755719401,1.45944932058279,
-3.88464205565829));
#143969=CARTESIAN_POINT('Ctrl Pts',(-6.12879707838804,1.4617060001656,-3.87312438131663));
#143970=CARTESIAN_POINT('Origin',(0.156639207923298,1.33928759898889,0.12295788907206));
#143971=CARTESIAN_POINT('Ctrl Pts',(-6.453729677,1.457192641,-3.820912621));
#143972=CARTESIAN_POINT('Ctrl Pts',(-6.662328427,1.391489877,-3.468577963));
#143973=CARTESIAN_POINT('Ctrl Pts',(-6.831331047,1.326325889,-3.095628551));
#143974=CARTESIAN_POINT('Ctrl Pts',(-6.11411803600001,1.457192641,-3.89615973));
#143975=CARTESIAN_POINT('Ctrl Pts',(-6.326824824,1.391489877,-3.562365816));
#143976=CARTESIAN_POINT('Ctrl Pts',(-6.501929476,1.326325889,-3.20739974));
#143977=CARTESIAN_POINT('',(-6.4998467281796,1.32710049370012,-3.21161836600255));
#143978=CARTESIAN_POINT('Origin',(0.164726821765547,1.48213093831918,0.109921952271952));
#143979=CARTESIAN_POINT('Ctrl Pts',(-6.723633543987,1.36645689999757,-3.32306364089608));
#143980=CARTESIAN_POINT('Ctrl Pts',(-6.68628217802592,1.3602037253718,-3.30450772682288));
#143981=CARTESIAN_POINT('Ctrl Pts',(-6.64893864914608,1.35380222444506,
-3.28593469975597));
#143982=CARTESIAN_POINT('Ctrl Pts',(-6.57435389535092,1.34069370829399,
-3.24879322648768));
#143983=CARTESIAN_POINT('Ctrl Pts',(-6.53707196030162,1.33397954224069,
-3.23020451101497));
#143984=CARTESIAN_POINT('Ctrl Pts',(-6.49984672601538,1.32710049388369,
-3.21161837026922));
#143985=CARTESIAN_POINT('Ctrl Pts',(-6.60933165067934,1.326318298,-3.54606893236592));
#143986=CARTESIAN_POINT('Ctrl Pts',(-6.80257182677962,1.391911284,-3.18589871739284));
#143987=CARTESIAN_POINT('Ctrl Pts',(-6.95552955380988,1.457192641,-2.80686272650075));
#143988=CARTESIAN_POINT('Ctrl Pts',(-6.9608170736095,1.45944931985099,-2.79376001933108));
#143989=CARTESIAN_POINT('Ctrl Pts',(-6.9661045934092,1.46170599870198,-2.7806573121614));
#143990=CARTESIAN_POINT('Ctrl Pts',(-6.497758313,1.326318298,-3.215841555));
#143991=CARTESIAN_POINT('Ctrl Pts',(-6.67300301300001,1.391911284,-2.86175144));
#143992=CARTESIAN_POINT('Ctrl Pts',(-6.808732526,1.457192641,-2.490715035));
#143993=CARTESIAN_POINT('Ctrl Pts',(-6.81342449221393,1.45944931985099,
-2.47788886154728));
#143994=CARTESIAN_POINT('Ctrl Pts',(-6.8181164584277,1.46170599870198,-2.46506268809461));
#143995=CARTESIAN_POINT('Origin',(0.179409394884619,1.33928762174604,0.0864104006243482));
#143996=CARTESIAN_POINT('Ctrl Pts',(-7.124228332,1.457192641,-2.344220698));
#143997=CARTESIAN_POINT('Ctrl Pts',(-7.252208622,1.391489877,-1.955280863));
#143998=CARTESIAN_POINT('Ctrl Pts',(-7.33708695600001,1.326325889,-1.554720233));
#143999=CARTESIAN_POINT('Ctrl Pts',(-6.808732526,1.457192641,-2.490715035));
#144000=CARTESIAN_POINT('Ctrl Pts',(-6.944710523,1.391489877,-2.118999365));
#144001=CARTESIAN_POINT('Ctrl Pts',(-7.039414112,1.326325889,-1.734689875));
#144002=CARTESIAN_POINT('',(-7.03828693677588,1.3271004934935,-1.73925759858549));
#144003=CARTESIAN_POINT('Origin',(0.184505602804806,1.48213091444911,0.0719406485621665));
#144004=CARTESIAN_POINT('Ctrl Pts',(-7.2807991818215,1.36645690001632,-1.79998979688873));
#144005=CARTESIAN_POINT('Ctrl Pts',(-7.2403320970141,1.36020372537985,-1.78989714928127));
#144006=CARTESIAN_POINT('Ctrl Pts',(-7.19986898733355,1.3538022244547,-1.7797861040923));
#144007=CARTESIAN_POINT('Ctrl Pts',(-7.1190436215013,1.34069370128852,-1.75954648444623));
#144008=CARTESIAN_POINT('Ctrl Pts',(-7.07863731480259,1.3339795386024,-1.74940688235601));
#144009=CARTESIAN_POINT('Ctrl Pts',(-7.03828693507949,1.32710049369933,
-1.73925760555958));
#144010=CARTESIAN_POINT('Ctrl Pts',(-7.21710914931238,1.326318298,-2.04235287662906));
#144011=CARTESIAN_POINT('Ctrl Pts',(-7.32840552681089,1.391911284,-1.64906231605164));
#144012=CARTESIAN_POINT('Ctrl Pts',(-7.39630565439733,1.457192641,-1.24600658618423));
#144013=CARTESIAN_POINT('Ctrl Pts',(-7.39865286098283,1.45944932057495,
-1.23207354810171));
#144014=CARTESIAN_POINT('Ctrl Pts',(-7.40100006756837,1.46170600014991,
-1.21814051001917));
#144015=CARTESIAN_POINT('Ctrl Pts',(-7.037155209,1.326318298,-1.743831002));
#144016=CARTESIAN_POINT('Ctrl Pts',(-7.13218387800001,1.391911284,-1.360346886));
#144017=CARTESIAN_POINT('Ctrl Pts',(-7.18497825100001,1.457192641,-0.968807273));
#144018=CARTESIAN_POINT('Ctrl Pts',(-7.18680327408004,1.45944932057495,
-0.955272329977257));
#144019=CARTESIAN_POINT('Ctrl Pts',(-7.18862829716009,1.46170600014991,
-0.941737386954499));
#144020=CARTESIAN_POINT('Origin',(0.193790514631866,1.33928765482181,0.0458224414306448));
#144021=CARTESIAN_POINT('Ctrl Pts',(-7.461605988,1.457192641,-0.75791562));
#144022=CARTESIAN_POINT('Ctrl Pts',(-7.502983602,1.391489877,-0.350557003));
#144023=CARTESIAN_POINT('Ctrl Pts',(-7.499768833,1.326325889,0.058885075));
#144024=CARTESIAN_POINT('Ctrl Pts',(-7.184978251,1.457192641,-0.968807273));
#144025=CARTESIAN_POINT('Ctrl Pts',(-7.237869276,1.391489877,-0.57655086));
#144026=CARTESIAN_POINT('Ctrl Pts',(-7.247743568,1.326325889,-0.180867839));
#144027=CARTESIAN_POINT('',(-7.24762467142716,1.32710049364435,-0.185571082245031));
#144028=CARTESIAN_POINT('Origin',(0.195657359581503,1.48213100007743,0.0305955037867436));
#144029=CARTESIAN_POINT('Ctrl Pts',(-7.4975227417753,1.36645690002419,-0.192750430437088));
#144030=CARTESIAN_POINT('Ctrl Pts',(-7.45583213413798,1.36020372540562,
-0.191592970424011));
#144031=CARTESIAN_POINT('Ctrl Pts',(-7.4141414537035,1.35380222448827,-0.190416688389667));
#144032=CARTESIAN_POINT('Ctrl Pts',(-7.3308554322295,1.34069379766143,-0.188025341830143));
#144033=CARTESIAN_POINT('Ctrl Pts',(-7.28921376232473,1.33397958603636,
-0.186808950438261));
#144034=CARTESIAN_POINT('Ctrl Pts',(-7.24762467122657,1.32710049376091,
-0.185571088336482));
#144035=CARTESIAN_POINT('Ctrl Pts',(-7.48742264462421,1.326318298,-0.443138670805058));
#144036=CARTESIAN_POINT('Ctrl Pts',(-7.51157113006944,1.391911284,-0.0351175931108654));
#144037=CARTESIAN_POINT('Ctrl Pts',(-7.49123872278317,1.457192641,0.373111438402629));
#144038=CARTESIAN_POINT('Ctrl Pts',(-7.49053586165044,1.45944932058945,
0.387223309931836));
#144039=CARTESIAN_POINT('Ctrl Pts',(-7.48983300051772,1.4617060001789,0.401335181461041));
#144040=CARTESIAN_POINT('Ctrl Pts',(-7.247502549,1.326318298,-0.190280849));
#144041=CARTESIAN_POINT('Ctrl Pts',(-7.257871751,1.391911284,0.204665976));
#144042=CARTESIAN_POINT('Ctrl Pts',(-7.225262378,1.457192641,0.59840084));
#144043=CARTESIAN_POINT('Ctrl Pts',(-7.22413512038993,1.45944932058945,
0.612011669677492));
#144044=CARTESIAN_POINT('Ctrl Pts',(-7.22300786277985,1.4617060001789,0.625622499354983));
#144045=CARTESIAN_POINT('Origin',(0.199110329142863,1.33928764733072,0.00309190139125497));
#144046=CARTESIAN_POINT('Ctrl Pts',(-7.450087241,1.457192641,0.86382875));
#144047=CARTESIAN_POINT('Ctrl Pts',(-7.402927409,1.391489877,1.270558513));
#144048=CARTESIAN_POINT('Ctrl Pts',(-7.311769855,1.326325889,1.669736982));
#144049=CARTESIAN_POINT('Ctrl Pts',(-7.225262378,1.457192641,0.59840084));
#144050=CARTESIAN_POINT('Ctrl Pts',(-7.192593307,1.391489877,0.992856524000001));
#144051=CARTESIAN_POINT('Ctrl Pts',(-7.11717659,1.326325889,1.381411376));
#144052=CARTESIAN_POINT('',(-7.11807153258829,1.32710049373858,1.37679253178578));
#144053=CARTESIAN_POINT('Origin',(0.197659878927633,1.48213093731636,-0.0121803272532719));
#144054=CARTESIAN_POINT('Ctrl Pts',(-7.36367047157635,1.36645689998419,
1.42350173179027));
#144055=CARTESIAN_POINT('Ctrl Pts',(-7.32270574734249,1.36020372535754,
1.41566988274934));
#144056=CARTESIAN_POINT('Ctrl Pts',(-7.28173690607024,1.3538022244682,1.40785640008115));
#144057=CARTESIAN_POINT('Ctrl Pts',(-7.19988399654352,1.34069379764131,
1.39228780563331));
#144058=CARTESIAN_POINT('Ctrl Pts',(-7.15895439847139,1.33397958617594,
1.38452403057887));
#144059=CARTESIAN_POINT('Ctrl Pts',(-7.11807153346691,1.32710049390419,
1.37679252699242));
#144060=CARTESIAN_POINT('Ctrl Pts',(-7.40763257896271,1.326318298,1.17679620739308));
#144061=CARTESIAN_POINT('Ctrl Pts',(-7.34350401581921,1.391911284,1.58046918964569));
#144062=CARTESIAN_POINT('Ctrl Pts',(-7.23588979397156,1.457192641,1.97478318634273));
#144063=CARTESIAN_POINT('Ctrl Pts',(-7.23216973004729,1.45944932061847,
1.98841403595307));
#144064=CARTESIAN_POINT('Ctrl Pts',(-7.22844966612306,1.46170600023695,
2.00204488556346));
#144065=CARTESIAN_POINT('Ctrl Pts',(-7.118964725,1.326318298,1.372166625));
#144066=CARTESIAN_POINT('Ctrl Pts',(-7.044189608,1.391911284,1.760108884));
#144067=CARTESIAN_POINT('Ctrl Pts',(-6.927701267,1.457192641,2.137628395));
#144068=CARTESIAN_POINT('Ctrl Pts',(-6.92367443794796,1.45944932061847,
2.1506786841668));
#144069=CARTESIAN_POINT('Ctrl Pts',(-6.9196476088959,1.46170600023695,2.16372897333358));
#144070=CARTESIAN_POINT('Origin',(0.195119959503641,1.33928761351094,-0.0397832256104988));
#144071=CARTESIAN_POINT('Ctrl Pts',(-7.090210694,1.457192641,2.445181447));
#144072=CARTESIAN_POINT('Ctrl Pts',(-6.956718557,1.391489877,2.832264125));
#144073=CARTESIAN_POINT('Ctrl Pts',(-6.781880645,1.326325889,3.202513844));
#144074=CARTESIAN_POINT('Ctrl Pts',(-6.927701267,1.457192641,2.137628395));
#144075=CARTESIAN_POINT('Ctrl Pts',(-6.810999668,1.391489877,2.515839039));
#144076=CARTESIAN_POINT('Ctrl Pts',(-6.653818345,1.326325889,2.87909733));
#144077=CARTESIAN_POINT('',(-6.65568527723499,1.32710049346833,2.8747788600681));
#144078=CARTESIAN_POINT('Origin',(0.19042055041486,1.48213096031789,-0.0543866830032513));
#144079=CARTESIAN_POINT('Ctrl Pts',(-6.88550115417648,1.36645690001224,
2.9731925354682));
#144080=CARTESIAN_POINT('Ctrl Pts',(-6.84717777853504,1.36020372538709,
2.95673758590746));
#144081=CARTESIAN_POINT('Ctrl Pts',(-6.80884643362966,1.35380222445678,
2.9402996881705));
#144082=CARTESIAN_POINT('Ctrl Pts',(-6.73225398731902,1.34069379761851,
2.90749912276099));
#144083=CARTESIAN_POINT('Ctrl Pts',(-6.6939502817044,1.33397958597253,2.89111820627741));
#144084=CARTESIAN_POINT('Ctrl Pts',(-6.65568528011168,1.32710049368268,
2.87477885338197));
#144085=CARTESIAN_POINT('Ctrl Pts',(-6.9814698473063,1.326318298,2.74170540229439));
#144086=CARTESIAN_POINT('Ctrl Pts',(-6.83206281608202,1.391911284,3.12215498942192));
#144087=CARTESIAN_POINT('Ctrl Pts',(-6.64219870107241,1.457192641,3.48411626705969));
#144088=CARTESIAN_POINT('Ctrl Pts',(-6.63563538022026,1.45944932068712,
3.49662873157185));
#144089=CARTESIAN_POINT('Ctrl Pts',(-6.62907205936814,1.46170600037424,
3.50914119608405));
#144090=CARTESIAN_POINT('Ctrl Pts',(-6.657552022,1.326318298,2.870453113));
#144091=CARTESIAN_POINT('Ctrl Pts',(-6.501128988,1.391911284,3.233251058));
#144092=CARTESIAN_POINT('Ctrl Pts',(-6.306208544,1.457192641,3.576902822));
#144093=CARTESIAN_POINT('Ctrl Pts',(-6.29947043335412,1.45944932068712,
3.58878235378212));
#144094=CARTESIAN_POINT('Ctrl Pts',(-6.29273232270823,1.46170600037424,
3.60066188556422));
#144095=CARTESIAN_POINT('Origin',(0.182005772061442,1.33928763056823,-0.0807980551483395));
#144096=CARTESIAN_POINT('Ctrl Pts',(-6.398803776,1.457192641,3.912200178));
#144097=CARTESIAN_POINT('Ctrl Pts',(-6.185221277,1.391489877,4.261536214));
#144098=CARTESIAN_POINT('Ctrl Pts',(-5.934878233,1.326325889,4.585544717));
#144099=CARTESIAN_POINT('Ctrl Pts',(-6.306208544,1.457192641,3.576902822));
#144100=CARTESIAN_POINT('Ctrl Pts',(-6.110931255,1.391489877,3.921183718));
#144101=CARTESIAN_POINT('Ctrl Pts',(-5.87933494900001,1.326325889,4.242159893));
#144102=CARTESIAN_POINT('',(-5.88208657716348,1.32710049351043,4.23834372171454));
#144103=CARTESIAN_POINT('Origin',(0.17427700323462,1.48213094100688,-0.0940498837865111));
#144104=CARTESIAN_POINT('Ctrl Pts',(-6.08537345500619,1.36645689999237,
4.38386016046963));
#144105=CARTESIAN_POINT('Ctrl Pts',(-6.05148338649333,1.36020372539536,
4.35955152564049));
#144106=CARTESIAN_POINT('Ctrl Pts',(-6.01758186916682,1.35380222445104,
4.33525783063649));
#144107=CARTESIAN_POINT('Ctrl Pts',(-5.94983126380686,1.34069379764136,
4.28675901230052));
#144108=CARTESIAN_POINT('Ctrl Pts',(-5.91594449053718,1.33397958603012,
4.26252690812683));
#144109=CARTESIAN_POINT('Ctrl Pts',(-5.88208658128532,1.32710049374011,
4.23834371587839));
#144110=CARTESIAN_POINT('Ctrl Pts',(-6.22886134497013,1.326318298,4.1784155004681));
#144111=CARTESIAN_POINT('Ctrl Pts',(-6.00116195121403,1.391911284,4.51785229157823));
#144112=CARTESIAN_POINT('Ctrl Pts',(-5.73792577853377,1.457192641,4.83053594383523));
#144113=CARTESIAN_POINT('Ctrl Pts',(-5.728826094617,1.45944932065123,4.84134495375397));
#144114=CARTESIAN_POINT('Ctrl Pts',(-5.7197264107004,1.46170600030247,4.85215396367269));
#144115=CARTESIAN_POINT('Ctrl Pts',(-5.88483958600001,1.326318298,4.234520403));
#144116=CARTESIAN_POINT('Ctrl Pts',(-5.654082801,1.391911284,4.555210005));
#144117=CARTESIAN_POINT('Ctrl Pts',(-5.389844518,1.457192641,4.848925249));
#144118=CARTESIAN_POINT('Ctrl Pts',(-5.38071019261637,1.45944932065123,
4.85907854918939));
#144119=CARTESIAN_POINT('Ctrl Pts',(-5.37157586723272,1.46170600030247,
4.86923184937878));
#144120=CARTESIAN_POINT('Origin',(0.160381593158633,1.33928762122271,-0.118035070517558));
#144121=CARTESIAN_POINT('Ctrl Pts',(-5.408195905,1.457192641,5.196288777));
#144122=CARTESIAN_POINT('Ctrl Pts',(-5.124509925,1.391489877,5.491543606));
#144123=CARTESIAN_POINT('Ctrl Pts',(-4.810367512,1.326325889,5.754160616));
#144124=CARTESIAN_POINT('Ctrl Pts',(-5.389844518,1.457192641,4.848925249));
#144125=CARTESIAN_POINT('Ctrl Pts',(-5.125122489,1.391489877,5.143178203));
#144126=CARTESIAN_POINT('Ctrl Pts',(-4.829940385,1.326325889,5.406863774));
#144127=CARTESIAN_POINT('',(-4.83344804852087,1.3271004938086,5.40372834108578));
#144128=CARTESIAN_POINT('Origin',(0.14998457613528,1.4821310466166,-0.129315447734775));
#144129=CARTESIAN_POINT('Ctrl Pts',(-5.00070045707493,1.36645689999032,
5.58954335620345));
#144130=CARTESIAN_POINT('Ctrl Pts',(-4.9728283573888,1.36020372537749,5.55851768078015));
#144131=CARTESIAN_POINT('Ctrl Pts',(-4.94494186503069,1.35380222444764,
5.52750413492136));
#144132=CARTESIAN_POINT('Ctrl Pts',(-4.88920104311748,1.34069379760003,
5.46557481462023));
#144133=CARTESIAN_POINT('Ctrl Pts',(-4.86131571074869,1.33397958624442,
5.43462459034137));
#144134=CARTESIAN_POINT('Ctrl Pts',(-4.83344805172475,1.32710049394251,
5.40372833816614));
#144135=CARTESIAN_POINT('Ctrl Pts',(-5.18499820863661,1.326318298,5.41974753300653));
#144136=CARTESIAN_POINT('Ctrl Pts',(-4.8896534235684,1.391911284,5.70229984158403));
#144137=CARTESIAN_POINT('Ctrl Pts',(-4.56535382460105,1.457192641,5.95108512861539));
#144138=CARTESIAN_POINT('Ctrl Pts',(-4.55414326908976,1.45944932056061,
5.95968526651115));
#144139=CARTESIAN_POINT('Ctrl Pts',(-4.54293271357833,1.46170600012122,
5.96828540440697));
#144140=CARTESIAN_POINT('Ctrl Pts',(-4.836958592,1.326318298,5.400586226));
#144141=CARTESIAN_POINT('Ctrl Pts',(-4.54265798800001,1.391911284,5.664172395));
#144142=CARTESIAN_POINT('Ctrl Pts',(-4.221457354,1.457192641,5.89421732));
#144143=CARTESIAN_POINT('Ctrl Pts',(-4.21035392510525,1.45944932056061,
5.90216963141211));
#144144=CARTESIAN_POINT('Ctrl Pts',(-4.1992504962105,1.46170600012122,5.91012194282422));
#144145=CARTESIAN_POINT('Origin',(0.131257950572324,1.3392875952123,-0.149752816308679));
#144146=CARTESIAN_POINT('Ctrl Pts',(-4.164706805,1.457192641,6.237404687));
#144147=CARTESIAN_POINT('Ctrl Pts',(-3.824182184,1.391489877,6.464772523));
#144148=CARTESIAN_POINT('Ctrl Pts',(-3.460929352,1.326325889,6.653718361));
#144149=CARTESIAN_POINT('Ctrl Pts',(-4.221457354,1.457192641,5.89421732));
#144150=CARTESIAN_POINT('Ctrl Pts',(-3.89966869,1.391489877,6.124683393));
#144151=CARTESIAN_POINT('Ctrl Pts',(-3.554703177,1.326325889,6.318748715));
#144152=CARTESIAN_POINT('',(-3.55880285644889,1.32710049347857,6.3164406300595));
#144153=CARTESIAN_POINT('Origin',(0.118678978891426,1.48213094058367,-0.158534356723926));
#144154=CARTESIAN_POINT('Ctrl Pts',(-3.68220026361416,1.36645690003059,
6.53386571770354));
#144155=CARTESIAN_POINT('Ctrl Pts',(-3.66164940112487,1.36020372540053,
6.49757372770157));
#144156=CARTESIAN_POINT('Ctrl Pts',(-3.64108187499581,1.35380222446052,
6.46129048970569));
#144157=CARTESIAN_POINT('Ctrl Pts',(-3.59995721578982,1.34069379762435,
6.38882641346529));
#144158=CARTESIAN_POINT('Ctrl Pts',(-3.57937720959691,1.33397958601979,
6.35260526465788));
#144159=CARTESIAN_POINT('Ctrl Pts',(-3.55880286204966,1.3271004937455,6.31644062682241));
#144160=CARTESIAN_POINT('Ctrl Pts',(-3.89869031899553,1.326318298,6.4076581951046));
#144161=CARTESIAN_POINT('Ctrl Pts',(-3.5495101372942,1.391911284,6.62011418952326));
#144162=CARTESIAN_POINT('Ctrl Pts',(-3.17931099982432,1.457192641,6.79336818647255));
#144163=CARTESIAN_POINT('Ctrl Pts',(-3.16651376501828,1.45944932063382,
6.79935732003778));
#144164=CARTESIAN_POINT('Ctrl Pts',(-3.15371653021228,1.46170600026764,
6.80534645360308));
#144165=CARTESIAN_POINT('Ctrl Pts',(-3.56290679,1.326318298,6.314126639));
#144166=CARTESIAN_POINT('Ctrl Pts',(-3.218823535,1.391911284,6.50828438));
#144167=CARTESIAN_POINT('Ctrl Pts',(-2.855679535,1.457192641,6.66390234));
#144168=CARTESIAN_POINT('Ctrl Pts',(-2.84312618582646,1.45944932063382,
6.66928182193984));
#144169=CARTESIAN_POINT('Ctrl Pts',(-2.83057283665291,1.46170600026764,
6.67466130387953));
#144170=CARTESIAN_POINT('Origin',(0.09599672438588,1.33928764452021,-0.174468164838252));
#144171=CARTESIAN_POINT('Ctrl Pts',(-2.726480643,1.457192641,6.986866487));
#144172=CARTESIAN_POINT('Ctrl Pts',(-2.345039935,1.391489877,7.135715861));
#144173=CARTESIAN_POINT('Ctrl Pts',(-1.949661982,1.326325889,7.242155629));
#144174=CARTESIAN_POINT('Ctrl Pts',(-2.855679535,1.457192641,6.66390234));
#144175=CARTESIAN_POINT('Ctrl Pts',(-2.491870718,1.391489877,6.81980519300001));
#144176=CARTESIAN_POINT('Ctrl Pts',(-2.113252,1.326325889,6.935175988));
#144177=CARTESIAN_POINT('',(-2.11775200048965,1.32710049345207,6.93380317484552));
#144178=CARTESIAN_POINT('Origin',(0.081824182827851,1.48213092866479,-0.180340533094112));
#144179=CARTESIAN_POINT('Ctrl Pts',(-2.19152447788043,1.3664568999714,7.17267177956051));
#144180=CARTESIAN_POINT('Ctrl Pts',(-2.17925578824896,1.36020372535492,
7.13281044820063));
#144181=CARTESIAN_POINT('Ctrl Pts',(-2.16696894311951,1.35380222440394,
7.09295408190761));
#144182=CARTESIAN_POINT('Ctrl Pts',(-2.14238322001099,1.34069370685812,
7.01334303852864));
#144183=CARTESIAN_POINT('Ctrl Pts',(-2.1300709296158,1.33397954135704,6.97354492030573));
#144184=CARTESIAN_POINT('Ctrl Pts',(-2.11775200705747,1.32710049367607,
6.9338031727709));
#144185=CARTESIAN_POINT('Ctrl Pts',(-2.43008400264679,1.326318298,7.09595388132399));
#144186=CARTESIAN_POINT('Ctrl Pts',(-2.04339570073183,1.391911284,7.22837935535174));
#144187=CARTESIAN_POINT('Ctrl Pts',(-1.64460712498484,1.457192641,7.31800089883336));
#144188=CARTESIAN_POINT('Ctrl Pts',(-1.63082159570203,1.45944932063747,
7.32109898259795));
#144189=CARTESIAN_POINT('Ctrl Pts',(-1.61703606641928,1.46170600027495,
7.32419706636265));
#144190=CARTESIAN_POINT('Ctrl Pts',(-2.122257426,1.326318298,6.932425508));
#144191=CARTESIAN_POINT('Ctrl Pts',(-1.744480471,1.391911284,7.04807622));
#144192=CARTESIAN_POINT('Ctrl Pts',(-1.356373314,1.457192641,7.121990693));
#144193=CARTESIAN_POINT('Ctrl Pts',(-1.34295702551262,1.45944932063747,
7.12454580664653));
#144194=CARTESIAN_POINT('Ctrl Pts',(-1.32954073702527,1.46170600027495,
7.1271009202929));
#144195=CARTESIAN_POINT('Origin',(0.0562468783962666,1.33928763488106,-0.191025668185087));
#144196=CARTESIAN_POINT('Ctrl Pts',(-1.160767276,1.457192641,7.409630175));
#144197=CARTESIAN_POINT('Ctrl Pts',(-0.756246224,1.391489877,7.473001057));
#144198=CARTESIAN_POINT('Ctrl Pts',(-0.347230585,1.326325889,7.49195775));
#144199=CARTESIAN_POINT('Ctrl Pts',(-1.356373314,1.457192641,7.121990693));
#144200=CARTESIAN_POINT('Ctrl Pts',(-0.967555641,1.391489877,7.196040483));
#144201=CARTESIAN_POINT('Ctrl Pts',(-0.572987507,1.326325889,7.22732214));
#144202=CARTESIAN_POINT('',(-0.577677415430962,1.32710049363407,7.22694878972836));
#144203=CARTESIAN_POINT('Origin',(0.0411433145576777,1.48213100234167,-0.193714029734774));
#144204=CARTESIAN_POINT('Ctrl Pts',(-0.598375443566073,1.36645689998275,
7.47609168121661));
#144205=CARTESIAN_POINT('Ctrl Pts',(-0.594962597040865,1.36020372536892,
7.43452488005759));
#144206=CARTESIAN_POINT('Ctrl Pts',(-0.591530952127597,1.35380222444649,
7.39295902513781));
#144207=CARTESIAN_POINT('Ctrl Pts',(-0.584634098175082,1.34069379761045,
7.30992461451379));
#144208=CARTESIAN_POINT('Ctrl Pts',(-0.581165056043418,1.33397958602485,
7.26840986999439));
#144209=CARTESIAN_POINT('Ctrl Pts',(-0.577677421155283,1.32710049373197,
7.2269487892306));
#144210=CARTESIAN_POINT('Ctrl Pts',(-0.847849659089698,1.326318298,7.45245065089731));
#144211=CARTESIAN_POINT('Ctrl Pts',(-0.441734353150813,1.391911284,7.49865353618925));
#144212=CARTESIAN_POINT('Ctrl Pts',(-0.0330032499786711,1.457192641,7.50045202179782));
#144213=CARTESIAN_POINT('Ctrl Pts',(-0.0188740223279256,1.45944932062933,
7.50051419277624));
#144214=CARTESIAN_POINT('Ctrl Pts',(-0.00474479467718063,1.46170600025867,
7.50057636375466));
#144215=CARTESIAN_POINT('Ctrl Pts',(-0.582373663,1.326318298,7.22657186500001));
#144216=CARTESIAN_POINT('Ctrl Pts',(-0.18856744,1.391911284,7.25830784900001));
#144217=CARTESIAN_POINT('Ctrl Pts',(0.206355414,1.457192641,7.247062677));
#144218=CARTESIAN_POINT('Ctrl Pts',(0.220007310969285,1.45944932062933,
7.24667394809262));
#144219=CARTESIAN_POINT('Ctrl Pts',(0.233659207938571,1.46170600025867,
7.24628521918508));
#144220=CARTESIAN_POINT('Origin',(0.0138669977767894,1.33928758393614,-0.198651021090203));
#144221=CARTESIAN_POINT('Ctrl Pts',(-1.360746905,4.560731746,7.121156357));
#144222=CARTESIAN_POINT('Ctrl Pts',(-0.969780916,4.495065281,7.195864134));
#144223=CARTESIAN_POINT('Ctrl Pts',(-0.572986203,4.430609079,7.227322244));
#144224=CARTESIAN_POINT('Ctrl Pts',(-1.648506461,4.560731746,7.31658571));
#144225=CARTESIAN_POINT('Ctrl Pts',(-1.246811002,4.495065281,7.407092072));
#144226=CARTESIAN_POINT('Ctrl Pts',(-0.837621771,4.430609079,7.453079214));
#144227=CARTESIAN_POINT('',(-1.35606856648098,4.55994605296445,7.12204874014566));
#144228=CARTESIAN_POINT('Origin',(0.0577273861491251,4.69628092964401,-0.182460475736631));
#144229=CARTESIAN_POINT('Ctrl Pts',(-1.40181135298698,4.5206323408617,7.36783040874985));
#144230=CARTESIAN_POINT('Ctrl Pts',(-1.39421544816574,4.52686607840845,
7.32681968872307));
#144231=CARTESIAN_POINT('Ctrl Pts',(-1.38660265533698,4.53325386659101,
7.28581108465512));
#144232=CARTESIAN_POINT('Ctrl Pts',(-1.37135868269627,4.54634733293425,
7.2038974290939));
#144233=CARTESIAN_POINT('Ctrl Pts',(-1.36371859852423,4.5530606542029,7.16294451736904));
#144234=CARTESIAN_POINT('Ctrl Pts',(-1.35606856762555,4.55994605042158,
7.12204873950343));
#144235=CARTESIAN_POINT('Ctrl Pts',(-2.113250748,4.430609079,6.93517637));
#144236=CARTESIAN_POINT('Ctrl Pts',(-1.73744496,4.495496505,7.04968994800001));
#144237=CARTESIAN_POINT('Ctrl Pts',(-1.351465456,4.560723991,7.122923636));
#144238=CARTESIAN_POINT('Ctrl Pts',(-1.949660675,4.430609079,7.242155981));
#144239=CARTESIAN_POINT('Ctrl Pts',(-1.557220167,4.495496505,7.34780488300001));
#144240=CARTESIAN_POINT('Ctrl Pts',(-1.155661261,4.560723991,7.410428264));
#144241=CARTESIAN_POINT('Origin',(0.0382436804201319,4.55356860646856,-0.195301735550543));
#144242=CARTESIAN_POINT('Ctrl Pts',(-2.859771516,4.560731746,6.662147317));
#144243=CARTESIAN_POINT('Ctrl Pts',(-2.494006057,4.495065281,6.819154599));
#144244=CARTESIAN_POINT('Ctrl Pts',(-2.113250748,4.430609079,6.93517637));
#144245=CARTESIAN_POINT('Ctrl Pts',(-3.182814947,4.560731746,6.79114784200001));
#144246=CARTESIAN_POINT('Ctrl Pts',(-2.809967097,4.495065281,6.965890866));
#144247=CARTESIAN_POINT('Ctrl Pts',(-2.420230359,4.430609079,7.098766443));
#144248=CARTESIAN_POINT('',(-2.85539438941292,4.5599460519018,6.66402454208368));
#144249=CARTESIAN_POINT('Origin',(0.0956012963018976,4.69628105067334,-0.16578473521602));
#144250=CARTESIAN_POINT('Ctrl Pts',(-2.9529035287323,4.52063234088232,6.89422662433444));
#144251=CARTESIAN_POINT('Ctrl Pts',(-2.93666913907048,4.52686607086783,
6.85580765366949));
#144252=CARTESIAN_POINT('Ctrl Pts',(-2.92041868087003,4.53325386292767,
6.81739430829154));
#144253=CARTESIAN_POINT('Ctrl Pts',(-2.88792208022279,4.54634733289054,
6.74067273052007));
#144254=CARTESIAN_POINT('Ctrl Pts',(-2.87165695187537,4.55306065400379,
6.70231966810698));
#144255=CARTESIAN_POINT('Ctrl Pts',(-2.85539439105084,4.55994605023122,
6.66402454108774));
#144256=CARTESIAN_POINT('Ctrl Pts',(-3.554702037,4.430609079,6.318749356));
#144257=CARTESIAN_POINT('Ctrl Pts',(-3.212299413,4.495496505,6.511372807));
#144258=CARTESIAN_POINT('Ctrl Pts',(-2.851086974,4.560723991,6.665868515));
#144259=CARTESIAN_POINT('Ctrl Pts',(-3.460928151,4.430609079,6.653718985));
#144260=CARTESIAN_POINT('Ctrl Pts',(-3.100374075,4.495496505,6.841260983));
#144261=CARTESIAN_POINT('Ctrl Pts',(-2.721665569,4.560723991,6.988743559));
#144262=CARTESIAN_POINT('Origin',(0.0793335642572862,4.55356866085514,-0.182514228437093));
#144263=CARTESIAN_POINT('Ctrl Pts',(-4.225076389,4.560731746,5.891623674));
#144264=CARTESIAN_POINT('Ctrl Pts',(-3.901614248,4.495065281,6.123588974));
#144265=CARTESIAN_POINT('Ctrl Pts',(-3.554702037,4.430609079,6.318749356));
#144266=CARTESIAN_POINT('Ctrl Pts',(-4.568298544,4.560731746,5.948163449));
#144267=CARTESIAN_POINT('Ctrl Pts',(-4.241732254,4.495065281,6.198972345));
#144268=CARTESIAN_POINT('Ctrl Pts',(-3.889671666,4.430609079,6.412523242));
#144269=CARTESIAN_POINT('',(-4.22120514517481,4.55994605119118,5.8943979632248));
#144270=CARTESIAN_POINT('Origin',(0.129005056016454,4.69628090110764,-0.141357475232535));
#144271=CARTESIAN_POINT('Ctrl Pts',(-4.36592121772473,4.52063234083099,
6.09825646575287));
#144272=CARTESIAN_POINT('Ctrl Pts',(-4.34180743928622,4.52686606998888,
6.0642256277437));
#144273=CARTESIAN_POINT('Ctrl Pts',(-4.31767917226126,4.53325386248918,
6.0302037307579));
#144274=CARTESIAN_POINT('Ctrl Pts',(-4.26944945116903,4.54634733287894,
5.96226166741484));
#144275=CARTESIAN_POINT('Ctrl Pts',(-4.24531981791809,4.553060653944,5.92830180049015));
#144276=CARTESIAN_POINT('Ctrl Pts',(-4.22120514626668,4.55994605018937,
5.89439796224474));
#144277=CARTESIAN_POINT('Ctrl Pts',(-4.829939409,4.430609079,5.406864646));
#144278=CARTESIAN_POINT('Ctrl Pts',(-4.536950317,4.495496505,5.66859111));
#144279=CARTESIAN_POINT('Ctrl Pts',(-4.217394834,4.560723991,5.89712479200001));
#144280=CARTESIAN_POINT('Ctrl Pts',(-4.810366473,4.430609079,5.754161485));
#144281=CARTESIAN_POINT('Ctrl Pts',(-4.498557937,4.495496505,6.014827323));
#144282=CARTESIAN_POINT('Ctrl Pts',(-4.16040782,4.560723991,6.240272973));
#144283=CARTESIAN_POINT('Origin',(0.11671398827705,4.55356860863053,-0.161192793785231));
#144284=CARTESIAN_POINT('Ctrl Pts',(-5.392821385,4.560731746,4.845614255));
#144285=CARTESIAN_POINT('Ctrl Pts',(-5.126787292,4.495065281,5.141691134));
#144286=CARTESIAN_POINT('Ctrl Pts',(-4.829939409,4.430609079,5.406864646));
#144287=CARTESIAN_POINT('Ctrl Pts',(-5.74017357700001,4.560731746,4.827049544));
#144288=CARTESIAN_POINT('Ctrl Pts',(-5.475158725,4.495065281,5.142196766));
#144289=CARTESIAN_POINT('Ctrl Pts',(-5.177236248,4.430609079,5.426437582));
#144290=CARTESIAN_POINT('',(-5.38963703994329,4.5599460529448,4.84915588573557));
#144291=CARTESIAN_POINT('Origin',(0.156376705075179,4.69628091630223,-0.110320379162516));
#144292=CARTESIAN_POINT('Ctrl Pts',(-5.57479328282146,4.52063234083508,
5.01713861212511));
#144293=CARTESIAN_POINT('Ctrl Pts',(-5.54392760548432,4.52686607834886,
4.98908710816598));
#144294=CARTESIAN_POINT('Ctrl Pts',(-5.51304976423063,4.53325386650049,
4.96104750887774));
#144295=CARTESIAN_POINT('Ctrl Pts',(-5.45134211096737,4.54634733285367,
4.90506187481746));
#144296=CARTESIAN_POINT('Ctrl Pts',(-5.42047624750108,4.55306065394299,
4.8770831284614));
#144297=CARTESIAN_POINT('Ctrl Pts',(-5.38963704040105,4.55994605021047,
4.84915588455593));
#144298=CARTESIAN_POINT('Ctrl Pts',(-5.879334183,4.430609079,4.242160954));
#144299=CARTESIAN_POINT('Ctrl Pts',(-5.649458466,4.495496505,4.560752393));
#144300=CARTESIAN_POINT('Ctrl Pts',(-5.386501999,4.560723991,4.852638067));
#144301=CARTESIAN_POINT('Ctrl Pts',(-5.934877406,4.430609079,4.585545789));
#144302=CARTESIAN_POINT('Ctrl Pts',(-5.68639423,4.495496505,4.907147023));
#144303=CARTESIAN_POINT('Ctrl Pts',(-5.404614025,4.560723991,5.200014158));
#144304=CARTESIAN_POINT('Origin',(0.148636968836049,4.55356862890809,-0.132334142890484));
#144305=CARTESIAN_POINT('Ctrl Pts',(-6.308404047,4.560731746,3.573029299));
#144306=CARTESIAN_POINT('Ctrl Pts',(-6.112237461,4.495065281,3.919373532));
#144307=CARTESIAN_POINT('Ctrl Pts',(-5.879334183,4.430609079,4.242160954));
#144308=CARTESIAN_POINT('Ctrl Pts',(-6.643644474,4.560731746,3.480228168));
#144309=CARTESIAN_POINT('Ctrl Pts',(-6.452572859,4.495065281,3.844977782));
#144310=CARTESIAN_POINT('Ctrl Pts',(-6.222719017,4.430609079,4.186617732));
#144311=CARTESIAN_POINT('',(-6.30605549550747,4.55994605292005,3.57717266853147));
#144312=CARTESIAN_POINT('Origin',(0.176436100078936,4.69628087970373,-0.0741246307395643));
#144313=CARTESIAN_POINT('Ctrl Pts',(-6.52299420951789,4.5206323408474,3.7014249337822));
#144314=CARTESIAN_POINT('Ctrl Pts',(-6.48681995482906,4.52686607071593,
3.68066449205128));
#144315=CARTESIAN_POINT('Ctrl Pts',(-6.45063631117384,4.53325386286174,
3.65991825214407));
#144316=CARTESIAN_POINT('Ctrl Pts',(-6.37833607187533,4.54634733289592,
3.61850684058568));
#144317=CARTESIAN_POINT('Ctrl Pts',(-6.34217723114368,4.55306065409343,
3.59781746951568));
#144318=CARTESIAN_POINT('Ctrl Pts',(-6.30605549594104,4.55994605029829,
3.57717266689845));
#144319=CARTESIAN_POINT('Ctrl Pts',(-6.653817825,4.430609079,2.879098531));
#144320=CARTESIAN_POINT('Ctrl Pts',(-6.497804216,4.495496505,3.239657963));
#144321=CARTESIAN_POINT('Ctrl Pts',(-6.303742317,4.560723991,3.58124738));
#144322=CARTESIAN_POINT('Ctrl Pts',(-6.781880067,4.430609079,3.202515068));
#144323=CARTESIAN_POINT('Ctrl Pts',(-6.60834104800001,4.495496505,3.570013982));
#144324=CARTESIAN_POINT('Ctrl Pts',(-6.396106485,4.560723991,3.916608461));
#144325=CARTESIAN_POINT('Origin',(0.173609964768517,4.55356862217885,-0.097287761415224));
#144326=CARTESIAN_POINT('Ctrl Pts',(-6.929012748,4.560731746,2.133373465));
#144327=CARTESIAN_POINT('Ctrl Pts',(-6.811886199,4.495065281,2.513790379));
#144328=CARTESIAN_POINT('Ctrl Pts',(-6.653817825,4.430609079,2.879098531));
#144329=CARTESIAN_POINT('Ctrl Pts',(-7.23646594,4.560731746,1.97067519));
#144330=CARTESIAN_POINT('Ctrl Pts',(-7.128271858,4.495065281,2.36797191));
#144331=CARTESIAN_POINT('Ctrl Pts',(-6.977234361,4.430609079,2.751036289));
#144332=CARTESIAN_POINT('',(-6.92760980555269,4.55994605295033,2.13792483369843));
#144333=CARTESIAN_POINT('Origin',(0.188246019437727,4.69628090910426,-0.0344631924695157));
#144334=CARTESIAN_POINT('Ctrl Pts',(-7.16618717754861,4.52063234083719,
2.21263673886221));
#144335=CARTESIAN_POINT('Ctrl Pts',(-7.12639577943664,4.52686607009583,
2.20013806147034));
#144336=CARTESIAN_POINT('Ctrl Pts',(-7.08659825869315,4.53325386258683,
2.18765527027095));
#144337=CARTESIAN_POINT('Ctrl Pts',(-7.00708612763528,4.54634733295565,
2.16275444828854));
#144338=CARTESIAN_POINT('Ctrl Pts',(-6.96732505701765,4.55306065423035,
2.15032186507111));
#144339=CARTESIAN_POINT('Ctrl Pts',(-6.92760980569743,4.5599460504648,2.13792483185427));
#144340=CARTESIAN_POINT('Ctrl Pts',(-7.11717634,4.430609079,1.381412661));
#144341=CARTESIAN_POINT('Ctrl Pts',(-7.04231986300001,4.495496505,1.767080728));
#144342=CARTESIAN_POINT('Ctrl Pts',(-6.926226651,4.560723991,2.142401545));
#144343=CARTESIAN_POINT('Ctrl Pts',(-7.311769554,4.430609079,1.669738302));
#144344=CARTESIAN_POINT('Ctrl Pts',(-7.221289184,4.495496505,2.065951054));
#144345=CARTESIAN_POINT('Ctrl Pts',(-7.08852411500001,4.560723991,2.450066505));
#144346=CARTESIAN_POINT('Origin',(0.190464918460429,4.55356864800771,-0.0576921838180541));
#144347=CARTESIAN_POINT('Ctrl Pts',(-7.22562851299999,4.560731746,0.593963458000001));
#144348=CARTESIAN_POINT('Ctrl Pts',(-7.193018709,4.495065281,0.990665182));
#144349=CARTESIAN_POINT('Ctrl Pts',(-7.11717634,4.430609079,1.381412661));
#144350=CARTESIAN_POINT('Ctrl Pts',(-7.4909183,4.560731746,0.36897563));
#144351=CARTESIAN_POINT('Ctrl Pts',(-7.470660787,4.495065281,0.780242304));
#144352=CARTESIAN_POINT('Ctrl Pts',(-7.405501982,4.430609079,1.186819448));
#144353=CARTESIAN_POINT('',(-7.22523678108189,4.55994605191336,0.598710009952617));
#144354=CARTESIAN_POINT('Origin',(0.191253352314371,4.69628107715055,0.006809920091582));
#144355=CARTESIAN_POINT('Ctrl Pts',(-7.47429719712508,4.52063234086681,
0.620388109190184));
#144356=CARTESIAN_POINT('Ctrl Pts',(-7.43274924743436,4.52686607103456,
0.616735617684281));
#144357=CARTESIAN_POINT('Ctrl Pts',(-7.39119874307093,4.53325386299204,
0.613099958047266));
#144358=CARTESIAN_POINT('Ctrl Pts',(-7.30819262379926,4.54634733285042,
0.605874061569169));
#144359=CARTESIAN_POINT('Ctrl Pts',(-7.26668850755719,4.55306065402255,
0.602279600214153));
#144360=CARTESIAN_POINT('Ctrl Pts',(-7.22523678098004,4.55994605025539,
0.598710007937322));
#144361=CARTESIAN_POINT('Ctrl Pts',(-7.2477436,4.430609079,-0.180866531));
#144362=CARTESIAN_POINT('Ctrl Pts',(-7.25754446000001,4.495496505,0.211876761));
#144363=CARTESIAN_POINT('Ctrl Pts',(-7.22484832400001,4.560723991,0.603379396));
#144364=CARTESIAN_POINT('Ctrl Pts',(-7.499768822,4.430609079,0.0588864280000001));
#144365=CARTESIAN_POINT('Ctrl Pts',(-7.496577864,4.495496505,0.465286552));
#144366=CARTESIAN_POINT('Ctrl Pts',(-7.449490235,4.560723991,0.868962162));
#144367=CARTESIAN_POINT('Origin',(0.198414091241863,4.55356862013888,-0.015399037139459));
#144368=CARTESIAN_POINT('Ctrl Pts',(-7.18438192,4.560731746,-0.97321962));
#144369=CARTESIAN_POINT('Ctrl Pts',(-7.23781366,4.495065281,-0.578782418));
#144370=CARTESIAN_POINT('Ctrl Pts',(-7.2477436,4.430609079,-0.180866531));
#144371=CARTESIAN_POINT('Ctrl Pts',(-7.39510364700001,4.560731746,-1.24997682));
#144372=CARTESIAN_POINT('Ctrl Pts',(-7.463729921,4.495065281,-0.843970566000001));
#144373=CARTESIAN_POINT('Ctrl Pts',(-7.48749656,4.430609079,-0.432891753));
#144374=CARTESIAN_POINT('',(-7.18501971399298,4.55994605292029,-0.968499829450406));
#144375=CARTESIAN_POINT('Origin',(0.185317934164564,4.69628089020531,0.0477644810005477));
#144376=CARTESIAN_POINT('Ctrl Pts',(-7.43291738742458,4.52063234081501,
-1.00086917885161));
#144377=CARTESIAN_POINT('Ctrl Pts',(-7.39155563326788,4.52686607020261,
-0.995504696753631));
#144378=CARTESIAN_POINT('Ctrl Pts',(-7.35019499414071,4.53325386262189,
-0.99012322604503));
#144379=CARTESIAN_POINT('Ctrl Pts',(-7.26757615490632,4.54634733292811,
-0.979336322679522));
#144380=CARTESIAN_POINT('Ctrl Pts',(-7.22626967855141,4.55306065415589,
-0.973924589329539));
#144381=CARTESIAN_POINT('Ctrl Pts',(-7.18501971341777,4.55994605038715,
-0.968499830609143));
#144382=CARTESIAN_POINT('Ctrl Pts',(-7.039414425,4.430609079,-1.734688604));
#144383=CARTESIAN_POINT('Ctrl Pts',(-7.133414344,4.495496505,-1.353234327));
#144384=CARTESIAN_POINT('Ctrl Pts',(-7.185644119,4.560723991,-0.963856104));
#144385=CARTESIAN_POINT('Ctrl Pts',(-7.337087236,4.430609079,-1.554718909));
#144386=CARTESIAN_POINT('Ctrl Pts',(-7.421334894,4.495496505,-1.157134232));
#144387=CARTESIAN_POINT('Ctrl Pts',(-7.462126472,4.560723991,-0.752773886));
#144388=CARTESIAN_POINT('Origin',(0.197085704958381,4.55356864071035,0.0276141514613945));
#144389=CARTESIAN_POINT('Ctrl Pts',(-6.807201613,4.560731746,-2.49489603));
#144390=CARTESIAN_POINT('Ctrl Pts',(-6.94417648700001,4.495065281,-2.121166795));
#144391=CARTESIAN_POINT('Ctrl Pts',(-7.039414425,4.430609079,-1.734688604));
#144392=CARTESIAN_POINT('Ctrl Pts',(-6.953502166,4.560731746,-2.810481743));
#144393=CARTESIAN_POINT('Ctrl Pts',(-7.107803339,4.495065281,-2.428720309));
#144394=CARTESIAN_POINT('Ctrl Pts',(-7.21938412,4.430609079,-2.032361415));
#144395=CARTESIAN_POINT('',(-6.80883911175384,4.5599460529445,-2.49042369268795));
#144396=CARTESIAN_POINT('Origin',(0.170717629805369,4.69628090722908,0.0864857378835263));
#144397=CARTESIAN_POINT('Ctrl Pts',(-7.043982621342,4.52063234084788,-2.57532693620973));
#144398=CARTESIAN_POINT('Ctrl Pts',(-7.00474108494821,4.52686607057047,
-2.56119631750548));
#144399=CARTESIAN_POINT('Ctrl Pts',(-6.9655042930369,4.5332538627838,-2.54704934835764));
#144400=CARTESIAN_POINT('Ctrl Pts',(-6.88713590294052,4.54634733289551,
-2.51875402924257));
#144401=CARTESIAN_POINT('Ctrl Pts',(-6.84795851182919,4.55306065412239,
-2.50458914798822));
#144402=CARTESIAN_POINT('Ctrl Pts',(-6.80883911077304,4.55994605037372,
-2.49042369414695));
#144403=CARTESIAN_POINT('Ctrl Pts',(-6.501930055,4.430609079,-3.207398566));
#144404=CARTESIAN_POINT('Ctrl Pts',(-6.675733702,4.495496505,-2.855069682));
#144405=CARTESIAN_POINT('Ctrl Pts',(-6.81044718200001,4.560723991,-2.486022764));
#144406=CARTESIAN_POINT('Ctrl Pts',(-6.831331606,4.430609079,-3.095627318));
#144407=CARTESIAN_POINT('Ctrl Pts',(-6.999078553,4.495496505,-2.725448706));
#144408=CARTESIAN_POINT('Ctrl Pts',(-7.12584196800001,4.560723991,-2.339311063));
#144409=CARTESIAN_POINT('Origin',(0.186541774057719,4.55356866174391,0.0693361714658935));
#144410=CARTESIAN_POINT('Ctrl Pts',(-6.111724124,4.560731746,-3.899913875));
#144411=CARTESIAN_POINT('Ctrl Pts',(-6.32583734,4.495065281,-3.564367771));
#144412=CARTESIAN_POINT('Ctrl Pts',(-6.501930055,4.430609079,-3.207398566));
#144413=CARTESIAN_POINT('Ctrl Pts',(-6.186762652,4.560731746,-4.239571663));
#144414=CARTESIAN_POINT('Ctrl Pts',(-6.419523772,4.495065281,-3.899905791));
#144415=CARTESIAN_POINT('Ctrl Pts',(-6.61370130300001,4.430609079,-3.536800117));
#144416=CARTESIAN_POINT('',(-6.11428476024427,4.55994605194144,-3.89589811155743));
#144417=CARTESIAN_POINT('Origin',(0.148134494419526,4.69628102985038,0.121163037151322));
#144418=CARTESIAN_POINT('Ctrl Pts',(-6.32567905648816,4.52063234086436,
-4.02936526868397));
#144419=CARTESIAN_POINT('Ctrl Pts',(-6.29039262764739,4.52686607114115,
-4.00712924358968));
#144420=CARTESIAN_POINT('Ctrl Pts',(-6.25511435220891,4.53325386303843,
-3.98487827339725));
#144421=CARTESIAN_POINT('Ctrl Pts',(-6.18466083040304,4.54634733283927,
-3.94039759680153));
#144422=CARTESIAN_POINT('Ctrl Pts',(-6.14944441594127,4.55306065401075,
-3.91814190177734));
#144423=CARTESIAN_POINT('Ctrl Pts',(-6.1142847585915,4.55994605024559,-3.89589811364495));
#144424=CARTESIAN_POINT('Ctrl Pts',(-5.660422662,4.430609079,-4.530134136));
#144425=CARTESIAN_POINT('Ctrl Pts',(-5.905903171,4.495496505,-4.223405152));
#144426=CARTESIAN_POINT('Ctrl Pts',(-6.116801304,4.560723991,-3.891945762));
#144427=CARTESIAN_POINT('Ctrl Pts',(-6.006150502,4.430609079,-4.491787634));
#144428=CARTESIAN_POINT('Ctrl Pts',(-6.249553078,4.495496505,-4.166324228));
#144429=CARTESIAN_POINT('Ctrl Pts',(-6.456361013,4.560723991,-3.816464655));
#144430=CARTESIAN_POINT('Origin',(0.167275480686609,4.55356864254791,0.107816230719945));
#144431=CARTESIAN_POINT('Ctrl Pts',(-5.130469208,4.560731746,-5.12257608100001));
#144432=CARTESIAN_POINT('Ctrl Pts',(-5.41170907,4.495065281,-4.840902871));
#144433=CARTESIAN_POINT('Ctrl Pts',(-5.660422662,4.430609079,-4.530134136));
#144434=CARTESIAN_POINT('Ctrl Pts',(-5.130736993,4.560731746,-5.47042392400001));
#144435=CARTESIAN_POINT('Ctrl Pts',(-5.431074409,4.495065281,-5.188736012));
#144436=CARTESIAN_POINT('Ctrl Pts',(-5.698769164,4.430609079,-4.875861977));
#144437=CARTESIAN_POINT('',(-5.13383324781926,4.55994605191712,-5.11920466472031));
#144438=CARTESIAN_POINT('Origin',(0.11862458411485,4.69628102230035,0.15017473185948));
#144439=CARTESIAN_POINT('Ctrl Pts',(-5.31159377015465,4.52063234085165,
-5.29499495952915));
#144440=CARTESIAN_POINT('Ctrl Pts',(-5.28191237189894,4.52686607840367,
-5.26569322704215));
#144441=CARTESIAN_POINT('Ctrl Pts',(-5.25224220241832,4.53325386656604,
-5.2363787040736));
#144442=CARTESIAN_POINT('Ctrl Pts',(-5.19299789108451,4.54634733290202,
-5.17779255156786));
#144443=CARTESIAN_POINT('Ctrl Pts',(-5.16338913336468,4.55306065406917,
-5.14848669395028));
#144444=CARTESIAN_POINT('Ctrl Pts',(-5.13383324626273,4.55994605026984,
-5.11920466590405));
#144445=CARTESIAN_POINT('Ctrl Pts',(-4.554240196,4.430609079,-5.641045669));
#144446=CARTESIAN_POINT('Ctrl Pts',(-4.859919172,4.495496505,-5.394258892));
#144447=CARTESIAN_POINT('Ctrl Pts',(-5.13714059500001,4.560723991,-5.11588570100001));
#144448=CARTESIAN_POINT('Ctrl Pts',(-4.900128476,4.430609079,-5.677916952));
#144449=CARTESIAN_POINT('Ctrl Pts',(-5.207805447,4.495496505,-5.412387059));
#144450=CARTESIAN_POINT('Ctrl Pts',(-5.48498779400001,4.560723991,-5.115164602));
#144451=CARTESIAN_POINT('Origin',(0.14018715816885,4.55356858826164,0.141254600293736));
#144452=CARTESIAN_POINT('Ctrl Pts',(-3.909319254,4.560731746,-6.105712323));
#144453=CARTESIAN_POINT('Ctrl Pts',(-4.244535298,4.495065281,-5.891082733));
#144454=CARTESIAN_POINT('Ctrl Pts',(-4.554240196,4.430609079,-5.64104566900001));
#144455=CARTESIAN_POINT('Ctrl Pts',(-3.834803774,4.560731746,-6.44548524300001));
#144456=CARTESIAN_POINT('Ctrl Pts',(-4.188674043,4.495065281,-6.234946704));
#144457=CARTESIAN_POINT('Ctrl Pts',(-4.517368912,4.430609079,-5.98693394900001));
#144458=CARTESIAN_POINT('',(-3.9133293995001,4.55994605192187,-6.10314289857883));
#144459=CARTESIAN_POINT('Origin',(0.0835682302581803,4.69628105622506,0.172164714886408));
#144460=CARTESIAN_POINT('Ctrl Pts',(-4.04914426237964,4.52063234081625,
-6.31303657046451));
#144461=CARTESIAN_POINT('Ctrl Pts',(-4.02645583639726,4.52686606975115,
-6.27803932140012));
#144462=CARTESIAN_POINT('Ctrl Pts',(-4.00378107790903,4.5332538623673,-6.24303192029104));
#144463=CARTESIAN_POINT('Ctrl Pts',(-3.95851614221154,4.54634733286745,
-6.17307968194309));
#144464=CARTESIAN_POINT('Ctrl Pts',(-3.93589951412824,4.553060653963,-6.13809397195535));
#144465=CARTESIAN_POINT('Ctrl Pts',(-3.91332939753393,4.55994605021214,
-6.10314289951169));
#144466=CARTESIAN_POINT('Ctrl Pts',(-3.23510652,4.430609079,-6.488188176));
#144467=CARTESIAN_POINT('Ctrl Pts',(-3.586690754,4.495496505,-6.31288308));
#144468=CARTESIAN_POINT('Ctrl Pts',(-3.917272901,4.560723991,-6.100612512));
#144469=CARTESIAN_POINT('Ctrl Pts',(-3.564981888,4.430609079,-6.59855318500001));
#144470=CARTESIAN_POINT('Ctrl Pts',(-3.922546621,4.495496505,-6.405372686));
#144471=CARTESIAN_POINT('Ctrl Pts',(-4.257142641,4.560723991,-6.174685136));
#144472=CARTESIAN_POINT('Origin',(0.106544188479404,4.55356864375883,0.16808840343761));
#144473=CARTESIAN_POINT('Ctrl Pts',(-2.505373877,4.560731746,-6.803352243));
#144474=CARTESIAN_POINT('Ctrl Pts',(-2.878891773,4.495065281,-6.665802114));
#144475=CARTESIAN_POINT('Ctrl Pts',(-3.23510652,4.430609079,-6.488188176));
#144476=CARTESIAN_POINT('Ctrl Pts',(-2.359559393,4.560731746,-7.119162835));
#144477=CARTESIAN_POINT('Ctrl Pts',(-2.750415934,4.495065281,-6.98961821800001));
#144478=CARTESIAN_POINT('Ctrl Pts',(-3.124741511,4.430609079,-6.818063544));
#144479=CARTESIAN_POINT('',(-2.50984261641909,4.5599460529582,-6.80170495217655));
#144480=CARTESIAN_POINT('Origin',(0.0446040535887426,4.69628092221338,0.186104077523651));
#144481=CARTESIAN_POINT('Ctrl Pts',(-2.5973612689532,4.52063234086582,-7.03588760830941));
#144482=CARTESIAN_POINT('Ctrl Pts',(-2.58272665904205,4.52686607014102,
-6.99683123235439));
#144483=CARTESIAN_POINT('Ctrl Pts',(-2.5681075806911,4.53325386260306,-6.95776788295559));
#144484=CARTESIAN_POINT('Ctrl Pts',(-2.53893857804763,4.54634733296754,
-6.87972046655687));
#144485=CARTESIAN_POINT('Ctrl Pts',(-2.52437160761346,4.5530606541495,-6.84069079594136));
#144486=CARTESIAN_POINT('Ctrl Pts',(-2.50984261543137,4.55994605040824,
-6.80170495209429));
#144487=CARTESIAN_POINT('Ctrl Pts',(-1.764702859,4.430609079,-7.03195021400001));
#144488=CARTESIAN_POINT('Ctrl Pts',(-2.145752663,4.495496505,-6.936323872));
#144489=CARTESIAN_POINT('Ctrl Pts',(-2.51423788,4.560723991,-6.800081461));
#144490=CARTESIAN_POINT('Ctrl Pts',(-2.06314071,4.430609079,-7.210648404));
#144491=CARTESIAN_POINT('Ctrl Pts',(-2.453873874,4.495496505,-7.098850206));
#144492=CARTESIAN_POINT('Ctrl Pts',(-2.83023823,4.560723991,-6.94548425700001));
#144493=CARTESIAN_POINT('Origin',(0.067919130555496,4.55356865389157,0.187062182693583));
#144494=CARTESIAN_POINT('Ctrl Pts',(-0.984280001000001,4.560731746,-7.182874973));
#144495=CARTESIAN_POINT('Ctrl Pts',(-1.378634468,4.495065281,-7.128835996));
#144496=CARTESIAN_POINT('Ctrl Pts',(-1.764702859,4.430609079,-7.03195021400001));
#144497=CARTESIAN_POINT('Ctrl Pts',(-0.773984637,4.560731746,-7.45995628600001));
#144498=CARTESIAN_POINT('Ctrl Pts',(-1.183551433,4.495065281,-7.417462952));
#144499=CARTESIAN_POINT('Ctrl Pts',(-1.586004669,4.430609079,-7.330388065));
#144500=CARTESIAN_POINT('',(-0.988998383218425,4.55994605292971,-7.18222684270952));
#144501=CARTESIAN_POINT('Origin',(0.00355437245004808,4.69628093008518,
0.191341631742465));
#144502=CARTESIAN_POINT('Ctrl Pts',(-1.02412854958252,4.52063234085322,
-7.42974836134486));
#144503=CARTESIAN_POINT('Ctrl Pts',(-1.01823205495643,4.52686607013125,
-7.38845909318625));
#144504=CARTESIAN_POINT('Ctrl Pts',(-1.01235222786182,4.53325386256596,
-7.34716635363535));
#144505=CARTESIAN_POINT('Ctrl Pts',(-1.00064306753655,4.54634733286283,
-7.26467316949526));
#144506=CARTESIAN_POINT('Ctrl Pts',(-0.994806890059503,4.55306065407803,
-7.22342452261306));
#144507=CARTESIAN_POINT('Ctrl Pts',(-0.988998381499585,4.55994605029681,
-7.18222684251182));
#144508=CARTESIAN_POINT('Ctrl Pts',(-0.211783654,4.430609079,-7.246906077));
#144509=CARTESIAN_POINT('Ctrl Pts',(-0.604481562,4.495496505,-7.235429869));
#144510=CARTESIAN_POINT('Ctrl Pts',(-0.993639891,4.560723991,-7.18158616));
#144511=CARTESIAN_POINT('Ctrl Pts',(-0.464829365,4.430609079,-7.485581718));
#144512=CARTESIAN_POINT('Ctrl Pts',(-0.870460713,4.495496505,-7.46039338));
#144513=CARTESIAN_POINT('Ctrl Pts',(-1.270995025,4.560723991,-7.391520253));
#144514=CARTESIAN_POINT('Origin',(0.0261184061916772,4.5535686433715,0.197289686172826));
#144515=CARTESIAN_POINT('Ctrl Pts',(0.582837713,4.560731746,-7.226534453));
#144516=CARTESIAN_POINT('Ctrl Pts',(0.186086252,4.495065281,-7.258533431));
#144517=CARTESIAN_POINT('Ctrl Pts',(-0.211783654,4.430609079,-7.246906077));
#144518=CARTESIAN_POINT('Ctrl Pts',(0.847780781,4.560731746,-7.451930471));
#144519=CARTESIAN_POINT('Ctrl Pts',(0.438654618,4.495065281,-7.498475363));
#144520=CARTESIAN_POINT('Ctrl Pts',(0.026891988,4.430609079,-7.499951788));
#144521=CARTESIAN_POINT('',(0.578090315769926,4.55994605294543,-7.22691578804906));
#144522=CARTESIAN_POINT('Origin',(-0.037661533011655,4.6962809452755,0.187632234919998));
#144523=CARTESIAN_POINT('Ctrl Pts',(0.596991283107554,4.52063234082553,
-7.47620233865752));
#144524=CARTESIAN_POINT('Ctrl Pts',(0.593873944611452,4.52686607835563,
-7.43461076353673));
#144525=CARTESIAN_POINT('Ctrl Pts',(0.590739588336727,4.533253866525,-7.39301946604933));
#144526=CARTESIAN_POINT('Ctrl Pts',(0.58444140058795,4.54634733287727,-7.30993782852142));
#144527=CARTESIAN_POINT('Ctrl Pts',(0.581273891583123,4.55306065410427,
-7.26839894647494));
#144528=CARTESIAN_POINT('Ctrl Pts',(0.578090316875135,4.55994605036328,
-7.22691578753565));
#144529=CARTESIAN_POINT('Ctrl Pts',(1.35103832,4.430609079,-7.123004665));
#144530=CARTESIAN_POINT('Ctrl Pts',(0.965054425,4.495496505,-7.196215207));
#144531=CARTESIAN_POINT('Ctrl Pts',(0.573419596,4.560723991,-7.227287871));
#144532=CARTESIAN_POINT('Ctrl Pts',(1.155216884,4.430609079,-7.410497551));
#144533=CARTESIAN_POINT('Ctrl Pts',(0.753654224,4.495496505,-7.473096852));
#144534=CARTESIAN_POINT('Ctrl Pts',(0.347678495,4.560723991,-7.491936977));
#144535=CARTESIAN_POINT('Origin',(-0.0169036609393039,4.55356866514041,
0.198291733154583));
#144536=CARTESIAN_POINT('Ctrl Pts',(2.122702584,4.560731746,-6.932289213));
#144537=CARTESIAN_POINT('Ctrl Pts',(1.742105785,4.495065281,-7.04882990900001));
#144538=CARTESIAN_POINT('Ctrl Pts',(1.35103832,4.430609079,-7.123004665));
#144539=CARTESIAN_POINT('Ctrl Pts',(2.429904911,4.560731746,-7.09546067));
#144540=CARTESIAN_POINT('Ctrl Pts',(2.040349667,4.495065281,-7.2288674));
#144541=CARTESIAN_POINT('Ctrl Pts',(1.638531205,4.430609079,-7.3188261));
#144542=CARTESIAN_POINT('',(2.11814815318168,4.5599460529599,-6.93368218303114));
#144543=CARTESIAN_POINT('Origin',(-0.0771164253400619,4.69628089233295,
0.17514947035037));
#144544=CARTESIAN_POINT('Ctrl Pts',(2.19019646628858,4.5206323408352,-7.1730774035426));
#144545=CARTESIAN_POINT('Ctrl Pts',(2.17821106626066,4.52686607006686,-7.13312840511856));
#144546=CARTESIAN_POINT('Ctrl Pts',(2.16620908142545,4.53325386254879,-7.09318325407002));
#144547=CARTESIAN_POINT('Ctrl Pts',(2.14219803858705,4.54634733288281,-7.0133979188787));
#144548=CARTESIAN_POINT('Ctrl Pts',(2.13017495246057,4.55306065418219,-6.9735111131108));
#144549=CARTESIAN_POINT('Ctrl Pts',(2.11814815529179,4.55994605040166,-6.93368218195171));
#144550=CARTESIAN_POINT('Ctrl Pts',(2.850687243,4.430609079,-6.666039472));
#144551=CARTESIAN_POINT('Ctrl Pts',(2.48946554,4.495496505,-6.82051352));
#144552=CARTESIAN_POINT('Ctrl Pts',(2.11366662,4.560723991,-6.935049634));
#144553=CARTESIAN_POINT('Ctrl Pts',(2.721246476,4.430609079,-6.988906754));
#144554=CARTESIAN_POINT('Ctrl Pts',(2.342529127,4.495496505,-7.13636662));
#144555=CARTESIAN_POINT('Ctrl Pts',(1.950094955,4.560723991,-7.242039054));
#144556=CARTESIAN_POINT('Origin',(-0.059135311493016,4.55356865186134,0.190021965440517));
#144557=CARTESIAN_POINT('Ctrl Pts',(3.563312241,4.560731746,-6.313897835));
#144558=CARTESIAN_POINT('Ctrl Pts',(3.216666389,4.495065281,-6.509530936));
#144559=CARTESIAN_POINT('Ctrl Pts',(2.850687243,4.430609079,-6.666039472));
#144560=CARTESIAN_POINT('Ctrl Pts',(3.898409388,4.560731746,-6.407215015));
#144561=CARTESIAN_POINT('Ctrl Pts',(3.546640232,4.495065281,-6.621245631));
#144562=CARTESIAN_POINT('Ctrl Pts',(3.173554525,4.430609079,-6.79548023900001));
#144563=CARTESIAN_POINT('',(3.55916373788445,4.55994605292436,-6.31623730607955));
#144564=CARTESIAN_POINT('Origin',(-0.112965338102915,4.69628090859361,0.154476604965065));
#144565=CARTESIAN_POINT('Ctrl Pts',(3.68099049666106,4.52063234085873,-6.53454734171104));
#144566=CARTESIAN_POINT('Ctrl Pts',(3.66069745650017,4.52686606958346,-6.49810883839098));
#144567=CARTESIAN_POINT('Ctrl Pts',(3.64038904380658,4.53325386231883,-6.46167765320372));
#144568=CARTESIAN_POINT('Ctrl Pts',(3.59978787616399,4.54634733292843,-6.38891931766763));
#144569=CARTESIAN_POINT('Ctrl Pts',(3.57947139933409,4.55306065404519,-6.35254965228119));
#144570=CARTESIAN_POINT('Ctrl Pts',(3.559163738865,4.55994605028106,-6.31623730502997));
#144571=CARTESIAN_POINT('Ctrl Pts',(4.217041199,4.430609079,-5.897377682));
#144572=CARTESIAN_POINT('Ctrl Pts',(3.897472013,4.495496505,-6.125892201));
#144573=CARTESIAN_POINT('Ctrl Pts',(3.555080941,4.560723991,-6.31853618300001));
#144574=CARTESIAN_POINT('Ctrl Pts',(4.160033607,4.430609079,-6.240522445));
#144575=CARTESIAN_POINT('Ctrl Pts',(3.821869971,4.495496505,-6.465947816));
#144576=CARTESIAN_POINT('Ctrl Pts',(3.461327142,4.560723991,-6.65351143500001));
#144577=CARTESIAN_POINT('Origin',(-0.0986017871400374,4.55356862974844,
0.172866876305883));
#144578=CARTESIAN_POINT('Ctrl Pts',(4.837305378,4.560731746,-5.400275611));
#144579=CARTESIAN_POINT('Ctrl Pts',(4.540819247,4.495065281,-5.66585353));
#144580=CARTESIAN_POINT('Ctrl Pts',(4.217041199,4.430609079,-5.897377682));
#144581=CARTESIAN_POINT('Ctrl Pts',(5.184628575,4.560731746,-5.419375106));
#144582=CARTESIAN_POINT('Ctrl Pts',(4.88709384300001,4.495065281,-5.704021776));
#144583=CARTESIAN_POINT('Ctrl Pts',(4.56018596200001,4.430609079,-5.954385274));
#144584=CARTESIAN_POINT('',(4.83375678100281,4.55994605293975,-5.40345219171606));
#144585=CARTESIAN_POINT('Origin',(-0.143532263022277,4.69628092208878,0.126580913645621));
#144586=CARTESIAN_POINT('Ctrl Pts',(4.99966550307942,4.52063234090427,-5.5904691084804));
#144587=CARTESIAN_POINT('Ctrl Pts',(4.97201370358798,4.52686606921442,-5.55924492289589));
#144588=CARTESIAN_POINT('Ctrl Pts',(4.94434846128484,4.53325386217182,-5.52803118575706));
#144589=CARTESIAN_POINT('Ctrl Pts',(4.88905563426124,4.54634733293204,-5.46570194974545));
#144590=CARTESIAN_POINT('Ctrl Pts',(4.86139574168964,4.55306065422027,-5.43455002807531));
#144591=CARTESIAN_POINT('Ctrl Pts',(4.83375678201757,4.55994605041382,-5.40345219025491));
#144592=CARTESIAN_POINT('Ctrl Pts',(5.386210996,4.430609079,-4.852961066));
#144593=CARTESIAN_POINT('Ctrl Pts',(5.123237026,4.495496505,-5.144830971));
#144594=CARTESIAN_POINT('Ctrl Pts',(4.830263629,4.560723991,-5.406575004));
#144595=CARTESIAN_POINT('Ctrl Pts',(5.40430219,4.430609079,-5.200338242));
#144596=CARTESIAN_POINT('Ctrl Pts',(5.122504424,4.495496505,-5.493188479));
#144597=CARTESIAN_POINT('Ctrl Pts',(4.810711519,4.560723991,-5.75387301500001));
#144598=CARTESIAN_POINT('Origin',(-0.133457977518899,4.55356864071217,0.147629070275643));
#144599=CARTESIAN_POINT('Ctrl Pts',(5.885111492,4.560731746,-4.234142502));
#144600=CARTESIAN_POINT('Ctrl Pts',(5.652648444,4.495065281,-4.557247111));
#144601=CARTESIAN_POINT('Ctrl Pts',(5.38621099600001,4.430609079,-4.852961066));
#144602=CARTESIAN_POINT('Ctrl Pts',(6.22842029200001,4.560731746,-4.17813124));
#144603=CARTESIAN_POINT('Ctrl Pts',(5.999032377,4.495065281,-4.520084201));
#144604=CARTESIAN_POINT('Ctrl Pts',(5.733588172,4.430609079,-4.83486987100001));
#144605=CARTESIAN_POINT('',(5.88232873095195,4.55994605189024,-4.23800766024314));
#144606=CARTESIAN_POINT('Origin',(-0.167387900492737,4.69628105601737,0.0927664531746669));
#144607=CARTESIAN_POINT('Ctrl Pts',(6.0845617075043,4.52063234085544,-4.38498675280473));
#144608=CARTESIAN_POINT('Ctrl Pts',(6.0508441043927,4.52686607108181,-4.36043688347114));
#144609=CARTESIAN_POINT('Ctrl Pts',(6.01711563512917,4.53325386299334,-4.33590011996221));
#144610=CARTESIAN_POINT('Ctrl Pts',(5.94971658496535,4.54634733284697,-4.28691443395888));
#144611=CARTESIAN_POINT('Ctrl Pts',(5.91600662413241,4.55306065390205,-4.26243688720519));
#144612=CARTESIAN_POINT('Ctrl Pts',(5.88232873168168,4.55994605017244,-4.23800765875298));
#144613=CARTESIAN_POINT('Ctrl Pts',(6.303527553,4.430609079,-3.581625384));
#144614=CARTESIAN_POINT('Ctrl Pts',(6.10944517,4.495496505,-3.923203163));
#144615=CARTESIAN_POINT('Ctrl Pts',(5.879588558,4.560723991,-4.241808386));
#144616=CARTESIAN_POINT('Ctrl Pts',(6.39587161000001,4.430609079,-3.916992003));
#144617=CARTESIAN_POINT('Ctrl Pts',(6.183616263,4.495496505,-4.263573754));
#144618=CARTESIAN_POINT('Ctrl Pts',(5.935152372,4.560723991,-4.585189889));
#144619=CARTESIAN_POINT('Origin',(-0.162073690401712,4.5535686417356,0.115488049281015));
#144620=CARTESIAN_POINT('Ctrl Pts',(6.657736333,4.560731746,-2.870025595));
#144621=CARTESIAN_POINT('Ctrl Pts',(6.500166082,4.495065281,-3.235548881));
#144622=CARTESIAN_POINT('Ctrl Pts',(6.303527553,4.430609079,-3.581625384));
#144623=CARTESIAN_POINT('Ctrl Pts',(6.980977999,4.560731746,-2.741522602));
#144624=CARTESIAN_POINT('Ctrl Pts',(6.830462824,4.495065281,-3.124792514));
#144625=CARTESIAN_POINT('Ctrl Pts',(6.638894171,4.430609079,-3.489281327));
#144626=CARTESIAN_POINT('',(6.65584952602707,4.55994605292527,-2.87439859900565));
#144627=CARTESIAN_POINT('Origin',(-0.183416398184002,4.6962809273909,0.0546141480217011));
#144628=CARTESIAN_POINT('Ctrl Pts',(6.88495056874341,4.52063234090296,-2.97446729084825));
#144629=CARTESIAN_POINT('Ctrl Pts',(6.84674376983872,4.52686607085981,-2.95773967239492));
#144630=CARTESIAN_POINT('Ctrl Pts',(6.80852917359772,4.5332538629194,-2.94102718811593));
#144631=CARTESIAN_POINT('Ctrl Pts',(6.73217540049566,4.54634733289709,-2.90767556313908));
#144632=CARTESIAN_POINT('Ctrl Pts',(6.69399161031044,4.5530606540368,-2.89101693261405));
#144633=CARTESIAN_POINT('Ctrl Pts',(6.65584952632393,4.5599460502987,-2.87439859723605));
#144634=CARTESIAN_POINT('Ctrl Pts',(6.926098167,4.430609079,-2.14281688));
#144635=CARTESIAN_POINT('Ctrl Pts',(6.809982448,4.495496505,-2.518130736));
#144636=CARTESIAN_POINT('Ctrl Pts',(6.653990461,4.560723991,-2.878699522));
#144637=CARTESIAN_POINT('Ctrl Pts',(7.08837718100001,4.430609079,-2.450491571));
#144638=CARTESIAN_POINT('Ctrl Pts',(6.95558907800001,4.495496505,-2.834599059));
#144639=CARTESIAN_POINT('Ctrl Pts',(6.782072097,4.560723991,-3.202108379));
#144640=CARTESIAN_POINT('Origin',(-0.183110903817996,4.55356867528369,0.0779469181040598));
#144641=CARTESIAN_POINT('Ctrl Pts',(7.119052823,4.560731746,-1.371709481));
#144642=CARTESIAN_POINT('Ctrl Pts',(7.043743179,4.495065281,-1.762559983));
#144643=CARTESIAN_POINT('Ctrl Pts',(6.926098167,4.430609079,-2.14281688));
#144644=CARTESIAN_POINT('Ctrl Pts',(7.407112933,4.560731746,-1.176723413));
#144645=CARTESIAN_POINT('Ctrl Pts',(7.342508421,4.495065281,-1.583389001));
#144646=CARTESIAN_POINT('Ctrl Pts',(7.233772858,4.430609079,-1.980537866));
#144647=CARTESIAN_POINT('',(7.11815019522467,4.55994605291902,-1.37638585417308));
#144648=CARTESIAN_POINT('Origin',(-0.190868400650031,4.69628087112419,0.0139081448837788));
#144649=CARTESIAN_POINT('Ctrl Pts',(7.3634067933585,4.52063234083335,-1.4248650437653));
#144650=CARTESIAN_POINT('Ctrl Pts',(7.32249725512444,4.52686607836689,-1.41674183026557));
#144651=CARTESIAN_POINT('Ctrl Pts',(7.28158343164322,4.53325386654012,-1.40863508849938));
#144652=CARTESIAN_POINT('Ctrl Pts',(7.1998451768763,4.54634733286553,-1.39247701472649));
#144653=CARTESIAN_POINT('Ctrl Pts',(7.15897298894386,4.55306065408668,-1.38441623981203));
#144654=CARTESIAN_POINT('Ctrl Pts',(7.11815019511434,4.55994605030007,-1.3763858524884));
#144655=CARTESIAN_POINT('Ctrl Pts',(7.224812129,4.430609079,-0.603812641));
#144656=CARTESIAN_POINT('Ctrl Pts',(7.192092516,4.495496505,-0.995313314));
#144657=CARTESIAN_POINT('Ctrl Pts',(7.117259166,4.560723991,-1.380985869));
#144658=CARTESIAN_POINT('Ctrl Pts',(7.449438113,4.430609079,-0.869408877));
#144659=CARTESIAN_POINT('Ctrl Pts',(7.402326278,4.495496505,-1.273081663));
#144660=CARTESIAN_POINT('Ctrl Pts',(7.311869668,4.560723991,-1.66929984));
#144661=CARTESIAN_POINT('Origin',(-0.195586225750846,4.55356863539642,0.0367611360508951));
#144662=CARTESIAN_POINT('Ctrl Pts',(7.247490315,4.560731746,0.190746244));
#144663=CARTESIAN_POINT('Ctrl Pts',(7.257962673,4.495065281,-0.207155738));
#144664=CARTESIAN_POINT('Ctrl Pts',(7.224812129,4.430609079,-0.603812641));
#144665=CARTESIAN_POINT('Ctrl Pts',(7.48689949900001,4.560731746,0.443098054));
#144666=CARTESIAN_POINT('Ctrl Pts',(7.511226485,4.495065281,0.032052021));
#144667=CARTESIAN_POINT('Ctrl Pts',(7.49040836500001,4.430609079,-0.379186656));
#144668=CARTESIAN_POINT('',(7.2476140724582,4.55994605190755,0.185985162743353));
#144669=CARTESIAN_POINT('Origin',(-0.189396225307772,4.69628103500228,-0.0274481071492781));
#144670=CARTESIAN_POINT('Ctrl Pts',(7.49755829989574,4.52063234091446,0.191362308830983));
#144671=CARTESIAN_POINT('Ctrl Pts',(7.45585900341303,4.52686607092702,0.19050126575676));
#144672=CARTESIAN_POINT('Ctrl Pts',(7.41415898547614,4.53325386295828,0.189623213282634));
#144673=CARTESIAN_POINT('Ctrl Pts',(7.3308581944994,4.5463473328595,0.187832211268426));
#144674=CARTESIAN_POINT('Ctrl Pts',(7.28920874762302,4.5530606540035,0.18691821756087));
#144675=CARTESIAN_POINT('Ctrl Pts',(7.24761407212469,4.55994605018931,0.185985164931052));
#144676=CARTESIAN_POINT('Ctrl Pts',(7.185701905,4.430609079,0.963425207));
#144677=CARTESIAN_POINT('Ctrl Pts',(7.237908331,4.495496505,0.574043853));
#144678=CARTESIAN_POINT('Ctrl Pts',(7.247732742,4.560723991,0.181301149));
#144679=CARTESIAN_POINT('Ctrl Pts',(7.462171599,4.430609079,0.75232641));
#144680=CARTESIAN_POINT('Ctrl Pts',(7.502938928,4.495496505,0.347963618));
#144681=CARTESIAN_POINT('Ctrl Pts',(7.49977234,4.560723991,-0.058436696));
#144682=CARTESIAN_POINT('Origin',(-0.198915958463134,4.5535685999915,-0.00614357805637192));
#144683=CARTESIAN_POINT('Ctrl Pts',(7.037043215,4.560731746,1.744282886));
#144684=CARTESIAN_POINT('Ctrl Pts',(7.13280789900001,4.495065281,1.357934879));
#144685=CARTESIAN_POINT('Ctrl Pts',(7.18570190500001,4.430609079,0.963425207));
#144686=CARTESIAN_POINT('Ctrl Pts',(7.21660696600001,4.560731746,2.042200749));
#144687=CARTESIAN_POINT('Ctrl Pts',(7.328727947,4.495065281,1.645994327));
#144688=CARTESIAN_POINT('Ctrl Pts',(7.396800703,4.430609079,1.239894901));
#144689=CARTESIAN_POINT('',(7.03818757051289,4.55994605127143,1.73965971993725));
#144690=CARTESIAN_POINT('Origin',(-0.179067437115114,4.69628090431665,-0.0675208998185697));
#144691=CARTESIAN_POINT('Ctrl Pts',(7.28113231396762,4.52063234088911,1.79864177274421));
#144692=CARTESIAN_POINT('Ctrl Pts',(7.24059302189612,4.52686607101429,1.78883674406937));
#144693=CARTESIAN_POINT('Ctrl Pts',(7.20005668260348,4.53325386303259,1.77901494874863));
#144694=CARTESIAN_POINT('Ctrl Pts',(7.11908843034963,4.54634733292347,1.75935861156909));
#144695=CARTESIAN_POINT('Ctrl Pts',(7.07860920609677,4.55306065405402,1.7495125865457));
#144696=CARTESIAN_POINT('Ctrl Pts',(7.03818756973783,4.55994605023828,1.73965972239497));
#144697=CARTESIAN_POINT('Ctrl Pts',(6.810596247,4.430609079,2.485614363));
#144698=CARTESIAN_POINT('Ctrl Pts',(6.945287596,4.495496505,2.116559367));
#144699=CARTESIAN_POINT('Ctrl Pts',(7.03931039,4.560723991,1.735110727));
#144700=CARTESIAN_POINT('Ctrl Pts',(7.125982234,4.430609079,2.33888375));
#144701=CARTESIAN_POINT('Ctrl Pts',(7.252722494,4.495496505,1.952738506));
#144702=CARTESIAN_POINT('Ctrl Pts',(7.33699399300001,4.560723991,1.555158883));
#144703=CARTESIAN_POINT('Origin',(-0.192944911290353,4.5535685917447,-0.0487610407490913));
#144704=CARTESIAN_POINT('Ctrl Pts',(6.49755179600001,4.560731746,3.216258799));
#144705=CARTESIAN_POINT('Ctrl Pts',(6.674130955,4.495065281,2.85952997));
#144706=CARTESIAN_POINT('Ctrl Pts',(6.810596247,4.430609079,2.485614363));
#144707=CARTESIAN_POINT('Ctrl Pts',(6.608873911,4.560731746,3.545812407));
#144708=CARTESIAN_POINT('Ctrl Pts',(6.803546235,4.495065281,3.182971767));
#144709=CARTESIAN_POINT('Ctrl Pts',(6.95732686000001,4.430609079,2.80100035));
#144710=CARTESIAN_POINT('',(6.49966323932526,4.55994605292362,3.21198972307321));
#144711=CARTESIAN_POINT('Origin',(-0.160366188328788,4.69628093058526,-0.1044366202835));
#144712=CARTESIAN_POINT('Ctrl Pts',(6.72424867288717,4.52063234084894,3.32181874645752));
#144713=CARTESIAN_POINT('Ctrl Pts',(6.68676491361815,4.5268660784116,3.30352818266225));
#144714=CARTESIAN_POINT('Ctrl Pts',(6.64928771115034,4.53325386662127,3.2852219124572));
#144715=CARTESIAN_POINT('Ctrl Pts',(6.57443800366556,4.54634733297343,3.24861935859961));
#144716=CARTESIAN_POINT('Ctrl Pts',(6.53702176458202,4.55306065431381,3.2303016909336));
#144717=CARTESIAN_POINT('Ctrl Pts',(6.49966323833264,4.55994605052893,3.21198972419786));
#144718=CARTESIAN_POINT('Ctrl Pts',(6.117034678,4.430609079,3.891578954));
#144719=CARTESIAN_POINT('Ctrl Pts',(6.327912933,4.495496505,3.560106917));
#144720=CARTESIAN_POINT('Ctrl Pts',(6.501737708,4.560723991,3.207788456));
#144721=CARTESIAN_POINT('Ctrl Pts',(6.45658986,4.430609079,3.816077485));
#144722=CARTESIAN_POINT('Ctrl Pts',(6.663376816,4.495496505,3.466205512));
#144723=CARTESIAN_POINT('Ctrl Pts',(6.831145961,4.560723991,3.096036961));
#144724=CARTESIAN_POINT('Origin',(-0.177951791260036,4.55356861253526,-0.0890984797097816));
#144725=CARTESIAN_POINT('Ctrl Pts',(5.654242076,4.560731746,4.537846025));
#144726=CARTESIAN_POINT('Ctrl Pts',(5.903379066,4.495065281,4.227416618));
#144727=CARTESIAN_POINT('Ctrl Pts',(6.117034678,4.430609079,3.891578954));
#144728=CARTESIAN_POINT('Ctrl Pts',(5.69211725800001,4.560731746,4.883625817));
#144729=CARTESIAN_POINT('Ctrl Pts',(5.960238263,4.495065281,4.571116985));
#144730=CARTESIAN_POINT('Ctrl Pts',(6.19253614600001,4.430609079,4.231134137));
#144731=CARTESIAN_POINT('',(5.65722188060532,4.55994605195593,4.53413065603272));
#144732=CARTESIAN_POINT('Origin',(-0.134165992850245,4.69628104438188,-0.136468870569518));
#144733=CARTESIAN_POINT('Ctrl Pts',(5.85294663755566,4.52063234086994,4.68967116711042));
#144734=CARTESIAN_POINT('Ctrl Pts',(5.82027120162022,4.52686607017123,4.66375036059968));
#144735=CARTESIAN_POINT('Ctrl Pts',(5.7876054789363,4.53325386263838,4.63781557160427));
#144736=CARTESIAN_POINT('Ctrl Pts',(5.72237416328767,4.54634733296961,4.58597827493659));
#144737=CARTESIAN_POINT('Ctrl Pts',(5.68977045243914,4.55306065424697,4.56004547916216));
#144738=CARTESIAN_POINT('Ctrl Pts',(5.6572218792048,4.55994605047594,4.53413065739853));
#144739=CARTESIAN_POINT('Ctrl Pts',(5.137447365,4.430609079,5.115577638));
#144740=CARTESIAN_POINT('Ctrl Pts',(5.41465209400001,4.495496505,4.837187824));
#144741=CARTESIAN_POINT('Ctrl Pts',(5.66015099700001,4.560723991,4.530473562));
#144742=CARTESIAN_POINT('Ctrl Pts',(5.48529452,4.430609079,5.114835679));
#144743=CARTESIAN_POINT('Ctrl Pts',(5.762459044,4.495496505,4.81759660100001));
#144744=CARTESIAN_POINT('Ctrl Pts',(6.005881136,4.560723991,4.492147791));
#144745=CARTESIAN_POINT('Origin',(-0.15463786334905,4.55356865057608,-0.125269808524199));
#144746=CARTESIAN_POINT('Ctrl Pts',(4.54654628,4.560731746,5.647248615));
#144747=CARTESIAN_POINT('Ctrl Pts',(4.856591733,4.495065281,5.397633963));
#144748=CARTESIAN_POINT('Ctrl Pts',(5.13744736500001,4.430609079,5.115577638));
#144749=CARTESIAN_POINT('Ctrl Pts',(4.509203528,4.560731746,5.993086312));
#144750=CARTESIAN_POINT('Ctrl Pts',(4.838236174,4.495065281,5.745521853));
#144751=CARTESIAN_POINT('Ctrl Pts',(5.138189324,4.430609079,5.463424793));
#144752=CARTESIAN_POINT('',(4.55025511321812,4.55994605292947,5.64426067931357));
#144753=CARTESIAN_POINT('Origin',(-0.101692449553174,4.69628087469097,-0.162119920184228));
#144754=CARTESIAN_POINT('Ctrl Pts',(4.70796732248972,4.52063234085653,5.83823977670622));
#144755=CARTESIAN_POINT('Ctrl Pts',(4.68162799240327,4.52686607840256,5.80590068860456));
#144756=CARTESIAN_POINT('Ctrl Pts',(4.65530120807513,4.53325386657975,5.77355009899121));
#144757=CARTESIAN_POINT('Ctrl Pts',(4.60273846663404,4.5463473329181,5.70890194445263));
#144758=CARTESIAN_POINT('Ctrl Pts',(4.57647179682458,4.55306065418861,5.67656660889885));
#144759=CARTESIAN_POINT('Ctrl Pts',(4.5502551116134,4.55994605040326,5.64426068007741));
#144760=CARTESIAN_POINT('Ctrl Pts',(3.917638724,4.430609079,6.100377597));
#144761=CARTESIAN_POINT('Ctrl Pts',(4.248208141,4.495496505,5.888087205));
#144762=CARTESIAN_POINT('Ctrl Pts',(4.553901916,4.560723991,5.64131875900001));
#144763=CARTESIAN_POINT('Ctrl Pts',(4.257512905,4.430609079,6.174429841));
#144764=CARTESIAN_POINT('Ctrl Pts',(4.592095092,4.495496505,5.94372222700001));
#144765=CARTESIAN_POINT('Ctrl Pts',(4.899787985,4.560723991,5.67821078400001));
#144766=CARTESIAN_POINT('Origin',(-0.124093184553192,4.55356863304782,-0.155583612145826));
#144767=CARTESIAN_POINT('Ctrl Pts',(3.226259034,4.560731746,6.492592136));
#144768=CARTESIAN_POINT('Ctrl Pts',(3.582715568,4.495065281,6.315463943));
#144769=CARTESIAN_POINT('Ctrl Pts',(3.917638724,4.430609079,6.100377597));
#144770=CARTESIAN_POINT('Ctrl Pts',(3.115444452,4.560731746,6.822316752));
#144771=CARTESIAN_POINT('Ctrl Pts',(3.490003539,4.495065281,6.651272505));
#144772=CARTESIAN_POINT('Ctrl Pts',(3.84358648,4.430609079,6.440251778));
#144773=CARTESIAN_POINT('',(3.2305234747432,4.55994605294443,6.4904713464554));
#144774=CARTESIAN_POINT('Origin',(-0.0644639989327161,4.69628088593423,
-0.180190601896851));
#144775=CARTESIAN_POINT('Ctrl Pts',(3.34284868775708,4.52063234083049,6.71381878287937));
#144776=CARTESIAN_POINT('Ctrl Pts',(3.32407710461589,4.52686607836884,6.6765735873874));
#144777=CARTESIAN_POINT('Ctrl Pts',(3.30532024644795,4.53325386652875,6.63931985630375));
#144778=CARTESIAN_POINT('Ctrl Pts',(3.2678838350263,4.54634733287855,6.56488370404862));
#144779=CARTESIAN_POINT('Ctrl Pts',(3.24918240690815,4.55306065410071,6.52765779341605));
#144780=CARTESIAN_POINT('Ctrl Pts',(3.23052347304825,4.55994605034044,6.49047134682372));
#144781=CARTESIAN_POINT('Ctrl Pts',(2.51464565,4.430609079,6.79993068));
#144782=CARTESIAN_POINT('Ctrl Pts',(2.883122697,4.495496505,6.663666173));
#144783=CARTESIAN_POINT('Ctrl Pts',(3.234717443,4.560723991,6.488382161));
#144784=CARTESIAN_POINT('Ctrl Pts',(2.830654719,4.430609079,6.945314526));
#144785=CARTESIAN_POINT('Ctrl Pts',(3.207009877,4.495496505,6.791926008));
#144786=CARTESIAN_POINT('Ctrl Pts',(3.564586193,4.560723991,6.598766951));
#144787=CARTESIAN_POINT('Origin',(-0.0877460033528399,4.55356862172701,
-0.178622367928359));
#144788=CARTESIAN_POINT('Ctrl Pts',(1.755115501,4.560731746,7.034349265));
#144789=CARTESIAN_POINT('Ctrl Pts',(2.141315605,4.495065281,6.937989849));
#144790=CARTESIAN_POINT('Ctrl Pts',(2.51464565,4.430609079,6.79993068000001));
#144791=CARTESIAN_POINT('Ctrl Pts',(1.576010657,4.560731746,7.332543243));
#144792=CARTESIAN_POINT('Ctrl Pts',(1.978582217,4.495065281,7.246017048));
#144793=CARTESIAN_POINT('Ctrl Pts',(2.369261804,4.430609079,7.115939748));
#144794=CARTESIAN_POINT('',(1.75973614927375,4.55994605189544,7.03319478739374));
#144795=CARTESIAN_POINT('Origin',(-0.0242212355240337,4.69628106280526,
-0.189835864139755));
#144796=CARTESIAN_POINT('Ctrl Pts',(1.82142216389954,4.52063234086191,7.27546708476632));
#144797=CARTESIAN_POINT('Ctrl Pts',(1.8110960794124,4.52686607033607,7.23505737799141));
#144798=CARTESIAN_POINT('Ctrl Pts',(1.80078618995318,4.5332538626486,7.19464242018641));
#144799=CARTESIAN_POINT('Ctrl Pts',(1.78022658737578,4.54634733288435,7.11389879786007));
#144800=CARTESIAN_POINT('Ctrl Pts',(1.76996485896719,4.55306065389986,7.07352295524677));
#144801=CARTESIAN_POINT('Ctrl Pts',(1.75973614734532,4.55994605016872,7.03319478758805));
#144802=CARTESIAN_POINT('Ctrl Pts',(0.994070541,4.430609079,7.181526562));
#144803=CARTESIAN_POINT('Ctrl Pts',(1.38322564,4.495496505,7.127659516));
#144804=CARTESIAN_POINT('Ctrl Pts',(1.764281177,4.560723991,7.03205602400001));
#144805=CARTESIAN_POINT('Ctrl Pts',(1.271438263,4.430609079,7.391444023));
#144806=CARTESIAN_POINT('Ctrl Pts',(1.671968444,4.495496505,7.32254687700001));
#144807=CARTESIAN_POINT('Ctrl Pts',(2.062708312,4.560723991,7.21077211));
#144808=CARTESIAN_POINT('Origin',(-0.0472960242996028,4.55356862061657,
-0.193309116276226));
#144809=CARTESIAN_POINT('Ctrl Pts',(0.201904718,4.560731746,7.24718804));
#144810=CARTESIAN_POINT('Ctrl Pts',(0.599790104,4.495065281,7.23610306));
#144811=CARTESIAN_POINT('Ctrl Pts',(0.994070541000001,4.430609079,7.18152656200001));
#144812=CARTESIAN_POINT('Ctrl Pts',(-0.037115645,4.560731746,7.499908161));
#144813=CARTESIAN_POINT('Ctrl Pts',(0.37464459,4.495065281,7.501945886));
#144814=CARTESIAN_POINT('Ctrl Pts',(0.78415308,4.430609079,7.458894285));
#144815=CARTESIAN_POINT('',(0.206665516131424,4.55994605293665,7.24705385453353));
#144816=CARTESIAN_POINT('Origin',(0.0171541522854927,4.69628090700534,-0.190604205424212));
#144817=CARTESIAN_POINT('Ctrl Pts',(0.21482796402738,4.52063234085271,7.49692263175493));
#144818=CARTESIAN_POINT('Ctrl Pts',(0.213430188247251,4.52686607841023,
7.45523782448));
#144819=CARTESIAN_POINT('Ctrl Pts',(0.212049360526979,4.53325386660713,
7.41355145322911));
#144820=CARTESIAN_POINT('Ctrl Pts',(0.209327922975149,4.54634733296248,
7.33027588971406));
#144821=CARTESIAN_POINT('Ctrl Pts',(0.207985720792377,4.55306065421451,
7.28863804207581));
#144822=CARTESIAN_POINT('Ctrl Pts',(0.206665514894415,4.55994605043467,
7.24705385415854));
#144823=CARTESIAN_POINT('Ctrl Pts',(-0.572986203,4.430609079,7.22732224400001));
#144824=CARTESIAN_POINT('Ctrl Pts',(-0.181349511,4.495496505,7.25837142200001));
#144825=CARTESIAN_POINT('Ctrl Pts',(0.211349085,4.560723991,7.246918763));
#144826=CARTESIAN_POINT('Ctrl Pts',(-0.347229232,4.430609079,7.491957812));
#144827=CARTESIAN_POINT('Ctrl Pts',(0.0587476260000001,4.495496505,7.510773593));
#144828=CARTESIAN_POINT('Ctrl Pts',(0.464380483,4.560723991,7.485609579));
#144829=CARTESIAN_POINT('Origin',(-0.00463454090715021,4.55356860745719,
-0.198957013389406));
#144830=CARTESIAN_POINT('Ctrl Pts',(0.201633249,1.457976823,7.247195598));
#144831=CARTESIAN_POINT('Ctrl Pts',(0.597296021,1.39227158,7.236187371));
#144832=CARTESIAN_POINT('Ctrl Pts',(0.989408718,1.327100493,7.18217031200001));
#144833=CARTESIAN_POINT('Ctrl Pts',(-0.03739658,1.457976823,7.499906766));
#144834=CARTESIAN_POINT('Ctrl Pts',(0.372063032,1.39227158,7.50194844300001));
#144835=CARTESIAN_POINT('Ctrl Pts',(0.779311259,1.327100493,7.459401716));
#144836=CARTESIAN_POINT('',(0.213145095072078,1.41778968871295,7.49697066565625));
#144837=CARTESIAN_POINT('',(0.77931126906081,1.32710049399577,7.45940171643651));
#144838=CARTESIAN_POINT('Origin',(0.00491638811184272,1.48212079817506,
-0.190660326973322));
#144839=CARTESIAN_POINT('',(0.884360005917485,1.32710049586377,7.32078601189595));
#144840=CARTESIAN_POINT('Ctrl Pts',(0.213145094523798,1.41778968832183,
7.49697066561295));
#144841=CARTESIAN_POINT('Ctrl Pts',(0.211973474313471,1.42404710663119,
7.45528012261522));
#144842=CARTESIAN_POINT('Ctrl Pts',(0.210820057394797,1.43045449292311,
7.41358844026421));
#144843=CARTESIAN_POINT('Ctrl Pts',(0.208555899831965,1.44357823944106,
7.33029933574109));
#144844=CARTESIAN_POINT('Ctrl Pts',(0.207443881005112,1.45030198445001,
7.28865500680507));
#144845=CARTESIAN_POINT('Ctrl Pts',(0.206355413393753,1.45719264070242,
7.24706267711513));
#144846=CARTESIAN_POINT('Ctrl Pts',(0.989408718000001,1.327100493,7.18217031200001));
#144847=CARTESIAN_POINT('Ctrl Pts',(1.380789714,1.392692987,7.128254051));
#144848=CARTESIAN_POINT('Ctrl Pts',(1.76399439,1.45796923,7.03212797));
#144849=CARTESIAN_POINT('Ctrl Pts',(1.266640122,1.327100493,7.392267771));
#144850=CARTESIAN_POINT('Ctrl Pts',(1.669470046,1.392692987,7.323244224));
#144851=CARTESIAN_POINT('Ctrl Pts',(2.062414236,1.45796923,7.210856227));
#144852=CARTESIAN_POINT('',(1.26664012713773,1.32710049307754,7.39226777165038));
#144853=CARTESIAN_POINT('',(1.81978896516141,1.41778968870968,7.27587576303884));
#144854=CARTESIAN_POINT('Origin',(-0.03450053467242,1.33928592015067,-0.18979919100365));
#144855=CARTESIAN_POINT('Ctrl Pts',(1.75943519295771,1.45719264068656,7.03327006476683));
#144856=CARTESIAN_POINT('Ctrl Pts',(1.76943932796608,1.45030198862715,7.07365597612469));
#144857=CARTESIAN_POINT('Ctrl Pts',(1.77947764044795,1.44357824830594,7.1140876026183));
#144858=CARTESIAN_POINT('Ctrl Pts',(1.79959357204886,1.43045449290407,7.19494278218988));
#144859=CARTESIAN_POINT('Ctrl Pts',(1.80968250183055,1.4240471066513,7.23541178548329));
#144860=CARTESIAN_POINT('Ctrl Pts',(1.81978896448098,1.41778968833587,7.27587576315098));
#144861=CARTESIAN_POINT('',(1.12802441867849,1.32710049321647,7.28721904170456));
#144862=CARTESIAN_POINT('Origin',(-6.83047368665868E-14,1.41887506699983,
9.2374025095765E-14));
#144863=CARTESIAN_POINT('',(1.82437897668122,1.23689319339462,7.27472620408252));
#144864=CARTESIAN_POINT('Origin',(-0.00664832877748628,1.48200505002726,
-0.185042883132719));
#144865=CARTESIAN_POINT('',(2.36464227492396,1.32710049399578,7.1174761632605));
#144866=CARTESIAN_POINT('Origin',(-0.0625461989580287,1.33928289225507,
-0.182027286444451));
#144867=CARTESIAN_POINT('Origin',(-0.0361848819786822,1.4821207899034,-0.187259632689556));
#144868=CARTESIAN_POINT('Ctrl Pts',(1.754852004,1.457976823,7.034415004));
#144869=CARTESIAN_POINT('Ctrl Pts',(2.138897957,1.39227158,6.938608343));
#144870=CARTESIAN_POINT('Ctrl Pts',(2.510231206,1.327100493,6.801561533));
#144871=CARTESIAN_POINT('Ctrl Pts',(1.57573599,1.457976823,7.332602273));
#144872=CARTESIAN_POINT('Ctrl Pts',(1.976061564,1.39227158,7.24657450400001));
#144873=CARTESIAN_POINT('Ctrl Pts',(2.364642265,1.327100493,7.11747616499999));
#144874=CARTESIAN_POINT('',(2.43743675205783,1.32710049586375,6.95951884320094));
#144875=CARTESIAN_POINT('Ctrl Pts',(2.510231206,1.327100493,6.801561533));
#144876=CARTESIAN_POINT('Ctrl Pts',(2.880871529,1.392692987,6.66477046000001));
#144877=CARTESIAN_POINT('Ctrl Pts',(3.234452827,1.45796923,6.488514076));
#144878=CARTESIAN_POINT('Ctrl Pts',(2.826145837,1.327100493,6.947150474));
#144879=CARTESIAN_POINT('Ctrl Pts',(3.204719799,1.392692987,6.793144133));
#144880=CARTESIAN_POINT('Ctrl Pts',(3.564317074,1.45796923,6.598912319));
#144881=CARTESIAN_POINT('',(2.82614584214365,1.32710049307753,6.94715047353126));
#144882=CARTESIAN_POINT('',(3.34134152620834,1.41778968874369,6.71456899583714));
#144883=CARTESIAN_POINT('Origin',(-0.0744950944575939,1.33928594525405,
-0.177945054765195));
#144884=CARTESIAN_POINT('Ctrl Pts',(3.23024573729235,1.45719264064239,6.49060956175589));
#144885=CARTESIAN_POINT('Ctrl Pts',(3.24869776185374,1.45030198734322,6.52790068625596));
#144886=CARTESIAN_POINT('Ctrl Pts',(3.26719299295515,1.44357824563603,6.56522911148062));
#144887=CARTESIAN_POINT('Ctrl Pts',(3.30422009154465,1.43045449289261,6.63986959596905));
#144888=CARTESIAN_POINT('Ctrl Pts',(3.32277278724771,1.42404710665793,6.67722363462803));
#144889=CARTESIAN_POINT('Ctrl Pts',(3.34134152552766,1.41778968836386,6.71456899611195));
#144890=CARTESIAN_POINT('',(2.66818852025337,1.32710049321647,6.87435600398386));
#144891=CARTESIAN_POINT('Origin',(-1.45283091113058E-14,1.41887506699983,
-7.37257477290143E-14));
#144892=CARTESIAN_POINT('',(3.34557710444283,1.23689319339271,6.71245959639036));
#144893=CARTESIAN_POINT('Origin',(-0.0462715736869412,1.48200502695773,
-0.179287315894316));
#144894=CARTESIAN_POINT('',(3.83940523733456,1.32710049399579,6.44274533515092));
#144895=CARTESIAN_POINT('Origin',(-0.100214493544963,1.33928284390673,-0.164326226279317));
#144896=CARTESIAN_POINT('Origin',(-0.0755943261787495,1.48212079376037,
-0.175103206174972));
#144897=CARTESIAN_POINT('Ctrl Pts',(3.226015829,1.457976823,6.492712982));
#144898=CARTESIAN_POINT('Ctrl Pts',(3.580487401,1.39227158,6.316587701));
#144899=CARTESIAN_POINT('Ctrl Pts',(3.913678072,1.327100493,6.102919297));
#144900=CARTESIAN_POINT('Ctrl Pts',(3.115188897,1.457976823,6.822433447));
#144901=CARTESIAN_POINT('Ctrl Pts',(3.487661654,1.39227158,6.652358794));
#144902=CARTESIAN_POINT('Ctrl Pts',(3.839405228,1.327100493,6.442745339));
#144903=CARTESIAN_POINT('',(3.87654166492425,1.32710049586378,6.27283230877697));
#144904=CARTESIAN_POINT('Ctrl Pts',(3.913678072,1.327100493,6.102919297));
#144905=CARTESIAN_POINT('Ctrl Pts',(4.246246993,1.392692987,5.889649609));
#144906=CARTESIAN_POINT('Ctrl Pts',(4.553671844,1.45796923,5.641504474));
#144907=CARTESIAN_POINT('Ctrl Pts',(4.253504114,1.327100493,6.177192142));
#144908=CARTESIAN_POINT('Ctrl Pts',(4.590120416,1.392692987,5.945404172));
#144909=CARTESIAN_POINT('Ctrl Pts',(4.899556408,1.45796923,5.678410606));
#144910=CARTESIAN_POINT('',(4.2535041188979,1.32710049307752,6.17719214044297));
#144911=CARTESIAN_POINT('',(4.70665667110046,1.41778968872295,5.83929644531604));
#144912=CARTESIAN_POINT('Origin',(-0.111006437282785,1.33928596431819,-0.157770636694248));
#144913=CARTESIAN_POINT('Ctrl Pts',(4.55001358209102,1.4571926406954,5.64445536825662));
#144914=CARTESIAN_POINT('Ctrl Pts',(4.57605069415297,1.45030198837447,5.67690800266822));
#144915=CARTESIAN_POINT('Ctrl Pts',(4.60213802035174,1.44357824776257,5.70938777653085));
#144916=CARTESIAN_POINT('Ctrl Pts',(4.65434495195885,1.43045449290745,5.77432348688941));
#144917=CARTESIAN_POINT('Ctrl Pts',(4.68049391001257,1.4240471066716,5.80681592778155));
#144918=CARTESIAN_POINT('Ctrl Pts',(4.70665667037991,1.41778968834624,5.83929644582386));
#144919=CARTESIAN_POINT('',(4.08359109188649,1.32710049321648,6.14005572024056));
#144920=CARTESIAN_POINT('Origin',(-8.70397504071363E-13,1.41887506700022,
-1.21430643318376E-12));
#144921=CARTESIAN_POINT('',(4.71033976529093,1.23689319339203,5.83632583826807));
#144922=CARTESIAN_POINT('Origin',(-0.0837313962564479,1.4820050646192,-0.165148862441861));
#144923=CARTESIAN_POINT('',(5.13464187728295,1.32710049399578,5.46675889524378));
#144924=CARTESIAN_POINT('Origin',(-0.133196764415154,1.3392828345734,-0.138941155274088));
#144925=CARTESIAN_POINT('Origin',(-0.111469039437913,1.4821207822942,-0.154758896047827));
#144926=CARTESIAN_POINT('Ctrl Pts',(4.54633474,1.457976823,5.647418918));
#144927=CARTESIAN_POINT('Ctrl Pts',(4.854657234,1.39227158,5.399210438));
#144928=CARTESIAN_POINT('Ctrl Pts',(5.134125702,1.327100493,5.118911337));
#144929=CARTESIAN_POINT('Ctrl Pts',(4.508979033,1.457976823,5.993255216));
#144930=CARTESIAN_POINT('Ctrl Pts',(4.836182561,1.39227158,5.747086181));
#144931=CARTESIAN_POINT('Ctrl Pts',(5.134641869,1.327100493,5.466758901));
#144932=CARTESIAN_POINT('',(5.13438379809266,1.32710049586378,5.29283510678433));
#144933=CARTESIAN_POINT('Ctrl Pts',(5.134125702,1.327100493,5.118911337));
#144934=CARTESIAN_POINT('Ctrl Pts',(5.413072667,1.392692987,4.839135289));
#144935=CARTESIAN_POINT('Ctrl Pts',(5.659966227,1.45796923,4.530704394));
#144936=CARTESIAN_POINT('Ctrl Pts',(5.481973265,1.327100493,5.11839517));
#144937=CARTESIAN_POINT('Ctrl Pts',(5.760892103,1.392692987,4.81966372));
#144938=CARTESIAN_POINT('Ctrl Pts',(6.005697929,1.45796923,4.492392723));
#144939=CARTESIAN_POINT('',(5.48197326949186,1.32710049307754,5.1183951674044));
#144940=CARTESIAN_POINT('',(5.85189378093044,1.41778968872863,4.69098488279759));
#144941=CARTESIAN_POINT('Origin',(-0.142327169791678,1.33928591042193,-0.130218947999294));
#144942=CARTESIAN_POINT('Ctrl Pts',(5.65702784793378,1.45719264077919,4.53437271583438));
#144943=CARTESIAN_POINT('Ctrl Pts',(5.68943258944673,1.45030198726807,4.56046942052694));
#144944=CARTESIAN_POINT('Ctrl Pts',(5.72189220655393,1.4435782453354,4.58658183662514));
#144945=CARTESIAN_POINT('Ctrl Pts',(5.78683781530013,1.43045449292487,4.63877642909337));
#144946=CARTESIAN_POINT('Ctrl Pts',(5.81936033988894,1.4240471066349,4.66488796186657));
#144947=CARTESIAN_POINT('Ctrl Pts',(5.85189378060671,1.41778968834312,4.69098488310873));
#144948=CARTESIAN_POINT('',(5.30804948257172,1.32710049321648,5.11865325446263));
#144949=CARTESIAN_POINT('Origin',(-8.16187395447088E-13,1.41887506700028,
-7.04731412115578E-13));
#144950=CARTESIAN_POINT('',(5.85485217362667,1.23689319338142,4.68729197077231));
#144951=CARTESIAN_POINT('Origin',(-0.117275698567805,1.48200509272981,-0.143287821712398));
#144952=CARTESIAN_POINT('',(6.18978836985319,1.32710049399578,4.23515288559396));
#144953=CARTESIAN_POINT('Origin',(-0.159950765827412,1.33928281164314,-0.107059299319675));
#144954=CARTESIAN_POINT('Origin',(-0.142131268964576,1.48212079248997,-0.127177973873037));
#144955=CARTESIAN_POINT('Ctrl Pts',(5.654072091,1.457976823,4.538057821));
#144956=CARTESIAN_POINT('Ctrl Pts',(5.90182869,1.39227158,4.229372095));
#144957=CARTESIAN_POINT('Ctrl Pts',(6.11450731900001,1.327100493,3.895548773));
#144958=CARTESIAN_POINT('Ctrl Pts',(5.691934321,1.457976823,4.883839032));
#144959=CARTESIAN_POINT('Ctrl Pts',(5.95856894700001,1.39227158,4.573086206));
#144960=CARTESIAN_POINT('Ctrl Pts',(6.189788363,1.327100493,4.235152893));
#144961=CARTESIAN_POINT('',(6.15214785067216,1.32710049586375,4.06535081836299));
#144962=CARTESIAN_POINT('Ctrl Pts',(6.114507319,1.327100493,3.895548773));
#144963=CARTESIAN_POINT('Ctrl Pts',(6.32678908000001,1.392692987,3.562348381));
#144964=CARTESIAN_POINT('Ctrl Pts',(6.50160688,1.45796923,3.208053611));
#144965=CARTESIAN_POINT('Ctrl Pts',(6.45411144,1.327100493,3.82026773));
#144966=CARTESIAN_POINT('Ctrl Pts',(6.662290879,1.392692987,3.468561149));
#144967=CARTESIAN_POINT('Ctrl Pts',(6.83101969100001,1.45796923,3.09631555));
#144968=CARTESIAN_POINT('',(6.45411144382818,1.32710049307764,3.82026772649141));
#144969=CARTESIAN_POINT('',(6.72350284172602,1.41778968869915,3.32332808088867));
#144970=CARTESIAN_POINT('Origin',(-0.166992936340966,1.33928594576275,-0.0965783880493759));
#144971=CARTESIAN_POINT('Ctrl Pts',(6.49952577937695,1.45719264070939,3.21226783447012));
#144972=CARTESIAN_POINT('Ctrl Pts',(6.53678293030639,1.45030198828831,3.2307883484457));
#144973=CARTESIAN_POINT('Ctrl Pts',(6.57409705006756,1.44357824756423,3.2493124091844));
#144974=CARTESIAN_POINT('Ctrl Pts',(6.64874457410277,1.43045449287878,3.28632534162432));
#144975=CARTESIAN_POINT('Ctrl Pts',(6.68611994757602,1.42404710663606,3.30483501978555));
#144976=CARTESIAN_POINT('Ctrl Pts',(6.72350284131941,1.41778968831898,3.323328081582));
#144977=CARTESIAN_POINT('',(6.28430937880036,1.32710049321648,3.85790825263968));
#144978=CARTESIAN_POINT('Origin',(-9.2070448487469E-13,1.41887506700011,
-4.28043017697277E-13));
#144979=CARTESIAN_POINT('',(6.72559820178556,1.23689319341789,3.31908553997918));
#144980=CARTESIAN_POINT('Origin',(-0.145336716879659,1.48200507781202,-0.114727120736509));
#144981=CARTESIAN_POINT('',(6.95550723709846,1.32710049399577,2.80551583431356));
#144982=CARTESIAN_POINT('Origin',(-0.179225865589576,1.33928283772879,-0.070171649672468));
#144983=CARTESIAN_POINT('Origin',(-0.166147914169609,1.48212074243726,-0.093650624888299));
#144984=CARTESIAN_POINT('Ctrl Pts',(6.497431315,1.457976823,3.216502185));
#144985=CARTESIAN_POINT('Ctrl Pts',(6.673037196,1.39227158,2.861773014));
#144986=CARTESIAN_POINT('Ctrl Pts',(6.808981371,1.327100493,2.490034677));
#144987=CARTESIAN_POINT('Ctrl Pts',(6.608741086,1.457976823,3.546059963));
#144988=CARTESIAN_POINT('Ctrl Pts',(6.802339271,1.39227158,3.185253802));
#144989=CARTESIAN_POINT('Ctrl Pts',(6.955507232,1.327100493,2.805515843));
#144990=CARTESIAN_POINT('',(6.88224430779951,1.32710049586375,2.64777524362598));
#144991=CARTESIAN_POINT('Ctrl Pts',(6.80898137100001,1.327100493,2.490034677));
#144992=CARTESIAN_POINT('Ctrl Pts',(6.94467186700001,1.392692987,2.118990022));
#144993=CARTESIAN_POINT('Ctrl Pts',(7.039239622,1.45796923,1.735397808));
#144994=CARTESIAN_POINT('Ctrl Pts',(7.124462536,1.327100493,2.343508816));
#144995=CARTESIAN_POINT('Ctrl Pts',(7.252168337,1.392692987,1.955272514));
#144996=CARTESIAN_POINT('Ctrl Pts',(7.336930563,1.45796923,1.555458103));
#144997=CARTESIAN_POINT('',(7.12446253897948,1.32710049307754,2.34350881176759));
#144998=CARTESIAN_POINT('',(7.28072838188157,1.41778968870772,1.80027615161597));
#144999=CARTESIAN_POINT('Origin',(-0.183850292341285,1.33928591987418,-0.0584219215698881));
#145000=CARTESIAN_POINT('Ctrl Pts',(7.03811310959639,1.45719264069764,1.7399608805707));
#145001=CARTESIAN_POINT('Ctrl Pts',(7.07848058142795,1.45030198665873,1.75003921115543));
#145002=CARTESIAN_POINT('Ctrl Pts',(7.11890445475644,1.44357824413122,1.76010875955486));
#145003=CARTESIAN_POINT('Ctrl Pts',(7.19976342611434,1.43045449288012,1.78020933350881));
#145004=CARTESIAN_POINT('Ctrl Pts',(7.24024401785159,1.42404710660719,1.79025166512369));
#145005=CARTESIAN_POINT('Ctrl Pts',(7.28072838168565,1.41778968831362,1.8002761521612));
#145006=CARTESIAN_POINT('',(6.96672195306172,1.32710049321648,2.41677174776343));
#145007=CARTESIAN_POINT('Origin',(1.22471477403963E-12,1.41887506700044,
2.97830336781768E-13));
#145008=CARTESIAN_POINT('',(7.2818627332403,1.23689319338706,1.79568235838578));
#145009=CARTESIAN_POINT('Origin',(-0.166601486859206,1.48200500153013,-0.0808016886821614));
#145010=CARTESIAN_POINT('',(7.3959943171118,1.32710049399578,1.24469598041886));
#145011=CARTESIAN_POINT('Origin',(-0.19012037374844,1.33928284375318,-0.0300027825352343));
#145012=CARTESIAN_POINT('Origin',(-0.182395433175825,1.48212077510888,-0.0557442137474637));
#145013=CARTESIAN_POINT('Ctrl Pts',(7.036977872,1.457976823,1.744546481));
#145014=CARTESIAN_POINT('Ctrl Pts',(7.1322219,1.39227158,1.360360608));
#145015=CARTESIAN_POINT('Ctrl Pts',(7.185075021,1.327100493,0.968089328));
#145016=CARTESIAN_POINT('Ctrl Pts',(7.216530463,1.457976823,2.042471071));
#145017=CARTESIAN_POINT('Ctrl Pts',(7.328039771,1.39227158,1.648482471));
#145018=CARTESIAN_POINT('Ctrl Pts',(7.395994314,1.327100493,1.24469599));
#145019=CARTESIAN_POINT('',(7.29053467013232,1.32710049586378,1.10639264165444));
#145020=CARTESIAN_POINT('Ctrl Pts',(7.185075021,1.327100493,0.968089328));
#145021=CARTESIAN_POINT('Ctrl Pts',(7.237829515,1.392692987,0.576550044));
#145022=CARTESIAN_POINT('Ctrl Pts',(7.247725342,1.45796923,0.181596731));
#145023=CARTESIAN_POINT('Ctrl Pts',(7.461681683,1.327100493,0.757170034));
#145024=CARTESIAN_POINT('Ctrl Pts',(7.502942465,1.392692987,0.350557509));
#145025=CARTESIAN_POINT('Ctrl Pts',(7.499774717,1.45796923,-0.058130836));
#145026=CARTESIAN_POINT('Ctrl Pts',(7.24760609256058,1.45719264067756,0.186295288436271));
#145027=CARTESIAN_POINT('Ctrl Pts',(7.28919633564811,1.45030198710193,0.187460180071232));
#145028=CARTESIAN_POINT('Ctrl Pts',(7.33083977304701,1.44357824510147,0.188604370185033));
#145029=CARTESIAN_POINT('Ctrl Pts',(7.41412934238839,1.43045449282631,0.190852715567777));
#145030=CARTESIAN_POINT('Ctrl Pts',(7.45582232469342,1.42404710658477,0.191958132493221));
#145031=CARTESIAN_POINT('Ctrl Pts',(7.49751515510443,1.41778968828417,0.193045311129516));
#145032=CARTESIAN_POINT('',(7.32337835184357,1.32710049321648,0.862629682328108));
#145033=CARTESIAN_POINT('Ctrl Pts',(7.247483165,1.457976823,0.191017723));
#145034=CARTESIAN_POINT('Ctrl Pts',(7.25791183400001,1.39227158,-0.204660748));
#145035=CARTESIAN_POINT('Ctrl Pts',(7.22520254800001,1.327100493,-0.599122803));
#145036=CARTESIAN_POINT('Ctrl Pts',(7.486882896,1.457976823,0.443378502));
#145037=CARTESIAN_POINT('Ctrl Pts',(7.511089276,1.39227158,0.034629932));
#145038=CARTESIAN_POINT('Ctrl Pts',(7.490652922,1.327100493,-0.374324464));
#145039=CARTESIAN_POINT('',(7.357927733842,1.32710049586375,-0.486723651005759));
#145040=CARTESIAN_POINT('Ctrl Pts',(7.225202548,1.327100493,-0.599122803));
#145041=CARTESIAN_POINT('Ctrl Pts',(7.1925543,1.392692987,-0.992848772000001));
#145042=CARTESIAN_POINT('Ctrl Pts',(7.11731548,1.45796923,-1.380695607));
#145043=CARTESIAN_POINT('Ctrl Pts',(7.450000887,1.327100493,-0.864573176000001));
#145044=CARTESIAN_POINT('Ctrl Pts',(7.402887342,1.392692987,-1.270549175));
#145045=CARTESIAN_POINT('Ctrl Pts',(7.311937741,1.45796923,-1.669001641));
#145046=CARTESIAN_POINT('',(7.45000088793103,1.32710049307756,-0.864573181109506));
#145047=CARTESIAN_POINT('',(7.3637264526154,1.41778968836978,-1.4232121145184));
#145048=CARTESIAN_POINT('Origin',(-0.191388337446107,1.33928597468727,0.0241743755201032));
#145049=CARTESIAN_POINT('Ctrl Pts',(7.11820906946345,1.45719264072522,-1.37608126440437));
#145050=CARTESIAN_POINT('Ctrl Pts',(7.15907737221457,1.45030198732391,-1.38388427974216));
#145051=CARTESIAN_POINT('Ctrl Pts',(7.19999317518224,1.44357824550689,-1.39171894784093));
#145052=CARTESIAN_POINT('Ctrl Pts',(7.28181881080215,1.4304544928872,-1.40742796307507));
#145053=CARTESIAN_POINT('Ctrl Pts',(7.32277466610963,1.42404710668474,-1.41531114880329));
#145054=CARTESIAN_POINT('Ctrl Pts',(7.36372645274274,1.41778968836392,-1.42321211385375));
#145055=CARTESIAN_POINT('',(7.33760171763273,1.32710049321648,-0.731847988169313));
#145056=CARTESIAN_POINT('Origin',(-1.76941794549634E-13,1.41887506699994,
1.32814766129474E-14));
#145057=CARTESIAN_POINT('',(7.36282707778784,1.23689319393736,-1.42785763063424));
#145058=CARTESIAN_POINT('Origin',(-0.185131207741326,1.48200499910506,-0.00337946924173715));
#145059=CARTESIAN_POINT('',(7.235056922811,1.32710049399576,-1.97584193198526));
#145060=CARTESIAN_POINT('Origin',(-0.185146488048183,1.33928285163288,0.0525997022622385));
#145061=CARTESIAN_POINT('Origin',(-0.18894410901323,1.48212075846602,0.025993811794856));
#145062=CARTESIAN_POINT('Ctrl Pts',(7.1191042,1.457976823,-1.371442812));
#145063=CARTESIAN_POINT('Ctrl Pts',(7.044229877,1.39227158,-1.760112396));
#145064=CARTESIAN_POINT('Ctrl Pts',(6.927487635,1.327100493,-2.138320617));
#145065=CARTESIAN_POINT('Ctrl Pts',(7.407157006,1.457976823,-1.176445953));
#145066=CARTESIAN_POINT('Ctrl Pts',(7.342928594,1.39227158,-1.580841865));
#145067=CARTESIAN_POINT('Ctrl Pts',(7.235056924,1.327100493,-1.975841922));
#145068=CARTESIAN_POINT('',(7.08127227460586,1.32710049586375,-2.05708128634755));
#145069=CARTESIAN_POINT('Ctrl Pts',(6.927487635,1.327100493,-2.138320617));
#145070=CARTESIAN_POINT('Ctrl Pts',(6.81096324000001,1.392692987,-2.515823084));
#145071=CARTESIAN_POINT('Ctrl Pts',(6.654107857,1.45796923,-2.878428153));
#145072=CARTESIAN_POINT('Ctrl Pts',(7.08996633,1.327100493,-2.445889906));
#145073=CARTESIAN_POINT('Ctrl Pts',(6.95668143399999,1.392692987,-2.832246392));
#145074=CARTESIAN_POINT('Ctrl Pts',(6.782202682,1.45796923,-3.201831785));
#145075=CARTESIAN_POINT('',(7.08996632981088,1.32710049307755,-2.44588991119078));
#145076=CARTESIAN_POINT('',(6.88561808541865,1.41778968873307,-2.97292172375148));
#145077=CARTESIAN_POINT('Origin',(-0.181717156461203,1.33928595031602,0.0647520808744406));
#145078=CARTESIAN_POINT('Ctrl Pts',(6.65597250213184,1.45719264070752,-2.87411378637646));
#145079=CARTESIAN_POINT('Ctrl Pts',(6.69420791070999,1.4503019869917,-2.89051984943257));
#145080=CARTESIAN_POINT('Ctrl Pts',(6.73248290497789,1.44357824482253,-2.90696703651909));
#145081=CARTESIAN_POINT('Ctrl Pts',(6.80901852462497,1.43045449289926,-2.93989887497759));
#145082=CARTESIAN_POINT('Ctrl Pts',(6.84732220312894,1.42404710664931,-2.95640205460633));
#145083=CARTESIAN_POINT('Ctrl Pts',(6.88561808565608,1.41778968834761,-2.97292172305506));
#145084=CARTESIAN_POINT('',(7.00872698291568,1.32710049321648,-2.29210526022896));
#145085=CARTESIAN_POINT('Origin',(-2.77555756156289E-14,1.41887506699994,
8.43509290193722E-14));
#145086=CARTESIAN_POINT('',(6.8837410893577,1.23689319389077,-2.97726529079312));
#145087=CARTESIAN_POINT('Origin',(-0.181529237000969,1.4820050380168,0.0364971907420908));
#145088=CARTESIAN_POINT('',(6.6411577026872,1.32710049399577,-3.48497121750172));
#145089=CARTESIAN_POINT('Origin',(-0.169510333087188,1.33928284453501,0.0911709027947322));
#145090=CARTESIAN_POINT('Origin',(-0.178938564863871,1.48212079557788,0.0660033679166011));
#145091=CARTESIAN_POINT('Ctrl Pts',(6.657843835,1.457976823,-2.869776205));
#145092=CARTESIAN_POINT('Ctrl Pts',(6.501167561,1.39227158,-3.233263144));
#145093=CARTESIAN_POINT('Ctrl Pts',(6.30585110000001,1.327100493,-3.577532936));
#145094=CARTESIAN_POINT('Ctrl Pts',(6.98108068700001,1.457976823,-2.741261103));
#145095=CARTESIAN_POINT('Ctrl Pts',(6.831420733,1.39227158,-3.122395253));
#145096=CARTESIAN_POINT('Ctrl Pts',(6.641157706,1.327100493,-3.484971208));
#145097=CARTESIAN_POINT('',(6.47350439459855,1.32710049586375,-3.53125208740157));
#145098=CARTESIAN_POINT('Ctrl Pts',(6.30585110000001,1.327100493,-3.577532936));
#145099=CARTESIAN_POINT('Ctrl Pts',(6.110899109,1.392692987,-3.921160304));
#145100=CARTESIAN_POINT('Ctrl Pts',(5.879761546,1.45796923,-4.241568597));
#145101=CARTESIAN_POINT('Ctrl Pts',(6.39841282800001,1.327100493,-3.912839543));
#145102=CARTESIAN_POINT('Ctrl Pts',(6.18518883400001,1.392692987,-4.261510916));
#145103=CARTESIAN_POINT('Ctrl Pts',(5.935339364,1.45796923,-4.584947834));
#145104=CARTESIAN_POINT('',(6.39841282671024,1.32710049307753,-3.91283954797586));
#145105=CARTESIAN_POINT('',(6.08554586929491,1.41778968832474,-4.38362081670148));
#145106=CARTESIAN_POINT('Origin',(-0.163549035479708,1.33928597081891,0.102302120919976));
#145107=CARTESIAN_POINT('Ctrl Pts',(5.88251005789048,1.4571926407563,-4.23775594170644));
#145108=CARTESIAN_POINT('Ctrl Pts',(5.91632472464706,1.45030198716551,-4.26199792231317));
#145109=CARTESIAN_POINT('Ctrl Pts',(5.95016921096982,1.44357824513485,-4.2862885751256));
#145110=CARTESIAN_POINT('Ctrl Pts',(6.01783610014625,1.43045449287505,-4.33490338257605));
#145111=CARTESIAN_POINT('Ctrl Pts',(6.05169656390113,1.42404710665394,-4.35925488554331));
#145112=CARTESIAN_POINT('Ctrl Pts',(6.08554586967107,1.41778968831878,-4.38362081617738));
#145113=CARTESIAN_POINT('',(6.3521319646792,1.32710049321648,-3.74518623834803));
#145114=CARTESIAN_POINT('Origin',(-1.2490009027033E-13,1.41887506700011,
1.69569219776733E-13));
#145115=CARTESIAN_POINT('',(6.08277901767368,1.23689319337626,-4.38745933493388));
#145116=CARTESIAN_POINT('Origin',(-0.169439546157523,1.4820050469827,0.07466746421667));
#145117=CARTESIAN_POINT('',(5.73672532969594,1.32710049399578,-4.8311471225857));
#145118=CARTESIAN_POINT('Origin',(-0.145948341934135,1.33928281056974,0.125479154956001));
#145119=CARTESIAN_POINT('Origin',(-0.160566641850736,1.48212079340995,0.102926998199179));
#145120=CARTESIAN_POINT('Ctrl Pts',(5.88527009200001,1.457976823,-4.233922052));
#145121=CARTESIAN_POINT('Ctrl Pts',(5.654117875,1.39227158,-4.555230101));
#145122=CARTESIAN_POINT('Ctrl Pts',(5.389359975,1.327100493,-4.849463791));
#145123=CARTESIAN_POINT('Ctrl Pts',(6.228576794,1.457976823,-4.17789793));
#145124=CARTESIAN_POINT('Ctrl Pts',(6.00048323,1.39227158,-4.517948909));
#145125=CARTESIAN_POINT('Ctrl Pts',(5.736725335,1.327100493,-4.831147114));
#145126=CARTESIAN_POINT('',(5.5630426434841,1.32710049586375,-4.84030546573543));
#145127=CARTESIAN_POINT('Ctrl Pts',(5.389359975,1.327100493,-4.84946379100001));
#145128=CARTESIAN_POINT('Ctrl Pts',(5.12509612700001,1.392692987,-5.143148427));
#145129=CARTESIAN_POINT('Ctrl Pts',(4.83048412,1.45796923,-5.406378008));
#145130=CARTESIAN_POINT('Ctrl Pts',(5.407676652,1.327100493,-5.19682915100001));
#145131=CARTESIAN_POINT('Ctrl Pts',(5.124483679,1.392692987,-5.491511925));
#145132=CARTESIAN_POINT('Ctrl Pts',(4.810946174,1.45796923,-5.753676817));
#145133=CARTESIAN_POINT('',(5.40767664965581,1.32710049307754,-5.19682915561586));
#145134=CARTESIAN_POINT('',(5.00092029201621,1.41778968872508,-5.58934667278783));
#145135=CARTESIAN_POINT('Origin',(-0.137733409524872,1.3392859291023,0.13506852863573));
#145136=CARTESIAN_POINT('Ctrl Pts',(4.83398798137623,1.4571926407555,-5.40324533971124));
#145137=CARTESIAN_POINT('Ctrl Pts',(4.86180076686648,1.45030198814266,-5.43418970569204));
#145138=CARTESIAN_POINT('Ctrl Pts',(4.88963221080027,1.44357824720297,-5.4651880153085));
#145139=CARTESIAN_POINT('Ctrl Pts',(4.94526634773805,1.43045449293385,-5.52721262607228));
#145140=CARTESIAN_POINT('Ctrl Pts',(4.97310031956659,1.4240471066704,-5.55827380345815));
#145141=CARTESIAN_POINT('Ctrl Pts',(5.00092029250508,1.41778968834774,-5.58934667227415));
#145142=CARTESIAN_POINT('',(5.39851831441096,1.32710049321648,-5.02314647002097));
#145143=CARTESIAN_POINT('Origin',(-2.20309881449055E-13,1.418875067,1.64365049348802E-13));
#145144=CARTESIAN_POINT('',(4.99739295983039,1.23689319338241,-5.592500657182));
#145145=CARTESIAN_POINT('Origin',(-0.149426903870843,1.48200504998636,0.109346318495925));
#145146=CARTESIAN_POINT('',(4.56405005599846,1.32710049399577,-5.95142395623471));
#145147=CARTESIAN_POINT('Origin',(-0.115561916453181,1.33928286887368,0.153920220597338));
#145148=CARTESIAN_POINT('Origin',(-0.134686256036152,1.48212078565201,0.135037521671934));
#145149=CARTESIAN_POINT('Ctrl Pts',(4.837507661,1.457976823,-5.40009441));
#145150=CARTESIAN_POINT('Ctrl Pts',(4.542687921,1.39227158,-5.66419956100001));
#145151=CARTESIAN_POINT('Ctrl Pts',(4.220868368,1.327100493,-5.894639109));
#145152=CARTESIAN_POINT('Ctrl Pts',(5.184831573,1.457976823,-5.419180894));
#145153=CARTESIAN_POINT('Ctrl Pts',(4.88896980099999,1.39227158,-5.702248296));
#145154=CARTESIAN_POINT('Ctrl Pts',(4.564050063,1.327100493,-5.95142394900001));
#145155=CARTESIAN_POINT('',(4.3924592014081,1.32710049586375,-5.92303153945041));
#145156=CARTESIAN_POINT('Ctrl Pts',(4.220868368,1.327100493,-5.894639109));
#145157=CARTESIAN_POINT('Ctrl Pts',(3.899649346,1.392692987,-6.12464864500001));
#145158=CARTESIAN_POINT('Ctrl Pts',(3.555338625,1.45796923,-6.318391192));
#145159=CARTESIAN_POINT('Ctrl Pts',(4.164083527,1.327100493,-6.23782080400001));
#145160=CARTESIAN_POINT('Ctrl Pts',(3.824163362,1.392692987,-6.46473594));
#145161=CARTESIAN_POINT('Ctrl Pts',(3.461598487,1.45796923,-6.653370267));
#145162=CARTESIAN_POINT('',(4.16408352373067,1.32710049307753,-6.23782080798727));
#145163=CARTESIAN_POINT('',(3.68245723961584,1.41778968871537,-6.53372089029738));
#145164=CARTESIAN_POINT('Origin',(-0.105477626068154,1.33928591507701,0.16151946653965));
#145165=CARTESIAN_POINT('Ctrl Pts',(3.55943399894129,1.45719264078608,-6.31608499055301));
#145166=CARTESIAN_POINT('Ctrl Pts',(3.57994441222619,1.45030198841067,-6.35228481987964));
#145167=CARTESIAN_POINT('Ctrl Pts',(3.60046145127134,1.44357824774572,-6.38854134236741));
#145168=CARTESIAN_POINT('Ctrl Pts',(3.64146143676512,1.4304544929359,-6.46107555007232));
#145169=CARTESIAN_POINT('Ctrl Pts',(3.66196743092277,1.4240471066378,-6.4973940157844));
#145170=CARTESIAN_POINT('Ctrl Pts',(3.68245724002035,1.41778968832776,-6.53372089000245));
#145171=CARTESIAN_POINT('',(4.19247594860012,1.32710049321648,-6.06622995573969));
#145172=CARTESIAN_POINT('Origin',(3.16587034365767E-14,1.41887506700044,
3.59955121265187E-14));
#145173=CARTESIAN_POINT('',(3.67833436110066,1.23689319337654,-6.53604286387826));
#145174=CARTESIAN_POINT('Origin',(-0.122427019057876,1.48200506328858,0.138912014578856));
#145175=CARTESIAN_POINT('',(3.17796487359877,1.32710049399579,-6.79341882156193));
#145176=CARTESIAN_POINT('Origin',(-0.0797718656725155,1.3392828592108,0.175164068385654));
#145177=CARTESIAN_POINT('Origin',(-0.102508324529246,1.48212078864541,0.160834037739207));
#145178=CARTESIAN_POINT('Ctrl Pts',(3.563548747,1.457976823,-6.313764355));
#145179=CARTESIAN_POINT('Ctrl Pts',(3.218846929,1.39227158,-6.508317345));
#145180=CARTESIAN_POINT('Ctrl Pts',(2.855013647,1.327100493,-6.664187653));
#145181=CARTESIAN_POINT('Ctrl Pts',(3.89864939,1.457976823,-6.407068982));
#145182=CARTESIAN_POINT('Ctrl Pts',(3.548853577,1.39227158,-6.61991689));
#145183=CARTESIAN_POINT('Ctrl Pts',(3.177964882,1.327100493,-6.793418816));
#145184=CARTESIAN_POINT('',(3.01648924849091,1.32710049586378,-6.7288032416768));
#145185=CARTESIAN_POINT('Ctrl Pts',(2.855013647,1.327100493,-6.664187653));
#145186=CARTESIAN_POINT('Ctrl Pts',(2.491859296,1.392692987,-6.8197671));
#145187=CARTESIAN_POINT('Ctrl Pts',(2.113949448,1.45796923,-6.934963427));
#145188=CARTESIAN_POINT('Ctrl Pts',(2.725782484,1.327100493,-6.987138889));
#145189=CARTESIAN_POINT('Ctrl Pts',(2.345029417,1.392692987,-7.135676088));
#145190=CARTESIAN_POINT('Ctrl Pts',(1.950390303,1.45796923,-7.241959518));
#145191=CARTESIAN_POINT('',(2.72578247995464,1.32710049307753,-6.98713889218714));
#145192=CARTESIAN_POINT('',(2.19180657984862,1.41778968871566,-7.17258558065227));
#145193=CARTESIAN_POINT('Origin',(-0.0682896582737541,1.3392859226996,0.180417665261952));
#145194=CARTESIAN_POINT('Ctrl Pts',(2.11844483962399,1.45719264080791,-6.93359152718499));
#145195=CARTESIAN_POINT('Ctrl Pts',(2.13069383942566,1.45030198735574,-6.97335416332043));
#145196=CARTESIAN_POINT('Ctrl Pts',(2.14293712316127,1.44357824549033,-7.01317359293416));
#145197=CARTESIAN_POINT('Ctrl Pts',(2.16738583696781,1.4304544929153,-7.09282576249553));
#145198=CARTESIAN_POINT('Ctrl Pts',(2.17960501575865,1.42404710663496,-7.13270330513909));
#145199=CARTESIAN_POINT('Ctrl Pts',(2.19180658033942,1.41778968833467,-7.17258558044234));
#145200=CARTESIAN_POINT('',(2.79039806673785,1.32710049321648,-6.82566327049396));
#145201=CARTESIAN_POINT('Origin',(3.71881345162528E-14,1.41887506700011,
-1.01047642475649E-13));
#145202=CARTESIAN_POINT('',(2.18728093607641,1.23689319391963,-7.17396697093756));
#145203=CARTESIAN_POINT('Origin',(-0.089702922527658,1.48200508663554,0.161982950661606));
#145204=CARTESIAN_POINT('',(1.64328158659184,1.32710049399579,-7.31776097262557));
#145205=CARTESIAN_POINT('Origin',(-0.0402517051760135,1.33928286958148,
0.188217277654796));
#145206=CARTESIAN_POINT('Origin',(-0.0655371205933414,1.48212079741191,
0.179109882251318));
#145207=CARTESIAN_POINT('Ctrl Pts',(2.122962255,1.457976823,-6.932209696));
#145208=CARTESIAN_POINT('Ctrl Pts',(1.744496231,1.39227158,-7.048113443));
#145209=CARTESIAN_POINT('Ctrl Pts',(1.355661661,1.327100493,-7.12212619));
#145210=CARTESIAN_POINT('Ctrl Pts',(2.430170694,1.457976823,-7.09536964500001));
#145211=CARTESIAN_POINT('Ctrl Pts',(2.042796905,1.39227158,-7.228045528));
#145212=CARTESIAN_POINT('Ctrl Pts',(1.643281596,1.327100493,-7.317760969));
#145213=CARTESIAN_POINT('',(1.49947161132239,1.32710049586378,-7.21994358306752));
#145214=CARTESIAN_POINT('Ctrl Pts',(1.355661661,1.327100493,-7.12212619));
#145215=CARTESIAN_POINT('Ctrl Pts',(0.967552675,1.392692987,-7.196000825));
#145216=CARTESIAN_POINT('Ctrl Pts',(0.573714344,1.45796923,-7.227264479));
#145217=CARTESIAN_POINT('Ctrl Pts',(1.160026882,1.327100493,-7.409746125));
#145218=CARTESIAN_POINT('Ctrl Pts',(0.756244503,1.392692987,-7.472959952));
#145219=CARTESIAN_POINT('Ctrl Pts',(0.347984036,1.45796923,-7.49192279100001));
#145220=CARTESIAN_POINT('',(1.16002687736292,1.32710049307753,-7.40974612724363));
#145221=CARTESIAN_POINT('',(0.598669480427782,1.41778968873146,-7.47606814079839));
#145222=CARTESIAN_POINT('Origin',(-0.0279086337482035,1.33928591269015,
0.190879995901798));
#145223=CARTESIAN_POINT('Ctrl Pts',(0.57839955397464,1.4571926407453,-7.22689102994081));
#145224=CARTESIAN_POINT('Ctrl Pts',(0.58181438724212,1.45030198803244,-7.26835720625018));
#145225=CARTESIAN_POINT('Ctrl Pts',(0.585211429058528,1.44357824698866,
-7.3098776184735));
#145226=CARTESIAN_POINT('Ctrl Pts',(0.591965684310373,1.43045449291614,
-7.39292332494198));
#145227=CARTESIAN_POINT('Ctrl Pts',(0.595326692564369,1.42404710663884,
-7.43449531507666));
#145228=CARTESIAN_POINT('Ctrl Pts',(0.598669481038226,1.41778968834016,
-7.4760681406904));
#145229=CARTESIAN_POINT('',(1.25784427281769,1.32710049321648,-7.26593615727189));
#145230=CARTESIAN_POINT('Origin',(-3.11030498231779E-14,1.41887506699989,
9.69710423071035E-13));
#145231=CARTESIAN_POINT('',(0.593952685545576,1.23689319338997,-7.47644435575005));
#145232=CARTESIAN_POINT('Origin',(-0.0527841180949516,1.48200502603679,
0.177478958827875));
#145233=CARTESIAN_POINT('',(0.0317602790409959,1.32710049399578,-7.49993275352055));
#145234=CARTESIAN_POINT('Origin',(0.00115051940608922,1.33928289169456,
0.192469725776021));
#145235=CARTESIAN_POINT('Origin',(-0.0255015599625236,1.48212074045013,
0.189010913845458));
#145236=CARTESIAN_POINT('Ctrl Pts',(0.583108408,1.457976823,-7.22651261599999));
#145237=CARTESIAN_POINT('Ctrl Pts',(0.188574829,1.39227158,-7.25834759));
#145238=CARTESIAN_POINT('Ctrl Pts',(-0.207079558,1.327100493,-7.247042021));
#145239=CARTESIAN_POINT('Ctrl Pts',(0.848059918,1.457976823,-7.451898709));
#145240=CARTESIAN_POINT('Ctrl Pts',(0.441221319,1.39227158,-7.49819879));
#145241=CARTESIAN_POINT('Ctrl Pts',(0.031760289,1.327100493,-7.499932752));
#145242=CARTESIAN_POINT('',(-0.0876596520427781,1.32710049586375,-7.37348738629144));
#145243=CARTESIAN_POINT('Ctrl Pts',(-0.207079558,1.327100493,-7.247042021));
#145244=CARTESIAN_POINT('Ctrl Pts',(-0.601995634,1.392692987,-7.235757549));
#145245=CARTESIAN_POINT('Ctrl Pts',(-0.993347006,1.45796923,-7.181626677));
#145246=CARTESIAN_POINT('Ctrl Pts',(-0.459970288,1.327100493,-7.485881867));
#145247=CARTESIAN_POINT('Ctrl Pts',(-0.867901564,1.392692987,-7.460816515));
#145248=CARTESIAN_POINT('Ctrl Pts',(-1.270693578,1.45796923,-7.391572081));
#145249=CARTESIAN_POINT('',(-0.459970293053227,1.32710049307755,-7.48588186820677));
#145250=CARTESIAN_POINT('',(-1.02246073861237,1.41778968870741,-7.42997806403628));
#145251=CARTESIAN_POINT('Origin',(0.0137773865831164,1.33928592088847,0.192416720129659));
#145252=CARTESIAN_POINT('Ctrl Pts',(-0.988691052623812,1.45719264069763,
-7.1822691405059));
#145253=CARTESIAN_POINT('Ctrl Pts',(-0.994270058772122,1.45030198759079,
-7.22349995135523));
#145254=CARTESIAN_POINT('Ctrl Pts',(-0.999878099571577,1.44357824609767,
-7.26477990600654));
#145255=CARTESIAN_POINT('Ctrl Pts',(-1.01113412627181,1.43045449289424,
-7.34733600981738));
#145256=CARTESIAN_POINT('Ctrl Pts',(-1.01678844545818,1.42404710661956,
-7.38865858731562));
#145257=CARTESIAN_POINT('Ctrl Pts',(-1.02246073805733,1.41778968831938,
-7.42997806405372));
#145258=CARTESIAN_POINT('',(-0.333524921664078,1.32710049321648,-7.36646194406049));
#145259=CARTESIAN_POINT('Origin',(1.71493678632895E-13,1.41887506700022,
1.13537651502682E-12));
#145260=CARTESIAN_POINT('',(-1.02714813242582,1.2368931933649,-7.42933151171882));
#145261=CARTESIAN_POINT('Origin',(-0.0133973341289943,1.48200503132719,
0.184676639741399));
#145262=CARTESIAN_POINT('',(-1.58124610403663,1.32710049399577,-7.33141601435253));
#145263=CARTESIAN_POINT('Origin',(0.0424989283865376,1.33928286297151,0.187722593615965));
#145264=CARTESIAN_POINT('Origin',(0.0157264465032626,1.48212080514855,0.190074241480158));
#145265=CARTESIAN_POINT('Ctrl Pts',(-0.984010941,1.457976823,-7.18291183800001));
#145266=CARTESIAN_POINT('Ctrl Pts',(-1.376164122,1.39227158,-7.129189471));
#145267=CARTESIAN_POINT('Ctrl Pts',(-1.760137966,1.327100493,-7.033094222));
#145268=CARTESIAN_POINT('Ctrl Pts',(-0.773705198,1.457976823,-7.459985273));
#145269=CARTESIAN_POINT('Ctrl Pts',(-1.180985284,1.39227158,-7.41774461));
#145270=CARTESIAN_POINT('Ctrl Pts',(-1.581246094,1.327100493,-7.331416015));
#145271=CARTESIAN_POINT('',(-1.67069204708794,1.32710049586378,-7.1822551145251));
#145272=CARTESIAN_POINT('Ctrl Pts',(-1.760137966,1.327100493,-7.033094222));
#145273=CARTESIAN_POINT('Ctrl Pts',(-2.143395296,1.392692987,-6.937178292));
#145274=CARTESIAN_POINT('Ctrl Pts',(-2.513960553,1.45796923,-6.800183993));
#145275=CARTESIAN_POINT('Ctrl Pts',(-2.058459759,1.327100493,-7.211986094));
#145276=CARTESIAN_POINT('Ctrl Pts',(-2.451465519,1.392692987,-7.09981359));
#145277=CARTESIAN_POINT('Ctrl Pts',(-2.829954972,1.45796923,-6.945599676));
#145278=CARTESIAN_POINT('',(-2.05845976416771,1.32710049307754,-7.21198609409039));
#145279=CARTESIAN_POINT('',(-2.59578182999002,1.41778968871659,-7.03647047077191));
#145280=CARTESIAN_POINT('Origin',(0.0548191445060356,1.33928597923113,0.184956220145635));
#145281=CARTESIAN_POINT('Ctrl Pts',(-2.50955156393115,1.45719264070531,
-6.80181232839606));
#145282=CARTESIAN_POINT('Ctrl Pts',(-2.52386354155141,1.45030198756959,
-6.84087986462242));
#145283=CARTESIAN_POINT('Ctrl Pts',(-2.53821443953213,1.44357824604334,
-6.87998915413039));
#145284=CARTESIAN_POINT('Ctrl Pts',(-2.56695442844666,1.43045449288437,
-6.95819542891081));
#145285=CARTESIAN_POINT('Ctrl Pts',(-2.58135968539634,1.42404710665183,
-6.99733639579766));
#145286=CARTESIAN_POINT('Ctrl Pts',(-2.59578182913589,1.41778968833431,
-7.03647047102556));
#145287=CARTESIAN_POINT('',(-1.90929886120832,1.32710049321648,-7.12254015834626));
#145288=CARTESIAN_POINT('Origin',(1.91036422791946E-13,1.41887506700006,
4.19369400317393E-13));
#145289=CARTESIAN_POINT('',(-2.6002206454442,1.23689319337841,-7.03483138298698));
#145290=CARTESIAN_POINT('Origin',(0.0266158908061881,1.4820050282617,0.183238948990568));
#145291=CARTESIAN_POINT('',(-3.1203151776828,1.32710049399577,-6.82009041119354));
#145292=CARTESIAN_POINT('Origin',(0.0818601302556743,1.33928285452991,0.174197751694014));
#145293=CARTESIAN_POINT('Origin',(0.0562190792265915,1.48212077788429,0.182249609777169));
#145294=CARTESIAN_POINT('Ctrl Pts',(-2.505119032,1.457976823,-6.803446085));
#145295=CARTESIAN_POINT('Ctrl Pts',(-2.876555169,1.39227158,-6.666678376));
#145296=CARTESIAN_POINT('Ctrl Pts',(-3.23089428,1.327100493,-6.490286754));
#145297=CARTESIAN_POINT('Ctrl Pts',(-2.359292718,1.457976823,-7.119251215));
#145298=CARTESIAN_POINT('Ctrl Pts',(-2.747970329,1.39227158,-6.990444937));
#145299=CARTESIAN_POINT('Ctrl Pts',(-3.120315168,1.327100493,-6.820090414));
#145300=CARTESIAN_POINT('',(-3.17560473983382,1.32710049586375,-6.6551885764447));
#145301=CARTESIAN_POINT('Ctrl Pts',(-3.23089428,1.327100493,-6.49028675400001));
#145302=CARTESIAN_POINT('Ctrl Pts',(-3.584572177,1.392692987,-6.314224288));
#145303=CARTESIAN_POINT('Ctrl Pts',(-3.917024099,1.45796923,-6.100772263));
#145304=CARTESIAN_POINT('Ctrl Pts',(-3.560697939,1.327100493,-6.600865866));
#145305=CARTESIAN_POINT('Ctrl Pts',(-3.92040167,1.392692987,-6.406831272));
#145306=CARTESIAN_POINT('Ctrl Pts',(-4.256890817,1.45796923,-6.174858749));
#145307=CARTESIAN_POINT('',(-3.5606979440883,1.32710049307754,-6.60086586497412));
#145308=CARTESIAN_POINT('',(-4.04772704802492,1.41778968875794,-6.31394533862323));
#145309=CARTESIAN_POINT('Origin',(0.0932976026754845,1.33928595488629,0.168847532117771));
#145310=CARTESIAN_POINT('Ctrl Pts',(-3.91306823383847,1.45719264065931,
-6.10331033138983));
#145311=CARTESIAN_POINT('Ctrl Pts',(-3.93544396831024,1.45030198834128,
-6.13838783413044));
#145312=CARTESIAN_POINT('Ctrl Pts',(-3.95786668826544,1.4435782477238,-6.17349774635459));
#145313=CARTESIAN_POINT('Ctrl Pts',(-4.00274679509976,1.43045449293981,
-6.24369736267065));
#145314=CARTESIAN_POINT('Ctrl Pts',(-4.02522941605326,1.42404710668986,
-6.27882653124007));
#145315=CARTESIAN_POINT('Ctrl Pts',(-4.0477270473829,1.41778968837934,-6.31394533896706));
#145316=CARTESIAN_POINT('',(-3.39579610831295,1.32710049321648,-6.54557631061584));
#145317=CARTESIAN_POINT('Origin',(-1.22948526359856E-13,1.41887506699989,
-2.29417179697933E-13));
#145318=CARTESIAN_POINT('',(-4.05170973089699,1.23689319338796,-6.31139035807528));
#145319=CARTESIAN_POINT('Origin',(0.065384597887963,1.4820050181001,0.173233331749791));
#145320=CARTESIAN_POINT('',(-4.5134817808578,1.32710049399579,-5.98986496017169));
#145321=CARTESIAN_POINT('Origin',(0.117393698840258,1.33928287631653,0.152527654543123));
#145322=CARTESIAN_POINT('Origin',(0.0940831752252352,1.48212079763046,0.165903555497967));
#145323=CARTESIAN_POINT('Ctrl Pts',(-3.909090541,1.457976823,-6.105858756));
#145324=CARTESIAN_POINT('Ctrl Pts',(-4.242441693,1.39227158,-5.89244081));
#145325=CARTESIAN_POINT('Ctrl Pts',(-4.550577568,1.327100493,-5.644000691));
#145326=CARTESIAN_POINT('Ctrl Pts',(-3.834562334,1.457976823,-6.445628884));
#145327=CARTESIAN_POINT('Ctrl Pts',(-4.186463335,1.39227158,-6.236279827));
#145328=CARTESIAN_POINT('Ctrl Pts',(-4.513481772,1.327100493,-5.989864965));
#145329=CARTESIAN_POINT('',(-4.53202968383947,1.32710049586375,-5.81693281721754));
#145330=CARTESIAN_POINT('Ctrl Pts',(-4.550577568,1.327100493,-5.64400069100001));
#145331=CARTESIAN_POINT('Ctrl Pts',(-4.85813844599999,1.392692987,-5.396024174));
#145332=CARTESIAN_POINT('Ctrl Pts',(-5.136931951,1.45796923,-5.116095203));
#145333=CARTESIAN_POINT('Ctrl Pts',(-4.896441841,1.327100493,-5.681096487));
#145334=CARTESIAN_POINT('Ctrl Pts',(-5.206024196,1.392692987,-5.414272644));
#145335=CARTESIAN_POINT('Ctrl Pts',(-5.484779179,1.45796923,-5.11538829));
#145336=CARTESIAN_POINT('',(-4.89644184573733,1.32710049307754,-5.68109648490863));
#145337=CARTESIAN_POINT('',(-5.31040504790184,1.41778968873636,-5.29618714009526));
#145338=CARTESIAN_POINT('Origin',(0.127413838397398,1.33928592785563,0.144844021089803));
#145339=CARTESIAN_POINT('Ctrl Pts',(-5.13361418158607,1.45719264066822,
-5.11942432679471));
#145340=CARTESIAN_POINT('Ctrl Pts',(-5.16300740979459,1.45030198839048,
-5.14887161529756));
#145341=CARTESIAN_POINT('Ctrl Pts',(-5.19245349208817,1.44357824782183,
-5.17834045502075));
#145342=CARTESIAN_POINT('Ctrl Pts',(-5.25137516994794,1.43045449293496,
-5.23725094736362));
#145343=CARTESIAN_POINT('Ctrl Pts',(-5.28088389277246,1.42404710665468,
-5.26672571666975));
#145344=CARTESIAN_POINT('Ctrl Pts',(-5.31040504754952,1.41778968836063,
-5.29618714036849));
#145345=CARTESIAN_POINT('',(-4.72350970347309,1.32710049321648,-5.66254858985662));
#145346=CARTESIAN_POINT('Origin',(1.14188172806173E-12,1.41887506700039,
1.19348975147204E-12));
#145347=CARTESIAN_POINT('',(-5.31374537261227,1.23689319338848,-5.29283573454965));
#145348=CARTESIAN_POINT('Origin',(0.101096017214738,1.48200506766614,0.155127518954754));
#145349=CARTESIAN_POINT('',(-5.69560299159707,1.32710049399576,-4.87956008041305));
#145350=CARTESIAN_POINT('Origin',(0.147437970801125,1.33928284907969,0.123725396097225));
#145351=CARTESIAN_POINT('Origin',(0.12754751488669,1.4821207950477,0.141799326758713));
#145352=CARTESIAN_POINT('Ctrl Pts',(-5.130277321,1.457976823,-5.122768257));
#145353=CARTESIAN_POINT('Ctrl Pts',(-5.409956358,1.39227158,-4.84267926));
#145354=CARTESIAN_POINT('Ctrl Pts',(-5.657480906,1.327100493,-4.533807429));
#145355=CARTESIAN_POINT('Ctrl Pts',(-5.130532076,1.457976823,-5.47061610999999));
#145356=CARTESIAN_POINT('Ctrl Pts',(-5.429201969,1.39227158,-5.190513205));
#145357=CARTESIAN_POINT('Ctrl Pts',(-5.695602984,1.327100493,-4.879560087));
#145358=CARTESIAN_POINT('',(-5.676541956198,1.32710049586375,-4.70668374449455));
#145359=CARTESIAN_POINT('Ctrl Pts',(-5.657480906,1.327100493,-4.533807429));
#145360=CARTESIAN_POINT('Ctrl Pts',(-5.904543561,1.392692987,-4.225511967));
#145361=CARTESIAN_POINT('Ctrl Pts',(-6.116642575,1.45796923,-3.892195218));
#145362=CARTESIAN_POINT('Ctrl Pts',(-6.00323356500001,1.327100493,-4.49568535));
#145363=CARTESIAN_POINT('Ctrl Pts',(-6.248218817,1.392692987,-4.168548645));
#145364=CARTESIAN_POINT('Ctrl Pts',(-6.456205362,1.45796923,-3.81672796));
#145365=CARTESIAN_POINT('',(-6.00323356916003,1.32710049307753,-4.49568534695027));
#145366=CARTESIAN_POINT('',(-6.32477440834189,1.41778968840243,-4.0307851183038));
#145367=CARTESIAN_POINT('Origin',(0.155571997664578,1.33928597345127,0.114067300424577));
#145368=CARTESIAN_POINT('Ctrl Pts',(-6.11411803582837,1.45719264067073,
-3.8961597311879));
#145369=CARTESIAN_POINT('Ctrl Pts',(-6.14915437013618,1.45030198703788,
-3.91859988746354));
#145370=CARTESIAN_POINT('Ctrl Pts',(-6.18424695723015,1.44357824495913,
-3.94104973005705));
#145371=CARTESIAN_POINT('Ctrl Pts',(-6.25445507822899,1.43045449290793,
-3.98591649887835));
#145372=CARTESIAN_POINT('Ctrl Pts',(-6.2896101072235,1.42404710669724,-4.00835866099077));
#145373=CARTESIAN_POINT('Ctrl Pts',(-6.32477440900803,1.41778968840232,
-4.03078511725927));
#145374=CARTESIAN_POINT('',(-5.83035723468124,1.32710049321648,-4.51474639055735));
#145375=CARTESIAN_POINT('Ctrl Pts',(-6.111578035,1.457976823,-3.900142807));
#145376=CARTESIAN_POINT('Ctrl Pts',(-6.324507477,1.39227158,-3.56647941));
#145377=CARTESIAN_POINT('Ctrl Pts',(-6.499846725,1.327100493,-3.21161837));
#145378=CARTESIAN_POINT('Ctrl Pts',(-6.18660384,1.457976823,-4.239803406));
#145379=CARTESIAN_POINT('Ctrl Pts',(-6.418077152,1.39227158,-3.902043953));
#145380=CARTESIAN_POINT('Ctrl Pts',(-6.611404132,1.327100493,-3.541092403));
#145381=CARTESIAN_POINT('',(-6.61140413777676,1.32710049397328,-3.54109239737487));
#145382=CARTESIAN_POINT('Origin',(0.155048589728213,1.48212078598296,0.111065447385177));
#145383=CARTESIAN_POINT('',(-6.55562543653298,1.32710049586378,-3.37635537090293));
#145384=CARTESIAN_POINT('Origin',(1.2190769227427E-12,1.41887506700017,
7.255480938273E-13));
#145385=CARTESIAN_POINT('',(-6.32731618627607,1.23689319339346,-4.0267939941612));
#145386=CARTESIAN_POINT('Origin',(0.132080172192659,1.4820050475739,0.129767978857629));
#145387=CARTESIAN_POINT('Origin',(0.170588507694899,1.33928286359429,0.0891381241734063));
#145388=CARTESIAN_POINT('Ctrl Pts',(-6.499846725,1.327100493,-3.21161837));
#145389=CARTESIAN_POINT('Ctrl Pts',(-6.67485878100001,1.392692987,-2.857419517));
#145390=CARTESIAN_POINT('Ctrl Pts',(-6.81034579,1.45796923,-2.48630051));
#145391=CARTESIAN_POINT('Ctrl Pts',(-6.829320759,1.327100493,-3.100060963));
#145392=CARTESIAN_POINT('Ctrl Pts',(-6.998253671,1.392692987,-2.727907945));
#145393=CARTESIAN_POINT('Ctrl Pts',(-7.125746559,1.45796923,-2.339601672));
#145394=CARTESIAN_POINT('',(-6.82932076240318,1.32710049307753,-3.10006095913137));
#145395=CARTESIAN_POINT('',(-6.66458374142768,1.32710049321648,-3.15583966770864));
#145396=CARTESIAN_POINT('',(-7.04340434993579,1.41778968871992,-2.57690806175739));
#145397=CARTESIAN_POINT('Origin',(0.176455929188738,1.33928593254331,0.0779571161467857));
#145398=CARTESIAN_POINT('Ctrl Pts',(-6.80873252634029,1.45719264069918,
-2.49071503621278));
#145399=CARTESIAN_POINT('Ctrl Pts',(-6.84777370210102,1.45030198685207,
-2.50509877827222));
#145400=CARTESIAN_POINT('Ctrl Pts',(-6.88687189798469,1.44357824454109,
-2.5194798876386));
#145401=CARTESIAN_POINT('Ctrl Pts',(-6.96508361886916,1.43045449287376,
-2.54820502485674));
#145402=CARTESIAN_POINT('Ctrl Pts',(-7.00424114436195,1.42404710665038,
-2.56256520971215));
#145403=CARTESIAN_POINT('Ctrl Pts',(-7.04340434957966,1.41778968834056,
-2.5769080625643));
#145404=CARTESIAN_POINT('Origin',(1.00050176476962E-12,1.41887506700017,
2.88180937446647E-13));
#145405=CARTESIAN_POINT('',(-7.21806337412951,1.32710049399578,-2.03704716480427));
#145406=CARTESIAN_POINT('Origin',(0.175299450457352,1.48212077473128,0.0751379289430554));
#145407=CARTESIAN_POINT('',(-7.04502872775174,1.23689319337173,-2.57246384258005));
#145408=CARTESIAN_POINT('Origin',(0.156888684396083,1.48200503551944,0.0983408221406673));
#145409=CARTESIAN_POINT('Origin',(0.18576194971784,1.33928286595704,0.0503825141191694));
#145410=CARTESIAN_POINT('Ctrl Pts',(-6.807108153,1.457976823,-2.495151015));
#145411=CARTESIAN_POINT('Ctrl Pts',(-6.94333165600001,1.39227158,-2.123514947));
#145412=CARTESIAN_POINT('Ctrl Pts',(-7.038286935,1.327100493,-1.739257605));
#145413=CARTESIAN_POINT('Ctrl Pts',(-6.953396885,1.457976823,-2.810742208));
#145414=CARTESIAN_POINT('Ctrl Pts',(-7.106850181,1.39227158,-2.431119463));
#145415=CARTESIAN_POINT('Ctrl Pts',(-7.21806337,1.327100493,-2.037047174));
#145416=CARTESIAN_POINT('',(-7.12817515699226,1.32710049586377,-1.88815237254077));
#145417=CARTESIAN_POINT('Ctrl Pts',(-7.03828693500001,1.327100493,-1.739257605));
#145418=CARTESIAN_POINT('Ctrl Pts',(-7.133065024,1.392692987,-1.355717306));
#145419=CARTESIAN_POINT('Ctrl Pts',(-7.185604805,1.45796923,-0.964149153));
#145420=CARTESIAN_POINT('Ctrl Pts',(-7.336076504,1.327100493,-1.55948117));
#145421=CARTESIAN_POINT('Ctrl Pts',(-7.421057961,1.392692987,-1.159713301));
#145422=CARTESIAN_POINT('Ctrl Pts',(-7.462095765,1.45796923,-0.753078211));
#145423=CARTESIAN_POINT('',(-7.33607650651547,1.32710049307755,-1.55948116545248));
#145424=CARTESIAN_POINT('',(-7.43269253076441,1.41778968874203,-1.00253764978341));
#145425=CARTESIAN_POINT('Origin',(0.189088830370302,1.33928591181856,0.0382017050499422));
#145426=CARTESIAN_POINT('Ctrl Pts',(-7.18497825126012,1.45719264073011,
-0.968807273831989));
#145427=CARTESIAN_POINT('Ctrl Pts',(-7.22619874120902,1.45030198757908,
-0.974462032848068));
#145428=CARTESIAN_POINT('Ctrl Pts',(-7.26747435133052,1.44357824604435,
-0.980101962887697));
#145429=CARTESIAN_POINT('Ctrl Pts',(-7.35003259024956,1.43045449292146,
-0.991342315629223));
#145430=CARTESIAN_POINT('Ctrl Pts',(-7.39136165010221,1.42404710665964,
-0.996949056884781));
#145431=CARTESIAN_POINT('Ctrl Pts',(-7.4326925306375,1.41778968836924,-1.00253765030459));
#145432=CARTESIAN_POINT('',(-7.18718171920089,1.32710049321647,-1.64936938880337));
#145433=CARTESIAN_POINT('Origin',(-4.55798593312906E-13,1.418875067,-1.81712284108571E-13));
#145434=CARTESIAN_POINT('',(-7.4333235556527,1.23689319336187,-0.997848140297996));
#145435=CARTESIAN_POINT('Origin',(0.174360937114771,1.48200502583182,0.0623152203927678));
#145436=CARTESIAN_POINT('',(-7.48721398905891,1.32710049399578,-0.437751873145054));
#145437=CARTESIAN_POINT('Origin',(0.192249680126575,1.33928287077358,0.00927126713742912));
#145438=CARTESIAN_POINT('Origin',(0.187353116954269,1.48212077437295,0.035697005883375));
#145439=CARTESIAN_POINT('Ctrl Pts',(-7.18434546000001,1.457976823,-0.973488735));
#145440=CARTESIAN_POINT('Ctrl Pts',(-7.237493363,1.39227158,-0.581257285));
#145441=CARTESIAN_POINT('Ctrl Pts',(-7.247624671,1.327100493,-0.185571088));
#145442=CARTESIAN_POINT('Ctrl Pts',(-7.39505682,1.457976823,-1.250253828));
#145443=CARTESIAN_POINT('Ctrl Pts',(-7.463314795,1.39227158,-0.846518529));
#145444=CARTESIAN_POINT('Ctrl Pts',(-7.487213987,1.327100493,-0.437751883));
#145445=CARTESIAN_POINT('',(-7.3674193297415,1.32710049586377,-0.311661467971566));
#145446=CARTESIAN_POINT('Ctrl Pts',(-7.247624671,1.327100493,-0.185571088));
#145447=CARTESIAN_POINT('Ctrl Pts',(-7.257737073,1.392692987,0.209376739));
#145448=CARTESIAN_POINT('Ctrl Pts',(-7.224872925,1.45796923,0.603084746));
#145449=CARTESIAN_POINT('Ctrl Pts',(-7.49980546600001,1.327100493,0.054018228));
#145450=CARTESIAN_POINT('Ctrl Pts',(-7.496861828,1.392692987,0.462708249000001));
#145451=CARTESIAN_POINT('Ctrl Pts',(-7.449525667,1.45796923,0.868658351));
#145452=CARTESIAN_POINT('',(-7.49980546747305,1.32710049307754,0.0540182329649172));
#145453=CARTESIAN_POINT('',(-7.47443626940087,1.41778968869693,0.618710308786432));
#145454=CARTESIAN_POINT('Origin',(0.192880487321588,1.33928596308834,-0.00333996688423702));
#145455=CARTESIAN_POINT('Ctrl Pts',(-7.22526237813834,1.45719264078058,
0.598400839381944));
#145456=CARTESIAN_POINT('Ctrl Pts',(-7.2667347605517,1.4503019878546,0.601739472284441));
#145457=CARTESIAN_POINT('Ctrl Pts',(-7.30825778632754,1.44357824657058,
0.605104436637895));
#145458=CARTESIAN_POINT('Ctrl Pts',(-7.39130220627353,1.43045449290774,
0.611874458356217));
#145459=CARTESIAN_POINT('Ctrl Pts',(-7.43287029941618,1.42404710661155,
0.615283325799165));
#145460=CARTESIAN_POINT('Ctrl Pts',(-7.47443626939145,1.41778968829495,
0.618710308166733));
#145461=CARTESIAN_POINT('',(-7.37371506848807,1.32710049321647,-0.0657764313371904));
#145462=CARTESIAN_POINT('Origin',(9.80118763926896E-13,1.41887506699967,
-1.8033670260223E-13));
#145463=CARTESIAN_POINT('',(-7.47404443556084,1.23689319340572,0.62342583135813));
#145464=CARTESIAN_POINT('Origin',(0.183680684593376,1.4820050856247,0.0233758683937176));
#145465=CARTESIAN_POINT('',(-7.40627079988776,1.32710049399577,1.182012209077));
#145466=CARTESIAN_POINT('Origin',(0.189748364559003,1.33928286084184,-0.0322735212225897));
#145467=CARTESIAN_POINT('Origin',(0.190646781264282,1.48212080209065,-0.00541294759872427));
#145468=CARTESIAN_POINT('Ctrl Pts',(-7.225650757,1.457976823,0.593692797));
#145469=CARTESIAN_POINT('Ctrl Pts',(-7.193237924,1.39227158,0.988179322000001));
#145470=CARTESIAN_POINT('Ctrl Pts',(-7.118071532,1.327100493,1.376792527));
#145471=CARTESIAN_POINT('Ctrl Pts',(-7.490932116,1.457976823,0.368695032));
#145472=CARTESIAN_POINT('Ctrl Pts',(-7.470803103,1.39227158,0.77766467));
#145473=CARTESIAN_POINT('Ctrl Pts',(-7.4062708,1.327100493,1.182012199));
#145474=CARTESIAN_POINT('',(-7.26217116295609,1.32710049586375,1.27940238027789));
#145475=CARTESIAN_POINT('Ctrl Pts',(-7.118071532,1.327100493,1.376792527));
#145476=CARTESIAN_POINT('Ctrl Pts',(-7.043045404,1.392692987,1.764680561));
#145477=CARTESIAN_POINT('Ctrl Pts',(-6.926314018,1.45796923,2.142119073));
#145478=CARTESIAN_POINT('Ctrl Pts',(-7.31285186,1.327100493,1.664991795));
#145479=CARTESIAN_POINT('Ctrl Pts',(-7.222120769,1.392692987,2.063494074));
#145480=CARTESIAN_POINT('Ctrl Pts',(-7.088624029,1.45796923,2.449777414));
#145481=CARTESIAN_POINT('',(-7.312851860368,1.32710049307753,1.66499180013895));
#145482=CARTESIAN_POINT('',(-7.1666836756946,1.41778968871963,2.21102806086381));
#145483=CARTESIAN_POINT('Origin',(0.187653049799481,1.33928591086236,-0.0447254774391825));
#145484=CARTESIAN_POINT('Ctrl Pts',(-6.9277012673583,1.45719264075247,2.13762839408098));
#145485=CARTESIAN_POINT('Ctrl Pts',(-6.9674863419721,1.45030198768196,2.14980430826909));
#145486=CARTESIAN_POINT('Ctrl Pts',(-7.00731521566478,1.44357824623667,
2.16201682514904));
#145487=CARTESIAN_POINT('Ctrl Pts',(-7.08696274679494,1.43045449289663,
2.18648066253496));
#145488=CARTESIAN_POINT('Ctrl Pts',(-7.12682619505161,1.4240471066461,2.19874574376936));
#145489=CARTESIAN_POINT('Ctrl Pts',(-7.16668367588273,1.41778968833019,
2.21102806005493));
#145490=CARTESIAN_POINT('',(-7.21546169627581,1.32710049321647,1.52089215969151));
#145491=CARTESIAN_POINT('Origin',(8.56953397132543E-13,1.41887506700022,
-3.25585912397397E-13));
#145492=CARTESIAN_POINT('',(-7.16528730475997,1.23689319336947,2.21554910444165));
#145493=CARTESIAN_POINT('Origin',(0.184411325039866,1.48200508223814,-0.0166565348855671));
#145494=CARTESIAN_POINT('',(-6.97901861873992,1.32710049399577,2.74650671479504));
#145495=CARTESIAN_POINT('Origin',(0.178374116318473,1.33928284139354,-0.0723092163023792));
#145496=CARTESIAN_POINT('Origin',(0.185026189465232,1.48212080143722,-0.0462699162185873));
#145497=CARTESIAN_POINT('Ctrl Pts',(-6.929092656,1.457976823,2.133113913));
#145498=CARTESIAN_POINT('Ctrl Pts',(-6.812634675,1.39227158,2.511409761));
#145499=CARTESIAN_POINT('Ctrl Pts',(-6.65568528,1.327100493,2.874778854));
#145500=CARTESIAN_POINT('Ctrl Pts',(-7.236539753,1.457976823,1.970404122));
#145501=CARTESIAN_POINT('Ctrl Pts',(-7.128964961,1.39227158,2.365485134));
#145502=CARTESIAN_POINT('Ctrl Pts',(-6.979018621,1.327100493,2.746506705));
#145503=CARTESIAN_POINT('',(-6.81735194381297,1.32710049586377,2.81064279571972));
#145504=CARTESIAN_POINT('Ctrl Pts',(-6.65568528000001,1.327100493,2.874778854));
#145505=CARTESIAN_POINT('Ctrl Pts',(-6.499028759,1.392692987,3.237469881));
#145506=CARTESIAN_POINT('Ctrl Pts',(-6.303888365,1.45796923,3.580990293));
#145507=CARTESIAN_POINT('Ctrl Pts',(-6.783957428,1.327100493,3.198112195));
#145508=CARTESIAN_POINT('Ctrl Pts',(-6.609681369,1.392692987,3.567793211));
#145509=CARTESIAN_POINT('Ctrl Pts',(-6.396266209,1.45796923,3.916347607));
#145510=CARTESIAN_POINT('',(-6.78395742725216,1.32710049307754,3.19811220012484));
#145511=CARTESIAN_POINT('',(-6.52382491847514,1.41778968868913,3.6999605981568));
#145512=CARTESIAN_POINT('Origin',(0.173651152695408,1.33928595551319,-0.0840196691405803));
#145513=CARTESIAN_POINT('Ctrl Pts',(-6.30620854436299,1.45719264078498,
3.57690282142813));
#145514=CARTESIAN_POINT('Ctrl Pts',(-6.34244600492938,1.45030198761464,
3.59734668484766));
#145515=CARTESIAN_POINT('Ctrl Pts',(-6.37871837217705,1.44357824605803,
3.61783571074209));
#145516=CARTESIAN_POINT('Ctrl Pts',(-6.45124478528863,1.43045449290822,
3.65884946141489));
#145517=CARTESIAN_POINT('Ctrl Pts',(-6.487539618582,1.42404710661262,3.67939725500589));
#145518=CARTESIAN_POINT('Ctrl Pts',(-6.52382491865153,1.41778968830209,
3.69996059772776));
#145519=CARTESIAN_POINT('',(-6.71982135455065,1.32710049321647,3.03644552328139));
#145520=CARTESIAN_POINT('Origin',(-4.71844785465692E-13,1.41887506699989,
3.31765864780564E-13));
#145521=CARTESIAN_POINT('',(-6.52148930308131,1.23689319340118,3.70407576405903));
#145522=CARTESIAN_POINT('Origin',(0.176518965345178,1.48200502730424,-0.0559099623388354));
#145523=CARTESIAN_POINT('',(-6.22543528466758,1.32710049399579,4.18257761909792));
#145524=CARTESIAN_POINT('Origin',(0.158659732073103,1.33928284933523,-0.108963977220405));
#145525=CARTESIAN_POINT('Origin',(0.170753578389468,1.48212083418589,-0.0849632151973495));
#145526=CARTESIAN_POINT('Ctrl Pts',(-6.308537883,1.457976823,3.572792994));
#145527=CARTESIAN_POINT('Ctrl Pts',(-6.113480201,1.39227158,3.917209472));
#145528=CARTESIAN_POINT('Ctrl Pts',(-5.882086581,1.327100493,4.238343716));
#145529=CARTESIAN_POINT('Ctrl Pts',(-6.643774834,1.457976823,3.479979305));
#145530=CARTESIAN_POINT('Ctrl Pts',(-6.453784342,1.39227158,3.842698142));
#145531=CARTESIAN_POINT('Ctrl Pts',(-6.225435289,1.327100493,4.18257761));
#145532=CARTESIAN_POINT('',(-6.05376092498255,1.32710049586377,4.210460677403));
#145533=CARTESIAN_POINT('Ctrl Pts',(-5.882086581,1.327100493,4.238343716));
#145534=CARTESIAN_POINT('Ctrl Pts',(-5.651124753,1.392692987,4.558878708));
#145535=CARTESIAN_POINT('Ctrl Pts',(-5.38669989800001,1.45796923,4.852418387));
#145536=CARTESIAN_POINT('Ctrl Pts',(-5.937852687,1.327100493,4.58169242400001));
#145537=CARTESIAN_POINT('Ctrl Pts',(-5.688180615,1.392692987,4.905266302));
#145538=CARTESIAN_POINT('Ctrl Pts',(-5.404826091,1.45796923,5.199793739));
#145539=CARTESIAN_POINT('',(-5.93785268517258,1.32710049307753,4.5816924288298));
#145540=CARTESIAN_POINT('',(-5.5759193587845,1.41778968871294,5.01588708998643));
#145541=CARTESIAN_POINT('Origin',(0.15152941117498,1.33928597138522,-0.11938510053391));
#145542=CARTESIAN_POINT('Ctrl Pts',(-5.38984451854538,1.45719264075697,
4.84892524811201));
#145543=CARTESIAN_POINT('Ctrl Pts',(-5.42083994031133,1.45030198781947,
4.87668112715906));
#145544=CARTESIAN_POINT('Ctrl Pts',(-5.45185974380203,1.44357824651703,
4.90448861659059));
#145545=CARTESIAN_POINT('Ctrl Pts',(-5.51387378814892,1.430454492903,4.96013452544236));
#145546=CARTESIAN_POINT('Ctrl Pts',(-5.54490290006085,1.42404710665486,
4.98800423913264));
#145547=CARTESIAN_POINT('Ctrl Pts',(-5.57591935929175,1.41778968833113,
5.0158870893365));
#145548=CARTESIAN_POINT('',(-5.90996963479974,1.32710049321647,4.41001806892825));
#145549=CARTESIAN_POINT('Origin',(5.01768765426291E-13,1.41887506700006,
-5.17814957579077E-13));
#145550=CARTESIAN_POINT('',(-5.57275370974732,1.23689319394209,5.01940395734413));
#145551=CARTESIAN_POINT('Origin',(0.160373399338236,1.48200502642637,-0.092549463413848));
#145552=CARTESIAN_POINT('',(-5.18075751483762,1.32710049399576,5.42307584194051));
#145553=CARTESIAN_POINT('Origin',(0.131526047477788,1.33928284504139,-0.140523358241085));
#145554=CARTESIAN_POINT('Origin',(0.148496874513592,1.48212079504295,-0.119683813909308));
#145555=CARTESIAN_POINT('Ctrl Pts',(-5.39300289,1.457976823,4.845412245));
#145556=CARTESIAN_POINT('Ctrl Pts',(-5.128466186,1.39227158,5.139844821));
#145557=CARTESIAN_POINT('Ctrl Pts',(-4.833448051,1.327100493,5.40372833700001));
#145558=CARTESIAN_POINT('Ctrl Pts',(-5.74035438700001,1.457976823,4.826834523));
#145559=CARTESIAN_POINT('Ctrl Pts',(-5.476831939,1.39227158,5.140230856));
#145560=CARTESIAN_POINT('Ctrl Pts',(-5.180757521,1.327100493,5.42307583399999));
#145561=CARTESIAN_POINT('',(-5.00710277312064,1.32710049586375,5.41340209741272));
#145562=CARTESIAN_POINT('Ctrl Pts',(-4.83344805100001,1.327100493,5.403728337));
#145563=CARTESIAN_POINT('Ctrl Pts',(-4.538980434,1.392692987,5.667119433));
#145564=CARTESIAN_POINT('Ctrl Pts',(-4.217635331,1.45796923,5.89695279));
#145565=CARTESIAN_POINT('Ctrl Pts',(-4.814100554,1.327100493,5.751037807));
#145566=CARTESIAN_POINT('Ctrl Pts',(-4.500706857,1.392692987,6.01337459200001));
#145567=CARTESIAN_POINT('Ctrl Pts',(-4.160662311,1.45796923,6.240103295));
#145568=CARTESIAN_POINT('',(-4.81410055117882,1.32710049307753,5.75103781132099));
#145569=CARTESIAN_POINT('',(-4.36729000692376,1.4177896887255,6.09727627632803));
#145570=CARTESIAN_POINT('Origin',(0.122322587513753,1.33928593777335,-0.149168433170697));
#145571=CARTESIAN_POINT('Ctrl Pts',(-4.22145735396846,1.45719264066533,
5.8942173198239));
#145572=CARTESIAN_POINT('Ctrl Pts',(-4.24576142183573,1.45030198902915,
5.92798737492905));
#145573=CARTESIAN_POINT('Ctrl Pts',(-4.27007820568039,1.44357824918164,
5.9618130737019));
#145574=CARTESIAN_POINT('Ctrl Pts',(-4.31868018037653,1.43045449292316,
6.02948921218209));
#145575=CARTESIAN_POINT('Ctrl Pts',(-4.34299268436843,1.42404710665061,
6.06337768943683));
#145576=CARTESIAN_POINT('Ctrl Pts',(-4.36729000739379,1.41778968834208,
6.09727627592036));
#145577=CARTESIAN_POINT('',(-4.82377430351144,1.32710049321647,5.57738307112523));
#145578=CARTESIAN_POINT('Origin',(-1.12475133373646E-12,1.41887506699978,
1.52178616930065E-12));
#145579=CARTESIAN_POINT('',(-4.36344234637142,1.23689319339394,6.10003040005458));
#145580=CARTESIAN_POINT('Origin',(0.136728527353329,1.48200503359054,-0.124861215505688));
#145581=CARTESIAN_POINT('',(-3.89383328225337,1.32710049399577,6.40999706643645));
#145582=CARTESIAN_POINT('Origin',(0.098242796547533,1.33928284083096,-0.165512376615569));
#145583=CARTESIAN_POINT('Origin',(0.119296622147308,1.48212081958442,-0.148808097778507));
#145584=CARTESIAN_POINT('Ctrl Pts',(-4.225297077,1.457976823,5.891465405));
#145585=CARTESIAN_POINT('Ctrl Pts',(-3.903650793,1.39227158,6.122146739));
#145586=CARTESIAN_POINT('Ctrl Pts',(-3.558802862,1.327100493,6.31644062700001));
#145587=CARTESIAN_POINT('Ctrl Pts',(-4.568521349,1.457976823,5.947992324));
#145588=CARTESIAN_POINT('Ctrl Pts',(-4.243788962,1.39227158,6.197412088));
#145589=CARTESIAN_POINT('Ctrl Pts',(-3.89383329,1.327100493,6.40999706));
#145590=CARTESIAN_POINT('',(-3.72631806086074,1.32710049586377,6.36321885236559));
#145591=CARTESIAN_POINT('Ctrl Pts',(-3.558802862,1.327100493,6.316440627));
#145592=CARTESIAN_POINT('Ctrl Pts',(-3.214598434,1.392692987,6.510371952));
#145593=CARTESIAN_POINT('Ctrl Pts',(-2.851358824,1.45796923,6.665752235));
#145594=CARTESIAN_POINT('Ctrl Pts',(-3.465246429,1.327100493,6.651471054));
#145595=CARTESIAN_POINT('Ctrl Pts',(-3.102785048,1.392692987,6.84030417));
#145596=CARTESIAN_POINT('Ctrl Pts',(-2.721950586,1.45796923,6.988632556));
#145597=CARTESIAN_POINT('',(-3.46524642530106,1.32710049307754,6.65147105762962));
#145598=CARTESIAN_POINT('',(-2.95445102820031,1.41778968870866,6.8935636005648));
#145599=CARTESIAN_POINT('Origin',(0.0873959663614748,1.33928595894931,-0.171976734249653));
#145600=CARTESIAN_POINT('Ctrl Pts',(-2.85567953540615,1.45719264073027,
6.66390233981683));
#145601=CARTESIAN_POINT('Ctrl Pts',(-2.87215582771297,1.45030198748113,
6.70210753480414));
#145602=CARTESIAN_POINT('Ctrl Pts',(-2.88863257782738,1.44357824583997,
6.7403698081076));
#145603=CARTESIAN_POINT('Ctrl Pts',(-2.92154988752125,1.43045449288956,
6.81691168460353));
#145604=CARTESIAN_POINT('Ctrl Pts',(-2.93800895772761,1.42404710660756,
6.85523433781912));
#145605=CARTESIAN_POINT('Ctrl Pts',(-2.95445102865523,1.41778968831593,
6.89356360030554));
#145606=CARTESIAN_POINT('',(-3.51202464667584,1.32710049321647,6.48395583986311));
#145607=CARTESIAN_POINT('Origin',(1.34441069388203E-13,1.41887506699994,
-3.36970035208495E-13));
#145608=CARTESIAN_POINT('',(-2.95010126896827,1.23689319338589,6.89542620135343));
#145609=CARTESIAN_POINT('Origin',(0.106690364867912,1.48200498463762,-0.151334503244875));
#145610=CARTESIAN_POINT('',(-2.42483773306109,1.32710049399578,7.09719395161996));
#145611=CARTESIAN_POINT('Origin',(0.0603656246863346,1.33928285255758,-0.182762001417611));
#145612=CARTESIAN_POINT('Origin',(0.0845181387472432,1.48212075608598,-0.170974189347677));
#145613=CARTESIAN_POINT('Ctrl Pts',(-2.860021067,1.457976823,6.66204019));
#145614=CARTESIAN_POINT('Ctrl Pts',(-2.496305027,1.39227158,6.81818388));
#145615=CARTESIAN_POINT('Ctrl Pts',(-2.117752007,1.327100493,6.933803173));
#145616=CARTESIAN_POINT('Ctrl Pts',(-3.183069331,1.457976823,6.791028614));
#145617=CARTESIAN_POINT('Ctrl Pts',(-2.812311129,1.39227158,6.964809219));
#145618=CARTESIAN_POINT('Ctrl Pts',(-2.424837742,1.327100493,7.09719394700001));
#145619=CARTESIAN_POINT('',(-2.27129485780885,1.32710049586377,7.01549856540383));
#145620=CARTESIAN_POINT('Ctrl Pts',(-2.117752007,1.327100493,6.933803173));
#145621=CARTESIAN_POINT('Ctrl Pts',(-1.739905385,1.392692987,7.049206714));
#145622=CARTESIAN_POINT('Ctrl Pts',(-1.351755947,1.45796923,7.122868513));
#145623=CARTESIAN_POINT('Ctrl Pts',(-1.954361232,1.327100493,7.240888908));
#145624=CARTESIAN_POINT('Ctrl Pts',(-1.55978046,1.392692987,7.347388728));
#145625=CARTESIAN_POINT('Ctrl Pts',(-1.155963477,1.45796923,7.410381126));
#145626=CARTESIAN_POINT('',(-1.95436122763021,1.32710049307753,7.24088891073354));
#145627=CARTESIAN_POINT('',(-1.40346520327497,1.41778968873029,7.36751555254718));
#145628=CARTESIAN_POINT('Origin',(0.0483827133056874,1.33928592280152,-0.18674325857323));
#145629=CARTESIAN_POINT('Ctrl Pts',(-1.35637331540349,1.4571926407211,7.12199069258409));
#145630=CARTESIAN_POINT('Ctrl Pts',(-1.3642514132043,1.45030198781702,7.16284458524739));
#145631=CARTESIAN_POINT('Ctrl Pts',(-1.3721176878921,1.4435782465617,7.20375431971896));
#145632=CARTESIAN_POINT('Ctrl Pts',(-1.38781116924433,1.43045449289558,
7.28558294295861));
#145633=CARTESIAN_POINT('Ctrl Pts',(-1.39564719791282,1.42404710664426,
7.32654784733475));
#145634=CARTESIAN_POINT('Ctrl Pts',(-1.40346520396996,1.41778968834456,
7.36751555235564));
#145635=CARTESIAN_POINT('',(-2.03605662078526,1.32710049321647,7.08734604013077));
#145636=CARTESIAN_POINT('Origin',(-3.24176449573166E-13,1.41887506699978,
1.41249859031412E-12));
#145637=CARTESIAN_POINT('',(-1.39881673462794,1.23689319337654,7.36839953684967));
#145638=CARTESIAN_POINT('Origin',(0.0716636014155367,1.48200507732621,-0.170731826487561));
#145639=CARTESIAN_POINT('',(-0.842459466245457,1.32710049399578,7.45253393658554));
#145640=CARTESIAN_POINT('Origin',(0.0196658882621228,1.33928282222093,-0.19146587916326));
#145641=CARTESIAN_POINT('Origin',(0.0457878018278116,1.48212077089942,-0.185146050959324));
#145642=CARTESIAN_POINT('Ctrl Pts',(-1.361013652,1.457976823,7.12110538));
#145643=CARTESIAN_POINT('Ctrl Pts',(-0.972234813,1.39227158,7.19541032));
#145644=CARTESIAN_POINT('Ctrl Pts',(-0.577677421,1.327100493,7.226948789));
#145645=CARTESIAN_POINT('Ctrl Pts',(-1.648780528,1.457976823,7.316523954));
#145646=CARTESIAN_POINT('Ctrl Pts',(-1.249332754,1.39227158,7.406539611));
#145647=CARTESIAN_POINT('Ctrl Pts',(-0.842459476,1.327100493,7.452533934));
#145648=CARTESIAN_POINT('',(-0.710068431037556,1.32710049586375,7.33974136318937));
#145649=CARTESIAN_POINT('Origin',(-3.47486796281604E-14,1.41887506699989,
1.1666015375944E-13));
#145650=CARTESIAN_POINT('',(0.217874905393073,1.23689319448374,7.49683470012955));
#145651=CARTESIAN_POINT('',(-0.352092272117407,1.32710049307754,7.49173084474164));
#145652=CARTESIAN_POINT('Origin',(0.0332858491289362,1.48200502004435,-0.182145603701761));
#145653=CARTESIAN_POINT('Origin',(-0.0219534349632636,1.33928287002982,
-0.191217377589924));
#145654=CARTESIAN_POINT('Origin',(0.00710727857594066,1.33928593431685,
-0.192778422559777));
#145655=CARTESIAN_POINT('Ctrl Pts',(-0.577677421000001,1.327100493,7.226948789));
#145656=CARTESIAN_POINT('Ctrl Pts',(-0.183856294,1.392692987,7.258428405));
#145657=CARTESIAN_POINT('Ctrl Pts',(0.211053536,1.45796923,7.246927377));
#145658=CARTESIAN_POINT('Ctrl Pts',(-0.352092277,1.327100493,7.49173084300001));
#145659=CARTESIAN_POINT('Ctrl Pts',(0.0561577300000001,1.392692987,7.510917554));
#145660=CARTESIAN_POINT('Ctrl Pts',(0.4640752,1.45796923,7.485628511));
#145661=CARTESIAN_POINT('',(-0.464884850334583,1.32710049321647,7.3593398159157));
#145662=CARTESIAN_POINT('Ctrl Pts',(-1.16045022,4.559946053,7.409679837));
#145663=CARTESIAN_POINT('Ctrl Pts',(-0.75366617,4.494288122,7.473387399));
#145664=CARTESIAN_POINT('Ctrl Pts',(-0.342352821,4.429844992,7.49218222900001));
#145665=CARTESIAN_POINT('Ctrl Pts',(-1.356068566,4.559946053,7.122048725));
#145666=CARTESIAN_POINT('Ctrl Pts',(-0.965075178000001,4.494288122,7.19649554));
#145667=CARTESIAN_POINT('Ctrl Pts',(-0.568281989,4.429844992,7.227693656));
#145668=CARTESIAN_POINT('',(-0.594913062081674,4.46959751864088,7.4763679983408));
#145669=CARTESIAN_POINT('Ctrl Pts',(-0.59491306336725,4.46959751863648,
7.47636799821831));
#145670=CARTESIAN_POINT('Ctrl Pts',(-0.591300604527993,4.46339351469901,
7.43481934129684));
#145671=CARTESIAN_POINT('Ctrl Pts',(-0.587666952126791,4.45704680092971,
7.39327085177197));
#145672=CARTESIAN_POINT('Ctrl Pts',(-0.580360792552427,4.44406034774631,
7.31026810206512));
#145673=CARTESIAN_POINT('Ctrl Pts',(-0.576684369626278,4.43741364858974,
7.26876929900358));
#145674=CARTESIAN_POINT('Ctrl Pts',(-0.572986203044206,4.43060907880598,
7.22732224375387));
#145675=CARTESIAN_POINT('',(-1.16045021425437,4.55994605309726,7.40967983744685));
#145676=CARTESIAN_POINT('Origin',(0.0501922216378608,4.6963258830081,-0.179678134303866));
#145677=CARTESIAN_POINT('',(-1.25825939098333,4.5599460533341,7.26586428134924));
#145678=CARTESIAN_POINT('Ctrl Pts',(-2.42543142521891,4.429837254,7.097537917381));
#145679=CARTESIAN_POINT('Ctrl Pts',(-2.04083356846316,4.494719353,7.22896598944729));
#145680=CARTESIAN_POINT('Ctrl Pts',(-1.64428585990226,4.559946053,7.31806573418139));
#145681=CARTESIAN_POINT('Ctrl Pts',(-1.63065611435896,4.56218796060514,
7.32112818246309));
#145682=CARTESIAN_POINT('Ctrl Pts',(-1.61702636881566,4.56442986821038,
7.32419063074491));
#145683=CARTESIAN_POINT('Ctrl Pts',(-2.117720602,4.429837254,6.933812764));
#145684=CARTESIAN_POINT('Ctrl Pts',(-1.741994603,4.494719353,7.048566756));
#145685=CARTESIAN_POINT('Ctrl Pts',(-1.356068566,4.559946053,7.122048725));
#145686=CARTESIAN_POINT('Ctrl Pts',(-1.34280389804382,4.56218796060514,
7.12457437454447));
#145687=CARTESIAN_POINT('Ctrl Pts',(-1.32953923008762,4.56442986821038,
7.12710002408904));
#145688=CARTESIAN_POINT('',(-1.64369966917306,4.55994605198798,7.3176670746967));
#145689=CARTESIAN_POINT('',(-1.49988410426399,4.55994605006201,7.21985790168456));
#145690=CARTESIAN_POINT('',(-2.18820244725389,4.46959751862817,7.17368594600435));
#145691=CARTESIAN_POINT('Origin',(0.0432519951682417,4.55357071574317,-0.187915365400194));
#145692=CARTESIAN_POINT('Ctrl Pts',(-2.11325074753863,4.43060907881227,
6.93517636918274));
#145693=CARTESIAN_POINT('Ctrl Pts',(-2.12577234002776,4.43741364592441,
6.97485940339133));
#145694=CARTESIAN_POINT('Ctrl Pts',(-2.13828382085451,4.44406034235223,
7.01459764794111));
#145695=CARTESIAN_POINT('Ctrl Pts',(-2.16326220951458,4.4570467462429,7.0940889297557));
#145696=CARTESIAN_POINT('Ctrl Pts',(-2.17574248873862,4.4633934037901,7.13388453421944));
#145697=CARTESIAN_POINT('Ctrl Pts',(-2.18820244614369,4.46959751862594,
7.17368594635225));
#145698=CARTESIAN_POINT('Ctrl Pts',(-2.726181675,4.559946053,6.986983146));
#145699=CARTESIAN_POINT('Ctrl Pts',(-2.342603253,4.494288122,7.136647807));
#145700=CARTESIAN_POINT('Ctrl Pts',(-1.944946514,4.429844992,7.243423435));
#145701=CARTESIAN_POINT('Ctrl Pts',(-2.855394386,4.559946053,6.664024527));
#145702=CARTESIAN_POINT('Ctrl Pts',(-2.489546071,4.494288122,6.82078283800001));
#145703=CARTESIAN_POINT('Ctrl Pts',(-2.108736358,4.429844992,6.936550365));
#145704=CARTESIAN_POINT('',(-2.72618166947526,4.55994605320497,6.98698314764743));
#145705=CARTESIAN_POINT('Origin',(0.087644175324966,4.69632600826713,-0.164687271233922));
#145706=CARTESIAN_POINT('',(-2.79078802860555,4.5599460533341,6.8255038372746));
#145707=CARTESIAN_POINT('Origin',(-4.74880551548651E-13,4.65175593299822,
1.38040620600854E-12));
#145708=CARTESIAN_POINT('',(-2.19171665066047,4.65066950022866,7.17261306109147));
#145709=CARTESIAN_POINT('Origin',(0.0629454791939865,4.69641603009044,-0.180826038642827));
#145710=CARTESIAN_POINT('Origin',(0.0709662625895141,4.55357344854477,-0.17904150220209));
#145711=CARTESIAN_POINT('Ctrl Pts',(-3.89448703711139,4.429837254,6.41020536374285));
#145712=CARTESIAN_POINT('Ctrl Pts',(-3.54713401530404,4.494719353,6.62123789183932));
#145713=CARTESIAN_POINT('Ctrl Pts',(-3.17901118206042,4.559946053,6.79350056986478));
#145714=CARTESIAN_POINT('Ctrl Pts',(-3.16635842794052,4.56218796065315,
6.79942141234521));
#145715=CARTESIAN_POINT('Ctrl Pts',(-3.15370567382063,4.56442986830639,
6.80534225482578));
#145716=CARTESIAN_POINT('Ctrl Pts',(-3.558774254,4.429837254,6.316456745));
#145717=CARTESIAN_POINT('Ctrl Pts',(-3.216501235,4.494719353,6.509297835));
#145718=CARTESIAN_POINT('Ctrl Pts',(-2.855394386,4.559946053,6.664024527));
#145719=CARTESIAN_POINT('Ctrl Pts',(-2.84298277835493,4.56218796065315,
6.66934263990384));
#145720=CARTESIAN_POINT('Ctrl Pts',(-2.83057117070987,4.56442986830639,
6.67466075280755));
#145721=CARTESIAN_POINT('',(-3.17835299299463,4.5599460519893,6.79323724515001));
#145722=CARTESIAN_POINT('',(-3.01687367847068,4.559946050062,6.72863089041115));
#145723=CARTESIAN_POINT('',(-3.67917391567943,4.46959751860266,6.53557031160943));
#145724=CARTESIAN_POINT('Origin',(0.0826369678524574,4.55357068133953,-0.174223947254913));
#145725=CARTESIAN_POINT('Ctrl Pts',(-3.55470203692773,4.43060907877665,
6.31874935623179));
#145726=CARTESIAN_POINT('Ctrl Pts',(-3.57546156005755,4.43741364568478,
6.3548128496631));
#145727=CARTESIAN_POINT('Ctrl Pts',(-3.59622307647419,4.44406034190139,
6.39093243628689));
#145728=CARTESIAN_POINT('Ctrl Pts',(-3.63770575509226,4.45704674429609,
6.46319563253993));
#145729=CARTESIAN_POINT('Ctrl Pts',(-3.65844912392703,4.46339339986109,
6.49937793472558));
#145730=CARTESIAN_POINT('Ctrl Pts',(-3.67917391449682,4.46959751860046,
6.535570312287));
#145731=CARTESIAN_POINT('Ctrl Pts',(-4.164439905,4.559946053,6.237582888));
#145732=CARTESIAN_POINT('Ctrl Pts',(-3.822002811,4.494288122,6.466206494));
#145733=CARTESIAN_POINT('Ctrl Pts',(-3.45659667,4.429844992,6.655970212));
#145734=CARTESIAN_POINT('Ctrl Pts',(-4.221205138,4.559946053,5.894397949));
#145735=CARTESIAN_POINT('Ctrl Pts',(-3.897608556,4.494288122,6.12613791));
#145736=CARTESIAN_POINT('Ctrl Pts',(-3.55058856,4.429844992,6.321061689));
#145737=CARTESIAN_POINT('',(-4.16443989995725,4.55994605320497,6.23758289079854));
#145738=CARTESIAN_POINT('Origin',(0.120998139083789,4.69632601466772,-0.141996301290852));
#145739=CARTESIAN_POINT('',(-4.19282251981636,4.5599460533341,6.06599041966374));
#145740=CARTESIAN_POINT('Origin',(-8.21825246744012E-13,4.65175593300022,
1.48665801891212E-12));
#145741=CARTESIAN_POINT('',(-3.68237532060303,4.65066950023331,6.53376706031242));
#145742=CARTESIAN_POINT('Origin',(0.100346144501832,4.69641608322633,-0.16306706225985));
#145743=CARTESIAN_POINT('Origin',(0.107795750829115,4.55357342128508,-0.159599980214508));
#145744=CARTESIAN_POINT('Ctrl Pts',(-5.18144076307036,4.429837254,5.42313873171298));
#145745=CARTESIAN_POINT('Ctrl Pts',(-4.88757441730978,4.494719353,5.70390806884768));
#145746=CARTESIAN_POINT('Ctrl Pts',(-4.56508947560136,4.559946053,5.95127886750963));
#145747=CARTESIAN_POINT('Ctrl Pts',(-4.55400534158494,4.56218796073192,
5.9597812523639));
#145748=CARTESIAN_POINT('Ctrl Pts',(-4.54292120756855,4.56442986846394,
5.96828363721818));
#145749=CARTESIAN_POINT('Ctrl Pts',(-4.833423576,4.429837254,5.403750228));
#145750=CARTESIAN_POINT('Ctrl Pts',(-4.540607845,4.494719353,5.665661383));
#145751=CARTESIAN_POINT('Ctrl Pts',(-4.221205138,4.559946053,5.894397949));
#145752=CARTESIAN_POINT('Ctrl Pts',(-4.21022694351181,4.56218796073192,
5.90225985640743));
#145753=CARTESIAN_POINT('Ctrl Pts',(-4.19924874902359,4.56442986846394,
5.91012176381473));
#145754=CARTESIAN_POINT('',(-4.56439006760927,4.55994605198929,5.95116319036086));
#145755=CARTESIAN_POINT('',(-4.39279759295034,4.55994605006201,5.92278057629117));
#145756=CARTESIAN_POINT('',(-4.99811130094148,4.46959751858828,5.59185867318702));
#145757=CARTESIAN_POINT('Origin',(0.118157854640977,4.55357071768602,-0.152386075058663));
#145758=CARTESIAN_POINT('Ctrl Pts',(-4.8299394093612,4.43060907886738,5.40686464598623));
#145759=CARTESIAN_POINT('Ctrl Pts',(-4.85796618330899,4.43741364862199,
5.43762232418592));
#145760=CARTESIAN_POINT('Ctrl Pts',(-4.88600696371074,4.44406034775626,
5.46843435724498));
#145761=CARTESIAN_POINT('Ctrl Pts',(-4.94205422368869,4.45704674368818,
5.53009049988148));
#145762=CARTESIAN_POINT('Ctrl Pts',(-4.97009074661369,4.46339339863389,
5.56096766560843));
#145763=CARTESIAN_POINT('Ctrl Pts',(-4.99811129988664,4.46959751858598,
5.5918586741443));
#145764=CARTESIAN_POINT('Ctrl Pts',(-5.407973553,4.559946053,5.196520186));
#145765=CARTESIAN_POINT('Ctrl Pts',(-5.122689766,4.494288122,5.493412553));
#145766=CARTESIAN_POINT('Ctrl Pts',(-4.806620207,4.429844992,5.75729121900001));
#145767=CARTESIAN_POINT('Ctrl Pts',(-5.38963702999999,4.559946053,4.849155874));
#145768=CARTESIAN_POINT('Ctrl Pts',(-5.123423198,4.494288122,5.145041583));
#145769=CARTESIAN_POINT('Ctrl Pts',(-4.826419186,4.429844992,5.410007194));
#145770=CARTESIAN_POINT('',(-5.40797354865546,4.55994605320499,5.19652018986508));
#145771=CARTESIAN_POINT('Origin',(0.148694027502743,4.6963259891713,-0.112665215829012));
#145772=CARTESIAN_POINT('',(-5.39880529010589,4.5599460533341,5.02283803149846));
#145773=CARTESIAN_POINT('Origin',(-1.28803218091278E-12,4.651755933,1.4510961876546E-12));
#145774=CARTESIAN_POINT('',(-5.00085021307748,4.65066950024506,5.58940937371014));
#145775=CARTESIAN_POINT('Origin',(0.133054720112198,4.69641603606148,-0.137683229129221));
#145776=CARTESIAN_POINT('Origin',(0.139584834903529,4.55357340357966,-0.132695705850141));
#145777=CARTESIAN_POINT('Ctrl Pts',(-6.22611607791649,4.429837254,4.1824921598369));
#145778=CARTESIAN_POINT('Ctrl Pts',(-5.99947727212079,4.494719353,4.51986984361682));
#145779=CARTESIAN_POINT('Ctrl Pts',(-5.73770925906248,4.559946053,4.83078198081904));
#145780=CARTESIAN_POINT('Ctrl Pts',(-5.72871202741551,4.56218796072055,
4.84146834577086));
#145781=CARTESIAN_POINT('Ctrl Pts',(-5.71971479576868,4.56442986844111,
4.85215471072267));
#145782=CARTESIAN_POINT('Ctrl Pts',(-5.882067385,4.429837254,4.238370357));
#145783=CARTESIAN_POINT('Ctrl Pts',(-5.65240067800001,4.494719353,4.557104901));
#145784=CARTESIAN_POINT('Ctrl Pts',(-5.38963703,4.559946053,4.849155874));
#145785=CARTESIAN_POINT('Ctrl Pts',(-5.38060557737204,4.56218796072055,
4.85919396164141));
#145786=CARTESIAN_POINT('Ctrl Pts',(-5.37157412474406,4.56442986844111,
4.86923204928272));
#145787=CARTESIAN_POINT('',(-5.73700133724454,4.55994605198842,4.83081935903903));
#145788=CARTESIAN_POINT('',(-5.56331917461028,4.55994605006201,4.83998762566662));
#145789=CARTESIAN_POINT('',(-6.08334255721317,4.46959751861104,4.38667793822612));
#145790=CARTESIAN_POINT('Origin',(0.148154028825501,4.55357072817546,-0.123423031031687));
#145791=CARTESIAN_POINT('Ctrl Pts',(-5.87933418335156,4.43060907880993,
4.2421609543172));
#145792=CARTESIAN_POINT('Ctrl Pts',(-5.9133176837977,4.43741364562489,4.2661745966159));
#145793=CARTESIAN_POINT('Ctrl Pts',(-5.94732654614253,4.44406034175098,
4.29023831074314));
#145794=CARTESIAN_POINT('Ctrl Pts',(-6.01531773827986,4.45704674491822,
4.3384044895316));
#145795=CARTESIAN_POINT('Ctrl Pts',(-6.04933646796366,4.46339340112161,
4.3625327456653));
#145796=CARTESIAN_POINT('Ctrl Pts',(-6.08334255646149,4.46959751860884,
4.38667793928535));
#145797=CARTESIAN_POINT('Ctrl Pts',(-6.398636369,4.559946053,3.912473977));
#145798=CARTESIAN_POINT('Ctrl Pts',(-6.183845441,4.494288122,4.263752746));
#145799=CARTESIAN_POINT('Ctrl Pts',(-5.93189152599999,4.429844992,4.589407688));
#145800=CARTESIAN_POINT('Ctrl Pts',(-6.306055484,4.559946053,3.577172659));
#145801=CARTESIAN_POINT('Ctrl Pts',(-6.109672265,4.494288122,3.92336883));
#145802=CARTESIAN_POINT('Ctrl Pts',(-5.876571816,4.429844992,4.245986775));
#145803=CARTESIAN_POINT('',(-6.39863636559543,4.55994605320497,3.91247398167052));
#145804=CARTESIAN_POINT('Origin',(0.16943747854313,4.69632601282118,-0.0780664411189724));
#145805=CARTESIAN_POINT('',(-6.35234592546061,4.5599460533341,3.74482331976313));
#145806=CARTESIAN_POINT('Origin',(-1.21864324187371E-13,4.65175593299933,
1.00613961606655E-13));
#145807=CARTESIAN_POINT('',(-6.08549090775826,4.65066949967397,4.38369711683319));
#145808=CARTESIAN_POINT('Origin',(0.159541818170423,4.69641603271111,-0.105861446073009));
#145809=CARTESIAN_POINT('Origin',(0.164847346774489,4.55357340755019,-0.0995869337445715));
#145810=CARTESIAN_POINT('Ctrl Pts',(-6.97966512498879,4.429837254,2.74627690292657));
#145811=CARTESIAN_POINT('Ctrl Pts',(-6.83085123720195,4.494719353,3.12448752840191));
#145812=CARTESIAN_POINT('Ctrl Pts',(-6.64204013411244,4.559946053,3.48440309746244));
#145813=CARTESIAN_POINT('Ctrl Pts',(-6.63555050530195,4.56218796073003,
3.49677376003527));
#145814=CARTESIAN_POINT('Ctrl Pts',(-6.62906087649148,4.56442986846015,
3.50914442260804));
#145815=CARTESIAN_POINT('Ctrl Pts',(-6.655672259,4.429837254,2.874808998));
#145816=CARTESIAN_POINT('Ctrl Pts',(-6.49989353800001,4.494719353,3.235463259));
#145817=CARTESIAN_POINT('Ctrl Pts',(-6.30605548400001,4.559946053,3.577172659));
#145818=CARTESIAN_POINT('Ctrl Pts',(-6.29939307379623,4.56218796073003,
3.58891755710594));
#145819=CARTESIAN_POINT('Ctrl Pts',(-6.29273066359246,4.56442986846015,
3.60066245521194));
#145820=CARTESIAN_POINT('',(-6.64135679832003,4.55994605198842,3.48459178406735));
#145821=CARTESIAN_POINT('',(-6.47370613432616,4.559946050062,3.53088223240309));
#145822=CARTESIAN_POINT('',(-6.88412347607716,4.46959751862992,2.97638101838741));
#145823=CARTESIAN_POINT('Origin',(0.171222655052026,4.55357076022744,-0.0886887757941202));
#145824=CARTESIAN_POINT('Ctrl Pts',(-6.65381782566217,4.43060907892645,
2.87909853088944));
#145825=CARTESIAN_POINT('Ctrl Pts',(-6.69216903292966,4.43741364556175,
2.89524529925262));
#145826=CARTESIAN_POINT('Ctrl Pts',(-6.7305557728328,4.44406034147083,2.91143551654796));
#145827=CARTESIAN_POINT('Ctrl Pts',(-6.80731167828225,4.45704674547839,
2.94385950258702));
#145828=CARTESIAN_POINT('Ctrl Pts',(-6.84572193411808,4.46339340219066,
2.96011063365308));
#145829=CARTESIAN_POINT('Ctrl Pts',(-6.8841234755912,4.46959751862791,2.97638101953514));
#145830=CARTESIAN_POINT('Ctrl Pts',(-7.090106059,4.559946053,2.445484832));
#145831=CARTESIAN_POINT('Ctrl Pts',(-6.955851376,4.494288122,2.8347246));
#145832=CARTESIAN_POINT('Ctrl Pts',(-6.779794189,4.429844992,3.206928554));
#145833=CARTESIAN_POINT('Ctrl Pts',(-6.927609792,4.559946053,2.137924827));
#145834=CARTESIAN_POINT('Ctrl Pts',(-6.81023984700001,4.494288122,2.518243711));
#145835=CARTESIAN_POINT('Ctrl Pts',(-6.65194247900001,4.429844992,2.883428734));
#145836=CARTESIAN_POINT('',(-7.09010605667977,4.55994605320498,2.44548483733953));
#145837=CARTESIAN_POINT('Origin',(0.182257792442442,4.69632597364402,-0.0398171190939184));
#145838=CARTESIAN_POINT('',(-7.00885792486393,4.5599460533341,2.29170483144534));
#145839=CARTESIAN_POINT('Origin',(-1.40946282423116E-13,4.65175593299845,
2.21177243187043E-14));
#145840=CARTESIAN_POINT('',(-6.8855808109066,4.65066950021868,2.97300805498941));
#145841=CARTESIAN_POINT('Origin',(0.178568934787088,4.69641602588422,-0.0690897061486873));
#145842=CARTESIAN_POINT('Origin',(0.182401267354205,4.55357341209628,-0.0618212237820231));
#145843=CARTESIAN_POINT('Ctrl Pts',(-7.40685278759499,4.429837254,1.18164879132162));
#145844=CARTESIAN_POINT('Ctrl Pts',(-7.34282219046977,4.494719353,1.58300764889506));
#145845=CARTESIAN_POINT('Ctrl Pts',(-7.23579659428889,4.559946053,1.97509739842135));
#145846=CARTESIAN_POINT('Ctrl Pts',(-7.23211801628928,4.56218796065734,
1.98857391972049));
#145847=CARTESIAN_POINT('Ctrl Pts',(-7.22843943828966,4.56442986831468,
2.00205044101955));
#145848=CARTESIAN_POINT('Ctrl Pts',(-7.118065296,4.429837254,1.376824766));
#145849=CARTESIAN_POINT('Ctrl Pts',(-7.0434586,4.494719353,1.762534951));
#145850=CARTESIAN_POINT('Ctrl Pts',(-6.927609792,4.559946053,2.137924827));
#145851=CARTESIAN_POINT('Ctrl Pts',(-6.92362795128529,4.56218796065734,
2.15082735675371));
#145852=CARTESIAN_POINT('Ctrl Pts',(-6.91964611057047,4.56442986831468,
2.16372988650748));
#145853=CARTESIAN_POINT('',(-7.23516979657245,4.55994605198842,1.97542857061927));
#145854=CARTESIAN_POINT('',(-7.08138978994764,4.559946050062,2.0566767108959));
#145855=CARTESIAN_POINT('',(-7.36301043261897,4.46959751860092,1.42691183008964));
#145856=CARTESIAN_POINT('Origin',(0.186285024016406,4.55357072321,-0.0498074645394533));
#145857=CARTESIAN_POINT('Ctrl Pts',(-7.11717634030228,4.43060907880928,
1.38141266024738));
#145858=CARTESIAN_POINT('Ctrl Pts',(-7.15810199827393,4.43741364586804,
1.38893755061707));
#145859=CARTESIAN_POINT('Ctrl Pts',(-7.19907169877002,4.44406034223659,
1.39649723577526));
#145860=CARTESIAN_POINT('Ctrl Pts',(-7.28100328301253,4.45704674475147,
1.41166291447601));
#145861=CARTESIAN_POINT('Ctrl Pts',(-7.32200903658237,4.46339340079517,
1.41927703266189));
#145862=CARTESIAN_POINT('Ctrl Pts',(-7.36301043237867,4.46959751859857,
1.42691183138207));
#145863=CARTESIAN_POINT('Ctrl Pts',(-7.450050271,4.559946053,0.864147535));
#145864=CARTESIAN_POINT('Ctrl Pts',(-7.402609431,4.494288122,1.273147882));
#145865=CARTESIAN_POINT('Ctrl Pts',(-7.310681212,4.429844992,1.674497005));
#145866=CARTESIAN_POINT('Ctrl Pts',(-7.225236766,4.559946053,0.598710006));
#145867=CARTESIAN_POINT('Ctrl Pts',(-7.192368183,4.494288122,0.995368314));
#145868=CARTESIAN_POINT('Ctrl Pts',(-7.116275704,4.429844992,1.386044769));
#145869=CARTESIAN_POINT('',(-7.45005026987186,4.55994605320497,0.86414754067111));
#145870=CARTESIAN_POINT('Origin',(0.186556548936415,4.69632596822184,0.000293759629906298));
#145871=CARTESIAN_POINT('',(-7.33764351829699,4.5599460533341,0.731428772536595));
#145872=CARTESIAN_POINT('Origin',(6.76542155630955E-13,4.65175593299956,
-1.68105546843877E-13));
#145873=CARTESIAN_POINT('',(-7.36370860840548,4.65066949966057,1.42330444080266));
#145874=CARTESIAN_POINT('Origin',(0.189246192904705,4.69641605414231,-0.0290873467067651));
#145875=CARTESIAN_POINT('Origin',(0.191426669989561,4.55357342761404,-0.0211650195628771));
#145876=CARTESIAN_POINT('Ctrl Pts',(-7.48770424678088,4.429837254,-0.438231905223869));
#145877=CARTESIAN_POINT('Ctrl Pts',(-7.51145093953738,4.494719353,-0.0324919097257988));
#145878=CARTESIAN_POINT('Ctrl Pts',(-7.49121524818656,4.559946053,0.373438339122528));
#145879=CARTESIAN_POINT('Ctrl Pts',(-7.4905197270101,4.56218796064393,0.387390572299871));
#145880=CARTESIAN_POINT('Ctrl Pts',(-7.48982420583371,4.56442986828785,
0.401342805477214));
#145881=CARTESIAN_POINT('Ctrl Pts',(-7.24762551100001,4.429837254,-0.185538262));
#145882=CARTESIAN_POINT('Ctrl Pts',(-7.257679367,4.494719353,0.207192467));
#145883=CARTESIAN_POINT('Ctrl Pts',(-7.225236766,4.559946053,0.598710006));
#145884=CARTESIAN_POINT('Ctrl Pts',(-7.22412168099383,4.56218796064393,
0.612166859764027));
#145885=CARTESIAN_POINT('Ctrl Pts',(-7.2230065959878,4.56442986828785,0.625623713528053));
#145886=CARTESIAN_POINT('',(-7.49067429688774,4.55994605198842,0.373896511680142));
#145887=CARTESIAN_POINT('',(-7.35795552980536,4.559946050062,0.486303271575305));
#145888=CARTESIAN_POINT('',(-7.49761120473734,4.4695975186588,-0.189278169159026));
#145889=CARTESIAN_POINT('Origin',(0.19263692254358,4.5535706981198,-0.00859721874756657));
#145890=CARTESIAN_POINT('Ctrl Pts',(-7.24774360047122,4.43060907884376,
-0.18086653100126));
#145891=CARTESIAN_POINT('Ctrl Pts',(-7.28933008475596,4.4374136486107,-0.18231537550547));
#145892=CARTESIAN_POINT('Ctrl Pts',(-7.33096706380868,4.44406034775353,
-0.183739706672199));
#145893=CARTESIAN_POINT('Ctrl Pts',(-7.41424328253091,4.45704674665977,
-0.186541461035159));
#145894=CARTESIAN_POINT('Ctrl Pts',(-7.45592716814081,4.463393404623,-0.187920382063682));
#145895=CARTESIAN_POINT('Ctrl Pts',(-7.49761120477416,4.46959751865698,
-0.189278168036705));
#145896=CARTESIAN_POINT('Ctrl Pts',(-7.461638412,4.559946053,-0.75759634));
#145897=CARTESIAN_POINT('Ctrl Pts',(-7.503229697,4.494288122,-0.347959816));
#145898=CARTESIAN_POINT('Ctrl Pts',(-7.499728906,4.429844992,0.063767838));
#145899=CARTESIAN_POINT('Ctrl Pts',(-7.185019699,4.559946053,-0.96849983));
#145900=CARTESIAN_POINT('Ctrl Pts',(-7.238189376,4.494288122,-0.574049398));
#145901=CARTESIAN_POINT('Ctrl Pts',(-7.247859787,4.429844992,-0.176149108));
#145902=CARTESIAN_POINT('',(-7.46163841211182,4.55994605320497,-0.757596334230097));
#145903=CARTESIAN_POINT('Origin',(0.182131760323845,4.69632599733105,0.0403910335739126));
#145904=CARTESIAN_POINT('',(-7.32332905573954,4.5599460533341,-0.863048082967379));
#145905=CARTESIAN_POINT('Origin',(-2.32886626649886E-13,4.65175593299889,
2.85958322993052E-14));
#145906=CARTESIAN_POINT('',(-7.49751757547009,4.65066949966848,-0.192951307338631));
#145907=CARTESIAN_POINT('Origin',(0.191074840713347,4.69641604436513,0.012275030549841));
#145908=CARTESIAN_POINT('Origin',(0.191501065218327,4.55357338433389,0.0204808851773172));
#145909=CARTESIAN_POINT('Ctrl Pts',(-7.21843897666819,4.429837254,-2.03762136479284));
#145910=CARTESIAN_POINT('Ctrl Pts',(-7.32885259013124,4.494719353,-1.6464721815396));
#145911=CARTESIAN_POINT('Ctrl Pts',(-7.39635300274173,4.559946053,-1.24568228100516));
#145912=CARTESIAN_POINT('Ctrl Pts',(-7.39867306023058,4.56218796068555,
-1.23190672654212));
#145913=CARTESIAN_POINT('Ctrl Pts',(-7.40099311771942,4.5644298683711,-1.21813117207905));
#145914=CARTESIAN_POINT('Ctrl Pts',(-7.038294813,4.429837254,-1.739225727));
#145915=CARTESIAN_POINT('Ctrl Pts',(-7.13253911200001,4.494719353,-1.357838106));
#145916=CARTESIAN_POINT('Ctrl Pts',(-7.18501969900001,4.559946053,-0.96849983));
#145917=CARTESIAN_POINT('Ctrl Pts',(-7.18682350988321,4.56218796068555,
-0.955117879460748));
#145918=CARTESIAN_POINT('Ctrl Pts',(-7.18862732076655,4.5644298683711,-0.941735928921482));
#145919=CARTESIAN_POINT('',(-7.39592319198274,4.5599460519893,-1.24511852975822));
#145920=CARTESIAN_POINT('',(-7.29047144671895,4.559946050062,-1.10680916809047));
#145921=CARTESIAN_POINT('',(-7.28163200963444,4.46959751863828,-1.79661773201414));
#145922=CARTESIAN_POINT('Origin',(0.189981499374506,4.55357071573259,0.0330150592422844));
#145923=CARTESIAN_POINT('Ctrl Pts',(-7.03941442542484,4.43060907878943,
-1.73468860428));
#145924=CARTESIAN_POINT('Ctrl Pts',(-7.07971718183903,4.43741364855799,
-1.74504344049464));
#145925=CARTESIAN_POINT('Ctrl Pts',(-7.12007452219301,4.44406034770598,
-1.75538519133325));
#145926=CARTESIAN_POINT('Ctrl Pts',(-7.20080148942712,4.45704674579273,
-1.77602336632061));
#145927=CARTESIAN_POINT('Ctrl Pts',(-7.24121439563693,4.46339340288238,
-1.78633085064295));
#145928=CARTESIAN_POINT('Ctrl Pts',(-7.28163200993332,4.46959751863633,
-1.79661773084098));
#145929=CARTESIAN_POINT('Ctrl Pts',(-7.124328633,4.559946053,-2.343915853));
#145930=CARTESIAN_POINT('Ctrl Pts',(-7.253007281,4.494288122,-1.9527973));
#145931=CARTESIAN_POINT('Ctrl Pts',(-7.33809761200001,4.429844992,-1.549943043));
#145932=CARTESIAN_POINT('Ctrl Pts',(-6.808839097,4.559946053,-2.49042369));
#145933=CARTESIAN_POINT('Ctrl Pts',(-6.945560879,4.494288122,-2.116625199));
#145934=CARTESIAN_POINT('Ctrl Pts',(-7.040542002,4.429844992,-1.730106449));
#145935=CARTESIAN_POINT('',(-7.12432863437108,4.55994605320498,-2.34391584736187));
#145936=CARTESIAN_POINT('Origin',(0.169190777109376,4.69632600021766,0.0785996732235539));
#145937=CARTESIAN_POINT('',(-6.9665838656709,4.5599460533341,-2.41716976956639));
#145938=CARTESIAN_POINT('Origin',(-2.4156024402977E-13,4.65175593299956,
-9.37834879199961E-14));
#145939=CARTESIAN_POINT('',(-7.2807509534696,4.65066950026038,-1.80018486640627));
#145940=CARTESIAN_POINT('Origin',(0.183968884340725,4.69641606226494,0.0530635059363921));
#145941=CARTESIAN_POINT('Origin',(0.182620780952183,4.55357342913923,0.0611690349759017));
#145942=CARTESIAN_POINT('Ctrl Pts',(-6.61164752302496,4.429837254,-3.54173391420354));
#145943=CARTESIAN_POINT('Ctrl Pts',(-6.80356523950422,4.494719353,-3.18346524451117));
#145944=CARTESIAN_POINT('Ctrl Pts',(-6.95564551170398,4.559946053,-2.80655618233065));
#145945=CARTESIAN_POINT('Ctrl Pts',(-6.96087266440988,4.56218796062203,
-2.79360143681524));
#145946=CARTESIAN_POINT('Ctrl Pts',(-6.96609981711593,4.56442986824406,
-2.78064669129977));
#145947=CARTESIAN_POINT('Ctrl Pts',(-6.499861271,4.429837254,-3.211588931));
#145948=CARTESIAN_POINT('Ctrl Pts',(-6.673889256,4.494719353,-2.859377679));
#145949=CARTESIAN_POINT('Ctrl Pts',(-6.808839097,4.559946053,-2.49042369));
#145950=CARTESIAN_POINT('Ctrl Pts',(-6.81347745946702,4.56218796062203,
-2.47774236839224));
#145951=CARTESIAN_POINT('Ctrl Pts',(-6.81811582193404,4.56442986824406,
-2.46506104678444));
#145952=CARTESIAN_POINT('',(-6.9553469395449,4.5599460519893,-2.80591321467404));
#145953=CARTESIAN_POINT('',(-6.8820930220054,4.559946050062,-2.64816844109368));
#145954=CARTESIAN_POINT('',(-6.72517179477355,4.46959751860838,-3.31994944661299));
#145955=CARTESIAN_POINT('Origin',(0.178442605709245,4.55357069923117,0.0730836126927792));
#145956=CARTESIAN_POINT('Ctrl Pts',(-6.50193005456292,4.43060907880055,
-3.2073985664642));
#145957=CARTESIAN_POINT('Ctrl Pts',(-6.53906455731207,4.43741364599209,
-3.2261752065072));
#145958=CARTESIAN_POINT('Ctrl Pts',(-6.57625517906146,4.44406034250236,
-3.24495080026111));
#145959=CARTESIAN_POINT('Ctrl Pts',(-6.65065821995069,4.45704674453893,
-3.28246038940059));
#145960=CARTESIAN_POINT('Ctrl Pts',(-6.68791048246892,4.46339340034464,
-3.3012144667574));
#145961=CARTESIAN_POINT('Ctrl Pts',(-6.72517179537509,4.46959751860623,
-3.31994944541732));
#145962=CARTESIAN_POINT('Ctrl Pts',(-6.453893166,4.559946053,-3.820636465));
#145963=CARTESIAN_POINT('Ctrl Pts',(-6.663642306,4.494288122,-3.466324153));
#145964=CARTESIAN_POINT('Ctrl Pts',(-6.833345029,4.429844992,-3.09118031));
#145965=CARTESIAN_POINT('Ctrl Pts',(-6.114284746,4.559946053,-3.895898106));
#145966=CARTESIAN_POINT('Ctrl Pts',(-6.328165675,4.494288122,-3.560229957));
#145967=CARTESIAN_POINT('Ctrl Pts',(-6.504016297,4.429844992,-3.203165935));
#145968=CARTESIAN_POINT('',(-6.45389316855401,4.55994605320497,-3.82063645978579));
#145969=CARTESIAN_POINT('Origin',(0.14833844391806,4.69632602799791,0.113133000893504));
#145970=CARTESIAN_POINT('',(-6.28408895707088,4.5599460533341,-3.85826728375583));
#145971=CARTESIAN_POINT('Origin',(-6.44883452194378E-13,4.65175593299956,
-3.41523684332934E-13));
#145972=CARTESIAN_POINT('',(-6.72354450891252,4.65066950025556,-3.32324378227745));
#145973=CARTESIAN_POINT('Origin',(0.168260763809682,4.69641606952771,0.0913708077746189));
#145974=CARTESIAN_POINT('Origin',(0.165201840700276,4.55357343561515,0.0989970932106476));
#145975=CARTESIAN_POINT('Ctrl Pts',(-5.69570277961821,4.429837254,-4.88023892213889));
#145976=CARTESIAN_POINT('Ctrl Pts',(-5.96015074082042,4.494719353,-4.57160301106179));
#145977=CARTESIAN_POINT('Ctrl Pts',(-6.18969976651714,4.559946053,-4.23619863575322));
#145978=CARTESIAN_POINT('Ctrl Pts',(-6.19758959864021,4.56218796063338,
-4.22467044822775));
#145979=CARTESIAN_POINT('Ctrl Pts',(-6.20547943076325,4.56442986826676,
-4.21314226070228));
#145980=CARTESIAN_POINT('Ctrl Pts',(-5.65750144,4.429837254,-4.533781805));
#145981=CARTESIAN_POINT('Ctrl Pts',(-5.903175755,4.494719353,-4.227215929));
#145982=CARTESIAN_POINT('Ctrl Pts',(-6.114284746,4.559946053,-3.895898106));
#145983=CARTESIAN_POINT('Ctrl Pts',(-6.12154077548477,4.56218796063338,
-3.88451037740953));
#145984=CARTESIAN_POINT('Ctrl Pts',(-6.12879680496953,4.56442986826676,
-3.87312264881898));
#145985=CARTESIAN_POINT('',(-6.18954639384237,4.55994605198929,-4.23550651616055));
#145986=CARTESIAN_POINT('',(-6.15191557598764,4.55994605006201,-4.06570230088745));
#145987=CARTESIAN_POINT('',(-5.85425002175765,4.46959751860776,-4.68804401444961));
#145988=CARTESIAN_POINT('Origin',(0.1585595244886,4.55357068783892,0.109734557183265));
#145989=CARTESIAN_POINT('Ctrl Pts',(-5.66042266109747,4.43060907880261,
-4.53013413644781));
#145990=CARTESIAN_POINT('Ctrl Pts',(-5.69265255780897,4.43741364610902,
-4.55645460991157));
#145991=CARTESIAN_POINT('Ctrl Pts',(-5.72493748651506,4.44406034273362,
-4.58278612547743));
#145992=CARTESIAN_POINT('Ctrl Pts',(-5.78953757171177,4.45704674451748,
-4.63541321458658));
#145993=CARTESIAN_POINT('Ctrl Pts',(-5.82188732474689,4.46339340029751,
-4.66173696713832));
#145994=CARTESIAN_POINT('Ctrl Pts',(-5.85425002260382,4.4695975186056,-4.68804401340916));
#145995=CARTESIAN_POINT('Ctrl Pts',(-5.481680828,4.559946053,-5.11870836300001));
#145996=CARTESIAN_POINT('Ctrl Pts',(-5.762692823,4.494288122,-4.81776954));
#145997=CARTESIAN_POINT('Ctrl Pts',(-6.00907282800001,4.429844992,-4.487877421));
#145998=CARTESIAN_POINT('Ctrl Pts',(-5.133833235,4.559946053,-5.119204656));
#145999=CARTESIAN_POINT('Ctrl Pts',(-5.414872477,4.494288122,-4.83736232));
#146000=CARTESIAN_POINT('Ctrl Pts',(-5.663370019,4.429844992,-4.526448942));
#146001=CARTESIAN_POINT('',(-5.48168083158206,4.55994605320496,-5.11870835847377));
#146002=CARTESIAN_POINT('Origin',(0.120550304306342,4.69632602559465,0.142376541637629));
#146003=CARTESIAN_POINT('',(-5.30775703292076,4.55994605333409,-5.11895650802684));
#146004=CARTESIAN_POINT('Origin',(5.39065320159793E-13,4.65175593300022,
3.36970035208495E-13));
#146005=CARTESIAN_POINT('',(-5.85195259583039,4.65066950024768,-4.69091151220871));
#146006=CARTESIAN_POINT('Origin',(0.144684649761533,4.69641602837144,0.125405500661173));
#146007=CARTESIAN_POINT('Origin',(0.140058261803594,4.55357342842715,0.132196269379788));
#146008=CARTESIAN_POINT('Ctrl Pts',(-4.51343330429278,4.429837254,-5.99054938131607));
#146009=CARTESIAN_POINT('Ctrl Pts',(-4.83804621685821,4.494719353,-5.7459777007136));
#146010=CARTESIAN_POINT('Ctrl Pts',(-5.13433054042936,4.559946053,-5.46776114990866));
#146011=CARTESIAN_POINT('Ctrl Pts',(-5.14451413247666,4.56218796068985,
-5.45819856549634));
#146012=CARTESIAN_POINT('Ctrl Pts',(-5.15469772452387,4.56442986837969,
-5.44863598108387));
#146013=CARTESIAN_POINT('Ctrl Pts',(-4.55060313,4.429837254,-5.643980081));
#146014=CARTESIAN_POINT('Ctrl Pts',(-4.856436318,4.494719353,-5.39739426));
#146015=CARTESIAN_POINT('Ctrl Pts',(-5.133833235,4.559946053,-5.119204656));
#146016=CARTESIAN_POINT('Ctrl Pts',(-5.14336764776899,4.56218796068985,
-5.10964299777661));
#146017=CARTESIAN_POINT('Ctrl Pts',(-5.15290206053796,4.56442986837969,
-5.10008133955327));
#146018=CARTESIAN_POINT('',(-5.13432953879072,4.5599460519893,-5.46705224104394));
#146019=CARTESIAN_POINT('',(-5.13408139500295,4.559946050062,-5.29312843988776));
#146020=CARTESIAN_POINT('',(-4.70959002385817,4.46959751859485,-5.83693085503733));
#146021=CARTESIAN_POINT('Origin',(0.131263059169311,4.5535707426612,0.141254927737274));
#146022=CARTESIAN_POINT('Ctrl Pts',(-4.5542401956578,4.43060907883754,-5.64104566896126));
#146023=CARTESIAN_POINT('Ctrl Pts',(-4.58005846073345,4.43741364857084,
-5.67367927117784));
#146024=CARTESIAN_POINT('Ctrl Pts',(-4.60592809864141,4.44406034769415,
-5.70633548909699));
#146025=CARTESIAN_POINT('Ctrl Pts',(-4.65770458035733,4.45704674427068,
-5.77161926884762));
#146026=CARTESIAN_POINT('Ctrl Pts',(-4.68363918425479,4.46339339978764,
-5.80428182597552));
#146027=CARTESIAN_POINT('Ctrl Pts',(-4.70959002492802,4.46959751859253,
-5.83693085418741));
#146028=CARTESIAN_POINT('Ctrl Pts',(-4.253151186,4.559946053,-6.177435146));
#146029=CARTESIAN_POINT('Ctrl Pts',(-4.592286229,4.494288122,-5.943941379));
#146030=CARTESIAN_POINT('Ctrl Pts',(-4.903823059,4.429844992,-5.674726372));
#146031=CARTESIAN_POINT('Ctrl Pts',(-3.913329389,4.559946053,-6.103142887));
#146032=CARTESIAN_POINT('Ctrl Pts',(-4.24838586,4.494288122,-5.888304997));
#146033=CARTESIAN_POINT('Ctrl Pts',(-4.557910854,4.429844992,-5.638080227));
#146034=CARTESIAN_POINT('',(-4.2531511905143,4.55994605320497,-6.17743514233839));
#146035=CARTESIAN_POINT('Origin',(0.0871248502457178,4.6963259767227,0.16496220389796));
#146036=CARTESIAN_POINT('',(-4.08324028920423,4.55994605333409,-6.14028901536671));
#146037=CARTESIAN_POINT('Origin',(-2.28549817959944E-13,4.65175593300044,
-3.36102673470506E-13));
#146038=CARTESIAN_POINT('',(-4.70672988344605,4.65066950023002,-5.83923743366366));
#146039=CARTESIAN_POINT('Origin',(0.114343684782978,4.69641603551555,0.153576699705674));
#146040=CARTESIAN_POINT('Origin',(0.10836526325891,4.55357338805645,0.159213713368659));
#146041=CARTESIAN_POINT('Ctrl Pts',(-3.12012070376652,4.429837254,-6.820748410091));
#146042=CARTESIAN_POINT('Ctrl Pts',(-3.48972002876384,4.494719353,-6.65167686041999));
#146043=CARTESIAN_POINT('Ctrl Pts',(-3.8388857240293,4.559946053,-6.44365722867717));
#146044=CARTESIAN_POINT('Ctrl Pts',(-3.85088690238008,4.56218796069755,
-6.43650738338921));
#146045=CARTESIAN_POINT('Ctrl Pts',(-3.86288808073079,4.5644298683951,-6.42935753810134));
#146046=CARTESIAN_POINT('Ctrl Pts',(-3.230923675,4.429837254,-6.490272121));
#146047=CARTESIAN_POINT('Ctrl Pts',(-3.582615315,4.494719353,-6.315196435));
#146048=CARTESIAN_POINT('Ctrl Pts',(-3.913329389,4.559946053,-6.10314288700001));
#146049=CARTESIAN_POINT('Ctrl Pts',(-3.92469636645225,4.56218796069755,
-6.09585439192739));
#146050=CARTESIAN_POINT('Ctrl Pts',(-3.93606334390451,4.56442986839511,
-6.08856589685482));
#146051=CARTESIAN_POINT('',(-3.83903713795967,4.55994605198798,-6.44296468060183));
#146052=CARTESIAN_POINT('',(-3.87618327441021,4.559946050062,-6.27305377597788));
#146053=CARTESIAN_POINT('',(-3.34471483088038,4.46959751863189,-6.71288929577102));
#146054=CARTESIAN_POINT('Origin',(0.0978285057877903,4.55357072668722,0.166170023237531));
#146055=CARTESIAN_POINT('Ctrl Pts',(-3.23510652003408,4.43060907887121,
-6.48818817562549));
#146056=CARTESIAN_POINT('Ctrl Pts',(-3.25330590093075,4.43741364578292,
-6.52560897073948));
#146057=CARTESIAN_POINT('Ctrl Pts',(-3.27155059093039,4.44406034200068,
-6.56306289439335));
#146058=CARTESIAN_POINT('Ctrl Pts',(-3.30808250473215,4.45704674581605,
-6.63795083042892));
#146059=CARTESIAN_POINT('Ctrl Pts',(-3.32638929257642,4.46339340290249,
-6.67542493817343));
#146060=CARTESIAN_POINT('Ctrl Pts',(-3.34471483196707,4.46959751862983,
-6.71288929523981));
#146061=CARTESIAN_POINT('Ctrl Pts',(-2.825748922,4.559946053,-6.947311928));
#146062=CARTESIAN_POINT('Ctrl Pts',(-3.207149434,4.494288122,-6.792181124));
#146063=CARTESIAN_POINT('Ctrl Pts',(-3.569275975,4.429844992,-6.596231425));
#146064=CARTESIAN_POINT('Ctrl Pts',(-2.509842609,4.559946053,-6.801704939));
#146065=CARTESIAN_POINT('Ctrl Pts',(-2.883249442,4.494288122,-6.663917077));
#146066=CARTESIAN_POINT('Ctrl Pts',(-3.239328843,4.429844992,-6.486081147));
#146067=CARTESIAN_POINT('',(-2.82574892719149,4.55994605320497,-6.94731192539453));
#146068=CARTESIAN_POINT('Origin',(0.0496260836622386,4.69632598118124,0.179835099128474));
#146069=CARTESIAN_POINT('',(-2.66779576740801,4.55994605333409,-6.87450843275956));
#146070=CARTESIAN_POINT('Origin',(-2.26381413614973E-13,4.65175593299933,
-4.36282954208167E-13));
#146071=CARTESIAN_POINT('',(-3.34142571261755,4.65066950023686,-6.71452710230812));
#146072=CARTESIAN_POINT('Origin',(0.0786558871157211,4.6964160462467,0.174566560371842));
#146073=CARTESIAN_POINT('Origin',(0.0716056046167174,4.55357341172417,0.178786917787327));
#146074=CARTESIAN_POINT('Ctrl Pts',(-1.58091472753821,4.429837254,-7.33201682376214));
#146075=CARTESIAN_POINT('Ctrl Pts',(-1.97821841095581,4.494719353,-7.24635100303436));
#146076=CARTESIAN_POINT('Ctrl Pts',(-2.36393887818029,4.559946053,-7.11825505773228));
#146077=CARTESIAN_POINT('Ctrl Pts',(-2.37719648110749,4.56218796070865,
-7.11385227041945));
#146078=CARTESIAN_POINT('Ctrl Pts',(-2.39045408403462,4.56442986841731,
-7.1094494831066));
#146079=CARTESIAN_POINT('Ctrl Pts',(-1.76016982,4.429837254,-7.03308625));
#146080=CARTESIAN_POINT('Ctrl Pts',(-2.141275202,4.494719353,-6.93770704300001));
#146081=CARTESIAN_POINT('Ctrl Pts',(-2.509842609,4.559946053,-6.801704939));
#146082=CARTESIAN_POINT('Ctrl Pts',(-2.52251064388306,4.56218796070865,
-6.79703040900924));
#146083=CARTESIAN_POINT('Ctrl Pts',(-2.53517867876617,4.56442986841731,
-6.79235587901837));
#146084=CARTESIAN_POINT('',(-2.36423563221371,4.55994605198929,-7.11761124890048));
#146085=CARTESIAN_POINT('',(-2.4370391315969,4.559946050062,-6.95965808951324));
#146086=CARTESIAN_POINT('',(-1.82344448969034,4.46959751861481,-7.27496049448271));
#146087=CARTESIAN_POINT('Origin',(0.0598196423639694,4.55357070591541,0.183315160238214));
#146088=CARTESIAN_POINT('Ctrl Pts',(-1.76470285870704,4.43060907887909,
-7.0319502148614));
#146089=CARTESIAN_POINT('Ctrl Pts',(-1.77443238755811,4.43741364865479,
-7.07240847849282));
#146090=CARTESIAN_POINT('Ctrl Pts',(-1.78419904508117,4.44406034779995,
-7.11290883835043));
#146091=CARTESIAN_POINT('Ctrl Pts',(-1.80377816159113,4.45704674566609,
-7.19389918059214));
#146092=CARTESIAN_POINT('Ctrl Pts',(-1.81360112122397,4.46339340257863,
-7.2344325816342));
#146093=CARTESIAN_POINT('Ctrl Pts',(-1.82344449088131,4.46959751861249,
-7.2749604941938));
#146094=CARTESIAN_POINT('Ctrl Pts',(-1.266217779,4.559946053,-7.392340126));
#146095=CARTESIAN_POINT('Ctrl Pts',(-1.672049896,4.494288122,-7.32282603));
#146096=CARTESIAN_POINT('Ctrl Pts',(-2.067833513,4.429844992,-7.209304028));
#146097=CARTESIAN_POINT('Ctrl Pts',(-0.988998379000001,4.559946053,-7.182226828));
#146098=CARTESIAN_POINT('Ctrl Pts',(-1.383295485,4.494288122,-7.127931801));
#146099=CARTESIAN_POINT('Ctrl Pts',(-1.769279415,4.429844992,-7.030800122));
#146100=CARTESIAN_POINT('',(-1.26621778460305,4.55994605320497,-7.39234012456675));
#146101=CARTESIAN_POINT('Origin',(0.00980662171595426,4.69632599299584,
0.186298799465782));
#146102=CARTESIAN_POINT('',(-1.12760808102257,4.55994605333409,-7.28728347668704));
#146103=CARTESIAN_POINT('Origin',(1.57968256531138E-13,4.65175593299933,
9.04224611852911E-13));
#146104=CARTESIAN_POINT('',(-1.81988018947367,4.65066950021795,-7.27585294622769));
#146105=CARTESIAN_POINT('Origin',(0.0392903191542862,4.69641605117287,0.187394070549128));
#146106=CARTESIAN_POINT('Origin',(0.0314976175481438,4.55357338755637,0.19000014053232));
#146107=CARTESIAN_POINT('Ctrl Pts',(0.032213064727789,4.429837254,-7.50044828046727));
#146108=CARTESIAN_POINT('Ctrl Pts',(-0.374217498669831,4.494719353,-7.50219382594903));
#146109=CARTESIAN_POINT('Ctrl Pts',(-0.778456877615826,4.559946053,-7.46001119121922));
#146110=CARTESIAN_POINT('Ctrl Pts',(-0.792350993964793,4.56218796065686,
-7.45856133139514));
#146111=CARTESIAN_POINT('Ctrl Pts',(-0.806245110313756,4.56442986831374,
-7.45711147157109));
#146112=CARTESIAN_POINT('Ctrl Pts',(-0.207112381,4.429837254,-7.247041083));
#146113=CARTESIAN_POINT('Ctrl Pts',(-0.599811441,4.494719353,-7.23581818000001));
#146114=CARTESIAN_POINT('Ctrl Pts',(-0.988998379000001,4.559946053,-7.182226828));
#146115=CARTESIAN_POINT('Ctrl Pts',(-1.00237512772787,4.56218796065686,
-7.18038483902323));
#146116=CARTESIAN_POINT('Ctrl Pts',(-1.01575187645574,4.56442986831373,
-7.1785428500466));
#146117=CARTESIAN_POINT('',(-0.883941747984119,4.559946050062,-7.32083652582854));
#146118=CARTESIAN_POINT('Ctrl Pts',(-0.211783653451348,4.43060907881915,
-7.246906076998));
#146119=CARTESIAN_POINT('Ctrl Pts',(-0.212588380606481,4.43741364861059,
-7.28851000997835));
#146120=CARTESIAN_POINT('Ctrl Pts',(-0.213420318918682,4.44406034776933,
-7.33016303659061));
#146121=CARTESIAN_POINT('Ctrl Pts',(-0.215131156787447,4.45704674389096,
-7.41346878958388));
#146122=CARTESIAN_POINT('Ctrl Pts',(-0.216010977713216,4.46339339902968,
-7.45516617567207));
#146123=CARTESIAN_POINT('Ctrl Pts',(-0.216911912140415,4.46959751859056,
-7.49686262530735));
#146124=CARTESIAN_POINT('Ctrl Pts',(0.3525203,4.559946053,-7.49171071500001));
#146125=CARTESIAN_POINT('Ctrl Pts',(-0.058767163,4.494288122,-7.51106372900001));
#146126=CARTESIAN_POINT('Ctrl Pts',(-0.469701454,4.429844992,-7.485277586));
#146127=CARTESIAN_POINT('Ctrl Pts',(0.578090317,4.559946053,-7.226915773));
#146128=CARTESIAN_POINT('Ctrl Pts',(0.181339832,4.494288122,-7.258652356));
#146129=CARTESIAN_POINT('Ctrl Pts',(-0.216500448,4.429844992,-7.246766697));
#146130=CARTESIAN_POINT('',(0.465305306457437,4.55994605333409,-7.35931324412915));
#146131=CARTESIAN_POINT('Ctrl Pts',(1.64383461034797,4.429837254,-7.31816711034348));
#146132=CARTESIAN_POINT('Ctrl Pts',(1.2472814078235,4.494719353,-7.4072424037483));
#146133=CARTESIAN_POINT('Ctrl Pts',(0.843424901631317,4.559946053,-7.45294549263354));
#146134=CARTESIAN_POINT('Ctrl Pts',(0.829543944671895,4.56218796071086,
-7.45451635406576));
#146135=CARTESIAN_POINT('Ctrl Pts',(0.81566298771247,4.56442986842169,-7.45608721549797));
#146136=CARTESIAN_POINT('Ctrl Pts',(1.355629403,4.429837254,-7.12213233));
#146137=CARTESIAN_POINT('Ctrl Pts',(0.969698837,4.494719353,-7.195590502));
#146138=CARTESIAN_POINT('Ctrl Pts',(0.578090316999999,4.559946053,-7.226915773));
#146139=CARTESIAN_POINT('Ctrl Pts',(0.564630335725178,4.56218796071085,
-7.22799245427621));
#146140=CARTESIAN_POINT('Ctrl Pts',(0.551170354450339,4.56442986842171,
-7.22906913555243));
#146141=CARTESIAN_POINT('',(0.842885249818538,4.55994605198798,-7.45248579171881));
#146142=CARTESIAN_POINT('',(0.71048776996954,4.559946050062,-7.33970078274536));
#146143=CARTESIAN_POINT('',(1.39976322824942,4.46959751862171,-7.36821979213623));
#146144=CARTESIAN_POINT('Origin',(-0.0226811960224843,4.55357073441964,
0.191489976544781));
#146145=CARTESIAN_POINT('Ctrl Pts',(1.35103831954934,4.43060907872896,-7.12300466507705));
#146146=CARTESIAN_POINT('Ctrl Pts',(1.35919602247054,4.43741364847978,-7.1638089133596));
#146147=CARTESIAN_POINT('Ctrl Pts',(1.36733770405226,4.44406034762445,-7.204666957255));
#146148=CARTESIAN_POINT('Ctrl Pts',(1.38357514172299,4.4570467456653,-7.28639285949099));
#146149=CARTESIAN_POINT('Ctrl Pts',(1.39167959854772,4.46339340262745,-7.3273045318516));
#146150=CARTESIAN_POINT('Ctrl Pts',(1.39976322704982,4.4695975186195,-7.36821979237357));
#146151=CARTESIAN_POINT('Ctrl Pts',(1.954774922,4.559946053,-7.240777238));
#146152=CARTESIAN_POINT('Ctrl Pts',(1.557263457,4.494288122,-7.348092436));
#146153=CARTESIAN_POINT('Ctrl Pts',(1.150393323,4.429844992,-7.411247884));
#146154=CARTESIAN_POINT('Ctrl Pts',(2.118148151,4.559946053,-6.933682168));
#146155=CARTESIAN_POINT('Ctrl Pts',(1.7374959,4.494288122,-7.049966394));
#146156=CARTESIAN_POINT('Ctrl Pts',(1.346401839,4.429844992,-7.123882515));
#146157=CARTESIAN_POINT('',(1.95477491632479,4.55994605320496,-7.2407772390435));
#146158=CARTESIAN_POINT('Origin',(-0.0693245532869646,4.69632599728337,
0.173197784951975));
#146159=CARTESIAN_POINT('',(2.03646153453295,4.55994605333409,-7.08722970356522));
#146160=CARTESIAN_POINT('Origin',(1.8550699171227E-13,4.65175593299889,
-4.97431956736349E-13));
#146161=CARTESIAN_POINT('',(1.4033728301242,4.65066950020261,-7.36753314876966));
#146162=CARTESIAN_POINT('Origin',(-0.043025793661835,4.69641605817414,0.186571819988643));
#146163=CARTESIAN_POINT('Origin',(-0.0511925248948061,4.5535734263607,0.185665015335107));
#146164=CARTESIAN_POINT('Ctrl Pts',(3.17859227584221,4.429837254,-6.79369658045487));
#146165=CARTESIAN_POINT('Ctrl Pts',(2.81045882140123,4.494719353,-6.96593655960307));
#146166=CARTESIAN_POINT('Ctrl Pts',(2.42586906973883,4.559946053,-7.09738834678343));
#146167=CARTESIAN_POINT('Ctrl Pts',(2.41265033056979,4.56218796072225,-7.10190647780624));
#146168=CARTESIAN_POINT('Ctrl Pts',(2.39943159140081,4.56442986844461,-7.1064246088291));
#146169=CARTESIAN_POINT('Ctrl Pts',(2.854983464,4.429837254,-6.664200584));
#146170=CARTESIAN_POINT('Ctrl Pts',(2.493867074,4.494719353,-6.818905009));
#146171=CARTESIAN_POINT('Ctrl Pts',(2.118148151,4.559946053,-6.933682168));
#146172=CARTESIAN_POINT('Ctrl Pts',(2.10523431119399,4.56218796072225,-6.93762717516887));
#146173=CARTESIAN_POINT('Ctrl Pts',(2.09232047138791,4.56442986844461,-6.94157218233777));
#146174=CARTESIAN_POINT('',(2.42524320939363,4.55994605198931,-7.09705540292355));
#146175=CARTESIAN_POINT('',(2.27169566876629,4.55994605006201,-7.01536878858058));
#146176=CARTESIAN_POINT('',(2.95098699365994,4.46959751860328,-6.8950471905747));
#146177=CARTESIAN_POINT('Origin',(-0.0633156292957315,4.55357075974186,
0.182137308187349));
#146178=CARTESIAN_POINT('Ctrl Pts',(2.85068724327673,4.43060907887691,-6.66603947209202));
#146179=CARTESIAN_POINT('Ctrl Pts',(2.86742593071851,4.43741364860001,-6.70413607486207));
#146180=CARTESIAN_POINT('Ctrl Pts',(2.88416053584548,4.44406034771747,-6.74228865957532));
#146181=CARTESIAN_POINT('Ctrl Pts',(2.91758700058967,4.45704674433851,-6.81861327845623));
#146182=CARTESIAN_POINT('Ctrl Pts',(2.934296775964,4.46339339992011,-6.85682623120992));
#146183=CARTESIAN_POINT('Ctrl Pts',(2.95098699241346,4.46959751860108,-6.89504719111936));
#146184=CARTESIAN_POINT('Ctrl Pts',(3.465626441,4.559946053,-6.651273064));
#146185=CARTESIAN_POINT('Ctrl Pts',(3.100478168,4.494288122,-6.841532507));
#146186=CARTESIAN_POINT('Ctrl Pts',(2.716696986,4.429844992,-6.99067646800001));
#146187=CARTESIAN_POINT('Ctrl Pts',(3.559163733,4.559946053,-6.316237292));
#146188=CARTESIAN_POINT('Ctrl Pts',(3.212408591,4.494288122,-6.511631839));
#146189=CARTESIAN_POINT('Ctrl Pts',(2.846347872,4.429844992,-6.667893505));
#146190=CARTESIAN_POINT('',(3.4656264356673,4.55994605320497,-6.6512730662547));
#146191=CARTESIAN_POINT('Origin',(-0.104936233793004,4.69632599638227,0.154245883139481));
#146192=CARTESIAN_POINT('',(3.51239508520045,4.55994605333409,-6.48375517897486));
#146193=CARTESIAN_POINT('Origin',(3.42391046070922E-13,4.65175593300022,
-6.35342473076506E-13));
#146194=CARTESIAN_POINT('',(2.95436459746952,4.65066950022452,-6.89360064298541));
#146195=CARTESIAN_POINT('Origin',(-0.0821273224085139,4.696416072966,0.17296062846072));
#146196=CARTESIAN_POINT('Origin',(-0.0899080840477851,4.55357343357433,
0.170319208237301));
#146197=CARTESIAN_POINT('Ctrl Pts',(4.56472249940374,4.429837254,-5.95156034962665));
#146198=CARTESIAN_POINT('Ctrl Pts',(4.24222230535834,4.494719353,-6.19891126290004));
#146199=CARTESIAN_POINT('Ctrl Pts',(3.89488229582998,4.559946053,-6.40996520963038));
#146200=CARTESIAN_POINT('Ctrl Pts',(3.88294386901984,4.56218796053342,-6.41721934686453));
#146201=CARTESIAN_POINT('Ctrl Pts',(3.87100544220972,4.56442986806685,-6.4244734840987));
#146202=CARTESIAN_POINT('Ctrl Pts',(4.22084167,4.429837254,-5.894658226));
#146203=CARTESIAN_POINT('Ctrl Pts',(3.90142486,4.494719353,-6.123375096));
#146204=CARTESIAN_POINT('Ctrl Pts',(3.559163733,4.559946053,-6.316237292));
#146205=CARTESIAN_POINT('Ctrl Pts',(3.54739987251013,4.56218796053342,-6.32286616039471));
#146206=CARTESIAN_POINT('Ctrl Pts',(3.53563601202026,4.56442986806685,-6.32949502878957));
#146207=CARTESIAN_POINT('',(3.89419949472673,4.5599460519893,-6.40977459130288));
#146208=CARTESIAN_POINT('',(3.72668160336882,4.559946050062,-6.36300594715486));
#146209=CARTESIAN_POINT('',(4.36422588747414,4.46959751861275,-6.0994698457803));
#146210=CARTESIAN_POINT('Origin',(-0.100989590094247,4.55357066949384,0.164268187817004));
#146211=CARTESIAN_POINT('Ctrl Pts',(4.21704119950273,4.43060907879527,-5.89737768206882));
#146212=CARTESIAN_POINT('Ctrl Pts',(4.24157817912082,4.43741364575208,-5.9309852706859));
#146213=CARTESIAN_POINT('Ctrl Pts',(4.26612320506791,4.44406034201518,-5.96464840814477));
#146214=CARTESIAN_POINT('Ctrl Pts',(4.31517573742189,4.45704674471917,-6.03200292935783));
#146215=CARTESIAN_POINT('Ctrl Pts',(4.33970950448323,4.46339340071594,-6.06573037899577));
#146216=CARTESIAN_POINT('Ctrl Pts',(4.36422588640664,4.46959751861062,-6.09946984655637));
#146217=CARTESIAN_POINT('Ctrl Pts',(4.814429119,4.559946053,-5.75076275500001));
#146218=CARTESIAN_POINT('Ctrl Pts',(4.498717966,4.494288122,-6.015070122));
#146219=CARTESIAN_POINT('Ctrl Pts',(4.155970918,4.429844992,-6.24322879));
#146220=CARTESIAN_POINT('Ctrl Pts',(4.833756773,4.559946053,-5.403452179));
#146221=CARTESIAN_POINT('Ctrl Pts',(4.537112626,4.494288122,-5.668820616));
#146222=CARTESIAN_POINT('Ctrl Pts',(4.213201843,4.429844992,-5.900121205));
#146223=CARTESIAN_POINT('',(4.81442911428777,4.55994605320496,-5.75076275832939));
#146224=CARTESIAN_POINT('Origin',(-0.135641291056955,4.69632602118281,0.128081646994533));
#146225=CARTESIAN_POINT('',(4.82409294445209,4.55994605333409,-5.57710746833892));
#146226=CARTESIAN_POINT('Origin',(6.16911036144252E-13,4.65175593299889,
-7.42461647718073E-13));
#146227=CARTESIAN_POINT('',(4.36721355993797,4.6506695002325,-6.09733103257101));
#146228=CARTESIAN_POINT('Origin',(-0.117388650771652,4.69641607718384,0.151261954901537));
#146229=CARTESIAN_POINT('Origin',(-0.124419609548201,4.55357341342025,0.147009578589056));
#146230=CARTESIAN_POINT('Ctrl Pts',(5.73741137231444,4.429837254,-4.83113577047493));
#146231=CARTESIAN_POINT('Ctrl Pts',(5.47562418788991,4.494719353,-5.14203176680074));
#146232=CARTESIAN_POINT('Ctrl Pts',(5.18177515549747,4.559946053,-5.4228192230677));
#146233=CARTESIAN_POINT('Ctrl Pts',(5.17167526673081,4.56218796072131,-5.43247017223801));
#146234=CARTESIAN_POINT('Ctrl Pts',(5.16157537796409,4.56442986844264,-5.4421211214084));
#146235=CARTESIAN_POINT('Ctrl Pts',(5.389338011,4.429837254,-4.8494882));
#146236=CARTESIAN_POINT('Ctrl Pts',(5.12655635500001,4.494719353,-5.14152297));
#146237=CARTESIAN_POINT('Ctrl Pts',(4.833756773,4.559946053,-5.403452179));
#146238=CARTESIAN_POINT('Ctrl Pts',(4.8236929549059,4.56218796072131,-5.41245495111771));
#146239=CARTESIAN_POINT('Ctrl Pts',(4.81362913681171,4.56442986844262,-5.42145772323545));
#146240=CARTESIAN_POINT('',(5.18106734053446,4.5599460519893,-5.42277984334128));
#146241=CARTESIAN_POINT('',(5.00741204770229,4.559946050062,-5.41311601880107));
#146242=CARTESIAN_POINT('',(5.57339842935792,4.46959751862925,-5.01868807039529));
#146243=CARTESIAN_POINT('Origin',(-0.133941263718198,4.55357075941831,0.138717887482821));
#146244=CARTESIAN_POINT('Ctrl Pts',(5.38621099636352,4.43060907884818,-4.85296106573666));
#146245=CARTESIAN_POINT('Ctrl Pts',(5.4173989660286,4.43741364861691,-4.88050821382468));
#146246=CARTESIAN_POINT('Ctrl Pts',(5.44860673686744,4.44406034776174,-4.90810788376682));
#146247=CARTESIAN_POINT('Ctrl Pts',(5.51099165518376,4.45704674542827,-4.96334282803468));
#146248=CARTESIAN_POINT('Ctrl Pts',(5.54220224478526,4.46339340212321,-4.99100771729885));
#146249=CARTESIAN_POINT('Ctrl Pts',(5.57339842852905,4.46959751862724,-5.01868807132989));
#146250=CARTESIAN_POINT('Ctrl Pts',(5.938114442,4.559946053,-4.58135317));
#146251=CARTESIAN_POINT('Ctrl Pts',(5.686602712,4.494288122,-4.907349744));
#146252=CARTESIAN_POINT('Ctrl Pts',(5.400916269,4.429844992,-5.203854673));
#146253=CARTESIAN_POINT('Ctrl Pts',(5.88232872,4.559946053,-4.238007649));
#146254=CARTESIAN_POINT('Ctrl Pts',(5.649666317,4.494288122,-4.560941642));
#146255=CARTESIAN_POINT('Ctrl Pts',(5.383051178,4.429844992,-4.856465795));
#146256=CARTESIAN_POINT('',(5.93811443809986,4.55994605320497,-4.58135317430663));
#146257=CARTESIAN_POINT('Origin',(-0.160003744045962,4.69632600536354,0.0959282054421384));
#146258=CARTESIAN_POINT('',(5.91022157977611,4.55994605333409,-4.40968041114037));
#146259=CARTESIAN_POINT('Origin',(4.79217360238593E-13,4.65175593299911,
-4.35849273339173E-13));
#146260=CARTESIAN_POINT('',(5.57585647005731,4.65066950023898,-5.01595699988356));
#146261=CARTESIAN_POINT('Origin',(-0.147161144742348,4.69641605607194,0.122490578288943));
#146262=CARTESIAN_POINT('Origin',(-0.153113438793119,4.55357339955597,0.116826006957307));
#146263=CARTESIAN_POINT('Ctrl Pts',(6.6418252657073,4.429837254,-3.48481265260984));
#146264=CARTESIAN_POINT('Ctrl Pts',(6.45299196933265,4.494719353,-3.84471657929806));
#146265=CARTESIAN_POINT('Ctrl Pts',(6.22637396687215,4.559946053,-4.18210823669494));
#146266=CARTESIAN_POINT('Ctrl Pts',(6.21858487707689,4.5621879606059,-4.19370472897313));
#146267=CARTESIAN_POINT('Ctrl Pts',(6.21079578728161,4.56442986821181,-4.20530122125132));
#146268=CARTESIAN_POINT('Ctrl Pts',(6.305834896,4.429837254,-3.577561496));
#146269=CARTESIAN_POINT('Ctrl Pts',(6.111975772,4.494719353,-3.919258944));
#146270=CARTESIAN_POINT('Ctrl Pts',(5.88232872,4.559946053,-4.238007649));
#146271=CARTESIAN_POINT('Ctrl Pts',(5.87443551871049,4.5621879606059,-4.24896336416124));
#146272=CARTESIAN_POINT('Ctrl Pts',(5.8665423174211,4.56442986821181,-4.25991907932242));
#146273=CARTESIAN_POINT('',(6.22567423713373,4.55994605198798,-4.18222193475396));
#146274=CARTESIAN_POINT('',(6.05400147015755,4.559946050062,-4.21011480237209));
#146275=CARTESIAN_POINT('',(6.52196505506052,4.4695975186242,-3.70323801853134));
#146276=CARTESIAN_POINT('Origin',(-0.160629967077706,4.55357073825245,0.106681286855047));
#146277=CARTESIAN_POINT('Ctrl Pts',(6.30352755236844,4.43060907884243,-3.58162538384939));
#146278=CARTESIAN_POINT('Ctrl Pts',(6.33990818728124,4.43741364858599,-3.60182400328828));
#146279=CARTESIAN_POINT('Ctrl Pts',(6.37631945111121,4.44406034772407,-3.62206966001857));
#146280=CARTESIAN_POINT('Ctrl Pts',(6.44911973644291,4.45704674738329,-3.66260233480473));
#146281=CARTESIAN_POINT('Ctrl Pts',(6.48554778545811,4.46339340605651,-3.68291108688962));
#146282=CARTESIAN_POINT('Ctrl Pts',(6.52196505462289,4.46959751862424,-3.70323801931538));
#146283=CARTESIAN_POINT('Ctrl Pts',(6.784140134,4.559946053,-3.197724603));
#146284=CARTESIAN_POINT('Ctrl Pts',(6.608588236,4.494288122,-3.570167146));
#146285=CARTESIAN_POINT('Ctrl Pts',(6.393320778,4.429844992,-3.921154095));
#146286=CARTESIAN_POINT('Ctrl Pts',(6.655849513,4.559946053,-2.874398591));
#146287=CARTESIAN_POINT('Ctrl Pts',(6.49804789100001,4.494288122,-3.239798106));
#146288=CARTESIAN_POINT('Ctrl Pts',(6.301195022,4.429844992,-3.585727442));
#146289=CARTESIAN_POINT('',(6.78414013111715,4.55994605320497,-3.19772460804592));
#146290=CARTESIAN_POINT('Origin',(-0.176884535946686,4.69632599893794,0.0592893052161192));
#146291=CARTESIAN_POINT('',(6.71999482265735,4.55994605333409,-3.03606159886512));
#146292=CARTESIAN_POINT('Origin',(-9.61036805691151E-13,4.65175593300111,
5.07406616723216E-13));
#146293=CARTESIAN_POINT('',(6.52377852861029,4.65066950021574,-3.70004239307048));
#146294=CARTESIAN_POINT('Origin',(-0.170052142681483,4.69641603453242,0.0879913437510177));
#146295=CARTESIAN_POINT('Origin',(-0.174647839359464,4.55357340829506,0.0811797979911044));
#146296=CARTESIAN_POINT('Ctrl Pts',(7.23567479167722,4.429837254,-1.97554356808722));
#146297=CARTESIAN_POINT('Ctrl Pts',(7.12862501940249,4.494719353,-2.36762671771851));
#146298=CARTESIAN_POINT('Ctrl Pts',(6.97983445281553,4.559946053,-2.74584651831669));
#146299=CARTESIAN_POINT('Ctrl Pts',(6.97472037041059,4.56218796071268,-2.75884631576231));
#146300=CARTESIAN_POINT('Ctrl Pts',(6.96960628800551,4.56442986842537,-2.77184611320786));
#146301=CARTESIAN_POINT('Ctrl Pts',(6.92747795,4.429837254,-2.138351993));
#146302=CARTESIAN_POINT('Ctrl Pts',(6.811605995,4.494719353,-2.513734725));
#146303=CARTESIAN_POINT('Ctrl Pts',(6.655849513,4.559946053,-2.874398591));
#146304=CARTESIAN_POINT('Ctrl Pts',(6.65049600503019,4.56218796071268,-2.88679497320036));
#146305=CARTESIAN_POINT('Ctrl Pts',(6.64514249706051,4.56442986842537,-2.89919135540066));
#146306=CARTESIAN_POINT('',(6.97917552223325,4.5599460519893,-2.74610798203999));
#146307=CARTESIAN_POINT('',(6.81751251259641,4.559946050062,-2.81025329724772));
#146308=CARTESIAN_POINT('',(7.16557184357888,4.46959751864651,-2.21462867260384));
#146309=CARTESIAN_POINT('Origin',(-0.179807800035303,4.55357071148901,0.0696564124873245));
#146310=CARTESIAN_POINT('Ctrl Pts',(6.92609816677978,4.43060907880938,-2.14281687978804));
#146311=CARTESIAN_POINT('Ctrl Pts',(6.96597033268021,4.43741364583551,-2.15472250080301));
#146312=CARTESIAN_POINT('Ctrl Pts',(7.00588252093412,4.44406034215875,-2.16666747446528));
#146313=CARTESIAN_POINT('Ctrl Pts',(7.0856941328782,4.45704674670509,-2.19060261753264));
#146314=CARTESIAN_POINT('Ctrl Pts',(7.12563629114524,4.46339340470248,-2.20260560724937));
#146315=CARTESIAN_POINT('Ctrl Pts',(7.1655718432567,4.46959751864448,-2.21462867367502));
#146316=CARTESIAN_POINT('Ctrl Pts',(7.312946974,4.559946053,-1.664573988));
#146317=CARTESIAN_POINT('Ctrl Pts',(7.221563518,4.494288122,-2.0660475));
#146318=CARTESIAN_POINT('Ctrl Pts',(7.086780713,4.429844992,-2.455104709));
#146319=CARTESIAN_POINT('Ctrl Pts',(7.118150181,4.559946053,-1.376385849));
#146320=CARTESIAN_POINT('Ctrl Pts',(7.042587967,4.494288122,-1.767165211));
#146321=CARTESIAN_POINT('Ctrl Pts',(6.924701991,4.429844992,-2.147324459));
#146322=CARTESIAN_POINT('',(7.31294697226375,4.55994605320496,-1.66457399350293));
#146323=CARTESIAN_POINT('Origin',(-0.185494785591154,4.69632599477243,0.0198782917454832));
#146324=CARTESIAN_POINT('',(7.215548577078,4.55994605333409,-1.52047992050266));
#146325=CARTESIAN_POINT('Origin',(-5.92841747915074E-13,4.65175593300089,
1.16443313324943E-13));
#146326=CARTESIAN_POINT('',(7.16665595397576,4.65066950024027,-2.21111791586517));
#146327=CARTESIAN_POINT('Origin',(-0.184992040221171,4.69641607107543,0.0493779806617184));
#146328=CARTESIAN_POINT('Origin',(-0.188016192785251,4.55357343082071,0.0417378214458519));
#146329=CARTESIAN_POINT('Ctrl Pts',(7.49119220642967,4.429837254,-0.373900262486289));
#146330=CARTESIAN_POINT('Ctrl Pts',(7.47093148527094,4.494719353,-0.779829261862813));
#146331=CARTESIAN_POINT('Ctrl Pts',(7.40692563610591,4.559946053,-1.18119206711108));
#146332=CARTESIAN_POINT('Ctrl Pts',(7.40472569036061,4.56218796062276,-1.19498731250253));
#146333=CARTESIAN_POINT('Ctrl Pts',(7.40252574461543,4.56442986824553,-1.20878255789398));
#146334=CARTESIAN_POINT('Ctrl Pts',(7.225199835,4.429837254,-0.599155527));
#146335=CARTESIAN_POINT('Ctrl Pts',(7.192733093,4.494719353,-0.990671065));
#146336=CARTESIAN_POINT('Ctrl Pts',(7.118150181,4.559946053,-1.376385849));
#146337=CARTESIAN_POINT('Ctrl Pts',(7.11558669091173,4.56218796062276,-1.3896432560811));
#146338=CARTESIAN_POINT('Ctrl Pts',(7.1130232008236,4.56442986824553,-1.40290066316219));
#146339=CARTESIAN_POINT('',(7.40633831916757,4.55994605198798,-1.18158906556642));
#146340=CARTESIAN_POINT('',(7.26224424685807,4.559946050062,-1.27898747034023));
#146341=CARTESIAN_POINT('',(7.47412445643191,4.46959751866284,-0.6224657513944));
#146342=CARTESIAN_POINT('Origin',(-0.190578005963635,4.55357068622208,0.0293745193372734));
#146343=CARTESIAN_POINT('Ctrl Pts',(7.22481212866711,4.43060907879567,-0.603812640051713));
#146344=CARTESIAN_POINT('Ctrl Pts',(7.26631146379532,4.43741364611699,-0.606868577470451));
#146345=CARTESIAN_POINT('Ctrl Pts',(7.30785834553731,4.44406034275429,-0.609954343799243));
#146346=CARTESIAN_POINT('Ctrl Pts',(7.3909493589693,4.45704674800733,-0.616172759455037));
#146347=CARTESIAN_POINT('Ctrl Pts',(7.43253798891272,4.46339340732277,-0.619308743220647));
#146348=CARTESIAN_POINT('Ctrl Pts',(7.4741244563576,4.46959751866076,-0.622465752377321));
#146349=CARTESIAN_POINT('Ctrl Pts',(7.49980854000001,4.559946053,-0.053589743));
#146350=CARTESIAN_POINT('Ctrl Pts',(7.496866517,4.494288122,-0.465321769));
#146351=CARTESIAN_POINT('Ctrl Pts',(7.448870658,4.429844992,-0.874257356));
#146352=CARTESIAN_POINT('Ctrl Pts',(7.24761405700001,4.559946053,0.185985165));
#146353=CARTESIAN_POINT('Ctrl Pts',(7.257824457,4.494288122,-0.211901635));
#146354=CARTESIAN_POINT('Ctrl Pts',(7.224417591,4.429844992,-0.608514971));
#146355=CARTESIAN_POINT('',(7.49980853949836,4.55994605320497,-0.0535897487794385));
#146356=CARTESIAN_POINT('Origin',(-0.185431009943602,4.69632599840029,-0.0204623678710566));
#146357=CARTESIAN_POINT('',(7.37371129851837,4.55994605333409,0.0661977089534413));
#146358=CARTESIAN_POINT('Origin',(-7.19910242530375E-13,4.65175593300133,
5.37188295148677E-14));
#146359=CARTESIAN_POINT('',(7.47442851198713,4.65066950021361,-0.618804022598333));
#146360=CARTESIAN_POINT('Origin',(-0.191281892709029,4.69641607058777,0.00845574572821542));
#146361=CARTESIAN_POINT('Origin',(-0.192592715119703,4.55357341345698,0.000344072612098205));
#146362=CARTESIAN_POINT('Ctrl Pts',(7.39642979952305,4.429837254,1.24522620453003));
#146363=CARTESIAN_POINT('Ctrl Pts',(7.46390549869833,4.494719353,0.844432143113364));
#146364=CARTESIAN_POINT('Ctrl Pts',(7.48767721008715,4.559946053,0.438693611329296));
#146365=CARTESIAN_POINT('Ctrl Pts',(7.48849426784609,4.56218796063773,0.424747967699879));
#146366=CARTESIAN_POINT('Ctrl Pts',(7.48931132560489,4.56442986827546,0.410802324070462));
#146367=CARTESIAN_POINT('Ctrl Pts',(7.185079405,4.429837254,0.968056785));
#146368=CARTESIAN_POINT('Ctrl Pts',(7.23753598500001,4.494719353,0.578715273));
#146369=CARTESIAN_POINT('Ctrl Pts',(7.247614057,4.559946053,0.185985165));
#146370=CARTESIAN_POINT('Ctrl Pts',(7.24796045052581,4.56218796063773,0.172486634050456));
#146371=CARTESIAN_POINT('Ctrl Pts',(7.2483068440517,4.56442986827546,0.158988103100911));
#146372=CARTESIAN_POINT('',(7.48718896703819,4.55994605198842,0.438179637481071));
#146373=CARTESIAN_POINT('',(7.36740151176666,4.559946050062,0.312082388401445));
#146374=CARTESIAN_POINT('',(7.43319531657439,4.4695975186378,0.998802976821275));
#146375=CARTESIAN_POINT('Origin',(-0.192437143755373,4.55357069465802,-0.0122808925480036));
#146376=CARTESIAN_POINT('Ctrl Pts',(7.18570190538655,4.43060907888725,0.963425207556993));
#146377=CARTESIAN_POINT('Ctrl Pts',(7.22688796026147,4.43741364866101,0.96936184889719));
#146378=CARTESIAN_POINT('Ctrl Pts',(7.26812686428265,4.44406034780755,0.975279579985857));
#146379=CARTESIAN_POINT('Ctrl Pts',(7.3506119895181,4.45704674642975,0.987068653242497));
#146380=CARTESIAN_POINT('Ctrl Pts',(7.39190243297708,4.46339340412326,0.992946311536157));
#146381=CARTESIAN_POINT('Ctrl Pts',(7.43319531673589,4.46959751863569,0.998802975684803));
#146382=CARTESIAN_POINT('Ctrl Pts',(7.335987395,4.559946053,1.559900299));
#146383=CARTESIAN_POINT('Ctrl Pts',(7.421624369,4.494288122,1.157161891));
#146384=CARTESIAN_POINT('Ctrl Pts',(7.46265969,4.429844992,0.7474693));
#146385=CARTESIAN_POINT('Ctrl Pts',(7.038187555,4.559946053,1.73965972));
#146386=CARTESIAN_POINT('Ctrl Pts',(7.133693143,4.494288122,1.353270226));
#146387=CARTESIAN_POINT('Ctrl Pts',(7.186327454,4.429844992,0.958748));
#146388=CARTESIAN_POINT('',(7.3359873957426,4.55994605320496,1.55990029326451));
#146389=CARTESIAN_POINT('Origin',(-0.176697108651742,4.69632600886521,-0.0598461802887937));
#146390=CARTESIAN_POINT('',(7.1870874754579,4.55994605333409,1.64978000750524));
#146391=CARTESIAN_POINT('Origin',(1.14665221762067E-12,4.65175593300044,
9.24553402587014E-14));
#146392=CARTESIAN_POINT('',(7.43270510019513,4.65066949966071,1.00244445928465));
#146393=CARTESIAN_POINT('Origin',(-0.188627616882,4.6964160553568,-0.0328619031159097));
#146394=CARTESIAN_POINT('Origin',(-0.188164155281143,4.55357342077206,-0.0410657367178158));
#146395=CARTESIAN_POINT('Ctrl Pts',(6.95581855635293,4.429837254,2.80612727792483));
#146396=CARTESIAN_POINT('Ctrl Pts',(7.10787558655233,4.494719353,2.42920883959616));
#146397=CARTESIAN_POINT('Ctrl Pts',(7.21831331923951,4.559946053,2.03806646436907));
#146398=CARTESIAN_POINT('Ctrl Pts',(7.2221091757923,4.56218796063961,2.0246225053892));
#146399=CARTESIAN_POINT('Ctrl Pts',(7.22590503234511,4.56442986827924,2.01117854640926));
#146400=CARTESIAN_POINT('Ctrl Pts',(6.80899264800001,4.429837254,2.490003838));
#146401=CARTESIAN_POINT('Ctrl Pts',(6.94391973900001,4.494719353,2.121041529));
#146402=CARTESIAN_POINT('Ctrl Pts',(7.038187555,4.559946053,1.73965972));
#146403=CARTESIAN_POINT('Ctrl Pts',(7.04142763516438,4.56218796063961,1.72655124155173));
#146404=CARTESIAN_POINT('Ctrl Pts',(7.04466771532879,4.56442986827924,1.71344276310344));
#146405=CARTESIAN_POINT('',(7.21794698028822,4.55994605198931,2.03745954714603));
#146406=CARTESIAN_POINT('',(7.12806727013933,4.55994605006204,1.88855962198961));
#146407=CARTESIAN_POINT('',(7.04469822507141,4.46959751858764,2.5733687876881));
#146408=CARTESIAN_POINT('Origin',(-0.185298059327718,4.55357068452273,-0.0533620764200804));
#146409=CARTESIAN_POINT('Ctrl Pts',(6.81059624699143,4.43060907888844,2.48561436359437));
#146410=CARTESIAN_POINT('Ctrl Pts',(6.84954319239936,4.43741364864356,2.50026599383168));
#146411=CARTESIAN_POINT('Ctrl Pts',(6.88854581649443,4.44406034777539,2.51491051693363));
#146412=CARTESIAN_POINT('Ctrl Pts',(6.9665681668036,4.4570467436724,2.54415582565878));
#146413=CARTESIAN_POINT('Ctrl Pts',(7.00562972159081,4.46339339858634,2.55877228550805));
#146414=CARTESIAN_POINT('Ctrl Pts',(7.04469822557119,4.46959751858535,2.57336878635138));
#146415=CARTESIAN_POINT('Ctrl Pts',(6.829143632,4.559946053,3.100451136));
#146416=CARTESIAN_POINT('Ctrl Pts',(6.999355314,4.494288122,2.725537947));
#146417=CARTESIAN_POINT('Ctrl Pts',(7.127503049,4.429844992,2.334245122));
#146418=CARTESIAN_POINT('Ctrl Pts',(6.499663225,4.559946053,3.211989719));
#146419=CARTESIAN_POINT('Ctrl Pts',(6.675998265,4.494288122,2.855164676));
#146420=CARTESIAN_POINT('Ctrl Pts',(6.812212632,4.429844992,2.481180981));
#146421=CARTESIAN_POINT('',(6.82914363398258,4.55994605320497,3.10045113053292));
#146422=CARTESIAN_POINT('Origin',(-0.159700845982542,4.69632603422239,-0.0964316664364823));
#146423=CARTESIAN_POINT('',(6.66440342937601,4.55994605333409,3.15622042565031));
#146424=CARTESIAN_POINT('Origin',(1.56038376664114E-12,4.65175593300044,
6.68735899989059E-13));
#146425=CARTESIAN_POINT('',(7.04343665848191,4.6506695002242,2.57681975219685));
#146426=CARTESIAN_POINT('Origin',(-0.177153273387559,4.69641602642132,-0.0726429733137191));
#146427=CARTESIAN_POINT('Origin',(-0.174936767560196,4.55357340111542,-0.0805552607661836));
#146428=CARTESIAN_POINT('Ctrl Pts',(6.18996096719782,4.429837254,4.23581695831155));
#146429=CARTESIAN_POINT('Ctrl Pts',(6.41948931138595,4.494719353,3.90039843069377));
#146430=CARTESIAN_POINT('Ctrl Pts',(6.61142911962848,4.559946053,3.5421415952428));
#146431=CARTESIAN_POINT('Ctrl Pts',(6.61802628507903,4.56218796068781,3.52982794525585));
#146432=CARTESIAN_POINT('Ctrl Pts',(6.62462345052944,4.56442986837561,3.51751429526898));
#146433=CARTESIAN_POINT('Ctrl Pts',(6.114524963,4.429837254,3.895521079));
#146434=CARTESIAN_POINT('Ctrl Pts',(6.32561352300001,4.494719353,3.564190239));
#146435=CARTESIAN_POINT('Ctrl Pts',(6.499663225,4.559946053,3.211989719));
#146436=CARTESIAN_POINT('Ctrl Pts',(6.50564548939436,4.5621879606878,3.19988423070406));
#146437=CARTESIAN_POINT('Ctrl Pts',(6.51162775378881,4.56442986837561,3.18777874240813));
#146438=CARTESIAN_POINT('',(6.61120181473443,4.5599460519893,3.54147011535814));
#146439=CARTESIAN_POINT('',(6.55543252479518,4.559946050062,3.37672990639611));
#146440=CARTESIAN_POINT('',(6.32679887445887,4.4695975186562,4.02760673392859));
#146441=CARTESIAN_POINT('Origin',(-0.169494590604762,4.55357069773733,-0.0919480823373431));
#146442=CARTESIAN_POINT('Ctrl Pts',(6.11703467734612,4.43060907876927,3.89157895395253));
#146443=CARTESIAN_POINT('Ctrl Pts',(6.15192138417053,4.43741364598305,3.91426047067408));
#146444=CARTESIAN_POINT('Ctrl Pts',(6.18686399414782,4.44406034250939,3.93694701468659));
#146445=CARTESIAN_POINT('Ctrl Pts',(6.25677539552244,4.45704674721445,3.98228111406106));
#146446=CARTESIAN_POINT('Ctrl Pts',(6.29178162727773,4.46339340574468,4.00495294261198));
#146447=CARTESIAN_POINT('Ctrl Pts',(6.32679887503795,4.46959751865421,4.02760673303402));
#146448=CARTESIAN_POINT('Ctrl Pts',(6.002976704,4.559946053,4.496028325));
#146449=CARTESIAN_POINT('Ctrl Pts',(6.24980418500001,4.494288122,4.166470877));
#146450=CARTESIAN_POINT('Ctrl Pts',(6.459072287,4.429844992,3.811874236));
#146451=CARTESIAN_POINT('Ctrl Pts',(5.657221867,4.559946053,4.534130649));
#146452=CARTESIAN_POINT('Ctrl Pts',(5.906141128,4.494288122,4.223554798));
#146453=CARTESIAN_POINT('Ctrl Pts',(6.119566318,4.429844992,3.887596697));
#146454=CARTESIAN_POINT('',(6.00297670706392,4.55994605320496,4.49602832011822));
#146455=CARTESIAN_POINT('Origin',(-0.135237164733756,4.69632598481314,-0.12850808202611));
#146456=CARTESIAN_POINT('',(5.83009928675316,4.55994605333409,4.51507948538187));
#146457=CARTESIAN_POINT('Origin',(-8.76469036237282E-13,4.65175593300044,
-4.99166680212326E-13));
#146458=CARTESIAN_POINT('',(6.32482494729382,4.65066950023528,4.03070581740142));
#146459=CARTESIAN_POINT('Origin',(-0.157395227798709,4.69641604213913,-0.109027212761467));
#146460=CARTESIAN_POINT('Origin',(-0.153530278004034,4.5535734277484,-0.11627844380942));
#146461=CARTESIAN_POINT('Ctrl Pts',(5.13466768313966,4.429837254,5.46744454587086));
#146462=CARTESIAN_POINT('Ctrl Pts',(5.43093485171026,4.494719353,5.18920972569578));
#146463=CARTESIAN_POINT('Ctrl Pts',(5.69540184317369,4.559946053,4.88059012097226));
#146464=CARTESIAN_POINT('Ctrl Pts',(5.70449184166015,4.56218796077457,4.86998255242729));
#146465=CARTESIAN_POINT('Ctrl Pts',(5.71358184014662,4.56442986854915,4.85937498388234));
#146466=CARTESIAN_POINT('Ctrl Pts',(5.134148886,4.429837254,5.118888084));
#146467=CARTESIAN_POINT('Ctrl Pts',(5.411528649,4.494719353,4.840681376));
#146468=CARTESIAN_POINT('Ctrl Pts',(5.657221867,4.559946053,4.534130649));
#146469=CARTESIAN_POINT('Ctrl Pts',(5.66566659186864,4.56218796077458,4.52359418987881));
#146470=CARTESIAN_POINT('Ctrl Pts',(5.67411131673747,4.56442986854915,4.51305773075765));
#146471=CARTESIAN_POINT('',(5.69532420086355,4.55994605198929,4.87988547605668));
#146472=CARTESIAN_POINT('',(5.67627304106311,4.559946050062,4.70700805305583));
#146473=CARTESIAN_POINT('',(5.31306543994044,4.46959751861898,5.29351826587812));
#146474=CARTESIAN_POINT('Origin',(-0.145765720939184,4.55357073318668,-0.126234648917299));
#146475=CARTESIAN_POINT('Ctrl Pts',(5.13744736506547,4.43060907879088,5.1155776381838));
#146476=CARTESIAN_POINT('Ctrl Pts',(5.16664258312233,4.43741364571329,5.1452284831325));
#146477=CARTESIAN_POINT('Ctrl Pts',(5.19589131650275,4.44406034193146,5.17489625514891));
#146478=CARTESIAN_POINT('Ctrl Pts',(5.2544227315973,4.45704674544457,5.23419934774933));
#146479=CARTESIAN_POINT('Ctrl Pts',(5.28373675530313,4.4633934021658,5.26386641755855));
#146480=CARTESIAN_POINT('Ctrl Pts',(5.31306544082685,4.46959751861678,5.29351826500183));
#146481=CARTESIAN_POINT('Ctrl Pts',(4.896117256,4.559946053,5.681376225));
#146482=CARTESIAN_POINT('Ctrl Pts',(5.208019157,4.494288122,5.41258426));
#146483=CARTESIAN_POINT('Ctrl Pts',(5.488622484,4.429844992,5.11126434800001));
#146484=CARTESIAN_POINT('Ctrl Pts',(4.550255102,4.559946053,5.644260669));
#146485=CARTESIAN_POINT('Ctrl Pts',(4.860119396,4.494288122,5.394456192));
#146486=CARTESIAN_POINT('Ctrl Pts',(5.14077588500001,4.429844992,5.112232712));
#146487=CARTESIAN_POINT('',(4.89611726008958,4.55994605320499,5.68137622087235));
#146488=CARTESIAN_POINT('Origin',(-0.104450017754835,4.69632601596199,-0.154575716975075));
#146489=CARTESIAN_POINT('',(4.72318618057174,4.5599460533341,5.66281844568906));
#146490=CARTESIAN_POINT('Origin',(5.52509427098613E-13,4.65175593299956,
5.20417042793042E-13));
#146491=CARTESIAN_POINT('',(5.31047145089206,4.65066950022844,5.29612055861478));
#146492=CARTESIAN_POINT('Origin',(-0.130277934192288,4.69641604863111,-0.140313671209675));
#146493=CARTESIAN_POINT('Origin',(-0.124944090093938,4.55357340165287,-0.146564086543545));
#146494=CARTESIAN_POINT('Ctrl Pts',(3.83928304573516,4.429837254,6.44342050301162));
#146495=CARTESIAN_POINT('Ctrl Pts',(4.18843591350799,4.494719353,6.23537934195569));
#146496=CARTESIAN_POINT('Ctrl Pts',(4.51306390582353,4.559946053,5.99082767770735));
#146497=CARTESIAN_POINT('Ctrl Pts',(4.52422169846457,4.56218796069278,5.98242218950456));
#146498=CARTESIAN_POINT('Ctrl Pts',(4.53537949110564,4.56442986838557,5.97401670130179));
#146499=CARTESIAN_POINT('Ctrl Pts',(3.913705713,4.429837254,6.10290157100001));
#146500=CARTESIAN_POINT('Ctrl Pts',(4.24440671,4.494719353,5.890827631));
#146501=CARTESIAN_POINT('Ctrl Pts',(4.550255102,4.559946053,5.644260669));
#146502=CARTESIAN_POINT('Ctrl Pts',(4.56076742077199,4.56218796069278,5.63578591297389));
#146503=CARTESIAN_POINT('Ctrl Pts',(4.57127973954398,4.56442986838555,5.62731115694767));
#146504=CARTESIAN_POINT('',(4.51313955453792,4.55994605198798,5.9901228186567));
#146505=CARTESIAN_POINT('',(4.53169733829032,4.559946050062,5.81719173486759));
#146506=CARTESIAN_POINT('',(4.05089897038185,4.46959751858392,6.31191076693112));
#146507=CARTESIAN_POINT('Origin',(-0.115221112852132,4.55357071772783,-0.154618720067957));
#146508=CARTESIAN_POINT('Ctrl Pts',(3.91763872356155,4.43060907883284,6.10037759741906));
#146509=CARTESIAN_POINT('Ctrl Pts',(3.93977732792986,4.43741364861268,6.13561134577958));
#146510=CARTESIAN_POINT('Ctrl Pts',(3.96196455879317,4.44406034776373,6.17087313154928));
#146511=CARTESIAN_POINT('Ctrl Pts',(4.00637910359353,4.45704674351445,6.24137223282395));
#146512=CARTESIAN_POINT('Ctrl Pts',(4.02863023130927,4.46339339827232,6.27664734001664));
#146513=CARTESIAN_POINT('Ctrl Pts',(4.05089897160215,4.4695975185816,6.31191076616091));
#146514=CARTESIAN_POINT('Ctrl Pts',(3.560320807,4.559946053,6.601069288));
#146515=CARTESIAN_POINT('Ctrl Pts',(3.922712942,4.494288122,6.405611219));
#146516=CARTESIAN_POINT('Ctrl Pts',(4.261530793,4.429844992,6.171657419));
#146517=CARTESIAN_POINT('Ctrl Pts',(3.230523466,4.559946053,6.49047133400001));
#146518=CARTESIAN_POINT('Ctrl Pts',(3.586843883,4.494288122,6.31311881));
#146519=CARTESIAN_POINT('Ctrl Pts',(3.921608485,4.429844992,6.09782640700001));
#146520=CARTESIAN_POINT('',(3.56032081188552,4.55994605320498,6.60106928484802));
#146521=CARTESIAN_POINT('Origin',(-0.0687787297306519,4.69632601369697,
-0.173415322549491));
#146522=CARTESIAN_POINT('',(3.39542213831681,4.5599460533341,6.54577031005758));
#146523=CARTESIAN_POINT('Origin',(1.1145598333151E-12,4.65175593300067,
1.71824360295503E-12));
#146524=CARTESIAN_POINT('',(4.04780621136812,4.65066950020758,6.31389458847702));
#146525=CARTESIAN_POINT('Origin',(-0.0970687103811368,4.69641607733215,
-0.165038982886628));
#146526=CARTESIAN_POINT('Origin',(-0.0905159256706362,4.55357342512397,
-0.169996615526339));
#146527=CARTESIAN_POINT('Ctrl Pts',(2.3643777998641,4.429837254,7.11810927906325));
#146528=CARTESIAN_POINT('Ctrl Pts',(2.75009036708087,4.494719353,6.98998954960996));
#146529=CARTESIAN_POINT('Ctrl Pts',(3.11970011632363,4.559946053,6.82094079018461));
#146530=CARTESIAN_POINT('Ctrl Pts',(3.13240397732229,4.56218796066586,6.81513041330432));
#146531=CARTESIAN_POINT('Ctrl Pts',(3.14510783832095,4.56442986833173,6.80932003642402));
#146532=CARTESIAN_POINT('Ctrl Pts',(2.510262011,4.429837254,6.801550164));
#146533=CARTESIAN_POINT('Ctrl Pts',(2.878821031,4.494719353,6.665525334));
#146534=CARTESIAN_POINT('Ctrl Pts',(3.230523466,4.559946053,6.490471334));
#146535=CARTESIAN_POINT('Ctrl Pts',(3.24261183449213,4.56218796066586,6.48445455092591));
#146536=CARTESIAN_POINT('Ctrl Pts',(3.25470020298429,4.56442986833173,6.47843776785193));
#146537=CARTESIAN_POINT('',(3.11992552026391,4.55994605198798,6.82026867260156));
#146538=CARTESIAN_POINT('',(3.17522450484931,4.55994605006201,6.65536999669987));
#146539=CARTESIAN_POINT('',(2.5993169674646,4.46959751859883,7.0351653357458));
#146540=CARTESIAN_POINT('Origin',(-0.0792889617611636,4.55357072500979,
-0.175773205964725));
#146541=CARTESIAN_POINT('Ctrl Pts',(2.51464564998812,4.43060907880633,6.79993067958229));
#146542=CARTESIAN_POINT('Ctrl Pts',(2.52869244599149,4.43741364583256,6.83909981235757));
#146543=CARTESIAN_POINT('Ctrl Pts',(2.54278070368981,4.44406034218614,6.87830677841121));
#146544=CARTESIAN_POINT('Ctrl Pts',(2.57100165160829,4.4570467441366,6.95670550167926));
#146545=CARTESIAN_POINT('Ctrl Pts',(2.58514945651061,4.46339339956602,6.99593923562996));
#146546=CARTESIAN_POINT('Ctrl Pts',(2.59931696875979,4.46959751859659,7.03516533527836));
#146547=CARTESIAN_POINT('Ctrl Pts',(2.058047714,4.559946053,7.212103688));
#146548=CARTESIAN_POINT('Ctrl Pts',(2.45398503,4.494288122,7.099118916));
#146549=CARTESIAN_POINT('Ctrl Pts',(2.835174659,4.429844992,6.943470649));
#146550=CARTESIAN_POINT('Ctrl Pts',(1.759736143,4.559946053,7.03319477300001));
#146551=CARTESIAN_POINT('Ctrl Pts',(2.145851537,4.494288122,6.936587009));
#146552=CARTESIAN_POINT('Ctrl Pts',(2.519071031,4.429844992,6.798292516));
#146553=CARTESIAN_POINT('',(2.05804771942638,4.55994605320498,7.21210368597038));
#146554=CARTESIAN_POINT('Origin',(-0.0298916218067086,4.69632598925499,
-0.184146545734074));
#146555=CARTESIAN_POINT('',(1.90889193047692,4.5599460533341,7.12264922997018));
#146556=CARTESIAN_POINT('Origin',(4.04190569902596E-13,4.651755933,1.11542719505309E-12));
#146557=CARTESIAN_POINT('',(2.59587005224224,4.65066950021632,7.03643792502342));
#146558=CARTESIAN_POINT('Origin',(-0.0593208284753782,4.69641607253455,
-0.182047421545034));
#146559=CARTESIAN_POINT('Origin',(-0.051855568022259,4.5535734567917,-0.185480708781655));
#146560=CARTESIAN_POINT('Ctrl Pts',(0.778916875458042,4.429837254,7.45996317561411));
#146561=CARTESIAN_POINT('Ctrl Pts',(1.18315365183431,4.494719353,7.4177556149989));
#146562=CARTESIAN_POINT('Ctrl Pts',(1.58046261703443,4.559946053,7.33211429230165));
#146563=CARTESIAN_POINT('Ctrl Pts',(1.59411852788503,4.56218796062931,7.32917071344912));
#146564=CARTESIAN_POINT('Ctrl Pts',(1.60777443873569,4.56442986825872,7.32622713459661));
#146565=CARTESIAN_POINT('Ctrl Pts',(0.989441248,4.429837254,7.182165831));
#146566=CARTESIAN_POINT('Ctrl Pts',(1.37862488,4.494719353,7.12855048));
#146567=CARTESIAN_POINT('Ctrl Pts',(1.759736143,4.559946053,7.033194773));
#146568=CARTESIAN_POINT('Ctrl Pts',(1.77283532244858,4.56218796062931,7.02991730093683));
#146569=CARTESIAN_POINT('Ctrl Pts',(1.78593450189721,4.56442986825872,7.02663982887367));
#146570=CARTESIAN_POINT('',(1.5808272365642,4.55994605198799,7.33150634364818));
#146571=CARTESIAN_POINT('',(1.67028170264388,4.55994605006201,7.18235055439685));
#146572=CARTESIAN_POINT('',(1.02619379194291,4.46959751861026,7.42946339227434));
#146573=CARTESIAN_POINT('Origin',(-0.0396491670115839,4.55357071019899,
-0.188708442845131));
#146574=CARTESIAN_POINT('Ctrl Pts',(0.994070540727967,4.4306090787179,7.18152656204117));
#146575=CARTESIAN_POINT('Ctrl Pts',(0.999368724674737,4.43741364584496,
7.22279958843321));
#146576=CARTESIAN_POINT('Ctrl Pts',(1.00469926796512,4.44406034229402,7.26411847670696));
#146577=CARTESIAN_POINT('Ctrl Pts',(1.0154070183226,4.45704674513233,7.346750956186));
#146578=CARTESIAN_POINT('Ctrl Pts',(1.02078996321937,4.46339340157552,7.38810879397391));
#146579=CARTESIAN_POINT('Ctrl Pts',(1.02619379320752,4.46959751860798,7.42946339210943));
#146580=CARTESIAN_POINT('Ctrl Pts',(0.459542598,4.559946053,7.485908135));
#146581=CARTESIAN_POINT('Ctrl Pts',(0.870511505,4.494288122,7.460679703));
#146582=CARTESIAN_POINT('Ctrl Pts',(1.276248909,4.429844992,7.390614908));
#146583=CARTESIAN_POINT('Ctrl Pts',(0.206665513,4.559946053,7.24705384000001));
#146584=CARTESIAN_POINT('Ctrl Pts',(0.604521557,4.494288122,7.235708109));
#146585=CARTESIAN_POINT('Ctrl Pts',(0.998744615,4.429844992,7.180878024));
#146586=CARTESIAN_POINT('',(0.459542603715409,4.55994605320497,7.48590813417827));
#146587=CARTESIAN_POINT('Origin',(0.0103932901638211,4.6963260159548,-0.186267111405733));
#146588=CARTESIAN_POINT('',(0.333104057544598,4.5599460533341,7.36648098740755));
#146589=CARTESIAN_POINT('Origin',(1.11808349037568E-13,4.65175593299867,
3.36970035208495E-13));
#146590=CARTESIAN_POINT('',(1.02255389523181,4.65066950018923,7.42996524430959));
#146591=CARTESIAN_POINT('Origin',(-0.0187991239028218,4.69641606393237,
-0.190543498803789));
#146592=CARTESIAN_POINT('Origin',(-0.010770327658639,4.55357343712198,-0.192291557691001));
#146593=CARTESIAN_POINT('Origin',(3.1413063881873E-14,4.65175593299889,
-5.35162192338845E-13));
#146594=CARTESIAN_POINT('',(-0.0321887715704092,4.55994605198799,7.49993092670762));
#146595=CARTESIAN_POINT('Origin',(0.00184455323510964,4.55357069936849,
-0.192820044880267));
#146596=CARTESIAN_POINT('',(-0.598575745926012,4.65066950019027,7.4760756466581));
#146597=CARTESIAN_POINT('Origin',(0.0226016159796813,4.69641607088498,-0.190129976565602));
#146598=CARTESIAN_POINT('Origin',(0.0308184870555671,4.55357345041732,-0.190111286116755));
#146599=CARTESIAN_POINT('Ctrl Pts',(-0.842965336257949,4.429837254,7.45299748588614));
#146600=CARTESIAN_POINT('Ctrl Pts',(-0.439106013265463,4.494719353,7.49867567223329));
#146601=CARTESIAN_POINT('Ctrl Pts',(-0.0326755574928418,4.559946053,7.50044627943846));
#146602=CARTESIAN_POINT('Ctrl Pts',(-0.0187061319879682,4.56218796059731,
7.50050713699747));
#146603=CARTESIAN_POINT('Ctrl Pts',(-0.00473670648309503,4.56442986819472,
7.50056799455651));
#146604=CARTESIAN_POINT('Ctrl Pts',(-0.577644689,4.429837254,7.226951405));
#146605=CARTESIAN_POINT('Ctrl Pts',(-0.186034238,4.494719353,7.25825252900001));
#146606=CARTESIAN_POINT('Ctrl Pts',(0.206665513,4.559946053,7.24705384));
#146607=CARTESIAN_POINT('Ctrl Pts',(0.220163000305543,4.56218796059731,
7.24666892974164));
#146608=CARTESIAN_POINT('Ctrl Pts',(0.233660487611081,4.56442986819472,
7.24628401948334));
#146609=CARTESIAN_POINT('',(0.087238384113425,4.55994605006201,7.37349238228569));
#146610=CARTESIAN_POINT('Ctrl Pts',(-0.0311662252067879,1.197203562,7.50045145207052));
#146611=CARTESIAN_POINT('Ctrl Pts',(0.374955034121473,1.261925886,7.50213898586559));
#146612=CARTESIAN_POINT('Ctrl Pts',(0.778884123117372,1.327100493,7.45996533766874));
#146613=CARTESIAN_POINT('Ctrl Pts',(0.792744303612179,1.32933685537475,
7.45851821639903));
#146614=CARTESIAN_POINT('Ctrl Pts',(0.80660448410698,1.33157321774951,7.45707109512947));
#146615=CARTESIAN_POINT('Ctrl Pts',(0.208122714,1.197203562,7.247012139));
#146616=CARTESIAN_POINT('Ctrl Pts',(0.600521186,1.261925886,7.235743076));
#146617=CARTESIAN_POINT('Ctrl Pts',(0.989408718000001,1.327100493,7.18217031200001));
#146618=CARTESIAN_POINT('Ctrl Pts',(1.00275277152954,1.32933685537475,7.18033204830749));
#146619=CARTESIAN_POINT('Ctrl Pts',(1.01609682505909,1.33157321774952,7.17849378461507));
#146620=CARTESIAN_POINT('',(0.212788489828452,1.19797317409522,7.24687664206066));
#146621=CARTESIAN_POINT('Origin',(-0.029119033607513,1.33927933890375,-0.196346974783305));
#146622=CARTESIAN_POINT('Ctrl Pts',(0.212788489729122,1.19797317409288,
7.2468766420302));
#146623=CARTESIAN_POINT('Ctrl Pts',(0.213408818267352,1.20265893835229,
7.27550948625658));
#146624=CARTESIAN_POINT('Ctrl Pts',(0.214002544381766,1.20726223981372,
7.30415652228153));
#146625=CARTESIAN_POINT('Ctrl Pts',(0.214571291475999,1.21178747097482,
7.33281625257192));
#146626=CARTESIAN_POINT('Ctrl Pts',(0.214676296681177,1.21262294394929,
7.33810756902866));
#146627=CARTESIAN_POINT('Ctrl Pts',(0.214780860070305,1.21345569336825,
7.34339933287842));
#146628=CARTESIAN_POINT('Ctrl Pts',(0.214885194021124,1.214285714,7.34869153090483));
#146629=CARTESIAN_POINT('Ctrl Pts',(0.215319481528753,1.21774065444455,
7.37072017354804));
#146630=CARTESIAN_POINT('Ctrl Pts',(0.215750821020856,1.22115495459576,
7.39275528414919));
#146631=CARTESIAN_POINT('Ctrl Pts',(0.216194451260588,1.2245278005957,7.41479644373849));
#146632=CARTESIAN_POINT('Ctrl Pts',(0.216744671851216,1.2287110350823,7.44213339861891));
#146633=CARTESIAN_POINT('Ctrl Pts',(0.217305051301642,1.23283187911727,
7.46947976624647));
#146634=CARTESIAN_POINT('Ctrl Pts',(0.217874905420452,1.23689319502459,
7.4968347000478));
#146635=CARTESIAN_POINT('Ctrl Pts',(1.25849016475008,1.32841655815206,7.39366423866198));
#146636=CARTESIAN_POINT('Ctrl Pts',(1.26256514337504,1.32775852557603,7.39296600483099));
#146637=CARTESIAN_POINT('Ctrl Pts',(1.266640122,1.327100493,7.392267771));
#146638=CARTESIAN_POINT('Ctrl Pts',(1.618926333,1.270212881,7.331904718));
#146639=CARTESIAN_POINT('Ctrl Pts',(1.963875725,1.214285714,7.238314178));
#146640=CARTESIAN_POINT('Ctrl Pts',(2.016468661,1.205758742,7.22404483400001));
#146641=CARTESIAN_POINT('Ctrl Pts',(2.068848696,1.197204389,7.209012767));
#146642=CARTESIAN_POINT('Ctrl Pts',(0.981490392688463,1.32841655815206,
7.18326113271219));
#146643=CARTESIAN_POINT('Ctrl Pts',(0.985449555344232,1.32775852557603,
7.18271572235609));
#146644=CARTESIAN_POINT('Ctrl Pts',(0.989408718,1.327100493,7.18217031200001));
#146645=CARTESIAN_POINT('Ctrl Pts',(1.331682516,1.270212881,7.13501901));
#146646=CARTESIAN_POINT('Ctrl Pts',(1.667921256,1.214285714,7.055532488));
#146647=CARTESIAN_POINT('Ctrl Pts',(1.719186117,1.205758742,7.043413523));
#146648=CARTESIAN_POINT('Ctrl Pts',(1.770269464,1.197204389,7.030550905));
#146649=CARTESIAN_POINT('',(1.76567787415336,1.19797317427034,7.03170545742107));
#146650=CARTESIAN_POINT('Ctrl Pts',(1.76567787426916,1.19797317415285,7.03170545796061));
#146651=CARTESIAN_POINT('Ctrl Pts',(1.73312358395914,1.20342302018589,7.03987991737876));
#146652=CARTESIAN_POINT('Ctrl Pts',(1.70053641067916,1.20886077954585,7.04782229606081));
#146653=CARTESIAN_POINT('Ctrl Pts',(1.66792125607932,1.21428571398681,7.05553248798125));
#146654=CARTESIAN_POINT('Ctrl Pts',(1.52423747091137,1.23818488470188,7.08949919970331));
#146655=CARTESIAN_POINT('Ctrl Pts',(1.37901947255166,1.26233328407548,7.11918993281469));
#146656=CARTESIAN_POINT('Ctrl Pts',(1.2326558542626,1.28666618647768,7.14444256381536));
#146657=CARTESIAN_POINT('Ctrl Pts',(1.15189907534906,1.30009197385974,7.158375815552));
#146658=CARTESIAN_POINT('Ctrl Pts',(1.07079398594151,1.31357385569416,7.17095875770949));
#146659=CARTESIAN_POINT('Ctrl Pts',(0.989408725594587,1.32710049182887,
7.18217031144485));
#146660=CARTESIAN_POINT('Ctrl Pts',(1.82437897686925,1.23689319179771,7.27472620427518));
#146661=CARTESIAN_POINT('Ctrl Pts',(1.81762552129248,1.23263224513668,7.24682614389789));
#146662=CARTESIAN_POINT('Ctrl Pts',(1.81088428609454,1.22830577224837,7.21893304355694));
#146663=CARTESIAN_POINT('Ctrl Pts',(1.80415624475797,1.22391046495537,7.19104769004101));
#146664=CARTESIAN_POINT('Ctrl Pts',(1.79774357016075,1.21972118102936,7.16446942020277));
#146665=CARTESIAN_POINT('Ctrl Pts',(1.79135285131702,1.21547100858144,7.1378953600032));
#146666=CARTESIAN_POINT('Ctrl Pts',(1.78494930497304,1.21115091644535,7.11133583589125));
#146667=CARTESIAN_POINT('Ctrl Pts',(1.77854559786201,1.20683071584928,7.08477564497744));
#146668=CARTESIAN_POINT('Ctrl Pts',(1.77212215308869,1.20243940496519,7.05823165975828));
#146669=CARTESIAN_POINT('Ctrl Pts',(1.76567787233811,1.19797317480699,7.0317054555096));
#146670=CARTESIAN_POINT('Ctrl Pts',(1.58193777457235,1.197203562,7.33179488248356));
#146671=CARTESIAN_POINT('Ctrl Pts',(1.9789269150576,1.261925886,7.24613889640439));
#146672=CARTESIAN_POINT('Ctrl Pts',(2.36434627734697,1.327100493,7.11811843102544));
#146673=CARTESIAN_POINT('Ctrl Pts',(2.37757132469114,1.32933685512278,7.11372561405432));
#146674=CARTESIAN_POINT('Ctrl Pts',(2.39079637203526,1.33157321724558,7.10933279708321));
#146675=CARTESIAN_POINT('Ctrl Pts',(1.76115031,1.197203562,7.032840791));
#146676=CARTESIAN_POINT('Ctrl Pts',(2.141952209,1.261925886,6.93748112));
#146677=CARTESIAN_POINT('Ctrl Pts',(2.510231206,1.327100493,6.801561533));
#146678=CARTESIAN_POINT('Ctrl Pts',(2.52286810919618,1.32933685512278,6.79689767033782));
#146679=CARTESIAN_POINT('Ctrl Pts',(2.53550501239241,1.33157321724559,6.79223380767549));
#146680=CARTESIAN_POINT('Origin',(-0.0706469541574262,1.33927932656119,
-0.185496486810866));
#146681=CARTESIAN_POINT('Ctrl Pts',(2.81848662049146,1.32841655815206,6.95026629291661));
#146682=CARTESIAN_POINT('Ctrl Pts',(2.82231622874573,1.32775852557603,6.9487083834583));
#146683=CARTESIAN_POINT('Ctrl Pts',(2.826145837,1.327100493,6.947150474));
#146684=CARTESIAN_POINT('Ctrl Pts',(3.15721952,1.270212881,6.812467554));
#146685=CARTESIAN_POINT('Ctrl Pts',(3.473984987,1.214285714,6.646911186));
#146686=CARTESIAN_POINT('Ctrl Pts',(3.522280843,1.205758742,6.62166952500001));
#146687=CARTESIAN_POINT('Ctrl Pts',(3.570204811,1.197204389,6.59572874));
#146688=CARTESIAN_POINT('Ctrl Pts',(2.50273250095792,1.32841655815206,6.80432905678979));
#146689=CARTESIAN_POINT('Ctrl Pts',(2.50648185347896,1.32775852557603,6.80294529489489));
#146690=CARTESIAN_POINT('Ctrl Pts',(2.510231206,1.327100493,6.801561533));
#146691=CARTESIAN_POINT('Ctrl Pts',(2.834366696,1.270212881,6.681933854));
#146692=CARTESIAN_POINT('Ctrl Pts',(3.145657109,1.214285714,6.532024292));
#146693=CARTESIAN_POINT('Ctrl Pts',(3.193118207,1.205758742,6.509168232));
#146694=CARTESIAN_POINT('Ctrl Pts',(3.240242171,1.197204389,6.485624925));
#146695=CARTESIAN_POINT('',(3.23600612405357,1.19797317421957,6.48773954035198));
#146696=CARTESIAN_POINT('Ctrl Pts',(3.23600612183536,1.19797317447889,6.48773953829102));
#146697=CARTESIAN_POINT('Ctrl Pts',(3.190985273,1.20614195,6.510195399));
#146698=CARTESIAN_POINT('Ctrl Pts',(3.145657109,1.214285714,6.532024292));
#146699=CARTESIAN_POINT('Ctrl Pts',(2.83436669912389,1.27021288012494,6.68193385275316));
#146700=CARTESIAN_POINT('Ctrl Pts',(2.5102312133073,1.32710049490568,6.80156153026079));
#146701=CARTESIAN_POINT('Ctrl Pts',(3.34557710467326,1.2368931917972,6.71245959653521));
#146702=CARTESIAN_POINT('Ctrl Pts',(3.33298385271176,1.23263224513067,6.6866636173957));
#146703=CARTESIAN_POINT('Ctrl Pts',(3.32040403182692,1.22830577224287,6.66087180846766));
#146704=CARTESIAN_POINT('Ctrl Pts',(3.30783876168844,1.22391046495352,6.63508472895175));
#146705=CARTESIAN_POINT('Ctrl Pts',(3.29586246955396,1.21972118103539,6.61050637972617));
#146706=CARTESIAN_POINT('Ctrl Pts',(3.28390852482557,1.21547100859969,6.58592742187279));
#146707=CARTESIAN_POINT('Ctrl Pts',(3.27194517730308,1.2111509164746,6.56136541780598));
#146708=CARTESIAN_POINT('Ctrl Pts',(3.25998152942953,1.20683071588954,6.53680279708701));
#146709=CARTESIAN_POINT('Ctrl Pts',(3.2480020891073,1.20243940502162,6.51226024618941));
#146710=CARTESIAN_POINT('Ctrl Pts',(3.23600612183536,1.19797317447889,6.48773953829102));
#146711=CARTESIAN_POINT('Ctrl Pts',(3.12107212213229,1.197203562,6.82031173226986));
#146712=CARTESIAN_POINT('Ctrl Pts',(3.49036637109644,1.261925886,6.65131740573583));
#146713=CARTESIAN_POINT('Ctrl Pts',(3.83925422858829,1.327100493,6.44343621778777));
#146714=CARTESIAN_POINT('Ctrl Pts',(3.85122575575511,1.32933685509038,6.43630310829271));
#146715=CARTESIAN_POINT('Ctrl Pts',(3.86319728292196,1.33157321718078,6.42916999879751));
#146716=CARTESIAN_POINT('Ctrl Pts',(3.231828475,1.197203562,6.489821624));
#146717=CARTESIAN_POINT('Ctrl Pts',(3.583227927,1.261925886,6.314830257));
#146718=CARTESIAN_POINT('Ctrl Pts',(3.913678072,1.327100493,6.102919297));
#146719=CARTESIAN_POINT('Ctrl Pts',(3.92501693863925,1.32933685509038,6.09564791234125));
#146720=CARTESIAN_POINT('Ctrl Pts',(3.93635580527844,1.33157321718077,6.08837652768251));
#146721=CARTESIAN_POINT('Origin',(-0.108871366719813,1.33927930073689,-0.165972435109042));
#146722=CARTESIAN_POINT('Ctrl Pts',(4.24669377469677,1.32841655815206,6.18188161995671));
#146723=CARTESIAN_POINT('Ctrl Pts',(4.25009894434838,1.32775852557603,6.17953688097835));
#146724=CARTESIAN_POINT('Ctrl Pts',(4.253504114,1.327100493,6.177192142));
#146725=CARTESIAN_POINT('Ctrl Pts',(4.547884631,1.270212881,5.974486978));
#146726=CARTESIAN_POINT('Ctrl Pts',(4.821654572,1.214285714,5.744706014));
#146727=CARTESIAN_POINT('Ctrl Pts',(4.863395087,1.205758742,5.709672308));
#146728=CARTESIAN_POINT('Ctrl Pts',(4.904622117,1.197204389,5.674035767));
#146729=CARTESIAN_POINT('Ctrl Pts',(3.90694961831175,1.32841655815206,6.10723411756124));
#146730=CARTESIAN_POINT('Ctrl Pts',(3.91031384515587,1.32775852557603,6.10507670728062));
#146731=CARTESIAN_POINT('Ctrl Pts',(3.913678072,1.327100493,6.102919297));
#146732=CARTESIAN_POINT('Ctrl Pts',(4.20451904,1.270212881,5.916408897));
#146733=CARTESIAN_POINT('Ctrl Pts',(4.476305531,1.214285714,5.703085901));
#146734=CARTESIAN_POINT('Ctrl Pts',(4.517743638,1.205758742,5.67056147000001));
#146735=CARTESIAN_POINT('Ctrl Pts',(4.55870475500001,1.197204389,5.637438333));
#146736=CARTESIAN_POINT('',(4.55502232464208,1.19797317423656,5.64041413517156));
#146737=CARTESIAN_POINT('Ctrl Pts',(4.5550223262341,1.19797317450824,5.64041413707271));
#146738=CARTESIAN_POINT('Ctrl Pts',(4.45269302247191,1.21932945754499,5.72305208213578));
#146739=CARTESIAN_POINT('Ctrl Pts',(4.34815191940103,1.24060038382255,5.80287856834028));
#146740=CARTESIAN_POINT('Ctrl Pts',(4.18786400048255,1.2728618071633,5.91850090968448));
#146741=CARTESIAN_POINT('Ctrl Pts',(4.13380351650863,1.28366385405618,5.95638525333352));
#146742=CARTESIAN_POINT('Ctrl Pts',(4.05190608929962,1.29991103400534,6.01212525060261));
#146743=CARTESIAN_POINT('Ctrl Pts',(4.02444922772756,1.30533866131656,6.03053905404981));
#146744=CARTESIAN_POINT('Ctrl Pts',(3.98306679322179,1.31349012124639,6.05788350614987));
#146745=CARTESIAN_POINT('Ctrl Pts',(3.96923445152479,1.31620998869334,6.06695570360523));
#146746=CARTESIAN_POINT('Ctrl Pts',(3.94843724190009,1.32029216629499,6.0804943727962));
#146747=CARTESIAN_POINT('Ctrl Pts',(3.94149544566517,1.32165353797213,6.08499647671232));
#146748=CARTESIAN_POINT('Ctrl Pts',(3.92791385812345,1.32431471601509,6.09377182750367));
#146749=CARTESIAN_POINT('Ctrl Pts',(3.92454773867684,1.32497441947025,6.09594880219572));
#146750=CARTESIAN_POINT('Ctrl Pts',(3.91367807818555,1.32710049214421,6.10291929458987));
#146751=CARTESIAN_POINT('Ctrl Pts',(4.71033976554031,1.23689319179788,5.83632583836518));
#146752=CARTESIAN_POINT('Ctrl Pts',(4.69249556405988,1.23263224512587,5.81384013165564));
#146753=CARTESIAN_POINT('Ctrl Pts',(4.67466537587517,1.22830577223152,5.79135561055883));
#146754=CARTESIAN_POINT('Ctrl Pts',(4.65685041491457,1.22391046493341,5.76887258033722));
#146755=CARTESIAN_POINT('Ctrl Pts',(4.63987050326617,1.21972118100769,5.74744340810409));
#146756=CARTESIAN_POINT('Ctrl Pts',(4.62291228568413,1.21547100855891,5.72600883746783));
#146757=CARTESIAN_POINT('Ctrl Pts',(4.60594852970562,1.21115091642268,5.70459284556852));
#146758=CARTESIAN_POINT('Ctrl Pts',(4.58898434783614,1.2068307158265,5.68317631600067));
#146759=CARTESIAN_POINT('Ctrl Pts',(4.5720090572157,1.20243940496165,5.66178278189173));
#146760=CARTESIAN_POINT('Ctrl Pts',(4.55502232146844,1.19797317447799,5.64041413304004));
#146761=CARTESIAN_POINT('Ctrl Pts',(4.51426860610597,1.197203562,5.98991838655528));
#146762=CARTESIAN_POINT('Ctrl Pts',(4.83860017587706,1.261925886,5.74548770562734));
#146763=CARTESIAN_POINT('Ctrl Pts',(5.13464291838637,1.327100493,5.46746608780804));
#146764=CARTESIAN_POINT('Ctrl Pts',(5.14480114980126,1.32933685500188,5.4579262223541));
#146765=CARTESIAN_POINT('Ctrl Pts',(5.15495938121626,1.33157321700378,5.44838635690018));
#146766=CARTESIAN_POINT('Ctrl Pts',(4.551389933,1.197203562,5.643345611));
#146767=CARTESIAN_POINT('Ctrl Pts',(4.85695589,1.261925886,5.39690495));
#146768=CARTESIAN_POINT('Ctrl Pts',(5.134125702,1.327100493,5.118911337));
#146769=CARTESIAN_POINT('Ctrl Pts',(5.14363633910482,1.32933685500188,5.10937243248646));
#146770=CARTESIAN_POINT('Ctrl Pts',(5.15314697620968,1.33157321700379,5.09983352797292));
#146771=CARTESIAN_POINT('Origin',(-0.14200526905505,1.33927922316676,-0.138688075081163));
#146772=CARTESIAN_POINT('Ctrl Pts',(5.47633024678037,1.32841655815206,5.12443903217739));
#146773=CARTESIAN_POINT('Ctrl Pts',(5.47915175589019,1.32775852557603,5.12141710108869));
#146774=CARTESIAN_POINT('Ctrl Pts',(5.481973265,1.327100493,5.11839517));
#146775=CARTESIAN_POINT('Ctrl Pts',(5.725895711,1.270212881,4.857146032));
#146776=CARTESIAN_POINT('Ctrl Pts',(5.943868948,1.214285714,4.573884774));
#146777=CARTESIAN_POINT('Ctrl Pts',(5.977102382,1.205758742,4.53069716));
#146778=CARTESIAN_POINT('Ctrl Pts',(6.009704745,1.197204389,4.487031188));
#146779=CARTESIAN_POINT('Ctrl Pts',(5.12848211471851,1.32841655815206,5.12457169809598));
#146780=CARTESIAN_POINT('Ctrl Pts',(5.13130390835926,1.32775852557603,5.121741517548));
#146781=CARTESIAN_POINT('Ctrl Pts',(5.134125702,1.327100493,5.118911337));
#146782=CARTESIAN_POINT('Ctrl Pts',(5.378072746,1.270212881,4.874239236));
#146783=CARTESIAN_POINT('Ctrl Pts',(5.597646882,1.214285714,4.607477551));
#146784=CARTESIAN_POINT('Ctrl Pts',(5.631124397,1.205758742,4.566805555));
#146785=CARTESIAN_POINT('Ctrl Pts',(5.664007371,1.197204389,4.52565139));
#146786=CARTESIAN_POINT('',(5.66105074323027,1.19797317421628,4.52934923308381));
#146787=CARTESIAN_POINT('Ctrl Pts',(5.66105074131956,1.19797317480725,4.52934923316803));
#146788=CARTESIAN_POINT('Ctrl Pts',(5.629619895,1.20614195,4.568633382));
#146789=CARTESIAN_POINT('Ctrl Pts',(5.597646882,1.214285714,4.607477551));
#146790=CARTESIAN_POINT('Ctrl Pts',(5.37807274867207,1.27021288013103,4.87423923389415));
#146791=CARTESIAN_POINT('Ctrl Pts',(5.13412570708811,1.32710049454013,5.11891133135881));
#146792=CARTESIAN_POINT('Ctrl Pts',(5.85485217388923,1.23689319179752,4.68729197081351));
#146793=CARTESIAN_POINT('Ctrl Pts',(5.83259139768625,1.23263224512641,4.66916794326474));
#146794=CARTESIAN_POINT('Ctrl Pts',(5.81034456199047,1.22830577224701,4.65104206117558));
#146795=CARTESIAN_POINT('Ctrl Pts',(5.78811291800978,1.22391046496545,4.63291436170114));
#146796=CARTESIAN_POINT('Ctrl Pts',(5.76692334865123,1.21972118105214,4.61563637066915));
#146797=CARTESIAN_POINT('Ctrl Pts',(5.74575380567806,1.2154710086199,4.59834844384771));
#146798=CARTESIAN_POINT('Ctrl Pts',(5.72458284762704,1.21115091649015,4.58107985205215));
#146799=CARTESIAN_POINT('Ctrl Pts',(5.70341135805905,1.20683071590039,4.56381082671223));
#146800=CARTESIAN_POINT('Ctrl Pts',(5.68223396277897,1.20243940503825,4.54656664728988));
#146801=CARTESIAN_POINT('Ctrl Pts',(5.66105074131956,1.19797317480725,4.52934923316803));
#146802=CARTESIAN_POINT('Ctrl Pts',(5.69638290676076,1.197203562,4.87944311363531));
#146803=CARTESIAN_POINT('Ctrl Pts',(5.96058641405332,1.261925886,4.57100538662929));
#146804=CARTESIAN_POINT('Ctrl Pts',(6.18994141211522,1.327100493,4.2358433205941));
#146805=CARTESIAN_POINT('Ctrl Pts',(6.19781136074892,1.32933685503111,4.22434277224787));
#146806=CARTESIAN_POINT('Ctrl Pts',(6.20568130938254,1.33157321706224,4.21284222390164));
#146807=CARTESIAN_POINT('Ctrl Pts',(5.658133455,1.197203562,4.532993029));
#146808=CARTESIAN_POINT('Ctrl Pts',(5.903577993,1.261925886,4.226626366));
#146809=CARTESIAN_POINT('Ctrl Pts',(6.114507319,1.327100493,3.895548773));
#146810=CARTESIAN_POINT('Ctrl Pts',(6.12174502027091,1.32933685503111,3.88418837679022));
#146811=CARTESIAN_POINT('Ctrl Pts',(6.12898272154169,1.33157321706224,3.87282798058039));
#146812=CARTESIAN_POINT('Origin',(-0.168499168376953,1.33927933743112,-0.104918689288322));
#146813=CARTESIAN_POINT('Ctrl Pts',(6.44989960413632,1.32841655815206,3.82738337217394));
#146814=CARTESIAN_POINT('Ctrl Pts',(6.45200552206816,1.32775852557603,3.82382555108697));
#146815=CARTESIAN_POINT('Ctrl Pts',(6.45411144,1.327100493,3.82026773));
#146816=CARTESIAN_POINT('Ctrl Pts',(6.636170272,1.270212881,3.512690335));
#146817=CARTESIAN_POINT('Ctrl Pts',(6.788154619,1.214285714,3.189193765));
#146818=CARTESIAN_POINT('Ctrl Pts',(6.811327012,1.205758742,3.139871648));
#146819=CARTESIAN_POINT('Ctrl Pts',(6.833780257,1.197204389,3.090218018));
#146820=CARTESIAN_POINT('Ctrl Pts',(6.110212485956,1.32841655815206,3.9022900024487));
#146821=CARTESIAN_POINT('Ctrl Pts',(6.112359902478,1.32775852557603,3.89891938772435));
#146822=CARTESIAN_POINT('Ctrl Pts',(6.114507319,1.327100493,3.895548773));
#146823=CARTESIAN_POINT('Ctrl Pts',(6.300153748,1.270212881,3.604155566));
#146824=CARTESIAN_POINT('Ctrl Pts',(6.457248486,1.214285714,3.296428672));
#146825=CARTESIAN_POINT('Ctrl Pts',(6.481200039,1.205758742,3.249510888));
#146826=CARTESIAN_POINT('Ctrl Pts',(6.504467298,1.197204389,3.202250017));
#146827=CARTESIAN_POINT('',(6.50237472112378,1.19797317411054,3.20649699370496));
#146828=CARTESIAN_POINT('Ctrl Pts',(6.50237471819508,1.1979731744789,3.2064969933566));
#146829=CARTESIAN_POINT('Ctrl Pts',(6.48012364,1.20614195,3.251619405));
#146830=CARTESIAN_POINT('Ctrl Pts',(6.457248486,1.214285714,3.296428672));
#146831=CARTESIAN_POINT('Ctrl Pts',(6.30015374986331,1.27021288013871,3.60415556227763));
#146832=CARTESIAN_POINT('Ctrl Pts',(6.11450732322867,1.32710049475556,3.89554876596969));
#146833=CARTESIAN_POINT('Ctrl Pts',(6.72559820205922,1.2368931917972,3.31908553995813));
#146834=CARTESIAN_POINT('Ctrl Pts',(6.69996174009863,1.23263224516912,3.30617065118014));
#146835=CARTESIAN_POINT('Ctrl Pts',(6.67433849417783,1.22830577227737,3.29325095419084));
#146836=CARTESIAN_POINT('Ctrl Pts',(6.6487296941165,1.22391046498266,3.28032621653173));
#146837=CARTESIAN_POINT('Ctrl Pts',(6.6243212678066,1.21972118106638,3.26800730639257));
#146838=CARTESIAN_POINT('Ctrl Pts',(6.59993026376815,1.21547100862723,3.25567438769194));
#146839=CARTESIAN_POINT('Ctrl Pts',(6.57554203423745,1.21115091650354,3.24336065608557));
#146840=CARTESIAN_POINT('Ctrl Pts',(6.55115319241728,1.20683071591987,3.23104661533138));
#146841=CARTESIAN_POINT('Ctrl Pts',(6.52676392411201,1.20243940506709,3.21875810912996));
#146842=CARTESIAN_POINT('Ctrl Pts',(6.50237471819508,1.1979731744789,3.2064969933566));
#146843=CARTESIAN_POINT('Ctrl Pts',(6.61214067371343,1.197203562,3.54081050413872));
#146844=CARTESIAN_POINT('Ctrl Pts',(6.80386225587355,1.261925886,3.18278793553475));
#146845=CARTESIAN_POINT('Ctrl Pts',(6.95580512444779,1.327100493,2.80615722777762));
#146846=CARTESIAN_POINT('Ctrl Pts',(6.96101880035735,1.32933685513807,2.79323374893157));
#146847=CARTESIAN_POINT('Ctrl Pts',(6.96623247626691,1.33157321727617,2.78031027008552));
#146848=CARTESIAN_POINT('Ctrl Pts',(6.500308946,1.197203562,3.210682731));
#146849=CARTESIAN_POINT('Ctrl Pts',(6.67415535,1.261925886,2.85871543));
#146850=CARTESIAN_POINT('Ctrl Pts',(6.80898137100001,1.327100493,2.490034677));
#146851=CARTESIAN_POINT('Ctrl Pts',(6.81360770973021,1.32933685513807,2.47738398810445));
#146852=CARTESIAN_POINT('Ctrl Pts',(6.81823404846052,1.33157321727617,2.46473329920893));
#146853=CARTESIAN_POINT('Origin',(-0.187113963710771,1.33927926563982,-0.0662433586541727));
#146854=CARTESIAN_POINT('Ctrl Pts',(7.12187882321818,1.32841655815206,2.35136351863108));
#146855=CARTESIAN_POINT('Ctrl Pts',(7.12317067960909,1.32775852557603,2.34743616731554));
#146856=CARTESIAN_POINT('Ctrl Pts',(7.124462536,1.327100493,2.343508816));
#146857=CARTESIAN_POINT('Ctrl Pts',(7.236144887,1.270212881,2.003985142));
#146858=CARTESIAN_POINT('Ctrl Pts',(7.315033724,1.214285714,1.655379601));
#146859=CARTESIAN_POINT('Ctrl Pts',(7.327061562,1.205758742,1.602229227));
#146860=CARTESIAN_POINT('Ctrl Pts',(7.3383158,1.197204389,1.548909688));
#146861=CARTESIAN_POINT('Ctrl Pts',(6.80623611384359,1.32841655815206,2.49754156239315));
#146862=CARTESIAN_POINT('Ctrl Pts',(6.8076087424218,1.32775852557603,2.49378811969658));
#146863=CARTESIAN_POINT('Ctrl Pts',(6.808981371,1.327100493,2.490034677));
#146864=CARTESIAN_POINT('Ctrl Pts',(6.927646563,1.270212881,2.165545587));
#146865=CARTESIAN_POINT('Ctrl Pts',(7.014916327,1.214285714,1.831242452));
#146866=CARTESIAN_POINT('Ctrl Pts',(7.02822197,1.205758742,1.780272704));
#146867=CARTESIAN_POINT('Ctrl Pts',(7.040785563,1.197204389,1.729114993));
#146868=CARTESIAN_POINT('',(7.03965488487991,1.1979731743181,1.73371252044924));
#146869=CARTESIAN_POINT('Ctrl Pts',(7.03965488692215,1.19797317452205,1.73371252091809));
#146870=CARTESIAN_POINT('Ctrl Pts',(7.00820159908294,1.21932945201026,1.86142703754406));
#146871=CARTESIAN_POINT('Ctrl Pts',(6.97328608937065,1.24060037606359,1.98824191820624));
#146872=CARTESIAN_POINT('Ctrl Pts',(6.91565362742755,1.27286181119524,2.17729024714639));
#146873=CARTESIAN_POINT('Ctrl Pts',(6.89554307007011,1.28366386197295,2.24016574396921));
#146874=CARTESIAN_POINT('Ctrl Pts',(6.86407752069048,1.29991103403137,2.33410213484067));
#146875=CARTESIAN_POINT('Ctrl Pts',(6.85336286270133,1.30533866133473,2.36537742066021));
#146876=CARTESIAN_POINT('Ctrl Pts',(6.83696675098894,1.31349012125373,2.41218973157219));
#146877=CARTESIAN_POINT('Ctrl Pts',(6.83144517969175,1.31620998869666,2.42778302154494));
#146878=CARTESIAN_POINT('Ctrl Pts',(6.82308191887862,1.32029216629291,2.45114699715551));
#146879=CARTESIAN_POINT('Ctrl Pts',(6.82028016025447,1.32165353796822,2.45893208693062));
#146880=CARTESIAN_POINT('Ctrl Pts',(6.81477856866167,1.32431471600427,2.47413730936304));
#146881=CARTESIAN_POINT('Ctrl Pts',(6.81341627267494,1.32497441974609,2.47790747414497));
#146882=CARTESIAN_POINT('Ctrl Pts',(6.80898137350066,1.32710049247487,2.49003467335198));
#146883=CARTESIAN_POINT('Ctrl Pts',(7.28186273349879,1.2368931917972,1.79568235830491));
#146884=CARTESIAN_POINT('Ctrl Pts',(7.25404931831883,1.23263224510378,1.78858049393525));
#146885=CARTESIAN_POINT('Ctrl Pts',(7.22624777665621,1.22830577220772,1.78147109270522));
#146886=CARTESIAN_POINT('Ctrl Pts',(7.19845925952399,1.22391046491094,1.77435366321102));
#146887=CARTESIAN_POINT('Ctrl Pts',(7.17197328713478,1.21972118100095,1.7675698524676));
#146888=CARTESIAN_POINT('Ctrl Pts',(7.14550131827908,1.21547100857743,1.76076861535022));
#146889=CARTESIAN_POINT('Ctrl Pts',(7.1190361837065,1.21115091645946,1.75398552037589));
#146890=CARTESIAN_POINT('Ctrl Pts',(7.09257038470169,1.20683071588149,1.74720225510554));
#146891=CARTESIAN_POINT('Ctrl Pts',(7.06610965831957,1.20243940500907,1.74044401924816));
#146892=CARTESIAN_POINT('Ctrl Pts',(7.0396548826297,1.19797317480768,1.73371252114897));
#146893=CARTESIAN_POINT('Ctrl Pts',(7.21872209223307,1.197203562,2.03661353051043));
#146894=CARTESIAN_POINT('Ctrl Pts',(7.32899706144694,1.261925886,1.64574685777119));
#146895=CARTESIAN_POINT('Ctrl Pts',(7.39642312066681,1.327100493,1.24525834149977));
#146896=CARTESIAN_POINT('Ctrl Pts',(7.39873673783603,1.32933685519434,1.23151621986247));
#146897=CARTESIAN_POINT('Ctrl Pts',(7.40105035500526,1.3315732173887,1.2177740982252));
#146898=CARTESIAN_POINT('Ctrl Pts',(7.038537216,1.197203562,1.738244478));
#146899=CARTESIAN_POINT('Ctrl Pts',(7.132656622,1.261925886,1.357134138));
#146900=CARTESIAN_POINT('Ctrl Pts',(7.185075021,1.327100493,0.968089328));
#146901=CARTESIAN_POINT('Ctrl Pts',(7.18687367435913,1.32933685519434,0.954739878804423));
#146902=CARTESIAN_POINT('Ctrl Pts',(7.1886723277183,1.3315732173887,0.941390429608839));
#146903=CARTESIAN_POINT('Origin',(-0.196980054139005,1.33927934730507,-0.0244706883502453));
#146904=CARTESIAN_POINT('Ctrl Pts',(7.46084690487036,1.32841655815206,0.765396519891663));
#146905=CARTESIAN_POINT('Ctrl Pts',(7.46126429393518,1.32775852557603,0.761283276945831));
#146906=CARTESIAN_POINT('Ctrl Pts',(7.46168168300001,1.327100493,0.757170034));
#146907=CARTESIAN_POINT('Ctrl Pts',(7.497765409,1.270212881,0.401575832));
#146908=CARTESIAN_POINT('Ctrl Pts',(7.499869982,1.214285714,0.044161726));
#146909=CARTESIAN_POINT('Ctrl Pts',(7.500190857,1.205758742,-0.010331651));
#146910=CARTESIAN_POINT('Ctrl Pts',(7.499719852,1.197204389,-0.064823938));
#146911=CARTESIAN_POINT('Ctrl Pts',(7.18400770487019,1.32841655815206,0.976010855747787));
#146912=CARTESIAN_POINT('Ctrl Pts',(7.18454136293509,1.32775852557603,0.972050091873894));
#146913=CARTESIAN_POINT('Ctrl Pts',(7.185075021,1.327100493,0.968089328));
#146914=CARTESIAN_POINT('Ctrl Pts',(7.23121032499999,1.270212881,0.625677103));
#146915=CARTESIAN_POINT('Ctrl Pts',(7.244574478,1.214285714,0.28042937));
#146916=CARTESIAN_POINT('Ctrl Pts',(7.246612053,1.205758742,0.227790947));
#146917=CARTESIAN_POINT('Ctrl Pts',(7.24788452,1.197204389,0.175128473));
#146918=CARTESIAN_POINT('',(7.24776860911715,1.19797317432174,0.179861575560411));
#146919=CARTESIAN_POINT('Ctrl Pts',(7.24776861100016,1.19797317454899,0.179861575570232));
#146920=CARTESIAN_POINT('Ctrl Pts',(7.24450553215528,1.21932945234802,0.311351727067775));
#146921=CARTESIAN_POINT('Ctrl Pts',(7.23766777176235,1.24060038425565,0.442707597301654));
#146922=CARTESIAN_POINT('Ctrl Pts',(7.2220225334039,1.27286180664125,0.639725279379605));
#146923=CARTESIAN_POINT('Ctrl Pts',(7.21589852742869,1.2836638529123,0.705453929640085));
#146924=CARTESIAN_POINT('Ctrl Pts',(7.20536216651482,1.29991103405708,0.803958358085943));
#146925=CARTESIAN_POINT('Ctrl Pts',(7.20162127323419,1.30533866136434,0.836805779906436));
#146926=CARTESIAN_POINT('Ctrl Pts',(7.19567175659462,1.31349012127948,0.886048324387821));
#146927=CARTESIAN_POINT('Ctrl Pts',(7.193631372977,1.31620998872371,0.902464026545407));
#146928=CARTESIAN_POINT('Ctrl Pts',(7.19048620468116,1.32029216631906,0.927079619271783));
#146929=CARTESIAN_POINT('Ctrl Pts',(7.189423513794,1.32165353799468,0.93528499327062));
#146930=CARTESIAN_POINT('Ctrl Pts',(7.18731921972352,1.32431471602432,0.951317405599425));
#146931=CARTESIAN_POINT('Ctrl Pts',(7.18679924745915,1.32497441974746,0.955292279283956));
#146932=CARTESIAN_POINT('Ctrl Pts',(7.18507502309713,1.32710049250219,0.968089323712349));
#146933=CARTESIAN_POINT('Ctrl Pts',(7.49763545644904,1.2368931917972,0.188315065585089));
#146934=CARTESIAN_POINT('Ctrl Pts',(7.4689456126465,1.23263224513807,0.187358300905372));
#146935=CARTESIAN_POINT('Ctrl Pts',(7.44026574456447,1.22830577226035,0.18639162315998));
#146936=CARTESIAN_POINT('Ctrl Pts',(7.41159687066663,1.22391046498252,0.185414304967323));
#146937=CARTESIAN_POINT('Ctrl Pts',(7.38427180671392,1.21972118106134,0.184482797081394));
#146938=CARTESIAN_POINT('Ctrl Pts',(7.35695667274409,1.21547100862243,0.183531259927491));
#146939=CARTESIAN_POINT('Ctrl Pts',(7.32965211329941,1.21115091648452,0.182595971637373));
#146940=CARTESIAN_POINT('Ctrl Pts',(7.3023468683482,1.20683071588664,0.181660659865967));
#146941=CARTESIAN_POINT('Ctrl Pts',(7.27505195801014,1.20243940502776,0.18074870167642));
#146942=CARTESIAN_POINT('Ctrl Pts',(7.24776860697027,1.19797317480768,0.179861576786875));
#146943=CARTESIAN_POINT('Ctrl Pts',(7.48749265123569,1.197203562,0.436901152368877));
#146944=CARTESIAN_POINT('Ctrl Pts',(7.51114920656008,1.261925886,0.0314815633877653));
#146945=CARTESIAN_POINT('Ctrl Pts',(7.49089190176009,1.327100493,-0.374122082468887));
#146946=CARTESIAN_POINT('Ctrl Pts',(7.4905840950171,1.32809081149028,-0.38028516973106));
#146947=CARTESIAN_POINT('Ctrl Pts',(7.49027628827411,1.32908112998057,-0.38644825699323));
#146948=CARTESIAN_POINT('Ctrl Pts',(7.247651307,1.197203562,0.184527844));
#146949=CARTESIAN_POINT('Ctrl Pts',(7.257642797,1.261925886,-0.207905238));
#146950=CARTESIAN_POINT('Ctrl Pts',(7.225202548,1.327100493,-0.599122803));
#146951=CARTESIAN_POINT('Ctrl Pts',(7.22470962322619,1.32809081149028,-0.605067295896501));
#146952=CARTESIAN_POINT('Ctrl Pts',(7.22421669845237,1.32908112998057,-0.611011788792999));
#146953=CARTESIAN_POINT('Origin',(-0.19763521706426,1.33927931706354,0.0184463046920125));
#146954=CARTESIAN_POINT('Ctrl Pts',(7.45095407682186,1.32841655815206,-0.856359568123177));
#146955=CARTESIAN_POINT('Ctrl Pts',(7.45047748191093,1.32775852557603,-0.860466372061588));
#146956=CARTESIAN_POINT('Ctrl Pts',(7.450000887,1.327100493,-0.864573176));
#146957=CARTESIAN_POINT('Ctrl Pts',(7.408798753,1.270212881,-1.219610719));
#146958=CARTESIAN_POINT('Ctrl Pts',(7.334020655,1.214285714,-1.569121102));
#146959=CARTESIAN_POINT('Ctrl Pts',(7.32261956300001,1.205758742,-1.622409433));
#146960=CARTESIAN_POINT('Ctrl Pts',(7.31044533900001,1.197204389,-1.675526468));
#146961=CARTESIAN_POINT('Ctrl Pts',(7.22586307942343,1.32841655815206,-0.591157034752268));
#146962=CARTESIAN_POINT('Ctrl Pts',(7.22553281371171,1.32775852557603,-0.595139918876134));
#146963=CARTESIAN_POINT('Ctrl Pts',(7.225202548,1.327100493,-0.599122803));
#146964=CARTESIAN_POINT('Ctrl Pts',(7.196650728,1.270212881,-0.943447347));
#146965=CARTESIAN_POINT('Ctrl Pts',(7.135484378,1.214285714,-1.283496277));
#146966=CARTESIAN_POINT('Ctrl Pts',(7.12615861,1.205758742,-1.335342062));
#146967=CARTESIAN_POINT('Ctrl Pts',(7.11608045300001,1.197204389,-1.387046859));
#146968=CARTESIAN_POINT('',(7.11698472862996,1.19797317408571,-1.3823994984479));
#146969=CARTESIAN_POINT('Ctrl Pts',(7.11698472875213,1.19797317391247,-1.382399498443));
#146970=CARTESIAN_POINT('Ctrl Pts',(7.12338474596396,1.2034230201217,-1.34945039439011));
#146971=CARTESIAN_POINT('Ctrl Pts',(7.12955124253131,1.20886077956071,-1.31648102053784));
#146972=CARTESIAN_POINT('Ctrl Pts',(7.13548437798228,1.21428571393588,-1.28349627746525));
#146973=CARTESIAN_POINT('Ctrl Pts',(7.16162230994452,1.23818480996542,-1.13818475088076));
#146974=CARTESIAN_POINT('Ctrl Pts',(7.18340750111566,1.26233313349311,-0.991572763403286));
#146975=CARTESIAN_POINT('Ctrl Pts',(7.20069910446844,1.2866659590878,-0.844057114460819));
#146976=CARTESIAN_POINT('Ctrl Pts',(7.21023990727024,1.3000918216798,-0.762663984626208));
#146977=CARTESIAN_POINT('Ctrl Pts',(7.21841350827149,1.31357377941461,-0.680996155908423));
#146978=CARTESIAN_POINT('Ctrl Pts',(7.22520254822916,1.32710049187612,-0.599122810739174));
#146979=CARTESIAN_POINT('Ctrl Pts',(7.36282707779834,1.23689319343748,-1.42785763095411));
#146980=CARTESIAN_POINT('Ctrl Pts',(7.33460231089359,1.23263224513027,-1.4226245583736));
#146981=CARTESIAN_POINT('Ctrl Pts',(7.30638515505452,1.22830577224184,-1.41740331178869));
#146982=CARTESIAN_POINT('Ctrl Pts',(7.27817644809364,1.2239104648102,-1.41219482011437));
#146983=CARTESIAN_POINT('Ctrl Pts',(7.25781973847191,1.22073860736887,-1.40843613125535));
#146984=CARTESIAN_POINT('Ctrl Pts',(7.23746645327191,1.21753001354952,-1.40468964664207));
#146985=CARTESIAN_POINT('Ctrl Pts',(7.21711934827861,1.214285714,-1.40094067785228));
#146986=CARTESIAN_POINT('Ctrl Pts',(7.21059267427628,1.21324505074959,-1.39973813346226));
#146987=CARTESIAN_POINT('Ctrl Pts',(7.20406674565574,1.21220011142664,-1.39853525699594));
#146988=CARTESIAN_POINT('Ctrl Pts',(7.19754166102725,1.21115091721806,-1.39733156272361));
#146989=CARTESIAN_POINT('Ctrl Pts',(7.17067372867402,1.2068307159293,-1.39237518619758));
#146990=CARTESIAN_POINT('Ctrl Pts',(7.14382091425827,1.20243940509642,-1.38739822438772));
#146991=CARTESIAN_POINT('Ctrl Pts',(7.11698472848221,1.19797317368262,-1.38239949983265));
#146992=CARTESIAN_POINT('Ctrl Pts',(7.40668655768148,1.197203562,-1.1826823537903));
#146993=CARTESIAN_POINT('Ctrl Pts',(7.34264875278482,1.261925886,-1.58372659622297));
#146994=CARTESIAN_POINT('Ctrl Pts',(7.23568222365081,1.327100493,-1.9755115968509));
#146995=CARTESIAN_POINT('Ctrl Pts',(7.23201183866211,1.32933685516968,-1.9889550711484));
#146996=CARTESIAN_POINT('Ctrl Pts',(7.22834145367339,1.33157321733938,-2.00239854544585));
#146997=CARTESIAN_POINT('Ctrl Pts',(7.117873279,1.197203562,-1.377817106));
#146998=CARTESIAN_POINT('Ctrl Pts',(7.043269661,1.261925886,-1.763223196));
#146999=CARTESIAN_POINT('Ctrl Pts',(6.927487635,1.327100493,-2.138320617));
#147000=CARTESIAN_POINT('Ctrl Pts',(6.92351476036686,1.32933685516968,-2.15119148375138));
#147001=CARTESIAN_POINT('Ctrl Pts',(6.91954188573374,1.33157321733938,-2.16406235050276));
#147002=CARTESIAN_POINT('Origin',(-0.189049009225389,1.3392792235055,0.0605006924093482));
#147003=CARTESIAN_POINT('Ctrl Pts',(7.09266291765338,1.32841655815206,-2.43807323536181));
#147004=CARTESIAN_POINT('Ctrl Pts',(7.09131462382669,1.32775852557603,-2.4419815706809));
#147005=CARTESIAN_POINT('Ctrl Pts',(7.08996633,1.327100493,-2.445889906));
#147006=CARTESIAN_POINT('Ctrl Pts',(6.973404903,1.270212881,-2.783769627));
#147007=CARTESIAN_POINT('Ctrl Pts',(6.825240674,1.214285714,-3.109033571));
#147008=CARTESIAN_POINT('Ctrl Pts',(6.802650717,1.205758742,-3.158625153));
#147009=CARTESIAN_POINT('Ctrl Pts',(6.779342527,1.197204389,-3.207883243));
#147010=CARTESIAN_POINT('Ctrl Pts',(6.92984512827001,1.32841655815206,-2.13068307872255));
#147011=CARTESIAN_POINT('Ctrl Pts',(6.928666381635,1.32775852557603,-2.13450184786127));
#147012=CARTESIAN_POINT('Ctrl Pts',(6.92748763500001,1.327100493,-2.138320617));
#147013=CARTESIAN_POINT('Ctrl Pts',(6.825583742,1.270212881,-2.468457247));
#147014=CARTESIAN_POINT('Ctrl Pts',(6.692746959,1.214285714,-2.787407065));
#147015=CARTESIAN_POINT('Ctrl Pts',(6.672493911,1.205758742,-2.83603596));
#147016=CARTESIAN_POINT('Ctrl Pts',(6.651536372,1.197204389,-2.884365422));
#147017=CARTESIAN_POINT('',(6.65341855209195,1.19797317421024,-2.88002110567815));
#147018=CARTESIAN_POINT('Ctrl Pts',(6.65341855208966,1.19797317415461,-2.88002110531445));
#147019=CARTESIAN_POINT('Ctrl Pts',(6.66675202366146,1.20342302010153,-2.84921814883435));
#147020=CARTESIAN_POINT('Ctrl Pts',(6.67986179183559,1.20886077946157,-2.8183451954448));
#147021=CARTESIAN_POINT('Ctrl Pts',(6.69274695873651,1.21428571388907,-2.78740706563265));
#147022=CARTESIAN_POINT('Ctrl Pts',(6.74951147156,1.23818480505845,-2.65111175178807));
#147023=CARTESIAN_POINT('Ctrl Pts',(6.80230457076466,1.26233312370905,-2.51261067121566));
#147024=CARTESIAN_POINT('Ctrl Pts',(6.85090340211003,1.28666594441934,-2.37226106832997));
#147025=CARTESIAN_POINT('Ctrl Pts',(6.87771827383148,1.30009181183023,-2.29482182764554));
#147026=CARTESIAN_POINT('Ctrl Pts',(6.90325695945089,1.31357377444449,-2.21682040196567));
#147027=CARTESIAN_POINT('Ctrl Pts',(6.92748763334545,1.32710049182833,-2.13832062464059));
#147028=CARTESIAN_POINT('Ctrl Pts',(6.88374108930052,1.2368931934011,-2.97726529110107));
#147029=CARTESIAN_POINT('Ctrl Pts',(6.85730115750648,1.23263224506685,-2.96608707433597));
#147030=CARTESIAN_POINT('Ctrl Pts',(6.83086611675,1.22830577218589,-2.95492204319668));
#147031=CARTESIAN_POINT('Ctrl Pts',(6.80443658539514,1.22391046475872,-2.94377128502051));
#147032=CARTESIAN_POINT('Ctrl Pts',(6.78536381140319,1.22073860733689,-2.93572438143839));
#147033=CARTESIAN_POINT('Ctrl Pts',(6.76629175820736,1.21753001353641,-2.92769013290503));
#147034=CARTESIAN_POINT('Ctrl Pts',(6.74722627473991,1.214285714,-2.9196547868689));
#147035=CARTESIAN_POINT('Ctrl Pts',(6.74111070209017,1.21324505072843,-2.9170773152643));
#147036=CARTESIAN_POINT('Ctrl Pts',(6.73499592878081,1.21220011138391,-2.91449967958569));
#147037=CARTESIAN_POINT('Ctrl Pts',(6.72888215553346,1.21115091715362,-2.91192142665918));
#147038=CARTESIAN_POINT('Ctrl Pts',(6.70370785482671,1.20683071586637,-2.90130511626558));
#147039=CARTESIAN_POINT('Ctrl Pts',(6.67855274380652,1.20243940503684,-2.89067195182176));
#147040=CARTESIAN_POINT('Ctrl Pts',(6.65341855208966,1.19797317415461,-2.88002110531445));
#147041=CARTESIAN_POINT('Ctrl Pts',(6.97928059608386,1.197203562,-2.74725056763781));
#147042=CARTESIAN_POINT('Ctrl Pts',(6.8305273023256,1.261925886,-3.12515238362192));
#147043=CARTESIAN_POINT('Ctrl Pts',(6.64183939663927,1.327100493,-3.48478302660899));
#147044=CARTESIAN_POINT('Ctrl Pts',(6.63536487355604,1.32933685518721,-3.49712317576157));
#147045=CARTESIAN_POINT('Ctrl Pts',(6.62889035047272,1.33157321737445,-3.50946332491413));
#147046=CARTESIAN_POINT('Ctrl Pts',(6.655271408,1.197203562,-2.87573686));
#147047=CARTESIAN_POINT('Ctrl Pts',(6.49956106400001,1.261925886,-3.236094797));
#147048=CARTESIAN_POINT('Ctrl Pts',(6.30585110000001,1.327100493,-3.577532936));
#147049=CARTESIAN_POINT('Ctrl Pts',(6.29920425303431,1.32933685518721,-3.58924883853445));
#147050=CARTESIAN_POINT('Ctrl Pts',(6.29255740606874,1.33157321737445,-3.6009647410689));
#147051=CARTESIAN_POINT('Origin',(-0.171623641713373,1.33927930011166,0.0997263771225571));
#147052=CARTESIAN_POINT('Ctrl Pts',(6.40272672408439,1.32841655815206,-3.90578530842664));
#147053=CARTESIAN_POINT('Ctrl Pts',(6.40056977604219,1.32775852557603,-3.90931242571332));
#147054=CARTESIAN_POINT('Ctrl Pts',(6.398412828,1.327100493,-3.912839543));
#147055=CARTESIAN_POINT('Ctrl Pts',(6.211942389,1.270212881,-4.217762562));
#147056=CARTESIAN_POINT('Ctrl Pts',(5.997320024,1.214285714,-4.503571086));
#147057=CARTESIAN_POINT('Ctrl Pts',(5.964597484,1.205758742,-4.547147072));
#147058=CARTESIAN_POINT('Ctrl Pts',(5.931245193,1.197204389,-4.590242963));
#147059=CARTESIAN_POINT('Ctrl Pts',(6.30979532136945,1.32841655815206,-3.57058075049654));
#147060=CARTESIAN_POINT('Ctrl Pts',(6.30782321068472,1.32775852557603,-3.57405684324827));
#147061=CARTESIAN_POINT('Ctrl Pts',(6.3058511,1.327100493,-3.577532936));
#147062=CARTESIAN_POINT('Ctrl Pts',(6.135360046,1.270212881,-3.87804483));
#147063=CARTESIAN_POINT('Ctrl Pts',(5.93706413,1.214285714,-4.160981797));
#147064=CARTESIAN_POINT('Ctrl Pts',(5.906830812,1.205758742,-4.204119968));
#147065=CARTESIAN_POINT('Ctrl Pts',(5.875973844,1.197204389,-4.246814263));
#147066=CARTESIAN_POINT('',(5.87874591871806,1.19797317422931,-4.24297612677607));
#147067=CARTESIAN_POINT('Ctrl Pts',(5.87874592077807,1.19797317443603,-4.24297612830428));
#147068=CARTESIAN_POINT('Ctrl Pts',(5.95572268929811,1.21932946232458,-4.1363229488652));
#147069=CARTESIAN_POINT('Ctrl Pts',(6.02977236921766,1.24060039083117,-4.02761342976386));
#147070=CARTESIAN_POINT('Ctrl Pts',(6.13654727984032,1.27286179973307,-3.86130099382886));
#147071=CARTESIAN_POINT('Ctrl Pts',(6.17144926667873,1.28366383961176,-3.80526881585095));
#147072=CARTESIAN_POINT('Ctrl Pts',(6.22267372412087,1.29991103381881,-3.72047372114034));
#147073=CARTESIAN_POINT('Ctrl Pts',(6.23957403768495,1.30533866114673,-3.69206022407433));
#147074=CARTESIAN_POINT('Ctrl Pts',(6.26463798703239,1.3134901210992,-3.6492580815018));
#147075=CARTESIAN_POINT('Ctrl Pts',(6.27294801147348,1.31620998855437,-3.63495486719273));
#147076=CARTESIAN_POINT('Ctrl Pts',(6.28534088684618,1.32029216616772,-3.61345518960003));
#147077=CARTESIAN_POINT('Ctrl Pts',(6.28946056677987,1.32165353784895,-3.60627983508245));
#147078=CARTESIAN_POINT('Ctrl Pts',(6.29748775538821,1.32431471587585,-3.5922430782577));
#147079=CARTESIAN_POINT('Ctrl Pts',(6.2994792991663,1.32497441927737,-3.58876403675979));
#147080=CARTESIAN_POINT('Ctrl Pts',(6.3058510974985,1.32710049205904,-3.57753294212463));
#147081=CARTESIAN_POINT('Ctrl Pts',(6.08277901777997,1.23689319179776,-4.38745933517958));
#147082=CARTESIAN_POINT('Ctrl Pts',(6.05936022279369,1.23263224511165,-4.37085865528992));
#147083=CARTESIAN_POINT('Ctrl Pts',(6.03594337023099,1.2283057722232,-4.35427190405315));
#147084=CARTESIAN_POINT('Ctrl Pts',(6.01252883073701,1.22391046493218,-4.33770027700123));
#147085=CARTESIAN_POINT('Ctrl Pts',(5.99021181229749,1.21972118100941,-4.32190541985337));
#147086=CARTESIAN_POINT('Ctrl Pts',(5.96789057786927,1.21547100856215,-4.30613251721398));
#147087=CARTESIAN_POINT('Ctrl Pts',(5.94558759502441,1.21115091644438,-4.2903530785531));
#147088=CARTESIAN_POINT('Ctrl Pts',(5.92328405224218,1.20683071586663,-4.27457324373457));
#147089=CARTESIAN_POINT('Ctrl Pts',(5.90100286981086,1.20243940501135,-4.25878107146338));
#147090=CARTESIAN_POINT('Ctrl Pts',(5.87874591645608,1.19797317447863,-4.24297612382197));
#147091=CARTESIAN_POINT('Ctrl Pts',(6.22553122981399,1.197203562,-4.18336039794212));
#147092=CARTESIAN_POINT('Ctrl Pts',(5.99901798618057,1.261925886,-4.52044951809398));
#147093=CARTESIAN_POINT('Ctrl Pts',(5.73743154150362,1.327100493,-4.83110987552457));
#147094=CARTESIAN_POINT('Ctrl Pts',(5.72845562219651,1.32933685510976,-4.84176968744128));
#147095=CARTESIAN_POINT('Ctrl Pts',(5.7194797028895,1.33157321721954,-4.85242949935788));
#147096=CARTESIAN_POINT('Ctrl Pts',(5.881476442,1.197203562,-4.239190355));
#147097=CARTESIAN_POINT('Ctrl Pts',(5.651940215,1.261925886,-4.557650202));
#147098=CARTESIAN_POINT('Ctrl Pts',(5.389359975,1.327100493,-4.84946379100001));
#147099=CARTESIAN_POINT('Ctrl Pts',(5.3803499552003,1.32933685510976,-4.85947690628512));
#147100=CARTESIAN_POINT('Ctrl Pts',(5.37133993540046,1.33157321721954,-4.86949002157024));
#147101=CARTESIAN_POINT('Origin',(-0.146172789174652,1.3392792791228,0.134288671367934));
#147102=CARTESIAN_POINT('Ctrl Pts',(5.41340614349393,1.32841655815206,-5.19086720064895));
#147103=CARTESIAN_POINT('Ctrl Pts',(5.41054139774696,1.32775852557603,-5.19384817582447));
#147104=CARTESIAN_POINT('Ctrl Pts',(5.407676652,1.327100493,-5.196829151));
#147105=CARTESIAN_POINT('Ctrl Pts',(5.160016353,1.270212881,-5.454537607));
#147106=CARTESIAN_POINT('Ctrl Pts',(4.888971356,1.214285714,-5.687526623));
#147107=CARTESIAN_POINT('Ctrl Pts',(4.847646301,1.205758742,-5.723049447));
#147108=CARTESIAN_POINT('Ctrl Pts',(4.805809426,1.197204389,-5.75796802300001));
#147109=CARTESIAN_POINT('Ctrl Pts',(5.3947064970428,1.32841655815206,-4.84352203473393));
#147110=CARTESIAN_POINT('Ctrl Pts',(5.3920332360214,1.32775852557603,-4.84649291286696));
#147111=CARTESIAN_POINT('Ctrl Pts',(5.389359975,1.327100493,-4.849463791));
#147112=CARTESIAN_POINT('Ctrl Pts',(5.158253733,1.270212881,-5.106299347));
#147113=CARTESIAN_POINT('Ctrl Pts',(4.903770781,1.214285714,-5.339993645));
#147114=CARTESIAN_POINT('Ctrl Pts',(4.86497087,1.205758742,-5.37562400000001));
#147115=CARTESIAN_POINT('Ctrl Pts',(4.825657309,1.197204389,-5.41068678999999));
#147116=CARTESIAN_POINT('',(4.82918966005797,1.19797317413119,-5.40753430064078));
#147117=CARTESIAN_POINT('Ctrl Pts',(4.82918965923873,1.1979731744789,-5.40753429774621));
#147118=CARTESIAN_POINT('Ctrl Pts',(4.866714564,1.20614195,-5.374022748));
#147119=CARTESIAN_POINT('Ctrl Pts',(4.903770781,1.214285714,-5.339993645));
#147120=CARTESIAN_POINT('Ctrl Pts',(5.1582537310117,1.2702128801536,-5.10629934886565));
#147121=CARTESIAN_POINT('Ctrl Pts',(5.38935996966452,1.32710049490569,-4.8494637968944));
#147122=CARTESIAN_POINT('Ctrl Pts',(4.99739295987831,1.2368931917972,-5.59250065744889));
#147123=CARTESIAN_POINT('Ctrl Pts',(4.97809033885803,1.23263224511286,-5.57125374342456));
#147124=CARTESIAN_POINT('Ctrl Pts',(4.95878662051537,1.2283057722275,-5.55002085012779));
#147125=CARTESIAN_POINT('Ctrl Pts',(4.93948190990829,1.22391046494225,-5.52880322466368));
#147126=CARTESIAN_POINT('Ctrl Pts',(4.92108207837026,1.21972118102846,-5.50858014325508));
#147127=CARTESIAN_POINT('Ctrl Pts',(4.90267340981734,1.21547100859722,-5.48837759677755));
#147128=CARTESIAN_POINT('Ctrl Pts',(4.88428397121444,1.21115091649139,-5.46817259061412));
#147129=CARTESIAN_POINT('Ctrl Pts',(4.8658940709274,1.20683071592559,-5.44796707718502));
#147130=CARTESIAN_POINT('Ctrl Pts',(4.84752866049305,1.20243940506542,-5.42775432148555));
#147131=CARTESIAN_POINT('Ctrl Pts',(4.82918965923873,1.1979731744789,-5.40753429774621));
#147132=CARTESIAN_POINT('Ctrl Pts',(5.18068294323111,1.197203562,-5.42386094580908));
#147133=CARTESIAN_POINT('Ctrl Pts',(4.88700125593062,1.261925886,-5.70437545777784));
#147134=CARTESIAN_POINT('Ctrl Pts',(4.56474776398113,1.327100493,-5.9515393946638));
#147135=CARTESIAN_POINT('Ctrl Pts',(4.55369015191196,1.32933685517751,-5.96002042900432));
#147136=CARTESIAN_POINT('Ctrl Pts',(4.54263253984269,1.33157321735505,-5.96850146334481));
#147137=CARTESIAN_POINT('Ctrl Pts',(4.832670174,1.197203562,-5.40442402));
#147138=CARTESIAN_POINT('Ctrl Pts',(4.540040923,1.261925886,-5.66609494900001));
#147139=CARTESIAN_POINT('Ctrl Pts',(4.220868368,1.327100493,-5.894639109));
#147140=CARTESIAN_POINT('Ctrl Pts',(4.20991647334412,1.32933685517751,-5.9024812355404));
#147141=CARTESIAN_POINT('Ctrl Pts',(4.1989645786882,1.33157321735505,-5.91032336208092));
#147142=CARTESIAN_POINT('Origin',(-0.113887131184427,1.33927922518391,0.162571745578474));
#147143=CARTESIAN_POINT('Ctrl Pts',(4.17096070925662,1.32841655815206,-6.23322991204394));
#147144=CARTESIAN_POINT('Ctrl Pts',(4.16752211812831,1.32775852557603,-6.23552535802196));
#147145=CARTESIAN_POINT('Ctrl Pts',(4.164083527,1.327100493,-6.237820804));
#147146=CARTESIAN_POINT('Ctrl Pts',(3.866813688,1.270212881,-6.436264536));
#147147=CARTESIAN_POINT('Ctrl Pts',(3.55201982,1.214285714,-6.605539735));
#147148=CARTESIAN_POINT('Ctrl Pts',(3.504024566,1.205758742,-6.63134839));
#147149=CARTESIAN_POINT('Ctrl Pts',(3.455659352,1.197204389,-6.656456899));
#147150=CARTESIAN_POINT('Ctrl Pts',(4.22736719328812,1.32841655815206,-5.88998561188718));
#147151=CARTESIAN_POINT('Ctrl Pts',(4.22411778064406,1.32775852557603,-5.89231236044358));
#147152=CARTESIAN_POINT('Ctrl Pts',(4.220868368,1.327100493,-5.894639109));
#147153=CARTESIAN_POINT('Ctrl Pts',(3.939953209,1.270212881,-6.095788982));
#147154=CARTESIAN_POINT('Ctrl Pts',(3.641182561,1.214285714,-6.269313324));
#147155=CARTESIAN_POINT('Ctrl Pts',(3.595630297,1.205758742,-6.29576982800001));
#147156=CARTESIAN_POINT('Ctrl Pts',(3.549698402,1.197204389,-6.321561615));
#147157=CARTESIAN_POINT('',(3.55382586037817,1.19797317422833,-6.31924218135152));
#147158=CARTESIAN_POINT('Ctrl Pts',(3.55382586159486,1.19797317443837,-6.31924218358456));
#147159=CARTESIAN_POINT('Ctrl Pts',(3.66847053387572,1.21932945129378,-6.25476811985903));
#147160=CARTESIAN_POINT('Ctrl Pts',(3.78132215100889,1.24060038065143,-6.18719868670361));
#147161=CARTESIAN_POINT('Ctrl Pts',(3.94806130701094,1.27286180742993,-6.08109117049854));
#147162=CARTESIAN_POINT('Ctrl Pts',(4.00326482999537,1.28366385468844,-6.04489267913147));
#147163=CARTESIAN_POINT('Ctrl Pts',(4.08535934885952,1.29991103391507,-5.98944337806926));
#147164=CARTESIAN_POINT('Ctrl Pts',(4.11262817573049,1.3053386612337,-5.97075224407891));
#147165=CARTESIAN_POINT('Ctrl Pts',(4.15334775316636,1.31349012116991,-5.94243015083713));
#147166=CARTESIAN_POINT('Ctrl Pts',(4.16689549086053,1.3162099886202,-5.932938193834));
#147167=CARTESIAN_POINT('Ctrl Pts',(4.18717044018716,1.32029216622577,-5.91862924827255));
#147168=CARTESIAN_POINT('Ctrl Pts',(4.19392221357816,1.32165353790458,-5.91384688160607));
#147169=CARTESIAN_POINT('Ctrl Pts',(4.20710137385622,1.32431471593206,-5.90447799516369));
#147170=CARTESIAN_POINT('Ctrl Pts',(4.21036966344095,1.32497441969706,-5.90215672886456));
#147171=CARTESIAN_POINT('Ctrl Pts',(4.22086836507627,1.32710049245079,-5.89463911222129));
#147172=CARTESIAN_POINT('Ctrl Pts',(3.67833436109359,1.2368931917972,-6.53604286414623));
#147173=CARTESIAN_POINT('Ctrl Pts',(3.66405048306732,1.23263224513278,-6.51114319839324));
#147174=CARTESIAN_POINT('Ctrl Pts',(3.64976251940711,1.2283057722557,-6.48625698950042));
#147175=CARTESIAN_POINT('Ctrl Pts',(3.63547030455459,1.22391046497494,-6.46138547817636));
#147176=CARTESIAN_POINT('Ctrl Pts',(3.6218480156065,1.21972118105975,-6.43767978124078));
#147177=CARTESIAN_POINT('Ctrl Pts',(3.60821268185683,1.21547100862238,-6.41399223943781));
#147178=CARTESIAN_POINT('Ctrl Pts',(3.59459665732802,1.21115091648973,-6.39030642927422));
#147179=CARTESIAN_POINT('Ctrl Pts',(3.58098029095612,1.2068307158971,-6.36662002445609));
#147180=CARTESIAN_POINT('Ctrl Pts',(3.56738939858888,1.20243940503687,-6.34293181137135));
#147181=CARTESIAN_POINT('Ctrl Pts',(3.55382585953398,1.1979731744789,-6.31924217758386));
#147182=CARTESIAN_POINT('Ctrl Pts',(3.89359167974831,1.197203562,-6.41074778369874));
#147183=CARTESIAN_POINT('Ctrl Pts',(3.54647377862539,1.261925886,-6.62157114079826));
#147184=CARTESIAN_POINT('Ctrl Pts',(3.17862145369144,1.327100493,-6.79368154768851));
#147185=CARTESIAN_POINT('Ctrl Pts',(3.16599919117411,1.3293368551031,-6.79958724024633));
#147186=CARTESIAN_POINT('Ctrl Pts',(3.15337692865672,1.33157321720621,-6.80549293280415));
#147187=CARTESIAN_POINT('Ctrl Pts',(3.55789362,1.197203562,-6.316952824));
#147188=CARTESIAN_POINT('Ctrl Pts',(3.215854364,1.261925886,-6.509599393));
#147189=CARTESIAN_POINT('Ctrl Pts',(2.855013647,1.327100493,-6.664187653));
#147190=CARTESIAN_POINT('Ctrl Pts',(2.84263197656271,1.3293368551031,-6.66949210119171));
#147191=CARTESIAN_POINT('Ctrl Pts',(2.83025030612543,1.33157321720621,-6.67479654938358));
#147192=CARTESIAN_POINT('Origin',(-0.0762763624267304,1.33927926043528,
0.183253217390437));
#147193=CARTESIAN_POINT('Ctrl Pts',(2.7334857876269,1.32841655815206,-6.98413372045931));
#147194=CARTESIAN_POINT('Ctrl Pts',(2.72963413581345,1.32775852557603,-6.98563630472966));
#147195=CARTESIAN_POINT('Ctrl Pts',(2.725782484,1.327100493,-6.987138889));
#147196=CARTESIAN_POINT('Ctrl Pts',(2.392803112,1.270212881,-7.117038888));
#147197=CARTESIAN_POINT('Ctrl Pts',(2.048979786,1.214285714,-7.214685152));
#147198=CARTESIAN_POINT('Ctrl Pts',(1.996558536,1.205758742,-7.229572853));
#147199=CARTESIAN_POINT('Ctrl Pts',(1.943926487,1.197204389,-7.243697248));
#147200=CARTESIAN_POINT('Ctrl Pts',(2.8623608976771,1.32841655815206,-6.661040007405));
#147201=CARTESIAN_POINT('Ctrl Pts',(2.85868727233855,1.32775852557603,-6.6626138302025));
#147202=CARTESIAN_POINT('Ctrl Pts',(2.855013647,1.327100493,-6.664187653));
#147203=CARTESIAN_POINT('Ctrl Pts',(2.537424852,1.270212881,-6.800246298));
#147204=CARTESIAN_POINT('Ctrl Pts',(2.208336691,1.214285714,-6.905486881));
#147205=CARTESIAN_POINT('Ctrl Pts',(2.158162048,1.205758742,-6.921532455));
#147206=CARTESIAN_POINT('Ctrl Pts',(2.107759543,1.197204389,-6.936847246));
#147207=CARTESIAN_POINT('',(2.11228911222365,1.19797317414004,-6.93546932052256));
#147208=CARTESIAN_POINT('Ctrl Pts',(2.11228911319232,1.1979731744789,-6.9354693168474));
#147209=CARTESIAN_POINT('Ctrl Pts',(2.16041693,1.20614195,-6.920811357));
#147210=CARTESIAN_POINT('Ctrl Pts',(2.208336691,1.214285714,-6.905486881));
#147211=CARTESIAN_POINT('Ctrl Pts',(2.53742484868758,1.27021288015463,-6.80024629937446));
#147212=CARTESIAN_POINT('Ctrl Pts',(2.85501363945865,1.32710049475556,-6.66418765610293));
#147213=CARTESIAN_POINT('Ctrl Pts',(2.1872809358002,1.23689319341796,-7.17396697109652));
#147214=CARTESIAN_POINT('Ctrl Pts',(2.17868369939942,1.23263224510868,-7.1465788341424));
#147215=CARTESIAN_POINT('Ctrl Pts',(2.17007957965209,1.22830577222041,-7.11920296110771));
#147216=CARTESIAN_POINT('Ctrl Pts',(2.16146814827954,1.22391046478458,-7.09184052727123));
#147217=CARTESIAN_POINT('Ctrl Pts',(2.15525374053095,1.22073860735404,-7.07209452762292));
#147218=CARTESIAN_POINT('Ctrl Pts',(2.14903015416926,1.21753001353903,-7.05235727007206));
#147219=CARTESIAN_POINT('Ctrl Pts',(2.14281165749886,1.214285714,-7.03262430918844));
#147220=CARTESIAN_POINT('Ctrl Pts',(2.14081697072266,1.21324505073512,-7.02629463208905));
#147221=CARTESIAN_POINT('Ctrl Pts',(2.13882292648665,1.21220011139562,-7.01996545799531));
#147222=CARTESIAN_POINT('Ctrl Pts',(2.13683000013097,1.21115091716963,-7.01363664650975));
#147223=CARTESIAN_POINT('Ctrl Pts',(2.12862385216706,1.2068307158552,-6.98757689606371));
#147224=CARTESIAN_POINT('Ctrl Pts',(2.12044297297646,1.20243940497546,-6.96152086016398));
#147225=CARTESIAN_POINT('Ctrl Pts',(2.11228911062145,1.19797317360287,-6.9354693220977));
#147226=CARTESIAN_POINT('Ctrl Pts',(2.42444039675648,1.197203562,-7.09787518030664));
#147227=CARTESIAN_POINT('Ctrl Pts',(2.0401171296216,1.261925886,-7.22914951711605));
#147228=CARTESIAN_POINT('Ctrl Pts',(1.64386633789125,1.327100493,-7.31815870169077));
#147229=CARTESIAN_POINT('Ctrl Pts',(1.63026962690392,1.32933685520693,-7.32121290923592));
#147230=CARTESIAN_POINT('Ctrl Pts',(1.61667291591659,1.33157321741388,-7.32426711678122));
#147231=CARTESIAN_POINT('Ctrl Pts',(2.116753915,1.197203562,-6.934107936));
#147232=CARTESIAN_POINT('Ctrl Pts',(1.741298029,1.261925886,-7.04872220500001));
#147233=CARTESIAN_POINT('Ctrl Pts',(1.355661661,1.327100493,-7.12212619));
#147234=CARTESIAN_POINT('Ctrl Pts',(1.342429166955,1.32933685520693,-7.12464493012668));
#147235=CARTESIAN_POINT('Ctrl Pts',(1.32919667290999,1.33157321741388,-7.12716367025349));
#147236=CARTESIAN_POINT('Origin',(-0.0350990746584939,1.3392792370096,0.195366164253897));
#147237=CARTESIAN_POINT('Ctrl Pts',(1.16819610908941,1.32841655815206,-7.40846719817911));
#147238=CARTESIAN_POINT('Ctrl Pts',(1.1641114955447,1.32775852557603,-7.40910666158955));
#147239=CARTESIAN_POINT('Ctrl Pts',(1.160026882,1.327100493,-7.409746125));
#147240=CARTESIAN_POINT('Ctrl Pts',(0.806907722,1.270212881,-7.465028413));
#147241=CARTESIAN_POINT('Ctrl Pts',(0.450131734,1.214285714,-7.486479909));
#147242=CARTESIAN_POINT('Ctrl Pts',(0.395735648,1.205758742,-7.489750525));
#147243=CARTESIAN_POINT('Ctrl Pts',(0.34129778,1.197204389,-7.492230364));
#147244=CARTESIAN_POINT('Ctrl Pts',(1.36351378779214,1.32841655815206,-7.12063157633199));
#147245=CARTESIAN_POINT('Ctrl Pts',(1.35958772439607,1.32775852557603,-7.12137888316599));
#147246=CARTESIAN_POINT('Ctrl Pts',(1.355661661,1.327100493,-7.12212619));
#147247=CARTESIAN_POINT('Ctrl Pts',(1.016249329,1.270212881,-7.186731656));
#147248=CARTESIAN_POINT('Ctrl Pts',(0.672231452,1.214285714,-7.218767545));
#147249=CARTESIAN_POINT('Ctrl Pts',(0.619780539,1.205758742,-7.223651918));
#147250=CARTESIAN_POINT('Ctrl Pts',(0.56726419,1.197204389,-7.227773609));
#147251=CARTESIAN_POINT('',(0.571984074779071,1.19797317419155,-7.22740162212021));
#147252=CARTESIAN_POINT('Ctrl Pts',(0.571984074867032,1.19797317412081,
-7.22740162308611));
#147253=CARTESIAN_POINT('Ctrl Pts',(0.605444369462677,1.2034230203102,-7.22475354015837));
#147254=CARTESIAN_POINT('Ctrl Pts',(0.638861721438653,1.20886077967912,
-7.22187502591681));
#147255=CARTESIAN_POINT('Ctrl Pts',(0.672231451661377,1.21428571395252,
-7.21876754508335));
#147256=CARTESIAN_POINT('Ctrl Pts',(0.819239089143573,1.23818482283999,
-7.20507779056777));
#147257=CARTESIAN_POINT('Ctrl Pts',(0.966335304119417,1.26233315949238,
-7.1868460377057));
#147258=CARTESIAN_POINT('Ctrl Pts',(1.11310007968281,1.28666599845873,-7.16404272835986));
#147259=CARTESIAN_POINT('Ctrl Pts',(1.19407878472327,1.30009184796444,-7.15146080974638));
#147260=CARTESIAN_POINT('Ctrl Pts',(1.27495641085275,1.31357379251701,-7.13748803685432));
#147261=CARTESIAN_POINT('Ctrl Pts',(1.3556616535332,1.32710049174852,-7.12212619142127));
#147262=CARTESIAN_POINT('Ctrl Pts',(0.593952685421233,1.2368931917972,-7.4764443559927));
#147263=CARTESIAN_POINT('Ctrl Pts',(0.59144408727556,1.2326322451142,-7.44784838639651));
#147264=CARTESIAN_POINT('Ctrl Pts',(0.588926130551418,1.22830577222365,
-7.41926291457609));
#147265=CARTESIAN_POINT('Ctrl Pts',(0.586398144197795,1.2239104649318,-7.39068899687834));
#147266=CARTESIAN_POINT('Ctrl Pts',(0.583988653383375,1.21972118102563,
-7.36345443838238));
#147267=CARTESIAN_POINT('Ctrl Pts',(0.581559700274736,1.2154710086013,-7.33623087966888));
#147268=CARTESIAN_POINT('Ctrl Pts',(0.579147544540276,1.21115091650039,
-7.30901700028623));
#147269=CARTESIAN_POINT('Ctrl Pts',(0.576735328246361,1.20683071593948,
-7.28180243767335));
#147270=CARTESIAN_POINT('Ctrl Pts',(0.574346991003699,1.20243940508096,
-7.25459693016565));
#147271=CARTESIAN_POINT('Ctrl Pts',(0.571984075606748,1.1979731744789,-7.22740161874848));
#147272=CARTESIAN_POINT('Ctrl Pts',(0.841924975632513,1.197203562,-7.45311382237692));
#147273=CARTESIAN_POINT('Ctrl Pts',(0.438366870731753,1.261925886,-7.49870089635555));
#147274=CARTESIAN_POINT('Ctrl Pts',(0.0322458591924727,1.327100493,-7.50044688815638));
#147275=CARTESIAN_POINT('Ctrl Pts',(0.0183104670971001,1.32933685526002,
-7.50050679906878));
#147276=CARTESIAN_POINT('Ctrl Pts',(0.00437507500172815,1.33157321752005,
-7.50056670998106));
#147277=CARTESIAN_POINT('Ctrl Pts',(0.57663715,1.197203562,-7.227031866));
#147278=CARTESIAN_POINT('Ctrl Pts',(0.185320533,1.261925886,-7.258254601));
#147279=CARTESIAN_POINT('Ctrl Pts',(-0.207079558,1.327100493,-7.247042021));
#147280=CARTESIAN_POINT('Ctrl Pts',(-0.220544138681554,1.32933685526002,
-7.2466572792746));
#147281=CARTESIAN_POINT('Ctrl Pts',(-0.234008719363109,1.33157321752005,
-7.24627253754923));
#147282=CARTESIAN_POINT('Origin',(0.00771948208620379,1.33927931000909,
0.19834381347634));
#147283=CARTESIAN_POINT('Ctrl Pts',(-0.451717121439883,1.32841655815206,
-7.48638898311077));
#147284=CARTESIAN_POINT('Ctrl Pts',(-0.455843704719942,1.32775852557603,
-7.48613542505538));
#147285=CARTESIAN_POINT('Ctrl Pts',(-0.459970288,1.327100493,-7.48588186700001));
#147286=CARTESIAN_POINT('Ctrl Pts',(-0.816717776000001,1.270212881,-7.46396150500001));
#147287=CARTESIAN_POINT('Ctrl Pts',(-1.169763977,1.214285714,-7.408215186));
#147288=CARTESIAN_POINT('Ctrl Pts',(-1.223591399,1.205758742,-7.399715786));
#147289=CARTESIAN_POINT('Ctrl Pts',(-1.277289632,1.197204389,-7.390435115));
#147290=CARTESIAN_POINT('Ctrl Pts',(-0.199089711805015,1.32841655815206,
-7.24727032571477));
#147291=CARTESIAN_POINT('Ctrl Pts',(-0.203084634902507,1.32775852557603,
-7.24715617335739));
#147292=CARTESIAN_POINT('Ctrl Pts',(-0.207079558,1.327100493,-7.247042021));
#147293=CARTESIAN_POINT('Ctrl Pts',(-0.552444884,1.270212881,-7.237173429));
#147294=CARTESIAN_POINT('Ctrl Pts',(-0.895306583,1.214285714,-7.194506663));
#147295=CARTESIAN_POINT('Ctrl Pts',(-0.947581218,1.205758742,-7.188001446));
#147296=CARTESIAN_POINT('Ctrl Pts',(-0.999755805999999,1.197204389,-7.180737311));
#147297=CARTESIAN_POINT('',(-0.995066303928726,1.19797317409232,-7.18138865723257));
#147298=CARTESIAN_POINT('Ctrl Pts',(-0.995066304282821,1.19797317433401,
-7.18138865950215));
#147299=CARTESIAN_POINT('Ctrl Pts',(-0.864780371989077,1.21932946147407,
-7.19944131181136));
#147300=CARTESIAN_POINT('Ctrl Pts',(-0.734048704424371,1.24060039054742,
-7.2139446398357));
#147301=CARTESIAN_POINT('Ctrl Pts',(-0.537095387670994,1.27286180063188,
-7.23037941102887));
#147302=CARTESIAN_POINT('Ctrl Pts',(-0.471241893446828,1.28366384129796,
-7.23496979160408));
#147303=CARTESIAN_POINT('Ctrl Pts',(-0.372330447545514,1.29991103390507,
-7.2405084779935));
#147304=CARTESIAN_POINT('Ctrl Pts',(-0.339310531179135,1.30533866123095,
-7.24213098669581));
#147305=CARTESIAN_POINT('Ctrl Pts',(-0.28975415731532,1.31349012118079,
-7.24422640291922));
#147306=CARTESIAN_POINT('Ctrl Pts',(-0.273224609628572,1.316209988635,-7.24486866327605));
#147307=CARTESIAN_POINT('Ctrl Pts',(-0.248424458125744,1.32029216624683,
-7.24574728745407));
#147308=CARTESIAN_POINT('Ctrl Pts',(-0.240155253142869,1.32165353792755,
-7.24602607766629));
#147309=CARTESIAN_POINT('Ctrl Pts',(-0.223993606449739,1.32431471596907,
-7.24654326009665));
#147310=CARTESIAN_POINT('Ctrl Pts',(-0.219986974589969,1.32497441951572,
-7.24667320063075));
#147311=CARTESIAN_POINT('Ctrl Pts',(-0.207079563538114,1.32710049222491,
-7.24704202165181));
#147312=CARTESIAN_POINT('Ctrl Pts',(-1.02714813259364,1.2368931917972,-7.42933151192617));
#147313=CARTESIAN_POINT('Ctrl Pts',(-1.02345079312789,1.23263224508648,
-7.40086482581375));
#147314=CARTESIAN_POINT('Ctrl Pts',(-1.01976484996718,1.22830577220348,
-7.37240638023503));
#147315=CARTESIAN_POINT('Ctrl Pts',(-1.01609118573003,1.22391046491851,
-7.34395706257801));
#147316=CARTESIAN_POINT('Ctrl Pts',(-1.01258971894321,1.21972118100939,
-7.31684126362269));
#147317=CARTESIAN_POINT('Ctrl Pts',(-1.00910962403246,1.21547100857855,
-7.28973202346733));
#147318=CARTESIAN_POINT('Ctrl Pts',(-1.00561520528948,1.21115091648241,
-7.26263584727502));
#147319=CARTESIAN_POINT('Ctrl Pts',(-1.00212069881583,1.20683071592629,
-7.2355389908077));
#147320=CARTESIAN_POINT('Ctrl Pts',(-0.998604818142201,1.20243940507305,
-7.20845611103345));
#147321=CARTESIAN_POINT('Ctrl Pts',(-0.995066302196114,1.1979731744789,
-7.1813886540959));
#147322=CARTESIAN_POINT('Ctrl Pts',(-0.779957922291379,1.197203562,-7.45985314609555));
#147323=CARTESIAN_POINT('Ctrl Pts',(-1.18388093561253,1.261925886,-7.41762135550114));
#147324=CARTESIAN_POINT('Ctrl Pts',(-1.58088240026032,1.327100493,-7.3320225141512));
#147325=CARTESIAN_POINT('Ctrl Pts',(-1.59450486913966,1.32933685516649,
-7.32908532712236));
#147326=CARTESIAN_POINT('Ctrl Pts',(-1.60812733801905,1.331573217333,-7.32614814009351));
#147327=CARTESIAN_POINT('Ctrl Pts',(-0.990442528,1.197203562,-7.182027819));
#147328=CARTESIAN_POINT('Ctrl Pts',(-1.379322344,1.261925886,-7.128399079));
#147329=CARTESIAN_POINT('Ctrl Pts',(-1.760137966,1.327100493,-7.033094222));
#147330=CARTESIAN_POINT('Ctrl Pts',(-1.77320504363426,1.32933685516649,
-7.02982398860254));
#147331=CARTESIAN_POINT('Ctrl Pts',(-1.78627212126847,1.33157321733301,
-7.0265537552051));
#147332=CARTESIAN_POINT('Origin',(0.0501770555670825,1.33927929947402,0.192047116197817));
#147333=CARTESIAN_POINT('Ctrl Pts',(-2.05050856186381,1.32841655815206,
-7.2142555408744));
#147334=CARTESIAN_POINT('Ctrl Pts',(-2.0544841604319,1.32775852557603,-7.2131208174372));
#147335=CARTESIAN_POINT('Ctrl Pts',(-2.058459759,1.327100493,-7.211986094));
#147336=CARTESIAN_POINT('Ctrl Pts',(-2.402154459,1.270212881,-7.11388805300001));
#147337=CARTESIAN_POINT('Ctrl Pts',(-2.734962825,1.214285714,-6.983550554));
#147338=CARTESIAN_POINT('Ctrl Pts',(-2.785704672,1.205758742,-6.963678562));
#147339=CARTESIAN_POINT('Ctrl Pts',(-2.836152401,1.197204389,-6.943071335));
#147340=CARTESIAN_POINT('Ctrl Pts',(-1.75238399671172,1.32841655815206,
-7.03503476980878));
#147341=CARTESIAN_POINT('Ctrl Pts',(-1.75626098135586,1.32775852557603,
-7.03406449590439));
#147342=CARTESIAN_POINT('Ctrl Pts',(-1.760137966,1.327100493,-7.033094222));
#147343=CARTESIAN_POINT('Ctrl Pts',(-2.095307388,1.270212881,-6.949213017));
#147344=CARTESIAN_POINT('Ctrl Pts',(-2.420981077,1.214285714,-6.833838645));
#147345=CARTESIAN_POINT('Ctrl Pts',(-2.470635131,1.205758742,-6.816248015));
#147346=CARTESIAN_POINT('Ctrl Pts',(-2.520028332,1.197204389,-6.797937717));
#147347=CARTESIAN_POINT('',(-2.515588486907,1.19797317420338,-6.79958194010459));
#147348=CARTESIAN_POINT('Ctrl Pts',(-2.51558848697322,1.1979731742374,-6.79958194026763));
#147349=CARTESIAN_POINT('Ctrl Pts',(-2.48410884521609,1.20342302033325,
-6.81122821864144));
#147350=CARTESIAN_POINT('Ctrl Pts',(-2.45257142183251,1.20886077966291,
-6.82264733217239));
#147351=CARTESIAN_POINT('Ctrl Pts',(-2.42098107736823,1.21428571399529,
-6.83383864515277));
#147352=CARTESIAN_POINT('Ctrl Pts',(-2.2818123815728,1.23818482264714,-6.88314106461257));
#147353=CARTESIAN_POINT('Ctrl Pts',(-2.1406561597672,1.2623331590456,-6.92835847082164));
#147354=CARTESIAN_POINT('Ctrl Pts',(-1.99788119768136,1.28666599770993,
-6.96928767690998));
#147355=CARTESIAN_POINT('Ctrl Pts',(-1.91910390320488,1.30009184751514,
-6.99187071299422));
#147356=CARTESIAN_POINT('Ctrl Pts',(-1.83983434093763,1.31357379235643,
-7.01314900188966));
#147357=CARTESIAN_POINT('Ctrl Pts',(-1.76013797324525,1.32710049185966,
-7.03309422063433));
#147358=CARTESIAN_POINT('Ctrl Pts',(-2.60022064565276,1.2368931917972,-7.03483138315546));
#147359=CARTESIAN_POINT('Ctrl Pts',(-2.59049025192455,1.23263224512833,
-7.00782505119041));
#147360=CARTESIAN_POINT('Ctrl Pts',(-2.58077275948662,1.22830577224818,
-6.98082431713158));
#147361=CARTESIAN_POINT('Ctrl Pts',(-2.57106922114835,1.22391046496396,
-6.95382985797731));
#147362=CARTESIAN_POINT('Ctrl Pts',(-2.56182052148295,1.21972118105618,
-6.92810072323856));
#147363=CARTESIAN_POINT('Ctrl Pts',(-2.55259410397172,1.21547100862086,
-6.90237339964068));
#147364=CARTESIAN_POINT('Ctrl Pts',(-2.5433565058699,1.2111509165129,-6.87666191378215));
#147365=CARTESIAN_POINT('Ctrl Pts',(-2.53411867584956,1.20683071594498,
-6.85094978241275));
#147366=CARTESIAN_POINT('Ctrl Pts',(-2.52486297614487,1.20243940511241,
-6.8252558957049));
#147367=CARTESIAN_POINT('Ctrl Pts',(-2.51558848481493,1.1979731744789,-6.79958193754073));
#147368=CARTESIAN_POINT('Ctrl Pts',(-2.36537085379973,1.197203562,-7.11777802662513));
#147369=CARTESIAN_POINT('Ctrl Pts',(-2.75077178539882,1.261925886,-6.9897020842389));
#147370=CARTESIAN_POINT('Ctrl Pts',(-3.12009035661124,1.327100493,-6.82076091693207));
#147371=CARTESIAN_POINT('Ctrl Pts',(-3.1327629312016,1.32933685513552,-6.81496397166328));
#147372=CARTESIAN_POINT('Ctrl Pts',(-3.14543550579188,1.33157321727106,
-6.80916702639437));
#147373=CARTESIAN_POINT('Ctrl Pts',(-2.511210214,1.197203562,-6.80120013400001));
#147374=CARTESIAN_POINT('Ctrl Pts',(-2.879469642,1.261925886,-6.665227538));
#147375=CARTESIAN_POINT('Ctrl Pts',(-3.23089428,1.327100493,-6.49028675400001));
#147376=CARTESIAN_POINT('Ctrl Pts',(-3.24295285296404,1.32933685513552,
-6.4842839415044));
#147377=CARTESIAN_POINT('Ctrl Pts',(-3.25501142592809,1.33157321727106,
-6.47828112900879));
#147378=CARTESIAN_POINT('Origin',(0.0902884086503142,1.33927920699605,0.176770638020913));
#147379=CARTESIAN_POINT('Ctrl Pts',(-3.55342050042447,1.32841655815206,
-6.60479152680991));
#147380=CARTESIAN_POINT('Ctrl Pts',(-3.55705921971224,1.32775852557603,
-6.60282869640496));
#147381=CARTESIAN_POINT('Ctrl Pts',(-3.560697939,1.327100493,-6.600865866));
#147382=CARTESIAN_POINT('Ctrl Pts',(-3.875269069,1.270212881,-6.431177102));
#147383=CARTESIAN_POINT('Ctrl Pts',(-4.172277851,1.214285714,-6.232342861));
#147384=CARTESIAN_POINT('Ctrl Pts',(-4.217561491,1.205758742,-6.202027467));
#147385=CARTESIAN_POINT('Ctrl Pts',(-4.262399835,1.197204389,-6.171057255));
#147386=CARTESIAN_POINT('Ctrl Pts',(-3.22373875465858,1.32841655815206,
-6.49384880706528));
#147387=CARTESIAN_POINT('Ctrl Pts',(-3.22731651732929,1.32775852557603,
-6.49206778053264));
#147388=CARTESIAN_POINT('Ctrl Pts',(-3.23089428,1.327100493,-6.490286754));
#147389=CARTESIAN_POINT('Ctrl Pts',(-3.540195646,1.270212881,-6.336315127));
#147390=CARTESIAN_POINT('Ctrl Pts',(-3.833453187,1.214285714,-6.153627927));
#147391=CARTESIAN_POINT('Ctrl Pts',(-3.878164891,1.205758742,-6.125774403));
#147392=CARTESIAN_POINT('Ctrl Pts',(-3.922467133,1.197204389,-6.097274111));
#147393=CARTESIAN_POINT('',(-3.91848454889701,1.19797317421983,-6.09983432791826));
#147394=CARTESIAN_POINT('Ctrl Pts',(-3.91848454655753,1.1979731744789,-6.09983432616152));
#147395=CARTESIAN_POINT('Ctrl Pts',(-3.876155517,1.20614195,-6.127026159));
#147396=CARTESIAN_POINT('Ctrl Pts',(-3.833453187,1.214285714,-6.153627927));
#147397=CARTESIAN_POINT('Ctrl Pts',(-3.54019564989936,1.27021288012461,
-6.3363151241931));
#147398=CARTESIAN_POINT('Ctrl Pts',(-3.23089428679994,1.32710049454013,
-6.49028675033807));
#147399=CARTESIAN_POINT('Ctrl Pts',(-4.05170973114006,1.2368931917972,-6.31139035819461));
#147400=CARTESIAN_POINT('Ctrl Pts',(-4.03640126539842,1.23263224511851,
-6.28710716620259));
#147401=CARTESIAN_POINT('Ctrl Pts',(-4.02110660284373,1.22830577222571,
-6.26282666784149));
#147402=CARTESIAN_POINT('Ctrl Pts',(-4.00582691709565,1.22391046493059,
-6.2385492979449));
#147403=CARTESIAN_POINT('Ctrl Pts',(-3.9912634435281,1.21972118102325,-6.21540989307704));
#147404=CARTESIAN_POINT('Ctrl Pts',(-3.9767221205835,1.21547100859937,-6.19226746695517));
#147405=CARTESIAN_POINT('Ctrl Pts',(-3.96217328298514,1.21115091647881,
-6.16914291186207));
#147406=CARTESIAN_POINT('Ctrl Pts',(-3.94762408012453,1.20683071589829,
-6.14601777620529));
#147407=CARTESIAN_POINT('Ctrl Pts',(-3.93306134734589,1.20243940503364,
-6.12291430016812));
#147408=CARTESIAN_POINT('Ctrl Pts',(-3.91848454655753,1.1979731744789,-6.09983432616152));
#147409=CARTESIAN_POINT('Ctrl Pts',(-3.84018167302787,1.197203562,-6.44288351854414));
#147410=CARTESIAN_POINT('Ctrl Pts',(-4.18903960369843,1.261925886,-6.23495211221092));
#147411=CARTESIAN_POINT('Ctrl Pts',(-4.51340635488509,1.327100493,-5.99056811976438));
#147412=CARTESIAN_POINT('Ctrl Pts',(-4.52453648009277,1.32933685518452,
-5.98218247473529));
#147413=CARTESIAN_POINT('Ctrl Pts',(-4.53566660530047,1.33157321736907,
-5.97379682970635));
#147414=CARTESIAN_POINT('Ctrl Pts',(-3.914556502,1.197203562,-6.102355889));
#147415=CARTESIAN_POINT('Ctrl Pts',(-4.24497614,1.261925886,-5.890397365));
#147416=CARTESIAN_POINT('Ctrl Pts',(-4.550577568,1.327100493,-5.64400069100001));
#147417=CARTESIAN_POINT('Ctrl Pts',(-4.56106379121753,1.32933685518452,
-5.63554598402913));
#147418=CARTESIAN_POINT('Ctrl Pts',(-4.57155001443505,1.33157321736907,
-5.62709127705826));
#147419=CARTESIAN_POINT('Origin',(0.126178134698828,1.33927923045498,0.15322871453506));
#147420=CARTESIAN_POINT('Ctrl Pts',(-4.8901784459381,1.32841655815206,-5.68649480220919));
#147421=CARTESIAN_POINT('Ctrl Pts',(-4.89331014346905,1.32775852557603,
-5.68379564460459));
#147422=CARTESIAN_POINT('Ctrl Pts',(-4.896441841,1.327100493,-5.681096487));
#147423=CARTESIAN_POINT('Ctrl Pts',(-5.167180404,1.270212881,-5.447751458));
#147424=CARTESIAN_POINT('Ctrl Pts',(-5.414501802,1.214285714,-5.189717742));
#147425=CARTESIAN_POINT('Ctrl Pts',(-5.452209822,1.205758742,-5.150376461));
#147426=CARTESIAN_POINT('Ctrl Pts',(-5.48934219,1.197204389,-5.110491397));
#147427=CARTESIAN_POINT('Ctrl Pts',(-4.5443550709688,1.32841655815206,-5.64901769170602));
#147428=CARTESIAN_POINT('Ctrl Pts',(-4.54746631948441,1.32775852557603,
-5.64650919135301));
#147429=CARTESIAN_POINT('Ctrl Pts',(-4.550577568,1.327100493,-5.64400069100001));
#147430=CARTESIAN_POINT('Ctrl Pts',(-4.819548292,1.270212881,-5.42713818300001));
#147431=CARTESIAN_POINT('Ctrl Pts',(-5.066677286,1.214285714,-5.185680407));
#147432=CARTESIAN_POINT('Ctrl Pts',(-5.104355971,1.205758742,-5.148866388));
#147433=CARTESIAN_POINT('Ctrl Pts',(-5.14149573100001,1.197204389,-5.111508744));
#147434=CARTESIAN_POINT('',(-5.138156628083,1.19797317418971,-5.11486524319787));
#147435=CARTESIAN_POINT('Ctrl Pts',(-5.13815662819914,1.1979731742527,-5.11486524329903));
#147436=CARTESIAN_POINT('Ctrl Pts',(-5.11447662531269,1.20342302023506,
-5.13865307776319));
#147437=CARTESIAN_POINT('Ctrl Pts',(-5.09064879615534,1.20886077956019,
-5.16225900494202));
#147438=CARTESIAN_POINT('Ctrl Pts',(-5.06667728625762,1.21428571394757,
-5.18568040677395));
#147439=CARTESIAN_POINT('Ctrl Pts',(-4.96107249736565,1.23818487921893,
-5.2888617335718));
#147440=CARTESIAN_POINT('Ctrl Pts',(-4.85194861090683,1.26233327307656,
-5.38917012841354));
#147441=CARTESIAN_POINT('Ctrl Pts',(-4.7395550123306,1.28666616990491,-5.48626633390387));
#147442=CARTESIAN_POINT('Ctrl Pts',(-4.67754130380628,1.30009196274881,
-5.53983963222664));
#147443=CARTESIAN_POINT('Ctrl Pts',(-4.61453298472437,1.31357385009881,
-5.59243548013358));
#147444=CARTESIAN_POINT('Ctrl Pts',(-4.55057757375112,1.32710049178363,
-5.64400068636306));
#147445=CARTESIAN_POINT('Ctrl Pts',(-5.31374537287477,1.2368931917972,-5.29283573461458));
#147446=CARTESIAN_POINT('Ctrl Pts',(-5.29357464216323,1.2326322451214,-5.27241113771948));
#147447=CARTESIAN_POINT('Ctrl Pts',(-5.27341797098529,1.2283057722396,-5.25198620429075));
#147448=CARTESIAN_POINT('Ctrl Pts',(-5.25327659895755,1.22391046495337,
-5.23156110664842));
#147449=CARTESIAN_POINT('Ctrl Pts',(-5.23407932319174,1.21972118102907,
-5.21209340447582));
#147450=CARTESIAN_POINT('Ctrl Pts',(-5.21490303063396,1.21547100857755,
-5.19261799002205));
#147451=CARTESIAN_POINT('Ctrl Pts',(-5.19572324093141,1.21115091645384,
-5.17316164412882));
#147452=CARTESIAN_POINT('Ctrl Pts',(-5.17654296970241,1.20683071587019,
-5.15370480976593));
#147453=CARTESIAN_POINT('Ctrl Pts',(-5.15735414107387,1.20243940501329,
-5.13427203714468));
#147454=CARTESIAN_POINT('Ctrl Pts',(-5.13815662496132,1.1979731744789,-5.11486524163069));
#147455=CARTESIAN_POINT('Ctrl Pts',(-5.1354298661806,1.197203562,-5.4667269377071));
#147456=CARTESIAN_POINT('Ctrl Pts',(-5.43143258568287,1.261925886,-5.1886627093742));
#147457=CARTESIAN_POINT('Ctrl Pts',(-5.69568048758388,1.327100493,-4.88026301484489));
#147458=CARTESIAN_POINT('Ctrl Pts',(-5.70474773081824,1.32933685518157,
-4.86968077361013));
#147459=CARTESIAN_POINT('Ctrl Pts',(-5.7138149740526,1.33157321736317,-4.85909853237526));
#147460=CARTESIAN_POINT('Ctrl Pts',(-5.134862478,1.197203562,-5.118172265));
#147461=CARTESIAN_POINT('Ctrl Pts',(-5.411992272,1.261925886,-4.840138759));
#147462=CARTESIAN_POINT('Ctrl Pts',(-5.657480906,1.327100493,-4.533807429));
#147463=CARTESIAN_POINT('Ctrl Pts',(-5.66590445502249,1.32933685518157,
-4.523296160379));
#147464=CARTESIAN_POINT('Ctrl Pts',(-5.67432800404486,1.33157321736317,
-4.51278489175806));
#147465=CARTESIAN_POINT('Origin',(0.156167784693459,1.3392793125037,0.122521716615214));
#147466=CARTESIAN_POINT('Ctrl Pts',(-5.99827708283658,1.32841655815206,
-4.502303900394));
#147467=CARTESIAN_POINT('Ctrl Pts',(-6.00075532391828,1.32775852557603,
-4.498994625197));
#147468=CARTESIAN_POINT('Ctrl Pts',(-6.003233565,1.327100493,-4.49568535));
#147469=CARTESIAN_POINT('Ctrl Pts',(-6.217480127,1.270212881,-4.20959501));
#147470=CARTESIAN_POINT('Ctrl Pts',(-6.403549666,1.214285714,-3.904427189));
#147471=CARTESIAN_POINT('Ctrl Pts',(-6.431918881,1.205758742,-3.857899576));
#147472=CARTESIAN_POINT('Ctrl Pts',(-6.459609006,1.197204389,-3.810964641));
#147473=CARTESIAN_POINT('Ctrl Pts',(-5.65248239434487,1.32841655815206,
-4.54004478794311));
#147474=CARTESIAN_POINT('Ctrl Pts',(-5.65498165017243,1.32775852557603,
-4.53692610847156));
#147475=CARTESIAN_POINT('Ctrl Pts',(-5.657480906,1.327100493,-4.533807429));
#147476=CARTESIAN_POINT('Ctrl Pts',(-5.873544215,1.270212881,-4.264194291));
#147477=CARTESIAN_POINT('Ctrl Pts',(-6.062989186,1.214285714,-3.975256234));
#147478=CARTESIAN_POINT('Ctrl Pts',(-6.091873039,1.205758742,-3.931203103));
#147479=CARTESIAN_POINT('Ctrl Pts',(-6.120113703,1.197204389,-3.88673491));
#147480=CARTESIAN_POINT('',(-6.11757421509193,1.19797317422572,-3.89073074390562));
#147481=CARTESIAN_POINT('Ctrl Pts',(-6.11757421698391,1.19797317448009,
-3.89073074505997));
#147482=CARTESIAN_POINT('Ctrl Pts',(-6.04698796875694,1.21932945204533,
-4.00171673013818));
#147483=CARTESIAN_POINT('Ctrl Pts',(-5.97340797643286,1.24060037954165,
-4.11074469498818));
#147484=CARTESIAN_POINT('Ctrl Pts',(-5.85842899190968,1.27286180860714,
-4.27149478000183));
#147485=CARTESIAN_POINT('Ctrl Pts',(-5.81929492630778,1.28366385684478,
-4.32465760012926));
#147486=CARTESIAN_POINT('Ctrl Pts',(-5.7594824465453,1.2999110339762,-4.4036297454828));
#147487=CARTESIAN_POINT('Ctrl Pts',(-5.73934242028341,1.30533866127671,
-4.42984666258494));
#147488=CARTESIAN_POINT('Ctrl Pts',(-5.70885735049756,1.31349012118794,
-4.46897319390663));
#147489=CARTESIAN_POINT('Ctrl Pts',(-5.69864585458784,1.31620998862927,
-4.48198717843723));
#147490=CARTESIAN_POINT('Ctrl Pts',(-5.6832602307808,1.32029216622185,-4.50145772203961));
#147491=CARTESIAN_POINT('Ctrl Pts',(-5.67811934425274,1.32165353789618,
-4.50794068123779));
#147492=CARTESIAN_POINT('Ctrl Pts',(-5.66805069280448,1.32431471591157,
-4.52059329179272));
#147493=CARTESIAN_POINT('Ctrl Pts',(-5.66555589084582,1.32497441924694,
-4.52373111528487));
#147494=CARTESIAN_POINT('Ctrl Pts',(-5.65748091102111,1.32710049205024,
-4.53380742434282));
#147495=CARTESIAN_POINT('Ctrl Pts',(-6.32731618654932,1.2368931917972,-4.02679399416497));
#147496=CARTESIAN_POINT('Ctrl Pts',(-6.30322635167544,1.23263224513509,
-4.01118302401817));
#147497=CARTESIAN_POINT('Ctrl Pts',(-6.279150175269,1.22830577224276,-3.99556870262379));
#147498=CARTESIAN_POINT('Ctrl Pts',(-6.25508890503236,1.22391046494856,
-3.97995093197957));
#147499=CARTESIAN_POINT('Ctrl Pts',(-6.23215547048253,1.21972118104266,
-3.96506522073654));
#147500=CARTESIAN_POINT('Ctrl Pts',(-6.20924087068471,1.2154710086209,-3.95016746669878));
#147501=CARTESIAN_POINT('Ctrl Pts',(-6.18632695457099,1.21115091649654,
-3.93528908736913));
#147502=CARTESIAN_POINT('Ctrl Pts',(-6.16341246318181,1.20683071591219,
-3.92041033450375));
#147503=CARTESIAN_POINT('Ctrl Pts',(-6.14049478700707,1.20243940505261,
-3.90555692044374));
#147504=CARTESIAN_POINT('Ctrl Pts',(-6.11757421157736,1.19797317447888,
-3.89073074300301));
#147505=CARTESIAN_POINT('Ctrl Pts',(-6.19055106550973,1.197203562,-4.2349522806284));
#147506=CARTESIAN_POINT('Ctrl Pts',(-6.41985781637798,1.261925886,-3.89975720421092));
#147507=CARTESIAN_POINT('Ctrl Pts',(-6.61163093231082,1.327100493,-3.54176223582509));
#147508=CARTESIAN_POINT('Ctrl Pts',(-6.61821131918263,1.32933685510004,
-3.52947821270389));
#147509=CARTESIAN_POINT('Ctrl Pts',(-6.62479170605458,1.3315732172001,-3.51719418958263));
#147510=CARTESIAN_POINT('Ctrl Pts',(-6.115067991,1.197203562,-3.894668594));
#147511=CARTESIAN_POINT('Ctrl Pts',(-6.32594966,1.261925886,-3.563560643));
#147512=CARTESIAN_POINT('Ctrl Pts',(-6.499846725,1.327100493,-3.21161837));
#147513=CARTESIAN_POINT('Ctrl Pts',(-6.50581372385702,1.32933685510004,
-3.19954203541252));
#147514=CARTESIAN_POINT('Ctrl Pts',(-6.51178072271392,1.3315732172001,-3.18746570082503));
#147515=CARTESIAN_POINT('Origin',(0.178855070989341,1.33927929116881,0.086085685520943));
#147516=CARTESIAN_POINT('Ctrl Pts',(-6.82590294932948,1.32841655815206,
-3.10759027252605));
#147517=CARTESIAN_POINT('Ctrl Pts',(-6.82761185416474,1.32775852557603,
-3.10382561776302));
#147518=CARTESIAN_POINT('Ctrl Pts',(-6.829320759,1.327100493,-3.100060963));
#147519=CARTESIAN_POINT('Ctrl Pts',(-6.977057389,1.270212881,-2.774602578));
#147520=CARTESIAN_POINT('Ctrl Pts',(-7.093174665,1.214285714,-2.436569961));
#147521=CARTESIAN_POINT('Ctrl Pts',(-7.11087856200001,1.205758742,-2.385031595));
#147522=CARTESIAN_POINT('Ctrl Pts',(-7.127831683,1.197204389,-2.333241414));
#147523=CARTESIAN_POINT('Ctrl Pts',(-6.49630592356605,1.32841655815206,
-3.21878443522406));
#147524=CARTESIAN_POINT('Ctrl Pts',(-6.49807632428302,1.32775852557603,
-3.21520140261203));
#147525=CARTESIAN_POINT('Ctrl Pts',(-6.499846725,1.327100493,-3.21161837));
#147526=CARTESIAN_POINT('Ctrl Pts',(-6.652899739,1.270212881,-2.901861412));
#147527=CARTESIAN_POINT('Ctrl Pts',(-6.775802451,1.214285714,-2.578953498));
#147528=CARTESIAN_POINT('Ctrl Pts',(-6.794540894,1.205758742,-2.52972113));
#147529=CARTESIAN_POINT('Ctrl Pts',(-6.81256196,1.197204389,-2.480221671));
#147530=CARTESIAN_POINT('',(-6.81094082973592,1.19797317417747,-2.48466999862016));
#147531=CARTESIAN_POINT('Ctrl Pts',(-6.81094083026715,1.19797317404191,
-2.48466999883739));
#147532=CARTESIAN_POINT('Ctrl Pts',(-6.7994376935698,1.20342302021377,-2.51620222837882));
#147533=CARTESIAN_POINT('Ctrl Pts',(-6.7877240128223,1.20886077960922,-2.54763143357809));
#147534=CARTESIAN_POINT('Ctrl Pts',(-6.77580245114939,1.21428571398706,
-2.57895349787104));
#147535=CARTESIAN_POINT('Ctrl Pts',(-6.72328286275153,1.23818487596032,
-2.71694061468588));
#147536=CARTESIAN_POINT('Ctrl Pts',(-6.66636311616781,1.26233326641375,
-2.85379796006965));
#147537=CARTESIAN_POINT('Ctrl Pts',(-6.60512709703676,1.28666615973806,
-2.98911291815804));
#147538=CARTESIAN_POINT('Ctrl Pts',(-6.57133981565453,1.30009195594851,
-3.06377362649663));
#147539=CARTESIAN_POINT('Ctrl Pts',(-6.5362394286992,1.313573846679,-3.13796485072405));
#147540=CARTESIAN_POINT('Ctrl Pts',(-6.49984672854157,1.32710049174616,
-3.21161836311582));
#147541=CARTESIAN_POINT('Ctrl Pts',(-7.0450287280152,1.23689319179729,-2.57246384252723));
#147542=CARTESIAN_POINT('Ctrl Pts',(-7.01814620294757,1.23263224510488,
-2.56239645050775));
#147543=CARTESIAN_POINT('Ctrl Pts',(-6.99127629662418,1.22830577222459,
-2.55232284955791));
#147544=CARTESIAN_POINT('Ctrl Pts',(-6.96442020648894,1.22391046493979,
-2.54224267560677));
#147545=CARTESIAN_POINT('Ctrl Pts',(-6.93882295490602,1.21972118102739,
-2.53263499454345));
#147546=CARTESIAN_POINT('Ctrl Pts',(-6.91324150887695,1.21547100859126,
-2.52301150334711));
#147547=CARTESIAN_POINT('Ctrl Pts',(-6.88766489559399,1.21115091647302,
-2.51340678675703));
#147548=CARTESIAN_POINT('Ctrl Pts',(-6.86208764018606,1.20683071589479,
-2.50380182903149));
#147549=CARTESIAN_POINT('Ctrl Pts',(-6.83651272154253,1.20243940503304,
-2.49422230234871));
#147550=CARTESIAN_POINT('Ctrl Pts',(-6.81094082624304,1.19797317447888,
-2.48466999852047));
#147551=CARTESIAN_POINT('Ctrl Pts',(-6.95620897777927,1.197203562,-2.80515596191497));
#147552=CARTESIAN_POINT('Ctrl Pts',(-7.10809763203512,1.261925886,-2.428503387158));
#147553=CARTESIAN_POINT('Ctrl Pts',(-7.2184288620977,1.327100493,-2.03765259113515));
#147554=CARTESIAN_POINT('Ctrl Pts',(-7.22221470149621,1.3293368552233,-2.02424117224969));
#147555=CARTESIAN_POINT('Ctrl Pts',(-7.2260005408947,1.33157321744662,-2.0108297533642));
#147556=CARTESIAN_POINT('Ctrl Pts',(-6.80933972200001,1.197203562,-2.489054549));
#147557=CARTESIAN_POINT('Ctrl Pts',(-6.94411267200001,1.261925886,-2.120354393));
#147558=CARTESIAN_POINT('Ctrl Pts',(-7.03828693500001,1.327100493,-1.739257605));
#147559=CARTESIAN_POINT('Ctrl Pts',(-7.04151837395874,1.3293368552233,-1.72618087927298));
#147560=CARTESIAN_POINT('Ctrl Pts',(-7.04474981291752,1.33157321744662,
-1.71310415354602));
#147561=CARTESIAN_POINT('Origin',(0.19317929026764,1.33927922477741,0.0456244733727038));
#147562=CARTESIAN_POINT('Ctrl Pts',(-7.33435717978959,1.32841655815206,
-1.56756917649812));
#147563=CARTESIAN_POINT('Ctrl Pts',(-7.33521684189479,1.32775852557603,
-1.56352517324906));
#147564=CARTESIAN_POINT('Ctrl Pts',(-7.336076504,1.327100493,-1.55948117));
#147565=CARTESIAN_POINT('Ctrl Pts',(-7.410395202,1.270212881,-1.209872813));
#147566=CARTESIAN_POINT('Ctrl Pts',(-7.4511307,1.214285714,-0.854781429));
#147567=CARTESIAN_POINT('Ctrl Pts',(-7.457341465,1.205758742,-0.800642187));
#147568=CARTESIAN_POINT('Ctrl Pts',(-7.462764873,1.197204389,-0.746418412));
#147569=CARTESIAN_POINT('Ctrl Pts',(-7.03636940770779,1.32841655815206,
-1.7470172992385));
#147570=CARTESIAN_POINT('Ctrl Pts',(-7.0373281713539,1.32775852557603,-1.74313745211925));
#147571=CARTESIAN_POINT('Ctrl Pts',(-7.038286935,1.327100493,-1.739257605));
#147572=CARTESIAN_POINT('Ctrl Pts',(-7.121173066,1.270212881,-1.403840719));
#147573=CARTESIAN_POINT('Ctrl Pts',(-7.171786724,1.214285714,-1.062061763));
#147574=CARTESIAN_POINT('Ctrl Pts',(-7.179503569,1.205758742,-1.009952209));
#147575=CARTESIAN_POINT('Ctrl Pts',(-7.186462392,1.197204389,-0.957736023));
#147576=CARTESIAN_POINT('',(-7.18583542174986,1.19797317417719,-0.962428846770062));
#147577=CARTESIAN_POINT('Ctrl Pts',(-7.18583542231247,1.19797317411523,
-0.962428846855556));
#147578=CARTESIAN_POINT('Ctrl Pts',(-7.18137971988736,1.20342302019982,
-0.995696704436819));
#147579=CARTESIAN_POINT('Ctrl Pts',(-7.17669624851764,1.20886077957267,
-1.02890920738066));
#147580=CARTESIAN_POINT('Ctrl Pts',(-7.17178672423234,1.21428571396036,
-1.06206176261196));
#147581=CARTESIAN_POINT('Ctrl Pts',(-7.15015817611276,1.23818486528209,
-1.20811291074965));
#147582=CARTESIAN_POINT('Ctrl Pts',(-7.12398947874848,1.26233324483327,
-1.35400660537596));
#147583=CARTESIAN_POINT('Ctrl Pts',(-7.09327385727488,1.28666612712761,
-1.49932184448164));
#147584=CARTESIAN_POINT('Ctrl Pts',(-7.0763263374022,1.30009193414236,-1.57950035900928));
#147585=CARTESIAN_POINT('Ctrl Pts',(-7.05799548418409,1.31357383577967,
-1.65950264433222));
#147586=CARTESIAN_POINT('Ctrl Pts',(-7.0382869371124,1.32710049183488,-1.7392575978799));
#147587=CARTESIAN_POINT('Ctrl Pts',(-7.43332355589694,1.23689319179771,
-0.997848140191201));
#147588=CARTESIAN_POINT('Ctrl Pts',(-7.4049053377193,1.23263224508818,-0.993795066420124));
#147589=CARTESIAN_POINT('Ctrl Pts',(-7.37649810848686,1.22830577220118,
-0.989733216274669));
#147590=CARTESIAN_POINT('Ctrl Pts',(-7.34810295942658,1.22391046490981,
-0.985661976730492));
#147591=CARTESIAN_POINT('Ctrl Pts',(-7.3210387899748,1.21972118099116,-0.981781570374163));
#147592=CARTESIAN_POINT('Ctrl Pts',(-7.29398665783928,1.21547100854749,
-0.977882325800221));
#147593=CARTESIAN_POINT('Ctrl Pts',(-7.26694328144624,1.21115091641908,
-0.974000378013044));
#147594=CARTESIAN_POINT('Ctrl Pts',(-7.23989922610388,1.20683071583071,
-0.970118332765928));
#147595=CARTESIAN_POINT('Ctrl Pts',(-7.21286291982689,1.20243940497373,
-0.966260621572256));
#147596=CARTESIAN_POINT('Ctrl Pts',(-7.18583541843957,1.19797317447885,
-0.962428847399313));
#147597=CARTESIAN_POINT('Ctrl Pts',(-7.39660228961004,1.197203562,-1.24419366777322));
#147598=CARTESIAN_POINT('Ctrl Pts',(-7.46397070148977,1.261925886,-0.843695450120498));
#147599=CARTESIAN_POINT('Ctrl Pts',(-7.48770108087841,1.327100493,-0.438264575817652));
#147600=CARTESIAN_POINT('Ctrl Pts',(-7.48851535082179,1.32933685520391,
-0.424352865025269));
#147601=CARTESIAN_POINT('Ctrl Pts',(-7.48932962076503,1.33157321740785,
-0.410441154232886));
#147602=CARTESIAN_POINT('Ctrl Pts',(-7.185214296,1.197203562,-0.967055079));
#147603=CARTESIAN_POINT('Ctrl Pts',(-7.237576694,1.261925886,-0.578002727000001));
#147604=CARTESIAN_POINT('Ctrl Pts',(-7.247624671,1.327100493,-0.185571088));
#147605=CARTESIAN_POINT('Ctrl Pts',(-7.24796945122994,1.32933685520391,
-0.17210542513716));
#147606=CARTESIAN_POINT('Ctrl Pts',(-7.24831423146002,1.33157321740785,
-0.158639762274315));
#147607=CARTESIAN_POINT('Origin',(0.198471074688573,1.33927925974612,0.00302998021384858));
#147608=CARTESIAN_POINT('Ctrl Pts',(-7.4998650209685,1.32841655815206,0.0457497107196035));
#147609=CARTESIAN_POINT('Ctrl Pts',(-7.49983524348425,1.32775852557603,
0.0498839693598018));
#147610=CARTESIAN_POINT('Ctrl Pts',(-7.499805466,1.327100493,0.054018228));
#147611=CARTESIAN_POINT('Ctrl Pts',(-7.497231171,1.270212881,0.411429259));
#147612=CARTESIAN_POINT('Ctrl Pts',(-7.460680145,1.214285714,0.766975733));
#147613=CARTESIAN_POINT('Ctrl Pts',(-7.455107369,1.205758742,0.82118436));
#147614=CARTESIAN_POINT('Ctrl Pts',(-7.448747472,1.197204389,0.875306286));
#147615=CARTESIAN_POINT('Ctrl Pts',(-7.24742007933239,1.32841655815206,
-0.193561576570007));
#147616=CARTESIAN_POINT('Ctrl Pts',(-7.24752237516619,1.32775852557603,
-0.189566332285004));
#147617=CARTESIAN_POINT('Ctrl Pts',(-7.247624671,1.327100493,-0.185571088));
#147618=CARTESIAN_POINT('Ctrl Pts',(-7.256468254,1.270212881,0.159822005));
#147619=CARTESIAN_POINT('Ctrl Pts',(-7.23242622,1.214285714,0.5044908));
#147620=CARTESIAN_POINT('Ctrl Pts',(-7.22876063600001,1.205758742,0.557040955));
#147621=CARTESIAN_POINT('Ctrl Pts',(-7.224331829,1.197204389,0.609532297));
#147622=CARTESIAN_POINT('',(-7.22472833605622,1.19797317423029,0.604814408844145));
#147623=CARTESIAN_POINT('Ctrl Pts',(-7.22472833840409,1.19797317450532,
0.604814409085507));
#147624=CARTESIAN_POINT('Ctrl Pts',(-7.23570097124237,1.21932945016343,
0.473742269969239));
#147625=CARTESIAN_POINT('Ctrl Pts',(-7.24310536311774,1.24060037865077,
0.342417143140362));
#147626=CARTESIAN_POINT('Ctrl Pts',(-7.24885319740134,1.27286180825459,
0.144862795239759));
#147627=CARTESIAN_POINT('Ctrl Pts',(-7.24987160719395,1.28366385610865,
0.0788573177664608));
#147628=CARTESIAN_POINT('Ctrl Pts',(-7.25004721285279,1.29991103404772,
-0.0202088349386995));
#147629=CARTESIAN_POINT('Ctrl Pts',(-7.24987967981377,1.30533866134997,
-0.0532681654429701));
#147630=CARTESIAN_POINT('Ctrl Pts',(-7.24928909500079,1.31349012126183,
-0.102865303901341));
#147631=CARTESIAN_POINT('Ctrl Pts',(-7.24903552177914,1.31620998870393,
-0.119405380772484));
#147632=CARTESIAN_POINT('Ctrl Pts',(-7.24857020427949,1.32029216629707,
-0.144216728339316));
#147633=CARTESIAN_POINT('Ctrl Pts',(-7.24840089990121,1.32165353797173,
-0.15248889917553));
#147634=CARTESIAN_POINT('Ctrl Pts',(-7.24804234995001,1.32431471600077,
-0.168654843025585));
#147635=CARTESIAN_POINT('Ctrl Pts',(-7.24795518524569,1.32497441954237,
-0.172662633619452));
#147636=CARTESIAN_POINT('Ctrl Pts',(-7.24762467222746,1.32710049226711,
-0.185571082492359));
#147637=CARTESIAN_POINT('Ctrl Pts',(-7.47404443578264,1.23689319179786,
0.623425831516707));
#147638=CARTESIAN_POINT('Ctrl Pts',(-7.44541932874534,1.23263224516357,
0.621275069824));
#147639=CARTESIAN_POINT('Ctrl Pts',(-7.4168030670333,1.22830577227991,0.619135241647015));
#147640=CARTESIAN_POINT('Ctrl Pts',(-7.38819658462302,1.22391046499459,
0.61700718021737));
#147641=CARTESIAN_POINT('Ctrl Pts',(-7.36093098775273,1.21972118108181,
0.614978868444404));
#147642=CARTESIAN_POINT('Ctrl Pts',(-7.33367309711137,1.21547100864985,
0.61297154213858));
#147643=CARTESIAN_POINT('Ctrl Pts',(-7.3064274758196,1.21115091651599,0.610949205513832));
#147644=CARTESIAN_POINT('Ctrl Pts',(-7.27918117050091,1.20683071592216,
0.608926818116424));
#147645=CARTESIAN_POINT('Ctrl Pts',(-7.25194766417653,1.20243940507204,
0.606882331437855));
#147646=CARTESIAN_POINT('Ctrl Pts',(-7.22472833267014,1.19797317447885,
0.604814407458392));
#147647=CARTESIAN_POINT('Ctrl Pts',(-7.49113869911298,1.197203562,0.374945738428602));
#147648=CARTESIAN_POINT('Ctrl Pts',(-7.47083679599597,1.261925886,0.780562747110606));
#147649=CARTESIAN_POINT('Ctrl Pts',(-7.40685671966889,1.327100493,1.18161620345816));
#147650=CARTESIAN_POINT('Ctrl Pts',(-7.40466134597188,1.32933685510107,
1.19537770953492));
#147651=CARTESIAN_POINT('Ctrl Pts',(-7.40246597227482,1.33157321720217,
1.20913921561166));
#147652=CARTESIAN_POINT('Ctrl Pts',(-7.225116234,1.197203562,0.600162811));
#147653=CARTESIAN_POINT('Ctrl Pts',(-7.192619674,1.261925886,0.991375703));
#147654=CARTESIAN_POINT('Ctrl Pts',(-7.118071532,1.327100493,1.376792527));
#147655=CARTESIAN_POINT('Ctrl Pts',(-7.11551353208027,1.32933685510107,
1.39001748711844));
#147656=CARTESIAN_POINT('Ctrl Pts',(-7.11295553216052,1.33157321720217,
1.40324244723689));
#147657=CARTESIAN_POINT('Origin',(0.194482044550137,1.33927923986393,-0.0397062397596998));
#147658=CARTESIAN_POINT('Ctrl Pts',(-7.31468750940415,1.32841655815206,
1.65692939362537));
#147659=CARTESIAN_POINT('Ctrl Pts',(-7.31376968470208,1.32775852557603,
1.66096059431268));
#147660=CARTESIAN_POINT('Ctrl Pts',(-7.31285186,1.327100493,1.664991795));
#147661=CARTESIAN_POINT('Ctrl Pts',(-7.233504944,1.270212881,2.013493357));
#147662=CARTESIAN_POINT('Ctrl Pts',(-7.121376478,1.214285714,2.352869961));
#147663=CARTESIAN_POINT('Ctrl Pts',(-7.104280738,1.205758742,2.404613239));
#147664=CARTESIAN_POINT('Ctrl Pts',(-7.08643491800001,1.197204389,2.456102635));
#147665=CARTESIAN_POINT('Ctrl Pts',(-7.11958944241024,1.32841655815206,
1.36894487045972));
#147666=CARTESIAN_POINT('Ctrl Pts',(-7.11883048720513,1.32775852557603,
1.37286869872986));
#147667=CARTESIAN_POINT('Ctrl Pts',(-7.118071532,1.327100493,1.376792527));
#147668=CARTESIAN_POINT('Ctrl Pts',(-7.052459052,1.270212881,1.71601163));
#147669=CARTESIAN_POINT('Ctrl Pts',(-6.954885505,1.214285714,2.047453934));
#147670=CARTESIAN_POINT('Ctrl Pts',(-6.94000889,1.205758742,2.097987503));
#147671=CARTESIAN_POINT('Ctrl Pts',(-6.924399539,1.197204389,2.148299564));
#147672=CARTESIAN_POINT('',(-6.92580098254477,1.19797317427717,2.14377721438708));
#147673=CARTESIAN_POINT('Ctrl Pts',(-6.92580098244253,1.19797317417169,
2.1437772143375));
#147674=CARTESIAN_POINT('Ctrl Pts',(-6.93572590728547,1.20342302016956,
2.11171322408074));
#147675=CARTESIAN_POINT('Ctrl Pts',(-6.94542087193241,1.20886077952329,
2.07960383451994));
#147676=CARTESIAN_POINT('Ctrl Pts',(-6.95488550517671,1.21428571404043,
2.04745393395516));
#147677=CARTESIAN_POINT('Ctrl Pts',(-6.99658133912896,1.23818491548697,
1.90581961217231));
#147678=CARTESIAN_POINT('Ctrl Pts',(-7.03409051482239,1.26233334606286,
1.76242182670478));
#147679=CARTESIAN_POINT('Ctrl Pts',(-7.06723010831685,1.28666628008868,
1.61763982428158));
#147680=CARTESIAN_POINT('Ctrl Pts',(-7.08551496087135,1.30009203653179,
1.53775599688052));
#147681=CARTESIAN_POINT('Ctrl Pts',(-7.10247034740864,1.31357388715097,
1.45745126759499));
#147682=CARTESIAN_POINT('Ctrl Pts',(-7.11807153122654,1.32710049190844,
1.3767925342273));
#147683=CARTESIAN_POINT('Ctrl Pts',(-7.16528730493939,1.2368931917972,2.21554910463667));
#147684=CARTESIAN_POINT('Ctrl Pts',(-7.13779378704583,1.23263224509684,
2.20729507488363));
#147685=CARTESIAN_POINT('Ctrl Pts',(-7.11030655738309,1.22830577220572,
2.19905362431552));
#147686=CARTESIAN_POINT('Ctrl Pts',(-7.08282634888458,1.22391046491265,
2.19082576765584));
#147687=CARTESIAN_POINT('Ctrl Pts',(-7.05663423357138,1.21972118099716,
2.18298357932519));
#147688=CARTESIAN_POINT('Ctrl Pts',(-7.03044513306688,1.21547100856121,
2.17516354243795));
#147689=CARTESIAN_POINT('Ctrl Pts',(-7.00427124181747,1.21115091643179,
2.16733148377018));
#147690=CARTESIAN_POINT('Ctrl Pts',(-6.97809669344801,1.2068307158424,2.15949922847124));
#147691=CARTESIAN_POINT('Ctrl Pts',(-6.95193939554073,1.20243940499078,
2.1516481419384));
#147692=CARTESIAN_POINT('Ctrl Pts',(-6.9258009810858,1.19797317480768,2.14377721262108));
#147693=CARTESIAN_POINT('Ctrl Pts',(-7.23539778916891,1.197203562,1.97655309987448));
#147694=CARTESIAN_POINT('Ctrl Pts',(-7.12837486615898,1.261925886,2.36832269907289));
#147695=CARTESIAN_POINT('Ctrl Pts',(-6.97967596952128,1.327100493,2.74624592302433));
#147696=CARTESIAN_POINT('Ctrl Pts',(-6.97457360543554,1.32933685508188,
2.75921375216535));
#147697=CARTESIAN_POINT('Ctrl Pts',(-6.96947124134975,1.33157321716379,
2.77218158130638));
#147698=CARTESIAN_POINT('Ctrl Pts',(-6.927179768,1.197203562,2.139317756));
#147699=CARTESIAN_POINT('Ctrl Pts',(-6.811343751,1.261925886,2.514398508));
#147700=CARTESIAN_POINT('Ctrl Pts',(-6.65568528000001,1.327100493,2.874778854));
#147701=CARTESIAN_POINT('Ctrl Pts',(-6.65034410928501,1.32933685508188,
2.88714472742753));
#147702=CARTESIAN_POINT('Ctrl Pts',(-6.64500293857002,1.33157321716379,
2.89951060085513));
#147703=CARTESIAN_POINT('Origin',(0.181399943194743,1.3392793125703,-0.0805860116453921));
#147704=CARTESIAN_POINT('Ctrl Pts',(-6.78748333890469,1.32841655815206,
3.1906328984192));
#147705=CARTESIAN_POINT('Ctrl Pts',(-6.78572038345235,1.32775852557603,
3.1943725467096));
#147706=CARTESIAN_POINT('Ctrl Pts',(-6.783957428,1.327100493,3.198112195));
#147707=CARTESIAN_POINT('Ctrl Pts',(-6.631548065,1.270212881,3.521408744));
#147708=CARTESIAN_POINT('Ctrl Pts',(-6.449085162,1.214285714,3.828746606));
#147709=CARTESIAN_POINT('Ctrl Pts',(-6.421265836,1.205758742,3.875605075));
#147710=CARTESIAN_POINT('Ctrl Pts',(-6.392768543,1.197204389,3.922054354));
#147711=CARTESIAN_POINT('Ctrl Pts',(-6.6588547166992,1.32841655815206,2.86744097718164));
#147712=CARTESIAN_POINT('Ctrl Pts',(-6.6572699983496,1.32775852557603,2.87110991559082));
#147713=CARTESIAN_POINT('Ctrl Pts',(-6.65568528,1.327100493,2.874778854));
#147714=CARTESIAN_POINT('Ctrl Pts',(-6.518684703,1.270212881,3.191962459));
#147715=CARTESIAN_POINT('Ctrl Pts',(-6.352142073,1.214285714,3.494680397));
#147716=CARTESIAN_POINT('Ctrl Pts',(-6.326750041,1.205758742,3.540834488));
#147717=CARTESIAN_POINT('Ctrl Pts',(-6.300690023,1.197204389,3.586614732));
#147718=CARTESIAN_POINT('',(-6.30303087216245,1.19797317413244,3.58249938059888));
#147719=CARTESIAN_POINT('Ctrl Pts',(-6.3030308742562,1.19797317443891,3.58249938184616));
#147720=CARTESIAN_POINT('Ctrl Pts',(-6.3680251451983,1.21932945586211,3.46814879049661));
#147721=CARTESIAN_POINT('Ctrl Pts',(-6.42988717670857,1.24060038374378,
3.35207035709678));
#147722=CARTESIAN_POINT('Ctrl Pts',(-6.51805466472989,1.2728618049945,3.17518838572025));
#147723=CARTESIAN_POINT('Ctrl Pts',(-6.54669392265111,1.28366385007748,
3.11571107208527));
#147724=CARTESIAN_POINT('Ctrl Pts',(-6.58845011078457,1.29991103381072,
3.02587476984802));
#147725=CARTESIAN_POINT('Ctrl Pts',(-6.60217931457941,1.30533866114479,
2.99580058862257));
#147726=CARTESIAN_POINT('Ctrl Pts',(-6.62246861232924,1.31349012110038,
2.9505394645095));
#147727=CARTESIAN_POINT('Ctrl Pts',(-6.62918347355876,1.31620998855811,
2.93542162458502));
#147728=CARTESIAN_POINT('Ctrl Pts',(-6.63917917732145,1.32029216617391,
2.91270807353505));
#147729=CARTESIAN_POINT('Ctrl Pts',(-6.64249891522654,1.32165353785643,
2.90512936551094));
#147730=CARTESIAN_POINT('Ctrl Pts',(-6.64896140772192,1.32431471587872,
2.8903070010599));
#147731=CARTESIAN_POINT('Ctrl Pts',(-6.65056512628387,1.32497441921909,
2.8866330304428));
#147732=CARTESIAN_POINT('Ctrl Pts',(-6.65568527803507,1.3271004920459,2.87477886015856));
#147733=CARTESIAN_POINT('Ctrl Pts',(-6.52148930321594,1.23689319179727,
3.70407576429506));
#147734=CARTESIAN_POINT('Ctrl Pts',(-6.49641294089309,1.2326322451282,3.69010441533616));
#147735=CARTESIAN_POINT('Ctrl Pts',(-6.47134001560237,1.22830577222934,
3.67614670344645));
#147736=CARTESIAN_POINT('Ctrl Pts',(-6.4462710250368,1.22391046492801,3.66220377698956));
#147737=CARTESIAN_POINT('Ctrl Pts',(-6.42237710548012,1.21972118100729,
3.64891440411775));
#147738=CARTESIAN_POINT('Ctrl Pts',(-6.39848136835551,1.21547100856151,
3.63564731287302));
#147739=CARTESIAN_POINT('Ctrl Pts',(-6.37460306918195,1.21115091643823,
3.62237175053087));
#147740=CARTESIAN_POINT('Ctrl Pts',(-6.35072417052125,1.20683071585497,
3.60909585489325));
#147741=CARTESIAN_POINT('Ctrl Pts',(-6.32686616717161,1.20243940501151,
3.59580527662948));
#147742=CARTESIAN_POINT('Ctrl Pts',(-6.30303086975239,1.1979731744788,3.58249937757813));
#147743=CARTESIAN_POINT('Ctrl Pts',(-6.64133771968192,1.197203562,3.48573903474642));
#147744=CARTESIAN_POINT('Ctrl Pts',(-6.45259804968267,1.261925886,3.84534251319514));
#147745=CARTESIAN_POINT('Ctrl Pts',(-6.22613332948749,1.327100493,4.18246423546586));
#147746=CARTESIAN_POINT('Ctrl Pts',(-6.21836255600276,1.32933685505903,
4.1940320264149));
#147747=CARTESIAN_POINT('Ctrl Pts',(-6.21059178251804,1.33157321711808,
4.20559981736393));
#147748=CARTESIAN_POINT('Ctrl Pts',(-6.305336075,1.197203562,3.57844058));
#147749=CARTESIAN_POINT('Ctrl Pts',(-6.111576965,1.261925886,3.919850833));
#147750=CARTESIAN_POINT('Ctrl Pts',(-5.882086581,1.327100493,4.238343716));
#147751=CARTESIAN_POINT('Ctrl Pts',(-5.87421198671683,1.32933685505903,
4.2492722882216));
#147752=CARTESIAN_POINT('Ctrl Pts',(-5.86633739243366,1.33157321711808,
4.26020086044316));
#147753=CARTESIAN_POINT('Origin',(0.159834875138244,1.33927926526417,-0.117697270307699));
#147754=CARTESIAN_POINT('Ctrl Pts',(-5.94290399176302,1.32841655815206,
4.57514595584754));
#147755=CARTESIAN_POINT('Ctrl Pts',(-5.94037833938151,1.32775852557603,
4.57841918992377));
#147756=CARTESIAN_POINT('Ctrl Pts',(-5.937852687,1.327100493,4.581692424));
#147757=CARTESIAN_POINT('Ctrl Pts',(-5.71950736800001,1.270212881,4.864666971));
#147758=CARTESIAN_POINT('Ctrl Pts',(-5.475241792,1.214285714,5.125595314));
#147759=CARTESIAN_POINT('Ctrl Pts',(-5.43799968,1.205758742,5.165377926));
#147760=CARTESIAN_POINT('Ctrl Pts',(-5.400183416,1.197204389,5.20461517));
#147761=CARTESIAN_POINT('Ctrl Pts',(-5.88675934464409,1.32841655815206,
4.23185872984856));
#147762=CARTESIAN_POINT('Ctrl Pts',(-5.88442296282204,1.32775852557603,
4.23510122292428));
#147763=CARTESIAN_POINT('Ctrl Pts',(-5.882086581,1.327100493,4.238343716));
#147764=CARTESIAN_POINT('Ctrl Pts',(-5.680103902,1.270212881,4.518660671));
#147765=CARTESIAN_POINT('Ctrl Pts',(-5.452379538,1.214285714,4.77849949));
#147766=CARTESIAN_POINT('Ctrl Pts',(-5.41765939300001,1.205758742,4.818115986));
#147767=CARTESIAN_POINT('Ctrl Pts',(-5.382367244,1.197204389,4.85722378));
#147768=CARTESIAN_POINT('',(-5.38553804369929,1.19797317410539,4.85370785820065));
#147769=CARTESIAN_POINT('Ctrl Pts',(-5.38553804399106,1.19797317394536,
4.85370785842864));
#147770=CARTESIAN_POINT('Ctrl Pts',(-5.40800898235996,1.20342302011357,
4.8287747357346));
#147771=CARTESIAN_POINT('Ctrl Pts',(-5.43029027688968,1.2088607795396,4.80370385279805));
#147772=CARTESIAN_POINT('Ctrl Pts',(-5.45237953797633,1.21428571399169,
4.77849949019284));
#147773=CARTESIAN_POINT('Ctrl Pts',(-5.54969238256278,1.23818492097584,
4.66746326117485));
#147774=CARTESIAN_POINT('Ctrl Pts',(-5.64394597677683,1.26233335717944,
4.55306862269188));
#147775=CARTESIAN_POINT('Ctrl Pts',(-5.73481506164025,1.28666629688152,
4.43558296187854));
#147776=CARTESIAN_POINT('Ctrl Pts',(-5.78495227115069,1.30009204775908,
4.37076000036721));
#147777=CARTESIAN_POINT('Ctrl Pts',(-5.83405962295373,1.31357389275472,
4.30499681124347));
#147778=CARTESIAN_POINT('Ctrl Pts',(-5.8820865770368,1.32710049184556,4.23834372252408));
#147779=CARTESIAN_POINT('Ctrl Pts',(-5.57275370959136,1.23689319345816,
5.01940395762015));
#147780=CARTESIAN_POINT('Ctrl Pts',(-5.55126704606301,1.23263224511414,
5.00036857440288));
#147781=CARTESIAN_POINT('Ctrl Pts',(-5.5297808073759,1.22830577223117,4.98134724825955));
#147782=CARTESIAN_POINT('Ctrl Pts',(-5.50829523230249,1.2239104648033,4.96234120710719));
#147783=CARTESIAN_POINT('Ctrl Pts',(-5.49279024607477,1.22073860736394,
4.94862556741388));
#147784=CARTESIAN_POINT('Ctrl Pts',(-5.47728190210846,1.2175300135409,4.93492215050233));
#147785=CARTESIAN_POINT('Ctrl Pts',(-5.46178013446649,1.214285714,4.92121979118411));
#147786=CARTESIAN_POINT('Ctrl Pts',(-5.45680768340001,1.2132450507382,4.91682453042089));
#147787=CARTESIAN_POINT('Ctrl Pts',(-5.45183604222682,1.21220011140555,
4.91242936939489));
#147788=CARTESIAN_POINT('Ctrl Pts',(-5.44686554586363,1.21115091718982,
4.9080339427415));
#147789=CARTESIAN_POINT('Ctrl Pts',(-5.42639884426299,1.20683071587282,
4.88993516967154));
#147790=CARTESIAN_POINT('Ctrl Pts',(-5.40595570935509,1.20243940501851,
4.87182655211498));
#147791=CARTESIAN_POINT('Ctrl Pts',(-5.38553804287434,1.19797317367453,
4.85370785966772));
#147792=CARTESIAN_POINT('Ctrl Pts',(-5.73673607986545,1.197203562,4.83193568617798));
#147793=CARTESIAN_POINT('Ctrl Pts',(-5.47510492068508,1.261925886,5.1425583858957));
#147794=CARTESIAN_POINT('Ctrl Pts',(-5.18146361388604,1.327100493,5.42311516817074));
#147795=CARTESIAN_POINT('Ctrl Pts',(-5.17138778328492,1.32933685513441,
5.43274202429333));
#147796=CARTESIAN_POINT('Ctrl Pts',(-5.16131195268384,1.33157321726885,
5.44236888041577));
#147797=CARTESIAN_POINT('Ctrl Pts',(-5.388661875,1.197203562,4.850239499));
#147798=CARTESIAN_POINT('Ctrl Pts',(-5.126039633,1.261925886,5.14201528900001));
#147799=CARTESIAN_POINT('Ctrl Pts',(-4.83344805100001,1.327100493,5.403728337));
#147800=CARTESIAN_POINT('Ctrl Pts',(-4.82340824002217,1.32933685513441,
5.41270860059607));
#147801=CARTESIAN_POINT('Ctrl Pts',(-4.81336842904435,1.33157321726885,
5.42168886419204));
#147802=CARTESIAN_POINT('Origin',(0.130796662513575,1.33927930361659,-0.149305428651654));
#147803=CARTESIAN_POINT('Ctrl Pts',(-4.82044105921187,1.32841655815206,
5.74573027284353));
#147804=CARTESIAN_POINT('Ctrl Pts',(-4.81727080660594,1.32775852557603,
5.74838403992177));
#147805=CARTESIAN_POINT('Ctrl Pts',(-4.81410055400001,1.327100493,5.751037807));
#147806=CARTESIAN_POINT('Ctrl Pts',(-4.540028864,1.270212881,5.980458777));
#147807=CARTESIAN_POINT('Ctrl Pts',(-4.2453822,1.214285714,6.182776882));
#147808=CARTESIAN_POINT('Ctrl Pts',(-4.200458702,1.205758742,6.213623445));
#147809=CARTESIAN_POINT('Ctrl Pts',(-4.155091715,1.197204389,6.243813966));
#147810=CARTESIAN_POINT('Ctrl Pts',(-4.83940564834473,1.32841655815206,
5.39839947227737));
#147811=CARTESIAN_POINT('Ctrl Pts',(-4.83642684967236,1.32775852557603,
5.40106390463868));
#147812=CARTESIAN_POINT('Ctrl Pts',(-4.83344805100001,1.327100493,5.403728337));
#147813=CARTESIAN_POINT('Ctrl Pts',(-4.575927756,1.270212881,5.634071332));
#147814=CARTESIAN_POINT('Ctrl Pts',(-4.297669796,1.214285714,5.838881257));
#147815=CARTESIAN_POINT('Ctrl Pts',(-4.255245012,1.205758742,5.870107737));
#147816=CARTESIAN_POINT('Ctrl Pts',(-4.212370955,1.197204389,5.900714443));
#147817=CARTESIAN_POINT('',(-4.21622344285429,1.19797317421792,5.89796234909753));
#147818=CARTESIAN_POINT('Ctrl Pts',(-4.21622344432245,1.19797317438231,
5.89796235119718));
#147819=CARTESIAN_POINT('Ctrl Pts',(-4.32322526032568,1.21932946512229,
5.8214709182476));
#147820=CARTESIAN_POINT('Ctrl Pts',(-4.42810978821949,1.24060039327363,
5.74209617395239));
#147821=CARTESIAN_POINT('Ctrl Pts',(-4.58239917712483,1.27286180032043,
5.61858306591172));
#147822=CARTESIAN_POINT('Ctrl Pts',(-4.63336531931438,1.28366384098551,
5.57662824920296));
#147823=CARTESIAN_POINT('Ctrl Pts',(-4.70898353566001,1.29991103378527,
5.51262796203305));
#147824=CARTESIAN_POINT('Ctrl Pts',(-4.7340716445523,1.30533866113643,5.4910981173484));
#147825=CARTESIAN_POINT('Ctrl Pts',(-4.7714903652932,1.31349012111498,5.45853948853499));
#147826=CARTESIAN_POINT('Ctrl Pts',(-4.78393242454547,1.31620998858104,
5.4476384056337));
#147827=CARTESIAN_POINT('Ctrl Pts',(-4.80254145216897,1.32029216620858,
5.43122123203128));
#147828=CARTESIAN_POINT('Ctrl Pts',(-4.80873658160936,1.32165353789512,
5.42573690466597));
#147829=CARTESIAN_POINT('Ctrl Pts',(-4.82082553029863,1.32431471593174,
5.41499802113977));
#147830=CARTESIAN_POINT('Ctrl Pts',(-4.82382368759139,1.32497441960859,
5.41233699830146));
#147831=CARTESIAN_POINT('Ctrl Pts',(-4.83344804840376,1.32710049244325,
5.40372834061765));
#147832=CARTESIAN_POINT('Ctrl Pts',(-4.36344234639536,1.2368931917972,6.10003040032343));
#147833=CARTESIAN_POINT('Ctrl Pts',(-4.34655007361735,1.23263224514028,
6.07682105633262));
#147834=CARTESIAN_POINT('Ctrl Pts',(-4.32965519414463,1.22830577224801,
6.05362553204983));
#147835=CARTESIAN_POINT('Ctrl Pts',(-4.31275767749973,1.22391046495372,
6.03044507880315));
#147836=CARTESIAN_POINT('Ctrl Pts',(-4.29665220633116,1.21972118102563,
6.00835117416118));
#147837=CARTESIAN_POINT('Ctrl Pts',(-4.28053572977284,1.21547100857371,
5.98627672859718));
#147838=CARTESIAN_POINT('Ctrl Pts',(-4.26443863631162,1.21115091646208,
5.96420191693392));
#147839=CARTESIAN_POINT('Ctrl Pts',(-4.24834113871775,1.20683071589047,
5.94212655106177));
#147840=CARTESIAN_POINT('Ctrl Pts',(-4.23226877044292,1.20243940502681,
5.92004663319214));
#147841=CARTESIAN_POINT('Ctrl Pts',(-4.21622344160552,1.19797317447889,
5.89796234547384));
#147842=CARTESIAN_POINT('Ctrl Pts',(-4.56389103632907,1.197203562,5.95219639508915));
#147843=CARTESIAN_POINT('Ctrl Pts',(-4.24160196994146,1.261925886,6.19931394307092));
#147844=CARTESIAN_POINT('Ctrl Pts',(-3.8945144191289,1.327100493,6.41018726365432));
#147845=CARTESIAN_POINT('Ctrl Pts',(-3.88260466660897,1.32933685508828,
6.41742304337422));
#147846=CARTESIAN_POINT('Ctrl Pts',(-3.87069491408911,1.33157321717659,
6.42465882309414));
#147847=CARTESIAN_POINT('Ctrl Pts',(-4.220019834,1.197203562,5.89524661));
#147848=CARTESIAN_POINT('Ctrl Pts',(-3.900814385,1.261925886,6.123744826));
#147849=CARTESIAN_POINT('Ctrl Pts',(-3.558802862,1.327100493,6.316440627));
#147850=CARTESIAN_POINT('Ctrl Pts',(-3.54706728523169,1.32933685508828,
6.3230526742952));
#147851=CARTESIAN_POINT('Ctrl Pts',(-3.53533170846331,1.33157321717659,
6.32966472159023));
#147852=CARTESIAN_POINT('Origin',(0.0956423502217701,1.33927920723841,-0.173931980984078));
#147853=CARTESIAN_POINT('Ctrl Pts',(-3.47257965967507,1.32841655815206,
6.64765062822451));
#147854=CARTESIAN_POINT('Ctrl Pts',(-3.46891304433754,1.32775852557603,
6.64956084111226));
#147855=CARTESIAN_POINT('Ctrl Pts',(-3.465246429,1.327100493,6.651471054));
#147856=CARTESIAN_POINT('Ctrl Pts',(-3.148263656,1.270212881,6.81661097799999));
#147857=CARTESIAN_POINT('Ctrl Pts',(-2.817013256,1.214285714,6.950858675));
#147858=CARTESIAN_POINT('Ctrl Pts',(-2.766508945,1.205758742,6.971326838));
#147859=CARTESIAN_POINT('Ctrl Pts',(-2.715712542,1.197204389,6.99105896000001));
#147860=CARTESIAN_POINT('Ctrl Pts',(-3.56576672243298,1.32841655815206,
6.31251705551099));
#147861=CARTESIAN_POINT('Ctrl Pts',(-3.56228479221649,1.32775852557603,
6.31447884125549));
#147862=CARTESIAN_POINT('Ctrl Pts',(-3.558802862,1.327100493,6.31644062700001));
#147863=CARTESIAN_POINT('Ctrl Pts',(-3.257786313,1.270212881,6.486039079));
#147864=CARTESIAN_POINT('Ctrl Pts',(-2.94200579,1.214285714,6.626243425));
#147865=CARTESIAN_POINT('Ctrl Pts',(-2.893860104,1.205758742,6.647619773));
#147866=CARTESIAN_POINT('Ctrl Pts',(-2.845408881,1.197204389,6.668294257));
#147867=CARTESIAN_POINT('',(-2.8497629195214,1.19797317420091,6.66643467637103));
#147868=CARTESIAN_POINT('Ctrl Pts',(-2.8497629196775,1.19797317419801,6.66643467673501));
#147869=CARTESIAN_POINT('Ctrl Pts',(-2.88062613759635,1.20342302042728,
6.65324128928377));
#147870=CARTESIAN_POINT('Ctrl Pts',(-2.91137508290018,1.20886077977041,
6.6398432452646));
#147871=CARTESIAN_POINT('Ctrl Pts',(-2.94200579033808,1.21428571409209,
6.62624342524151));
#147872=CARTESIAN_POINT('Ctrl Pts',(-3.07694694590982,1.23818483384919,
6.56633049468183));
#147873=CARTESIAN_POINT('Ctrl Pts',(-3.21052177357322,1.26233318155733,
6.50208503886017));
#147874=CARTESIAN_POINT('Ctrl Pts',(-3.34232280477992,1.28666603166305,
6.43361315836795));
#147875=CARTESIAN_POINT('Ctrl Pts',(-3.41504504490551,1.30009187023295,
6.39583326780551));
#147876=CARTESIAN_POINT('Ctrl Pts',(-3.48722739618415,1.31357380373224,
6.3567676065478));
#147877=CARTESIAN_POINT('Ctrl Pts',(-3.55880285574871,1.3271004918186,6.3164406305221));
#147878=CARTESIAN_POINT('Ctrl Pts',(-2.95010126892948,1.23689319179796,
6.89542620162164));
#147879=CARTESIAN_POINT('Ctrl Pts',(-2.93859325105436,1.23263224511884,
6.86912813973384));
#147880=CARTESIAN_POINT('Ctrl Pts',(-2.92707971648569,1.22830577223091,
6.84284301422456));
#147881=CARTESIAN_POINT('Ctrl Pts',(-2.91556036655635,1.22391046494234,
6.81657204049203));
#147882=CARTESIAN_POINT('Ctrl Pts',(-2.9045809687198,1.21972118103039,6.7915324788907));
#147883=CARTESIAN_POINT('Ctrl Pts',(-2.89358663965225,1.21547100859607,
6.76650955559761));
#147884=CARTESIAN_POINT('Ctrl Pts',(-2.88261131919966,1.2111509165027,6.74149044156448));
#147885=CARTESIAN_POINT('Ctrl Pts',(-2.87163572320136,1.20683071594937,
6.716470699403));
#147886=CARTESIAN_POINT('Ctrl Pts',(-2.86068564753189,1.20243940510623,
6.69145191373865));
#147887=CARTESIAN_POINT('Ctrl Pts',(-2.84976291926544,1.19797317447889,
6.66643467296224));
#147888=CARTESIAN_POINT('Ctrl Pts',(-3.17764352089231,1.197203562,6.79413901620443));
#147889=CARTESIAN_POINT('Ctrl Pts',(-2.80976642584269,1.261925886,6.96619647104677));
#147890=CARTESIAN_POINT('Ctrl Pts',(-2.42546205857299,1.327100493,7.09752612644195));
#147891=CARTESIAN_POINT('Ctrl Pts',(-2.41227527010536,1.32933685518884,
7.10203249309483));
#147892=CARTESIAN_POINT('Ctrl Pts',(-2.39908848163773,1.33157321737771,
7.1065388597478));
#147893=CARTESIAN_POINT('Ctrl Pts',(-2.854054357,1.197203562,6.664598542));
#147894=CARTESIAN_POINT('Ctrl Pts',(-2.493191391,1.261925886,6.81913486));
#147895=CARTESIAN_POINT('Ctrl Pts',(-2.117752007,1.327100493,6.933803173));
#147896=CARTESIAN_POINT('Ctrl Pts',(-2.10486940622604,1.32933685518884,
6.93773783239047));
#147897=CARTESIAN_POINT('Ctrl Pts',(-2.09198680545205,1.33157321737771,
6.94167249178079));
#147898=CARTESIAN_POINT('Origin',(0.0560160757373296,1.33927925412577,-0.190425938296791));
#147899=CARTESIAN_POINT('Ctrl Pts',(-1.96234429440288,1.32841655815206,
7.23873422950782));
#147900=CARTESIAN_POINT('Ctrl Pts',(-1.95835276320144,1.32775852557603,
7.23981156875392));
#147901=CARTESIAN_POINT('Ctrl Pts',(-1.954361232,1.327100493,7.240888908));
#147902=CARTESIAN_POINT('Ctrl Pts',(-1.609289139,1.270212881,7.334026025));
#147903=CARTESIAN_POINT('Ctrl Pts',(-1.256923902,1.214285714,7.393926041));
#147904=CARTESIAN_POINT('Ctrl Pts',(-1.203200304,1.205758742,7.403058737));
#147905=CARTESIAN_POINT('Ctrl Pts',(-1.14934967,1.197204389,7.411409808));
#147906=CARTESIAN_POINT('Ctrl Pts',(-2.1253965081304,1.32841655815206,6.93146835656078));
#147907=CARTESIAN_POINT('Ctrl Pts',(-2.1215742575652,1.32775852557603,6.93263576478039));
#147908=CARTESIAN_POINT('Ctrl Pts',(-2.117752007,1.327100493,6.933803173));
#147909=CARTESIAN_POINT('Ctrl Pts',(-1.787314404,1.270212881,7.034726848));
#147910=CARTESIAN_POINT('Ctrl Pts',(-1.448776863,1.214285714,7.103769816));
#147911=CARTESIAN_POINT('Ctrl Pts',(-1.397161514,1.205758742,7.114296498));
#147912=CARTESIAN_POINT('Ctrl Pts',(-1.345398651,1.197204389,7.124072043));
#147913=CARTESIAN_POINT('',(-1.35005064865986,1.19797317421996,7.12319192784027));
#147914=CARTESIAN_POINT('Ctrl Pts',(-1.35005064910984,1.19797317440035,
7.12319193037176));
#147915=CARTESIAN_POINT('Ctrl Pts',(-1.47928071219414,1.21932945282983,
7.09869909662958));
#147916=CARTESIAN_POINT('Ctrl Pts',(-1.60779992972453,1.24060038228738,
7.07070040217712));
#147917=CARTESIAN_POINT('Ctrl Pts',(-1.7996910921651,1.27286180569472,7.02338735035821));
#147918=CARTESIAN_POINT('Ctrl Pts',(-1.86356310852297,1.2836638510999,7.0067103081862));
#147919=CARTESIAN_POINT('Ctrl Pts',(-1.95906530747638,1.29991103392261,
6.98037650178806));
#147920=CARTESIAN_POINT('Ctrl Pts',(-1.99087480528982,1.30533866122108,
6.97137076754721));
#147921=CARTESIAN_POINT('Ctrl Pts',(-2.03850612946368,1.31349012112496,
6.95753306948214));
#147922=CARTESIAN_POINT('Ctrl Pts',(-2.05437548237295,1.3162099885649,6.95286379971252));
#147923=CARTESIAN_POINT('Ctrl Pts',(-2.07815797049138,1.32029216615428,
6.94577770443496));
#147924=CARTESIAN_POINT('Ctrl Pts',(-2.08608332691097,1.32165353782778,
6.94340153107818));
#147925=CARTESIAN_POINT('Ctrl Pts',(-2.10156409950636,1.32431471582199,
6.93873120222481));
#147926=CARTESIAN_POINT('Ctrl Pts',(-2.10540248571035,1.32497441912895,
6.93757501752879));
#147927=CARTESIAN_POINT('Ctrl Pts',(-2.11775200093844,1.32710049202878,
6.93380317551267));
#147928=CARTESIAN_POINT('Ctrl Pts',(-1.39881673453843,1.23689319179734,
7.3683995371008));
#147929=CARTESIAN_POINT('Ctrl Pts',(-1.39323107349378,1.23263224512494,
7.34024242578046));
#147930=CARTESIAN_POINT('Ctrl Pts',(-1.38763724397553,1.22830577224665,
7.31209676235928));
#147931=CARTESIAN_POINT('Ctrl Pts',(-1.38203469282474,1.22391046496842,
7.28396366972702));
#147932=CARTESIAN_POINT('Ctrl Pts',(-1.37669475276434,1.21972118105452,
7.2571492731554));
#147933=CARTESIAN_POINT('Ctrl Pts',(-1.3713366537356,1.21547100862847,7.23034791613787));
#147934=CARTESIAN_POINT('Ctrl Pts',(-1.36599630035224,1.21115091648819,
7.20355436555754));
#147935=CARTESIAN_POINT('Ctrl Pts',(-1.36065581289424,1.20683071588789,
7.1767601422997));
#147936=CARTESIAN_POINT('Ctrl Pts',(-1.35534004338375,1.20243940501276,
7.14997233931328));
#147937=CARTESIAN_POINT('Ctrl Pts',(-1.35005064905439,1.1979731744787,7.12319192419207));
#147938=CARTESIAN_POINT('Ctrl Pts',(-1.64281292560465,1.197203562,7.31839524783592));
#147939=CARTESIAN_POINT('Ctrl Pts',(-1.24654932631938,1.261925886,7.40734739431066));
#147940=CARTESIAN_POINT('Ctrl Pts',(-0.842997787614654,1.327100493,7.45299255686116));
#147941=CARTESIAN_POINT('Ctrl Pts',(-0.829150563903604,1.3293368550922,
7.45455879739437));
#147942=CARTESIAN_POINT('Ctrl Pts',(-0.81530334019254,1.33157321718442,
7.45612503792762));
#147943=CARTESIAN_POINT('Ctrl Pts',(-1.354636469,1.197203562,7.122321253));
#147944=CARTESIAN_POINT('Ctrl Pts',(-0.968989539,1.261925886,7.195669727));
#147945=CARTESIAN_POINT('Ctrl Pts',(-0.577677421000001,1.327100493,7.226948789));
#147946=CARTESIAN_POINT('Ctrl Pts',(-0.564250173377097,1.3293368550922,
7.22802207983758));
#147947=CARTESIAN_POINT('Ctrl Pts',(-0.550822925754192,1.33157321718442,
7.22909537067527));
#147948=CARTESIAN_POINT('Origin',(0.013770519155653,1.33927931061205,-0.198015818953889));
#147949=CARTESIAN_POINT('Ctrl Pts',(-0.360351892041104,1.32841655815206,
7.49134266211465));
#147950=CARTESIAN_POINT('Ctrl Pts',(-0.356222084520552,1.32775852557603,
7.49153675255733));
#147951=CARTESIAN_POINT('Ctrl Pts',(-0.352092277,1.327100493,7.491730843));
#147952=CARTESIAN_POINT('Ctrl Pts',(0.00493395,1.270212881,7.508510167));
#147953=CARTESIAN_POINT('Ctrl Pts',(0.361937816,1.214285714,7.491261644));
#147954=CARTESIAN_POINT('Ctrl Pts',(0.416368646,1.205758742,7.488631836));
#147955=CARTESIAN_POINT('Ctrl Pts',(0.470755515,1.197204389,7.485211369));
#147956=CARTESIAN_POINT('Ctrl Pts',(-0.585645114452639,1.32841655815206,
7.22631190105834));
#147957=CARTESIAN_POINT('Ctrl Pts',(-0.58166126772632,1.32775852557603,
7.22663034502917));
#147958=CARTESIAN_POINT('Ctrl Pts',(-0.577677420999999,1.327100493,7.226948789));
#147959=CARTESIAN_POINT('Ctrl Pts',(-0.233269659,1.270212881,7.25447860700001));
#147960=CARTESIAN_POINT('Ctrl Pts',(0.112195259,1.214285714,7.249131826));
#147961=CARTESIAN_POINT('Ctrl Pts',(0.164866796,1.205758742,7.24831662500001));
#147962=CARTESIAN_POINT('Ctrl Pts',(0.217520925,1.197204389,7.246736138));
#147963=CARTESIAN_POINT('Ctrl Pts',(0.212788489902239,1.19797317430066,
7.24687664343713));
#147964=CARTESIAN_POINT('Ctrl Pts',(0.0813144678011027,1.21932946130748,
7.25073708450024));
#147965=CARTESIAN_POINT('Ctrl Pts',(-0.0502189469217795,1.24060039265624,
7.25102081258366));
#147966=CARTESIAN_POINT('Ctrl Pts',(-0.24779461253972,1.27286180050114,
7.24606484346783));
#147967=CARTESIAN_POINT('Ctrl Pts',(-0.31375837853524,1.28366384122101,
7.24350829985415));
#147968=CARTESIAN_POINT('Ctrl Pts',(-0.412688838702702,1.29991103383973,
7.23832030978511));
#147969=CARTESIAN_POINT('Ctrl Pts',(-0.445690615054844,1.30533866118305,
7.23636322632265));
#147970=CARTESIAN_POINT('Ctrl Pts',(-0.495183041810729,1.3134901211564,
7.2330883726259));
#147971=CARTESIAN_POINT('Ctrl Pts',(-0.511685133188544,1.31620998861918,
7.23193970955356));
#147972=CARTESIAN_POINT('Ctrl Pts',(-0.536434901191604,1.3202921662431,
7.23013181516178));
#147973=CARTESIAN_POINT('Ctrl Pts',(-0.544685774288287,1.32165353792807,
7.22951491276793));
#147974=CARTESIAN_POINT('Ctrl Pts',(-0.560808598010649,1.32431471597657,
7.22828168207693));
#147975=CARTESIAN_POINT('Ctrl Pts',(-0.564805791744118,1.32497441950331,
7.22797766780088));
#147976=CARTESIAN_POINT('Ctrl Pts',(-0.577677415696369,1.32710049223466,
7.22694879015694));
#147977=CARTESIAN_POINT('Ctrl Pts',(-1.356068566,4.559946053,7.122048725));
#147978=CARTESIAN_POINT('Ctrl Pts',(-0.967605761,4.62560150099999,7.196013706));
#147979=CARTESIAN_POINT('Ctrl Pts',(-0.573402753,4.690829639,7.227289207));
#147980=CARTESIAN_POINT('Ctrl Pts',(-1.16045022,4.559946053,7.409679837));
#147981=CARTESIAN_POINT('Ctrl Pts',(-0.756298953,4.62560150099999,7.472975072));
#147982=CARTESIAN_POINT('Ctrl Pts',(-0.347661035,4.690829639,7.491937787));
#147983=CARTESIAN_POINT('',(-0.578090309697558,4.69005394722626,7.22691577233048));
#147984=CARTESIAN_POINT('Ctrl Pts',(-0.578090316489442,4.69005394650282,
7.22691577311486));
#147985=CARTESIAN_POINT('Ctrl Pts',(-0.581541766825931,4.6831682404923,
7.2683793815881));
#147986=CARTESIAN_POINT('Ctrl Pts',(-0.584975039978215,4.67644844968185,
7.30989694698229));
#147987=CARTESIAN_POINT('Ctrl Pts',(-0.591801078376235,4.66333077530932,
7.39293693911767));
#147988=CARTESIAN_POINT('Ctrl Pts',(-0.595197661045881,4.65692555576185,
7.43450584453084));
#147989=CARTESIAN_POINT('Ctrl Pts',(-0.598575746204779,4.65066950057451,
7.47607564640176));
#147990=CARTESIAN_POINT('Origin',(0.0382219043895207,4.55357680227839,-0.194944154157056));
#147991=CARTESIAN_POINT('Ctrl Pts',(-2.122659554,4.690837228,6.932302389));
#147992=CARTESIAN_POINT('Ctrl Pts',(-1.744538893,4.625180297,7.04808231200001));
#147993=CARTESIAN_POINT('Ctrl Pts',(-1.356068566,4.559946053,7.122048725));
#147994=CARTESIAN_POINT('Ctrl Pts',(-1.34263297146768,4.55768986818721,
7.12460691970628));
#147995=CARTESIAN_POINT('Ctrl Pts',(-1.32919737693536,4.55543368337429,
7.12716511441254));
#147996=CARTESIAN_POINT('Ctrl Pts',(-2.4304970474152,4.690837228,7.09581366670855));
#147997=CARTESIAN_POINT('Ctrl Pts',(-2.04345770499716,4.625180297,7.22838450695184));
#147998=CARTESIAN_POINT('Ctrl Pts',(-1.64429532972506,4.559946053,7.31807217462192));
#147999=CARTESIAN_POINT('Ctrl Pts',(-1.63048994111758,4.55768986818721,
7.32117410301548));
#148000=CARTESIAN_POINT('Ctrl Pts',(-1.6166845525101,4.55543368337429,7.32427603140891));
#148001=CARTESIAN_POINT('',(-2.11814814960832,4.69005394728041,6.93368216963888));
#148002=CARTESIAN_POINT('Origin',(0.0590761079533894,4.69642264267046,-0.189672411948689));
#148003=CARTESIAN_POINT('Ctrl Pts',(-2.19171665082087,4.6506695006115,7.17261306095222));
#148004=CARTESIAN_POINT('Ctrl Pts',(-2.17948126558908,4.65692555540451,
7.13274132882446));
#148005=CARTESIAN_POINT('Ctrl Pts',(-2.16722800709513,4.66333077501547,
7.09287444557865));
#148006=CARTESIAN_POINT('Ctrl Pts',(-2.14271041380535,4.67644844946209,
7.01324327791012));
#148007=CARTESIAN_POINT('Ctrl Pts',(-2.13043235929365,4.6831682402748,6.97343442208798));
#148008=CARTESIAN_POINT('Ctrl Pts',(-2.11814815155723,4.69005394634728,
6.93368216887499));
#148009=CARTESIAN_POINT('Ctrl Pts',(-2.855394386,4.559946053,6.664024527));
#148010=CARTESIAN_POINT('Ctrl Pts',(-2.491913911,4.625601501,6.819768268));
#148011=CARTESIAN_POINT('Ctrl Pts',(-2.113650457,4.690829639,6.93505456));
#148012=CARTESIAN_POINT('Ctrl Pts',(-2.726181675,4.559946053,6.986983146));
#148013=CARTESIAN_POINT('Ctrl Pts',(-2.345085845,4.62560150099999,7.135679149));
#148014=CARTESIAN_POINT('Ctrl Pts',(-1.950078078,4.690829639,7.24204359900001));
#148015=CARTESIAN_POINT('Origin',(0.0792368453391867,4.55357610284578,-0.182173073954132));
#148016=CARTESIAN_POINT('Ctrl Pts',(-3.563273049,4.690837228,6.313919953));
#148017=CARTESIAN_POINT('Ctrl Pts',(-3.2188819,4.625180297,6.508277771));
#148018=CARTESIAN_POINT('Ctrl Pts',(-2.855394386,4.559946053,6.664024527));
#148019=CARTESIAN_POINT('Ctrl Pts',(-2.84282284356996,4.55768986802873,
6.66941116856532));
#148020=CARTESIAN_POINT('Ctrl Pts',(-2.83025130113985,4.55543368305734,
6.67479781013075));
#148021=CARTESIAN_POINT('Ctrl Pts',(-3.89906356435433,4.690837228,6.40743246670585));
#148022=CARTESIAN_POINT('Ctrl Pts',(-3.54957179938072,4.625180297,6.62010589188558));
#148023=CARTESIAN_POINT('Ctrl Pts',(-3.17902181502321,4.559946053,6.7935048240134));
#148024=CARTESIAN_POINT('Ctrl Pts',(-3.16620601070701,4.55768986802873,
6.79950198195862));
#148025=CARTESIAN_POINT('Ctrl Pts',(-3.15339020639086,4.55543368305734,
6.8054991399038));
#148026=CARTESIAN_POINT('',(-3.55916373143488,4.69005394733074,6.31623729381741));
#148027=CARTESIAN_POINT('Origin',(0.0984688797849448,4.69642269253522,-0.172538298857151));
#148028=CARTESIAN_POINT('Ctrl Pts',(-3.68237532007636,4.65066950063932,
6.53376706035625));
#148029=CARTESIAN_POINT('Ctrl Pts',(-3.66185475179114,4.65692555415041,
6.49745776078882));
#148030=CARTESIAN_POINT('Ctrl Pts',(-3.64131776398155,4.66333077444185,
6.46115702742171));
#148031=CARTESIAN_POINT('Ctrl Pts',(-3.60025502954068,4.67644844950924,
6.38865814667701));
#148032=CARTESIAN_POINT('Ctrl Pts',(-3.57970630213485,4.68316824029048,
6.35241941876875));
#148033=CARTESIAN_POINT('Ctrl Pts',(-3.55916373320053,4.69005394637357,
6.31623729263279));
#148034=CARTESIAN_POINT('Ctrl Pts',(-4.221205138,4.559946053,5.894397949));
#148035=CARTESIAN_POINT('Ctrl Pts',(-3.899702935,4.625601501,6.124638046));
#148036=CARTESIAN_POINT('Ctrl Pts',(-3.555066216,4.690829639,6.318544469));
#148037=CARTESIAN_POINT('Ctrl Pts',(-4.164439905,4.559946053,6.237582888));
#148038=CARTESIAN_POINT('Ctrl Pts',(-3.824219129,4.62560150099999,6.464726799));
#148039=CARTESIAN_POINT('Ctrl Pts',(-3.461311636,4.690829639,6.653519501));
#148040=CARTESIAN_POINT('Origin',(0.116546219047508,4.55357609998137,-0.160880490426645));
#148041=CARTESIAN_POINT('Ctrl Pts',(-4.837271857,4.690837228,5.400305637));
#148042=CARTESIAN_POINT('Ctrl Pts',(-4.54271356700001,4.625180297,5.664153394));
#148043=CARTESIAN_POINT('Ctrl Pts',(-4.221205138,4.559946053,5.894397949));
#148044=CARTESIAN_POINT('Ctrl Pts',(-4.21008548002964,4.55768986804247,
5.90236116386531));
#148045=CARTESIAN_POINT('Ctrl Pts',(-4.19896582205929,4.55543368308483,
5.91032437873072));
#148046=CARTESIAN_POINT('Ctrl Pts',(-5.18531420308181,4.690837228,5.41944684537354));
#148047=CARTESIAN_POINT('Ctrl Pts',(-4.8897118604343,4.625180297,5.70227848261148));
#148048=CARTESIAN_POINT('Ctrl Pts',(-4.56510077445871,4.559946053,5.95128073642111));
#148049=CARTESIAN_POINT('Ctrl Pts',(-4.55387380830834,4.55768986804247,
5.95989270315809));
#148050=CARTESIAN_POINT('Ctrl Pts',(-4.54264684215807,4.55543368308483,
5.9685046698951));
#148051=CARTESIAN_POINT('',(-4.83375677188436,4.69005394729794,5.40345218106921));
#148052=CARTESIAN_POINT('Origin',(0.133257365750999,4.6964226808519,-0.147336525368674));
#148053=CARTESIAN_POINT('Ctrl Pts',(-5.00085021302195,4.65066950061665,
5.58940937375438));
#148054=CARTESIAN_POINT('Ctrl Pts',(-4.97300397526571,4.65692555475222,
5.55836027793321));
#148055=CARTESIAN_POINT('Ctrl Pts',(-4.94514354744579,4.66333077475262,
5.52732308234134));
#148056=CARTESIAN_POINT('Ctrl Pts',(-4.8894557215615,4.6764484495377,5.46534646051497));
#148057=CARTESIAN_POINT('Ctrl Pts',(-4.86159715617397,4.68316824040816,
5.43437234245755));
#148058=CARTESIAN_POINT('Ctrl Pts',(-4.83375677343035,4.69005394646861,
5.40345217949458));
#148059=CARTESIAN_POINT('Ctrl Pts',(-5.38963703,4.559946053,4.849155874));
#148060=CARTESIAN_POINT('Ctrl Pts',(-5.125146184,4.625601501,5.143126555));
#148061=CARTESIAN_POINT('Ctrl Pts',(-4.830251029,4.690829639,5.406586261));
#148062=CARTESIAN_POINT('Ctrl Pts',(-5.407973553,4.559946053,5.196520186));
#148063=CARTESIAN_POINT('Ctrl Pts',(-5.124536177,4.62560150099999,5.491491009));
#148064=CARTESIAN_POINT('Ctrl Pts',(-4.81069811,4.690829639,5.753884227));
#148065=CARTESIAN_POINT('Origin',(0.148405940700649,4.55357613816343,-0.132065186293442));
#148066=CARTESIAN_POINT('Ctrl Pts',(-5.88508521,4.690837228,4.234179032));
#148067=CARTESIAN_POINT('Ctrl Pts',(-5.65413299700001,4.625180297,4.5551795));
#148068=CARTESIAN_POINT('Ctrl Pts',(-5.38963702999999,4.559946053,4.849155874));
#148069=CARTESIAN_POINT('Ctrl Pts',(-5.38048919998591,4.55768986821966,
4.85932331030542));
#148070=CARTESIAN_POINT('Ctrl Pts',(-5.37134136997195,4.55543368343922,
4.86949074661071));
#148071=CARTESIAN_POINT('Ctrl Pts',(-6.22910531267341,4.690837228,4.17805391238254));
#148072=CARTESIAN_POINT('Ctrl Pts',(-6.00121443024345,4.625180297,4.51781886922404));
#148073=CARTESIAN_POINT('Ctrl Pts',(-5.73772069546451,4.559946053,4.83078137711897));
#148074=CARTESIAN_POINT('Ctrl Pts',(-5.72860752854982,4.55768986821967,
4.84160546587721));
#148075=CARTESIAN_POINT('Ctrl Pts',(-5.71949436163511,4.55543368343922,
4.85242955463548));
#148076=CARTESIAN_POINT('',(-5.8823287196018,4.69005394733027,4.23800765141649));
#148077=CARTESIAN_POINT('Origin',(0.161815073408853,4.69642264836266,-0.115245659539057));
#148078=CARTESIAN_POINT('Ctrl Pts',(-6.08549090773312,4.6506695005771,4.38369711687511));
#148079=CARTESIAN_POINT('Ctrl Pts',(-6.05162106171909,4.65692555473231,
4.35936004960284));
#148080=CARTESIAN_POINT('Ctrl Pts',(-6.01773991589036,4.663330774701,4.33503765500821));
#148081=CARTESIAN_POINT('Ctrl Pts',(-5.95003089877631,4.67644844951874,
4.2864812486659));
#148082=CARTESIAN_POINT('Ctrl Pts',(-5.91616513215525,4.68316824025294,
4.26222005696167));
#148083=CARTESIAN_POINT('Ctrl Pts',(-5.88232872077917,4.69005394638316,
4.23800764950179));
#148084=CARTESIAN_POINT('Ctrl Pts',(-6.306055484,4.559946053,3.577172659));
#148085=CARTESIAN_POINT('Ctrl Pts',(-6.110943294,4.625601501,3.921128183));
#148086=CARTESIAN_POINT('Ctrl Pts',(-5.879578673,4.690829639,4.241822088));
#148087=CARTESIAN_POINT('Ctrl Pts',(-6.398636369,4.559946053,3.912473977));
#148088=CARTESIAN_POINT('Ctrl Pts',(-6.185235608,4.62560150099999,4.261479203));
#148089=CARTESIAN_POINT('Ctrl Pts',(-5.935141687,4.690829639,4.585203721));
#148090=CARTESIAN_POINT('Origin',(0.173326479962918,4.55357612721855,-0.0970747065674799));
#148091=CARTESIAN_POINT('Ctrl Pts',(-6.657718518,4.690837228,2.870066921));
#148092=CARTESIAN_POINT('Ctrl Pts',(-6.501171452,4.625180297,3.233210475));
#148093=CARTESIAN_POINT('Ctrl Pts',(-6.306055484,4.559946053,3.577172659));
#148094=CARTESIAN_POINT('Ctrl Pts',(-6.29930722346074,4.55768986823408,
3.58906889925688));
#148095=CARTESIAN_POINT('Ctrl Pts',(-6.29255896292154,4.55543368346804,
3.60096513951376));
#148096=CARTESIAN_POINT('Ctrl Pts',(-6.98163038082113,4.690837228,2.7412998228952));
#148097=CARTESIAN_POINT('Ctrl Pts',(-6.83210688278231,4.625180297,3.12211106708368));
#148098=CARTESIAN_POINT('Ctrl Pts',(-6.64205117335276,4.559946053,3.48440004939021));
#148099=CARTESIAN_POINT('Ctrl Pts',(-6.63547792638916,4.55768986823408,
3.49693013838376));
#148100=CARTESIAN_POINT('Ctrl Pts',(-6.62890467942558,4.55543368346802,
3.50946022737734));
#148101=CARTESIAN_POINT('',(-6.65584951362986,4.69005394733147,2.87439859321748));
#148102=CARTESIAN_POINT('Origin',(0.182806036133766,4.69642265498479,-0.0777656857180081));
#148103=CARTESIAN_POINT('Ctrl Pts',(-6.885580810478,4.65066950062011,2.97300805530623));
#148104=CARTESIAN_POINT('Ctrl Pts',(-6.84727107633065,4.65692555415897,
2.95652099241279));
#148105=CARTESIAN_POINT('Ctrl Pts',(-6.8089534551083,4.66333077442245,2.9400506858322));
#148106=CARTESIAN_POINT('Ctrl Pts',(-6.73238924394089,4.6764484494647,2.90718493774101));
#148107=CARTESIAN_POINT('Ctrl Pts',(-6.69409980081816,4.68316824025995,
2.89077109770168));
#148108=CARTESIAN_POINT('Ctrl Pts',(-6.65584951439294,4.69005394636003,
2.87439859102618));
#148109=CARTESIAN_POINT('Ctrl Pts',(-6.927609792,4.559946053,2.137924827));
#148110=CARTESIAN_POINT('Ctrl Pts',(-6.810999487,4.625601501,2.515782215));
#148111=CARTESIAN_POINT('Ctrl Pts',(-6.653983753,4.690829639,2.87871503));
#148112=CARTESIAN_POINT('Ctrl Pts',(-7.090106059,4.559946053,2.445484832));
#148113=CARTESIAN_POINT('Ctrl Pts',(-6.956720297,4.62560150099999,2.832205366));
#148114=CARTESIAN_POINT('Ctrl Pts',(-6.782064634,4.690829639,3.202124185));
#148115=CARTESIAN_POINT('Origin',(0.190142418624709,4.5535761338538,-0.0575450919829879));
#148116=CARTESIAN_POINT('Ctrl Pts',(-7.11904430900001,4.690837228,1.371753671));
#148117=CARTESIAN_POINT('Ctrl Pts',(-7.044222355,4.625180297,1.760060122));
#148118=CARTESIAN_POINT('Ctrl Pts',(-6.927609792,4.559946053,2.137924827));
#148119=CARTESIAN_POINT('Ctrl Pts',(-6.92357664196433,4.55768986818812,
2.15099361658192));
#148120=CARTESIAN_POINT('Ctrl Pts',(-6.91954349192857,4.55543368337614,
2.16406240616389));
#148121=CARTESIAN_POINT('Ctrl Pts',(-7.40770217163727,4.690837228,1.17636559945564));
#148122=CARTESIAN_POINT('Ctrl Pts',(-7.34353761129185,4.625180297,1.58041682072324));
#148123=CARTESIAN_POINT('Ctrl Pts',(-7.23580672022578,4.559946053,1.97509204848342));
#148124=CARTESIAN_POINT('Ctrl Pts',(-7.23208075077643,4.55768986818812,
1.98874224506581));
#148125=CARTESIAN_POINT('Ctrl Pts',(-7.22835478132707,4.55543368337614,
2.00239244164813));
#148126=CARTESIAN_POINT('',(-7.11815018154454,4.69005394731783,1.37638585135298));
#148127=CARTESIAN_POINT('Origin',(0.195249511375112,4.69642264758951,-0.0366496854463455));
#148128=CARTESIAN_POINT('Ctrl Pts',(-7.36370860838712,4.65066950056237,
1.42330444072716));
#148129=CARTESIAN_POINT('Ctrl Pts',(-7.32275029711851,4.6569255550511,1.41543829550915));
#148130=CARTESIAN_POINT('Ctrl Pts',(-7.28178789480078,4.66333077483531,
1.40759021220586));
#148131=CARTESIAN_POINT('Ctrl Pts',(-7.19994855029538,4.67644844951645,
1.39195189002702));
#148132=CARTESIAN_POINT('Ctrl Pts',(-7.15902580303485,4.68316824025603,
1.3841528952024));
#148133=CARTESIAN_POINT('Ctrl Pts',(-7.11815018169184,4.69005394643278,
1.37638584979319));
#148134=CARTESIAN_POINT('Ctrl Pts',(-7.225236766,4.559946053,0.598710006));
#148135=CARTESIAN_POINT('Ctrl Pts',(-7.192580914,4.625601501,0.992801067));
#148136=CARTESIAN_POINT('Ctrl Pts',(-7.11725594700001,4.690829639,1.381002455));
#148137=CARTESIAN_POINT('Ctrl Pts',(-7.450050271,4.559946053,0.864147535));
#148138=CARTESIAN_POINT('Ctrl Pts',(-7.402916477,4.625601501,1.270500754));
#148139=CARTESIAN_POINT('Ctrl Pts',(-7.311865778,4.690829639,1.669316881));
#148140=CARTESIAN_POINT('Origin',(0.198067364172025,4.55357616421649,-0.015324714123944));
#148141=CARTESIAN_POINT('Ctrl Pts',(-7.24749149900001,4.690837228,-0.190701257));
#148142=CARTESIAN_POINT('Ctrl Pts',(-7.25789325,4.625180297,0.204611314));
#148143=CARTESIAN_POINT('Ctrl Pts',(-7.225236766,4.559946053,0.598710006));
#148144=CARTESIAN_POINT('Ctrl Pts',(-7.22410731225297,4.55768986824605,
0.612340262226292));
#148145=CARTESIAN_POINT('Ctrl Pts',(-7.2229778585061,4.55543368349199,0.625970518452585));
#148146=CARTESIAN_POINT('Ctrl Pts',(-7.48739804276081,4.690837228,-0.443574171164436));
#148147=CARTESIAN_POINT('Ctrl Pts',(-7.51159268225325,4.625180297,-0.035175959275478));
#148148=CARTESIAN_POINT('Ctrl Pts',(-7.49122398729528,4.559946053,0.37343093749525));
#148149=CARTESIAN_POINT('Ctrl Pts',(-7.49051951773749,4.55768986824605,
0.387562972977406));
#148150=CARTESIAN_POINT('Ctrl Pts',(-7.48981504817983,4.55543368349199,
0.401695008459564));
#148151=CARTESIAN_POINT('',(-7.24761405802198,4.69005394733152,-0.185985163060938));
#148152=CARTESIAN_POINT('Origin',(0.198563202849756,4.69642265207484,0.00618004660821885));
#148153=CARTESIAN_POINT('Ctrl Pts',(-7.49751757546059,4.65066950057572,
-0.19295130721211));
#148154=CARTESIAN_POINT('Ctrl Pts',(-7.4558258610395,4.65692555461459,-0.191828720249321));
#148155=CARTESIAN_POINT('Ctrl Pts',(-7.41413402924507,4.66333077464523,
-0.190687614096624));
#148156=CARTESIAN_POINT('Ctrl Pts',(-7.33084626478274,4.67644844950723,
-0.188367281286426));
#148157=CARTESIAN_POINT('Ctrl Pts',(-7.28920371489588,4.68316824028114,
-0.187186759113336));
#148158=CARTESIAN_POINT('Ctrl Pts',(-7.24761405780493,4.69005394640255,
-0.185985165250032));
#148159=CARTESIAN_POINT('Ctrl Pts',(-7.18501969900001,4.559946053,-0.96849983));
#148160=CARTESIAN_POINT('Ctrl Pts',(-7.237845252,4.625601501,-0.576602356));
#148161=CARTESIAN_POINT('Ctrl Pts',(-7.247733164,4.690829639,-0.181284259));
#148162=CARTESIAN_POINT('Ctrl Pts',(-7.461638412,4.559946053,-0.75759634));
#148163=CARTESIAN_POINT('Ctrl Pts',(-7.50296051,4.625601501,-0.350611062));
#148164=CARTESIAN_POINT('Ctrl Pts',(-7.499772204,4.690829639,0.058454175));
#148165=CARTESIAN_POINT('Origin',(0.196730823850354,4.55357617794149,0.0276121826918264));
#148166=CARTESIAN_POINT('Ctrl Pts',(-7.037054042,4.690837228,-1.744239205));
#148167=CARTESIAN_POINT('Ctrl Pts',(-7.132193124,4.625180297,-1.360404892));
#148168=CARTESIAN_POINT('Ctrl Pts',(-7.185019699,4.559946053,-0.96849983));
#148169=CARTESIAN_POINT('Ctrl Pts',(-7.18684675352726,4.55768986810005,
-0.954945441554801));
#148170=CARTESIAN_POINT('Ctrl Pts',(-7.1886738080545,4.55543368319999,-0.941391053109596));
#148171=CARTESIAN_POINT('Ctrl Pts',(-7.21699150217716,4.690837228,-2.04277290610587));
#148172=CARTESIAN_POINT('Ctrl Pts',(-7.32841402767017,4.625180297,-1.64912395008705));
#148173=CARTESIAN_POINT('Ctrl Pts',(-7.39635994642545,4.559946053,-1.24569138826482));
#148174=CARTESIAN_POINT('Ctrl Pts',(-7.39870991703153,4.55768986810005,
-1.23173831088819));
#148175=CARTESIAN_POINT('Ctrl Pts',(-7.40105988763752,4.55543368319998,
-1.21778523351154));
#148176=CARTESIAN_POINT('',(-7.03818755607615,4.69005394729387,-1.73965971772344));
#148177=CARTESIAN_POINT('Origin',(0.192592371211763,4.69642264078062,0.0487207763574957));
#148178=CARTESIAN_POINT('Ctrl Pts',(-7.28075095342903,4.65066950062243,
-1.80018486679472));
#148179=CARTESIAN_POINT('Ctrl Pts',(-7.24027528496446,4.65692555561415,
-1.79012603745073));
#148180=CARTESIAN_POINT('Ctrl Pts',(-7.19980349256061,4.66333077513083,
-1.78004909900782));
#148181=CARTESIAN_POINT('Ctrl Pts',(-7.11896175532797,4.67644844955349,
-1.7598786072466));
#148182=CARTESIAN_POINT('Ctrl Pts',(-7.07854656244168,4.683168240323,-1.74977376756505));
#148183=CARTESIAN_POINT('Ctrl Pts',(-7.03818755555002,4.69005394643001,
-1.7396597192348));
#148184=CARTESIAN_POINT('Ctrl Pts',(-6.808839097,4.559946053,-2.49042369));
#148185=CARTESIAN_POINT('Ctrl Pts',(-6.94467599,4.625601501,-2.119044493));
#148186=CARTESIAN_POINT('Ctrl Pts',(-7.039314433,4.690829639,-1.735094322));
#148187=CARTESIAN_POINT('Ctrl Pts',(-7.124328633,4.559946053,-2.343915853));
#148188=CARTESIAN_POINT('Ctrl Pts',(-7.252174449,4.625601501,-1.955328694));
#148189=CARTESIAN_POINT('Ctrl Pts',(-7.336997617,4.690829639,-1.555141784));
#148190=CARTESIAN_POINT('Origin',(0.186195839981054,4.55357613693572,0.0692580166496981));
#148191=CARTESIAN_POINT('Ctrl Pts',(-6.49757176,4.690837228,-3.216218467));
#148192=CARTESIAN_POINT('Ctrl Pts',(-6.672999573,4.625180297,-2.861810077));
#148193=CARTESIAN_POINT('Ctrl Pts',(-6.808839097,4.559946053,-2.49042369));
#148194=CARTESIAN_POINT('Ctrl Pts',(-6.81353722888779,4.55768986810709,
-2.47757895839265));
#148195=CARTESIAN_POINT('Ctrl Pts',(-6.81823536077545,4.55543368321406,
-2.46473422678533));
#148196=CARTESIAN_POINT('Ctrl Pts',(-6.60912646082549,4.690837228,-3.546453851052));
#148197=CARTESIAN_POINT('Ctrl Pts',(-6.80256687881719,4.625180297,-3.18596073831595));
#148198=CARTESIAN_POINT('Ctrl Pts',(-6.95565033526412,4.559946053,-2.80656656937056));
#148199=CARTESIAN_POINT('Ctrl Pts',(-6.96094486403635,4.55768986810709,
-2.79344488143564));
#148200=CARTESIAN_POINT('Ctrl Pts',(-6.96623939280858,4.55543368321407,
-2.78032319350065));
#148201=CARTESIAN_POINT('',(-6.49966322680666,4.69005394729517,-3.21198971733521));
#148202=CARTESIAN_POINT('Origin',(0.177616129444476,4.6964226569031,0.0889833830679743));
#148203=CARTESIAN_POINT('Ctrl Pts',(-6.72354450891878,4.65066950062616,
-3.32324378223984));
#148204=CARTESIAN_POINT('Ctrl Pts',(-6.68617749493491,4.65692555480842,
-3.3047190529955));
#148205=CARTESIAN_POINT('Ctrl Pts',(-6.64881815156918,4.6633307747993,-3.28617746743296));
#148206=CARTESIAN_POINT('Ctrl Pts',(-6.57420250684019,4.67644844959452,
-3.24909996596324));
#148207=CARTESIAN_POINT('Ctrl Pts',(-6.53690444003399,4.68316824048538,
-3.23054329983003));
#148208=CARTESIAN_POINT('Ctrl Pts',(-6.49966322605803,4.69005394657573,
-3.21198971904582));
#148209=CARTESIAN_POINT('Ctrl Pts',(-6.114284746,4.559946053,-3.895898106));
#148210=CARTESIAN_POINT('Ctrl Pts',(-6.326781397,4.625601501,-3.562402465));
#148211=CARTESIAN_POINT('Ctrl Pts',(-6.501745184,4.690829639,-3.207773304));
#148212=CARTESIAN_POINT('Ctrl Pts',(-6.453893166,4.559946053,-3.820636465));
#148213=CARTESIAN_POINT('Ctrl Pts',(-6.66228477,4.625601501,-3.468617329));
#148214=CARTESIAN_POINT('Ctrl Pts',(-6.831153176,4.690829639,-3.096021041));
#148215=CARTESIAN_POINT('Origin',(0.166954016505535,4.55357622549867,0.107665247459791));
#148216=CARTESIAN_POINT('Ctrl Pts',(-5.654270243,4.690837228,-4.537810928));
#148217=CARTESIAN_POINT('Ctrl Pts',(-5.90178398,4.625180297,-4.229400204));
#148218=CARTESIAN_POINT('Ctrl Pts',(-6.114284746,4.559946053,-3.895898106));
#148219=CARTESIAN_POINT('Ctrl Pts',(-6.1216342760813,4.55768986801004,-3.88436363604226));
#148220=CARTESIAN_POINT('Ctrl Pts',(-6.12898380616261,4.55543368301997,
-3.87282916608446));
#148221=CARTESIAN_POINT('Ctrl Pts',(-5.69222601069263,4.690837228,-4.88430655563121));
#148222=CARTESIAN_POINT('Ctrl Pts',(-5.9586392635831,4.625180297,-4.57382554315651));
#148223=CARTESIAN_POINT('Ctrl Pts',(-6.1897022444045,4.559946053,-4.2362098168995));
#148224=CARTESIAN_POINT('Ctrl Pts',(-6.19769376537727,4.55768986801004,
-4.22453307340936));
#148225=CARTESIAN_POINT('Ctrl Pts',(-6.20568528634992,4.55543368301996,
-4.2128563299192));
#148226=CARTESIAN_POINT('',(-5.65722186911748,4.69005394727052,-4.5341306477488));
#148227=CARTESIAN_POINT('Origin',(0.154334891420042,4.69642268872752,0.125085317682646));
#148228=CARTESIAN_POINT('Ctrl Pts',(-5.85195259570583,4.65066950062562,
-4.69091151222382));
#148229=CARTESIAN_POINT('Ctrl Pts',(-5.81944146920557,4.65692555514123,
-4.66478707599278));
#148230=CARTESIAN_POINT('Ctrl Pts',(-5.78694146035984,4.66333077493862,
-4.63864782873607));
#148231=CARTESIAN_POINT('Ctrl Pts',(-5.72204085546351,4.67644844957531,
-4.58639702126181));
#148232=CARTESIAN_POINT('Ctrl Pts',(-5.68960393149243,4.68316824044095,
-4.56025621791814));
#148233=CARTESIAN_POINT('Ctrl Pts',(-5.6572218677117,4.69005394654428,-4.53413064929983));
#148234=CARTESIAN_POINT('Ctrl Pts',(-5.133833235,4.559946053,-5.119204656));
#148235=CARTESIAN_POINT('Ctrl Pts',(-5.413053537,4.62560150099999,-4.839186457));
#148236=CARTESIAN_POINT('Ctrl Pts',(-5.660161555,4.690829639,-4.530460371));
#148237=CARTESIAN_POINT('Ctrl Pts',(-5.481680828,4.559946053,-5.118708363));
#148238=CARTESIAN_POINT('Ctrl Pts',(-5.76087406,4.62560150099999,-4.819717273));
#148239=CARTESIAN_POINT('Ctrl Pts',(-6.00589160500001,4.690829639,-4.492133795));
#148240=CARTESIAN_POINT('Origin',(0.139906077312633,4.55357614863355,0.141038475289471));
#148241=CARTESIAN_POINT('Ctrl Pts',(-4.546581334,4.690837228,-5.647220394));
#148242=CARTESIAN_POINT('Ctrl Pts',(-4.85460752600001,4.625180297,-5.399228277));
#148243=CARTESIAN_POINT('Ctrl Pts',(-5.133833235,4.559946053,-5.119204656));
#148244=CARTESIAN_POINT('Ctrl Pts',(-5.1434905069197,4.55768986808407,-5.1095197875772));
#148245=CARTESIAN_POINT('Ctrl Pts',(-5.15314777883924,4.55543368316826,
-5.09983491915429));
#148246=CARTESIAN_POINT('Ctrl Pts',(-4.50916339980099,4.690837228,-5.99377451448871));
#148247=CARTESIAN_POINT('Ctrl Pts',(-4.83609229828384,4.625180297,-5.74782334933595));
#148248=CARTESIAN_POINT('Ctrl Pts',(-5.13433055676911,4.55994605300001,
-5.46777260227703));
#148249=CARTESIAN_POINT('Ctrl Pts',(-5.14464539478797,4.55768986808407,
-5.45808679567509));
#148250=CARTESIAN_POINT('Ctrl Pts',(-5.15496023280698,4.55543368316826,
-5.44840098907329));
#148251=CARTESIAN_POINT('',(-4.55025510439708,4.6900539473003,-5.64426066861927));
#148252=CARTESIAN_POINT('Origin',(0.123836918956326,4.69642264566216,0.155338239191032));
#148253=CARTESIAN_POINT('Ctrl Pts',(-4.70672988353111,4.65066950059933,
-5.83923743366634));
#148254=CARTESIAN_POINT('Ctrl Pts',(-4.68059483217912,4.65692555473698,
-5.80673484297425));
#148255=CARTESIAN_POINT('Ctrl Pts',(-4.65447382010427,4.66333077472239,
-5.7742201744936));
#148256=CARTESIAN_POINT('Ctrl Pts',(-4.60232293359513,4.67644844953836,
-5.70923924922473));
#148257=CARTESIAN_POINT('Ctrl Pts',(-4.5762638670516,4.68316824035594,-5.67673662366901));
#148258=CARTESIAN_POINT('Ctrl Pts',(-4.55025510284291,4.6900539464758,-5.64426066968913));
#148259=CARTESIAN_POINT('Ctrl Pts',(-3.913329389,4.559946053,-6.10314288700001));
#148260=CARTESIAN_POINT('Ctrl Pts',(-4.246217311,4.62560150099999,-5.889695469));
#148261=CARTESIAN_POINT('Ctrl Pts',(-4.553915063,4.690829639,-5.641308146));
#148262=CARTESIAN_POINT('Ctrl Pts',(-4.253151186,4.559946053,-6.177435146));
#148263=CARTESIAN_POINT('Ctrl Pts',(-4.590091282,4.62560150099999,-5.945452595));
#148264=CARTESIAN_POINT('Ctrl Pts',(-4.899801218,4.690829639,-5.678199365));
#148265=CARTESIAN_POINT('Origin',(0.106316165810689,4.55357608865779,0.167816914275922));
#148266=CARTESIAN_POINT('Ctrl Pts',(-3.226299335,4.690837228,-6.49257211000001));
#148267=CARTESIAN_POINT('Ctrl Pts',(-3.58043502,4.625180297,-6.316594438));
#148268=CARTESIAN_POINT('Ctrl Pts',(-3.913329389,4.559946053,-6.103142887));
#148269=CARTESIAN_POINT('Ctrl Pts',(-3.92484283910021,4.55768986820667,
-6.09576047380798));
#148270=CARTESIAN_POINT('Ctrl Pts',(-3.93635628920047,4.55543368341347,
-6.08837806061598));
#148271=CARTESIAN_POINT('Ctrl Pts',(-3.11525731968891,4.690837228,-6.82298023806261));
#148272=CARTESIAN_POINT('Ctrl Pts',(-3.48741503215406,4.625180297,-6.6530593240067));
#148273=CARTESIAN_POINT('Ctrl Pts',(-3.83888327807568,4.559946053,-6.44366841676536));
#148274=CARTESIAN_POINT('Ctrl Pts',(-3.8510391223556,4.55768986820667,-6.43642644457697));
#148275=CARTESIAN_POINT('Ctrl Pts',(-3.86319496663552,4.55543368341345,
-6.42918447238861));
#148276=CARTESIAN_POINT('',(-3.23052346845693,4.69005394729118,-6.49047133413896));
#148277=CARTESIAN_POINT('Origin',(0.087548756417985,4.69642265196506,0.178328165779703));
#148278=CARTESIAN_POINT('Ctrl Pts',(-3.3414257128972,4.65066950063507,-6.71452710196661));
#148279=CARTESIAN_POINT('Ctrl Pts',(-3.32288878222841,4.65692555427717,
-6.67716614327895));
#148280=CARTESIAN_POINT('Ctrl Pts',(-3.30436815677363,4.66333077449093,
-6.63979640280476));
#148281=CARTESIAN_POINT('Ctrl Pts',(-3.2674055064748,4.67644844951943,-6.56512379521447));
#148282=CARTESIAN_POINT('Ctrl Pts',(-3.24894279044509,4.6831682402169,-6.5277791346204));
#148283=CARTESIAN_POINT('Ctrl Pts',(-3.23052346675912,4.6900539463452,-6.4904713348026));
#148284=CARTESIAN_POINT('Ctrl Pts',(-2.509842609,4.559946053,-6.801704939));
#148285=CARTESIAN_POINT('Ctrl Pts',(-2.880832682,4.62560150099999,-6.66480886600001));
#148286=CARTESIAN_POINT('Ctrl Pts',(-3.234732564,4.690829639,-6.488374622));
#148287=CARTESIAN_POINT('Ctrl Pts',(-2.825748922,4.559946053,-6.947311928));
#148288=CARTESIAN_POINT('Ctrl Pts',(-3.204680937,4.62560150099999,-6.79318516));
#148289=CARTESIAN_POINT('Ctrl Pts',(-3.564601571,4.690829639,-6.598758644));
#148290=CARTESIAN_POINT('Origin',(0.0677547936467743,4.55357613660652,0.186748104515124));
#148291=CARTESIAN_POINT('Ctrl Pts',(-1.755159165,4.690837228,-7.03433837));
#148292=CARTESIAN_POINT('Ctrl Pts',(-2.138845352,4.625180297,-6.938603662));
#148293=CARTESIAN_POINT('Ctrl Pts',(-2.509842609,4.559946053,-6.801704939));
#148294=CARTESIAN_POINT('Ctrl Pts',(-2.5226738823718,4.55768986807635,-6.79697017369941));
#148295=CARTESIAN_POINT('Ctrl Pts',(-2.5355051557436,4.55543368315257,-6.79223540839867));
#148296=CARTESIAN_POINT('Ctrl Pts',(-1.57568526882399,4.690837228,-7.33315098852527));
#148297=CARTESIAN_POINT('Ctrl Pts',(-1.97567011476171,4.625180297,-7.2472056382896));
#148298=CARTESIAN_POINT('Ctrl Pts',(-2.36393408428663,4.559946053,-7.11826545847802));
#148299=CARTESIAN_POINT('Ctrl Pts',(-2.37736254242049,4.55768986807635,
-7.11380594654213));
#148300=CARTESIAN_POINT('Ctrl Pts',(-2.39079100055429,4.55543368315257,
-7.10934643460628));
#148301=CARTESIAN_POINT('',(-1.75973614522046,4.69005394734215,-7.0331947738758));
#148302=CARTESIAN_POINT('Origin',(0.0471665917159619,4.69642264847688,0.192979168038592));
#148303=CARTESIAN_POINT('Ctrl Pts',(-1.81988018914674,4.6506695006064,-7.27585294610869));
#148304=CARTESIAN_POINT('Ctrl Pts',(-1.80980814109728,4.65692555564396,
-7.23538056476313));
#148305=CARTESIAN_POINT('Ctrl Pts',(-1.7997539084123,4.66333077509884,-7.19490312626228));
#148306=CARTESIAN_POINT('Ctrl Pts',(-1.77970782869064,4.67644844946861,
-7.11403044988764));
#148307=CARTESIAN_POINT('Ctrl Pts',(-1.76970475880949,4.68316824019229,
-7.07358994854362));
#148308=CARTESIAN_POINT('Ctrl Pts',(-1.75973614281127,4.69005394634804,
-7.03319477430088));
#148309=CARTESIAN_POINT('Ctrl Pts',(-0.988998379000001,4.559946053,-7.182226828));
#148310=CARTESIAN_POINT('Ctrl Pts',(-1.380743519,4.62560150099999,-7.128283209));
#148311=CARTESIAN_POINT('Ctrl Pts',(-1.764297565,4.690829639,-7.032051913));
#148312=CARTESIAN_POINT('Ctrl Pts',(-1.266217779,4.559946053,-7.392340126));
#148313=CARTESIAN_POINT('Ctrl Pts',(-1.669423273,4.62560150099999,-7.323275938));
#148314=CARTESIAN_POINT('Ctrl Pts',(-2.062725117,4.690829639,-7.210767303));
#148315=CARTESIAN_POINT('Origin',(0.0260254480465574,4.55357606320967,0.196947624641689));
#148316=CARTESIAN_POINT('Ctrl Pts',(-0.201949703,4.690837228,-7.247186786));
#148317=CARTESIAN_POINT('Ctrl Pts',(-0.597245653,4.625180297,-7.236171492));
#148318=CARTESIAN_POINT('Ctrl Pts',(-0.988998379000001,4.559946053,-7.182226828));
#148319=CARTESIAN_POINT('Ctrl Pts',(-1.00254749810723,4.55768986821006,
-7.18036110345178));
#148320=CARTESIAN_POINT('Ctrl Pts',(-1.01609661721445,4.55543368342,-7.17849537890344));
#148321=CARTESIAN_POINT('Ctrl Pts',(0.0375640730718744,4.690837228,-7.50043175005402));
#148322=CARTESIAN_POINT('Ctrl Pts',(-0.371545059360647,4.625180297,-7.50248067266783));
#148323=CARTESIAN_POINT('Ctrl Pts',(-0.778449959965024,4.559946053,-7.46002031823318));
#148324=CARTESIAN_POINT('Ctrl Pts',(-0.792523130609923,4.55768986821006,
-7.45855178882321));
#148325=CARTESIAN_POINT('Ctrl Pts',(-0.80659630125483,4.55543368342001,
-7.45708325941323));
#148326=CARTESIAN_POINT('',(-0.206665515392902,4.69005394729617,-7.24705384059663));
#148327=CARTESIAN_POINT('Origin',(0.00457900162748118,4.69642265313607,
0.198606590580912));
#148328=CARTESIAN_POINT('Ctrl Pts',(-0.213239090823364,4.65066950319989,
-7.49696797599281));
#148329=CARTESIAN_POINT('Ctrl Pts',(-0.212102887474093,4.65692555718157,
-7.45527663113703));
#148330=CARTESIAN_POINT('Ctrl Pts',(-0.210985170253372,4.66333077468,-7.41358418236226));
#148331=CARTESIAN_POINT('Ctrl Pts',(-0.20879299148723,4.67644844957351,
-7.33029294597433));
#148332=CARTESIAN_POINT('Ctrl Pts',(-0.207717300189202,4.68316824044063,
-7.28864755558494));
#148333=CARTESIAN_POINT('Ctrl Pts',(-0.206665513338619,4.69005394649188,
-7.24705384051543));
#148334=CARTESIAN_POINT('Ctrl Pts',(0.578090316999999,4.559946053,-7.226915773));
#148335=CARTESIAN_POINT('Ctrl Pts',(0.183907677,4.62560150099999,-7.258446951));
#148336=CARTESIAN_POINT('Ctrl Pts',(-0.211365974,4.690829639,-7.246918271));
#148337=CARTESIAN_POINT('Ctrl Pts',(0.3525203,4.559946053,-7.491710715));
#148338=CARTESIAN_POINT('Ctrl Pts',(-0.056105233,4.62560150099999,-7.510938472));
#148339=CARTESIAN_POINT('Ctrl Pts',(-0.464397928,4.690829639,-7.485608497));
#148340=CARTESIAN_POINT('Origin',(-0.0169208918346127,4.55357611859478,
0.197937287104135));
#148341=CARTESIAN_POINT('Ctrl Pts',(1.360702703,4.690837228,-7.12116480300001));
#148342=CARTESIAN_POINT('Ctrl Pts',(0.97228059,4.625180297,-7.19538398400001));
#148343=CARTESIAN_POINT('Ctrl Pts',(0.578090317,4.559946053,-7.226915773));
#148344=CARTESIAN_POINT('Ctrl Pts',(0.564456893314398,4.55768986823804,
-7.22800632816698));
#148345=CARTESIAN_POINT('Ctrl Pts',(0.550823469628794,4.55543368347596,
-7.22909688333405));
#148346=CARTESIAN_POINT('Ctrl Pts',(1.64905696119275,4.690837228,-7.31700065792814));
#148347=CARTESIAN_POINT('Ctrl Pts',(1.24995303106491,4.625180297,-7.40694804796946));
#148348=CARTESIAN_POINT('Ctrl Pts',(0.843433619569688,4.559946053,-7.45295291915567));
#148349=CARTESIAN_POINT('Ctrl Pts',(0.829373781585471,4.55768986823804,
-7.45454403883429));
#148350=CARTESIAN_POINT('Ctrl Pts',(0.815313943601237,4.55543368347595,
-7.45613515851278));
#148351=CARTESIAN_POINT('',(1.35606856387976,4.6900539472633,-7.12204872627897));
#148352=CARTESIAN_POINT('Origin',(-0.0382226035133557,4.69642263628286,
0.194947726860468));
#148353=CARTESIAN_POINT('Ctrl Pts',(1.40337283024095,4.65066950057685,-7.36753314860582));
#148354=CARTESIAN_POINT('Ctrl Pts',(1.39552006198328,4.65692555525109,-7.32657226924565));
#148355=CARTESIAN_POINT('Ctrl Pts',(1.3876490007401,4.66333077493922,-7.28561427662822));
#148356=CARTESIAN_POINT('Ctrl Pts',(1.371884774107,4.67644844949167,-7.20379909165715));
#148357=CARTESIAN_POINT('Ctrl Pts',(1.36398278850602,4.68316824027346,-7.16289610614497));
#148358=CARTESIAN_POINT('Ctrl Pts',(1.35606856587716,4.69005394638793,-7.12204872574441));
#148359=CARTESIAN_POINT('Ctrl Pts',(2.118148151,4.559946053,-6.933682168));
#148360=CARTESIAN_POINT('Ctrl Pts',(1.739959553,4.62560150099999,-7.04921378));
#148361=CARTESIAN_POINT('Ctrl Pts',(1.351448856,4.690829639,-7.122926785));
#148362=CARTESIAN_POINT('Ctrl Pts',(1.954774922,4.559946053,-7.24077723800001));
#148363=CARTESIAN_POINT('Ctrl Pts',(1.559836226,4.62560150099999,-7.347397871));
#148364=CARTESIAN_POINT('Ctrl Pts',(1.155643991,4.690829639,-7.410430957));
#148365=CARTESIAN_POINT('Origin',(-0.0590759568647822,4.55357616882721,
0.189672134404391));
#148366=CARTESIAN_POINT('Ctrl Pts',(2.859730162,4.690837228,-6.662165068));
#148367=CARTESIAN_POINT('Ctrl Pts',(2.496344072,4.625180297,-6.818148319));
#148368=CARTESIAN_POINT('Ctrl Pts',(2.118148151,4.559946053,-6.933682168));
#148369=CARTESIAN_POINT('Ctrl Pts',(2.10506790544386,4.55768986808944,-6.93767800991962));
#148370=CARTESIAN_POINT('Ctrl Pts',(2.09198765988772,4.55543368317901,-6.94167385183935));
#148371=CARTESIAN_POINT('Ctrl Pts',(3.18344177798669,4.690837228,-6.7914347477429));
#148372=CARTESIAN_POINT('Ctrl Pts',(2.8130047063723,4.625180297,-6.96507476535647));
#148373=CARTESIAN_POINT('Ctrl Pts',(2.42587918037998,4.559946053,-7.09739372560017));
#148374=CARTESIAN_POINT('Ctrl Pts',(2.41249009641619,4.55768986808944,-7.10197009566556));
#148375=CARTESIAN_POINT('Ctrl Pts',(2.39910101245242,4.55543368317901,-7.10654646573097));
#148376=CARTESIAN_POINT('',(2.85539438454128,4.69005394734903,-6.66402452886225));
#148377=CARTESIAN_POINT('Origin',(-0.0792369470889415,4.69642268535183,
0.18217313625983));
#148378=CARTESIAN_POINT('Ctrl Pts',(2.95436459788649,4.65066950058357,-6.89360064286475));
#148379=CARTESIAN_POINT('Ctrl Pts',(2.93789004392934,4.65692555558273,-6.85528551722975));
#148380=CARTESIAN_POINT('Ctrl Pts',(2.92139824654535,4.66333077509932,-6.81697714636908));
#148381=CARTESIAN_POINT('Ctrl Pts',(2.88841473289329,4.67644844951969,-6.74046359853245));
#148382=CARTESIAN_POINT('Ctrl Pts',(2.871904558448,4.68316824035792,-6.70221559510132));
#148383=CARTESIAN_POINT('Ctrl Pts',(2.8553943867348,4.69005394645179,-6.66402452775221));
#148384=CARTESIAN_POINT('Ctrl Pts',(3.559163733,4.559946053,-6.316237292));
#148385=CARTESIAN_POINT('Ctrl Pts',(3.214652856,4.62560150099999,-6.51036720800001));
#148386=CARTESIAN_POINT('Ctrl Pts',(2.85107144,4.690829639,-6.66587516));
#148387=CARTESIAN_POINT('Ctrl Pts',(3.465626441,4.559946053,-6.651273064));
#148388=CARTESIAN_POINT('Ctrl Pts',(3.102841477,4.62560150099999,-6.840301112));
#148389=CARTESIAN_POINT('Ctrl Pts',(2.721649282,4.690829639,-6.988749902));
#148390=CARTESIAN_POINT('Origin',(-0.0984686841105226,4.55357616529912,
0.172538095315817));
#148391=CARTESIAN_POINT('Ctrl Pts',(4.225039818,4.690837228,-5.891649899));
#148392=CARTESIAN_POINT('Ctrl Pts',(3.903681281,4.625180297,-6.122103616));
#148393=CARTESIAN_POINT('Ctrl Pts',(3.559163733,4.559946053,-6.316237292));
#148394=CARTESIAN_POINT('Ctrl Pts',(3.54724828415092,4.55768986807677,-6.32295157955862));
#148395=CARTESIAN_POINT('Ctrl Pts',(3.53533283530178,4.55543368315343,-6.32966586711737));
#148396=CARTESIAN_POINT('Ctrl Pts',(4.5689723957904,4.690837228,-5.94830889693407));
#148397=CARTESIAN_POINT('Ctrl Pts',(4.2445234080404,4.625180297,-6.19752232790761));
#148398=CARTESIAN_POINT('Ctrl Pts',(3.89489332643794,4.559946053,-6.40996828922153));
#148399=CARTESIAN_POINT('Ctrl Pts',(3.88280105602207,4.55768986807677,-6.41731592361615));
#148400=CARTESIAN_POINT('Ctrl Pts',(3.87070878560611,4.55543368315345,-6.42466355801077));
#148401=CARTESIAN_POINT('',(4.22120513711781,4.69005394729203,-5.89439795128933));
#148402=CARTESIAN_POINT('Origin',(-0.116546242049927,4.69642265312355,0.160880395786349));
#148403=CARTESIAN_POINT('Ctrl Pts',(4.36721356001129,4.65066950061697,-6.09733103232014));
#148404=CARTESIAN_POINT('Ctrl Pts',(4.34288755318521,4.65692555542693,-6.06345323611052));
#148405=CARTESIAN_POINT('Ctrl Pts',(4.31854615715426,4.66333077500663,-6.02958574219209));
#148406=CARTESIAN_POINT('Ctrl Pts',(4.26988562827294,4.67644844947529,-5.96195151866449));
#148407=CARTESIAN_POINT('Ctrl Pts',(4.24553926283835,4.68316824016109,-5.92814693247655));
#148408=CARTESIAN_POINT('Ctrl Pts',(4.22120513897642,4.69005394628535,-5.89439794974382));
#148409=CARTESIAN_POINT('Ctrl Pts',(4.833756773,4.559946053,-5.403452179));
#148410=CARTESIAN_POINT('Ctrl Pts',(4.539032563,4.62560150099999,-5.667103101));
#148411=CARTESIAN_POINT('Ctrl Pts',(4.217381091,4.690829639,-5.89713462));
#148412=CARTESIAN_POINT('Ctrl Pts',(4.814429119,4.559946053,-5.750762755));
#148413=CARTESIAN_POINT('Ctrl Pts',(4.500761309,4.62560150099999,-6.013359475));
#148414=CARTESIAN_POINT('Ctrl Pts',(4.160393277,4.690829639,-6.240282668));
#148415=CARTESIAN_POINT('Origin',(-0.133257209622126,4.55357610187738,0.147336455412355));
#148416=CARTESIAN_POINT('Ctrl Pts',(5.392791307,4.690837228,-4.845647729));
#148417=CARTESIAN_POINT('Ctrl Pts',(5.128486691,4.625180297,-5.139796152));
#148418=CARTESIAN_POINT('Ctrl Pts',(4.833756773,4.559946053,-5.403452179));
#148419=CARTESIAN_POINT('Ctrl Pts',(4.82356327437088,4.55768986814676,-5.41257095923113));
#148420=CARTESIAN_POINT('Ctrl Pts',(4.81336977574183,4.55543368329364,-5.42168973946224));
#148421=CARTESIAN_POINT('Ctrl Pts',(5.74086294257771,4.690837228,-4.82704673403762));
#148422=CARTESIAN_POINT('Ctrl Pts',(5.4775729123286,4.625180297,-5.14018063457471));
#148423=CARTESIAN_POINT('Ctrl Pts',(5.18178659015542,4.559946053,-5.42281985940054));
#148424=CARTESIAN_POINT('Ctrl Pts',(5.17155655484025,4.55768986814676,-5.43259519055912));
#148425=CARTESIAN_POINT('Ctrl Pts',(5.16132651952504,4.55543368329364,-5.44237052171769));
#148426=CARTESIAN_POINT('',(5.38963702945794,4.69005394731139,-4.84915587636755));
#148427=CARTESIAN_POINT('Origin',(-0.14840603322689,4.69642265777085,0.132065168005893));
#148428=CARTESIAN_POINT('Ctrl Pts',(5.57585646967172,4.65066950063289,-5.01595700001295));
#148429=CARTESIAN_POINT('Ctrl Pts',(5.54481647208783,4.65692555434243,-4.98810062512853));
#148430=CARTESIAN_POINT('Ctrl Pts',(5.51376365132302,4.66333077450115,-4.96025761229812));
#148431=CARTESIAN_POINT('Ctrl Pts',(5.45170141738881,4.67644844948845,-4.90466521235817));
#148432=CARTESIAN_POINT('Ctrl Pts',(5.42065726996585,4.68316824012357,-4.87688470765217));
#148433=CARTESIAN_POINT('Ctrl Pts',(5.38963703080559,4.69005394625158,-4.84915587459676));
#148434=CARTESIAN_POINT('Ctrl Pts',(5.88232872,4.559946053,-4.238007649));
#148435=CARTESIAN_POINT('Ctrl Pts',(5.651172152,4.62560150099999,-4.55885155200001));
#148436=CARTESIAN_POINT('Ctrl Pts',(5.38649069,4.690829639,-4.85265062));
#148437=CARTESIAN_POINT('Ctrl Pts',(5.938114442,4.559946053,-4.58135317));
#148438=CARTESIAN_POINT('Ctrl Pts',(5.688230544,4.62560150099999,-4.905239832));
#148439=CARTESIAN_POINT('Ctrl Pts',(5.404601906,4.690829639,-5.200026753));
#148440=CARTESIAN_POINT('Origin',(-0.161814908908519,4.55357611144126,0.115245624276269));
#148441=CARTESIAN_POINT('Ctrl Pts',(6.308381869,4.690837228,-3.573068457));
#148442=CARTESIAN_POINT('Ctrl Pts',(6.113489763,4.625180297,-3.917157533));
#148443=CARTESIAN_POINT('Ctrl Pts',(5.88232872,4.559946053,-4.238007649));
#148444=CARTESIAN_POINT('Ctrl Pts',(5.87433380809871,4.55768986819065,-4.24910453789466));
#148445=CARTESIAN_POINT('Ctrl Pts',(5.86633889619729,4.55543368338141,-4.26020142678927));
#148446=CARTESIAN_POINT('Ctrl Pts',(6.64431711846052,4.690837228,-3.48007722958924));
#148447=CARTESIAN_POINT('Ctrl Pts',(6.45449719567473,4.625180297,-3.84248980808535));
#148448=CARTESIAN_POINT('Ctrl Pts',(6.22638527100694,4.559946053,-4.18210640003392));
#148449=CARTESIAN_POINT('Ctrl Pts',(6.2184958155966,4.55768986819065,-4.19385234432286));
#148450=CARTESIAN_POINT('Ctrl Pts',(6.21060636018626,4.55543368338141,-4.20559828861183));
#148451=CARTESIAN_POINT('',(6.30605548334288,4.69005394732156,-3.57717266141838));
#148452=CARTESIAN_POINT('Origin',(-0.173326514540458,4.6964226515756,0.097074634998458));
#148453=CARTESIAN_POINT('Ctrl Pts',(6.52377852850537,4.65066950058853,-3.70004239318149));
#148454=CARTESIAN_POINT('Ctrl Pts',(6.48747592977033,4.65692555462453,-3.67950996574764));
#148455=CARTESIAN_POINT('Ctrl Pts',(6.45116368268525,4.66333077467253,-3.65899334604125));
#148456=CARTESIAN_POINT('Ctrl Pts',(6.37860170737359,4.67644844952994,-3.61804221178828));
#148457=CARTESIAN_POINT('Ctrl Pts',(6.34231136657993,4.6831682403472,-3.59758477342315));
#148458=CARTESIAN_POINT('Ctrl Pts',(6.30605548408511,4.69005394644704,-3.57717265980503));
#148459=CARTESIAN_POINT('Ctrl Pts',(6.655849513,4.559946053,-2.874398591));
#148460=CARTESIAN_POINT('Ctrl Pts',(6.499069213,4.62560150099999,-3.237433171));
#148461=CARTESIAN_POINT('Ctrl Pts',(6.303733971,4.690829639,-3.581262071));
#148462=CARTESIAN_POINT('Ctrl Pts',(6.784140134,4.559946053,-3.197724603));
#148463=CARTESIAN_POINT('Ctrl Pts',(6.609724441,4.62560150099999,-3.567756627));
#148464=CARTESIAN_POINT('Ctrl Pts',(6.396097357,4.690829639,-3.916623367));
#148465=CARTESIAN_POINT('Origin',(-0.182805944568682,4.55357610379343,0.0777657167856155));
#148466=CARTESIAN_POINT('Ctrl Pts',(6.928999505,4.690837228,-2.133416475));
#148467=CARTESIAN_POINT('Ctrl Pts',(6.81263284900001,4.625180297,-2.511356981));
#148468=CARTESIAN_POINT('Ctrl Pts',(6.655849513,4.559946053,-2.874398591));
#148469=CARTESIAN_POINT('Ctrl Pts',(6.65042702044375,4.55768986805376,-2.88695471129988));
#148470=CARTESIAN_POINT('Ctrl Pts',(6.64500452788751,4.55543368310764,-2.89951083159971));
#148471=CARTESIAN_POINT('Ctrl Pts',(7.23709041011188,4.690837228,-1.97038318210181));
#148472=CARTESIAN_POINT('Ctrl Pts',(7.12961636364939,4.625180297,-2.36512842791059));
#148473=CARTESIAN_POINT('Ctrl Pts',(6.97984509784936,4.559946053,-2.74584229453652));
#148474=CARTESIAN_POINT('Ctrl Pts',(6.97466512404182,4.55768986805376,-2.75900962571157));
#148475=CARTESIAN_POINT('Ctrl Pts',(6.96948515023431,4.55543368310764,-2.77217695688653));
#148476=CARTESIAN_POINT('',(6.92760979279972,4.69005394727773,-2.13792482936519));
#148477=CARTESIAN_POINT('Origin',(-0.190142576289496,4.69642264810554,0.0575450801682964));
#148478=CARTESIAN_POINT('Ctrl Pts',(7.16665595397255,4.65066950061211,-2.21111791583262));
#148479=CARTESIAN_POINT('Ctrl Pts',(7.12678822298077,4.65692555494341,-2.19886951017351));
#148480=CARTESIAN_POINT('Ctrl Pts',(7.08691447053393,4.66333077480341,-2.18663861775419));
#148481=CARTESIAN_POINT('Ctrl Pts',(7.00724567148053,4.67644844950687,-2.16224357833835));
#148482=CARTESIAN_POINT('Ctrl Pts',(6.967406034475,4.68316824027248,-2.15006577416036));
#148483=CARTESIAN_POINT('Ctrl Pts',(6.92760979323705,4.69005394638669,-2.13792482742635));
#148484=CARTESIAN_POINT('Ctrl Pts',(7.118150181,4.559946053,-1.376385849));
#148485=CARTESIAN_POINT('Ctrl Pts',(7.04307702,4.62560150099999,-1.764636013));
#148486=CARTESIAN_POINT('Ctrl Pts',(6.926221658,4.690829639,-2.142417687));
#148487=CARTESIAN_POINT('Ctrl Pts',(7.31294697400001,4.559946053,-1.664573988));
#148488=CARTESIAN_POINT('Ctrl Pts',(7.222154969,4.62560150099999,-2.063449087));
#148489=CARTESIAN_POINT('Ctrl Pts',(7.088518405,4.690829639,-2.450083024));
#148490=CARTESIAN_POINT('Origin',(-0.195249611847796,4.55357612535333,0.0366497801067472));
#148491=CARTESIAN_POINT('Ctrl Pts',(7.225624826,4.690837228,-0.594008309));
#148492=CARTESIAN_POINT('Ctrl Pts',(7.193224795,4.625180297,-0.988128168));
#148493=CARTESIAN_POINT('Ctrl Pts',(7.118150181,4.559946053,-1.376385849));
#148494=CARTESIAN_POINT('Ctrl Pts',(7.11555365822817,4.55768986823893,-1.38981408867173));
#148495=CARTESIAN_POINT('Ctrl Pts',(7.11295713545635,4.55543368347798,-1.40324232834349));
#148496=CARTESIAN_POINT('Ctrl Pts',(7.49146539823089,4.690837228,-0.368556206901194));
#148497=CARTESIAN_POINT('Ctrl Pts',(7.47136259377661,4.625180297,-0.77717627114012));
#148498=CARTESIAN_POINT('Ctrl Pts',(7.40693512424965,4.55994605300001,-1.18118565373131));
#148499=CARTESIAN_POINT('Ctrl Pts',(7.40470684250641,4.55768986823893,-1.19515868011186));
#148500=CARTESIAN_POINT('Ctrl Pts',(7.40247856076304,4.55543368347799,-1.20913170649241));
#148501=CARTESIAN_POINT('',(7.22523676694344,4.69005394732446,-0.598710008128546));
#148502=CARTESIAN_POINT('Origin',(-0.198067624172564,4.69642264164339,0.0153246688116216));
#148503=CARTESIAN_POINT('Ctrl Pts',(7.47442851183213,4.65066950059866,-0.618804022328881));
#148504=CARTESIAN_POINT('Ctrl Pts',(7.43285981682515,4.65692555558568,-0.615412360954817));
#148505=CARTESIAN_POINT('Ctrl Pts',(7.39128901259814,4.66333077511546,-0.612039098318582));
#148506=CARTESIAN_POINT('Ctrl Pts',(7.30823861545105,4.67644844951654,-0.605340838244193));
#148507=CARTESIAN_POINT('Ctrl Pts',(7.26671253877903,4.68316824033724,-0.602012088546937));
#148508=CARTESIAN_POINT('Ctrl Pts',(7.22523676698526,4.69005394643149,-0.598710005741081));
#148509=CARTESIAN_POINT('Ctrl Pts',(7.247614057,4.559946053,0.185985165));
#148510=CARTESIAN_POINT('Ctrl Pts',(7.257758374,4.62560150099999,-0.209326436));
#148511=CARTESIAN_POINT('Ctrl Pts',(7.224846918,4.690829639,-0.603396233));
#148512=CARTESIAN_POINT('Ctrl Pts',(7.49980854,4.559946053,-0.053589743));
#148513=CARTESIAN_POINT('Ctrl Pts',(7.496885558,4.62560150099999,-0.462656961));
#148514=CARTESIAN_POINT('Ctrl Pts',(7.44948821,4.690829639,-0.868979523));
#148515=CARTESIAN_POINT('Origin',(-0.198563393855347,4.55357609619741,-0.00617996657845194));
#148516=CARTESIAN_POINT('Ctrl Pts',(7.184387961,4.690837228,0.973175025));
#148517=CARTESIAN_POINT('Ctrl Pts',(7.237469544,4.625180297,0.581304421));
#148518=CARTESIAN_POINT('Ctrl Pts',(7.24761405700001,4.559946053,0.185985165));
#148519=CARTESIAN_POINT('Ctrl Pts',(7.24796491406655,4.55768986825367,0.172312694520973));
#148520=CARTESIAN_POINT('Ctrl Pts',(7.24831577113324,4.55543368350747,0.158640224041953));
#148521=CARTESIAN_POINT('Ctrl Pts',(7.39554779057242,4.690837228,1.2505040473491));
#148522=CARTESIAN_POINT('Ctrl Pts',(7.46375621382002,4.625180297,0.84711578386299));
#148523=CARTESIAN_POINT('Ctrl Pts',(7.48768509770983,4.559946053,0.438701914431396));
#148524=CARTESIAN_POINT('Ctrl Pts',(7.48851269958758,4.55768986825367,0.424576555020551));
#148525=CARTESIAN_POINT('Ctrl Pts',(7.48934030146532,4.55543368350747,0.4104511956097));
#148526=CARTESIAN_POINT('',(7.18501970007959,4.69005394731586,0.968499827817111));
#148527=CARTESIAN_POINT('Origin',(-0.196731074506683,4.69642264982952,-0.0276122896330641));
#148528=CARTESIAN_POINT('Ctrl Pts',(7.43270510014593,4.650669500567,1.00244445911309));
#148529=CARTESIAN_POINT('Ctrl Pts',(7.39137915761362,4.65692555457027,0.996820785595503));
#148530=CARTESIAN_POINT('Ctrl Pts',(7.35005510013836,4.66333077464795,0.991178688674949));
#148531=CARTESIAN_POINT('Ctrl Pts',(7.26750644425091,4.6764484495285,0.979866966376405));
#148532=CARTESIAN_POINT('Ctrl Pts',(7.22623564101667,4.68316824042381,0.974191012739663));
#148533=CARTESIAN_POINT('Ctrl Pts',(7.18501969968291,4.69005394651994,0.968499829781918));
#148534=CARTESIAN_POINT('Ctrl Pts',(7.038187555,4.559946053,1.73965972));
#148535=CARTESIAN_POINT('Ctrl Pts',(7.133075012,4.62560150099999,1.355771012));
#148536=CARTESIAN_POINT('Ctrl Pts',(7.185646366,4.690829639,0.963839358));
#148537=CARTESIAN_POINT('Ctrl Pts',(7.335987395,4.559946053,1.559900299));
#148538=CARTESIAN_POINT('Ctrl Pts',(7.42107011,4.62560150099999,1.15976849));
#148539=CARTESIAN_POINT('Ctrl Pts',(7.462128226,4.690829639,0.752756495));
#148540=CARTESIAN_POINT('Origin',(-0.192592118064199,4.5535762464635,-0.0487206342586846));
#148541=CARTESIAN_POINT('Ctrl Pts',(6.807217099,4.690837228,2.494853776));
#148542=CARTESIAN_POINT('Ctrl Pts',(6.94329826,4.625180297,2.12355586));
#148543=CARTESIAN_POINT('Ctrl Pts',(7.03818755500001,4.559946053,1.73965972));
#148544=CARTESIAN_POINT('Ctrl Pts',(7.04146938649328,4.55768986808048,1.72638232719811));
#148545=CARTESIAN_POINT('Ctrl Pts',(7.04475121798669,4.55543368316111,1.71310493439622));
#148546=CARTESIAN_POINT('Ctrl Pts',(6.95382258706274,4.690837228,2.81109212166975));
#148547=CARTESIAN_POINT('Ctrl Pts',(7.10715288827251,4.625180297,2.43179764591603));
#148548=CARTESIAN_POINT('Ctrl Pts',(7.21831923756182,4.55994605300001,2.03807626900362));
#148549=CARTESIAN_POINT('Ctrl Pts',(7.22216402559709,4.55768986808048,2.02445906155847));
#148550=CARTESIAN_POINT('Ctrl Pts',(7.22600881363248,4.55543368316112,2.01084185411338));
#148551=CARTESIAN_POINT('',(6.80883909872424,4.69005394729676,2.49042368830192));
#148552=CARTESIAN_POINT('Origin',(-0.186195767971943,4.69642263429418,-0.0692580676992791));
#148553=CARTESIAN_POINT('Ctrl Pts',(7.04343665837363,4.6506695006056,2.57681975190767));
#148554=CARTESIAN_POINT('Ctrl Pts',(7.00428581767017,4.65692555448949,2.56244370101792));
#148555=CARTESIAN_POINT('Ctrl Pts',(6.96514077763763,4.66333077457468,2.54805006238074));
#148556=CARTESIAN_POINT('Ctrl Pts',(6.88695374923352,4.67644844946909,2.51925728100585));
#148557=CARTESIAN_POINT('Ctrl Pts',(6.84786799736152,4.68316824024888,2.50484202554462));
#148558=CARTESIAN_POINT('Ctrl Pts',(6.80883909785788,4.69005394636529,2.49042369020222));
#148559=CARTESIAN_POINT('Ctrl Pts',(6.499663225,4.559946053,3.211989719));
#148560=CARTESIAN_POINT('Ctrl Pts',(6.674856991,4.62560150099999,2.857474115));
#148561=CARTESIAN_POINT('Ctrl Pts',(6.810452976,4.690829639,2.486006892));
#148562=CARTESIAN_POINT('Ctrl Pts',(6.829143632,4.559946053,3.100451136));
#148563=CARTESIAN_POINT('Ctrl Pts',(6.998253672,4.62560150099999,2.727964456));
#148564=CARTESIAN_POINT('Ctrl Pts',(7.125847419,4.690829639,2.339294456));
#148565=CARTESIAN_POINT('Origin',(-0.177616212431316,4.55357612871005,-0.0889833422622244));
#148566=CARTESIAN_POINT('Ctrl Pts',(6.111748332,4.690837228,3.899875938));
#148567=CARTESIAN_POINT('Ctrl Pts',(6.324466068,4.625180297,3.566512188));
#148568=CARTESIAN_POINT('Ctrl Pts',(6.499663225,4.559946053,3.211989719));
#148569=CARTESIAN_POINT('Ctrl Pts',(6.50572257618686,4.55768986802202,3.19972824067412));
#148570=CARTESIAN_POINT('Ctrl Pts',(6.51178192737385,4.55543368304416,3.1874667623483));
#148571=CARTESIAN_POINT('Ctrl Pts',(6.18694436872914,4.690837228,4.24023665216603));
#148572=CARTESIAN_POINT('Ctrl Pts',(6.41822699307544,4.625180297,3.90277135387362));
#148573=CARTESIAN_POINT('Ctrl Pts',(6.61143279187819,4.559946053,3.54215244291806));
#148574=CARTESIAN_POINT('Ctrl Pts',(6.61811498813259,4.55768986802201,3.52968011366611));
#148575=CARTESIAN_POINT('Ctrl Pts',(6.62479718438698,4.55543368304417,3.51720778441416));
#148576=CARTESIAN_POINT('',(6.11428474814677,4.69005394729447,3.89589810483793));
#148577=CARTESIAN_POINT('Origin',(-0.166954220894603,4.69642263991986,-0.107665456760926));
#148578=CARTESIAN_POINT('Ctrl Pts',(6.32482494729747,4.65066950060335,4.03070581739704));
#148579=CARTESIAN_POINT('Ctrl Pts',(6.28967985561794,4.65692555483078,4.00824959584556));
#148580=CARTESIAN_POINT('Ctrl Pts',(6.25454421281184,4.66333077473281,3.9857774466005));
#148581=CARTESIAN_POINT('Ctrl Pts',(6.18437475129858,4.67644844948546,3.94084992472931));
#148582=CARTESIAN_POINT('Ctrl Pts',(6.14930165691324,4.68316824015411,3.91836940879909));
#148583=CARTESIAN_POINT('Ctrl Pts',(6.11428474714911,4.69005394626956,3.89589810607852));
#148584=CARTESIAN_POINT('Ctrl Pts',(5.657221867,4.559946053,4.534130649));
#148585=CARTESIAN_POINT('Ctrl Pts',(5.904530075,4.62560150099999,4.225564904));
#148586=CARTESIAN_POINT('Ctrl Pts',(6.116810374,4.690829639,3.891931506));
#148587=CARTESIAN_POINT('Ctrl Pts',(6.00297670400001,4.559946053,4.496028325));
#148588=CARTESIAN_POINT('Ctrl Pts',(6.24820667,4.62560150099999,4.168603835));
#148589=CARTESIAN_POINT('Ctrl Pts',(6.456369908,4.690829639,3.816449609));
#148590=CARTESIAN_POINT('Origin',(-0.154334695471594,4.5535761299946,-0.125085081307957));
#148591=CARTESIAN_POINT('Ctrl Pts',(5.130501005,4.690837228,5.122544235));
#148592=CARTESIAN_POINT('Ctrl Pts',(5.40990887,4.625180297,4.842702369));
#148593=CARTESIAN_POINT('Ctrl Pts',(5.657221867,4.559946053,4.534130649));
#148594=CARTESIAN_POINT('Ctrl Pts',(5.66577540917009,4.55768986806935,4.52345841886434));
#148595=CARTESIAN_POINT('Ctrl Pts',(5.67432895134019,4.55543368313859,4.51278618872872));
#148596=CARTESIAN_POINT('Ctrl Pts',(5.13077150802369,4.690837228,5.47111243079801));
#148597=CARTESIAN_POINT('Ctrl Pts',(5.42919193653825,4.625180297,5.19125581030626));
#148598=CARTESIAN_POINT('Ctrl Pts',(5.69540309763406,4.559946053,4.88060150441775));
#148599=CARTESIAN_POINT('Ctrl Pts',(5.7046102497862,4.55768986806935,4.86985724617828));
#148600=CARTESIAN_POINT('Ctrl Pts',(5.71381740193835,4.5554336831386,4.85911298793895));
#148601=CARTESIAN_POINT('',(5.13383323721505,4.69005394730716,5.11920465513332));
#148602=CARTESIAN_POINT('Origin',(-0.139906057811033,4.69642266906896,-0.141038569018334));
#148603=CARTESIAN_POINT('Ctrl Pts',(5.31047145097426,4.65066950059662,5.29612055860463));
#148604=CARTESIAN_POINT('Ctrl Pts',(5.280975456191,4.65692555473346,5.26663419557849));
#148605=CARTESIAN_POINT('Ctrl Pts',(5.25149211254357,4.66333077471736,5.23713430764837));
#148606=CARTESIAN_POINT('Ctrl Pts',(5.1926212628331,4.67644844953227,5.17817280592589));
#148607=CARTESIAN_POINT('Ctrl Pts',(5.16320080379083,4.68316824031384,5.14867819294403));
#148608=CARTESIAN_POINT('Ctrl Pts',(5.13383323576555,4.69005394642875,5.11920465637239));
#148609=CARTESIAN_POINT('Ctrl Pts',(4.550255102,4.559946053,5.644260669));
#148610=CARTESIAN_POINT('Ctrl Pts',(4.858113896,4.625601501,5.396072974));
#148611=CARTESIAN_POINT('Ctrl Pts',(5.13715251700001,4.690829639,5.115873729));
#148612=CARTESIAN_POINT('Ctrl Pts',(4.896117256,4.559946053,5.681376225));
#148613=CARTESIAN_POINT('Ctrl Pts',(5.206000469,4.62560150099999,5.41432393300001));
#148614=CARTESIAN_POINT('Ctrl Pts',(5.484999715,4.690829639,5.115151819));
#148615=CARTESIAN_POINT('Origin',(-0.123836949338866,4.55357611375428,-0.155338165372497));
#148616=CARTESIAN_POINT('Ctrl Pts',(3.909357153,4.690837228,6.105688057));
#148617=CARTESIAN_POINT('Ctrl Pts',(4.242390347,4.625180297,5.89245317));
#148618=CARTESIAN_POINT('Ctrl Pts',(4.550255102,4.559946053,5.644260669));
#148619=CARTESIAN_POINT('Ctrl Pts',(4.56090288055171,4.55768986818893,5.63567670884894));
#148620=CARTESIAN_POINT('Ctrl Pts',(4.57155065910353,4.55543368337775,5.62709274869774));
#148621=CARTESIAN_POINT('Ctrl Pts',(3.83468947317842,4.690837228,6.44616507150887));
#148622=CARTESIAN_POINT('Ctrl Pts',(4.1862938986332,4.625180297,6.23700291524664));
#148623=CARTESIAN_POINT('Ctrl Pts',(4.51306268385255,4.559946053,5.99083906467175));
#148624=CARTESIAN_POINT('Ctrl Pts',(4.52436427523683,4.55768986818893,5.98232526721429));
#148625=CARTESIAN_POINT('Ctrl Pts',(4.53566586662106,4.55543368337774,5.97381146975693));
#148626=CARTESIAN_POINT('',(3.91332939128576,4.6900539473128,6.10314288704862));
#148627=CARTESIAN_POINT('Origin',(-0.106316020040327,4.69642264970412,-0.167816826224749));
#148628=CARTESIAN_POINT('Ctrl Pts',(4.04780621107473,4.65066950059032,6.31389458846495));
#148629=CARTESIAN_POINT('Ctrl Pts',(4.02533850998926,4.65692555549962,6.27875682893648));
#148630=CARTESIAN_POINT('Ctrl Pts',(4.00288607620138,4.66333077502009,6.24360858738517));
#148631=CARTESIAN_POINT('Ctrl Pts',(3.95806657571596,4.67644844940684,6.17337008282733));
#148632=CARTESIAN_POINT('Ctrl Pts',(3.93567442061857,4.6831682401762,6.13824050868851));
#148633=CARTESIAN_POINT('Ctrl Pts',(3.91332938909123,4.69005394628826,6.10314288824477));
#148634=CARTESIAN_POINT('Ctrl Pts',(3.230523466,4.559946053,6.490471334));
#148635=CARTESIAN_POINT('Ctrl Pts',(3.58453771,4.625601501,6.314266669));
#148636=CARTESIAN_POINT('Ctrl Pts',(3.917287119,4.690829639,6.100603383));
#148637=CARTESIAN_POINT('Ctrl Pts',(3.560320807,4.559946053,6.601069288));
#148638=CARTESIAN_POINT('Ctrl Pts',(3.920367472,4.625601501,6.406876261));
#148639=CARTESIAN_POINT('Ctrl Pts',(4.257157031,4.690829639,6.174675215));
#148640=CARTESIAN_POINT('Origin',(-0.0875486605970938,4.55357615413023,
-0.178327839154758));
#148641=CARTESIAN_POINT('Ctrl Pts',(2.505416106,4.690837228,6.803336691));
#148642=CARTESIAN_POINT('Ctrl Pts',(2.876502367,4.625180297,6.66667941000001));
#148643=CARTESIAN_POINT('Ctrl Pts',(3.230523466,4.559946053,6.49047133400001));
#148644=CARTESIAN_POINT('Ctrl Pts',(3.24276760300522,4.55768986820418,6.48437701976261));
#148645=CARTESIAN_POINT('Ctrl Pts',(3.2550117400105,4.55543368340826,6.47828270552523));
#148646=CARTESIAN_POINT('Ctrl Pts',(2.35930162164539,4.690837228,7.11980219913421));
#148647=CARTESIAN_POINT('Ctrl Pts',(2.74764941145802,4.625180297,6.99111469553954));
#148648=CARTESIAN_POINT('Ctrl Pts',(3.11969647505973,4.559946053,6.8209516482439));
#148649=CARTESIAN_POINT('Ctrl Pts',(3.13256405620673,4.55768986820418,6.81506640674221));
#148650=CARTESIAN_POINT('Ctrl Pts',(3.14543163735375,4.55543368340825,6.8091811652404));
#148651=CARTESIAN_POINT('',(2.50984261151385,4.69005394727773,6.80170493911411));
#148652=CARTESIAN_POINT('Origin',(-0.0677547966760533,4.69642265928317,
-0.186748302139411));
#148653=CARTESIAN_POINT('Ctrl Pts',(2.59587005248643,4.65066950060226,7.03643792480017));
#148654=CARTESIAN_POINT('Ctrl Pts',(2.58148121593871,4.6569255544196,6.99729178184832));
#148655=CARTESIAN_POINT('Ctrl Pts',(2.5671095390213,4.66333077457138,6.9581386729951));
#148656=CARTESIAN_POINT('Ctrl Pts',(2.53843709451609,4.67644844951328,6.87990743449515));
#148657=CARTESIAN_POINT('Ctrl Pts',(2.52412027548077,4.68316824029878,6.84078551863943));
#148658=CARTESIAN_POINT('Ctrl Pts',(2.50984260926869,4.69005394637568,6.80170493977542));
#148659=CARTESIAN_POINT('Ctrl Pts',(1.759736143,4.559946053,7.033194773));
#148660=CARTESIAN_POINT('Ctrl Pts',(2.143352525,4.625601501,6.937212273));
#148661=CARTESIAN_POINT('Ctrl Pts',(2.514253728,4.690829639,6.800075602));
#148662=CARTESIAN_POINT('Ctrl Pts',(2.058047714,4.559946053,7.212103688));
#148663=CARTESIAN_POINT('Ctrl Pts',(2.451422449,4.62560150099999,7.099850175));
#148664=CARTESIAN_POINT('Ctrl Pts',(2.830254416,4.690829639,6.945477661));
#148665=CARTESIAN_POINT('Origin',(-0.0471666674588023,4.55357609672683,
-0.192979181603469));
#148666=CARTESIAN_POINT('Ctrl Pts',(0.984324587,4.690837228,7.182868863));
#148667=CARTESIAN_POINT('Ctrl Pts',(1.376112332,4.625180297,7.12917913000001));
#148668=CARTESIAN_POINT('Ctrl Pts',(1.759736143,4.559946053,7.03319477300001));
#148669=CARTESIAN_POINT('Ctrl Pts',(1.77300411626669,4.55768986821522,7.02987506800209));
#148670=CARTESIAN_POINT('Ctrl Pts',(1.78627208953345,4.55543368343031,7.02655536300417));
#148671=CARTESIAN_POINT('Ctrl Pts',(0.773595447487644,4.690837228,7.46052528797172));
#148672=CARTESIAN_POINT('Ctrl Pts',(1.18052789164313,4.625180297,7.41832972190833));
#148673=CARTESIAN_POINT('Ctrl Pts',(1.58045672673534,4.559946053,7.33212411374831));
#148674=CARTESIAN_POINT('Ctrl Pts',(1.5942886238711,4.55768986821521,7.32914261554172));
#148675=CARTESIAN_POINT('Ctrl Pts',(1.60812052100694,4.55543368343032,7.32616111733499));
#148676=CARTESIAN_POINT('',(0.988998381079286,4.69005394732039,7.18222682883565));
#148677=CARTESIAN_POINT('Origin',(-0.0260253471886281,4.696422661911,-0.196947453086742));
#148678=CARTESIAN_POINT('Ctrl Pts',(1.02255389472724,4.65066950055004,7.42996524443305));
#148679=CARTESIAN_POINT('Ctrl Pts',(1.01691672373786,4.65692555553897,7.3886411342729));
#148680=CARTESIAN_POINT('Ctrl Pts',(1.01129781035109,4.6633307750339,7.34731392216206));
#148681=CARTESIAN_POINT('Ctrl Pts',(1.00011311603079,4.67644844948152,7.26474796181685));
#148682=CARTESIAN_POINT('Ctrl Pts',(0.994541071871806,4.68316824025307,
7.22346300196127));
#148683=CARTESIAN_POINT('Ctrl Pts',(0.988998378924648,4.69005394639712,
7.18222682897109));
#148684=CARTESIAN_POINT('Ctrl Pts',(0.206665513,4.559946053,7.24705384));
#148685=CARTESIAN_POINT('Ctrl Pts',(0.601946558,4.625601501,7.235781541));
#148686=CARTESIAN_POINT('Ctrl Pts',(0.993656627,4.690829639,7.18158384400001));
#148687=CARTESIAN_POINT('Ctrl Pts',(0.459542598,4.559946053,7.48590813500001));
#148688=CARTESIAN_POINT('Ctrl Pts',(0.867851637,4.625601501,7.460842987));
#148689=CARTESIAN_POINT('Ctrl Pts',(1.271012251,4.690829639,7.391517291));
#148690=CARTESIAN_POINT('Origin',(-0.00457906475628513,4.55357619680332,
-0.198606302057152));
#148691=CARTESIAN_POINT('Ctrl Pts',(-0.582792857,4.690837228,7.226538071));
#148692=CARTESIAN_POINT('Ctrl Pts',(-0.188623186,4.625180297,7.25832635800001));
#148693=CARTESIAN_POINT('Ctrl Pts',(0.206665513,4.559946053,7.24705384000001));
#148694=CARTESIAN_POINT('Ctrl Pts',(0.220336926796758,4.55768986822747,
7.24666396986584));
#148695=CARTESIAN_POINT('Ctrl Pts',(0.23400834059351,4.55543368345483,7.24627409973171));
#148696=CARTESIAN_POINT('Ctrl Pts',(-0.848283189425317,4.690837228,7.4524025062321));
#148697=CARTESIAN_POINT('Ctrl Pts',(-0.441793800398394,4.625180297,7.49867189599384));
#148698=CARTESIAN_POINT('Ctrl Pts',(-0.0326834214049662,4.559946053,7.50045460502951));
#148699=CARTESIAN_POINT('Ctrl Pts',(-0.0185339724226994,4.55768986822747,
7.50051626161866));
#148700=CARTESIAN_POINT('Ctrl Pts',(-0.00438452344043182,4.55543368345484,
7.50057791820777));
#148701=CARTESIAN_POINT('Origin',(0.0169209768713816,4.69642267005817,-0.197936617773742));
#148702=CARTESIAN_POINT('Ctrl Pts',(0.185936733414184,1.19354381562152,
7.24766508350195));
#148703=CARTESIAN_POINT('Ctrl Pts',(0.199362613707092,1.19575849481077,
7.24727086225092));
#148704=CARTESIAN_POINT('Ctrl Pts',(0.212788494,1.197973174,7.24687664100001));
#148705=CARTESIAN_POINT('Ctrl Pts',(0.605187736,1.262701774,7.235354706));
#148706=CARTESIAN_POINT('Ctrl Pts',(0.994048608,1.327878141,7.181529598));
#148707=CARTESIAN_POINT('Ctrl Pts',(0.438644102144323,1.19354381562152,
7.48773050957685));
#148708=CARTESIAN_POINT('Ctrl Pts',(0.452512997286711,1.19575849481077,
7.48686647008995));
#148709=CARTESIAN_POINT('Ctrl Pts',(0.4663818924291,1.197973174,7.48600243060295));
#148710=CARTESIAN_POINT('Ctrl Pts',(0.871729163708226,1.262701774,7.46074908167134));
#148711=CARTESIAN_POINT('Ctrl Pts',(1.27197966967496,1.327878141,7.39187474060707));
#148712=CARTESIAN_POINT('',(0.465867290474915,1.19797317454244,7.48551719487009));
#148713=CARTESIAN_POINT('',(1.02478075909889,1.28783500463657,7.42965843038126));
#148714=CARTESIAN_POINT('Origin',(-0.0343001365998186,1.3392712291817,-0.188172451741534));
#148715=CARTESIAN_POINT('Ctrl Pts',(0.989408718109874,1.32710049318168,
7.18217031322073));
#148716=CARTESIAN_POINT('Ctrl Pts',(0.995257838777893,1.32022179850708,
7.22336221123387));
#148717=CARTESIAN_POINT('Ctrl Pts',(1.00113448834787,1.31351590008605,7.26460533817788));
#148718=CARTESIAN_POINT('Ctrl Pts',(1.01292420902814,1.30043858906419,7.34708728067027));
#148719=CARTESIAN_POINT('Ctrl Pts',(1.01884421512627,1.29405949360237,7.38837459858889));
#148720=CARTESIAN_POINT('Ctrl Pts',(1.02478075183884,1.28783500497465,7.42965843147621));
#148721=CARTESIAN_POINT('',(0.33932788589724,1.19797317561448,7.36619691796539));
#148722=CARTESIAN_POINT('Origin',(1.68105546843877E-13,1.28891220999972,
1.7056668577542E-12));
#148723=CARTESIAN_POINT('',(1.03018391903461,1.10830076261691,7.42891116439694));
#148724=CARTESIAN_POINT('Origin',(-0.0506334157325571,0.946580201577215,
-0.177557611465953));
#148725=CARTESIAN_POINT('',(1.58702106594482,1.19797317379345,7.33016808366918));
#148726=CARTESIAN_POINT('Origin',(-0.0611523990559881,1.3391753255225,-0.175905147922946));
#148727=CARTESIAN_POINT('Ctrl Pts',(1.02478076605977,1.28783500273371,7.42965842925219));
#148728=CARTESIAN_POINT('Ctrl Pts',(1.17943657663153,1.26310656756624,7.40832658743055));
#148729=CARTESIAN_POINT('Ctrl Pts',(1.33303195897402,1.23856749894444,7.38221557285522));
#148730=CARTESIAN_POINT('Ctrl Pts',(1.48513956610284,1.21428571401564,7.35148695569467));
#148731=CARTESIAN_POINT('Ctrl Pts',(1.51912281059599,1.20886077966551,7.3446216968484));
#148732=CARTESIAN_POINT('Ctrl Pts',(1.55308500096562,1.20342302059143,7.33751542487673));
#148733=CARTESIAN_POINT('Ctrl Pts',(1.58702106529159,1.1979731751026,7.33016808322343));
#148734=CARTESIAN_POINT('Ctrl Pts',(0.984685745,1.327885473,7.182819362));
#148735=CARTESIAN_POINT('Ctrl Pts',(1.329357467,1.27059961,7.135568649));
#148736=CARTESIAN_POINT('Ctrl Pts',(1.667921256,1.214285714,7.055532488));
#148737=CARTESIAN_POINT('Ctrl Pts',(1.71688224,1.20614195,7.043958157));
#148738=CARTESIAN_POINT('Ctrl Pts',(1.76567788,1.197973174,7.031705456));
#148739=CARTESIAN_POINT('Ctrl Pts',(0.774406033,1.327885473,7.45991255300001));
#148740=CARTESIAN_POINT('Ctrl Pts',(1.132374232,1.27059961,7.422752234));
#148741=CARTESIAN_POINT('Ctrl Pts',(1.485139566,1.214285714,7.351486956));
#148742=CARTESIAN_POINT('Ctrl Pts',(1.536154289,1.20614195,7.341181016));
#148743=CARTESIAN_POINT('Ctrl Pts',(1.587021072,1.197973174,7.330168082));
#148744=CARTESIAN_POINT('',(1.67634947204994,1.19797317334243,7.18093676992212));
#148745=CARTESIAN_POINT('Ctrl Pts',(1.73962338946964,1.19354381543301,7.03824780020232));
#148746=CARTESIAN_POINT('Ctrl Pts',(1.75265063473478,1.19575849471651,7.03497662810107));
#148747=CARTESIAN_POINT('Ctrl Pts',(1.76567788,1.197973174,7.031705456));
#148748=CARTESIAN_POINT('Ctrl Pts',(2.146426169,1.262701774,6.93609866));
#148749=CARTESIAN_POINT('Ctrl Pts',(2.514624883,1.327878141,6.79993836));
#148750=CARTESIAN_POINT('Ctrl Pts',(2.0380295685556,1.19354381543301,7.21837601620528));
#148751=CARTESIAN_POINT('Ctrl Pts',(2.05138847430055,1.19575849471651,7.21455077483569));
#148752=CARTESIAN_POINT('Ctrl Pts',(2.06474738004543,1.197973174,7.21072553346622));
#148753=CARTESIAN_POINT('Ctrl Pts',(2.45518913513104,1.262701774,7.09892491278304));
#148754=CARTESIAN_POINT('Ctrl Pts',(2.83127605897128,1.327878141,6.94561878728958));
#148755=CARTESIAN_POINT('',(2.06414049783414,1.19797317454228,7.21036226646249));
#148756=CARTESIAN_POINT('',(2.59797889809418,1.28783500532718,7.03565957433808));
#148757=CARTESIAN_POINT('Origin',(-0.0739496577934162,1.33927125484505,
-0.176399334544752));
#148758=CARTESIAN_POINT('Ctrl Pts',(2.51023120581304,1.32710049342706,6.80156153359947));
#148759=CARTESIAN_POINT('Ctrl Pts',(2.52479861772659,1.32022179873707,6.84053299994383));
#148760=CARTESIAN_POINT('Ctrl Pts',(2.53940392803343,1.31351590010745,6.879548580739));
#148761=CARTESIAN_POINT('Ctrl Pts',(2.56864919096453,1.30043858906367,6.9575676999095));
#148762=CARTESIAN_POINT('Ctrl Pts',(2.58330634344234,1.29405949359074,6.9966171170184));
#148763=CARTESIAN_POINT('Ctrl Pts',(2.59797889086842,1.2878350049529,7.03565957699392));
#148764=CARTESIAN_POINT('',(1.91490918273655,1.19797317561398,7.12103386262548));
#148765=CARTESIAN_POINT('Origin',(-5.00684563253806E-13,1.28891221000011,
-1.27068494615301E-12));
#148766=CARTESIAN_POINT('',(2.60309509487799,1.10830076264129,7.03376825908983));
#148767=CARTESIAN_POINT('Origin',(-0.0876193715913992,0.946580153350199,
-0.162521999439057));
#148768=CARTESIAN_POINT('',(3.12568685541228,1.19797317358554,6.81763021082559));
#148769=CARTESIAN_POINT('Origin',(-0.0975371600697084,1.33917533439657,
-0.158646804040897));
#148770=CARTESIAN_POINT('Ctrl Pts',(2.59797890492865,1.28783500479139,7.03565957174917));
#148771=CARTESIAN_POINT('Ctrl Pts',(2.74443323278555,1.26310656825283,6.98158002875429));
#148772=CARTESIAN_POINT('Ctrl Pts',(2.88882454394555,1.23856749894685,6.92306100842335));
#148773=CARTESIAN_POINT('Ctrl Pts',(3.03077021551452,1.21428571428671,6.86035217031531));
#148774=CARTESIAN_POINT('Ctrl Pts',(3.06248312300961,1.20886077964635,6.84634202432027));
#148775=CARTESIAN_POINT('Ctrl Pts',(3.09412365775973,1.20342302038954,6.83210102606699));
#148776=CARTESIAN_POINT('Ctrl Pts',(3.12568685454725,1.19797317447889,6.8176302105138));
#148777=CARTESIAN_POINT('Ctrl Pts',(2.50575818,1.327885473,6.803210709));
#148778=CARTESIAN_POINT('Ctrl Pts',(2.832214162,1.27059961,6.68297046));
#148779=CARTESIAN_POINT('Ctrl Pts',(3.145657109,1.214285714,6.532024292));
#148780=CARTESIAN_POINT('Ctrl Pts',(3.190985273,1.20614195,6.510195399));
#148781=CARTESIAN_POINT('Ctrl Pts',(3.236006129,1.197973174,6.487739539));
#148782=CARTESIAN_POINT('Ctrl Pts',(2.359961536,1.327885473,7.119029537));
#148783=CARTESIAN_POINT('Ctrl Pts',(2.701572267,1.27059961,7.005785424));
#148784=CARTESIAN_POINT('Ctrl Pts',(3.030770215,1.214285714,6.86035217));
#148785=CARTESIAN_POINT('Ctrl Pts',(3.07837677,1.20614195,6.83932052));
#148786=CARTESIAN_POINT('Ctrl Pts',(3.125686861,1.197973174,6.817630208));
#148787=CARTESIAN_POINT('',(3.18084649134048,1.19797317334242,6.65268487524972));
#148788=CARTESIAN_POINT('Ctrl Pts',(3.21196718935855,1.19354381559223,6.49972987172989));
#148789=CARTESIAN_POINT('Ctrl Pts',(3.22398665917931,1.19575849479612,6.49373470536499));
#148790=CARTESIAN_POINT('Ctrl Pts',(3.236006129,1.197973174,6.487739539));
#148791=CARTESIAN_POINT('Ctrl Pts',(3.587300101,1.262701774,6.312518349));
#148792=CARTESIAN_POINT('Ctrl Pts',(3.917620093,1.327878141,6.100389562));
#148793=CARTESIAN_POINT('Ctrl Pts',(3.54211904043812,1.19354381559227,6.61149828219364));
#148794=CARTESIAN_POINT('Ctrl Pts',(3.55434330812815,1.19575849479612,6.60489070320868));
#148795=CARTESIAN_POINT('Ctrl Pts',(3.56656757581818,1.197973174,6.59828312422371));
#148796=CARTESIAN_POINT('Ctrl Pts',(3.92384719094914,1.262701774,6.40516290331904));
#148797=CARTESIAN_POINT('Ctrl Pts',(4.2581851262025,1.327878141,6.17459341925963));
#148798=CARTESIAN_POINT('',(3.56589679053256,1.19797317454273,6.59805881195249));
#148799=CARTESIAN_POINT('',(4.04969843096104,1.28783500531603,6.31268109581324));
#148800=CARTESIAN_POINT('Origin',(-0.110141529144904,1.33927128274808,-0.156378435332287));
#148801=CARTESIAN_POINT('Ctrl Pts',(3.91367807191636,1.32710049343035,6.10291929740531));
#148802=CARTESIAN_POINT('Ctrl Pts',(3.93628261917909,1.32022179874713,6.13784806949174));
#148803=CARTESIAN_POINT('Ctrl Pts',(3.95893366204737,1.31351590012205,6.17281177761949));
#148804=CARTESIAN_POINT('Ctrl Pts',(4.00426699143525,1.30043858907086,6.24271998600702));
#148805=CARTESIAN_POINT('Ctrl Pts',(4.02697593828508,1.2940594935786,6.27770559496417));
#148806=CARTESIAN_POINT('Ctrl Pts',(4.04969842453934,1.28783500493535,6.31268109991297));
#148807=CARTESIAN_POINT('',(3.40095145402154,1.19797317561536,6.54289917816694));
#148808=CARTESIAN_POINT('Origin',(-1.27719015918792E-13,1.28891221000006,
-3.73399228204008E-13));
#148809=CARTESIAN_POINT('',(4.05428843735942,1.10830076263197,6.30973416717019));
#148810=CARTESIAN_POINT('Origin',(-0.120508283964545,0.946580168666976,
-0.139886719195316));
#148811=CARTESIAN_POINT('',(4.5181990013075,1.19797317358556,5.98630752524413));
#148812=CARTESIAN_POINT('Origin',(-0.12936110692105,1.33917530843295,-0.133970025641706));
#148813=CARTESIAN_POINT('Ctrl Pts',(4.0496984370823,1.28783500479117,6.31268109195239));
#148814=CARTESIAN_POINT('Ctrl Pts',(4.18110324087616,1.26310656824494,6.22838254735657));
#148815=CARTESIAN_POINT('Ctrl Pts',(4.30953890387345,1.2385674989391,6.14019180548056));
#148816=CARTESIAN_POINT('Ctrl Pts',(4.43468541808166,1.21428571428671,6.04843494159059));
#148817=CARTESIAN_POINT('Ctrl Pts',(4.46264512820046,1.20886077964635,6.0279350073175));
#148818=CARTESIAN_POINT('Ctrl Pts',(4.49048453128707,1.20342302038954,6.00722517591836));
#148819=CARTESIAN_POINT('Ctrl Pts',(4.51819900073097,1.1979731744789,5.98630752549464));
#148820=CARTESIAN_POINT('Ctrl Pts',(3.909664147,1.327885473,6.105491484));
#148821=CARTESIAN_POINT('Ctrl Pts',(4.202639671,1.27059961,5.917883999));
#148822=CARTESIAN_POINT('Ctrl Pts',(4.476305531,1.214285714,5.703085901));
#148823=CARTESIAN_POINT('Ctrl Pts',(4.515881381,1.20614195,5.672023139));
#148824=CARTESIAN_POINT('Ctrl Pts',(4.555022329,1.197973174,5.640414132));
#148825=CARTESIAN_POINT('Ctrl Pts',(3.83516786,1.327885473,6.445268612));
#148826=CARTESIAN_POINT('Ctrl Pts',(4.144447785,1.27059961,6.261235875));
#148827=CARTESIAN_POINT('Ctrl Pts',(4.434685418,1.214285714,6.048434942));
#148828=CARTESIAN_POINT('Ctrl Pts',(4.476657775,1.20614195,6.017660998));
#148829=CARTESIAN_POINT('Ctrl Pts',(4.518199006,1.197973174,5.986307521));
#148830=CARTESIAN_POINT('',(4.53661066430225,1.19797317334244,5.81336082899545));
#148831=CARTESIAN_POINT('Ctrl Pts',(4.53412297316432,1.19354381550648,5.65729179919426));
#148832=CARTESIAN_POINT('Ctrl Pts',(4.54457265108221,1.19575849475325,5.64885296559718));
#148833=CARTESIAN_POINT('Ctrl Pts',(4.555022329,1.197973174,5.640414132));
#148834=CARTESIAN_POINT('Ctrl Pts',(4.860435866,1.262701774,5.393771696));
#148835=CARTESIAN_POINT('Ctrl Pts',(5.137431742,1.327878141,5.115593328));
#148836=CARTESIAN_POINT('Ctrl Pts',(4.88058296147161,1.19354381550649,5.6954742368475));
#148837=CARTESIAN_POINT('Ctrl Pts',(4.89110099861214,1.19575849475325,5.68639328303249));
#148838=CARTESIAN_POINT('Ctrl Pts',(4.90161903575277,1.197973174,5.67731232921733));
#148839=CARTESIAN_POINT('Ctrl Pts',(5.20903051299453,1.262701774,5.41190259641749));
#148840=CARTESIAN_POINT('Ctrl Pts',(5.48598619042316,1.327878141,5.11485092450687));
#148841=CARTESIAN_POINT('',(4.90091571257073,1.19797317454213,5.67723746024605));
#148842=CARTESIAN_POINT('',(5.3120585661549,1.28783500526933,5.29452866540395));
#148843=CARTESIAN_POINT('Origin',(-0.141183120933982,1.33927122549754,-0.129045132535002));
#148844=CARTESIAN_POINT('Ctrl Pts',(5.13412570213364,1.32710049328122,5.11891133824004));
#148845=CARTESIAN_POINT('Ctrl Pts',(5.16371042111886,1.32022179857526,5.14816418556892));
#148846=CARTESIAN_POINT('Ctrl Pts',(5.19334805826089,1.31351590007935,5.1774411563661));
#148847=CARTESIAN_POINT('Ctrl Pts',(5.25264971787425,1.30043858901147,5.2359696239467));
#148848=CARTESIAN_POINT('Ctrl Pts',(5.28234861391981,1.29405949351238,5.26525553654629));
#148849=CARTESIAN_POINT('Ctrl Pts',(5.31205856075306,1.28783500486646,5.29452867077809));
#148850=CARTESIAN_POINT('',(4.72796901574343,1.19797317561354,5.65882579998064));
#148851=CARTESIAN_POINT('Origin',(-1.15055534544162E-12,1.28891221000022,
-1.02955838299224E-12));
#148852=CARTESIAN_POINT('',(5.31590775787216,1.1083007626196,5.29066391891825));
#148853=CARTESIAN_POINT('Origin',(-0.147762399972118,0.946580160935038,
-0.110710555889455));
#148854=CARTESIAN_POINT('',(5.69944518326462,1.19797317358555,4.87507175408001));
#148855=CARTESIAN_POINT('Origin',(-0.155136266855465,1.33917526459104,-0.103029040302565));
#148856=CARTESIAN_POINT('Ctrl Pts',(5.31205857130684,1.28783500479147,5.29452866032525));
#148857=CARTESIAN_POINT('Ctrl Pts',(5.4222695085429,1.26310656822242,5.18395282036736));
#148858=CARTESIAN_POINT('Ctrl Pts',(5.52874401441177,1.23856749891666,5.07021405812116));
#148859=CARTESIAN_POINT('Ctrl Pts',(5.63123965918988,1.21428571428671,4.95369961753505));
#148860=CARTESIAN_POINT('Ctrl Pts',(5.65413880693855,1.20886077964635,4.92766844913164));
#148861=CARTESIAN_POINT('Ctrl Pts',(5.67687533869773,1.20342302038954,4.90145815332447));
#148862=CARTESIAN_POINT('Ctrl Pts',(5.69944518263217,1.1979731744789,4.87507175436124));
#148863=CARTESIAN_POINT('Ctrl Pts',(5.130758564,1.327885473,5.122286263));
#148864=CARTESIAN_POINT('Ctrl Pts',(5.376554419,1.27059961,4.87608386));
#148865=CARTESIAN_POINT('Ctrl Pts',(5.597646882,1.214285714,4.607477551));
#148866=CARTESIAN_POINT('Ctrl Pts',(5.629619895,1.20614195,4.568633382));
#148867=CARTESIAN_POINT('Ctrl Pts',(5.661050747,1.197973174,4.529349229));
#148868=CARTESIAN_POINT('Ctrl Pts',(5.131045997,1.327885473,5.470134091));
#148869=CARTESIAN_POINT('Ctrl Pts',(5.393533531,1.27059961,5.223917895));
#148870=CARTESIAN_POINT('Ctrl Pts',(5.631239659,1.214285714,4.953699618));
#148871=CARTESIAN_POINT('Ctrl Pts',(5.66561523700001,1.20614195,4.914622335));
#148872=CARTESIAN_POINT('Ctrl Pts',(5.69944518700001,1.197973174,4.875071749));
#148873=CARTESIAN_POINT('',(5.68005599221442,1.19797317334244,4.70048187952442));
#148874=CARTESIAN_POINT('Ctrl Pts',(5.64426820565414,1.19354381542033,4.5503250498189));
#148875=CARTESIAN_POINT('Ctrl Pts',(5.65265947632706,1.19575849471018,4.53983713940944));
#148876=CARTESIAN_POINT('Ctrl Pts',(5.661050747,1.197973174,4.529349229));
#148877=CARTESIAN_POINT('Ctrl Pts',(5.906303053,1.262701774,4.222818274));
#148878=CARTESIAN_POINT('Ctrl Pts',(6.117022792,1.327878141,3.891597635));
#148879=CARTESIAN_POINT('Ctrl Pts',(5.99083624772278,1.19354381542033,4.51313614705207));
#148880=CARTESIAN_POINT('Ctrl Pts',(5.99915624252742,1.19575849471018,4.50200643361165));
#148881=CARTESIAN_POINT('Ctrl Pts',(6.00747623733207,1.197973174,4.49087672017117));
#148882=CARTESIAN_POINT('Ctrl Pts',(6.2506453581102,1.262701774,4.16558773918303));
#148883=CARTESIAN_POINT('Ctrl Pts',(6.45726863652832,1.327878141,3.81594368619315));
#148884=CARTESIAN_POINT('',(6.00677326593869,1.19797317455196,4.49095479280212));
#148885=CARTESIAN_POINT('',(6.32603274683486,1.28783500530512,4.02880995908792));
#148886=CARTESIAN_POINT('Origin',(-0.165623100425537,1.33927121971452,-0.0956778453126561));
#148887=CARTESIAN_POINT('Ctrl Pts',(6.11450732031872,1.32710049321789,3.89554877299147));
#148888=CARTESIAN_POINT('Ctrl Pts',(6.14968886265092,1.32022179849916,3.91775786528613));
#148889=CARTESIAN_POINT('Ctrl Pts',(6.18492727127714,1.31351590008441,3.93997914081815));
#148890=CARTESIAN_POINT('Ctrl Pts',(6.25542438165227,1.3004385890187,3.9843911417831));
#148891=CARTESIAN_POINT('Ctrl Pts',(6.29072453942237,1.29405949355432,4.00660798123664));
#148892=CARTESIAN_POINT('Ctrl Pts',(6.32603274273498,1.28783500492533,4.02880996550155));
#148893=CARTESIAN_POINT('',(5.83391200081423,1.1979731756145,4.51015201700134));
#148894=CARTESIAN_POINT('Origin',(-2.24213009270002E-13,1.28891221000022,
-1.85615411929518E-13));
#148895=CARTESIAN_POINT('',(6.3289611403479,1.10830076260042,4.02420810597705));
#148896=CARTESIAN_POINT('Origin',(-0.16810700650616,0.94658017581024,-0.0763574613611706));
#148897=CARTESIAN_POINT('',(6.61419164333604,1.19797317358555,3.53588304568532));
#148898=CARTESIAN_POINT('Origin',(-0.173657580831476,1.33917535067201,-0.0672706207730239));
#148899=CARTESIAN_POINT('Ctrl Pts',(6.32603275069163,1.2878350047913,4.02880995297333));
#148900=CARTESIAN_POINT('Ctrl Pts',(6.40989648052783,1.26310656823714,3.89712722091806));
#148901=CARTESIAN_POINT('Ctrl Pts',(6.4894311999038,1.23856749893131,3.76315873619561));
#148902=CARTESIAN_POINT('Ctrl Pts',(6.56448339291637,1.21428571428671,3.62733480452593));
#148903=CARTESIAN_POINT('Ctrl Pts',(6.58125123958283,1.20886077964635,3.59698959050278));
#148904=CARTESIAN_POINT('Ctrl Pts',(6.59782176496324,1.20342302038954,3.5665043947356));
#148905=CARTESIAN_POINT('Ctrl Pts',(6.61419164258928,1.1979731744789,3.53588304601582));
#148906=CARTESIAN_POINT('Ctrl Pts',(6.11194441300001,1.327885473,3.89956863));
#148907=CARTESIAN_POINT('Ctrl Pts',(6.299067458,1.27059961,3.606283458));
#148908=CARTESIAN_POINT('Ctrl Pts',(6.457248486,1.214285714,3.296428672));
#148909=CARTESIAN_POINT('Ctrl Pts',(6.48012364,1.20614195,3.251619405));
#148910=CARTESIAN_POINT('Ctrl Pts',(6.50237472400001,1.197973174,3.20649699));
#148911=CARTESIAN_POINT('Ctrl Pts',(6.187002127,1.327885473,4.239222179));
#148912=CARTESIAN_POINT('Ctrl Pts',(6.390423644,1.27059961,3.94233532));
#148913=CARTESIAN_POINT('Ctrl Pts',(6.564483393,1.214285714,3.627334805));
#148914=CARTESIAN_POINT('Ctrl Pts',(6.589654828,1.20614195,3.581781394));
#148915=CARTESIAN_POINT('Ctrl Pts',(6.61419164600001,1.197973174,3.53588304));
#148916=CARTESIAN_POINT('',(6.55772409853652,1.19797317334244,3.36954308835721));
#148917=CARTESIAN_POINT('Ctrl Pts',(6.49049373074944,1.19354381548256,3.23059015776105));
#148918=CARTESIAN_POINT('Ctrl Pts',(6.49643422737473,1.19575849474129,3.21854357388049));
#148919=CARTESIAN_POINT('Ctrl Pts',(6.502374724,1.197973174,3.20649699));
#148920=CARTESIAN_POINT('Ctrl Pts',(6.675998073,1.262701774,2.854410562));
#148921=CARTESIAN_POINT('Ctrl Pts',(6.810588656,1.327878141,2.485635163));
#148922=CARTESIAN_POINT('Ctrl Pts',(6.82096468986463,1.19354381548255,3.11976882592563));
#148923=CARTESIAN_POINT('Ctrl Pts',(6.82669760832052,1.19575849474129,3.10711076623171));
#148924=CARTESIAN_POINT('Ctrl Pts',(6.83243052677644,1.197973174,3.09445270653778));
#148925=CARTESIAN_POINT('Ctrl Pts',(6.99998697275172,1.262701774,2.72449462819314));
#148926=CARTESIAN_POINT('Ctrl Pts',(7.12661637784409,1.327878141,2.3386071622032));
#148927=CARTESIAN_POINT('',(6.83176077378476,1.19797317455225,3.09468007193932));
#148928=CARTESIAN_POINT('',(7.04420866687487,1.28783500530334,2.57470857667843));
#148929=CARTESIAN_POINT('Origin',(-0.182318938186159,1.33927122879218,-0.0578369172733556));
#148930=CARTESIAN_POINT('Ctrl Pts',(6.80898137204789,1.32710049322087,2.49003467782965));
#148931=CARTESIAN_POINT('Ctrl Pts',(6.84811468746185,1.32022179853825,2.50416154198524));
#148932=CARTESIAN_POINT('Ctrl Pts',(6.88730615901088,1.31351590010567,2.51828808012451));
#148933=CARTESIAN_POINT('Ctrl Pts',(6.96570235315265,1.30043858905459,2.54650695806681));
#148934=CARTESIAN_POINT('Ctrl Pts',(7.00495317668262,1.29405949355901,2.5606158896811));
#148935=CARTESIAN_POINT('Ctrl Pts',(7.04420866416314,1.28783500491492,2.574708583835));
#148936=CARTESIAN_POINT('',(6.66706774467661,1.19797317561536,3.1505885381489));
#148937=CARTESIAN_POINT('Origin',(8.38738800634786E-13,1.28891221000011,
2.08600497986211E-13));
#148938=CARTESIAN_POINT('',(7.04607933373821,1.10830076258659,2.56958479416805));
#148939=CARTESIAN_POINT('Origin',(-0.180591217215621,0.946580170630017,
-0.0384341701045315));
#148940=CARTESIAN_POINT('',(7.21966585287252,1.19797317358556,2.03136037523598));
#148941=CARTESIAN_POINT('Origin',(-0.184058831876451,1.33917531484635,-0.0283666496420124));
#148942=CARTESIAN_POINT('Ctrl Pts',(7.04420866953866,1.28783500479116,2.57470856991552));
#148943=CARTESIAN_POINT('Ctrl Pts',(7.09780381709453,1.26310656824127,2.42807628404456));
#148944=CARTESIAN_POINT('Ctrl Pts',(7.1466797948153,1.23856749893545,2.28014229432938));
#148945=CARTESIAN_POINT('Ctrl Pts',(7.19077917881114,1.21428571428671,2.13135984797882));
#148946=CARTESIAN_POINT('Ctrl Pts',(7.20063167850662,1.20886077964635,2.09811949687777));
#148947=CARTESIAN_POINT('Ctrl Pts',(7.21026137828297,1.20342302038954,2.06478485484036));
#148948=CARTESIAN_POINT('Ctrl Pts',(7.21966585263086,1.1979731744789,2.03136037579649));
#148949=CARTESIAN_POINT('Ctrl Pts',(6.80734253400001,1.327885473,2.494511501));
#148950=CARTESIAN_POINT('Ctrl Pts',(6.927043104,1.27059961,2.167857251));
#148951=CARTESIAN_POINT('Ctrl Pts',(7.014916327,1.214285714,1.831242452));
#148952=CARTESIAN_POINT('Ctrl Pts',(7.02762400500001,1.20614195,1.782563319));
#148953=CARTESIAN_POINT('Ctrl Pts',(7.039654886,1.197973174,1.733712515));
#148954=CARTESIAN_POINT('Ctrl Pts',(6.953660913,1.327885473,2.810088949));
#148955=CARTESIAN_POINT('Ctrl Pts',(7.088504649,1.27059961,2.476413527));
#148956=CARTESIAN_POINT('Ctrl Pts',(7.190779179,1.214285714,2.131359848));
#148957=CARTESIAN_POINT('Ctrl Pts',(7.20556948400001,1.20614195,2.081460337));
#148958=CARTESIAN_POINT('Ctrl Pts',(7.219665854,1.197973174,2.031360369));
#148959=CARTESIAN_POINT('',(7.12966036896448,1.19797317334244,1.88253644592181));
#148960=CARTESIAN_POINT('Ctrl Pts',(7.03323098254006,1.19354381539971,1.75979646067424));
#148961=CARTESIAN_POINT('Ctrl Pts',(7.03644293427003,1.19575849469986,1.74675448783709));
#148962=CARTESIAN_POINT('Ctrl Pts',(7.039654886,1.197973174,1.733712515));
#148963=CARTESIAN_POINT('Ctrl Pts',(7.133530843,1.262701774,1.352533785));
#148964=CARTESIAN_POINT('Ctrl Pts',(7.185698963,1.327878141,0.963447153));
#148965=CARTESIAN_POINT('Ctrl Pts',(7.33215240352332,1.19354381539971,1.58052458316709));
#148966=CARTESIAN_POINT('Ctrl Pts',(7.33503018093462,1.19575849469986,1.56693005361739));
#148967=CARTESIAN_POINT('Ctrl Pts',(7.33790795834591,1.197973174,1.55333552406776));
#148968=CARTESIAN_POINT('Ctrl Pts',(7.4220169771698,1.262701774,1.15600717709109));
#148969=CARTESIAN_POINT('Ctrl Pts',(7.46273145832251,1.327878141,0.751919966756011));
#148970=CARTESIAN_POINT('',(7.33730273884919,1.19797317454273,1.55370155447371));
#148971=CARTESIAN_POINT('',(7.43300521898484,1.28783500531797,1.0002166830984));
#148972=CARTESIAN_POINT('Origin',(-0.190489516960962,1.33927123107037,-0.0172915188586062));
#148973=CARTESIAN_POINT('Ctrl Pts',(7.18507502228507,1.32710049324288,0.968089327893436));
#148974=CARTESIAN_POINT('Ctrl Pts',(7.22633028080292,1.3202217985532,0.973473407793488));
#148975=CARTESIAN_POINT('Ctrl Pts',(7.26764226558942,1.31351590013534,0.978844667424469));
#148976=CARTESIAN_POINT('Ctrl Pts',(7.35027182497301,1.30043858907801,0.989550939350619));
#148977=CARTESIAN_POINT('Ctrl Pts',(7.39163798930367,1.29405949358365,0.994892245192935));
#148978=CARTESIAN_POINT('Ctrl Pts',(7.4330052179612,1.28783500493846,1.00021669060776));
#148979=CARTESIAN_POINT('',(7.18847881074442,1.19797317561536,1.64370704086441));
#148980=CARTESIAN_POINT('Origin',(1.31838984174237E-13,1.28891221000017,
6.00648003556969E-14));
#148981=CARTESIAN_POINT('',(7.43373068909104,1.10830076258966,0.994810553290111));
#148982=CARTESIAN_POINT('Origin',(-0.184631607997902,0.946580187296585,
0.00128611533052506));
#148983=CARTESIAN_POINT('',(7.48755651189144,1.19797317358555,0.431853552262778));
#148984=CARTESIAN_POINT('Origin',(-0.185853746529759,1.33917529040736,0.0118637316038857));
#148985=CARTESIAN_POINT('Ctrl Pts',(7.43300522003748,1.28783500479117,1.00021667597356));
#148986=CARTESIAN_POINT('Ctrl Pts',(7.45382573580307,1.26310656824412,0.845491198897445));
#148987=CARTESIAN_POINT('Ctrl Pts',(7.46975758543086,1.23856749893828,0.690508933277066));
#148988=CARTESIAN_POINT('Ctrl Pts',(7.48084212235679,1.21428571428671,0.535724873766687));
#148989=CARTESIAN_POINT('Ctrl Pts',(7.4833185831773,1.20886077964635,0.501143667390705));
#148990=CARTESIAN_POINT('Ctrl Pts',(7.48555718325301,1.20342302038954,0.466518269919723));
#148991=CARTESIAN_POINT('Ctrl Pts',(7.48755651123012,1.1979731744789,0.431853552880365));
#148992=CARTESIAN_POINT('Ctrl Pts',(7.18443688400001,1.327885473,0.972813787));
#148993=CARTESIAN_POINT('Ctrl Pts',(7.231117913,1.27059961,0.628064447));
#148994=CARTESIAN_POINT('Ctrl Pts',(7.244574478,1.214285714,0.28042937));
#148995=CARTESIAN_POINT('Ctrl Pts',(7.246520483,1.20614195,0.230156553));
#148996=CARTESIAN_POINT('Ctrl Pts',(7.247768609,1.197973174,0.17986157));
#148997=CARTESIAN_POINT('Ctrl Pts',(7.395174244,1.327885473,1.249559084));
#148998=CARTESIAN_POINT('Ctrl Pts',(7.455135056,1.27059961,0.894697389999999));
#148999=CARTESIAN_POINT('Ctrl Pts',(7.480842122,1.214285714,0.535724874));
#149000=CARTESIAN_POINT('Ctrl Pts',(7.484559718,1.20614195,0.483812507));
#149001=CARTESIAN_POINT('Ctrl Pts',(7.487556512,1.197973174,0.431853546));
#149002=CARTESIAN_POINT('',(7.36766256033176,1.19797317334244,0.305857562052724));
#149003=CARTESIAN_POINT('Ctrl Pts',(7.24710217013975,1.19354381559283,0.206716635708786));
#149004=CARTESIAN_POINT('Ctrl Pts',(7.24743538956988,1.19575849479642,0.193289102854393));
#149005=CARTESIAN_POINT('Ctrl Pts',(7.247768609,1.197973174,0.17986157));
#149006=CARTESIAN_POINT('Ctrl Pts',(7.25750763900001,1.262701774,-0.212585969));
#149007=CARTESIAN_POINT('Ctrl Pts',(7.224813973,1.327878141,-0.603790576));
#149008=CARTESIAN_POINT('Ctrl Pts',(7.50049682043428,1.19354381559283,-0.0326232345733736));
#149009=CARTESIAN_POINT('Ctrl Pts',(7.50038489498958,1.19575849479642,-0.0465185680631247));
#149010=CARTESIAN_POINT('Ctrl Pts',(7.50027296954502,1.197973174,-0.0604139015528768));
#149011=CARTESIAN_POINT('Ctrl Pts',(7.49700171593858,1.262701774,-0.466533885824836));
#149012=CARTESIAN_POINT('Ctrl Pts',(7.44989751091891,1.327878141,-0.869926171191936));
#149013=CARTESIAN_POINT('',(7.4997605859831,1.19797317455027,-0.0599263262953898));
#149014=CARTESIAN_POINT('',(7.47424270829533,1.28783500531214,-0.621044231484297));
#149015=CARTESIAN_POINT('Origin',(-0.189753473192996,1.3392712669591,0.0240623826805827));
#149016=CARTESIAN_POINT('Ctrl Pts',(7.22520254964774,1.32710049321762,-0.599122803118063));
#149017=CARTESIAN_POINT('Ctrl Pts',(7.26665070116499,1.32022179856296,-0.602733261078277));
#149018=CARTESIAN_POINT('Ctrl Pts',(7.30815149716335,1.31351590009954,-0.60636843412573));
#149019=CARTESIAN_POINT('Ctrl Pts',(7.39115075537979,1.30043858906754,-0.613675381739156));
#149020=CARTESIAN_POINT('Ctrl Pts',(7.43269802464555,1.29405949358074,-0.617351455288066));
#149021=CARTESIAN_POINT('Ctrl Pts',(7.47424270891332,1.28783500493303,-0.621044223892722));
#149022=CARTESIAN_POINT('',(7.37376459691771,1.19797317561536,0.0599676291186608));
#149023=CARTESIAN_POINT('Origin',(-5.98913280080993E-13,1.28891220999994,
7.57958962521038E-14));
#149024=CARTESIAN_POINT('',(7.47378905921366,1.10830076262361,-0.626479923766747));
#149025=CARTESIAN_POINT('Origin',(-0.180038565926405,0.946580182915173,
0.0409463866725945));
#149026=CARTESIAN_POINT('',(7.40533734948143,1.19797317358556,-1.18784626286482));
#149027=CARTESIAN_POINT('Origin',(-0.178957929364433,1.33917531698094,0.0515394024328136));
#149028=CARTESIAN_POINT('Ctrl Pts',(7.47424270769856,1.28783500479116,-0.621044238693877));
#149029=CARTESIAN_POINT('Ctrl Pts',(7.46131504745461,1.26310656824169,-0.776628115470739));
#149030=CARTESIAN_POINT('Ctrl Pts',(7.44355781343537,1.23856749893588,-0.93141185843771));
#149031=CARTESIAN_POINT('Ctrl Pts',(7.4211092026572,1.21428571428671,-1.08496000029333));
#149032=CARTESIAN_POINT('Ctrl Pts',(7.41609382804624,1.20886077964635,-1.11926508312602));
#149033=CARTESIAN_POINT('Ctrl Pts',(7.41083665397242,1.20342302038954,-1.15356219079986));
#149034=CARTESIAN_POINT('Ctrl Pts',(7.40533734932788,1.1979731744789,-1.18784626221134));
#149035=CARTESIAN_POINT('Ctrl Pts',(7.22559495,1.327885473,-0.594371618));
#149036=CARTESIAN_POINT('Ctrl Pts',(7.197073686,1.27059961,-0.941095951));
#149037=CARTESIAN_POINT('Ctrl Pts',(7.135484378,1.214285714,-1.283496277));
#149038=CARTESIAN_POINT('Ctrl Pts',(7.126577716,1.20614195,-1.333012078));
#149039=CARTESIAN_POINT('Ctrl Pts',(7.116984728,1.197973174,-1.382399502));
#149040=CARTESIAN_POINT('Ctrl Pts',(7.490897446,1.327885473,-0.369398776));
#149041=CARTESIAN_POINT('Ctrl Pts',(7.473171633,1.27059961,-0.728853803));
#149042=CARTESIAN_POINT('Ctrl Pts',(7.421109203,1.214285714,-1.08496));
#149043=CARTESIAN_POINT('Ctrl Pts',(7.413580259,1.20614195,-1.136457858));
#149044=CARTESIAN_POINT('Ctrl Pts',(7.405337348,1.197973174,-1.187846269));
#149045=CARTESIAN_POINT('',(7.26116103870691,1.19797317334244,-1.28512288150586));
#149046=CARTESIAN_POINT('Ctrl Pts',(7.1221069156548,1.19354381541858,-1.35602902712435));
#149047=CARTESIAN_POINT('Ctrl Pts',(7.1195458218274,1.1957584947093,-1.3692142645622));
#149048=CARTESIAN_POINT('Ctrl Pts',(7.116984728,1.197973174,-1.382399502));
#149049=CARTESIAN_POINT('Ctrl Pts',(7.04213144400001,1.262701774,-1.767765439));
#149050=CARTESIAN_POINT('Ctrl Pts',(6.926104711,1.327878141,-2.142795728));
#149051=CARTESIAN_POINT('Ctrl Pts',(7.31812634173865,1.19354381541858,-1.64424562360488));
#149052=CARTESIAN_POINT('Ctrl Pts',(7.31502994699515,1.1957584947093,-1.65779203180329));
#149053=CARTESIAN_POINT('Ctrl Pts',(7.31193355225165,1.197973174,-1.67133844000171));
#149054=CARTESIAN_POINT('Ctrl Pts',(7.22143498767998,1.262701774,-2.06726034228003));
#149055=CARTESIAN_POINT('Ctrl Pts',(7.08871463480692,1.327878141,-2.45109552827173));
#149056=CARTESIAN_POINT('',(7.31153796209935,1.19797317454273,-1.67075211474223));
#149057=CARTESIAN_POINT('',(7.1659929155684,1.28783500526628,-2.21326580745523));
#149058=CARTESIAN_POINT('Origin',(-0.180144164879942,1.33927126523448,0.0642911260606757));
#149059=CARTESIAN_POINT('Ctrl Pts',(6.9274876363475,1.32710049319203,-2.13832061771533));
#149060=CARTESIAN_POINT('Ctrl Pts',(6.96719061146471,1.32022179851475,-2.1507567924955));
#149061=CARTESIAN_POINT('Ctrl Pts',(7.00693968702447,1.31351590007216,-2.16322842146589));
#149062=CARTESIAN_POINT('Ctrl Pts',(7.0864276911202,1.30043858901132,-2.18820692365546));
#149063=CARTESIAN_POINT('Ctrl Pts',(7.12621336121677,1.29405949351721,-2.20072848734333));
#149064=CARTESIAN_POINT('Ctrl Pts',(7.16599291782655,1.28783500485895,-2.21326580008813));
#149065=CARTESIAN_POINT('',(7.21426134609485,1.19797317561536,-1.52657580210022));
#149066=CARTESIAN_POINT('Origin',(-8.25294693695966E-13,1.28891221000017,
3.3436794999453E-13));
#149067=CARTESIAN_POINT('',(7.16438135929131,1.10830076263124,-2.21847689478545));
#149068=CARTESIAN_POINT('Origin',(-0.167026977383227,0.9465801840733,0.07869201776906));
#149069=CARTESIAN_POINT('',(6.9768528436404,1.19797317358556,-2.75200370729668));
#149070=CARTESIAN_POINT('Origin',(-0.163694659924108,1.33917530233932,0.0888051357193126));
#149071=CARTESIAN_POINT('Ctrl Pts',(7.16599291338407,1.28783500479116,-2.2132658144311));
#149072=CARTESIAN_POINT('Ctrl Pts',(7.11992156021712,1.2631065682245,-2.36243316168405));
#149073=CARTESIAN_POINT('Ctrl Pts',(7.06930555112514,1.23856749891882,-2.50978086632341));
#149074=CARTESIAN_POINT('Ctrl Pts',(7.01437346458419,1.21428571428671,-2.65491335062694));
#149075=CARTESIAN_POINT('Ctrl Pts',(7.00210076784224,1.20886077964635,-2.68733824251475));
#149076=CARTESIAN_POINT('Ctrl Pts',(6.98959363920698,1.20342302038954,-2.71970336592745));
#149077=CARTESIAN_POINT('Ctrl Pts',(6.97685284345389,1.1979731744789,-2.75200370653627));
#149078=CARTESIAN_POINT('Ctrl Pts',(6.928892227,1.327885473,-2.133764867));
#149079=CARTESIAN_POINT('Ctrl Pts',(6.826502291,1.27059961,-2.466251749));
#149080=CARTESIAN_POINT('Ctrl Pts',(6.692746959,1.214285714,-2.787407065));
#149081=CARTESIAN_POINT('Ctrl Pts',(6.673404096,1.20614195,-2.833850545));
#149082=CARTESIAN_POINT('Ctrl Pts',(6.65341855,1.197973174,-2.88002111));
#149083=CARTESIAN_POINT('Ctrl Pts',(7.236354609,1.327885473,-1.971083959));
#149084=CARTESIAN_POINT('Ctrl Pts',(7.14177101,1.27059961,-2.318324601));
#149085=CARTESIAN_POINT('Ctrl Pts',(7.014373465,1.214285714,-2.65491335));
#149086=CARTESIAN_POINT('Ctrl Pts',(6.995950026,1.20614195,-2.703588717));
#149087=CARTESIAN_POINT('Ctrl Pts',(6.976852841,1.197973174,-2.752003713));
#149088=CARTESIAN_POINT('',(6.815135697049,1.19797317334244,-2.8160124077512));
#149089=CARTESIAN_POINT('Ctrl Pts',(6.66408985650852,1.19354381535312,-2.85536828075232));
#149090=CARTESIAN_POINT('Ctrl Pts',(6.65875420325428,1.19575849467657,-2.86769469537616));
#149091=CARTESIAN_POINT('Ctrl Pts',(6.65341854999999,1.197973174,-2.88002111));
#149092=CARTESIAN_POINT('Ctrl Pts',(6.497473009,1.262701774,-3.240286162));
#149093=CARTESIAN_POINT('Ctrl Pts',(6.303538491,1.327878141,-3.581606133));
#149094=CARTESIAN_POINT('Ctrl Pts',(6.79356840984586,1.19354381535312,-3.17898491578651));
#149095=CARTESIAN_POINT('Ctrl Pts',(6.78763232966878,1.19575849467657,-3.19154898332476));
#149096=CARTESIAN_POINT('Ctrl Pts',(6.7816962494918,1.197973174,-3.20411305086303));
#149097=CARTESIAN_POINT('Ctrl Pts',(6.60820198543364,1.262701774,-3.57132400255763));
#149098=CARTESIAN_POINT('Ctrl Pts',(6.39607134065686,1.327878141,-3.91765438273399));
#149099=CARTESIAN_POINT('',(6.78143595059185,1.19797317454273,-3.20345539331613));
#149100=CARTESIAN_POINT('',(6.52266925830075,1.28783500530872,-3.70199753484471));
#149101=CARTESIAN_POINT('Origin',(-0.162111689526208,1.3392712357706,0.101513649847844));
#149102=CARTESIAN_POINT('Ctrl Pts',(6.30585109992902,1.32710049333678,-3.57753293576106));
#149103=CARTESIAN_POINT('Ctrl Pts',(6.34195246648704,1.32022179198259,-3.59821334618977));
#149104=CARTESIAN_POINT('Ctrl Pts',(6.37809124102865,1.31351588629104,-3.61893829604711));
#149105=CARTESIAN_POINT('Ctrl Pts',(6.45035114375322,1.30043858906411,-3.66042034248003));
#149106=CARTESIAN_POINT('Ctrl Pts',(6.48651488093728,1.29405949358396,-3.68120190204836));
#149107=CARTESIAN_POINT('Ctrl Pts',(6.52266926205248,1.28783500493332,-3.70199752820974));
#149108=CARTESIAN_POINT('',(6.71742725267403,1.19797317561536,-3.041738245782));
#149109=CARTESIAN_POINT('Origin',(-1.56775634141404E-12,1.28891220999994,
7.56556275960385E-13));
#149110=CARTESIAN_POINT('',(6.51997514986712,1.10830076264337,-3.70674035236029));
#149111=CARTESIAN_POINT('Origin',(-0.146205722694455,0.946580186364563,
0.112758217822082));
#149112=CARTESIAN_POINT('',(6.22213845282096,1.19797317358555,-4.18748051700546));
#149113=CARTESIAN_POINT('Origin',(-0.140777006185144,1.33917528229682,0.121918379441862));
#149114=CARTESIAN_POINT('Ctrl Pts',(6.52266925465969,1.28783500479116,-3.70199754110091));
#149115=CARTESIAN_POINT('Ctrl Pts',(6.44560845380337,1.26310656823854,-3.83777345961638));
#149116=CARTESIAN_POINT('Ctrl Pts',(6.364500417915,1.23856749893275,-3.97079531107751));
#149117=CARTESIAN_POINT('Ctrl Pts',(6.27965341901354,1.21428571428671,-4.10072590367506));
#149118=CARTESIAN_POINT('Ctrl Pts',(6.26069725783425,1.20886077964635,-4.12975445256057));
#149119=CARTESIAN_POINT('Ctrl Pts',(6.24152499419278,1.20342302038954,-4.15867423426439));
#149120=CARTESIAN_POINT('Ctrl Pts',(6.22213845282379,1.1979731744789,-4.18748051624025));
#149121=CARTESIAN_POINT('Ctrl Pts',(6.308202204,1.327885473,-3.573385642));
#149122=CARTESIAN_POINT('Ctrl Pts',(6.136731237,1.27059961,-3.876088357));
#149123=CARTESIAN_POINT('Ctrl Pts',(5.93706413,1.214285714,-4.160981797));
#149124=CARTESIAN_POINT('Ctrl Pts',(5.908189518,1.20614195,-4.20218131));
#149125=CARTESIAN_POINT('Ctrl Pts',(5.878745916,1.197973174,-4.242976131));
#149126=CARTESIAN_POINT('Ctrl Pts',(6.643447873,1.327885473,-3.480603448));
#149127=CARTESIAN_POINT('Ctrl Pts',(6.476429113,1.27059961,-3.799393119));
#149128=CARTESIAN_POINT('Ctrl Pts',(6.279653419,1.214285714,-4.100725903));
#149129=CARTESIAN_POINT('Ctrl Pts',(6.25119694500001,1.20614195,-4.144302772));
#149130=CARTESIAN_POINT('Ctrl Pts',(6.222138449,1.197973174,-4.187480522));
#149131=CARTESIAN_POINT('',(6.0504421848187,1.19797317334243,-4.2152283231718));
#149132=CARTESIAN_POINT('Ctrl Pts',(5.89446736251345,1.19354381545263,-4.22119368712617));
#149133=CARTESIAN_POINT('Ctrl Pts',(5.88660663925671,1.19575849472632,-4.23208490906309));
#149134=CARTESIAN_POINT('Ctrl Pts',(5.878745916,1.197973174,-4.242976131));
#149135=CARTESIAN_POINT('Ctrl Pts',(5.648999958,1.262701774,-4.56129470500001));
#149136=CARTESIAN_POINT('Ctrl Pts',(5.386225817,1.327878141,-4.852944616));
#149137=CARTESIAN_POINT('Ctrl Pts',(5.95135076798055,1.19354381545264,-4.56507840749032));
#149138=CARTESIAN_POINT('Ctrl Pts',(5.94285256712257,1.19575849472632,-4.57607265208447));
#149139=CARTESIAN_POINT('Ctrl Pts',(5.93435436626472,1.197973174,-4.58706689667855));
#149140=CARTESIAN_POINT('Ctrl Pts',(5.68597680180873,1.262701774,-4.9083965217357));
#149141=CARTESIAN_POINT('Ctrl Pts',(5.40435486065015,1.327878141,-5.20102807168802));
#149142=CARTESIAN_POINT('',(5.93424152994601,1.19797317454255,-4.58636865826812));
#149143=CARTESIAN_POINT('',(5.57435283624376,1.28783500529315,-5.01762797127261));
#149144=CARTESIAN_POINT('Origin',(-0.136499289031298,1.33927126171856,0.133989635138438));
#149145=CARTESIAN_POINT('Ctrl Pts',(5.38935997513011,1.32710049341366,-4.8494637911487));
#149146=CARTESIAN_POINT('Ctrl Pts',(5.42017160522032,1.3202217986986,-4.87742140436003));
#149147=CARTESIAN_POINT('Ctrl Pts',(5.451010188688,1.31351590010789,-4.90543055249013));
#149148=CARTESIAN_POINT('Ctrl Pts',(5.51266334654728,1.30043858903252,-4.9614765737824));
#149149=CARTESIAN_POINT('Ctrl Pts',(5.54351417461199,1.29405949355007,-4.98954640642331));
#149150=CARTESIAN_POINT('Ctrl Pts',(5.57435284139363,1.28783500490135,-5.01762796553027));
#149151=CARTESIAN_POINT('',(5.906493726556,1.19797317561482,-4.41467238939753));
#149152=CARTESIAN_POINT('Origin',(2.43772016461641E-12,1.28891220999983,
-2.21610924056037E-12));
#149153=CARTESIAN_POINT('',(5.57070214838859,1.1083007626525,-5.02168075129053));
#149154=CARTESIAN_POINT('Origin',(-0.118547812998999,0.94658017878209,0.141551885277263));
#149155=CARTESIAN_POINT('',(5.17648378289701,1.19797317358556,-5.42715539201615));
#149156=CARTESIAN_POINT('Origin',(-0.111276857755188,1.33917532586237,0.149330892566997));
#149157=CARTESIAN_POINT('Ctrl Pts',(5.57435283129608,1.28783500479126,-5.01762797666601));
#149158=CARTESIAN_POINT('Ctrl Pts',(5.46990586017375,1.26310656823713,-5.13366373537583));
#149159=CARTESIAN_POINT('Ctrl Pts',(5.36209831904503,1.23856749893132,-5.2461397797822));
#149160=CARTESIAN_POINT('Ctrl Pts',(5.25130375913421,1.21428571428671,-5.35479307063336));
#149161=CARTESIAN_POINT('Ctrl Pts',(5.22655050253382,1.20886077964635,-5.37906793386744));
#149162=CARTESIAN_POINT('Ctrl Pts',(5.20160957745708,1.20342302038954,-5.40319011729261));
#149163=CARTESIAN_POINT('Ctrl Pts',(5.17648378317611,1.1979731744789,-5.42715539141038));
#149164=CARTESIAN_POINT('Ctrl Pts',(5.392547658,1.327885473,-4.845918877));
#149165=CARTESIAN_POINT('Ctrl Pts',(5.160013451,1.27059961,-5.10468338));
#149166=CARTESIAN_POINT('Ctrl Pts',(4.903770781,1.214285714,-5.339993645));
#149167=CARTESIAN_POINT('Ctrl Pts',(4.866714564,1.20614195,-5.374022748));
#149168=CARTESIAN_POINT('Ctrl Pts',(4.829189657,1.197973174,-5.40753430500001));
#149169=CARTESIAN_POINT('Ctrl Pts',(5.739900898,1.327885473,-4.827373787));
#149170=CARTESIAN_POINT('Ctrl Pts',(5.50825658799999,1.27059961,-5.102806236));
#149171=CARTESIAN_POINT('Ctrl Pts',(5.251303759,1.214285714,-5.35479307));
#149172=CARTESIAN_POINT('Ctrl Pts',(5.214144843,1.20614195,-5.391233835));
#149173=CARTESIAN_POINT('Ctrl Pts',(5.176483778,1.197973174,-5.427155396));
#149174=CARTESIAN_POINT('',(5.00110024987486,1.19797317334244,-5.41724674229405));
#149175=CARTESIAN_POINT('Ctrl Pts',(4.84922612612734,1.19354381550591,-5.38964076904563));
#149176=CARTESIAN_POINT('Ctrl Pts',(4.83920789156366,1.19575849475297,-5.39858753702288));
#149177=CARTESIAN_POINT('Ctrl Pts',(4.829189657,1.197973174,-5.407534305));
#149178=CARTESIAN_POINT('Ctrl Pts',(4.536385948,1.262701774,-5.669022178));
#149179=CARTESIAN_POINT('Ctrl Pts',(4.21705921,1.327878141,-5.897364803));
#149180=CARTESIAN_POINT('Ctrl Pts',(4.8308545800179,1.19354381550591,-5.73771390554859));
#149181=CARTESIAN_POINT('Ctrl Pts',(4.82019162486587,1.19575849475297,-5.74662424873047));
#149182=CARTESIAN_POINT('Ctrl Pts',(4.80952866971385,1.197973174,-5.75553459191248));
#149183=CARTESIAN_POINT('Ctrl Pts',(4.49788166269152,1.262701774,-6.01595787463447));
#149184=CARTESIAN_POINT('Ctrl Pts',(4.15993675249693,1.327878141,-6.24120746922401));
#149185=CARTESIAN_POINT('',(4.80956857104774,1.19797317455043,-5.75482842296611));
#149186=CARTESIAN_POINT('',(4.36538587067711,1.28783500456851,-6.09863970055502));
#149187=CARTESIAN_POINT('Origin',(-0.104504270684904,1.33927127350409,0.160200449407045));
#149188=CARTESIAN_POINT('Ctrl Pts',(4.22086836875467,1.32710049315245,-5.8946391097756));
#149189=CARTESIAN_POINT('Ctrl Pts',(4.24494957945847,1.3202217984799,-5.9285666791748));
#149190=CARTESIAN_POINT('Ctrl Pts',(4.26904603430032,1.31351590009086,-5.96255037194016));
#149191=CARTESIAN_POINT('Ctrl Pts',(4.3172095375045,1.30043858904136,-6.03053967491418));
#149192=CARTESIAN_POINT('Ctrl Pts',(4.34130490602236,1.29405949355654,-6.06458526663132));
#149193=CARTESIAN_POINT('Ctrl Pts',(4.36538587674004,1.2878350049083,-6.09863969632983));
#149194=CARTESIAN_POINT('',(4.81937911915879,1.19797317561536,-5.5811813588866));
#149195=CARTESIAN_POINT('Origin',(-6.17561557447743E-13,1.28891221000039,
8.67795418857398E-13));
#149196=CARTESIAN_POINT('',(4.36094930658774,1.10830076259545,-6.10181293897598));
#149197=CARTESIAN_POINT('Origin',(-0.0853466450309831,0.946580177243603,
0.16372661055274));
#149198=CARTESIAN_POINT('',(3.8887824855194,1.19797317379345,-6.41306251204082));
#149199=CARTESIAN_POINT('Origin',(-0.0765736300821324,1.33917535499471,
0.169761002796281));
#149200=CARTESIAN_POINT('Ctrl Pts',(4.36538586477892,1.28783500266228,-6.09863970449737));
#149201=CARTESIAN_POINT('Ctrl Pts',(4.23843654752548,1.26310656752412,-6.18950960074403));
#149202=CARTESIAN_POINT('Ctrl Pts',(4.10897046193337,1.23856749892619,-6.27618058321672));
#149203=CARTESIAN_POINT('Ctrl Pts',(3.97740897184098,1.2142857140719,-6.35847606461084));
#149204=CARTESIAN_POINT('Ctrl Pts',(3.94801605496087,1.20886077973443,-6.37686217615265));
#149205=CARTESIAN_POINT('Ctrl Pts',(3.91847267837239,1.20342302059143,-6.39505883492393));
#149206=CARTESIAN_POINT('Ctrl Pts',(3.88878248571163,1.1979731751026,-6.41306251127484));
#149207=CARTESIAN_POINT('Ctrl Pts',(4.224743576,1.327885473,-5.89186233000001));
#149208=CARTESIAN_POINT('Ctrl Pts',(3.94201917,1.27059961,-6.094589083));
#149209=CARTESIAN_POINT('Ctrl Pts',(3.641182561,1.214285714,-6.269313324));
#149210=CARTESIAN_POINT('Ctrl Pts',(3.597677446,1.20614195,-6.294580855));
#149211=CARTESIAN_POINT('Ctrl Pts',(3.553825856,1.197973174,-6.319242184));
#149212=CARTESIAN_POINT('Ctrl Pts',(4.567962537,1.327885473,-5.948421493));
#149213=CARTESIAN_POINT('Ctrl Pts',(4.282524107,1.27059961,-6.167617806));
#149214=CARTESIAN_POINT('Ctrl Pts',(3.977408972,1.214285714,-6.358476065));
#149215=CARTESIAN_POINT('Ctrl Pts',(3.933285124,1.20614195,-6.38607679600001));
#149216=CARTESIAN_POINT('Ctrl Pts',(3.88878248,1.197973174,-6.413062515));
#149217=CARTESIAN_POINT('',(3.72130417150183,1.19797317334244,-6.36615234745303));
#149218=CARTESIAN_POINT('Ctrl Pts',(3.5772404657506,1.19354381534562,-6.30607423705896));
#149219=CARTESIAN_POINT('Ctrl Pts',(3.56553316087531,1.19575849467282,-6.31265821052942));
#149220=CARTESIAN_POINT('Ctrl Pts',(3.553825856,1.197973174,-6.319242184));
#149221=CARTESIAN_POINT('Ctrl Pts',(3.211655572,1.262701774,-6.511672474));
#149222=CARTESIAN_POINT('Ctrl Pts',(2.850707601,1.327878141,-6.666030766));
#149223=CARTESIAN_POINT('Ctrl Pts',(3.48447300063436,1.19354381534562,-6.64206027784984));
#149224=CARTESIAN_POINT('Ctrl Pts',(3.47214387864852,1.19575849467282,-6.64847008224919));
#149225=CARTESIAN_POINT('Ctrl Pts',(3.45981475666261,1.197973174,-6.65487988664856));
#149226=CARTESIAN_POINT('Ctrl Pts',(3.09947057699739,1.262701774,-6.84221972404721));
#149227=CARTESIAN_POINT('Ctrl Pts',(2.72100462632398,1.327878141,-6.98955494174905));
#149228=CARTESIAN_POINT('',(3.46000553056191,1.19797317455044,-6.6541988051439));
#149229=CARTESIAN_POINT('',(2.95229831384228,1.28783500532053,-6.89448581602087));
#149230=CARTESIAN_POINT('Origin',(-0.0676225476017656,1.33927124513901,
0.178920113634683));
#149231=CARTESIAN_POINT('Ctrl Pts',(2.85501364690942,1.32710049333567,-6.66418765315929));
#149232=CARTESIAN_POINT('Ctrl Pts',(2.87123842778919,1.32022179868456,-6.70249876327353));
#149233=CARTESIAN_POINT('Ctrl Pts',(2.88746603208701,1.31351590010048,-6.74086796289427));
#149234=CARTESIAN_POINT('Ctrl Pts',(2.91988780911154,1.30043858907498,-6.81762144325761));
#149235=CARTESIAN_POINT('Ctrl Pts',(2.93610104555493,1.29405949359601,-6.85605085997186));
#149236=CARTESIAN_POINT('Ctrl Pts',(2.95229832091699,1.28783500494432,-6.89448581297852));
#149237=CARTESIAN_POINT('',(3.50691569940141,1.19797317561536,-6.48672049068763));
#149238=CARTESIAN_POINT('Origin',(-5.07406616723216E-13,1.28891220999994,
1.13364179155084E-12));
#149239=CARTESIAN_POINT('',(2.94728332132464,1.10830076261527,-6.89663113553974));
#149240=CARTESIAN_POINT('Origin',(-0.048155014798249,0.946580161353691,
0.178246000753397));
#149241=CARTESIAN_POINT('',(2.41924604010438,1.19797317358556,-7.09910195741526));
#149242=CARTESIAN_POINT('Origin',(-0.0382896729873458,1.33917527452691,
0.182252827141014));
#149243=CARTESIAN_POINT('Ctrl Pts',(2.95229830709036,1.28783500479117,-6.894485818823));
#149244=CARTESIAN_POINT('Ctrl Pts',(2.8087826528535,1.26310656824939,-6.95594087641231));
#149245=CARTESIAN_POINT('Ctrl Pts',(2.66371171324971,1.23856749894351,-7.01275415801446));
#149246=CARTESIAN_POINT('Ctrl Pts',(2.51753496156429,1.21428571428671,-7.06484378576778));
#149247=CARTESIAN_POINT('Ctrl Pts',(2.48487676386419,1.20886077964635,-7.0764814322586));
#149248=CARTESIAN_POINT('Ctrl Pts',(2.45211235138882,1.20342302038954,-7.08790171038468));
#149249=CARTESIAN_POINT('Ctrl Pts',(2.41924604060176,1.1979731744789,-7.09910195694024));
#149250=CARTESIAN_POINT('Ctrl Pts',(2.85939518,1.327885473,-6.66230884900001));
#149251=CARTESIAN_POINT('Ctrl Pts',(2.539700455,1.27059961,-6.799518573));
#149252=CARTESIAN_POINT('Ctrl Pts',(2.208336691,1.214285714,-6.905486881));
#149253=CARTESIAN_POINT('Ctrl Pts',(2.16041693,1.20614195,-6.920811357));
#149254=CARTESIAN_POINT('Ctrl Pts',(2.112289109,1.197973174,-6.93546932199999));
#149255=CARTESIAN_POINT('Ctrl Pts',(3.182431324,1.327885473,-6.791327622));
#149256=CARTESIAN_POINT('Ctrl Pts',(2.856545558,1.27059961,-6.944038421));
#149257=CARTESIAN_POINT('Ctrl Pts',(2.517534962,1.214285714,-7.064843786));
#149258=CARTESIAN_POINT('Ctrl Pts',(2.468509363,1.20614195,-7.082313904));
#149259=CARTESIAN_POINT('Ctrl Pts',(2.419246034,1.197973174,-7.099101959));
#149260=CARTESIAN_POINT('',(2.26576757536,1.19797317334244,-7.01728563925367));
#149261=CARTESIAN_POINT('Ctrl Pts',(2.13798701621293,1.19354381558494,-6.92764268374129));
#149262=CARTESIAN_POINT('Ctrl Pts',(2.12513806260643,1.19575849479248,-6.93155600287059));
#149263=CARTESIAN_POINT('Ctrl Pts',(2.112289109,1.197973174,-6.935469322));
#149264=CARTESIAN_POINT('Ctrl Pts',(1.736751751,1.262701774,-7.049844202));
#149265=CARTESIAN_POINT('Ctrl Pts',(1.351060074,1.327878141,-7.123000539));
#149266=CARTESIAN_POINT('Ctrl Pts',(1.97516133521341,1.19354381558494,-7.2358312953567));
#149267=CARTESIAN_POINT('Ctrl Pts',(1.96174254347939,1.19575849479248,-7.23944084507777));
#149268=CARTESIAN_POINT('Ctrl Pts',(1.94832375174542,1.197973174,-7.24305039479882));
#149269=CARTESIAN_POINT('Ctrl Pts',(1.55613169084436,1.262701774,-7.34854698287401));
#149270=CARTESIAN_POINT('Ctrl Pts',(1.15484134686268,1.327878141,-7.41107859406688));
#149271=CARTESIAN_POINT('',(1.94865647594488,1.19797317455223,-7.2424262484091));
#149272=CARTESIAN_POINT('',(1.40116456872723,1.28783500529828,-7.3679534371202));
#149273=CARTESIAN_POINT('Origin',(-0.0275791123912514,1.33927124802198,
0.189274290450747));
#149274=CARTESIAN_POINT('Ctrl Pts',(1.3556616617783,1.3271004931861,-7.12212619073517));
#149275=CARTESIAN_POINT('Ctrl Pts',(1.363271367675,1.32022179142973,-7.1630294988622));
#149276=CARTESIAN_POINT('Ctrl Pts',(1.37087134459537,1.31351588546559,-7.20399015161181));
#149277=CARTESIAN_POINT('Ctrl Pts',(1.38603537174766,1.30043858905527,-7.28591881024255));
#149278=CARTESIAN_POINT('Ctrl Pts',(1.39360836300028,1.29405949356432,-7.32693513514737));
#149279=CARTESIAN_POINT('Ctrl Pts',(1.40116457621226,1.28783500491313,-7.3679534356829));
#149280=CARTESIAN_POINT('',(2.03047280022782,1.19797317561536,-7.08894778221368));
#149281=CARTESIAN_POINT('Origin',(3.27049585330252E-13,1.28891220999989,
-1.46757606067638E-12));
#149282=CARTESIAN_POINT('',(1.39580564426377,1.10830076261413,-7.36897052498051));
#149283=CARTESIAN_POINT('Origin',(-0.00871150746413529,0.946580172873321,
0.184430426260994));
#149284=CARTESIAN_POINT('',(0.83658833931585,1.19797317358555,-7.45319528481688));
#149285=CARTESIAN_POINT('Origin',(0.00178446839071103,1.33917534057801,
0.186223212724637));
#149286=CARTESIAN_POINT('Ctrl Pts',(1.40116456161428,1.28783500479117,-7.36795343845741));
#149287=CARTESIAN_POINT('Ctrl Pts',(1.24779320284748,1.26310656823488,-7.39712008757723));
#149288=CARTESIAN_POINT('Ctrl Pts',(1.0939007651504,1.23856749892911,-7.42141914245925));
#149289=CARTESIAN_POINT('Ctrl Pts',(0.939943814464729,1.21428571428671,
-7.44086726300433));
#149290=CARTESIAN_POINT('Ctrl Pts',(0.905547397265625,1.20886077964635,
-7.44521228065392));
#149291=CARTESIAN_POINT('Ctrl Pts',(0.871093976328095,1.20342302038954,
-7.4493221788494));
#149292=CARTESIAN_POINT('Ctrl Pts',(0.836588339905451,1.1979731744789,-7.45319528454301));
#149293=CARTESIAN_POINT('Ctrl Pts',(1.360344644,1.327885473,-7.121233211));
#149294=CARTESIAN_POINT('Ctrl Pts',(1.018628168,1.27059961,-7.186510132));
#149295=CARTESIAN_POINT('Ctrl Pts',(0.672231452,1.214285714,-7.218767545));
#149296=CARTESIAN_POINT('Ctrl Pts',(0.622137718,1.20614195,-7.223432411));
#149297=CARTESIAN_POINT('Ctrl Pts',(0.57198407,1.197973174,-7.227401623));
#149298=CARTESIAN_POINT('Ctrl Pts',(1.64809316,1.327885473,-7.316678819));
#149299=CARTESIAN_POINT('Ctrl Pts',(1.296998114,1.27059961,-7.395763518));
#149300=CARTESIAN_POINT('Ctrl Pts',(0.939943815,1.214285714,-7.440867263));
#149301=CARTESIAN_POINT('Ctrl Pts',(0.888308847999999,1.20614195,-7.447389885));
#149302=CARTESIAN_POINT('Ctrl Pts',(0.836588333,1.197973174,-7.453195285));
#149303=CARTESIAN_POINT('',(0.704286205537718,1.19797317334243,-7.34029845361259));
#149304=CARTESIAN_POINT('Ctrl Pts',(0.58215939042632,1.19629017123951,-7.22659633756481));
#149305=CARTESIAN_POINT('Ctrl Pts',(0.577071730213161,1.19713167261975,
-7.2269989802824));
#149306=CARTESIAN_POINT('Ctrl Pts',(0.57198407,1.197973174,-7.227401623));
#149307=CARTESIAN_POINT('Ctrl Pts',(0.180639349,1.262701774,-7.258373051));
#149308=CARTESIAN_POINT('Ctrl Pts',(-0.211761522,1.327878141,-7.246906723));
#149309=CARTESIAN_POINT('Ctrl Pts',(0.356564099953848,1.19629017123951,
-7.49172316926537));
#149310=CARTESIAN_POINT('Ctrl Pts',(0.351290030198813,1.19713167261975,
-7.49196674389207));
#149311=CARTESIAN_POINT('Ctrl Pts',(0.346015960443778,1.197973174,-7.49221031851878));
#149312=CARTESIAN_POINT('Ctrl Pts',(-0.0596674520371902,1.262701774,-7.51094616964391));
#149313=CARTESIAN_POINT('Ctrl Pts',(-0.465002005850376,1.327878141,-7.48576753873542));
#149314=CARTESIAN_POINT('Ctrl Pts',(-0.207079557678091,1.32710049326789,
-7.24704202133301));
#149315=CARTESIAN_POINT('Ctrl Pts',(-0.208440763000792,1.32022179860809,
-7.28862485198612));
#149316=CARTESIAN_POINT('Ctrl Pts',(-0.209823796958759,1.31351590008895,
-7.33026158825384));
#149317=CARTESIAN_POINT('Ctrl Pts',(-0.212626538934049,1.3004385890535,
-7.41353471129152));
#149318=CARTESIAN_POINT('Ctrl Pts',(-0.214047897279587,1.29405949356574,
-7.4552200665951));
#149319=CARTESIAN_POINT('Ctrl Pts',(-0.215486066129174,1.28783500491842,
-7.49690374451352));
#149320=CARTESIAN_POINT('',(0.459087249099366,1.19797317561536,-7.35970375387002));
#149321=CARTESIAN_POINT('Ctrl Pts',(-0.202314096,1.327885473,-7.247176623));
#149322=CARTESIAN_POINT('Ctrl Pts',(-0.550074039,1.27059961,-7.237468465));
#149323=CARTESIAN_POINT('Ctrl Pts',(-0.895306583,1.214285714,-7.194506663));
#149324=CARTESIAN_POINT('Ctrl Pts',(-0.945231961,1.20614195,-7.188293795));
#149325=CARTESIAN_POINT('Ctrl Pts',(-0.995066308,1.197973174,-7.18138865700001));
#149326=CARTESIAN_POINT('Ctrl Pts',(0.036691991,1.327885473,-7.499910246));
#149327=CARTESIAN_POINT('Ctrl Pts',(-0.32319552,1.27059961,-7.501670932));
#149328=CARTESIAN_POINT('Ctrl Pts',(-0.68159806,1.214285714,-7.468964057));
#149329=CARTESIAN_POINT('Ctrl Pts',(-0.733428001,1.20614195,-7.464234193));
#149330=CARTESIAN_POINT('Ctrl Pts',(-0.785187309000001,1.197973174,-7.458785484));
#149331=CARTESIAN_POINT('',(-0.891176199469163,1.19797317334243,-7.31870008685522));
#149332=CARTESIAN_POINT('Ctrl Pts',(-0.968457199100814,1.19354381560796,
-7.18507566364082));
#149333=CARTESIAN_POINT('Ctrl Pts',(-0.981761753550408,1.19575849480399,
-7.18323216032035));
#149334=CARTESIAN_POINT('Ctrl Pts',(-0.995066308,1.197973174,-7.181388657));
#149335=CARTESIAN_POINT('Ctrl Pts',(-1.383919549,1.262701774,-7.127508443));
#149336=CARTESIAN_POINT('Ctrl Pts',(-1.764681383,1.327878141,-7.031955604));
#149337=CARTESIAN_POINT('Ctrl Pts',(-1.2456388240592,1.19354381560796,-7.39641134329257));
#149338=CARTESIAN_POINT('Ctrl Pts',(-1.25933300010969,1.19575849480399,
-7.39405287748723));
#149339=CARTESIAN_POINT('Ctrl Pts',(-1.27302717616021,1.197973174,-7.39169441168189));
#149340=CARTESIAN_POINT('Ctrl Pts',(-1.67326791779803,1.262701774,-7.3227633493398));
#149341=CARTESIAN_POINT('Ctrl Pts',(-2.06372551153718,1.327878141,-7.21101806044767));
#149342=CARTESIAN_POINT('',(-1.27246312940616,1.19797317455041,-7.39126765888065));
#149343=CARTESIAN_POINT('',(-1.82206082722797,1.28783500530981,-7.27530716460066));
#149344=CARTESIAN_POINT('Origin',(0.0544441017013819,1.33927126085593,0.183360881233009));
#149345=CARTESIAN_POINT('Ctrl Pts',(-1.76013796609859,1.32710049327885,
-7.03309422332733));
#149346=CARTESIAN_POINT('Ctrl Pts',(-1.77040642661513,1.32022179858301,
-7.07341225150022));
#149347=CARTESIAN_POINT('Ctrl Pts',(-1.78070779347286,1.31351590010311,
-7.11377823212063));
#149348=CARTESIAN_POINT('Ctrl Pts',(-1.80134626890961,1.30043858904812,
-7.19450196890768));
#149349=CARTESIAN_POINT('Ctrl Pts',(-1.81169551593028,1.29405949356084,
-7.23490719362557));
#149350=CARTESIAN_POINT('Ctrl Pts',(-1.82206081984535,1.28783500492573,
-7.27530716638796));
#149351=CARTESIAN_POINT('',(-1.13376471150132,1.19797317561536,-7.28632815855581));
#149352=CARTESIAN_POINT('Origin',(-2.23020386880268E-13,1.28891221000011,
-6.04551131377917E-13));
#149353=CARTESIAN_POINT('',(-1.82735151989587,1.10830076259781,-7.27398009464002));
#149354=CARTESIAN_POINT('Origin',(0.0695339604227713,0.946580200554579,
0.171042320190786));
#149355=CARTESIAN_POINT('',(-2.37024845919407,1.19797317358555,-7.11561116450251));
#149356=CARTESIAN_POINT('Origin',(0.0798126674574673,1.33917527750901,0.168262470116188));
#149357=CARTESIAN_POINT('Ctrl Pts',(-1.82206083427004,1.28783500479117,
-7.27530716301513));
#149358=CARTESIAN_POINT('Ctrl Pts',(-1.97350366785731,1.26310656824179,
-7.23737913475084));
#149359=CARTESIAN_POINT('Ctrl Pts',(-2.12337557015445,1.23856749893597,
-7.19481460220206));
#149360=CARTESIAN_POINT('Ctrl Pts',(-2.27126916793713,1.21428571428671,
-7.14782039273359));
#149361=CARTESIAN_POINT('Ctrl Pts',(-2.30431093621273,1.20886077964635,
-7.13732114325402));
#149362=CARTESIAN_POINT('Ctrl Pts',(-2.33730571565235,1.20342302038954,
-7.12658456987032));
#149363=CARTESIAN_POINT('Ctrl Pts',(-2.37024845855447,1.1979731744789,-7.11561116452552));
#149364=CARTESIAN_POINT('Ctrl Pts',(-1.755512854,1.327885473,-7.034250111));
#149365=CARTESIAN_POINT('Ctrl Pts',(-2.093055395,1.27059961,-6.950010816));
#149366=CARTESIAN_POINT('Ctrl Pts',(-2.420981077,1.214285714,-6.833838645));
#149367=CARTESIAN_POINT('Ctrl Pts',(-2.468403645,1.20614195,-6.81703855));
#149368=CARTESIAN_POINT('Ctrl Pts',(-2.515588492,1.197973174,-6.799581939));
#149369=CARTESIAN_POINT('Ctrl Pts',(-1.576424854,1.327885473,-7.332454206));
#149370=CARTESIAN_POINT('Ctrl Pts',(-1.928276891,1.27059961,-7.256808551));
#149371=CARTESIAN_POINT('Ctrl Pts',(-2.271269168,1.214285714,-7.147820393));
#149372=CARTESIAN_POINT('Ctrl Pts',(-2.320870572,1.20614195,-7.132059205));
#149373=CARTESIAN_POINT('Ctrl Pts',(-2.370248465,1.197973174,-7.115611162));
#149374=CARTESIAN_POINT('',(-2.44291847467279,1.19797317334243,-6.95759655184379));
#149375=CARTESIAN_POINT('Ctrl Pts',(-2.49039408591104,1.1935438154537,-6.80890291765712));
#149376=CARTESIAN_POINT('Ctrl Pts',(-2.50299128895552,1.19575849472686,
-6.80424242832863));
#149377=CARTESIAN_POINT('Ctrl Pts',(-2.515588492,1.197973174,-6.799581939));
#149378=CARTESIAN_POINT('Ctrl Pts',(-2.883767906,1.262701774,-6.663369462));
#149379=CARTESIAN_POINT('Ctrl Pts',(-3.235086705,1.327878141,-6.488198056));
#149380=CARTESIAN_POINT('Ctrl Pts',(-2.80652628216,1.1935438154537,-6.95571182999812));
#149381=CARTESIAN_POINT('Ctrl Pts',(-2.81939329600743,1.19575849472686,
-6.95046466061263));
#149382=CARTESIAN_POINT('Ctrl Pts',(-2.8322603098548,1.197973174,-6.94521749122715));
#149383=CARTESIAN_POINT('Ctrl Pts',(-3.20832550476615,1.262701774,-6.79185807146668));
#149384=CARTESIAN_POINT('Ctrl Pts',(-3.56563248304387,1.327878141,-6.59878848428515));
#149385=CARTESIAN_POINT('',(-2.8316177091298,1.19797317454273,-6.94492196922394));
#149386=CARTESIAN_POINT('',(-3.34343804166085,1.28783500532529,-6.7135253081941));
#149387=CARTESIAN_POINT('Origin',(0.0925882930369026,1.33927124656572,0.1673699350441));
#149388=CARTESIAN_POINT('Ctrl Pts',(-3.23089427947231,1.32710049338896,
-6.49028675465296));
#149389=CARTESIAN_POINT('Ctrl Pts',(-3.24958985330599,1.32022179872908,
-6.52745475421011));
#149390=CARTESIAN_POINT('Ctrl Pts',(-3.26832787295305,1.31351590012493,
-6.56466251208682));
#149391=CARTESIAN_POINT('Ctrl Pts',(-3.30583704956096,1.30043858908713,
-6.63906231072451));
#149392=CARTESIAN_POINT('Ctrl Pts',(-3.32463026587,1.2940594936109,-6.67629810155961));
#149393=CARTESIAN_POINT('Ctrl Pts',(-3.34343803473179,1.28783500495311,
-6.71352531163254));
#149394=CARTESIAN_POINT('',(-2.67360309456954,1.19797317561536,-6.87225195616886));
#149395=CARTESIAN_POINT('Origin',(5.89589141397617E-13,1.28891220999994,
1.17961196366423E-12));
#149396=CARTESIAN_POINT('',(-3.34831975995875,1.10830076259067,-6.71109192160037));
#149397=CARTESIAN_POINT('Origin',(0.104677516905148,0.9465801534167,0.15209608589477));
#149398=CARTESIAN_POINT('',(-3.84447943177203,1.19797317358555,-6.43971877546426));
#149399=CARTESIAN_POINT('Origin',(0.11411821151431,1.33917529218569,0.147171347802511));
#149400=CARTESIAN_POINT('Ctrl Pts',(-3.34343804816636,1.28783500479116,
-6.71352530479133));
#149401=CARTESIAN_POINT('Ctrl Pts',(-3.48318682739452,1.26310656825249,
-6.6439282802113));
#149402=CARTESIAN_POINT('Ctrl Pts',(-3.62040469149621,1.23856749894659,
-6.57014085403775));
#149403=CARTESIAN_POINT('Ctrl Pts',(-3.75473825356999,1.21428571428671,
-6.49245259106127));
#149404=CARTESIAN_POINT('Ctrl Pts',(-3.78475049544037,1.20886077964635,
-6.47509580469347));
#149405=CARTESIAN_POINT('Ctrl Pts',(-3.81466582933347,1.20342302038954,
-6.45751734418185));
#149406=CARTESIAN_POINT('Ctrl Pts',(-3.84447943092854,1.1979731744789,-6.43971877531678));
#149407=CARTESIAN_POINT('Ctrl Pts',(-3.226625782,1.327885473,-6.492409881));
#149408=CARTESIAN_POINT('Ctrl Pts',(-3.538167808,1.27059961,-6.337578385));
#149409=CARTESIAN_POINT('Ctrl Pts',(-3.833453187,1.214285714,-6.153627927));
#149410=CARTESIAN_POINT('Ctrl Pts',(-3.876155517,1.20614195,-6.127026159));
#149411=CARTESIAN_POINT('Ctrl Pts',(-3.918484554,1.197973174,-6.099834326));
#149412=CARTESIAN_POINT('Ctrl Pts',(-3.115829826,1.327885473,-6.822140756));
#149413=CARTESIAN_POINT('Ctrl Pts',(-3.443194178,1.27059961,-6.672625868));
#149414=CARTESIAN_POINT('Ctrl Pts',(-3.754738253,1.214285714,-6.492452591));
#149415=CARTESIAN_POINT('Ctrl Pts',(-3.799791815,1.20614195,-6.466397055));
#149416=CARTESIAN_POINT('Ctrl Pts',(-3.844479437,1.197973174,-6.439718772));
#149417=CARTESIAN_POINT('',(-3.88148199205115,1.19797317334243,-6.26977655113511));
#149418=CARTESIAN_POINT('Ctrl Pts',(-3.89588291386022,1.19354381541423,
-6.11435343807459));
#149419=CARTESIAN_POINT('Ctrl Pts',(-3.90718373393015,1.19575849470712,
-6.10709388203729));
#149420=CARTESIAN_POINT('Ctrl Pts',(-3.918484554,1.197973174,-6.099834326));
#149421=CARTESIAN_POINT('Ctrl Pts',(-4.248774481,1.262701774,-5.88765873000001));
#149422=CARTESIAN_POINT('Ctrl Pts',(-4.554222968,1.327878141,-5.64105957800001));
#149423=CARTESIAN_POINT('Ctrl Pts',(-4.23618369053357,1.19354381541423,
-6.18977096269262));
#149424=CARTESIAN_POINT('Ctrl Pts',(-4.24762189454677,1.19575849470712,
-6.18188044151138));
#149425=CARTESIAN_POINT('Ctrl Pts',(-4.25906009855998,1.197973174,-6.17398992033001));
#149426=CARTESIAN_POINT('Ctrl Pts',(-4.59336535651276,1.262701774,-5.94337305811416));
#149427=CARTESIAN_POINT('Ctrl Pts',(-4.90081444214904,1.327878141,-5.67800689188693));
#149428=CARTESIAN_POINT('',(-4.25836899300359,1.19797317454273,-6.17383944762984));
#149429=CARTESIAN_POINT('',(-4.70847980871937,1.28783500530451,-5.8378264697988));
#149430=CARTESIAN_POINT('Origin',(0.126403182263362,1.33927124458626,0.143553125576412));
#149431=CARTESIAN_POINT('Ctrl Pts',(-4.55057756705452,1.32710049336331,
-5.64400069165213));
#149432=CARTESIAN_POINT('Ctrl Pts',(-4.57682609843695,1.32022179125174,
-5.67628076316447));
#149433=CARTESIAN_POINT('Ctrl Pts',(-4.60312463505521,1.31351588473637,
-5.70859054488373));
#149434=CARTESIAN_POINT('Ctrl Pts',(-4.65575056354625,1.30043858906023,
-5.77318747748391));
#149435=CARTESIAN_POINT('Ctrl Pts',(-4.68210899927401,1.29405949356967,
-5.80551273035381));
#149436=CARTESIAN_POINT('Ctrl Pts',(-4.70847980266873,1.28783500491202,
-5.83782647466103));
#149437=CARTESIAN_POINT('',(-4.08842676807871,1.19797317561536,-6.13683689011035));
#149438=CARTESIAN_POINT('Origin',(4.31512464649231E-13,1.28891221,4.57533316788883E-13));
#149439=CARTESIAN_POINT('',(-4.7127242894234,1.10830076263122,-5.83440054895487));
#149440=CARTESIAN_POINT('Origin',(0.134926314667311,0.946580160217586,0.126037513835028));
#149441=CARTESIAN_POINT('',(-5.13894681866872,1.19797317358555,-5.46271229354926));
#149442=CARTESIAN_POINT('Origin',(0.143087622784005,1.33917531549964,0.119198448529405));
#149443=CARTESIAN_POINT('Ctrl Pts',(-4.70847981442621,1.28783500479116,
-5.83782646514444));
#149444=CARTESIAN_POINT('Ctrl Pts',(-4.83000004185364,1.26310656824579,
-5.73981472373645));
#149445=CARTESIAN_POINT('Ctrl Pts',(-4.9481477130839,1.23856749893994,-5.63825462191149));
#149446=CARTESIAN_POINT('Ctrl Pts',(-5.06263995080713,1.21428571428671,
-5.5335049226048));
#149447=CARTESIAN_POINT('Ctrl Pts',(-5.0882193270905,1.20886077964635,-5.51010218345481));
#149448=CARTESIAN_POINT('Ctrl Pts',(-5.11365640767485,1.20342302038954,
-5.48650378512226));
#149449=CARTESIAN_POINT('Ctrl Pts',(-5.13894681787265,1.1979731744789,-5.46271229363917));
#149450=CARTESIAN_POINT('Ctrl Pts',(-4.546865274,1.327885473,-5.646991781));
#149451=CARTESIAN_POINT('Ctrl Pts',(-4.817839426,1.27059961,-5.428807833));
#149452=CARTESIAN_POINT('Ctrl Pts',(-5.066677286,1.214285714,-5.185680407));
#149453=CARTESIAN_POINT('Ctrl Pts',(-5.102662666,1.20614195,-5.150520834));
#149454=CARTESIAN_POINT('Ctrl Pts',(-5.138156632,1.197973174,-5.11486524));
#149455=CARTESIAN_POINT('Ctrl Pts',(-4.509542057,1.327885473,-5.992831587));
#149456=CARTESIAN_POINT('Ctrl Pts',(-4.79711153099999,1.27059961,-5.776438615));
#149457=CARTESIAN_POINT('Ctrl Pts',(-5.062639951,1.214285714,-5.533504923));
#149458=CARTESIAN_POINT('Ctrl Pts',(-5.101039015,1.20614195,-5.498373367));
#149459=CARTESIAN_POINT('Ctrl Pts',(-5.138946823,1.197973174,-5.462712289));
#149460=CARTESIAN_POINT('',(-5.1385517245908,1.19797317334244,-5.28878876732656));
#149461=CARTESIAN_POINT('Ctrl Pts',(-5.11920458538267,1.19354381539211,
-5.13390358796375));
#149462=CARTESIAN_POINT('Ctrl Pts',(-5.12868060869134,1.19575849469606,
-5.12438441398191));
#149463=CARTESIAN_POINT('Ctrl Pts',(-5.138156632,1.197973174,-5.11486524));
#149464=CARTESIAN_POINT('Ctrl Pts',(-5.415113084,1.262701774,-4.83664762));
#149465=CARTESIAN_POINT('Ctrl Pts',(-5.660408826,1.327878141,-4.530151423));
#149466=CARTESIAN_POINT('Ctrl Pts',(-5.46776185838861,1.19354381539211,
-5.13440328426325));
#149467=CARTESIAN_POINT('Ctrl Pts',(-5.47723641480399,1.19575849469606,
-5.12423836326934));
#149468=CARTESIAN_POINT('Ctrl Pts',(-5.48671097121949,1.197973174,-5.11407344227553));
#149469=CARTESIAN_POINT('Ctrl Pts',(-5.76362455022114,1.262701774,-4.81698252537818));
#149470=CARTESIAN_POINT('Ctrl Pts',(-6.00683976539369,1.327878141,-4.491728007792));
#149471=CARTESIAN_POINT('',(-5.48600367772827,1.19797317455045,-5.11407505386022));
#149472=CARTESIAN_POINT('',(-5.85335829410381,1.28783500453097,-4.68915735316194));
#149473=CARTESIAN_POINT('Origin',(0.154307624290183,1.33927127224265,0.113023985986638));
#149474=CARTESIAN_POINT('Ctrl Pts',(-5.65748090612999,1.32710049329292,
-4.53380742867848));
#149475=CARTESIAN_POINT('Ctrl Pts',(-5.69005498758505,1.32022179858842,
-4.55969012397402));
#149476=CARTESIAN_POINT('Ctrl Pts',(-5.72268428531977,1.31351590006272,
-4.585591079946));
#149477=CARTESIAN_POINT('Ctrl Pts',(-5.78796635628563,1.30043858911412,
-4.63736481368175));
#149478=CARTESIAN_POINT('Ctrl Pts',(-5.82065751952999,1.29405949377568,
-4.6632680349132));
#149479=CARTESIAN_POINT('Ctrl Pts',(-5.85335828919288,1.28783500490905,
-4.68915735945583));
#149480=CARTESIAN_POINT('',(-5.31208014948166,1.19797317561536,-5.11447015178951));
#149481=CARTESIAN_POINT('Ctrl Pts',(-5.6544984,1.327885473,-4.537526622));
#149482=CARTESIAN_POINT('Ctrl Pts',(-5.87223422700001,1.27059961,-4.266192261));
#149483=CARTESIAN_POINT('Ctrl Pts',(-6.062989186,1.214285714,-3.975256234));
#149484=CARTESIAN_POINT('Ctrl Pts',(-6.090574979,1.20614195,-3.93318288));
#149485=CARTESIAN_POINT('Ctrl Pts',(-6.117574218,1.197973174,-3.89073074));
#149486=CARTESIAN_POINT('Ctrl Pts',(-5.692393115,1.327885473,-4.883304274));
#149487=CARTESIAN_POINT('Ctrl Pts',(-5.926721282,1.27059961,-4.610151513));
#149488=CARTESIAN_POINT('Ctrl Pts',(-6.133818231,1.214285714,-4.315816714));
#149489=CARTESIAN_POINT('Ctrl Pts',(-6.163767301,1.20614195,-4.27325185));
#149490=CARTESIAN_POINT('Ctrl Pts',(-6.193122768,1.197973174,-4.23027545));
#149491=CARTESIAN_POINT('',(-6.19312276474044,1.19797317358555,-4.23027545534309));
#149492=CARTESIAN_POINT('Ctrl Pts',(-5.85335829882788,1.28783500243923,
-4.68915734706597));
#149493=CARTESIAN_POINT('Ctrl Pts',(-5.95096782342481,1.26310656739011,
-4.56731380918563));
#149494=CARTESIAN_POINT('Ctrl Pts',(-6.04452084762123,1.23856749886486,
-4.44272986964504));
#149495=CARTESIAN_POINT('Ctrl Pts',(-6.13381823140048,1.21428571428671,
-4.31581671345517));
#149496=CARTESIAN_POINT('Ctrl Pts',(-6.15376867898799,1.20886077964635,
-4.28746230749643));
#149497=CARTESIAN_POINT('Ctrl Pts',(-6.17353809688187,1.20342302038954,
-4.25894740590532));
#149498=CARTESIAN_POINT('Ctrl Pts',(-6.19312276398085,1.1979731744789,-4.23027545560123));
#149499=CARTESIAN_POINT('',(-6.15534849076645,1.19797317334244,-4.06050309838586));
#149500=CARTESIAN_POINT('Origin',(-4.3454823073219E-13,1.28891221000039,
-3.61689844741164E-13));
#149501=CARTESIAN_POINT('',(-5.85676706859327,1.10830076259405,-4.68489909144703));
#149502=CARTESIAN_POINT('Origin',(0.158866080899274,0.946580167380763,0.0940856020174308));
#149503=CARTESIAN_POINT('Origin',(0.165366462737506,1.33917528531327,0.0856520574936748));
#149504=CARTESIAN_POINT('Ctrl Pts',(-6.10315794204819,1.19354381548963,
-3.91339811126932));
#149505=CARTESIAN_POINT('Ctrl Pts',(-6.11036608002404,1.19575849474482,
-3.9020644256347));
#149506=CARTESIAN_POINT('Ctrl Pts',(-6.117574218,1.197973174,-3.89073074));
#149507=CARTESIAN_POINT('Ctrl Pts',(-6.328247018,1.262701774,-3.559480243));
#149508=CARTESIAN_POINT('Ctrl Pts',(-6.501920259,1.327878141,-3.207418423));
#149509=CARTESIAN_POINT('Ctrl Pts',(-6.4436735601197,1.19354381548963,-3.83895661449708));
#149510=CARTESIAN_POINT('Ctrl Pts',(-6.45074144893707,1.19575849474482,
-3.82699259442523));
#149511=CARTESIAN_POINT('Ctrl Pts',(-6.45780933775458,1.197973174,-3.81502857435344));
#149512=CARTESIAN_POINT('Ctrl Pts',(-6.66438306487192,1.262701774,-3.46535524454349));
#149513=CARTESIAN_POINT('Ctrl Pts',(-6.83199193698954,1.327878141,-3.09542091445431));
#149514=CARTESIAN_POINT('',(-6.45711892681566,1.19797317455041,-3.81518219547778));
#149515=CARTESIAN_POINT('',(-6.28734656821292,1.19797317561532,-3.85295647362759));
#149516=CARTESIAN_POINT('',(-6.72454025005821,1.28783500528777,-3.32122845155774));
#149517=CARTESIAN_POINT('Origin',(0.17499692100152,1.33927123071157,0.0772100261152464));
#149518=CARTESIAN_POINT('Ctrl Pts',(-6.49984672608352,1.32710049312117,
-3.21161837007158));
#149519=CARTESIAN_POINT('Ctrl Pts',(-6.53722325789545,1.32022179843905,
-3.22989347770123));
#149520=CARTESIAN_POINT('Ctrl Pts',(-6.57465763980289,1.31351590006666,
-3.24817454885908));
#149521=CARTESIAN_POINT('Ctrl Pts',(-6.64954327505303,1.30043858901477,
-3.28470412634283));
#149522=CARTESIAN_POINT('Ctrl Pts',(-6.68703856467982,1.29405949354876,
-3.30297411135391));
#149523=CARTESIAN_POINT('Ctrl Pts',(-6.72454024663977,1.2878350049003,-3.32122845844845));
#149524=CARTESIAN_POINT('Origin',(1.40729441988618E-12,1.28891221000011,
6.29704621779581E-13));
#149525=CARTESIAN_POINT('',(-6.95771517296809,1.19797317358553,-2.80003563894104));
#149526=CARTESIAN_POINT('Ctrl Pts',(-6.72454025316532,1.28783500479118,
-3.32122844495214));
#149527=CARTESIAN_POINT('Ctrl Pts',(-6.79367496246426,1.26310656823154,
-3.18125037862002));
#149528=CARTESIAN_POINT('Ctrl Pts',(-6.85825890481461,1.2385674989258,-3.03946800716173));
#149529=CARTESIAN_POINT('Ctrl Pts',(-6.91818598841636,1.21428571428671,
-2.896325711946));
#149530=CARTESIAN_POINT('Ctrl Pts',(-6.93157464648079,1.20886077964635,
-2.86434545977925));
#149531=CARTESIAN_POINT('Ctrl Pts',(-6.94475200541248,1.20342302038954,
-2.83224738030942));
#149532=CARTESIAN_POINT('Ctrl Pts',(-6.9577151722647,1.19797317447889,-2.80003563935131));
#149533=CARTESIAN_POINT('',(-6.72695392951754,1.10830076261231,-3.31633695910702));
#149534=CARTESIAN_POINT('Origin',(0.175377431229771,0.946580208288621,0.0577343816384296));
#149535=CARTESIAN_POINT('Origin',(0.179912927810285,1.33917528002472,0.0481006479961876));
#149536=CARTESIAN_POINT('Ctrl Pts',(-6.497733465,1.327885473,-3.215891761));
#149537=CARTESIAN_POINT('Ctrl Pts',(-6.652049883,1.27059961,-2.90409428));
#149538=CARTESIAN_POINT('Ctrl Pts',(-6.775802451,1.214285714,-2.578953498));
#149539=CARTESIAN_POINT('Ctrl Pts',(-6.793698776,1.20614195,-2.531933665));
#149540=CARTESIAN_POINT('Ctrl Pts',(-6.810940832,1.197973174,-2.484669994));
#149541=CARTESIAN_POINT('Ctrl Pts',(-6.609074196,1.327885473,-3.54543908));
#149542=CARTESIAN_POINT('Ctrl Pts',(-6.779204132,1.27059961,-3.22829885));
#149543=CARTESIAN_POINT('Ctrl Pts',(-6.918185988,1.214285714,-2.896325712));
#149544=CARTESIAN_POINT('Ctrl Pts',(-6.938284678,1.20614195,-2.848317827));
#149545=CARTESIAN_POINT('Ctrl Pts',(-6.957715175,1.197973174,-2.800035633));
#149546=CARTESIAN_POINT('',(-6.88432800204646,1.19797317334241,-2.64235281728703));
#149547=CARTESIAN_POINT('Ctrl Pts',(-6.80173441512177,1.19354381538544,
-2.50990648843726));
#149548=CARTESIAN_POINT('Ctrl Pts',(-6.80633762356097,1.19575849469273,
-2.49728824121862));
#149549=CARTESIAN_POINT('Ctrl Pts',(-6.81094083199999,1.197973174,-2.484669994));
#149550=CARTESIAN_POINT('Ctrl Pts',(-6.945479154,1.262701774,-2.115875526));
#149551=CARTESIAN_POINT('Ctrl Pts',(-7.039409127,1.327878141,-1.734710103));
#149552=CARTESIAN_POINT('Ctrl Pts',(-7.11828624563922,1.19354381538545,
-2.36400460114487));
#149553=CARTESIAN_POINT('Ctrl Pts',(-7.12261698060608,1.19575849469273,
-2.35080090573385));
#149554=CARTESIAN_POINT('Ctrl Pts',(-7.12694771557288,1.197973174,-2.33759721032276));
#149555=CARTESIAN_POINT('Ctrl Pts',(-7.25352243474422,1.262701774,-1.9516918036216));
#149556=CARTESIAN_POINT('Ctrl Pts',(-7.33768775821218,1.327878141,-1.55437537983679));
#149557=CARTESIAN_POINT('',(-7.12630647006304,1.19797317455045,-2.33789565779545));
#149558=CARTESIAN_POINT('',(-7.2812901780632,1.287835005315,-1.79800259824859));
#149559=CARTESIAN_POINT('Origin',(0.187503276413901,1.33927124186361,0.0377856823255016));
#149560=CARTESIAN_POINT('Ctrl Pts',(-7.03828693514388,1.32710049342982,
-1.73925760526499));
#149561=CARTESIAN_POINT('Ctrl Pts',(-7.07871823223496,1.32022179874537,
-1.74907060143247));
#149562=CARTESIAN_POINT('Ctrl Pts',(-7.11920731040392,1.31351590012465,
-1.75887698603503));
#149563=CARTESIAN_POINT('Ctrl Pts',(-7.20019494033615,1.30043858906984,
-1.77845432421383));
#149564=CARTESIAN_POINT('Ctrl Pts',(-7.24074111772171,1.29405949358374,
-1.78823678820374));
#149565=CARTESIAN_POINT('Ctrl Pts',(-7.28129017620987,1.28783500493425,
-1.79800260570121));
#149566=CARTESIAN_POINT('',(-6.96862364819113,1.19797317561536,-2.41128283256266));
#149567=CARTESIAN_POINT('Origin',(-1.96891114523368E-13,1.28891221000006,
3.64291929955129E-14));
#149568=CARTESIAN_POINT('',(-7.28259590084126,1.10830076259393,-1.79270659643711));
#149569=CARTESIAN_POINT('Origin',(0.183688148092492,0.946580188782692,0.0186835548852868));
#149570=CARTESIAN_POINT('',(-7.39697255240153,1.19797317358549,-1.23886926827323));
#149571=CARTESIAN_POINT('Origin',(0.186046560972666,1.33917528776439,0.00830004920121169));
#149572=CARTESIAN_POINT('Ctrl Pts',(-7.28129017978068,1.28783500479116,
-1.79800259116314));
#149573=CARTESIAN_POINT('Ctrl Pts',(-7.31871741147635,1.26310656824645,
-1.64643521526425));
#149574=CARTESIAN_POINT('Ctrl Pts',(-7.35131239835908,1.23856749894059,
-1.49408399825204));
#149575=CARTESIAN_POINT('Ctrl Pts',(-7.37906705786735,1.21428571428673,
-1.34140573858062));
#149576=CARTESIAN_POINT('Ctrl Pts',(-7.38526788766403,1.20886077964635,
-1.30729500118915));
#149577=CARTESIAN_POINT('Ctrl Pts',(-7.39123702897003,1.20342302038953,
-1.2731146144405));
#149578=CARTESIAN_POINT('Ctrl Pts',(-7.39697255197882,1.19797317447889,
-1.23886926883833));
#149579=CARTESIAN_POINT('Ctrl Pts',(-7.037141735,1.327885473,-1.743885375));
#149580=CARTESIAN_POINT('Ctrl Pts',(-7.120823079,1.27059961,-1.406204078));
#149581=CARTESIAN_POINT('Ctrl Pts',(-7.171786724,1.214285714,-1.062061763));
#149582=CARTESIAN_POINT('Ctrl Pts',(-7.179156768,1.20614195,-1.012294047));
#149583=CARTESIAN_POINT('Ctrl Pts',(-7.185835423,1.197973174,-0.962428842));
#149584=CARTESIAN_POINT('Ctrl Pts',(-7.216722314,1.327885473,-2.041793095));
#149585=CARTESIAN_POINT('Ctrl Pts',(-7.314698931,1.27059961,-1.69549452));
#149586=CARTESIAN_POINT('Ctrl Pts',(-7.379067058,1.214285714,-1.341405739));
#149587=CARTESIAN_POINT('Ctrl Pts',(-7.38837557500001,1.20614195,-1.290199627));
#149588=CARTESIAN_POINT('Ctrl Pts',(-7.396972553,1.197973174,-1.238869262));
#149589=CARTESIAN_POINT('',(-7.29140398739447,1.19797317334234,-1.10064905601137));
#149590=CARTESIAN_POINT('Ctrl Pts',(-7.18226934733144,1.19354381530488,
-0.989054429223104));
#149591=CARTESIAN_POINT('Ctrl Pts',(-7.18405238516571,1.19575849465245,
-0.97574163561155));
#149592=CARTESIAN_POINT('Ctrl Pts',(-7.185835423,1.197973174,-0.962428841999999));
#149593=CARTESIAN_POINT('Ctrl Pts',(-7.23794840400001,1.262701774,-0.573334821));
#149594=CARTESIAN_POINT('Ctrl Pts',(-7.247743048,1.327878141,-0.180888666));
#149595=CARTESIAN_POINT('Ctrl Pts',(-7.46005577827158,1.19354381530488,
-0.778514360307321));
#149596=CARTESIAN_POINT('Ctrl Pts',(-7.46144685888638,1.19575849465245,
-0.764688379697061));
#149597=CARTESIAN_POINT('Ctrl Pts',(-7.46283793950117,1.197973174,-0.750862399086782));
#149598=CARTESIAN_POINT('Ctrl Pts',(-7.50349515734272,1.262701774,-0.346769423045057));
#149599=CARTESIAN_POINT('Ctrl Pts',(-7.50028145566704,1.327878141,0.0593510209700458));
#149600=CARTESIAN_POINT('',(-7.46227584405872,1.19797317455226,-0.751291715791706));
#149601=CARTESIAN_POINT('',(-7.49757506980534,1.28783500459391,-0.19070414176217));
#149602=CARTESIAN_POINT('Origin',(0.191242272114438,1.33927122495846,-0.00340538665022094));
#149603=CARTESIAN_POINT('Ctrl Pts',(-7.24762467125097,1.32710049336744,
-0.185571088325219));
#149604=CARTESIAN_POINT('Ctrl Pts',(-7.28922021123486,1.32022179866829,
-0.186463128251078));
#149605=CARTESIAN_POINT('Ctrl Pts',(-7.33087075978761,1.31351590009004,
-0.187336290002792));
#149606=CARTESIAN_POINT('Ctrl Pts',(-7.414173492925,1.30043858903658,-0.189045974345836));
#149607=CARTESIAN_POINT('Ctrl Pts',(-7.45587466365107,1.2940594935756,-0.189883500134146));
#149608=CARTESIAN_POINT('Ctrl Pts',(-7.4975750697091,1.28783500493827,-0.190704149264586));
#149609=CARTESIAN_POINT('',(-7.32405563182418,1.19797317561536,-0.856860287050402));
#149610=CARTESIAN_POINT('Origin',(-1.21127066710081E-12,1.28891221000044,
-1.97595845935483E-14));
#149611=CARTESIAN_POINT('',(-7.49771178195635,1.10830076263343,-0.185251266036125));
#149612=CARTESIAN_POINT('Origin',(0.183410112802487,0.946580183562984,-0.0212407687145654));
#149613=CARTESIAN_POINT('',(-7.49035571664319,1.19797317379343,0.380225251774696));
#149614=CARTESIAN_POINT('Origin',(0.183481502120748,1.33917532238901,-0.0318885222450997));
#149615=CARTESIAN_POINT('Ctrl Pts',(-7.49757506964849,1.28783500267511,
-0.190704134563331));
#149616=CARTESIAN_POINT('Ctrl Pts',(-7.50154476801412,1.26310656754432,
-0.0346345710151447));
#149617=CARTESIAN_POINT('Ctrl Pts',(-7.50062669414218,1.23856749894096,
0.121161718051112));
#149618=CARTESIAN_POINT('Ctrl Pts',(-7.49491115271031,1.21428571404002,
0.276236876004533));
#149619=CARTESIAN_POINT('Ctrl Pts',(-7.49363421046727,1.20886077969537,
0.310883118078491));
#149620=CARTESIAN_POINT('Ctrl Pts',(-7.49211602372626,1.20342302059146,
0.345547575253918));
#149621=CARTESIAN_POINT('Ctrl Pts',(-7.49035571612108,1.19797317510268,
0.380225251182368));
#149622=CARTESIAN_POINT('Ctrl Pts',(-7.247501079,1.327885473,-0.190336848));
#149623=CARTESIAN_POINT('Ctrl Pts',(-7.256634502,1.27059961,0.157438664));
#149624=CARTESIAN_POINT('Ctrl Pts',(-7.23242622,1.214285714,0.5044908));
#149625=CARTESIAN_POINT('Ctrl Pts',(-7.22892537,1.20614195,0.554679316));
#149626=CARTESIAN_POINT('Ctrl Pts',(-7.224728336,1.197973174,0.604814414));
#149627=CARTESIAN_POINT('Ctrl Pts',(-7.486924517,1.327885473,-0.442675134));
#149628=CARTESIAN_POINT('Ctrl Pts',(-7.50816653800001,1.27059961,-0.0834107510000001));
#149629=CARTESIAN_POINT('Ctrl Pts',(-7.494911153,1.214285714,0.276236876));
#149630=CARTESIAN_POINT('Ctrl Pts',(-7.492994242,1.20614195,0.328246873));
#149631=CARTESIAN_POINT('Ctrl Pts',(-7.490355716,1.197973174,0.380225258));
#149632=CARTESIAN_POINT('',(-7.35754202627095,1.19797317334235,0.492519831952287));
#149633=CARTESIAN_POINT('Ctrl Pts',(-7.22696934725185,1.19354381553843,
0.578044718798007));
#149634=CARTESIAN_POINT('Ctrl Pts',(-7.22584884162587,1.19575849476922,
0.59142956639901));
#149635=CARTESIAN_POINT('Ctrl Pts',(-7.224728336,1.197973174,0.604814414));
#149636=CARTESIAN_POINT('Ctrl Pts',(-7.191979232,1.262701774,0.996014383));
#149637=CARTESIAN_POINT('Ctrl Pts',(-7.117180559,1.327878141,1.381390924));
#149638=CARTESIAN_POINT('Ctrl Pts',(-7.45300139473422,1.19354381553843,
0.843378349190491));
#149639=CARTESIAN_POINT('Ctrl Pts',(-7.45138777556092,1.19575849476922,
0.857180126555084));
#149640=CARTESIAN_POINT('Ctrl Pts',(-7.44977415638769,1.197973174,0.870981903919677));
#149641=CARTESIAN_POINT('Ctrl Pts',(-7.40261278486015,1.262701774,1.27436751114721));
#149642=CARTESIAN_POINT('Ctrl Pts',(-7.31217032832715,1.327878141,1.67030223292065));
#149643=CARTESIAN_POINT('',(-7.44931749258291,1.19797317455044,0.870441788346016));
#149644=CARTESIAN_POINT('',(-7.36328168430241,1.28783500460275,1.42551142857604));
#149645=CARTESIAN_POINT('Origin',(0.18603945373218,1.33927128329711,-0.0444372817464886));
#149646=CARTESIAN_POINT('Ctrl Pts',(-7.11807153346965,1.32710049315711,
1.37679252683296));
#149647=CARTESIAN_POINT('Ctrl Pts',(-7.1588863551378,1.32022179848698,1.38486315380969));
#149648=CARTESIAN_POINT('Ctrl Pts',(-7.19975083979558,1.31351590012017,
1.39296404265902));
#149649=CARTESIAN_POINT('Ctrl Pts',(-7.28147353295054,1.30043858906693,
1.40920195516011));
#149650=CARTESIAN_POINT('Ctrl Pts',(-7.32237979679447,1.29405949359075,
1.41734852940739));
#149651=CARTESIAN_POINT('Ctrl Pts',(-7.36328168579721,1.2878350049424,1.42551142134503));
#149652=CARTESIAN_POINT('',(-7.33702291451221,1.19797317561536,0.737628093931804));
#149653=CARTESIAN_POINT('Origin',(-1.02912470212324E-12,1.28891221000017,
3.18809648819363E-13));
#149654=CARTESIAN_POINT('',(-7.36224299305575,1.10830076258289,1.43086620813176));
#149655=CARTESIAN_POINT('Origin',(0.1745561198956,0.946580177742715,-0.0601719581631782));
#149656=CARTESIAN_POINT('',(-7.23349817293615,1.19797317379341,1.98154086307437));
#149657=CARTESIAN_POINT('Origin',(0.172336708625885,1.33917532517151,-0.070586075733608));
#149658=CARTESIAN_POINT('Ctrl Pts',(-7.36328168274246,1.28783500269651,
1.42551143549193));
#149659=CARTESIAN_POINT('Ctrl Pts',(-7.33360822908143,1.26310656754608,
1.57878554712408));
#149660=CARTESIAN_POINT('Ctrl Pts',(-7.29922002229186,1.23856749893657,
1.73074204666147));
#149661=CARTESIAN_POINT('Ctrl Pts',(-7.2603015315847,1.21428571404458,1.88096296098956));
#149662=CARTESIAN_POINT('Ctrl Pts',(-7.25160652535969,1.20886077970096,
1.91452468837021));
#149663=CARTESIAN_POINT('Ctrl Pts',(-7.24267199974596,1.20342302059146,
1.94805234476405));
#149664=CARTESIAN_POINT('Ctrl Pts',(-7.23349817258391,1.19797317510269,
1.98154086236766));
#149665=CARTESIAN_POINT('Ctrl Pts',(-7.118975327,1.327885473,1.372111619));
#149666=CARTESIAN_POINT('Ctrl Pts',(-7.053133761,1.27059961,1.713719749));
#149667=CARTESIAN_POINT('Ctrl Pts',(-6.954885505,1.214285714,2.047453934));
#149668=CARTESIAN_POINT('Ctrl Pts',(-6.940677455,1.20614195,2.095716491));
#149669=CARTESIAN_POINT('Ctrl Pts',(-6.925800981,1.197973174,2.14377722));
#149670=CARTESIAN_POINT('Ctrl Pts',(-7.407046451,1.327885473,1.177141824));
#149671=CARTESIAN_POINT('Ctrl Pts',(-7.35056062300001,1.27059961,1.532573212));
#149672=CARTESIAN_POINT('Ctrl Pts',(-7.260301532,1.214285714,1.880962961));
#149673=CARTESIAN_POINT('Ctrl Pts',(-7.247248825,1.20614195,1.931344914));
#149674=CARTESIAN_POINT('Ctrl Pts',(-7.233498171,1.197973174,1.981540869));
#149675=CARTESIAN_POINT('',(-7.0796495771348,1.19797317334232,2.06265904060503));
#149676=CARTESIAN_POINT('Ctrl Pts',(-6.93374429210158,1.19354381539086,
2.11811513570332));
#149677=CARTESIAN_POINT('Ctrl Pts',(-6.92977263655074,1.19575849469544,
2.13094617785169));
#149678=CARTESIAN_POINT('Ctrl Pts',(-6.925800981,1.197973174,2.14377722));
#149679=CARTESIAN_POINT('Ctrl Pts',(-6.809721103,1.262701774,2.518791062));
#149680=CARTESIAN_POINT('Ctrl Pts',(-6.653826618,1.327878141,2.87907821));
#149681=CARTESIAN_POINT('Ctrl Pts',(-7.09745294900091,1.19354381539086,
2.42583562210593));
#149682=CARTESIAN_POINT('Ctrl Pts',(-7.09291008107509,1.19575849469544,
2.43896784156803));
#149683=CARTESIAN_POINT('Ctrl Pts',(-7.0883672131494,1.197973174,2.45210006103019));
#149684=CARTESIAN_POINT('Ctrl Pts',(-6.95559246774463,1.262701774,2.83591643522334));
#149685=CARTESIAN_POINT('Ctrl Pts',(-6.78215024268148,1.327878141,3.20315196996456));
#149686=CARTESIAN_POINT('',(-7.08803733486135,1.19797317454272,2.45147440199206));
#149687=CARTESIAN_POINT('',(-6.88468943126012,1.28783500530378,2.9750716687908));
#149688=CARTESIAN_POINT('Origin',(0.172137015649187,1.33927119313551,-0.0833912361227418));
#149689=CARTESIAN_POINT('Ctrl Pts',(-6.65568528020384,1.32710049335983,
2.87477885322754));
#149690=CARTESIAN_POINT('Ctrl Pts',(-6.69381092757056,1.3202217986674,2.89143477361773));
#149691=CARTESIAN_POINT('Ctrl Pts',(-6.73197857279038,1.3135159000738,2.90813092494699));
#149692=CARTESIAN_POINT('Ctrl Pts',(-6.80829996347872,1.3004385890334,2.9415571672601));
#149693=CARTESIAN_POINT('Ctrl Pts',(-6.84649858912149,1.29405949354624,
2.95830691665649));
#149694=CARTESIAN_POINT('Ctrl Pts',(-6.8846894342928,1.28783500491216,2.97507166173683));
#149695=CARTESIAN_POINT('',(-7.00691915965291,1.19797317561536,2.29762580488479));
#149696=CARTESIAN_POINT('Origin',(-1.52525561625261E-12,1.28891220999967,
5.94576471391051E-13));
#149697=CARTESIAN_POINT('',(-6.8825239041631,1.10830076262221,2.98007796857407));
#149698=CARTESIAN_POINT('Origin',(0.157539934978953,0.946580157411726,-0.0962895971539018));
#149699=CARTESIAN_POINT('',(-6.63841029328656,1.19797317358555,3.49020182563242));
#149700=CARTESIAN_POINT('Origin',(0.153133620362348,1.33917525765928,-0.105983085559498));
#149701=CARTESIAN_POINT('Ctrl Pts',(-6.88468942840868,1.28783500479116,
2.97507167549922));
#149702=CARTESIAN_POINT('Ctrl Pts',(-6.82276032021009,1.26310656824261,
3.11838340813306));
#149703=CARTESIAN_POINT('Ctrl Pts',(-6.75650993499366,1.23856749893679,
3.25939480124276));
#149704=CARTESIAN_POINT('Ctrl Pts',(-6.68620828108259,1.21428571428671,
3.39773730914892));
#149705=CARTESIAN_POINT('Ctrl Pts',(-6.67050177997188,1.20886077964635,
3.42864521292078));
#149706=CARTESIAN_POINT('Ctrl Pts',(-6.65456868331845,1.20342302038954,
3.45946835206213));
#149707=CARTESIAN_POINT('Ctrl Pts',(-6.63841029324666,1.19797317447889,
3.49020182489734));
#149708=CARTESIAN_POINT('Ctrl Pts',(-6.657574201,1.327885473,2.870401672));
#149709=CARTESIAN_POINT('Ctrl Pts',(-6.51983632400001,1.27059961,3.189869203));
#149710=CARTESIAN_POINT('Ctrl Pts',(-6.352142073,1.214285714,3.494680397));
#149711=CARTESIAN_POINT('Ctrl Pts',(-6.327891176,1.20614195,3.538760292));
#149712=CARTESIAN_POINT('Ctrl Pts',(-6.30303087,1.197973174,3.582499385));
#149713=CARTESIAN_POINT('Ctrl Pts',(-6.980823125,1.327885473,2.741916938));
#149714=CARTESIAN_POINT('Ctrl Pts',(-6.849250662,1.27059961,3.076895755));
#149715=CARTESIAN_POINT('Ctrl Pts',(-6.686208281,1.214285714,3.397737309));
#149716=CARTESIAN_POINT('Ctrl Pts',(-6.662630109,1.20614195,3.444135414));
#149717=CARTESIAN_POINT('Ctrl Pts',(-6.63841029,1.197973174,3.490201831));
#149718=CARTESIAN_POINT('',(-6.46904368484552,1.19797317334243,3.53681209221154));
#149719=CARTESIAN_POINT('Ctrl Pts',(-6.31630506021735,1.19354381545683,
3.55914484335768));
#149720=CARTESIAN_POINT('Ctrl Pts',(-6.30966796510867,1.19575849472843,
3.57082211417883));
#149721=CARTESIAN_POINT('Ctrl Pts',(-6.30303087,1.197973174,3.582499385));
#149722=CARTESIAN_POINT('Ctrl Pts',(-6.109047985,1.262701774,3.92379187));
#149723=CARTESIAN_POINT('Ctrl Pts',(-5.879347139,1.327878141,4.242142999));
#149724=CARTESIAN_POINT('Ctrl Pts',(-6.41003549123835,1.19354381545683,
3.8948635183192));
#149725=CARTESIAN_POINT('Ctrl Pts',(-6.4027757941272,1.19575849472843,3.90671213131973));
#149726=CARTESIAN_POINT('Ctrl Pts',(-6.39551609701611,1.197973174,3.91856074432019));
#149727=CARTESIAN_POINT('Ctrl Pts',(-6.1833363758006,1.262701774,4.26486106026454));
#149728=CARTESIAN_POINT('Ctrl Pts',(-5.93500435021084,1.327878141,4.5862258796775));
#149729=CARTESIAN_POINT('',(-6.3953284293054,1.19797317454266,3.91787879879043));
#149730=CARTESIAN_POINT('',(-6.0841767517999,1.28783500457832,4.38552086391292));
#149731=CARTESIAN_POINT('Origin',(0.150185964198979,1.33927126630319,-0.118446022870446));
#149732=CARTESIAN_POINT('Ctrl Pts',(-5.88208658127338,1.32710049336774,
4.23834371602909));
#149733=CARTESIAN_POINT('Ctrl Pts',(-5.91574034173286,1.32022179868773,
4.26280611729209));
#149734=CARTESIAN_POINT('Ctrl Pts',(-5.94942646977985,1.31351590006783,
4.28731683742319));
#149735=CARTESIAN_POINT('Ctrl Pts',(-6.0167778546574,1.30043858903083,4.33636843565603));
#149736=CARTESIAN_POINT('Ctrl Pts',(-6.05048271649278,1.29405949355569,
4.36093816053791));
#149737=CARTESIAN_POINT('Ctrl Pts',(-6.08417675618337,1.28783500491729,
4.38552085799059));
#149738=CARTESIAN_POINT('',(-6.34917965264557,1.19797317561517,3.7501890862884));
#149739=CARTESIAN_POINT('Origin',(-3.20056481317721E-13,1.28891220999967,
3.15719672627779E-13));
#149740=CARTESIAN_POINT('',(-6.08098564727152,1.10830076263549,4.38994459505371));
#149741=CARTESIAN_POINT('Origin',(0.133157366289638,0.946580186166513,-0.127904849618447));
#149742=CARTESIAN_POINT('',(-5.73291772724531,1.19797317379345,4.83566482943543));
#149743=CARTESIAN_POINT('Origin',(0.126770238043511,1.33917530768453,-0.136424485866898));
#149744=CARTESIAN_POINT('Ctrl Pts',(-6.08417674749869,1.2878350026744,4.38552086952979));
#149745=CARTESIAN_POINT('Ctrl Pts',(-5.99288772115719,1.26310656752983,
4.51216912600509));
#149746=CARTESIAN_POINT('Ctrl Pts',(-5.89787295184485,1.23856749892762,
4.63564187660495));
#149747=CARTESIAN_POINT('Ctrl Pts',(-5.79947536162801,1.21428571401319,
4.75563723596286));
#149748=CARTESIAN_POINT('Ctrl Pts',(-5.77749178415566,1.20886077966251,
4.78244609664098));
#149749=CARTESIAN_POINT('Ctrl Pts',(-5.7553051308146,1.20342302059143,4.80912346338656));
#149750=CARTESIAN_POINT('Ctrl Pts',(-5.73291772722294,1.1979731751026,4.8356648286461));
#149751=CARTESIAN_POINT('Ctrl Pts',(-5.884872305,1.327885473,4.234474933));
#149752=CARTESIAN_POINT('Ctrl Pts',(-5.681678587,1.27059961,4.516863918));
#149753=CARTESIAN_POINT('Ctrl Pts',(-5.452379538,1.214285714,4.77849949));
#149754=CARTESIAN_POINT('Ctrl Pts',(-5.419219739,1.20614195,4.81633559500001));
#149755=CARTESIAN_POINT('Ctrl Pts',(-5.385538041,1.197973174,4.853707861));
#149756=CARTESIAN_POINT('Ctrl Pts',(-6.228184269,1.327885473,4.178483064));
#149757=CARTESIAN_POINT('Ctrl Pts',(-6.027677353,1.27059961,4.477346072));
#149758=CARTESIAN_POINT('Ctrl Pts',(-5.799475362,1.214285714,4.755637236));
#149759=CARTESIAN_POINT('Ctrl Pts',(-5.766474213,1.20614195,4.795881969));
#149760=CARTESIAN_POINT('Ctrl Pts',(-5.73291772300001,1.197973174,4.835664834));
#149761=CARTESIAN_POINT('',(-5.55922788466497,1.19797317334242,4.84468634444197));
#149762=CARTESIAN_POINT('Ctrl Pts',(-5.4035224239318,1.19354381550955,4.8337528943271));
#149763=CARTESIAN_POINT('Ctrl Pts',(-5.39453023246583,1.19575849475478,
4.84373037766356));
#149764=CARTESIAN_POINT('Ctrl Pts',(-5.385538041,1.197973174,4.853707861));
#149765=CARTESIAN_POINT('Ctrl Pts',(-5.122722572,1.262701774,5.145320531));
#149766=CARTESIAN_POINT('Ctrl Pts',(-4.829955922,1.327878141,5.406849895));
#149767=CARTESIAN_POINT('Ctrl Pts',(-5.4228918982709,1.19354381550955,5.18177192569324));
#149768=CARTESIAN_POINT('Ctrl Pts',(-5.41325482741167,1.19575849475478,
5.19178290428964));
#149769=CARTESIAN_POINT('Ctrl Pts',(-5.40361775655257,1.197973174,5.20179388288622));
#149770=CARTESIAN_POINT('Ctrl Pts',(-5.12195434811186,1.262701774,5.49438552141966));
#149771=CARTESIAN_POINT('Ctrl Pts',(-4.81034425078659,1.327878141,5.7548529655605));
#149772=CARTESIAN_POINT('',(-5.40358107453905,1.19797317454273,5.20108753783366));
#149773=CARTESIAN_POINT('',(-4.9991747298791,1.28783500529405,5.59090797826665));
#149774=CARTESIAN_POINT('Origin',(0.121212383058121,1.33927125351804,-0.147962438566965));
#149775=CARTESIAN_POINT('Ctrl Pts',(-4.83344805204249,1.32710049314202,
5.40372833781476));
#149776=CARTESIAN_POINT('Ctrl Pts',(-4.86105631324101,1.32022179845642,
5.43485338557291));
#149777=CARTESIAN_POINT('Ctrl Pts',(-4.88868579701985,1.31351590010628,
5.46603257927555));
#149778=CARTESIAN_POINT('Ctrl Pts',(-4.94391790055482,1.30043858904295,
5.52841593545202));
#149779=CARTESIAN_POINT('Ctrl Pts',(-4.97155299698495,1.29405949356062,
5.55965678285503));
#149780=CARTESIAN_POINT('Ctrl Pts',(-4.99917473559828,1.28783500490659,
5.59090797313452));
#149781=CARTESIAN_POINT('',(-5.39455956189882,1.19797317561536,5.02739769459734));
#149782=CARTESIAN_POINT('Origin',(5.11309744544164E-13,1.28891220999989,
-5.71591385334358E-13));
#149783=CARTESIAN_POINT('',(-4.99510726048495,1.1083007625976,5.59454229148354));
#149784=CARTESIAN_POINT('Origin',(0.10254829428874,0.946580187984479,-0.153539229833606));
#149785=CARTESIAN_POINT('',(-4.55936029919686,1.19797317358555,5.95501752046846));
#149786=CARTESIAN_POINT('Origin',(0.0944792294308422,1.33917530994407,-0.16048687199922));
#149787=CARTESIAN_POINT('Ctrl Pts',(-4.99917472438475,1.28783500479116,
5.59090798306256));
#149788=CARTESIAN_POINT('Ctrl Pts',(-4.88279435342643,1.26310656823528,
5.69497083129256));
#149789=CARTESIAN_POINT('Ctrl Pts',(-4.76345798519044,1.23856749892951,
5.79513149076926));
#149790=CARTESIAN_POINT('Ctrl Pts',(-4.64156542093359,1.21428571428671,
5.89116885203553));
#149791=CARTESIAN_POINT('Ctrl Pts',(-4.61433269467536,1.20886077964635,
5.91262511711513));
#149792=CARTESIAN_POINT('Ctrl Pts',(-4.58692990753181,1.20342302038954,
5.93390930696844));
#149793=CARTESIAN_POINT('Ctrl Pts',(-4.55936029942225,1.19797317447889,
5.95501751970994));
#149794=CARTESIAN_POINT('Ctrl Pts',(-4.83700032,1.327885473,5.400548852));
#149795=CARTESIAN_POINT('Ctrl Pts',(-4.577851874,1.27059961,5.632655097));
#149796=CARTESIAN_POINT('Ctrl Pts',(-4.297669796,1.214285714,5.838881257));
#149797=CARTESIAN_POINT('Ctrl Pts',(-4.25715161,1.20614195,5.868704398));
#149798=CARTESIAN_POINT('Ctrl Pts',(-4.216223439,1.197973174,5.897962352));
#149799=CARTESIAN_POINT('Ctrl Pts',(-5.18432243800001,1.327885473,5.419667966));
#149800=CARTESIAN_POINT('Ctrl Pts',(-4.92425655,1.27059961,5.668440663));
#149801=CARTESIAN_POINT('Ctrl Pts',(-4.641565421,1.214285714,5.891168852));
#149802=CARTESIAN_POINT('Ctrl Pts',(-4.600684393,1.20614195,5.923378414));
#149803=CARTESIAN_POINT('Ctrl Pts',(-4.55936029400001,1.197973174,5.955017524));
#149804=CARTESIAN_POINT('',(-4.38779186976006,1.19797317334242,5.92648993558636));
#149805=CARTESIAN_POINT('Ctrl Pts',(-4.23807708524811,1.19354381545801,
5.88234003187642));
#149806=CARTESIAN_POINT('Ctrl Pts',(-4.2271502621241,1.19575849472901,5.89015119193821));
#149807=CARTESIAN_POINT('Ctrl Pts',(-4.216223439,1.197973174,5.897962352));
#149808=CARTESIAN_POINT('Ctrl Pts',(-3.896864346,1.262701774,6.126259723));
#149809=CARTESIAN_POINT('Ctrl Pts',(-3.554721335,1.327878141,6.3187385));
#149810=CARTESIAN_POINT('Ctrl Pts',(-4.18217990780254,1.193543815458,6.22638643642344));
#149811=CARTESIAN_POINT('Ctrl Pts',(-4.17061608171156,1.19575849472901,
6.23409167861179));
#149812=CARTESIAN_POINT('Ctrl Pts',(-4.15905225562061,1.197973174,6.24179692080016));
#149813=CARTESIAN_POINT('Ctrl Pts',(-3.82107542831418,1.262701774,6.46699862203382));
#149814=CARTESIAN_POINT('Ctrl Pts',(-3.46075780018589,1.327878141,6.65438952165839));
#149815=CARTESIAN_POINT('',(-4.1591682718737,1.19797317455222,6.24109920712169));
#149816=CARTESIAN_POINT('',(-3.68041685394524,1.28783500529536,6.53487044871798));
#149817=CARTESIAN_POINT('Origin',(0.0865708812706306,1.33927122581219,-0.170560125300614));
#149818=CARTESIAN_POINT('Ctrl Pts',(-3.5588028629224,1.32710049336213,6.31644062642552));
#149819=CARTESIAN_POINT('Ctrl Pts',(-3.57907469298459,1.32022179868322,
6.35277294787677));
#149820=CARTESIAN_POINT('Ctrl Pts',(-3.59935561044513,1.31351590010244,
6.38916271284325));
#149821=CARTESIAN_POINT('Ctrl Pts',(-3.63988584051283,1.30043858904339,
6.4619608502902));
#149822=CARTESIAN_POINT('Ctrl Pts',(-3.66015898505743,1.29405949355478,
6.49841203285239));
#149823=CARTESIAN_POINT('Ctrl Pts',(-3.68041686065727,1.28783500490144,
6.53487044492123));
#149824=CARTESIAN_POINT('',(-4.18769586182889,1.19797317561536,6.06953077425346));
#149825=CARTESIAN_POINT('Origin',(-4.98516158908835E-13,1.28891221000006,
6.29270940910587E-13));
#149826=CARTESIAN_POINT('',(-3.67566320884938,1.10830076262376,6.53754540854673));
#149827=CARTESIAN_POINT('Origin',(0.0671445181503139,0.946580160389495,
-0.171994674781133));
#149828=CARTESIAN_POINT('',(-3.17261225178722,1.19797317358555,6.79592021059555));
#149829=CARTESIAN_POINT('Origin',(0.0577704175746957,1.33917529164855,-0.177044994166941));
#149830=CARTESIAN_POINT('Ctrl Pts',(-3.68041684755842,1.28783500479116,
6.53487045228963));
#149831=CARTESIAN_POINT('Ctrl Pts',(-3.54438694874804,1.26310656823919,
6.6114820293681));
#149832=CARTESIAN_POINT('Ctrl Pts',(-3.40630901743123,1.23856749893339,
6.68364719669204));
#149833=CARTESIAN_POINT('Ctrl Pts',(-3.26662103946597,1.21428571428671,
6.75123595977197));
#149834=CARTESIAN_POINT('Ctrl Pts',(-3.23541253640364,1.20886077964635,
6.76633635817622));
#149835=CARTESIAN_POINT('Ctrl Pts',(-3.20407493953323,1.20342302038954,
6.78123214628162));
#149836=CARTESIAN_POINT('Ctrl Pts',(-3.17261225212519,1.19797317447889,
6.7959202097777));
#149837=CARTESIAN_POINT('Ctrl Pts',(-3.562955577,1.327885473,6.31409910900001));
#149838=CARTESIAN_POINT('Ctrl Pts',(-3.259969896,1.27059961,6.485069584));
#149839=CARTESIAN_POINT('Ctrl Pts',(-2.94200579,1.214285714,6.626243425));
#149840=CARTESIAN_POINT('Ctrl Pts',(-2.896023804,1.20614195,6.646659106));
#149841=CARTESIAN_POINT('Ctrl Pts',(-2.849762915,1.197973174,6.666434679));
#149842=CARTESIAN_POINT('Ctrl Pts',(-3.898047452,1.327885473,6.407435217));
#149843=CARTESIAN_POINT('Ctrl Pts',(-3.590582984,1.27059961,6.594485268));
#149844=CARTESIAN_POINT('Ctrl Pts',(-3.26662104,1.214285714,6.75123596));
#149845=CARTESIAN_POINT('Ctrl Pts',(-3.219771683,1.20614195,6.77390426700001));
#149846=CARTESIAN_POINT('Ctrl Pts',(-3.172612246,1.197973174,6.795920213));
#149847=CARTESIAN_POINT('',(-3.01118758420266,1.19797317334243,6.73117744434362));
#149848=CARTESIAN_POINT('Ctrl Pts',(-2.87446397243517,1.19354381542134,
6.65587548794217));
#149849=CARTESIAN_POINT('Ctrl Pts',(-2.86211344371758,1.19575849471068,
6.66115508347108));
#149850=CARTESIAN_POINT('Ctrl Pts',(-2.849762915,1.197973174,6.666434679));
#149851=CARTESIAN_POINT('Ctrl Pts',(-2.488793073,1.262701774,6.82074181900001));
#149852=CARTESIAN_POINT('Ctrl Pts',(-2.113271928,1.327878141,6.935169916));
#149853=CARTESIAN_POINT('Ctrl Pts',(-2.74591383263932,1.19354381542133,
6.97986203707782));
#149854=CARTESIAN_POINT('Ctrl Pts',(-2.73296396296722,1.19575849471068,
6.98490125425597));
#149855=CARTESIAN_POINT('Ctrl Pts',(-2.72001409329518,1.197973174,6.98994047143423));
#149856=CARTESIAN_POINT('Ctrl Pts',(-2.34152726764351,1.262701774,7.13722205509973));
#149857=CARTESIAN_POINT('Ctrl Pts',(-1.94935016118734,1.327878141,7.24277422096479));
#149858=CARTESIAN_POINT('',(-2.72027738496142,1.19797317455223,6.98928400998415));
#149859=CARTESIAN_POINT('',(-2.18956677597955,1.28783500531006,7.17326964054042));
#149860=CARTESIAN_POINT('Origin',(0.0478815178840269,1.33927122556283,-0.185182686033522));
#149861=CARTESIAN_POINT('Ctrl Pts',(-2.11775200747474,1.32710049331763,
6.9338031727206));
#149862=CARTESIAN_POINT('Ctrl Pts',(-2.12973953050717,1.32022179165342,
6.97364394945073));
#149863=CARTESIAN_POINT('Ctrl Pts',(-2.14172358183174,1.31351588565602,
7.01354278723912));
#149864=CARTESIAN_POINT('Ctrl Pts',(-2.16565676360449,1.30043858906236,
7.09335165801813));
#149865=CARTESIAN_POINT('Ctrl Pts',(-2.17762000653844,1.29405949359197,
7.13330875899285));
#149866=CARTESIAN_POINT('Ctrl Pts',(-2.18956678342661,1.28783500492658,
7.1732696382543));
#149867=CARTESIAN_POINT('',(-2.7850201573695,1.19797317561536,6.82785934067827));
#149868=CARTESIAN_POINT('Origin',(-1.96565853871622E-13,1.28891221000028,
6.45317133063372E-13));
#149869=CARTESIAN_POINT('',(-2.18434923164404,1.1083007626404,7.17486016787826));
#149870=CARTESIAN_POINT('Origin',(0.0286009841952251,0.946580155216993,
-0.182407723267577));
#149871=CARTESIAN_POINT('',(-1.63751638118294,1.19797317358554,7.31905322493337));
#149872=CARTESIAN_POINT('Origin',(0.0183603401137666,1.33917530561268,-0.185324740845644));
#149873=CARTESIAN_POINT('Ctrl Pts',(-2.1895667688656,1.28783500479116,7.17326964254652));
#149874=CARTESIAN_POINT('Ctrl Pts',(-2.04024794910754,1.26310656824512,
7.21884767627459));
#149875=CARTESIAN_POINT('Ctrl Pts',(-1.88988482534072,1.23856749893928,
7.25964298840125));
#149876=CARTESIAN_POINT('Ctrl Pts',(-1.73893308847782,1.21428571428671,
7.29562277765216));
#149877=CARTESIAN_POINT('Ctrl Pts',(-1.70520808358027,1.20886077964635,
7.30366123149123));
#149878=CARTESIAN_POINT('Ctrl Pts',(-1.6714009882543,1.20342302038954,7.31147210733639));
#149879=CARTESIAN_POINT('Ctrl Pts',(-1.63751638169677,1.19797317447889,
7.31905322426847));
#149880=CARTESIAN_POINT('Ctrl Pts',(-2.12231099,1.327885473,6.932409109));
#149881=CARTESIAN_POINT('Ctrl Pts',(-1.789655348,1.27059961,7.034249424));
#149882=CARTESIAN_POINT('Ctrl Pts',(-1.448776863,1.214285714,7.103769816));
#149883=CARTESIAN_POINT('Ctrl Pts',(-1.399481142,1.20614195,7.11382342199999));
#149884=CARTESIAN_POINT('Ctrl Pts',(-1.350050644,1.197973174,7.12319192899999));
#149885=CARTESIAN_POINT('Ctrl Pts',(-2.429504099,1.327885473,7.095597919));
#149886=CARTESIAN_POINT('Ctrl Pts',(-2.089017748,1.27059961,7.212179072));
#149887=CARTESIAN_POINT('Ctrl Pts',(-1.738933089,1.214285714,7.295622778));
#149888=CARTESIAN_POINT('Ctrl Pts',(-1.688306028,1.20614195,7.307689886));
#149889=CARTESIAN_POINT('Ctrl Pts',(-1.637516375,1.197973174,7.319053226));
#149890=CARTESIAN_POINT('',(-1.49378351347216,1.19797317334243,7.2211225766783));
#149891=CARTESIAN_POINT('Ctrl Pts',(-1.37644411718142,1.19354381561821,
7.11818960337276));
#149892=CARTESIAN_POINT('Ctrl Pts',(-1.36324738059071,1.19575849480912,
7.12069076618631));
#149893=CARTESIAN_POINT('Ctrl Pts',(-1.350050644,1.197973174,7.12319192900001));
#149894=CARTESIAN_POINT('Ctrl Pts',(-0.964348603,1.262701774,7.196293608));
#149895=CARTESIAN_POINT('Ctrl Pts',(-0.573008275,1.327878141,7.227320494));
#149896=CARTESIAN_POINT('Ctrl Pts',(-1.18125187711363,1.19354381561821,
7.40696704708603));
#149897=CARTESIAN_POINT('Ctrl Pts',(-1.16752148607158,1.19575849480912,
7.40910461085876));
#149898=CARTESIAN_POINT('Ctrl Pts',(-1.15379109502954,1.197973174,7.41124217463135));
#149899=CARTESIAN_POINT('Ctrl Pts',(-0.752491894106228,1.262701774,7.47371691633682));
#149900=CARTESIAN_POINT('Ctrl Pts',(-0.346793074702295,1.327878141,7.49249484662523));
#149901=CARTESIAN_POINT('',(-1.15418935087267,1.19797317455211,7.41065766083517));
#149902=CARTESIAN_POINT('',(-0.596334988833152,1.28783500530699,7.47625471614313));
#149903=CARTESIAN_POINT('Origin',(0.00695329922591664,1.33927121911688,
-0.191146606717507));
#149904=CARTESIAN_POINT('Ctrl Pts',(-0.577677421890293,1.32710049333146,
7.22694878924593));
#149905=CARTESIAN_POINT('Ctrl Pts',(-0.580820090687207,1.32022179867905,
7.26843503156666));
#149906=CARTESIAN_POINT('Ctrl Pts',(-0.583946887107583,1.31351590008168,
7.30997722414324));
#149907=CARTESIAN_POINT('Ctrl Pts',(-0.590163983057832,1.30043858905469,
7.39306522602624));
#149908=CARTESIAN_POINT('Ctrl Pts',(-0.593257936403517,1.29405949356778,
7.43465989577418));
#149909=CARTESIAN_POINT('Ctrl Pts',(-0.596334996445522,1.28783500492151,
7.47625471552231));
#149910=CARTESIAN_POINT('',(-1.25212000546965,1.19797317561497,7.26692479278219));
#149911=CARTESIAN_POINT('Origin',(1.50546553847296E-13,1.28891221000011,
-1.49446427455402E-12));
#149912=CARTESIAN_POINT('',(-0.590897511552974,1.10830076263119,7.47668644041972));
#149913=CARTESIAN_POINT('Origin',(-0.0112799890895166,0.946580205613589,
-0.184291155937752));
#149914=CARTESIAN_POINT('',(-0.0258520642582035,1.19797317358555,7.49995544522267));
#149915=CARTESIAN_POINT('Origin',(-0.0219082601936706,1.33917534714528,
-0.184938943114152));
#149916=CARTESIAN_POINT('Ctrl Pts',(-0.596334981605594,1.28783500479122,
7.47625471674912));
#149917=CARTESIAN_POINT('Ctrl Pts',(-0.440709222886166,1.26310656824116,
7.4886680289595));
#149918=CARTESIAN_POINT('Ctrl Pts',(-0.285091719071053,1.23856749893533,
7.49618594244474));
#149919=CARTESIAN_POINT('Ctrl Pts',(-0.129934559142799,1.21428571428671,
7.49887438288844));
#149920=CARTESIAN_POINT('Ctrl Pts',(-0.0952699962297192,1.20886077964635,
7.49947502299387));
#149921=CARTESIAN_POINT('Ctrl Pts',(-0.0605741846837616,1.20342302038954,
7.49983575874006));
#149922=CARTESIAN_POINT('Ctrl Pts',(-0.0258520649117424,1.19797317447889,
7.49995544458365));
#149923=CARTESIAN_POINT('Ctrl Pts',(-0.582429501,1.327885473,7.226567365));
#149924=CARTESIAN_POINT('Ctrl Pts',(-0.235658505,1.27059961,7.25451558));
#149925=CARTESIAN_POINT('Ctrl Pts',(0.112195259,1.214285714,7.249131826));
#149926=CARTESIAN_POINT('Ctrl Pts',(0.162499702,1.20614195,7.248353261));
#149927=CARTESIAN_POINT('Ctrl Pts',(0.212788494,1.197973174,7.246876641));
#149928=CARTESIAN_POINT('Ctrl Pts',(-0.847359835,1.327885473,7.451978349));
#149929=CARTESIAN_POINT('Ctrl Pts',(-0.489772364,1.27059961,7.492639398));
#149930=CARTESIAN_POINT('Ctrl Pts',(-0.129934559,1.214285714,7.498874383));
#149931=CARTESIAN_POINT('Ctrl Pts',(-0.07789706,1.20614195,7.499776047));
#149932=CARTESIAN_POINT('Ctrl Pts',(-0.025852058,1.197973174,7.499955445));
#149933=CARTESIAN_POINT('',(0.0946614167047613,1.19797317334243,7.37215064903207));
#149934=CARTESIAN_POINT('Ctrl Pts',(-1.64905696123129,4.559162772,7.31700065795431));
#149935=CARTESIAN_POINT('Ctrl Pts',(-1.24995303110202,4.624819703,7.40694804799773));
#149936=CARTESIAN_POINT('Ctrl Pts',(-0.843433619605153,4.690053947,7.45295291918589));
#149937=CARTESIAN_POINT('Ctrl Pts',(-0.829373780711526,4.69231013190792,
7.45454403896745));
#149938=CARTESIAN_POINT('Ctrl Pts',(-0.815313941817894,4.69456631681569,
7.45613515874913));
#149939=CARTESIAN_POINT('Ctrl Pts',(-1.360702703,4.559162772,7.12116480300001));
#149940=CARTESIAN_POINT('Ctrl Pts',(-0.97228059,4.624819703,7.19538398400001));
#149941=CARTESIAN_POINT('Ctrl Pts',(-0.578090317,4.690053947,7.226915773));
#149942=CARTESIAN_POINT('Ctrl Pts',(-0.564456892432628,4.69231013190792,
7.22800632823754));
#149943=CARTESIAN_POINT('Ctrl Pts',(-0.550823467865264,4.69456631681568,
7.2290968834751));
#149944=CARTESIAN_POINT('',(-0.842885263317961,4.69005394784289,7.45248581030807));
#149945=CARTESIAN_POINT('',(-0.710487785962877,4.69005394666591,7.33970078119719));
#149946=CARTESIAN_POINT('',(-1.40337283195863,4.59933049943207,7.36753314834207));
#149947=CARTESIAN_POINT('Origin',(0.0430257849586406,4.5535839336865,-0.186571753848842));
#149948=CARTESIAN_POINT('Ctrl Pts',(-1.35606856849621,4.55994605589074,
7.12204873926192));
#149949=CARTESIAN_POINT('Ctrl Pts',(-1.36398279156896,4.56683176235715,
7.1628961219797));
#149950=CARTESIAN_POINT('Ctrl Pts',(-1.37188477500109,4.57355155126864,
7.2037990962851));
#149951=CARTESIAN_POINT('Ctrl Pts',(-1.3876490014487,4.58666922563405,7.28561428031784));
#149952=CARTESIAN_POINT('Ctrl Pts',(-1.39552006202443,4.59307444478169,
7.32657226946014));
#149953=CARTESIAN_POINT('Ctrl Pts',(-1.40337283024197,4.59933049942395,
7.36753314861101));
#149954=CARTESIAN_POINT('Origin',(1.4658413372004E-13,4.78597145200391,
-9.49761103097301E-14));
#149955=CARTESIAN_POINT('',(-1.58832892089749,4.74999999914956,7.32988480407119));
#149956=CARTESIAN_POINT('',(-1.39282737490266,4.78575691075475,7.33314099135338));
#149957=CARTESIAN_POINT('Origin',(-1.36764295382465,4.80792738371137,-0.48930545689145));
#149958=CARTESIAN_POINT('',(-1.21292875863641,4.75000000020817,7.401270399065));
#149959=CARTESIAN_POINT('Origin',(0.,4.75,0.));
#149960=CARTESIAN_POINT('Origin',(1.42856873648812,5.02638720352195,0.290380960526179));
#149961=CARTESIAN_POINT('Ctrl Pts',(-1.954774922,4.690053947,7.24077723800001));
#149962=CARTESIAN_POINT('Ctrl Pts',(-1.559836226,4.624398499,7.347397871));
#149963=CARTESIAN_POINT('Ctrl Pts',(-1.155643991,4.559170361,7.410430957));
#149964=CARTESIAN_POINT('Ctrl Pts',(-2.118148151,4.690053947,6.933682168));
#149965=CARTESIAN_POINT('Ctrl Pts',(-1.739959553,4.624398499,7.04921378));
#149966=CARTESIAN_POINT('Ctrl Pts',(-1.351448856,4.559170361,7.122926785));
#149967=CARTESIAN_POINT('',(-1.95477491753716,4.69005394803158,7.24077722740733));
#149968=CARTESIAN_POINT('Origin',(0.0511912506964596,4.6964256407958,-0.185659103279333));
#149969=CARTESIAN_POINT('',(-2.03646151908971,4.690053949938,7.08722970800272));
#149970=CARTESIAN_POINT('Origin',(1.11347563114261E-13,4.75000000000022,
-6.74373751285984E-13));
#149971=CARTESIAN_POINT('Origin',(0.0695854055266315,4.55370521606813,-0.174272083749276));
#149972=CARTESIAN_POINT('Origin',(0.0227099788655557,4.69643082077873,-0.19168659541468));
#149973=CARTESIAN_POINT('Ctrl Pts',(-3.18344177802041,4.559162772,6.79143474775637));
#149974=CARTESIAN_POINT('Ctrl Pts',(-2.81300470640529,4.624819703,6.96507476537178));
#149975=CARTESIAN_POINT('Ctrl Pts',(-2.42587918041204,4.690053947,7.09739372561723));
#149976=CARTESIAN_POINT('Ctrl Pts',(-2.41249009668655,4.6923101318704,7.10197009560121));
#149977=CARTESIAN_POINT('Ctrl Pts',(-2.39910101296107,4.69456631674065,
7.10654646558524));
#149978=CARTESIAN_POINT('Ctrl Pts',(-2.859730162,4.559162772,6.662165068));
#149979=CARTESIAN_POINT('Ctrl Pts',(-2.496344072,4.624819703,6.818148319));
#149980=CARTESIAN_POINT('Ctrl Pts',(-2.118148151,4.690053947,6.933682168));
#149981=CARTESIAN_POINT('Ctrl Pts',(-2.1050679056767,4.6923101318704,6.93767800984849));
#149982=CARTESIAN_POINT('Ctrl Pts',(-2.09198766035339,4.69456631674065,
6.94167385169711));
#149983=CARTESIAN_POINT('',(-2.42524322977434,4.69005394784288,7.09705541788261));
#149984=CARTESIAN_POINT('',(-2.2716956840529,4.69005394666591,7.01536878363051));
#149985=CARTESIAN_POINT('',(-2.95436459941101,4.5993304993972,6.89360064207624));
#149986=CARTESIAN_POINT('Origin',(0.082127310480036,4.55358392275416,-0.172960595508864));
#149987=CARTESIAN_POINT('Ctrl Pts',(-2.85539439212089,4.55994605579451,
6.66402454021117));
#149988=CARTESIAN_POINT('Ctrl Pts',(-2.87190456475552,4.56683176223659,
6.7022156097041));
#149989=CARTESIAN_POINT('Ctrl Pts',(-2.88841473474086,4.57355155123228,
6.74046360281252));
#149990=CARTESIAN_POINT('Ctrl Pts',(-2.92139824828119,4.58666922557382,
6.81697715040149));
#149991=CARTESIAN_POINT('Ctrl Pts',(-2.93789004470618,4.59307444471158,
6.85528551903663));
#149992=CARTESIAN_POINT('Ctrl Pts',(-2.95436459776838,4.59933049937157,
6.89360064259002));
#149993=CARTESIAN_POINT('Origin',(-1.83338587367299E-12,4.78597145199609,
4.7045700668491E-12));
#149994=CARTESIAN_POINT('',(-3.12690323603191,4.74999999914954,6.81707240326556));
#149995=CARTESIAN_POINT('',(-2.9366723912812,4.78575691078144,6.86227951640224));
#149996=CARTESIAN_POINT('Origin',(-1.23048235575978,4.80792820156638,-0.771867751245));
#149997=CARTESIAN_POINT('',(-2.77562551529351,4.75000000043579,6.96748898019576));
#149998=CARTESIAN_POINT('Origin',(0.,4.75,0.));
#149999=CARTESIAN_POINT('Origin',(1.33274604232867,5.02638717842108,0.590692412348867));
#150000=CARTESIAN_POINT('Ctrl Pts',(-3.465626441,4.690053947,6.651273064));
#150001=CARTESIAN_POINT('Ctrl Pts',(-3.102841477,4.624398499,6.840301112));
#150002=CARTESIAN_POINT('Ctrl Pts',(-2.721649282,4.559170361,6.988749902));
#150003=CARTESIAN_POINT('Ctrl Pts',(-3.559163733,4.690053947,6.31623729200001));
#150004=CARTESIAN_POINT('Ctrl Pts',(-3.214652856,4.624398499,6.51036720800001));
#150005=CARTESIAN_POINT('Ctrl Pts',(-2.85107144,4.559170361,6.66587516));
#150006=CARTESIAN_POINT('',(-3.4656264343989,4.69005394803158,6.65127305476895));
#150007=CARTESIAN_POINT('Origin',(0.0899055760333051,4.69642563605647,-0.170313721247756));
#150008=CARTESIAN_POINT('',(-3.51239507107219,4.690053949938,6.48375518662845));
#150009=CARTESIAN_POINT('Origin',(-3.12467066110322E-13,4.75000000000067,
8.85142653617166E-13));
#150010=CARTESIAN_POINT('Origin',(0.105421885409696,4.55370520201922,-0.155238891963012));
#150011=CARTESIAN_POINT('Origin',(0.0633858622240569,4.69643084883136,-0.182322700843673));
#150012=CARTESIAN_POINT('Ctrl Pts',(-4.56897239582895,4.559162772,5.94830889694042));
#150013=CARTESIAN_POINT('Ctrl Pts',(-4.24452340807861,4.624819703,6.19752232791606));
#150014=CARTESIAN_POINT('Ctrl Pts',(-3.89489332647558,4.690053947,6.40996828923204));
#150015=CARTESIAN_POINT('Ctrl Pts',(-3.88280105622734,4.69231013189195,
6.41731592352486));
#150016=CARTESIAN_POINT('Ctrl Pts',(-3.87070878597903,4.69456631678401,
6.42466355781763));
#150017=CARTESIAN_POINT('Ctrl Pts',(-4.225039818,4.559162772,5.891649899));
#150018=CARTESIAN_POINT('Ctrl Pts',(-3.903681281,4.624819703,6.122103616));
#150019=CARTESIAN_POINT('Ctrl Pts',(-3.559163733,4.690053947,6.316237292));
#150020=CARTESIAN_POINT('Ctrl Pts',(-3.54724828431613,4.69231013189195,
6.32295157946552));
#150021=CARTESIAN_POINT('Ctrl Pts',(-3.53533283563221,4.69456631678401,
6.32966586693117));
#150022=CARTESIAN_POINT('',(-3.89419951784842,4.69005394784288,6.409774601533));
#150023=CARTESIAN_POINT('',(-3.72668161723396,4.69005394666591,6.36300593903434));
#150024=CARTESIAN_POINT('',(-4.36721356148467,4.59933049939503,6.09733103136705));
#150025=CARTESIAN_POINT('Origin',(0.117388618729205,4.55358391550433,-0.151261904255742));
#150026=CARTESIAN_POINT('Ctrl Pts',(-4.22120514702725,4.55994605599275,
5.89439796090948));
#150027=CARTESIAN_POINT('Ctrl Pts',(-4.24553927227261,4.56683176247112,
5.9281469455694));
#150028=CARTESIAN_POINT('Ctrl Pts',(-4.2698856310428,4.57355155128922,5.96195152251035));
#150029=CARTESIAN_POINT('Ctrl Pts',(-4.3185461596293,4.58666922564275,6.02958574563612));
#150030=CARTESIAN_POINT('Ctrl Pts',(-4.34288755391428,4.59307444476057,
6.06345323712583));
#150031=CARTESIAN_POINT('Ctrl Pts',(-4.36721356001292,4.59933049938345,
6.09733103232237));
#150032=CARTESIAN_POINT('Origin',(6.50174358796107E-12,4.78597145200196,
-8.92428492216268E-12));
#150033=CARTESIAN_POINT('',(-4.51926703050333,4.74999999914954,5.985501274402));
#150034=CARTESIAN_POINT('',(-4.34320187092104,4.78575691083943,6.07054547816828));
#150035=CARTESIAN_POINT('Origin',(-1.03578489673937,4.80792705939401,-1.01834026732815));
#150036=CARTESIAN_POINT('',(-4.20853710611605,4.75000000032413,6.2079155212003));
#150037=CARTESIAN_POINT('Origin',(0.,4.75,0.));
#150038=CARTESIAN_POINT('Origin',(1.17460506913819,5.02638735993946,0.86338410375381));
#150039=CARTESIAN_POINT('Ctrl Pts',(-4.814429119,4.690053947,5.750762755));
#150040=CARTESIAN_POINT('Ctrl Pts',(-4.500761309,4.624398499,6.013359475));
#150041=CARTESIAN_POINT('Ctrl Pts',(-4.160393277,4.559170361,6.240282668));
#150042=CARTESIAN_POINT('Ctrl Pts',(-4.833756773,4.690053947,5.403452179));
#150043=CARTESIAN_POINT('Ctrl Pts',(-4.539032563,4.624398499,5.667103101));
#150044=CARTESIAN_POINT('Ctrl Pts',(-4.217381091,4.559170361,5.89713462));
#150045=CARTESIAN_POINT('',(-4.8144291105,4.69005394803159,5.75076274725657));
#150046=CARTESIAN_POINT('Origin',(0.124415970663431,4.6964256537254,-0.147004747925249));
#150047=CARTESIAN_POINT('',(-4.82409293229943,4.690053949938,5.57710747885074));
#150048=CARTESIAN_POINT('Origin',(7.6739829768524E-13,4.75000000000111,
-9.20270804005696E-13));
#150049=CARTESIAN_POINT('Origin',(0.136328968154141,4.55370504339895,-0.12894688215776));
#150050=CARTESIAN_POINT('Origin',(0.101098175086282,4.69643090266516,-0.164434388615765));
#150051=CARTESIAN_POINT('Ctrl Pts',(-5.74086294261692,4.559162772,4.82704673403553));
#150052=CARTESIAN_POINT('Ctrl Pts',(-5.47757291236792,4.624819703,5.14018063457475));
#150053=CARTESIAN_POINT('Ctrl Pts',(-5.18178659019463,4.690053947,5.42281985940272));
#150054=CARTESIAN_POINT('Ctrl Pts',(-5.17155655501913,4.69231013182244,
5.43259519042792));
#150055=CARTESIAN_POINT('Ctrl Pts',(-5.1613265198436,4.69456631664473,5.44237052145306));
#150056=CARTESIAN_POINT('Ctrl Pts',(-5.392791307,4.559162772,4.845647729));
#150057=CARTESIAN_POINT('Ctrl Pts',(-5.128486691,4.624819703,5.139796152));
#150058=CARTESIAN_POINT('Ctrl Pts',(-4.833756773,4.690053947,5.403452179));
#150059=CARTESIAN_POINT('Ctrl Pts',(-4.82356327451006,4.69231013182244,
5.41257095910662));
#150060=CARTESIAN_POINT('Ctrl Pts',(-4.81336977602019,4.69456631664474,
5.42168973921324));
#150061=CARTESIAN_POINT('',(-5.18106736531322,4.69005394784288,5.42277984836034));
#150062=CARTESIAN_POINT('',(-5.0074120594976,4.69005394666591,5.4131160078898));
#150063=CARTESIAN_POINT('',(-5.57585647103438,4.59933049939397,5.01595699876924));
#150064=CARTESIAN_POINT('Origin',(0.147161107532244,4.55358393747605,-0.122490540720301));
#150065=CARTESIAN_POINT('Ctrl Pts',(-5.38963704103988,4.55994605602018,
4.84915588374512));
#150066=CARTESIAN_POINT('Ctrl Pts',(-5.42065728195095,4.56683176249916,
4.87688471837224));
#150067=CARTESIAN_POINT('Ctrl Pts',(-5.45170142089153,4.57355155126975,
4.90466521549262));
#150068=CARTESIAN_POINT('Ctrl Pts',(-5.51376365214984,4.58666922565576,
4.96025761304181));
#150069=CARTESIAN_POINT('Ctrl Pts',(-5.54481646773506,4.5930744447807,4.98810062122209));
#150070=CARTESIAN_POINT('Ctrl Pts',(-5.57585646980821,4.59933049939462,
5.0159570001354));
#150071=CARTESIAN_POINT('Origin',(6.74980904502576E-12,4.78597145199218,
-6.06632799549089E-12));
#150072=CARTESIAN_POINT('',(-5.70031492331358,4.74999999914956,4.87405475696322));
#150073=CARTESIAN_POINT('',(-5.54664805908661,4.78575691071307,4.99495947977542));
#150074=CARTESIAN_POINT('Origin',(-0.79265687257552,4.80792843462252,-1.21719416012186));
#150075=CARTESIAN_POINT('',(-5.44466217910404,4.75000000024935,5.15806683250066));
#150076=CARTESIAN_POINT('Origin',(0.,4.75,0.));
#150077=CARTESIAN_POINT('Origin',(0.961543110245088,5.02638714566244,1.09570289596845));
#150078=CARTESIAN_POINT('Ctrl Pts',(-5.938114442,4.690053947,4.58135317));
#150079=CARTESIAN_POINT('Ctrl Pts',(-5.688230544,4.624398499,4.905239832));
#150080=CARTESIAN_POINT('Ctrl Pts',(-5.404601906,4.559170361,5.200026753));
#150081=CARTESIAN_POINT('Ctrl Pts',(-5.88232872,4.690053947,4.238007649));
#150082=CARTESIAN_POINT('Ctrl Pts',(-5.651172152,4.624398499,4.55885155200001));
#150083=CARTESIAN_POINT('Ctrl Pts',(-5.38649069,4.559170361,4.85265062));
#150084=CARTESIAN_POINT('',(-5.93811443220641,4.69005394803172,4.58135316459078));
#150085=CARTESIAN_POINT('Origin',(0.153108846385023,4.69642566755726,-0.116822071375633));
#150086=CARTESIAN_POINT('',(-5.9102215701673,4.690053949938,4.40968042401888));
#150087=CARTESIAN_POINT('Origin',(7.66314095512755E-13,4.75000000000111,
-5.6248408708548E-13));
#150088=CARTESIAN_POINT('Origin',(0.1608614299865,4.55370522017207,-0.0966255048229053));
#150089=CARTESIAN_POINT('Origin',(0.134082974767383,4.69643082048456,-0.138856792678627));
#150090=CARTESIAN_POINT('Ctrl Pts',(-6.64431711850405,4.559162772,3.48007722957719));
#150091=CARTESIAN_POINT('Ctrl Pts',(-6.45449719571892,4.624819703,3.84248980807567));
#150092=CARTESIAN_POINT('Ctrl Pts',(-6.22638527105153,4.690053947,4.18210640002668));
#150093=CARTESIAN_POINT('Ctrl Pts',(-6.21849581514646,4.69231013195081,
4.19385234505228));
#150094=CARTESIAN_POINT('Ctrl Pts',(-6.21060635924137,4.69456631690173,
4.20559829007785));
#150095=CARTESIAN_POINT('Ctrl Pts',(-6.308381869,4.559162772,3.573068457));
#150096=CARTESIAN_POINT('Ctrl Pts',(-6.113489763,4.624819703,3.917157533));
#150097=CARTESIAN_POINT('Ctrl Pts',(-5.88232872,4.690053947,4.238007649));
#150098=CARTESIAN_POINT('Ctrl Pts',(-5.87433380759733,4.69231013195081,
4.24910453859052));
#150099=CARTESIAN_POINT('Ctrl Pts',(-5.86633889519477,4.69456631690174,
4.2602014281811));
#150100=CARTESIAN_POINT('',(-6.22567426174319,4.69005394784375,4.18222193495617));
#150101=CARTESIAN_POINT('',(-6.05400147933149,4.69005394666591,4.21011478918028));
#150102=CARTESIAN_POINT('',(-6.52377852944664,4.59933049942132,3.70004239165948));
#150103=CARTESIAN_POINT('Origin',(0.170052081414587,4.55358395657544,-0.0879913042010755));
#150104=CARTESIAN_POINT('Ctrl Pts',(-6.30605549606936,4.559946055829,3.57717266655216));
#150105=CARTESIAN_POINT('Ctrl Pts',(-6.34231138060885,4.56683176227916,
3.59758478132714));
#150106=CARTESIAN_POINT('Ctrl Pts',(-6.37860171146201,4.57355155122711,
3.61804221409297));
#150107=CARTESIAN_POINT('Ctrl Pts',(-6.45116368431535,4.58666922560421,
3.65899334696384));
#150108=CARTESIAN_POINT('Ctrl Pts',(-6.48747592626896,4.59307444477225,
3.67950996376723));
#150109=CARTESIAN_POINT('Ctrl Pts',(-6.52377852856624,4.59933049942196,
3.70004239321589));
#150110=CARTESIAN_POINT('Origin',(-2.42731182376055E-12,4.78597145201565,
1.54542177666084E-12));
#150111=CARTESIAN_POINT('',(-6.61482242500904,4.74999999914956,3.53470285698283));
#150112=CARTESIAN_POINT('',(-6.49073914775451,4.78575691081326,3.6858147281543));
#150113=CARTESIAN_POINT('Origin',(-0.512463312253307,4.80792746182712,-1.35913516485433));
#150114=CARTESIAN_POINT('',(-6.42620090124917,4.75000000041766,3.86703266952255));
#150115=CARTESIAN_POINT('Origin',(0.,4.75,0.));
#150116=CARTESIAN_POINT('Origin',(0.703517659165372,5.02638719619019,1.27678982373001));
#150117=CARTESIAN_POINT('Ctrl Pts',(-6.784140134,4.690053947,3.197724603));
#150118=CARTESIAN_POINT('Ctrl Pts',(-6.609724441,4.624398499,3.567756627));
#150119=CARTESIAN_POINT('Ctrl Pts',(-6.396097357,4.559170361,3.916623367));
#150120=CARTESIAN_POINT('Ctrl Pts',(-6.655849513,4.690053947,2.874398591));
#150121=CARTESIAN_POINT('Ctrl Pts',(-6.499069213,4.624398499,3.237433171));
#150122=CARTESIAN_POINT('Ctrl Pts',(-6.303733971,4.559170361,3.581262071));
#150123=CARTESIAN_POINT('',(-6.78414012329034,4.69005394803158,3.19772459975686));
#150124=CARTESIAN_POINT('Origin',(0.174642508548841,4.69642565886706,-0.0811769417586056));
#150125=CARTESIAN_POINT('',(-6.71999481604169,4.690053949938,3.03606161350816));
#150126=CARTESIAN_POINT('Origin',(-1.83880688453542E-13,4.75,9.34582272682505E-14));
#150127=CARTESIAN_POINT('Origin',(0.177872206404633,4.55370521646147,-0.0597860011261758));
#150128=CARTESIAN_POINT('Origin',(0.160798419335299,4.69643083574111,-0.106786606827317));
#150129=CARTESIAN_POINT('Ctrl Pts',(-7.23709041014682,4.559162772,1.97038318208332));
#150130=CARTESIAN_POINT('Ctrl Pts',(-7.12961636368533,4.624819703,2.36512842789401));
#150131=CARTESIAN_POINT('Ctrl Pts',(-6.9798450978861,4.690053947,2.74584229452194));
#150132=CARTESIAN_POINT('Ctrl Pts',(-6.97466512414919,4.69231013191546,
2.7590096255176));
#150133=CARTESIAN_POINT('Ctrl Pts',(-6.96948515041213,4.69456631683104,
2.77217695651325));
#150134=CARTESIAN_POINT('Ctrl Pts',(-6.928999505,4.559162772,2.133416475));
#150135=CARTESIAN_POINT('Ctrl Pts',(-6.81263284900001,4.624819703,2.511356981));
#150136=CARTESIAN_POINT('Ctrl Pts',(-6.655849513,4.690053947,2.874398591));
#150137=CARTESIAN_POINT('Ctrl Pts',(-6.65042702051765,4.69231013191547,
2.88695471112877));
#150138=CARTESIAN_POINT('Ctrl Pts',(-6.64500452803529,4.69456631683105,
2.89951083125753));
#150139=CARTESIAN_POINT('',(-6.97917554816538,4.69005394784373,2.74610797431514));
#150140=CARTESIAN_POINT('',(-6.81751251872002,4.69005394666591,2.81025328239219));
#150141=CARTESIAN_POINT('',(-7.16665595452082,4.59933049939104,2.21111791413529));
#150142=CARTESIAN_POINT('Origin',(0.184991967529409,4.55358391946441,-0.0493779535858213));
#150143=CARTESIAN_POINT('Ctrl Pts',(-6.92760980580543,4.55994605578795,
2.13792483126066));
#150144=CARTESIAN_POINT('Ctrl Pts',(-6.96740604917396,4.56683176223428,
2.15006577864964));
#150145=CARTESIAN_POINT('Ctrl Pts',(-7.00724567573898,4.57355155121141,
2.16224357964001));
#150146=CARTESIAN_POINT('Ctrl Pts',(-7.08691447293298,4.58666922557449,
2.18663861849105));
#150147=CARTESIAN_POINT('Ctrl Pts',(-7.12678822097081,4.59307444474121,
2.19886950955597));
#150148=CARTESIAN_POINT('Ctrl Pts',(-7.16665595398282,4.5993304993895,2.21111791583575));
#150149=CARTESIAN_POINT('Origin',(-8.44376651931711E-12,4.78597145200978,
2.51209643364891E-12));
#150150=CARTESIAN_POINT('',(-7.2200281815243,4.74999999914955,2.03007218087754));
#150151=CARTESIAN_POINT('',(-7.13133048793648,4.78575691086606,2.20432537650669));
#150152=CARTESIAN_POINT('Origin',(-0.208307341171341,4.80792652016166,-1.43752411711541));
#150153=CARTESIAN_POINT('',(-7.10725761039956,4.75000000036324,2.39518035872432));
#150154=CARTESIAN_POINT('Origin',(0.,4.75,0.));
#150155=CARTESIAN_POINT('Origin',(0.412597202993568,5.02638727525261,1.39817477437911));
#150156=CARTESIAN_POINT('Ctrl Pts',(-7.31294697400001,4.690053947,1.664573988));
#150157=CARTESIAN_POINT('Ctrl Pts',(-7.222154969,4.624398499,2.063449087));
#150158=CARTESIAN_POINT('Ctrl Pts',(-7.088518405,4.559170361,2.450083024));
#150159=CARTESIAN_POINT('Ctrl Pts',(-7.118150181,4.690053947,1.376385849));
#150160=CARTESIAN_POINT('Ctrl Pts',(-7.04307702,4.624398499,1.764636013));
#150161=CARTESIAN_POINT('Ctrl Pts',(-6.926221658,4.559170361,2.142417687));
#150162=CARTESIAN_POINT('',(-7.31294696254952,4.69005394803158,1.66457398698021));
#150163=CARTESIAN_POINT('Origin',(0.188010372622518,4.69642563634723,-0.0417361779614356));
#150164=CARTESIAN_POINT('',(-7.21554857376483,4.690053949938,1.52047993622552));
#150165=CARTESIAN_POINT('Origin',(-1.26721549920106E-12,4.749999999998,
4.4202922572234E-13));
#150166=CARTESIAN_POINT('Origin',(0.186565874649461,4.55370510921501,-0.0201509532732519));
#150167=CARTESIAN_POINT('Origin',(0.179994575064681,4.6964308930497,-0.0697229056221557));
#150168=CARTESIAN_POINT('Ctrl Pts',(-7.49146539826354,4.559162772,0.368556206873501));
#150169=CARTESIAN_POINT('Ctrl Pts',(-7.47136259381077,4.624819703,0.777176271114208));
#150170=CARTESIAN_POINT('Ctrl Pts',(-7.40693512428512,4.690053947,1.18118565370734));
#150171=CARTESIAN_POINT('Ctrl Pts',(-7.40470684240947,4.69231013189519,
1.19515868091854));
#150172=CARTESIAN_POINT('Ctrl Pts',(-7.40247856053368,4.69456631679024,
1.20913170812974));
#150173=CARTESIAN_POINT('Ctrl Pts',(-7.225624826,4.559162772,0.594008309));
#150174=CARTESIAN_POINT('Ctrl Pts',(-7.193224795,4.624819703,0.988128168));
#150175=CARTESIAN_POINT('Ctrl Pts',(-7.118150181,4.690053947,1.376385849));
#150176=CARTESIAN_POINT('Ctrl Pts',(-7.11555365807383,4.69231013189516,
1.38981408946994));
#150177=CARTESIAN_POINT('Ctrl Pts',(-7.11295713514763,4.69456631679043,
1.40324232993988));
#150178=CARTESIAN_POINT('',(-7.40633834158946,4.69005394784375,1.18158905541658));
#150179=CARTESIAN_POINT('',(-7.26224424964502,4.69005394666591,1.27898745451562));
#150180=CARTESIAN_POINT('',(-7.4744285120745,4.59933049941584,0.618804020612643));
#150181=CARTESIAN_POINT('Origin',(0.191281838050076,4.5535839226781,-0.00845573802668184));
#150182=CARTESIAN_POINT('Ctrl Pts',(-7.22523678067821,4.55994605584178,
0.598710006831215));
#150183=CARTESIAN_POINT('Ctrl Pts',(-7.26671255482508,4.56683176228833,
0.602012089829403));
#150184=CARTESIAN_POINT('Ctrl Pts',(-7.3082386201527,4.57355155124429,0.605340838621054));
#150185=CARTESIAN_POINT('Ctrl Pts',(-7.39128901723494,4.5866692255987,0.612039098694847));
#150186=CARTESIAN_POINT('Ctrl Pts',(-7.4328598190213,4.59307444474485,0.615412361133979));
#150187=CARTESIAN_POINT('Ctrl Pts',(-7.47442851183252,4.5993304994014,0.618804022328887));
#150188=CARTESIAN_POINT('Origin',(1.75944328550948E-12,4.78597145199609,
-4.27175655959289E-14));
#150189=CARTESIAN_POINT('',(-7.48763344518716,4.74999999914954,0.430517586105534));
#150190=CARTESIAN_POINT('',(-7.43846874086193,4.78575691070391,0.619764219138516));
#150191=CARTESIAN_POINT('Origin',(0.105587353985421,4.80792502932653,-1.44869507804596));
#150192=CARTESIAN_POINT('',(-7.45598685320312,4.75000000025783,0.81133207620068));
#150193=CARTESIAN_POINT('Origin',(0.,4.75,0.));
#150194=CARTESIAN_POINT('Origin',(0.102386161494812,5.02638459270935,1.45418205555291));
#150195=CARTESIAN_POINT('Ctrl Pts',(-7.49980854,4.690053947,0.053589743));
#150196=CARTESIAN_POINT('Ctrl Pts',(-7.496885558,4.624398499,0.462656961));
#150197=CARTESIAN_POINT('Ctrl Pts',(-7.44948821,4.559170361,0.868979523));
#150198=CARTESIAN_POINT('Ctrl Pts',(-7.247614057,4.690053947,-0.185985165));
#150199=CARTESIAN_POINT('Ctrl Pts',(-7.257758374,4.624398499,0.209326436));
#150200=CARTESIAN_POINT('Ctrl Pts',(-7.224846918,4.559170361,0.603396233));
#150201=CARTESIAN_POINT('',(-7.49980852884078,4.69005394803158,0.0535897445321675));
#150202=CARTESIAN_POINT('Origin',(0.192586677601929,4.6964256536905,-0.000343718717236777));
#150203=CARTESIAN_POINT('',(-7.37371129866262,4.690053949938,-0.0661976928859446));
#150204=CARTESIAN_POINT('Origin',(8.89045781438114E-13,4.75000000000067,
-3.97631146759059E-14));
#150205=CARTESIAN_POINT('Origin',(0.186535920086122,4.55370495027973,0.0204263384372728));
#150206=CARTESIAN_POINT('Origin',(0.190775278630512,4.69643086004083,-0.0293994050625012));
#150207=CARTESIAN_POINT('Ctrl Pts',(-7.39554779059847,4.559162772,-1.25050404738331));
#150208=CARTESIAN_POINT('Ctrl Pts',(-7.46375621384794,4.624819703,-0.847115783895782));
#150209=CARTESIAN_POINT('Ctrl Pts',(-7.48768509773944,4.690053947,-0.438701914462572));
#150210=CARTESIAN_POINT('Ctrl Pts',(-7.48851269966669,4.692310131881,-0.424576554208365));
#150211=CARTESIAN_POINT('Ctrl Pts',(-7.48934030159381,4.69456631676211,
-0.410451193954152));
#150212=CARTESIAN_POINT('Ctrl Pts',(-7.184387961,4.559162772,-0.973175025));
#150213=CARTESIAN_POINT('Ctrl Pts',(-7.237469544,4.624819703,-0.581304421));
#150214=CARTESIAN_POINT('Ctrl Pts',(-7.247614057,4.690053947,-0.185985165));
#150215=CARTESIAN_POINT('Ctrl Pts',(-7.24796491408752,4.692310131881,-0.172312693704705));
#150216=CARTESIAN_POINT('Ctrl Pts',(-7.24831577117507,4.6945663167621,-0.158640222409418));
#150217=CARTESIAN_POINT('',(-7.4871889869311,4.69005394784374,-0.438179653401754));
#150218=CARTESIAN_POINT('',(-7.36740151108662,4.69005394666591,-0.312082404455189));
#150219=CARTESIAN_POINT('',(-7.43270509999558,4.59933049944584,-1.00244446088511));
#150220=CARTESIAN_POINT('Origin',(0.188627548303029,4.55358393625757,0.0328618978331841));
#150221=CARTESIAN_POINT('Ctrl Pts',(-7.18501971321785,4.55994605574127,
-0.96849983165087));
#150222=CARTESIAN_POINT('Ctrl Pts',(-7.22623565686466,4.56683176218549,
-0.974191014923011));
#150223=CARTESIAN_POINT('Ctrl Pts',(-7.26750644887087,4.57355155122374,
-0.979866967011814));
#150224=CARTESIAN_POINT('Ctrl Pts',(-7.35005510186625,4.58666922560854,
-0.991178688909446));
#150225=CARTESIAN_POINT('Ctrl Pts',(-7.39137915337171,4.5930744447878,-0.996820785018313));
#150226=CARTESIAN_POINT('Ctrl Pts',(-7.43270510023496,4.59933049944648,
-1.00244445912524));
#150227=CARTESIAN_POINT('Origin',(-1.53384249745869E-11,4.78597145198239,
-2.16975959768662E-12));
#150228=CARTESIAN_POINT('',(-7.40512529081742,4.74999999776862,-1.18916754046224));
#150229=CARTESIAN_POINT('',(-7.39779246229846,4.78575691078591,-0.993776423367131));
#150230=CARTESIAN_POINT('Origin',(0.414536447211268,4.80792594780388,-1.39212700636851));
#150231=CARTESIAN_POINT('',(-7.45608243946475,4.74999999872292,-0.810453186416921));
#150232=CARTESIAN_POINT('Origin',(0.,4.74999999751669,0.));
#150233=CARTESIAN_POINT('Origin',(-0.212620297068353,5.02638752233421,1.44219252886256));
#150234=CARTESIAN_POINT('Ctrl Pts',(-7.335987395,4.690053947,-1.559900299));
#150235=CARTESIAN_POINT('Ctrl Pts',(-7.42107011,4.624398499,-1.15976849));
#150236=CARTESIAN_POINT('Ctrl Pts',(-7.462128226,4.559170361,-0.752756495));
#150237=CARTESIAN_POINT('Ctrl Pts',(-7.038187555,4.690053947,-1.73965972));
#150238=CARTESIAN_POINT('Ctrl Pts',(-7.133075012,4.624398499,-1.355771012));
#150239=CARTESIAN_POINT('Ctrl Pts',(-7.185646366,4.559170361,-0.963839358));
#150240=CARTESIAN_POINT('',(-7.33598738428273,4.69005394803158,-1.55990029511267));
#150241=CARTESIAN_POINT('Origin',(0.188158183055879,4.69642564641174,0.0410647845106853));
#150242=CARTESIAN_POINT('',(-7.18708747905281,4.690053949938,-1.6497799918444));
#150243=CARTESIAN_POINT('Origin',(1.421172207694E-12,4.75090401630852,1.44659674863878E-13));
#150244=CARTESIAN_POINT('Origin',(0.17778370261965,4.55370429861311,0.0600485860377439));
#150245=CARTESIAN_POINT('Origin',(0.192635712568098,4.69643090866594,0.0122990365265791));
#150246=CARTESIAN_POINT('Ctrl Pts',(-6.95382258707868,4.559162772,-2.81109212170412));
#150247=CARTESIAN_POINT('Ctrl Pts',(-7.10715288829031,4.624819703,-2.43179764594953));
#150248=CARTESIAN_POINT('Ctrl Pts',(-7.21831923758139,4.690053947,-2.03807626903604));
#150249=CARTESIAN_POINT('Ctrl Pts',(-7.22216402555688,4.69231013188439,
-2.02445906180291));
#150250=CARTESIAN_POINT('Ctrl Pts',(-7.2260088135324,4.69456631676863,-2.01084185456972));
#150251=CARTESIAN_POINT('Ctrl Pts',(-6.807217099,4.559162772,-2.494853776));
#150252=CARTESIAN_POINT('Ctrl Pts',(-6.94329826,4.624819703,-2.12355586));
#150253=CARTESIAN_POINT('Ctrl Pts',(-7.038187555,4.690053947,-1.73965972));
#150254=CARTESIAN_POINT('Ctrl Pts',(-7.04146938644222,4.69231013188436,
-1.72638232740484));
#150255=CARTESIAN_POINT('Ctrl Pts',(-7.04475121788429,4.69456631676882,
-1.71310493480973));
#150256=CARTESIAN_POINT('',(-7.21794699633072,4.69005394784288,-2.03745956668756));
#150257=CARTESIAN_POINT('',(-7.12806726602417,4.69005394666591,-1.88855963752162));
#150258=CARTESIAN_POINT('',(-7.04343665786128,4.59933049941141,-2.57681975364456));
#150259=CARTESIAN_POINT('Origin',(0.177153211421694,4.55358396568391,0.072642954591845));
#150260=CARTESIAN_POINT('Ctrl Pts',(-6.80883911044133,4.55994605585476,
-2.49042369485092));
#150261=CARTESIAN_POINT('Ctrl Pts',(-6.84786801208649,4.56683176231117,
-2.50484203097927));
#150262=CARTESIAN_POINT('Ctrl Pts',(-6.88695375350926,4.57355155126602,
-2.51925728258282));
#150263=CARTESIAN_POINT('Ctrl Pts',(-6.9651407789688,4.5866692256309,-2.5480500628686));
#150264=CARTESIAN_POINT('Ctrl Pts',(-7.00428581311489,4.59307444478289,
-2.5624436993453));
#150265=CARTESIAN_POINT('Ctrl Pts',(-7.04343665848406,4.59933049941205,
-2.57681975194824));
#150266=CARTESIAN_POINT('Origin',(-6.99180296992452E-12,4.78597145200196,
-2.51990268929081E-12));
#150267=CARTESIAN_POINT('',(-6.97636170828729,4.74999999998991,-2.75324850177502));
#150268=CARTESIAN_POINT('',(-7.01120363040642,4.78575691087914,-2.56084918463864));
#150269=CARTESIAN_POINT('Origin',(0.704118751076819,4.80792822099414,-1.27046583472849));
#150270=CARTESIAN_POINT('',(-7.10753989332788,4.75000000059599,-2.39434257212809));
#150271=CARTESIAN_POINT('Origin',(0.,4.750000000594,0.));
#150272=CARTESIAN_POINT('Origin',(-0.517673241365713,5.02638728507947,1.3627706118265));
#150273=CARTESIAN_POINT('Ctrl Pts',(-6.829143632,4.690053947,-3.100451136));
#150274=CARTESIAN_POINT('Ctrl Pts',(-6.998253672,4.624398499,-2.727964456));
#150275=CARTESIAN_POINT('Ctrl Pts',(-7.125847419,4.559170361,-2.339294456));
#150276=CARTESIAN_POINT('Ctrl Pts',(-6.499663225,4.690053947,-3.211989719));
#150277=CARTESIAN_POINT('Ctrl Pts',(-6.674856991,4.624398499,-2.857474115));
#150278=CARTESIAN_POINT('Ctrl Pts',(-6.810452976,4.559170361,-2.486006892));
#150279=CARTESIAN_POINT('',(-6.82914362262778,4.69005394803157,-3.10045112994256));
#150280=CARTESIAN_POINT('Origin',(0.174931139540757,4.69642566604463,0.0805530469035581));
#150281=CARTESIAN_POINT('',(-6.66440343625348,4.690053949938,-3.15622041112841));
#150282=CARTESIAN_POINT('Origin',(-4.90926743701436E-13,4.74999999999889,
-1.89735380184963E-13));
#150283=CARTESIAN_POINT('Origin',(0.160718645717512,4.55370518580565,0.0968628134508132));
#150284=CARTESIAN_POINT('Origin',(0.185486980252586,4.69643091730784,0.0534221683155373));
#150285=CARTESIAN_POINT('Ctrl Pts',(-6.18694436873807,4.559162772,-4.24023665220644));
#150286=CARTESIAN_POINT('Ctrl Pts',(-6.41822699308657,4.624819703,-3.90277135391354));
#150287=CARTESIAN_POINT('Ctrl Pts',(-6.61143279189146,4.690053947,-3.54215244295726));
#150288=CARTESIAN_POINT('Ctrl Pts',(-6.61811498807727,4.6923101319548,-3.52968011383345));
#150289=CARTESIAN_POINT('Ctrl Pts',(-6.62479718426306,4.69456631690948,
-3.51720778470964));
#150290=CARTESIAN_POINT('Ctrl Pts',(-6.111748332,4.559162772,-3.899875938));
#150291=CARTESIAN_POINT('Ctrl Pts',(-6.324466068,4.624819703,-3.566512188));
#150292=CARTESIAN_POINT('Ctrl Pts',(-6.499663225,4.690053947,-3.211989719));
#150293=CARTESIAN_POINT('Ctrl Pts',(-6.50572257612459,4.6923101319548,-3.19972824080011));
#150294=CARTESIAN_POINT('Ctrl Pts',(-6.51178192724931,4.69456631690947,
-3.1874667626003));
#150295=CARTESIAN_POINT('',(-6.61120182620016,4.69005394784288,-3.54147013788702));
#150296=CARTESIAN_POINT('',(-6.55543251743721,4.69005394666591,-3.37672992068055));
#150297=CARTESIAN_POINT('',(-6.324824946348,4.59933049939799,-4.03070581890792));
#150298=CARTESIAN_POINT('Origin',(0.15739515689109,4.55358394795306,0.109027173086295));
#150299=CARTESIAN_POINT('Ctrl Pts',(-6.11428475835871,4.5599460559347,-3.89589811327206));
#150300=CARTESIAN_POINT('Ctrl Pts',(-6.14930167003365,4.56683176238811,
-3.91836941721311));
#150301=CARTESIAN_POINT('Ctrl Pts',(-6.18437475511205,4.57355155124519,
-3.94084992717363));
#150302=CARTESIAN_POINT('Ctrl Pts',(-6.25454421474505,4.58666922561086,
-3.98577744783568));
#150303=CARTESIAN_POINT('Ctrl Pts',(-6.28967985332806,4.59307444476164,
-4.00824959438245));
#150304=CARTESIAN_POINT('Ctrl Pts',(-6.32482494730784,4.5993304993985,-4.0307058174037));
#150305=CARTESIAN_POINT('Origin',(6.25367813089639E-12,4.78597145201565,
3.54599162533109E-12));
#150306=CARTESIAN_POINT('',(-6.22139120646213,4.74999999914955,-4.18859062908611));
#150307=CARTESIAN_POINT('',(-6.29677870893683,4.7857569106907,-4.00817948537505));
#150308=CARTESIAN_POINT('Origin',(0.960770280213318,4.80792507653282,-1.08939736573568));
#150309=CARTESIAN_POINT('',(-6.42665668426536,4.75000000025304,-3.86627515258916));
#150310=CARTESIAN_POINT('Origin',(0.,4.75,0.));
#150311=CARTESIAN_POINT('Origin',(-0.79852459252602,5.02638720279362,1.21962634968895));
#150312=CARTESIAN_POINT('Ctrl Pts',(-6.002976704,4.690053947,-4.496028325));
#150313=CARTESIAN_POINT('Ctrl Pts',(-6.24820667,4.624398499,-4.168603835));
#150314=CARTESIAN_POINT('Ctrl Pts',(-6.456369908,4.559170361,-3.816449609));
#150315=CARTESIAN_POINT('Ctrl Pts',(-5.657221867,4.690053947,-4.534130649));
#150316=CARTESIAN_POINT('Ctrl Pts',(-5.904530075,4.624398499,-4.225564904));
#150317=CARTESIAN_POINT('Ctrl Pts',(-6.116810374,4.559170361,-3.891931506));
#150318=CARTESIAN_POINT('',(-6.00297669575905,4.69005394803158,-4.496028316913));
#150319=CARTESIAN_POINT('Origin',(0.153525257493488,4.69642563941649,0.11627507186809));
#150320=CARTESIAN_POINT('',(-5.83009929659162,4.690053949938,-4.51507947267794));
#150321=CARTESIAN_POINT('Origin',(-5.55111512312578E-14,4.75,5.42101086242752E-15));
#150322=CARTESIAN_POINT('Origin',(0.136138464028436,4.55370498751413,0.129147991651934));
#150323=CARTESIAN_POINT('Origin',(0.169666505435107,4.69643086886799,0.0920475538402357));
#150324=CARTESIAN_POINT('Ctrl Pts',(-5.13077150802372,4.559162772,-5.47111243083583));
#150325=CARTESIAN_POINT('Ctrl Pts',(-5.42919193654034,4.624819703,-5.19125581034408));
#150326=CARTESIAN_POINT('Ctrl Pts',(-5.69540309763819,4.690053947,-4.88060150445534));
#150327=CARTESIAN_POINT('Ctrl Pts',(-5.70461024965117,4.69231013189656,
-4.86985724637842));
#150328=CARTESIAN_POINT('Ctrl Pts',(-5.71381740166407,4.69456631679295,
-4.85911298830139));
#150329=CARTESIAN_POINT('Ctrl Pts',(-5.130501005,4.559162772,-5.122544235));
#150330=CARTESIAN_POINT('Ctrl Pts',(-5.40990887,4.624819703,-4.842702369));
#150331=CARTESIAN_POINT('Ctrl Pts',(-5.657221867,4.690053947,-4.534130649));
#150332=CARTESIAN_POINT('Ctrl Pts',(-5.66577540904071,4.69231013189655,
-4.52345841902579));
#150333=CARTESIAN_POINT('Ctrl Pts',(-5.67432895108152,4.69456631679296,
-4.51278618905156));
#150334=CARTESIAN_POINT('',(-5.6953242072177,4.69005394784288,-4.87988550052245));
#150335=CARTESIAN_POINT('',(-5.67627303080642,4.69005394666591,-4.70700806542456));
#150336=CARTESIAN_POINT('',(-5.3104714497277,4.5993304994063,-5.29612055988535));
#150337=CARTESIAN_POINT('Origin',(0.130277873032469,4.55358394138756,0.140313616842009));
#150338=CARTESIAN_POINT('Ctrl Pts',(-5.13383324548519,4.55994605585018,
-5.11920466612713));
#150339=CARTESIAN_POINT('Ctrl Pts',(-5.16320081518432,4.56683176231821,
-5.14867820437159));
#150340=CARTESIAN_POINT('Ctrl Pts',(-5.19262126617189,4.57355155123034,
-5.17817280927312));
#150341=CARTESIAN_POINT('Ctrl Pts',(-5.25149211409,4.58666922560857,-5.23713430919394));
#150342=CARTESIAN_POINT('Ctrl Pts',(-5.28097545383409,4.59307444476671,
-5.26663419322239));
#150343=CARTESIAN_POINT('Ctrl Pts',(-5.31047145099105,4.59933049940695,
-5.29612055862145));
#150344=CARTESIAN_POINT('Origin',(6.03206720684035E-12,4.78597145201174,
5.96918348083619E-12));
#150345=CARTESIAN_POINT('',(-5.17551536425395,4.74999999914956,-5.42807891551251));
#150346=CARTESIAN_POINT('',(-5.2879234136685,4.78575691078485,-5.26809176705119));
#150347=CARTESIAN_POINT('Origin',(1.17249541205182,4.80792850072533,-0.857391987530597));
#150348=CARTESIAN_POINT('',(-5.4452701498066,4.75000000047412,-5.15742500529851));
#150349=CARTESIAN_POINT('Origin',(0.,4.75,0.));
#150350=CARTESIAN_POINT('Origin',(-1.04203959986824,5.02638720628501,1.01945233902109));
#150351=CARTESIAN_POINT('Ctrl Pts',(-4.896117256,4.690053947,-5.681376225));
#150352=CARTESIAN_POINT('Ctrl Pts',(-5.206000469,4.624398499,-5.414323933));
#150353=CARTESIAN_POINT('Ctrl Pts',(-5.484999715,4.559170361,-5.115151819));
#150354=CARTESIAN_POINT('Ctrl Pts',(-4.550255102,4.690053947,-5.644260669));
#150355=CARTESIAN_POINT('Ctrl Pts',(-4.858113896,4.624398499,-5.396072974));
#150356=CARTESIAN_POINT('Ctrl Pts',(-5.13715251700001,4.559170361,-5.115873729));
#150357=CARTESIAN_POINT('',(-4.89611725000693,4.69005394803158,-5.68137621554656));
#150358=CARTESIAN_POINT('Origin',(0.124939912224816,4.69642566560811,0.14655971460778));
#150359=CARTESIAN_POINT('',(-4.72318619291109,4.690053949938,-5.66281843539718));
#150360=CARTESIAN_POINT('Origin',(-1.17354043149831E-12,4.74999999999845,
-1.13190706807487E-12));
#150361=CARTESIAN_POINT('Origin',(0.105192656758101,4.5537052143291,0.155394314114667));
#150362=CARTESIAN_POINT('Origin',(0.145911959404404,4.696430882499,0.126368526012341));
#150363=CARTESIAN_POINT('Ctrl Pts',(-3.83468947316923,4.559162772,-6.44616507155078));
#150364=CARTESIAN_POINT('Ctrl Pts',(-4.18629389862629,4.624819703,-6.23700291528905));
#150365=CARTESIAN_POINT('Ctrl Pts',(-4.51306268384797,4.690053947,-5.99083906471441));
#150366=CARTESIAN_POINT('Ctrl Pts',(-4.52436427590561,4.69231013194548,
-5.98232526674977));
#150367=CARTESIAN_POINT('Ctrl Pts',(-4.53566586796319,4.69456631689107,
-5.97381146878521));
#150368=CARTESIAN_POINT('Ctrl Pts',(-3.909357153,4.559162772,-6.105688057));
#150369=CARTESIAN_POINT('Ctrl Pts',(-4.242390347,4.624819703,-5.89245317));
#150370=CARTESIAN_POINT('Ctrl Pts',(-4.550255102,4.690053947,-5.644260669));
#150371=CARTESIAN_POINT('Ctrl Pts',(-4.56090288118604,4.69231013194548,
-5.63567670833756));
#150372=CARTESIAN_POINT('Ctrl Pts',(-4.57155066037219,4.69456631689108,
-5.62709274767499));
#150373=CARTESIAN_POINT('',(-4.5131395575211,4.69005394784288,-5.99012284143654));
#150374=CARTESIAN_POINT('',(-4.53169732561459,4.69005394666591,-5.8171917447422));
#150375=CARTESIAN_POINT('',(-4.04780620967149,4.5993304994234,-6.31389458947704));
#150376=CARTESIAN_POINT('Origin',(0.0970686768313267,4.55358391569743,0.165038936601301));
#150377=CARTESIAN_POINT('Ctrl Pts',(-3.91332939641532,4.55994605596869,
-6.10314289974883));
#150378=CARTESIAN_POINT('Ctrl Pts',(-3.93567442920366,4.5668317624299,-6.13824052216406));
#150379=CARTESIAN_POINT('Ctrl Pts',(-3.95806657822901,4.57355155134733,
-6.17337008676992));
#150380=CARTESIAN_POINT('Ctrl Pts',(-4.00288607861997,4.58666922566913,
-6.24360859117123));
#150381=CARTESIAN_POINT('Ctrl Pts',(-4.02533851102381,4.59307444478845,
-6.27875683055447));
#150382=CARTESIAN_POINT('Ctrl Pts',(-4.04780621107526,4.59933049940983,
-6.31389458846582));
#150383=CARTESIAN_POINT('Origin',(-6.75284481110872E-12,4.78597145199413,
-1.08307460222612E-11));
#150384=CARTESIAN_POINT('',(-3.88763817760581,4.74999999914954,-6.41375626277432));
#150385=CARTESIAN_POINT('',(-4.03181069685682,4.78575691085142,-6.2816739328473));
#150386=CARTESIAN_POINT('Origin',(1.32939753871551,4.80792768536083,-0.585294039397131));
#150387=CARTESIAN_POINT('',(-4.20926883649175,4.75000000037377,-6.20741939563398));
#150388=CARTESIAN_POINT('Origin',(0.,4.75,0.));
#150389=CARTESIAN_POINT('Origin',(-1.23682972024279,5.02638723642215,0.771609693634924));
#150390=CARTESIAN_POINT('Ctrl Pts',(-3.560320807,4.690053947,-6.601069288));
#150391=CARTESIAN_POINT('Ctrl Pts',(-3.920367472,4.624398499,-6.406876261));
#150392=CARTESIAN_POINT('Ctrl Pts',(-4.257157031,4.559170361,-6.174675215));
#150393=CARTESIAN_POINT('Ctrl Pts',(-3.230523466,4.690053947,-6.490471334));
#150394=CARTESIAN_POINT('Ctrl Pts',(-3.58453771,4.624398499,-6.314266669));
#150395=CARTESIAN_POINT('Ctrl Pts',(-3.917287119,4.559170361,-6.100603383));
#150396=CARTESIAN_POINT('',(-3.56032080319409,4.69005394803158,-6.60106927749502));
#150397=CARTESIAN_POINT('Origin',(0.0905127851222914,4.69642564207801,0.169991447369243));
#150398=CARTESIAN_POINT('',(-3.39542215258012,4.690053949938,-6.54577030265893));
#150399=CARTESIAN_POINT('Origin',(1.18394877235417E-13,4.75000000000067,
1.196959198424E-13));
#150400=CARTESIAN_POINT('Origin',(0.0693281085175074,4.55370510242446,0.17437459689732));
#150401=CARTESIAN_POINT('Origin',(0.115335243645399,4.69643087673821,0.154781016914751));
#150402=CARTESIAN_POINT('Ctrl Pts',(-2.35930162162706,4.559162772,-7.11980219917393));
#150403=CARTESIAN_POINT('Ctrl Pts',(-2.74764941144185,4.624819703,-6.99111469558026));
#150404=CARTESIAN_POINT('Ctrl Pts',(-3.11969647504582,4.690053947,-6.82095164828537));
#150405=CARTESIAN_POINT('Ctrl Pts',(-3.1325640569744,4.69231013193285,-6.81506640642627));
#150406=CARTESIAN_POINT('Ctrl Pts',(-3.14543163890304,4.69456631686582,
-6.80918116456703));
#150407=CARTESIAN_POINT('Ctrl Pts',(-2.505416106,4.559162772,-6.803336691));
#150408=CARTESIAN_POINT('Ctrl Pts',(-2.876502367,4.624819703,-6.66667941000001));
#150409=CARTESIAN_POINT('Ctrl Pts',(-3.230523466,4.690053947,-6.49047133400001));
#150410=CARTESIAN_POINT('Ctrl Pts',(-3.24276760374887,4.69231013193285,
-6.48437701939248));
#150411=CARTESIAN_POINT('Ctrl Pts',(-3.2550117414978,4.69456631686581,-6.47828270478494));
#150412=CARTESIAN_POINT('',(-3.11992551648257,4.69005394784374,-6.82026869691982));
#150413=CARTESIAN_POINT('',(-3.17522449034723,4.6900539466659,-6.6553700036187));
#150414=CARTESIAN_POINT('',(-2.59587005084126,4.59933049942066,-7.03643792557235));
#150415=CARTESIAN_POINT('Origin',(0.0593208058217742,4.55358392054283,0.18204736950036));
#150416=CARTESIAN_POINT('Ctrl Pts',(-2.50984261394196,4.55994605587811,
-6.80170495256708));
#150417=CARTESIAN_POINT('Ctrl Pts',(-2.52412028095697,4.56683176230192,
-6.84078553361449));
#150418=CARTESIAN_POINT('Ctrl Pts',(-2.53843709611326,4.57355155123639,
-6.87990743885963));
#150419=CARTESIAN_POINT('Ctrl Pts',(-2.56710953945787,4.58666922560941,
-6.9581386741797));
#150420=CARTESIAN_POINT('Ctrl Pts',(-2.5814812140756,4.59307444477075,-6.99729177677978));
#150421=CARTESIAN_POINT('Ctrl Pts',(-2.5958700525406,4.5993304994213,-7.03643792494762));
#150422=CARTESIAN_POINT('Origin',(1.46215504981395E-12,4.78597145199609,
3.35495520253914E-12));
#150423=CARTESIAN_POINT('',(-2.41797935133364,4.74999999914954,-7.09953349559792));
#150424=CARTESIAN_POINT('',(-2.5871749920055,4.78575691069861,-7.00153200784835));
#150425=CARTESIAN_POINT('Origin',(1.42413838529096,4.80792638182854,-0.28582768614912));
#150426=CARTESIAN_POINT('',(-2.77644679082714,4.75000000025891,-6.9671617542923));
#150427=CARTESIAN_POINT('Origin',(0.,4.75,0.));
#150428=CARTESIAN_POINT('Origin',(-1.37378626611183,5.02638716985328,0.487689787695301));
#150429=CARTESIAN_POINT('Ctrl Pts',(-2.058047714,4.690053947,-7.212103688));
#150430=CARTESIAN_POINT('Ctrl Pts',(-2.451422449,4.624398499,-7.099850175));
#150431=CARTESIAN_POINT('Ctrl Pts',(-2.830254416,4.559170361,-6.945477661));
#150432=CARTESIAN_POINT('Ctrl Pts',(-1.759736143,4.690053947,-7.033194773));
#150433=CARTESIAN_POINT('Ctrl Pts',(-2.143352525,4.624398499,-6.937212273));
#150434=CARTESIAN_POINT('Ctrl Pts',(-2.514253728,4.559170361,-6.800075602));
#150435=CARTESIAN_POINT('',(-2.05804771252564,4.69005394803173,-7.21210367677717));
#150436=CARTESIAN_POINT('Origin',(0.051853611895134,4.69642561041417,0.185474986327538));
#150437=CARTESIAN_POINT('',(-1.90889194599726,4.690053949938,-7.12264922581068));
#150438=CARTESIAN_POINT('Origin',(1.95806912350882E-13,4.75000000000067,
1.39211558947139E-13));
#150439=CARTESIAN_POINT('Origin',(0.0302218524976797,4.55370498643004,0.185201308694485));
#150440=CARTESIAN_POINT('Origin',(0.0793656699151506,4.696430839033,0.175956526080664));
#150441=CARTESIAN_POINT('Ctrl Pts',(-0.773595447463978,4.559162772,-7.4605252880029));
#150442=CARTESIAN_POINT('Ctrl Pts',(-1.18052789162116,4.624819703,-7.41832972194081));
#150443=CARTESIAN_POINT('Ctrl Pts',(-1.5804567267152,4.690053947,-7.33212411378188));
#150444=CARTESIAN_POINT('Ctrl Pts',(-1.59428862460278,4.6923101319074,-7.32914261541329));
#150445=CARTESIAN_POINT('Ctrl Pts',(-1.60812052249042,4.69456631681494,
-7.32616111704456));
#150446=CARTESIAN_POINT('Ctrl Pts',(-0.984324587,4.559162772,-7.182868863));
#150447=CARTESIAN_POINT('Ctrl Pts',(-1.376112332,4.624819703,-7.12917913000001));
#150448=CARTESIAN_POINT('Ctrl Pts',(-1.759736143,4.690053947,-7.03319477300001));
#150449=CARTESIAN_POINT('Ctrl Pts',(-1.77300411698779,4.69231013190741,
-7.02987506782166));
#150450=CARTESIAN_POINT('Ctrl Pts',(-1.78627209097565,4.69456631681493,
-7.02655536264332));
#150451=CARTESIAN_POINT('',(-1.58082722970849,4.69005394784289,-7.33150636557383));
#150452=CARTESIAN_POINT('',(-1.6702816869935,4.6900539466659,-7.18235055803641));
#150453=CARTESIAN_POINT('',(-1.02255389306326,4.59933049943543,-7.42996524456859));
#150454=CARTESIAN_POINT('Origin',(0.0187991191944201,4.55358393308258,0.190543474815297));
#150455=CARTESIAN_POINT('Ctrl Pts',(-0.988998380749847,4.55994605587036,
-7.18222684255029));
#150456=CARTESIAN_POINT('Ctrl Pts',(-0.994541074017316,4.56683176236791,
-7.22346301788626));
#150457=CARTESIAN_POINT('Ctrl Pts',(-1.00011311666342,4.57355155128146,
-7.26474796650435));
#150458=CARTESIAN_POINT('Ctrl Pts',(-1.01129781094312,4.58666922563949,
-7.34731392651533));
#150459=CARTESIAN_POINT('Ctrl Pts',(-1.0169167240055,4.59307444475724,-7.38864113623438));
#150460=CARTESIAN_POINT('Ctrl Pts',(-1.02255389468507,4.5993304994032,-7.42996524412411));
#150461=CARTESIAN_POINT('Origin',(1.82026702738591E-12,4.78597145200587,
1.19509437068732E-11));
#150462=CARTESIAN_POINT('',(-0.835258513063531,4.75000000340508,-7.45334442874213));
#150463=CARTESIAN_POINT('',(-1.0215658608059,4.78575691075516,-7.39400622716639));
#150464=CARTESIAN_POINT('Origin',(1.45228678331533,4.8079250825528,0.0270015665869461));
#150465=CARTESIAN_POINT('',(-1.21380116044022,4.75000000415435,-7.4011273722088));
#150466=CARTESIAN_POINT('Origin',(0.,4.7500000057058,0.));
#150467=CARTESIAN_POINT('Origin',(-1.44650689480819,5.02638711396738,0.180966637540554));
#150468=CARTESIAN_POINT('Ctrl Pts',(-0.459542598,4.690053947,-7.48590813500001));
#150469=CARTESIAN_POINT('Ctrl Pts',(-0.867851637,4.624398499,-7.460842987));
#150470=CARTESIAN_POINT('Ctrl Pts',(-1.271012251,4.559170361,-7.391517291));
#150471=CARTESIAN_POINT('Ctrl Pts',(-0.206665513,4.690053947,-7.24705384));
#150472=CARTESIAN_POINT('Ctrl Pts',(-0.601946558,4.624398499,-7.235781541));
#150473=CARTESIAN_POINT('Ctrl Pts',(-0.993656627,4.559170361,-7.18158384400001));
#150474=CARTESIAN_POINT('',(-0.459542598855283,4.69005394803158,-7.48590812356305));
#150475=CARTESIAN_POINT('Origin',(0.0107696487616114,4.69642563687689,0.192285589499794));
#150476=CARTESIAN_POINT('',(-0.333104073596248,4.690053949938,-7.36648098668171));
#150477=CARTESIAN_POINT('Origin',(-7.98243849492453E-14,4.75000000000044,
-2.38524477946811E-13));
#150478=CARTESIAN_POINT('Origin',(-0.010297498977334,4.55370514355358,0.187368216690001));
#150479=CARTESIAN_POINT('Origin',(0.039684243872064,4.6964308192229,0.188901957144474));
#150480=CARTESIAN_POINT('Ctrl Pts',(0.848283189457317,4.559162772,-7.45240250625932));
#150481=CARTESIAN_POINT('Ctrl Pts',(0.441793800428909,4.624819703,-7.49867189602281));
#150482=CARTESIAN_POINT('Ctrl Pts',(0.0326834214338154,4.690053947,-7.50045460506005));
#150483=CARTESIAN_POINT('Ctrl Pts',(0.0185339716261254,4.69231013190414,
-7.50051626165285));
#150484=CARTESIAN_POINT('Ctrl Pts',(0.00438452181843482,4.69456631680839,
-7.50057791824562));
#150485=CARTESIAN_POINT('Ctrl Pts',(0.582792857,4.559162772,-7.226538071));
#150486=CARTESIAN_POINT('Ctrl Pts',(0.188623186,4.624819703,-7.25832635800001));
#150487=CARTESIAN_POINT('Ctrl Pts',(-0.206665513,4.690053947,-7.24705384000001));
#150488=CARTESIAN_POINT('Ctrl Pts',(-0.220336927594239,4.69231013190414,
-7.2466639698431));
#150489=CARTESIAN_POINT('Ctrl Pts',(-0.234008342188472,4.69456631680839,
-7.24627409968621));
#150490=CARTESIAN_POINT('',(0.0321887829827294,4.69005394784288,-7.49993094664959));
#150491=CARTESIAN_POINT('',(-0.0872383680465477,4.6900539466659,-7.37349238247579));
#150492=CARTESIAN_POINT('',(0.598575747913816,4.59933049944211,-7.47607564637949));
#150493=CARTESIAN_POINT('Origin',(-0.0226016148045383,4.55358392282057,
0.190129924982587));
#150494=CARTESIAN_POINT('Ctrl Pts',(0.578090317678936,4.5599460558702,-7.22691578740445));
#150495=CARTESIAN_POINT('Ctrl Pts',(0.581541768273302,4.5668317623654,-7.26837939903823));
#150496=CARTESIAN_POINT('Ctrl Pts',(0.584975040463299,4.57355155126758,
-7.30989695284797));
#150497=CARTESIAN_POINT('Ctrl Pts',(0.591801078882446,4.58666922564616,
-7.39293694531079));
#150498=CARTESIAN_POINT('Ctrl Pts',(0.595197661341285,4.59307444478516,
-7.43450584816564));
#150499=CARTESIAN_POINT('Ctrl Pts',(0.598575746204673,4.59933049942523,
-7.47607564640007));
#150500=CARTESIAN_POINT('Origin',(-5.73082163321526E-13,4.7859714520137,
8.00574884163296E-12));
#150501=CARTESIAN_POINT('',(0.786518118240955,4.74999999914956,-7.45864526901614));
#150502=CARTESIAN_POINT('',(0.591810554745355,4.78575691077897,-7.44074493328967));
#150503=CARTESIAN_POINT('Origin',(1.41252907240432,4.807928318978,0.338567896634023));
#150504=CARTESIAN_POINT('',(0.405600429422982,4.7500000004036,-7.48902450137449));
#150505=CARTESIAN_POINT('Origin',(0.,4.75,0.));
#150506=CARTESIAN_POINT('Origin',(-1.45158988728563,5.0263873102246,-0.134224246665127));
#150507=CARTESIAN_POINT('Ctrl Pts',(1.16045022,4.690053947,-7.409679837));
#150508=CARTESIAN_POINT('Ctrl Pts',(0.756298953000001,4.624398499,-7.47297507200001));
#150509=CARTESIAN_POINT('Ctrl Pts',(0.347661035,4.559170361,-7.491937787));
#150510=CARTESIAN_POINT('Ctrl Pts',(1.356068566,4.690053947,-7.122048725));
#150511=CARTESIAN_POINT('Ctrl Pts',(0.967605761,4.624398499,-7.196013706));
#150512=CARTESIAN_POINT('Ctrl Pts',(0.573402753,4.559170361,-7.227289207));
#150513=CARTESIAN_POINT('',(1.16045021669141,4.69005394803158,-7.40967982615787));
#150514=CARTESIAN_POINT('Origin',(-0.0308178595828214,4.69642561677658,
0.190105271132082));
#150515=CARTESIAN_POINT('',(1.25825937515092,4.690053949938,-7.265864284091));
#150516=CARTESIAN_POINT('Origin',(-3.05101267600999E-14,4.75000000000067,
7.27716498172271E-13));
#150517=CARTESIAN_POINT('Origin',(-0.0503353653922689,4.55370522141256,
0.180773999130557));
#150518=CARTESIAN_POINT('Origin',(-0.00185191242419259,4.69643088564423,
0.193018537816066));
#150519=CARTESIAN_POINT('Ctrl Pts',(2.43049704745381,4.559162772,-7.09581366672906));
#150520=CARTESIAN_POINT('Ctrl Pts',(2.04345770503465,4.624819703,-7.22838450697445));
#150521=CARTESIAN_POINT('Ctrl Pts',(1.64429532976121,4.690053947,-7.31807217464651));
#150522=CARTESIAN_POINT('Ctrl Pts',(1.63048994031571,4.69231013194975,-7.32117410322842));
#150523=CARTESIAN_POINT('Ctrl Pts',(1.61668455087021,4.6945663168996,-7.32427603181019));
#150524=CARTESIAN_POINT('Ctrl Pts',(2.122659554,4.559162772,-6.932302389));
#150525=CARTESIAN_POINT('Ctrl Pts',(1.744538893,4.624819703,-7.04808231200001));
#150526=CARTESIAN_POINT('Ctrl Pts',(1.356068566,4.690053947,-7.122048725));
#150527=CARTESIAN_POINT('Ctrl Pts',(1.34263297065216,4.69231013194975,-7.12460691986156));
#150528=CARTESIAN_POINT('Ctrl Pts',(1.32919737530432,4.69456631689961,-7.12716511472311));
#150529=CARTESIAN_POINT('',(1.64369968460078,4.69005394784289,-7.3176670917166));
#150530=CARTESIAN_POINT('',(1.49988411999609,4.69005394666591,-7.2198578984163));
#150531=CARTESIAN_POINT('',(2.19171665251882,4.5993304993999,-7.17261306051613));
#150532=CARTESIAN_POINT('Origin',(-0.0629454646808558,4.55358396244398,
0.180825979175384));
#150533=CARTESIAN_POINT('Ctrl Pts',(2.11814815554888,4.55994605589016,-6.93368218179206));
#150534=CARTESIAN_POINT('Ctrl Pts',(2.13043236396242,4.56683176230701,-6.97343443721287));
#150535=CARTESIAN_POINT('Ctrl Pts',(2.14271041516511,4.57355155128209,-7.01324328231874));
#150536=CARTESIAN_POINT('Ctrl Pts',(2.16722800827723,4.58666922560028,-7.09287444942555));
#150537=CARTESIAN_POINT('Ctrl Pts',(2.17948126587846,4.59307444474345,-7.13274132976735));
#150538=CARTESIAN_POINT('Ctrl Pts',(2.19171665082185,4.59933049938899,-7.17261306095534));
#150539=CARTESIAN_POINT('Origin',(8.5717023756704E-13,4.78597145200391,
-2.99760216648792E-12));
#150540=CARTESIAN_POINT('',(2.37151803891094,4.7499999938475,-7.11518813706192));
#150541=CARTESIAN_POINT('',(2.17751456608805,4.78575691087531,-7.13956267624426));
#150542=CARTESIAN_POINT('Origin',(1.30672564833516,4.8079276597757,0.634279716635853));
#150543=CARTESIAN_POINT('',(2.00603658800724,4.74999999555741,-7.22674317728731));
#150544=CARTESIAN_POINT('Origin',(0.,4.74999999326975,0.));
#150545=CARTESIAN_POINT('Origin',(-1.38878602413738,5.02638845336712,-0.443159275849884));
#150546=CARTESIAN_POINT('Ctrl Pts',(2.726181675,4.690053947,-6.986983146));
#150547=CARTESIAN_POINT('Ctrl Pts',(2.345085845,4.624398499,-7.135679149));
#150548=CARTESIAN_POINT('Ctrl Pts',(1.950078078,4.559170361,-7.24204359900001));
#150549=CARTESIAN_POINT('Ctrl Pts',(2.855394386,4.690053947,-6.664024527));
#150550=CARTESIAN_POINT('Ctrl Pts',(2.491913911,4.624398499,-6.819768268));
#150551=CARTESIAN_POINT('Ctrl Pts',(2.113650457,4.559170361,-6.93505456));
#150552=CARTESIAN_POINT('',(2.72618166935645,4.69005394803174,-6.98698313594653));
#150553=CARTESIAN_POINT('Origin',(-0.0709643567426155,4.69642561864978,
0.179035762751935));
#150554=CARTESIAN_POINT('',(2.7907880137327,4.690053949938,-6.82550384335576));
#150555=CARTESIAN_POINT('Origin',(-4.50052321798733E-13,4.75090401395802,
1.38300829122251E-12));
#150556=CARTESIAN_POINT('Origin',(-0.0880199733596998,4.55370251574272,
0.165726709096222));
#150557=CARTESIAN_POINT('Origin',(-0.0433024939353446,4.69643084185895,
0.188110501452672));
#150558=CARTESIAN_POINT('Ctrl Pts',(3.89906356438713,4.559162772,-6.40743246671499));
#150559=CARTESIAN_POINT('Ctrl Pts',(3.54957179941302,4.624819703,-6.6201058918965));
#150560=CARTESIAN_POINT('Ctrl Pts',(3.17902181505483,4.690053947,-6.79350482402605));
#150561=CARTESIAN_POINT('Ctrl Pts',(3.16620601100702,4.69231013192402,-6.79950198184572));
#150562=CARTESIAN_POINT('Ctrl Pts',(3.15339020695927,4.69456631684815,-6.80549913966536));
#150563=CARTESIAN_POINT('Ctrl Pts',(3.563273049,4.559162772,-6.313919953));
#150564=CARTESIAN_POINT('Ctrl Pts',(3.2188819,4.624819703,-6.508277771));
#150565=CARTESIAN_POINT('Ctrl Pts',(2.855394386,4.690053947,-6.664024527));
#150566=CARTESIAN_POINT('Ctrl Pts',(2.84282284383327,4.69231013192402,-6.66941116845251));
#150567=CARTESIAN_POINT('Ctrl Pts',(2.83025130166646,4.69456631684816,-6.67479780990509));
#150568=CARTESIAN_POINT('',(3.1783530148737,4.69005394784287,-6.79323725781927));
#150569=CARTESIAN_POINT('',(3.01687369313244,4.69005394666591,-6.72863088383735));
#150570=CARTESIAN_POINT('',(3.68237532182294,4.59933049940066,-6.53376705968035));
#150571=CARTESIAN_POINT('Origin',(-0.10034614614094,4.55358391768731,0.163067068109141));
#150572=CARTESIAN_POINT('Ctrl Pts',(3.55916373987557,4.55994605586385,-6.31623730438967));
#150573=CARTESIAN_POINT('Ctrl Pts',(3.5797063099409,4.56683176228965,-6.35241943252761));
#150574=CARTESIAN_POINT('Ctrl Pts',(3.60025503180654,4.57355155123174,-6.38865815067293));
#150575=CARTESIAN_POINT('Ctrl Pts',(3.64131776415789,4.58666922559734,-6.46115702773757));
#150576=CARTESIAN_POINT('Ctrl Pts',(3.66185474822864,4.59307444476411,-6.49745775448508));
#150577=CARTESIAN_POINT('Ctrl Pts',(3.68237532020963,4.59933049940131,-6.53376706059202));
#150578=CARTESIAN_POINT('Origin',(1.14600169631718E-12,4.78597145199413,
-1.87566975839992E-12));
#150579=CARTESIAN_POINT('',(3.84562837013886,4.74999999914954,-6.43903272537783));
#150580=CARTESIAN_POINT('',(3.66140041776986,4.78575691070765,-6.50454240333656));
#150581=CARTESIAN_POINT('Origin',(1.1398144114279,4.80792588123016,0.900383793170842));
#150582=CARTESIAN_POINT('',(3.51267274782531,4.75000000027185,-6.62654735586201));
#150583=CARTESIAN_POINT('Origin',(0.,4.75,0.));
#150584=CARTESIAN_POINT('Origin',(-1.2610691785014,5.02638720208912,-0.731323920078562));
#150585=CARTESIAN_POINT('Ctrl Pts',(4.164439905,4.690053947,-6.237582888));
#150586=CARTESIAN_POINT('Ctrl Pts',(3.824219129,4.624398499,-6.464726799));
#150587=CARTESIAN_POINT('Ctrl Pts',(3.461311636,4.559170361,-6.653519501));
#150588=CARTESIAN_POINT('Ctrl Pts',(4.221205138,4.690053947,-5.894397949));
#150589=CARTESIAN_POINT('Ctrl Pts',(3.899702935,4.624398499,-6.124638046));
#150590=CARTESIAN_POINT('Ctrl Pts',(3.555066216,4.559170361,-6.318544469));
#150591=CARTESIAN_POINT('',(4.16443989737977,4.69005394803158,-6.23758287935845));
#150592=CARTESIAN_POINT('Origin',(-0.107792655760439,4.69642564592103,0.159594784685343));
#150593=CARTESIAN_POINT('',(4.1928225065985,4.690053949938,-6.06599042879994));
#150594=CARTESIAN_POINT('Origin',(-1.8995222061946E-13,4.74999999999911,
2.71917904859365E-13));
#150595=CARTESIAN_POINT('Origin',(-0.121588202048631,4.55370494317573,0.142930731139171));
#150596=CARTESIAN_POINT('Origin',(-0.0827268737517912,4.69643090457438,
0.174400752628615));
#150597=CARTESIAN_POINT('Ctrl Pts',(5.18531420312347,4.559162772,-5.41944684537583));
#150598=CARTESIAN_POINT('Ctrl Pts',(4.88971186047583,4.624819703,-5.70227848261605));
#150599=CARTESIAN_POINT('Ctrl Pts',(4.56510077449987,4.690053947,-5.95128073642792));
#150600=CARTESIAN_POINT('Ctrl Pts',(4.55387380845167,4.692310131937,-5.9598927030866));
#150601=CARTESIAN_POINT('Ctrl Pts',(4.54264684240356,4.6945663168741,-5.96850466974531));
#150602=CARTESIAN_POINT('Ctrl Pts',(4.837271857,4.559162772,-5.400305637));
#150603=CARTESIAN_POINT('Ctrl Pts',(4.54271356700001,4.624819703,-5.664153394));
#150604=CARTESIAN_POINT('Ctrl Pts',(4.221205138,4.690053947,-5.894397949));
#150605=CARTESIAN_POINT('Ctrl Pts',(4.21008548013084,4.692310131937,-5.90236116379284));
#150606=CARTESIAN_POINT('Ctrl Pts',(4.19896582226168,4.69456631687411,-5.91032437858578));
#150607=CARTESIAN_POINT('',(4.56439009168813,4.69005394784288,-5.9511631980305));
#150608=CARTESIAN_POINT('',(4.39279760585611,4.69005394666591,-5.92278056671925));
#150609=CARTESIAN_POINT('',(5.00085021438104,4.59933049938672,-5.58940937257166));
#150610=CARTESIAN_POINT('Origin',(-0.133054669290137,4.55358395399458,0.137683165336694));
#150611=CARTESIAN_POINT('Ctrl Pts',(4.83375678258189,4.55994605579482,-5.40345218965846));
#150612=CARTESIAN_POINT('Ctrl Pts',(4.86159716688665,4.56683176220404,-5.43437235436266));
#150613=CARTESIAN_POINT('Ctrl Pts',(4.88945572468579,4.57355155121591,-5.46534646398862));
#150614=CARTESIAN_POINT('Ctrl Pts',(4.94514354884021,4.58666922555817,-5.52732308389661));
#150615=CARTESIAN_POINT('Ctrl Pts',(4.97300397295751,4.59307444472928,-5.55836027535948));
#150616=CARTESIAN_POINT('Ctrl Pts',(5.00085021303988,4.59933049938737,-5.58940937377434));
#150617=CARTESIAN_POINT('Origin',(-5.44833275717416E-12,4.78597145200978,
6.35385841163405E-12));
#150618=CARTESIAN_POINT('',(5.13992141746291,4.74999999882868,-5.46179529326095));
#150619=CARTESIAN_POINT('',(4.97408325416057,4.7857569107727,-5.56537695720217));
#150620=CARTESIAN_POINT('Origin',(0.919614054641487,4.80792560169836,1.12435350215151));
#150621=CARTESIAN_POINT('',(4.85506021308921,4.7500000000112,-5.71650155458869));
#150622=CARTESIAN_POINT('Origin',(0.,4.74999999935832,0.));
#150623=CARTESIAN_POINT('Origin',(-1.07437204041214,5.02638715273715,-0.985319364612672));
#150624=CARTESIAN_POINT('Ctrl Pts',(5.407973553,4.690053947,-5.196520186));
#150625=CARTESIAN_POINT('Ctrl Pts',(5.124536177,4.624398499,-5.491491009));
#150626=CARTESIAN_POINT('Ctrl Pts',(4.81069811,4.559170361,-5.753884227));
#150627=CARTESIAN_POINT('Ctrl Pts',(5.38963703,4.690053947,-4.849155874));
#150628=CARTESIAN_POINT('Ctrl Pts',(5.125146184,4.624398499,-5.143126555));
#150629=CARTESIAN_POINT('Ctrl Pts',(4.830251029,4.559170361,-5.406586261));
#150630=CARTESIAN_POINT('',(5.40797354386518,4.69005394803172,-5.19652017958922));
#150631=CARTESIAN_POINT('Origin',(-0.139580695309564,4.69642566362389,0.132691297140924));
#150632=CARTESIAN_POINT('',(5.39880527916107,4.690053949938,-5.02283804326252));
#150633=CARTESIAN_POINT('Origin',(-1.26287869051112E-12,4.74999999999956,
1.40512601554121E-12));
#150634=CARTESIAN_POINT('Origin',(-0.149471413819263,4.55370501835464,0.113451231802965));
#150635=CARTESIAN_POINT('Origin',(-0.118283791850866,4.69643088939873,0.152539578053445));
#150636=CARTESIAN_POINT('Ctrl Pts',(6.22910531271845,4.559162772,-4.17805391237519));
#150637=CARTESIAN_POINT('Ctrl Pts',(6.0012144302889,4.624819703,-4.51781886921915));
#150638=CARTESIAN_POINT('Ctrl Pts',(5.73772069551008,4.690053947,-4.83078137711657));
#150639=CARTESIAN_POINT('Ctrl Pts',(5.72860752801795,4.6923101319233,-4.84160546656077));
#150640=CARTESIAN_POINT('Ctrl Pts',(5.71949436052576,4.69456631684671,-4.85242955600499));
#150641=CARTESIAN_POINT('Ctrl Pts',(5.88508521,4.559162772,-4.234179032));
#150642=CARTESIAN_POINT('Ctrl Pts',(5.65413299700001,4.624819703,-4.5551795));
#150643=CARTESIAN_POINT('Ctrl Pts',(5.38963702999999,4.690053947,-4.849155874));
#150644=CARTESIAN_POINT('Ctrl Pts',(5.38048919940626,4.6923101319233,-4.85932331094969));
#150645=CARTESIAN_POINT('Ctrl Pts',(5.37134136881263,4.69456631684671,-4.86949074789924));
#150646=CARTESIAN_POINT('',(5.73700136077215,4.69005394784288,-4.83081936251135));
#150647=CARTESIAN_POINT('',(5.56331918515664,4.6900539466659,-4.83998761354413));
#150648=CARTESIAN_POINT('',(6.08549090878228,4.59933049942498,-4.38369711544624));
#150649=CARTESIAN_POINT('Origin',(-0.159541754778343,4.55358395733858,0.105861394661615));
#150650=CARTESIAN_POINT('Ctrl Pts',(5.8823287320493,4.55994605591031,-4.23800765756635));
#150651=CARTESIAN_POINT('Ctrl Pts',(5.91616514536365,4.5668317623968,-4.26222006641938));
#150652=CARTESIAN_POINT('Ctrl Pts',(5.95003090265298,4.57355155125049,-4.28648125144309));
#150653=CARTESIAN_POINT('Ctrl Pts',(6.01773991774795,4.5866692256407,-4.3350376563432));
#150654=CARTESIAN_POINT('Ctrl Pts',(6.05162105914308,4.59307444479192,-4.35936004775182));
#150655=CARTESIAN_POINT('Ctrl Pts',(6.08549090774786,4.59933049942563,-4.38369711688568));
#150656=CARTESIAN_POINT('Origin',(-3.96991467477292E-12,4.7859714520137,
2.91780488659299E-12));
#150657=CARTESIAN_POINT('',(6.19387744881142,4.74999999914954,-4.22917038556074));
#150658=CARTESIAN_POINT('',(6.05418348610776,4.78575691089176,-4.36598066988852));
#150659=CARTESIAN_POINT('Origin',(0.656406945464102,4.80792672811356,1.29576130127513));
#150660=CARTESIAN_POINT('',(5.97043045959225,4.75000000037016,-4.53915849232614));
#150661=CARTESIAN_POINT('Origin',(0.,4.75,0.));
#150662=CARTESIAN_POINT('Origin',(-0.837438612039119,5.02638723124253,-1.19324172669549));
#150663=CARTESIAN_POINT('Ctrl Pts',(6.398636369,4.690053947,-3.912473977));
#150664=CARTESIAN_POINT('Ctrl Pts',(6.185235608,4.624398499,-4.261479203));
#150665=CARTESIAN_POINT('Ctrl Pts',(5.935141687,4.559170361,-4.585203721));
#150666=CARTESIAN_POINT('Ctrl Pts',(6.306055484,4.690053947,-3.577172659));
#150667=CARTESIAN_POINT('Ctrl Pts',(6.110943294,4.624398499,-3.921128183));
#150668=CARTESIAN_POINT('Ctrl Pts',(5.879578673,4.559170361,-4.241822088));
#150669=CARTESIAN_POINT('',(6.39863635852685,4.69005394803158,-3.91247397243082));
#150670=CARTESIAN_POINT('Origin',(-0.164842356092871,4.69642565962801,0.0995835179095694));
#150671=CARTESIAN_POINT('',(6.35234591730059,4.690053949938,-3.74482333360496));
#150672=CARTESIAN_POINT('Origin',(-1.02261948908833E-12,4.75,7.79324521582581E-13));
#150673=CARTESIAN_POINT('Origin',(-0.170365513633566,4.55370509620838,0.0786668822203401));
#150674=CARTESIAN_POINT('Origin',(-0.148309793580546,4.69643087912402,0.123545680302601));
#150675=CARTESIAN_POINT('Ctrl Pts',(6.98163038085746,4.559162772,-2.74129982288076));
#150676=CARTESIAN_POINT('Ctrl Pts',(6.83210688281943,4.624819703,-3.12211106707122));
#150677=CARTESIAN_POINT('Ctrl Pts',(6.64205117339044,4.690053947,-3.4844000493798));
#150678=CARTESIAN_POINT('Ctrl Pts',(6.63547792607009,4.69231013188838,-3.49693013905352));
#150679=CARTESIAN_POINT('Ctrl Pts',(6.62890467874978,4.69456631677688,-3.50946022872725));
#150680=CARTESIAN_POINT('Ctrl Pts',(6.657718518,4.559162772,-2.870066921));
#150681=CARTESIAN_POINT('Ctrl Pts',(6.501171452,4.624819703,-3.233210475));
#150682=CARTESIAN_POINT('Ctrl Pts',(6.306055484,4.690053947,-3.577172659));
#150683=CARTESIAN_POINT('Ctrl Pts',(6.29930722309448,4.69231013188838,-3.58906889990256));
#150684=CARTESIAN_POINT('Ctrl Pts',(6.29255896218899,4.69456631677687,-3.60096514080513));
#150685=CARTESIAN_POINT('',(6.64135682204414,4.69005394784288,-3.48459178239997));
#150686=CARTESIAN_POINT('',(6.47370614201999,4.69005394666591,-3.53088221829681));
#150687=CARTESIAN_POINT('',(6.88558081144145,4.59933049941794,-2.97300805372012));
#150688=CARTESIAN_POINT('Origin',(-0.178568932337102,4.55358397399639,0.0690897059675322));
#150689=CARTESIAN_POINT('Ctrl Pts',(6.65584952666731,4.55994605584957,-2.87439859628003));
#150690=CARTESIAN_POINT('Ctrl Pts',(6.6940998151804,4.5668317622885,-2.89077110385448));
#150691=CARTESIAN_POINT('Ctrl Pts',(6.73238924811481,4.57355155126783,-2.90718493953025));
#150692=CARTESIAN_POINT('Ctrl Pts',(6.80895345550018,4.58666922562728,-2.9400506860028));
#150693=CARTESIAN_POINT('Ctrl Pts',(6.84727106988585,4.59307444478919,-2.95652098963909));
#150694=CARTESIAN_POINT('Ctrl Pts',(6.88558081071488,4.59933049941858,-2.97300805540815));
#150695=CARTESIAN_POINT('Origin',(3.95473584435813E-12,4.78597145199804,
-1.96283961306776E-12));
#150696=CARTESIAN_POINT('',(6.95821465503485,4.74999999914954,-2.79879417147286));
#150697=CARTESIAN_POINT('',(6.8511968275965,4.78575691069479,-2.9624359783415));
#150698=CARTESIAN_POINT('Origin',(0.362509295536758,4.80792588316658,1.40657558479531));
#150699=CARTESIAN_POINT('',(6.80663001231747,4.75000000027878,-3.14956942582316));
#150700=CARTESIAN_POINT('Origin',(0.,4.75,0.));
#150701=CARTESIAN_POINT('Origin',(-0.561349968343476,5.0263871185875,-1.3453684552072));
#150702=CARTESIAN_POINT('Ctrl Pts',(7.090106059,4.690053947,-2.445484832));
#150703=CARTESIAN_POINT('Ctrl Pts',(6.95672029700001,4.624398499,-2.832205366));
#150704=CARTESIAN_POINT('Ctrl Pts',(6.782064634,4.559170361,-3.202124185));
#150705=CARTESIAN_POINT('Ctrl Pts',(6.927609792,4.690053947,-2.137924827));
#150706=CARTESIAN_POINT('Ctrl Pts',(6.810999487,4.624398499,-2.515782215));
#150707=CARTESIAN_POINT('Ctrl Pts',(6.653983753,4.559170361,-2.87871503));
#150708=CARTESIAN_POINT('',(7.09010604806595,4.69005394803172,-2.44548483005023));
#150709=CARTESIAN_POINT('Origin',(-0.182395659034899,4.69642565507823,0.0618189606728303));
#150710=CARTESIAN_POINT('',(7.00885791987027,4.690053949938,-2.29170484671772));
#150711=CARTESIAN_POINT('Origin',(1.12757025938492E-13,4.74999999999867,
-4.25007251614318E-14));
#150712=CARTESIAN_POINT('Origin',(-0.183293516937355,4.55370498131794,0.0402041254209368));
#150713=CARTESIAN_POINT('Origin',(-0.17140124332232,4.69643083059612,0.0887751290949265));
#150714=CARTESIAN_POINT('Ctrl Pts',(7.40770217167405,4.559162772,-1.17636559943074));
#150715=CARTESIAN_POINT('Ctrl Pts',(7.34353761132999,4.624819703,-1.58041682070035));
#150716=CARTESIAN_POINT('Ctrl Pts',(7.23580672026506,4.690053947,-1.97509204846267));
#150717=CARTESIAN_POINT('Ctrl Pts',(7.23208075058599,4.692310131951,-1.98874224588683));
#150718=CARTESIAN_POINT('Ctrl Pts',(7.22835478090692,4.69456631690211,-2.00239244331094));
#150719=CARTESIAN_POINT('Ctrl Pts',(7.11904430900001,4.559162772,-1.371753671));
#150720=CARTESIAN_POINT('Ctrl Pts',(7.044222355,4.624819703,-1.760060122));
#150721=CARTESIAN_POINT('Ctrl Pts',(6.927609792,4.690053947,-2.137924827));
#150722=CARTESIAN_POINT('Ctrl Pts',(6.92357664171564,4.692310131951,-2.15099361738777));
#150723=CARTESIAN_POINT('Ctrl Pts',(6.91954349143118,4.69456631690211,-2.1640624077756));
#150724=CARTESIAN_POINT('',(7.23516982050699,4.69005394784373,-1.97542856188366));
#150725=CARTESIAN_POINT('',(7.08138979442916,4.69005394666591,-2.05667669546547));
#150726=CARTESIAN_POINT('',(7.36370860875662,4.59933049944325,-1.42330443902713));
#150727=CARTESIAN_POINT('Origin',(-0.189246121424158,4.55358393686277,0.0290873285901153));
#150728=CARTESIAN_POINT('Ctrl Pts',(7.11815019508415,4.55994605582322,-1.37638585233793));
#150729=CARTESIAN_POINT('Ctrl Pts',(7.15902581871411,4.56683176234725,-1.38415289818672));
#150730=CARTESIAN_POINT('Ctrl Pts',(7.1999485548656,4.57355155123402,-1.39195189089798));
#150731=CARTESIAN_POINT('Ctrl Pts',(7.28178789791662,4.58666922564619,-1.40759021280355));
#150732=CARTESIAN_POINT('Ctrl Pts',(7.32275029616096,4.59307444480266,-1.41543829532522));
#150733=CARTESIAN_POINT('Ctrl Pts',(7.36370860839515,4.59933049943885,-1.42330444072867));
#150734=CARTESIAN_POINT('Origin',(-2.30674854218016E-12,4.785971452,5.12827627585644E-13));
#150735=CARTESIAN_POINT('',(7.39719347865309,4.74999999914955,-1.23754944963554));
#150736=CARTESIAN_POINT('',(7.32785581920364,4.78575691081595,-1.42037107383782));
#150737=CARTESIAN_POINT('Origin',(0.0516638793933411,4.80792777455635,1.45161900251207));
#150738=CARTESIAN_POINT('',(7.32455911116738,4.75000000048191,-1.61270999145831));
#150739=CARTESIAN_POINT('Origin',(0.,4.75,0.));
#150740=CARTESIAN_POINT('Origin',(-0.2590104406192,5.02638720502974,-1.43458817797988));
#150741=CARTESIAN_POINT('Ctrl Pts',(7.450050271,4.690053947,-0.864147535));
#150742=CARTESIAN_POINT('Ctrl Pts',(7.402916477,4.624398499,-1.270500754));
#150743=CARTESIAN_POINT('Ctrl Pts',(7.311865778,4.559170361,-1.669316881));
#150744=CARTESIAN_POINT('Ctrl Pts',(7.225236766,4.690053947,-0.598710006));
#150745=CARTESIAN_POINT('Ctrl Pts',(7.192580914,4.624398499,-0.992801067));
#150746=CARTESIAN_POINT('Ctrl Pts',(7.11725594700001,4.559170361,-1.381002455));
#150747=CARTESIAN_POINT('',(7.45005025959605,4.69005394803157,-0.86414753525958));
#150748=CARTESIAN_POINT('Origin',(-0.1914207062953,4.69642563955896,0.0211640149895437));
#150749=CARTESIAN_POINT('',(7.3376435167032,4.690053949938,-0.731428788525407));
#150750=CARTESIAN_POINT('Origin',(-3.65592972562112E-13,4.74999999999956,
3.09539720244612E-14));
#150751=CARTESIAN_POINT('Origin',(-0.187650922791914,4.55370525479523,-0.000138467856823088));
#150752=CARTESIAN_POINT('Origin',(-0.186477895557537,4.69643089301974,0.0498533727623198));
#150753=CARTESIAN_POINT('Ctrl Pts',(7.48711801033638,4.559162772,0.44327900366248));
#150754=CARTESIAN_POINT('Ctrl Pts',(7.51129654999285,4.624819703,0.0348960660702782));
#150755=CARTESIAN_POINT('Ctrl Pts',(7.49091351203571,4.690053947,-0.373693895907041));
#150756=CARTESIAN_POINT('Ctrl Pts',(7.49060672318581,4.69103579959394,-0.379843658507606));
#150757=CARTESIAN_POINT('Ctrl Pts',(7.49029993433593,4.6920176521879,-0.385993421108172));
#150758=CARTESIAN_POINT('Ctrl Pts',(7.24749149900001,4.559162772,0.190701257));
#150759=CARTESIAN_POINT('Ctrl Pts',(7.25789325,4.624819703,-0.204611314));
#150760=CARTESIAN_POINT('Ctrl Pts',(7.225236766,4.690053947,-0.598710006));
#150761=CARTESIAN_POINT('Ctrl Pts',(7.22474524725832,4.69103579959394,-0.604641657833209));
#150762=CARTESIAN_POINT('Ctrl Pts',(7.22425372851668,4.6920176521879,-0.610573309666416));
#150763=CARTESIAN_POINT('',(7.35795553086503,4.69005394666591,-0.486303255542236));
#150764=CARTESIAN_POINT('Ctrl Pts',(7.24761407171314,4.55994605590014,0.185985165651878));
#150765=CARTESIAN_POINT('Ctrl Pts',(7.28920373119989,4.56683176237926,0.18718675957936));
#150766=CARTESIAN_POINT('Ctrl Pts',(7.3308462695689,4.57355155126511,0.188367281422137));
#150767=CARTESIAN_POINT('Ctrl Pts',(7.41413403124873,4.58666922565181,0.190687614150122));
#150768=CARTESIAN_POINT('Ctrl Pts',(7.45582585715068,4.59307444480204,0.191828720144647));
#150769=CARTESIAN_POINT('Ctrl Pts',(7.49751757552699,4.59933049943424,0.192951307213912));
#150770=CARTESIAN_POINT('Ctrl Pts',(7.461638412,4.690053947,0.75759634));
#150771=CARTESIAN_POINT('Ctrl Pts',(7.50296051,4.624398499,0.350611062));
#150772=CARTESIAN_POINT('Ctrl Pts',(7.499772204,4.559170361,-0.058454175));
#150773=CARTESIAN_POINT('Ctrl Pts',(7.18501969900001,4.690053947,0.96849983));
#150774=CARTESIAN_POINT('Ctrl Pts',(7.237845252,4.624398499,0.576602356));
#150775=CARTESIAN_POINT('Ctrl Pts',(7.247733164,4.559170361,0.181284259));
#150776=CARTESIAN_POINT('',(7.32332905762013,4.690053949938,0.863048067009758));
#150777=CARTESIAN_POINT('Ctrl Pts',(7.21699150219654,4.559162772,2.04277290613802));
#150778=CARTESIAN_POINT('Ctrl Pts',(7.3284140276913,4.624819703,1.64912395011814));
#150779=CARTESIAN_POINT('Ctrl Pts',(7.39635994644821,4.690053947,1.24569138829467));
#150780=CARTESIAN_POINT('Ctrl Pts',(7.3987099170171,4.6923101318642,1.23173831113913));
#150781=CARTESIAN_POINT('Ctrl Pts',(7.40105988758591,4.69456631672851,1.21778523398357));
#150782=CARTESIAN_POINT('Ctrl Pts',(7.037054042,4.559162772,1.744239205));
#150783=CARTESIAN_POINT('Ctrl Pts',(7.132193124,4.624819703,1.360404892));
#150784=CARTESIAN_POINT('Ctrl Pts',(7.185019699,4.690053947,0.96849983));
#150785=CARTESIAN_POINT('Ctrl Pts',(7.1868467534983,4.6923101318642,0.954945441769616));
#150786=CARTESIAN_POINT('Ctrl Pts',(7.18867380799659,4.69456631672851,0.941391053539225));
#150787=CARTESIAN_POINT('',(7.39592321004275,4.69005394784287,1.24511854744902));
#150788=CARTESIAN_POINT('',(7.29047144430719,4.69005394666591,1.10680918397654));
#150789=CARTESIAN_POINT('',(7.28075095287772,4.5993304993567,1.80018486846075));
#150790=CARTESIAN_POINT('Origin',(-0.183968844695832,4.55358393281124,-0.053063498517215));
#150791=CARTESIAN_POINT('Ctrl Pts',(7.03818756905549,4.55994605587417,1.73965972261931));
#150792=CARTESIAN_POINT('Ctrl Pts',(7.07854657820646,4.5668317623275,1.74977377151055));
#150793=CARTESIAN_POINT('Ctrl Pts',(7.11896175983951,4.57355155119665,1.75987860837463));
#150794=CARTESIAN_POINT('Ctrl Pts',(7.19980349683551,4.58666922554476,1.7800491000721));
#150795=CARTESIAN_POINT('Ctrl Pts',(7.24027528686319,4.59307444467864,1.79012603792251));
#150796=CARTESIAN_POINT('Ctrl Pts',(7.2807509531506,4.59933049933453,1.80018486672554));
#150797=CARTESIAN_POINT('Origin',(2.78509854068076E-12,4.78597145200391,
5.46546315149943E-13));
#150798=CARTESIAN_POINT('',(7.23314450266305,4.74999999914954,1.98283146086299));
#150799=CARTESIAN_POINT('',(7.24698015455017,4.78575691066646,1.78779292319316));
#150800=CARTESIAN_POINT('Origin',(-0.562631375081327,4.80792660290743,1.33914652932568));
#150801=CARTESIAN_POINT('',(7.32474915907361,4.75000000027873,1.61184659604922));
#150802=CARTESIAN_POINT('Origin',(0.,4.75,0.));
#150803=CARTESIAN_POINT('Origin',(0.367295502146805,5.02638722262568,-1.4107530368421));
#150804=CARTESIAN_POINT('Ctrl Pts',(7.124328633,4.690053947,2.343915853));
#150805=CARTESIAN_POINT('Ctrl Pts',(7.252174449,4.624398499,1.955328694));
#150806=CARTESIAN_POINT('Ctrl Pts',(7.336997617,4.559170361,1.555141784));
#150807=CARTESIAN_POINT('Ctrl Pts',(6.808839097,4.690053947,2.49042369));
#150808=CARTESIAN_POINT('Ctrl Pts',(6.94467599,4.624398499,2.119044493));
#150809=CARTESIAN_POINT('Ctrl Pts',(7.03931443300001,4.559170361,1.735094322));
#150810=CARTESIAN_POINT('',(7.12432862295937,4.69005394803173,2.34391584792582));
#150811=CARTESIAN_POINT('Origin',(-0.182614947261295,4.69642563816072,-0.0611674429381026));
#150812=CARTESIAN_POINT('',(6.96658387093794,4.690053949938,2.41716975438613));
#150813=CARTESIAN_POINT('Origin',(7.34221711207184E-13,4.75,1.25116930704827E-13));
#150814=CARTESIAN_POINT('Origin',(-0.170249199545465,4.55370499927494,-0.0789182823346504));
#150815=CARTESIAN_POINT('Origin',(-0.19017611680666,4.69643086195197,-0.0330544205486318));
#150816=CARTESIAN_POINT('Ctrl Pts',(6.60912646083892,4.559162772,3.54645385109177));
#150817=CARTESIAN_POINT('Ctrl Pts',(6.80256687883279,4.624819703,3.18596073835499));
#150818=CARTESIAN_POINT('Ctrl Pts',(6.95565033528179,4.690053947,2.80656656940863));
#150819=CARTESIAN_POINT('Ctrl Pts',(6.96094486400092,4.69231013187025,2.79344488160548));
#150820=CARTESIAN_POINT('Ctrl Pts',(6.96623939272004,4.69456631674062,2.78032319380227));
#150821=CARTESIAN_POINT('Ctrl Pts',(6.49757176,4.559162772,3.216218467));
#150822=CARTESIAN_POINT('Ctrl Pts',(6.672999573,4.624819703,2.861810077));
#150823=CARTESIAN_POINT('Ctrl Pts',(6.808839097,4.690053947,2.49042369));
#150824=CARTESIAN_POINT('Ctrl Pts',(6.81353722884059,4.69231013187025,2.47757895852168));
#150825=CARTESIAN_POINT('Ctrl Pts',(6.81823536068105,4.69456631674061,2.46473422704338));
#150826=CARTESIAN_POINT('',(6.95534695338064,4.69005394784287,2.80591323583707));
#150827=CARTESIAN_POINT('',(6.88209301623501,4.6900539466659,2.64816845608985));
#150828=CARTESIAN_POINT('',(6.72354450812389,4.59933049937433,3.32324378386072));
#150829=CARTESIAN_POINT('Origin',(-0.168260686740129,4.55358392025965,-0.0913707750342646));
#150830=CARTESIAN_POINT('Ctrl Pts',(6.49966323789616,4.55994605561308,3.21198972494361));
#150831=CARTESIAN_POINT('Ctrl Pts',(6.53690445392065,4.56683176204481,3.23054330674303));
#150832=CARTESIAN_POINT('Ctrl Pts',(6.57420251092965,4.57355155114227,3.24909996799787));
#150833=CARTESIAN_POINT('Ctrl Pts',(6.64881815344445,4.58666922551254,3.28617746836234));
#150834=CARTESIAN_POINT('Ctrl Pts',(6.68617749202659,4.59307444470469,3.30471905155373));
#150835=CARTESIAN_POINT('Ctrl Pts',(6.72354450892563,4.59933049937499,3.32324378224326));
#150836=CARTESIAN_POINT('Origin',(-1.869164545365E-13,4.78597145201174,
-3.26128013483639E-13));
#150837=CARTESIAN_POINT('',(6.63778745075527,4.74999999914955,3.49138622286761));
#150838=CARTESIAN_POINT('',(6.69322715409837,4.78575691073401,3.30388183192065));
#150839=CARTESIAN_POINT('Origin',(-0.837352477505402,4.80792844078444,1.18688978329396));
#150840=CARTESIAN_POINT('',(6.80700122224742,4.7500000001894,3.14876706890607));
#150841=CARTESIAN_POINT('Origin',(0.,4.75,0.));
#150842=CARTESIAN_POINT('Origin',(0.661979220930704,5.02638726725762,-1.29881225515525));
#150843=CARTESIAN_POINT('Ctrl Pts',(6.453893166,4.690053947,3.820636465));
#150844=CARTESIAN_POINT('Ctrl Pts',(6.66228477,4.624398499,3.468617329));
#150845=CARTESIAN_POINT('Ctrl Pts',(6.831153176,4.559170361,3.096021041));
#150846=CARTESIAN_POINT('Ctrl Pts',(6.114284746,4.690053947,3.895898106));
#150847=CARTESIAN_POINT('Ctrl Pts',(6.326781397,4.624398499,3.562402465));
#150848=CARTESIAN_POINT('Ctrl Pts',(6.501745184,4.559170361,3.207773304));
#150849=CARTESIAN_POINT('',(6.45389315726572,4.69005394803157,3.82063645794471));
#150850=CARTESIAN_POINT('Origin',(-0.165196485025554,4.69642563154551,-0.0989942838258595));
#150851=CARTESIAN_POINT('',(6.28408896547809,4.690053949938,3.85826727006272));
#150852=CARTESIAN_POINT('Origin',(-6.24500451351651E-14,4.75000000000111,
-7.78457159844592E-14));
#150853=CARTESIAN_POINT('Origin',(-0.149303794360807,4.55370519153356,-0.1136717409559));
#150854=CARTESIAN_POINT('Origin',(-0.178624331970231,4.69643085591105,-0.0731639354625961));
#150855=CARTESIAN_POINT('Ctrl Pts',(5.69222601069705,4.559162772,4.88430655567154));
#150856=CARTESIAN_POINT('Ctrl Pts',(5.95863926358972,4.624819703,4.57382554319661));
#150857=CARTESIAN_POINT('Ctrl Pts',(6.18970224441328,4.690053947,4.23620981693912));
#150858=CARTESIAN_POINT('Ctrl Pts',(6.19769376529829,4.69231013196517,4.22453307357731));
#150859=CARTESIAN_POINT('Ctrl Pts',(6.20568528618318,4.69456631693044,4.21285633021548));
#150860=CARTESIAN_POINT('Ctrl Pts',(5.654270243,4.559162772,4.537810928));
#150861=CARTESIAN_POINT('Ctrl Pts',(5.90178398,4.624819703,4.229400204));
#150862=CARTESIAN_POINT('Ctrl Pts',(6.114284746,4.690053947,3.895898106));
#150863=CARTESIAN_POINT('Ctrl Pts',(6.12163427600051,4.69231013196517,3.88436363616904));
#150864=CARTESIAN_POINT('Ctrl Pts',(6.12898380600107,4.69456631693045,3.87282916633803));
#150865=CARTESIAN_POINT('',(6.1895464028051,4.69005394784288,4.23550653979359));
#150866=CARTESIAN_POINT('',(6.15191556712846,4.69005394666591,4.0657023142925));
#150867=CARTESIAN_POINT('',(5.8519525946259,4.59933049938055,4.69091151364114));
#150868=CARTESIAN_POINT('Origin',(-0.144684591781463,4.55358396295006,-0.125405459411204));
#150869=CARTESIAN_POINT('Ctrl Pts',(5.65722187832806,4.55994605571318,4.53413065786506));
#150870=CARTESIAN_POINT('Ctrl Pts',(5.68960394393214,4.56683176216541,4.56025622794808));
#150871=CARTESIAN_POINT('Ctrl Pts',(5.72204085910156,4.57355155117837,4.58639702419375));
#150872=CARTESIAN_POINT('Ctrl Pts',(5.78694146285736,4.58666922554783,4.6386478307439));
#150873=CARTESIAN_POINT('Ctrl Pts',(5.819441468473,4.59307444471782,4.66478707540416));
#150874=CARTESIAN_POINT('Ctrl Pts',(5.85195259571213,4.5993304993756,4.69091151222891));
#150875=CARTESIAN_POINT('Origin',(1.34874750257197E-13,4.78597145199609,
-2.00360561475321E-13));
#150876=CARTESIAN_POINT('',(5.82650629123494,4.78575691079304,4.66548489794723));
#150877=CARTESIAN_POINT('',(5.97096547238726,4.75000000041425,4.53845469496143));
#150878=CARTESIAN_POINT('Origin',(0.92570899729587,5.02638719854594,-1.12614049721395));
#150879=CARTESIAN_POINT('',(5.73205483608437,4.74999999914954,4.8366876429795));
#150880=CARTESIAN_POINT('Origin',(-1.07292243168096,4.80792777578605,0.97913448072838));
#150881=CARTESIAN_POINT('Origin',(0.,4.75,0.));
#150882=CARTESIAN_POINT('Ctrl Pts',(5.481680828,4.690053947,5.118708363));
#150883=CARTESIAN_POINT('Ctrl Pts',(5.76087406,4.624398499,4.819717273));
#150884=CARTESIAN_POINT('Ctrl Pts',(6.005891605,4.559170361,4.492133795));
#150885=CARTESIAN_POINT('Ctrl Pts',(5.133833235,4.690053947,5.119204656));
#150886=CARTESIAN_POINT('Ctrl Pts',(5.413053537,4.624398499,4.839186457));
#150887=CARTESIAN_POINT('Ctrl Pts',(5.660161555,4.559170361,4.530460371));
#150888=CARTESIAN_POINT('',(5.48168082074437,4.69005394803159,5.11870835410218));
#150889=CARTESIAN_POINT('Origin',(-0.14005363540327,4.69642563875725,-0.132192374471661));
#150890=CARTESIAN_POINT('',(5.30775704407508,4.690053949938,5.11895649646111));
#150891=CARTESIAN_POINT('Origin',(8.36136715420821E-13,4.74999999999978,
7.61543605953818E-13));
#150892=CARTESIAN_POINT('Origin',(-0.121377084426482,4.55370515177357,-0.143110064267615));
#150893=CARTESIAN_POINT('Origin',(-0.158719385570818,4.69643090990026,-0.109851836851031));
#150894=CARTESIAN_POINT('Ctrl Pts',(4.50916339979654,4.559162772,5.99377451452989));
#150895=CARTESIAN_POINT('Ctrl Pts',(4.83609229828164,4.624819703,5.74782334937737));
#150896=CARTESIAN_POINT('Ctrl Pts',(5.13433055676917,4.690053947,5.46777260231845));
#150897=CARTESIAN_POINT('Ctrl Pts',(5.14464539467451,4.69231013189109,5.45808679582318));
#150898=CARTESIAN_POINT('Ctrl Pts',(5.15496023257999,4.69456631678204,5.44840098932806));
#150899=CARTESIAN_POINT('Ctrl Pts',(4.546581334,4.559162772,5.647220394));
#150900=CARTESIAN_POINT('Ctrl Pts',(4.85460752600001,4.624819703,5.399228277));
#150901=CARTESIAN_POINT('Ctrl Pts',(5.133833235,4.690053947,5.119204656));
#150902=CARTESIAN_POINT('Ctrl Pts',(5.14349050681334,4.69231013189109,5.10951978768387));
#150903=CARTESIAN_POINT('Ctrl Pts',(5.15314777862652,4.69456631678204,5.09983491936761));
#150904=CARTESIAN_POINT('',(5.13432954246051,4.69005394784287,5.46705226606116));
#150905=CARTESIAN_POINT('',(5.1340813834691,4.69005394666591,5.29312845107505));
#150906=CARTESIAN_POINT('',(4.70672988215593,4.59933049940442,5.83923743480986));
#150907=CARTESIAN_POINT('Origin',(-0.11434362949745,4.55358395443845,-0.153576638647377));
#150908=CARTESIAN_POINT('Ctrl Pts',(4.55025511129988,4.55994605576316,5.644260680249));
#150909=CARTESIAN_POINT('Ctrl Pts',(4.57626387695763,4.5668317622278,5.67673663603041));
#150910=CARTESIAN_POINT('Ctrl Pts',(4.60232293648434,4.57355155120668,5.70923925282838));
#150911=CARTESIAN_POINT('Ctrl Pts',(4.65447382140656,4.58666922558688,5.7742201761127));
#150912=CARTESIAN_POINT('Ctrl Pts',(4.68059483006131,4.59307444475615,5.80673484034052));
#150913=CARTESIAN_POINT('Ctrl Pts',(4.70672988354947,4.59933049940507,5.83923743368921));
#150914=CARTESIAN_POINT('Origin',(-9.19533546528406E-12,4.7859714520137,
-1.14287919406042E-11));
#150915=CARTESIAN_POINT('',(4.55829770857552,4.74999999914954,5.95583092444217));
#150916=CARTESIAN_POINT('',(4.68734446911356,4.78575691068609,5.8089350766075));
#150917=CARTESIAN_POINT('Origin',(-1.25832423490427,4.80792609755448,0.725594838512503));
#150918=CARTESIAN_POINT('',(4.85573401490558,4.75000000031464,5.71592922179221));
#150919=CARTESIAN_POINT('Origin',(0.,4.75,0.));
#150920=CARTESIAN_POINT('Origin',(1.14615261721564,5.02638715152315,-0.900813176263141));
#150921=CARTESIAN_POINT('Ctrl Pts',(4.253151186,4.690053947,6.17743514600001));
#150922=CARTESIAN_POINT('Ctrl Pts',(4.590091282,4.624398499,5.945452595));
#150923=CARTESIAN_POINT('Ctrl Pts',(4.899801218,4.559170361,5.678199365));
#150924=CARTESIAN_POINT('Ctrl Pts',(3.913329389,4.690053947,6.103142887));
#150925=CARTESIAN_POINT('Ctrl Pts',(4.246217311,4.624398499,5.889695469));
#150926=CARTESIAN_POINT('Ctrl Pts',(4.553915063,4.559170361,5.641308146));
#150927=CARTESIAN_POINT('',(4.25315118114086,4.69005394803172,6.17743513593807));
#150928=CARTESIAN_POINT('Origin',(-0.108361582184732,4.69642567909109,-0.159208914794227));
#150929=CARTESIAN_POINT('',(4.08324030258406,4.690053949938,6.14028900646922));
#150930=CARTESIAN_POINT('Origin',(-1.77809156287623E-14,4.74999999999956,
-1.17961196366423E-13));
#150931=CARTESIAN_POINT('Origin',(-0.0877749029782665,4.5537050316539,-0.165856721729633));
#150932=CARTESIAN_POINT('Origin',(-0.131394108785226,4.6964308432268,-0.141403975757775));
#150933=CARTESIAN_POINT('Ctrl Pts',(3.1152573196754,4.559162772,6.82298023810282));
#150934=CARTESIAN_POINT('Ctrl Pts',(3.48741503214274,4.624819703,6.65305932404764));
#150935=CARTESIAN_POINT('Ctrl Pts',(3.83888327806662,4.690053947,6.4436684168068));
#150936=CARTESIAN_POINT('Ctrl Pts',(3.85103912306244,4.6923101319262,6.43642644419198));
#150937=CARTESIAN_POINT('Ctrl Pts',(3.86319496805827,4.69456631685225,6.42918447157713));
#150938=CARTESIAN_POINT('Ctrl Pts',(3.226299335,4.559162772,6.49257211000001));
#150939=CARTESIAN_POINT('Ctrl Pts',(3.58043502,4.624819703,6.316594438));
#150940=CARTESIAN_POINT('Ctrl Pts',(3.913329389,4.690053947,6.10314288700001));
#150941=CARTESIAN_POINT('Ctrl Pts',(3.9248428397782,4.69231013192617,6.09576047337325));
#150942=CARTESIAN_POINT('Ctrl Pts',(3.93635629055647,4.69456631685245,6.08837805974651));
#150943=CARTESIAN_POINT('',(3.83903713682742,4.69005394784374,6.44296470519193));
#150944=CARTESIAN_POINT('',(3.87618326074108,4.69005394666591,6.27305378442417));
#150945=CARTESIAN_POINT('',(3.34142571134262,4.59933049939646,6.71452710297746));
#150946=CARTESIAN_POINT('Origin',(-0.0786558691804817,4.55358394933083,
-0.174566528440784));
#150947=CARTESIAN_POINT('Ctrl Pts',(3.23052347273378,4.55994605588832,6.49047134690414));
#150948=CARTESIAN_POINT('Ctrl Pts',(3.24894279744353,4.56683176235996,6.52777914878455));
#150949=CARTESIAN_POINT('Ctrl Pts',(3.26740550851356,4.57355155122262,6.56512379933834));
#150950=CARTESIAN_POINT('Ctrl Pts',(3.30436815712275,4.58666922561447,6.63979640350505));
#150951=CARTESIAN_POINT('Ctrl Pts',(3.32288877939436,4.5930744447669,6.67716613756715));
#150952=CARTESIAN_POINT('Ctrl Pts',(3.3414257129925,4.5993304993971,6.71452710215876));
#150953=CARTESIAN_POINT('Origin',(-8.93903007170849E-12,4.78597145200196,
-1.72535596920653E-11));
#150954=CARTESIAN_POINT('',(3.17139962945521,4.74999999503922,6.79648618146043));
#150955=CARTESIAN_POINT('',(3.32900762991155,4.78575691070129,6.68076590640131));
#150956=CARTESIAN_POINT('Origin',(-1.38487057762148,4.80792772181027,0.438150558516112));
#150957=CARTESIAN_POINT('',(3.51345384874766,4.74999999648354,6.62613324541698));
#150958=CARTESIAN_POINT('Origin',(0.,4.74999999465775,0.));
#150959=CARTESIAN_POINT('Origin',(1.3130107249243,5.02638811558047,-0.633342583323322));
#150960=CARTESIAN_POINT('Ctrl Pts',(2.825748922,4.690053947,6.947311928));
#150961=CARTESIAN_POINT('Ctrl Pts',(3.204680937,4.624398499,6.79318516));
#150962=CARTESIAN_POINT('Ctrl Pts',(3.564601571,4.559170361,6.598758644));
#150963=CARTESIAN_POINT('Ctrl Pts',(2.509842609,4.690053947,6.801704939));
#150964=CARTESIAN_POINT('Ctrl Pts',(2.880832682,4.624398499,6.66480886600001));
#150965=CARTESIAN_POINT('Ctrl Pts',(3.234732564,4.559170361,6.488374622));
#150966=CARTESIAN_POINT('',(2.82574891932962,4.69005394803157,6.947311917114));
#150967=CARTESIAN_POINT('Origin',(-0.0716030411419838,4.69642565541896,
-0.178781440042297));
#150968=CARTESIAN_POINT('',(2.66779578238773,4.690053949938,6.87450842694637));
#150969=CARTESIAN_POINT('Origin',(2.90566182226115E-13,4.75090401457722,
5.6768825751341E-13));
#150970=CARTESIAN_POINT('Origin',(-0.0500682004489761,4.55370333648812,
-0.180848118809921));
#150971=CARTESIAN_POINT('Origin',(-0.0979257211822305,4.69643083360533,
-0.16634588287032));
#150972=CARTESIAN_POINT('Ctrl Pts',(1.57568526880443,4.559162772,7.33315098855785));
#150973=CARTESIAN_POINT('Ctrl Pts',(1.97567011474391,4.624819703,7.24720563832325));
#150974=CARTESIAN_POINT('Ctrl Pts',(2.36393408427073,4.690053947,7.11826545851253));
#150975=CARTESIAN_POINT('Ctrl Pts',(2.37736254220013,4.69231013188933,7.11380594664459));
#150976=CARTESIAN_POINT('Ctrl Pts',(2.39079100012952,4.69456631677851,7.10934643477668));
#150977=CARTESIAN_POINT('Ctrl Pts',(1.755159165,4.559162772,7.03433837));
#150978=CARTESIAN_POINT('Ctrl Pts',(2.138845352,4.624819703,6.938603662));
#150979=CARTESIAN_POINT('Ctrl Pts',(2.509842609,4.690053947,6.801704939));
#150980=CARTESIAN_POINT('Ctrl Pts',(2.52267388217639,4.6923101318893,6.79697017377152));
#150981=CARTESIAN_POINT('Ctrl Pts',(2.53550515535279,4.69456631677871,6.79223540854287));
#150982=CARTESIAN_POINT('',(2.36423562309891,4.69005394784373,7.11761127437326));
#150983=CARTESIAN_POINT('',(2.43703911643164,4.69005394666591,6.9596580948236));
#150984=CARTESIAN_POINT('',(1.81988018749594,4.59933049940976,7.27585294663606));
#150985=CARTESIAN_POINT('Origin',(-0.0392903036502423,4.55358394247595,
-0.187394020872271));
#150986=CARTESIAN_POINT('Ctrl Pts',(1.7597361460689,4.55994605590214,7.03319478750165));
#150987=CARTESIAN_POINT('Ctrl Pts',(1.76970476263088,4.56683176240597,7.07358996400831));
#150988=CARTESIAN_POINT('Ctrl Pts',(1.77970782980979,4.57355155128323,7.11403045441226));
#150989=CARTESIAN_POINT('Ctrl Pts',(1.79975390958325,4.58666922564794,7.19490313097691));
#150990=CARTESIAN_POINT('Ctrl Pts',(1.80980814176314,4.59307444476964,7.23538056743884));
#150991=CARTESIAN_POINT('Ctrl Pts',(1.81988018914646,4.59933049939345,7.27585294610767));
#150992=CARTESIAN_POINT('Origin',(2.55438031837585E-12,4.78597145199022,
1.08931960673964E-11));
#150993=CARTESIAN_POINT('',(1.63621045854496,4.74999999914954,7.31934528063922));
#150994=CARTESIAN_POINT('',(1.81501009377767,4.78575691086147,7.24021154754731));
#150995=CARTESIAN_POINT('Origin',(-1.4466932228166,4.80792715097801,0.130176519892637));
#150996=CARTESIAN_POINT('',(2.00688844986046,4.75000000041905,7.22650665538518));
#150997=CARTESIAN_POINT('Origin',(0.,4.75,0.));
#150998=CARTESIAN_POINT('Origin',(1.41846174566267,5.02638723621362,-0.336296958183587));
#150999=CARTESIAN_POINT('Ctrl Pts',(1.266217779,4.690053947,7.392340126));
#151000=CARTESIAN_POINT('Ctrl Pts',(1.669423273,4.624398499,7.323275938));
#151001=CARTESIAN_POINT('Ctrl Pts',(2.062725117,4.559170361,7.210767303));
#151002=CARTESIAN_POINT('Ctrl Pts',(0.988998379,4.690053947,7.182226828));
#151003=CARTESIAN_POINT('Ctrl Pts',(1.380743519,4.624398499,7.128283209));
#151004=CARTESIAN_POINT('Ctrl Pts',(1.764297565,4.559170361,7.032051913));
#151005=CARTESIAN_POINT('',(1.26621777864668,4.69005394803159,7.39234011460805));
#151006=CARTESIAN_POINT('Origin',(-0.0314962915716327,4.69642567960048,
-0.189994239868742));
#151007=CARTESIAN_POINT('',(1.12760809690174,4.690053949938,7.28728347422995));
#151008=CARTESIAN_POINT('Origin',(1.29453739394769E-13,4.74999999999889,
3.15719672627779E-13));
#151009=CARTESIAN_POINT('Origin',(-0.0100209414025748,4.55370519417284,
-0.187383212253678));
#151010=CARTESIAN_POINT('Origin',(-0.0598759400814782,4.69643089876513,
-0.183505306097708));
#151011=CARTESIAN_POINT('Ctrl Pts',(-0.0375640731032268,4.559162772,7.50043175008717));
#151012=CARTESIAN_POINT('Ctrl Pts',(0.371545059331102,4.624819703,7.50248067270269));
#151013=CARTESIAN_POINT('Ctrl Pts',(0.778449959937463,4.690053947,7.46002031826955));
#151014=CARTESIAN_POINT('Ctrl Pts',(0.792523131473887,4.69231013193289,
7.45855178876658));
#151015=CARTESIAN_POINT('Ctrl Pts',(0.806596303010307,4.69456631686565,
7.45708325926374));
#151016=CARTESIAN_POINT('Ctrl Pts',(0.201949703,4.559162772,7.247186786));
#151017=CARTESIAN_POINT('Ctrl Pts',(0.597245653,4.624819703,7.236171492));
#151018=CARTESIAN_POINT('Ctrl Pts',(0.988998379000001,4.690053947,7.182226828));
#151019=CARTESIAN_POINT('Ctrl Pts',(1.00254749896548,4.69231013193286,7.1803611033336));
#151020=CARTESIAN_POINT('Ctrl Pts',(1.01609661893097,4.69456631686583,7.17849537866705));
#151021=CARTESIAN_POINT('',(0.778885079207504,4.69005394784374,7.45944625051968));
#151022=CARTESIAN_POINT('',(0.883941732031887,4.69005394666591,7.32083652775466));
#151023=CARTESIAN_POINT('',(0.213239089478733,4.59933049939522,7.49696799334096));
#151024=CARTESIAN_POINT('Origin',(0.00191245021496908,4.55358395884049,
-0.191459008319693));
#151025=CARTESIAN_POINT('Ctrl Pts',(0.206665513682815,4.5599460557616,7.24705385412779));
#151026=CARTESIAN_POINT('Ctrl Pts',(0.207717300597014,4.56683176215896,
7.28864757151797));
#151027=CARTESIAN_POINT('Ctrl Pts',(0.208792991606958,4.5735515511746,7.33029295061067));
#151028=CARTESIAN_POINT('Ctrl Pts',(0.210985170295593,4.58666922554127,
7.41358418388105));
#151029=CARTESIAN_POINT('Ctrl Pts',(0.21210288780751,4.5930744447238,7.45527664356005));
#151030=CARTESIAN_POINT('Ctrl Pts',(0.213239091294778,4.59933049939587,
7.49696799329137));
#151031=CARTESIAN_POINT('Origin',(1.09604369308812E-13,4.78597145199218,
9.84672413051335E-12));
#151032=CARTESIAN_POINT('',(0.0245138913552423,4.74999999914955,7.49995993786108));
#151033=CARTESIAN_POINT('',(0.216144702052854,4.78575691069572,7.46111294405876));
#151034=CARTESIAN_POINT('Origin',(-1.44085448015335,4.80792622602611,-0.183864222010178));
#151035=CARTESIAN_POINT('',(0.40648319694277,4.75000000032292,7.48897663920438));
#151036=CARTESIAN_POINT('Origin',(0.,4.75,0.));
#151037=CARTESIAN_POINT('Origin',(1.45759308339514,5.02638715698334,-0.0235092780933521));
#151038=CARTESIAN_POINT('Ctrl Pts',(-0.3525203,4.690053947,7.491710715));
#151039=CARTESIAN_POINT('Ctrl Pts',(0.056105233,4.624398499,7.510938472));
#151040=CARTESIAN_POINT('Ctrl Pts',(0.464397928,4.559170361,7.485608497));
#151041=CARTESIAN_POINT('Ctrl Pts',(-0.578090317,4.690053947,7.226915773));
#151042=CARTESIAN_POINT('Ctrl Pts',(-0.183907677,4.624398499,7.258446951));
#151043=CARTESIAN_POINT('Ctrl Pts',(0.211365974,4.559170361,7.246918271));
#151044=CARTESIAN_POINT('',(-0.352520297877153,4.69005394803158,7.49171070388639));
#151045=CARTESIAN_POINT('Origin',(0.0100832141964853,4.69642563255268,-0.192323046541649));
#151046=CARTESIAN_POINT('',(-0.465305290421314,4.690053949938,7.35931324514306));
#151047=CARTESIAN_POINT('Origin',(4.69730591229345E-14,4.74999999999911,
1.17961196366423E-13));
#151048=CARTESIAN_POINT('Origin',(0.0304952220692588,4.55370501744875,-0.185156493585492));
#151049=CARTESIAN_POINT('Origin',(-0.0190278903796856,4.69643087780134,
-0.192086882849298));
#151050=CARTESIAN_POINT('Ctrl Pts',(0.438256130634989,1.20239769764516,
7.48776619102291));
#151051=CARTESIAN_POINT('Ctrl Pts',(0.452324716730529,1.20018543582258,
7.48688969052746));
#151052=CARTESIAN_POINT('Ctrl Pts',(0.46639330282608,1.197973174,7.48601319003203));
#151053=CARTESIAN_POINT('Ctrl Pts',(0.874198775531821,1.13384644,7.4606061095738));
#151054=CARTESIAN_POINT('Ctrl Pts',(1.27683106164612,1.068610636,7.39104990055959));
#151055=CARTESIAN_POINT('Ctrl Pts',(0.185550148104057,1.20239769764516,
7.24767643469913));
#151056=CARTESIAN_POINT('Ctrl Pts',(0.199169321052031,1.20018543582258,
7.24727653784951));
#151057=CARTESIAN_POINT('Ctrl Pts',(0.212788494,1.197973174,7.246876641));
#151058=CARTESIAN_POINT('Ctrl Pts',(0.607566848,1.13384644,7.235284849));
#151059=CARTESIAN_POINT('Ctrl Pts',(0.998749843,1.068610636,7.180877297));
#151060=CARTESIAN_POINT('',(0.994070539475332,1.06939092015758,7.18152655971494));
#151061=CARTESIAN_POINT('Origin',(-0.0464232246320195,0.946547068832668,
-0.186800079907797));
#151062=CARTESIAN_POINT('Ctrl Pts',(1.03018392039921,1.1083007626151,7.4289111642017));
#151063=CARTESIAN_POINT('Ctrl Pts',(1.02426895890853,1.10211922686966,7.38762652912021));
#151064=CARTESIAN_POINT('Ctrl Pts',(1.01830226328052,1.09579054188193,7.34634686826034));
#151065=CARTESIAN_POINT('Ctrl Pts',(1.00603423691539,1.08257775698825,7.26228722585719));
#151066=CARTESIAN_POINT('Ctrl Pts',(0.999993344786955,1.07598455113782,
7.2214109573584));
#151067=CARTESIAN_POINT('Ctrl Pts',(0.994070540471644,1.06939092064321,
7.18152656222649));
#151068=CARTESIAN_POINT('Ctrl Pts',(0.779321499,1.068630405,7.45940064599999));
#151069=CARTESIAN_POINT('Ctrl Pts',(0.788211976,1.070029867,7.458471813));
#151070=CARTESIAN_POINT('Ctrl Pts',(0.797100213,1.071428571,7.45752179));
#151071=CARTESIAN_POINT('Ctrl Pts',(1.195462099,1.134117105,7.41494272));
#151072=CARTESIAN_POINT('Ctrl Pts',(1.587021072,1.197973174,7.330168082));
#151073=CARTESIAN_POINT('Ctrl Pts',(0.989418578,1.068630405,7.182168954));
#151074=CARTESIAN_POINT('Ctrl Pts',(0.997978637,1.070029867,7.18098971600001));
#151075=CARTESIAN_POINT('Ctrl Pts',(1.00653586,1.071428571,7.179790078));
#151076=CARTESIAN_POINT('Ctrl Pts',(1.390062022,1.134117105,7.126023487));
#151077=CARTESIAN_POINT('Ctrl Pts',(1.76567788,1.197973174,7.031705456));
#151078=CARTESIAN_POINT('Origin',(-0.0687907708237448,1.33885358158439,
-0.178199474963884));
#151079=CARTESIAN_POINT('Ctrl Pts',(2.03765834002557,1.20239769750531,7.21849426533476));
#151080=CARTESIAN_POINT('Ctrl Pts',(2.05120958830638,1.20018543575265,7.21461392687758));
#151081=CARTESIAN_POINT('Ctrl Pts',(2.06476083658723,1.197973174,7.21073358842053));
#151082=CARTESIAN_POINT('Ctrl Pts',(2.45757027373109,1.13384644,7.09825438844889));
#151083=CARTESIAN_POINT('Ctrl Pts',(2.83583671227409,1.068610636,6.94377032609197));
#151084=CARTESIAN_POINT('Ctrl Pts',(1.73924828446017,1.20239769750532,7.03834198997261));
#151085=CARTESIAN_POINT('Ctrl Pts',(1.75246308223009,1.20018543575264,7.03502372298625));
#151086=CARTESIAN_POINT('Ctrl Pts',(1.76567788,1.197973174,7.031705456));
#151087=CARTESIAN_POINT('Ctrl Pts',(2.148734641,1.13384644,6.935518997));
#151088=CARTESIAN_POINT('Ctrl Pts',(2.519075981,1.068610636,6.798290683));
#151089=CARTESIAN_POINT('',(2.5146456483084,1.06939092019803,6.79993067800517));
#151090=CARTESIAN_POINT('Origin',(-0.085494427019141,0.946547140040651,
-0.172453402570524));
#151091=CARTESIAN_POINT('Ctrl Pts',(2.60309509616357,1.10830076263949,7.03376825860774));
#151092=CARTESIAN_POINT('Ctrl Pts',(2.58844344688322,1.10211922687875,6.99472037711221));
#151093=CARTESIAN_POINT('Ctrl Pts',(2.57374234231561,1.09579054188358,6.95568847492214));
#151094=CARTESIAN_POINT('Ctrl Pts',(2.54369085516861,1.08257778252019,6.87623151676588));
#151095=CARTESIAN_POINT('Ctrl Pts',(2.52900400578861,1.07598457750415,6.83760952313978));
#151096=CARTESIAN_POINT('Ctrl Pts',(2.5146456500351,1.06939092077411,6.79993068076175));
#151097=CARTESIAN_POINT('Ctrl Pts',(2.364652037,1.068630405,7.117472919));
#151098=CARTESIAN_POINT('Ctrl Pts',(2.373134987,1.070029867,7.114654611));
#151099=CARTESIAN_POINT('Ctrl Pts',(2.381611195,1.071428571,7.111816091));
#151100=CARTESIAN_POINT('Ctrl Pts',(2.76150636,1.134117105,6.984596466));
#151101=CARTESIAN_POINT('Ctrl Pts',(3.125686861,1.197973174,6.817630208));
#151102=CARTESIAN_POINT('Ctrl Pts',(2.510240543,1.068630405,6.801558087));
#151103=CARTESIAN_POINT('Ctrl Pts',(2.518346971,1.070029867,6.79856626));
#151104=CARTESIAN_POINT('Ctrl Pts',(2.526446244,1.071428571,6.795555119));
#151105=CARTESIAN_POINT('Ctrl Pts',(2.88944755,1.134117105,6.660598773));
#151106=CARTESIAN_POINT('Ctrl Pts',(3.236006129,1.197973174,6.487739539));
#151107=CARTESIAN_POINT('Origin',(-0.105490039867763,1.33885356374272,-0.15924516305883));
#151108=CARTESIAN_POINT('Ctrl Pts',(3.54178191010228,1.20239769752864,6.61169357039341));
#151109=CARTESIAN_POINT('Ctrl Pts',(3.55418217973039,1.20018543576431,6.60499083425077));
#151110=CARTESIAN_POINT('Ctrl Pts',(3.5665824493585,1.197973174,6.59828809810826));
#151111=CARTESIAN_POINT('Ctrl Pts',(3.9260285170885,1.13384644,6.4039961817453));
#151112=CARTESIAN_POINT('Ctrl Pts',(4.26224178946224,1.068610636,6.17180776755949));
#151113=CARTESIAN_POINT('Ctrl Pts',(3.2116211011738,1.20239769752864,6.49990249637725));
#151114=CARTESIAN_POINT('Ctrl Pts',(3.2238136150869,1.20018543576431,6.49382101768858));
#151115=CARTESIAN_POINT('Ctrl Pts',(3.236006129,1.197973174,6.487739539));
#151116=CARTESIAN_POINT('Ctrl Pts',(3.589429991,1.13384644,6.311455985));
#151117=CARTESIAN_POINT('Ctrl Pts',(3.921612925,1.068610636,6.097823552));
#151118=CARTESIAN_POINT('',(3.91763872170611,1.06939092016878,6.10037759559883));
#151119=CARTESIAN_POINT('Origin',(-0.120568015468822,0.946547110816421,
-0.150042782148584));
#151120=CARTESIAN_POINT('Ctrl Pts',(4.05428843853725,1.10830076263012,6.30973416640618));
#151121=CARTESIAN_POINT('Ctrl Pts',(4.03158519654434,1.10211922687914,6.27474887425661));
#151122=CARTESIAN_POINT('Ctrl Pts',(4.00883709045277,1.09579054186242,6.23978981908073));
#151123=CARTESIAN_POINT('Ctrl Pts',(3.96240709072474,1.08257772486597,6.16865039166828));
#151124=CARTESIAN_POINT('Ctrl Pts',(3.93976101702381,1.07598451458819,6.13408858623298));
#151125=CARTESIAN_POINT('Ctrl Pts',(3.91763872389687,1.06939092074616,6.10037759762989));
#151126=CARTESIAN_POINT('Ctrl Pts',(3.839414072,1.068630405,6.442740068));
#151127=CARTESIAN_POINT('Ctrl Pts',(3.847092844,1.070029867,6.438164067));
#151128=CARTESIAN_POINT('Ctrl Pts',(3.854760685,1.071428571,6.433569776));
#151129=CARTESIAN_POINT('Ctrl Pts',(4.198425653,1.134117105,6.227658244));
#151130=CARTESIAN_POINT('Ctrl Pts',(4.518199006,1.197973174,5.986307521));
#151131=CARTESIAN_POINT('Ctrl Pts',(3.91368645,1.068630405,6.10291392400001));
#151132=CARTESIAN_POINT('Ctrl Pts',(3.9209602,1.070029867,6.09824940200001));
#151133=CARTESIAN_POINT('Ctrl Pts',(3.928222811,1.071428571,6.093567555));
#151134=CARTESIAN_POINT('Ctrl Pts',(4.253725723,1.134117105,5.883731863));
#151135=CARTESIAN_POINT('Ctrl Pts',(4.555022329,1.197973174,5.640414132));
#151136=CARTESIAN_POINT('Origin',(-0.137256662328351,1.33885360303372,-0.132844741481347));
#151137=CARTESIAN_POINT('Ctrl Pts',(4.88029569482903,1.20239769749146,5.69573743188663));
#151138=CARTESIAN_POINT('Ctrl Pts',(4.89096516280296,1.20018543574573,5.68652571066418));
#151139=CARTESIAN_POINT('Ctrl Pts',(4.90163463077696,1.197973174,5.67731398944164));
#151140=CARTESIAN_POINT('Ctrl Pts',(5.21091003004155,1.13384644,5.41029423119707));
#151141=CARTESIAN_POINT('Ctrl Pts',(5.48934917737148,1.068610636,5.11125833880414));
#151142=CARTESIAN_POINT('Ctrl Pts',(4.53382208607388,1.20239769749146,5.65753478623849));
#151143=CARTESIAN_POINT('Ctrl Pts',(4.54442220753694,1.20018543574573,5.64897445911926));
#151144=CARTESIAN_POINT('Ctrl Pts',(4.555022329,1.197973174,5.640414132));
#151145=CARTESIAN_POINT('Ctrl Pts',(4.862287584,1.13384644,5.392276306));
#151146=CARTESIAN_POINT('Ctrl Pts',(5.140779607,1.068610636,5.112228969));
#151147=CARTESIAN_POINT('',(5.137447362684,1.06939092021347,5.11557763715341));
#151148=CARTESIAN_POINT('Origin',(-0.150003984783348,0.946547102134927,
-0.120616314865802));
#151149=CARTESIAN_POINT('Ctrl Pts',(5.31590775884627,1.10830076261777,5.290663917931));
#151150=CARTESIAN_POINT('Ctrl Pts',(5.28621450234346,1.10211922685411,5.26137708832615));
#151151=CARTESIAN_POINT('Ctrl Pts',(5.25648307089843,1.09579054184443,5.23212552680139));
#151152=CARTESIAN_POINT('Ctrl Pts',(5.1958457848372,1.08257774230565,5.17263045558175));
#151153=CARTESIAN_POINT('Ctrl Pts',(5.16629941641204,1.07598453760999,5.14374494207106));
#151154=CARTESIAN_POINT('Ctrl Pts',(5.13744736516035,1.06939092066855,5.11557763789017));
#151155=CARTESIAN_POINT('Ctrl Pts',(5.134649374,1.068630405,5.466751852));
#151156=CARTESIAN_POINT('Ctrl Pts',(5.141164914,1.070029867,5.460632127));
#151157=CARTESIAN_POINT('Ctrl Pts',(5.147665849,1.071428571,5.454496888));
#151158=CARTESIAN_POINT('Ctrl Pts',(5.439031228,1.134117105,5.179521645));
#151159=CARTESIAN_POINT('Ctrl Pts',(5.69944518700001,1.197973174,4.875071749));
#151160=CARTESIAN_POINT('Ctrl Pts',(5.134132729,1.068630405,5.118904289));
#151161=CARTESIAN_POINT('Ctrl Pts',(5.140233688,1.070029867,5.11278518));
#151162=CARTESIAN_POINT('Ctrl Pts',(5.146320044,1.071428571,5.106651545));
#151163=CARTESIAN_POINT('Ctrl Pts',(5.419104408,1.134117105,4.831748191));
#151164=CARTESIAN_POINT('Ctrl Pts',(5.661050747,1.197973174,4.529349229));
#151165=CARTESIAN_POINT('Ctrl Pts',(5.13412756255,1.068630405,5.11542581337));
#151166=CARTESIAN_POINT('Ctrl Pts',(5.14022437574001,1.070029867,5.10930671053001));
#151167=CARTESIAN_POINT('Ctrl Pts',(5.14630658595,1.071428571,5.10317309157));
#151168=CARTESIAN_POINT('Ctrl Pts',(5.4189051398,1.134117105,4.82827045646));
#151169=CARTESIAN_POINT('Ctrl Pts',(5.6606668026,1.197973174,4.5258920038));
#151170=CARTESIAN_POINT('Origin',(-0.162605461207993,1.33885360462888,-0.100232851893934));
#151171=CARTESIAN_POINT('Ctrl Pts',(6.00190831268338,1.19924836941368,4.49746179671395));
#151172=CARTESIAN_POINT('Ctrl Pts',(6.00434078984169,1.19861077170684,4.49420829285698));
#151173=CARTESIAN_POINT('Ctrl Pts',(6.006773267,1.197973174,4.490954789));
#151174=CARTESIAN_POINT('Ctrl Pts',(6.251420972,1.13384644,4.16373188));
#151175=CARTESIAN_POINT('Ctrl Pts',(6.459075062,1.068610636,3.811869534));
#151176=CARTESIAN_POINT('Ctrl Pts',(5.6561442008214,1.19924836941368,4.53548172299217));
#151177=CARTESIAN_POINT('Ctrl Pts',(5.6585974739107,1.19861077170684,4.53241547599609));
#151178=CARTESIAN_POINT('Ctrl Pts',(5.661050747,1.197973174,4.529349229));
#151179=CARTESIAN_POINT('Ctrl Pts',(5.907790014,1.13384644,4.22095978));
#151180=CARTESIAN_POINT('Ctrl Pts',(6.119569149,1.068610636,3.887592241));
#151181=CARTESIAN_POINT('',(6.11703467512529,1.06939092025812,3.89157895330992));
#151182=CARTESIAN_POINT('Origin',(-0.172425869117308,0.946547096142826,
-0.0855499160264561));
#151183=CARTESIAN_POINT('Ctrl Pts',(6.32896114107968,1.10830076259861,4.02420810481511));
#151184=CARTESIAN_POINT('Ctrl Pts',(6.29366629386755,1.10211922687242,4.00198915746824));
#151185=CARTESIAN_POINT('Ctrl Pts',(6.25834174588014,1.09579054191023,3.97981286015405));
#151186=CARTESIAN_POINT('Ctrl Pts',(6.18633291489277,1.08257782875722,3.93474426913298));
#151187=CARTESIAN_POINT('Ctrl Pts',(6.15126776956136,1.07598462355285,3.91288566099629));
#151188=CARTESIAN_POINT('Ctrl Pts',(6.11703467769023,1.06939092074784,3.89157895377656));
#151189=CARTESIAN_POINT('Ctrl Pts',(6.189794177,1.068630405,4.235144395));
#151190=CARTESIAN_POINT('Ctrl Pts',(6.194841828,1.070029867,4.227767098));
#151191=CARTESIAN_POINT('Ctrl Pts',(6.199871879,1.071428571,4.220377789));
#151192=CARTESIAN_POINT('Ctrl Pts',(6.425313749,1.134117105,3.889196369));
#151193=CARTESIAN_POINT('Ctrl Pts',(6.614191646,1.197973174,3.53588304));
#151194=CARTESIAN_POINT('Ctrl Pts',(6.114512667,1.068630405,3.895540379));
#151195=CARTESIAN_POINT('Ctrl Pts',(6.119155562,1.070029867,3.888252805));
#151196=CARTESIAN_POINT('Ctrl Pts',(6.123781072,1.071428571,3.880954185));
#151197=CARTESIAN_POINT('Ctrl Pts',(6.331091794,1.134117105,3.553837343));
#151198=CARTESIAN_POINT('Ctrl Pts',(6.502374724,1.197973174,3.20649699));
#151199=CARTESIAN_POINT('Ctrl Pts',(6.11375985189999,1.068630405,3.89214433884));
#151200=CARTESIAN_POINT('Ctrl Pts',(6.11839869934,1.070029867,3.88485766207));
#151201=CARTESIAN_POINT('Ctrl Pts',(6.12302016393,1.071428571,3.87755994896));
#151202=CARTESIAN_POINT('Ctrl Pts',(6.33014957445,1.134117105,3.55048375274));
#151203=CARTESIAN_POINT('Ctrl Pts',(6.50125655478,1.197973174,3.2032031295));
#151204=CARTESIAN_POINT('Origin',(-0.180351123912226,1.33885356480351,-0.0629342094144608));
#151205=CARTESIAN_POINT('Ctrl Pts',(6.82840837392086,1.19924836941368,3.10208076685929));
#151206=CARTESIAN_POINT('Ctrl Pts',(6.83008457396043,1.19861077170684,3.09838041742964));
#151207=CARTESIAN_POINT('Ctrl Pts',(6.83176077400001,1.197973174,3.094680068));
#151208=CARTESIAN_POINT('Ctrl Pts',(7.000345499,1.13384644,2.722515424));
#151209=CARTESIAN_POINT('Ctrl Pts',(7.127504748,1.068610636,2.334239933));
#151210=CARTESIAN_POINT('Ctrl Pts',(6.4989011950665,1.19924836941368,3.21354087208441));
#151211=CARTESIAN_POINT('Ctrl Pts',(6.50063795953325,1.19861077170684,3.2100189310422));
#151212=CARTESIAN_POINT('Ctrl Pts',(6.50237472400001,1.197973174,3.20649699));
#151213=CARTESIAN_POINT('Ctrl Pts',(6.677050749,1.13384644,2.852275866));
#151214=CARTESIAN_POINT('Ctrl Pts',(6.812214438,1.068610636,2.481176021));
#151215=CARTESIAN_POINT('',(6.81059624420825,1.06939092016605,2.48561436300061));
#151216=CARTESIAN_POINT('Origin',(-0.186785148316005,0.946547087643834,
-0.0464832497890674));
#151217=CARTESIAN_POINT('Ctrl Pts',(7.04607933419032,1.1083007625848,2.56958479291152));
#151218=CARTESIAN_POINT('Ctrl Pts',(7.00683324387316,1.10211922682975,2.55547266099491));
#151219=CARTESIAN_POINT('Ctrl Pts',(6.96756731588649,1.09579054187649,2.54140856685189));
#151220=CARTESIAN_POINT('Ctrl Pts',(6.88755313081598,1.08257775182071,2.5128732584833));
#151221=CARTESIAN_POINT('Ctrl Pts',(6.84860885007912,1.07598454567715,2.49906367012202));
#151222=CARTESIAN_POINT('Ctrl Pts',(6.81059624670237,1.06939092071402,2.48561436286733));
#151223=CARTESIAN_POINT('Ctrl Pts',(6.955511084,1.068630405,2.805506294));
#151224=CARTESIAN_POINT('Ctrl Pts',(6.958854823,1.070029867,2.797216377));
#151225=CARTESIAN_POINT('Ctrl Pts',(6.962178791,1.071428571,2.788918514));
#151226=CARTESIAN_POINT('Ctrl Pts',(7.11115573900001,1.134117105,2.417016594));
#151227=CARTESIAN_POINT('Ctrl Pts',(7.219665854,1.197973174,2.031360369));
#151228=CARTESIAN_POINT('Ctrl Pts',(6.808984789,1.068630405,2.49002533));
#151229=CARTESIAN_POINT('Ctrl Pts',(6.811952522,1.070029867,2.48191005));
#151230=CARTESIAN_POINT('Ctrl Pts',(6.814900903,1.071428571,2.47378772));
#151231=CARTESIAN_POINT('Ctrl Pts',(6.947044364,1.134117105,2.109753011));
#151232=CARTESIAN_POINT('Ctrl Pts',(7.039654886,1.197973174,1.733712515));
#151233=CARTESIAN_POINT('Origin',(-0.189663442092307,1.33885358139159,-0.0226926323759727));
#151234=CARTESIAN_POINT('Ctrl Pts',(7.33208299134599,1.20239769762439,1.5809079574551));
#151235=CARTESIAN_POINT('Ctrl Pts',(7.33500218475563,1.20018543581218,1.56711768275349));
#151236=CARTESIAN_POINT('Ctrl Pts',(7.33792137816545,1.197973174,1.55332740805189));
#151237=CARTESIAN_POINT('Ctrl Pts',(7.422539906702,1.13384644,1.15358933333221));
#151238=CARTESIAN_POINT('Ctrl Pts',(7.46323456897324,1.068610636,0.747024740058699));
#151239=CARTESIAN_POINT('Ctrl Pts',(7.03313849789318,1.20239769762439,1.76017199027748));
#151240=CARTESIAN_POINT('Ctrl Pts',(7.03639669194659,1.20018543581218,1.74694225263871));
#151241=CARTESIAN_POINT('Ctrl Pts',(7.039654886,1.197973174,1.733712515));
#151242=CARTESIAN_POINT('Ctrl Pts',(7.134100011,1.13384644,1.350222703));
#151243=CARTESIAN_POINT('Ctrl Pts',(7.186328152,1.068610636,0.958742768));
#151244=CARTESIAN_POINT('',(7.18570190259806,1.06939092016506,0.96342520766622));
#151245=CARTESIAN_POINT('Origin',(-0.192410959439872,0.94654712134076,-0.00524326309847709));
#151246=CARTESIAN_POINT('Ctrl Pts',(7.43373068926975,1.10830076258783,0.994810551909359));
#151247=CARTESIAN_POINT('Ctrl Pts',(7.39236845954229,1.10211922682979,0.989465103128043));
#151248=CARTESIAN_POINT('Ctrl Pts',(7.35099718228751,1.09579054181713,0.984170833502873));
#151249=CARTESIAN_POINT('Ctrl Pts',(7.26671952059379,1.08257776491292,0.973503360110995));
#151250=CARTESIAN_POINT('Ctrl Pts',(7.22571707860721,1.07598455880364,0.968388500652465));
#151251=CARTESIAN_POINT('Ctrl Pts',(7.18570190540487,1.06939092071891,0.963425207231068));
#151252=CARTESIAN_POINT('Ctrl Pts',(7.395996023,1.068630405,1.244685836));
#151253=CARTESIAN_POINT('Ctrl Pts',(7.3974795,1.070029867,1.235870928));
#151254=CARTESIAN_POINT('Ctrl Pts',(7.398941961,1.071428571,1.227052509));
#151255=CARTESIAN_POINT('Ctrl Pts',(7.464487991,1.134117105,0.83181981));
#151256=CARTESIAN_POINT('Ctrl Pts',(7.487556512,1.197973174,0.431853546));
#151257=CARTESIAN_POINT('Ctrl Pts',(7.18507635,1.068630405,0.968079464));
#151258=CARTESIAN_POINT('Ctrl Pts',(7.186230154,1.070029867,0.95951594));
#151259=CARTESIAN_POINT('Ctrl Pts',(7.187363542,1.071428571,0.95094969));
#151260=CARTESIAN_POINT('Ctrl Pts',(7.238160861,1.134117105,0.567018973000001));
#151261=CARTESIAN_POINT('Ctrl Pts',(7.247768609,1.197973174,0.17986157));
#151262=CARTESIAN_POINT('Origin',(-0.19010752046501,1.33885360244533,0.0186099469742334));
#151263=CARTESIAN_POINT('Ctrl Pts',(7.50051144518414,1.20239769728923,-0.032233902738517));
#151264=CARTESIAN_POINT('Ctrl Pts',(7.50039788805664,1.2001854356446,-0.0463293077195174));
#151265=CARTESIAN_POINT('Ctrl Pts',(7.50028433092912,1.197973174,-0.0604247127005174));
#151266=CARTESIAN_POINT('Ctrl Pts',(7.49699265531406,1.13384644,-0.469007616103169));
#151267=CARTESIAN_POINT('Ctrl Pts',(7.44933652902291,1.068610636,-0.87481510443479));
#151268=CARTESIAN_POINT('Ctrl Pts',(7.24709257550854,1.20239769728923,0.207103266246919));
#151269=CARTESIAN_POINT('Ctrl Pts',(7.24743059225433,1.2001854356446,0.193482418123463));
#151270=CARTESIAN_POINT('Ctrl Pts',(7.247768609,1.197973174,0.17986157));
#151271=CARTESIAN_POINT('Ctrl Pts',(7.257566686,1.13384644,-0.214965374));
#151272=CARTESIAN_POINT('Ctrl Pts',(7.224417148,1.068610636,-0.608520231));
#151273=CARTESIAN_POINT('',(7.22481212632975,1.06939092020671,-0.603812639258374));
#151274=CARTESIAN_POINT('Origin',(-0.189039560576042,0.946547077688595,
0.0362419940864935));
#151275=CARTESIAN_POINT('Ctrl Pts',(7.47378905908849,1.10830076262173,-0.626479925186409));
#151276=CARTESIAN_POINT('Ctrl Pts',(7.43224474213266,1.10211922691993,-0.622808743525731));
#151277=CARTESIAN_POINT('Ctrl Pts',(7.39070259099799,1.0957905419375,-0.61908563424013));
#151278=CARTESIAN_POINT('Ctrl Pts',(7.30610202034383,1.08257775218037,-0.611386494120737));
#151279=CARTESIAN_POINT('Ctrl Pts',(7.26495866855718,1.07598454873877,-0.607567458552055));
#151280=CARTESIAN_POINT('Ctrl Pts',(7.22481212871226,1.06939092068975,-0.603812640279786));
#151281=CARTESIAN_POINT('Ctrl Pts',(7.49065240800001,1.068630405,-0.374334748));
#151282=CARTESIAN_POINT('Ctrl Pts',(7.490206258,1.070029867,-0.383262472));
#151283=CARTESIAN_POINT('Ctrl Pts',(7.489738828,1.071428571,-0.392189107));
#151284=CARTESIAN_POINT('Ctrl Pts',(7.468789081,1.134117105,-0.792271945));
#151285=CARTESIAN_POINT('Ctrl Pts',(7.405337348,1.197973174,-1.187846269));
#151286=CARTESIAN_POINT('Ctrl Pts',(7.225201726,1.068630405,-0.599132722));
#151287=CARTESIAN_POINT('Ctrl Pts',(7.22448765000001,1.070029867,-0.607744069));
#151288=CARTESIAN_POINT('Ctrl Pts',(7.22375305,1.071428571,-0.616353689));
#151289=CARTESIAN_POINT('Ctrl Pts',(7.190829,1.134117105,-1.002228242));
#151290=CARTESIAN_POINT('Ctrl Pts',(7.116984728,1.197973174,-1.382399502));
#151291=CARTESIAN_POINT('Origin',(-0.181662547489728,1.33885359185878,0.0590423750210464));
#151292=CARTESIAN_POINT('Ctrl Pts',(7.31822431973493,1.20239769767987,-1.64386853669405));
#151293=CARTESIAN_POINT('Ctrl Pts',(7.31508332183255,1.20018543583992,-1.65760998871918));
#151294=CARTESIAN_POINT('Ctrl Pts',(7.31194232393021,1.197973174,-1.67135144074435));
#151295=CARTESIAN_POINT('Ctrl Pts',(7.22089435965082,1.13384644,-2.06967428973483));
#151296=CARTESIAN_POINT('Ctrl Pts',(7.08711579269105,1.068610636,-2.45574956582236));
#151297=CARTESIAN_POINT('Ctrl Pts',(7.12218065971982,1.20239769767987,-1.35564937192039));
#151298=CARTESIAN_POINT('Ctrl Pts',(7.11958269385989,1.20018543583992,-1.36902443696019));
#151299=CARTESIAN_POINT('Ctrl Pts',(7.116984728,1.197973174,-1.382399502));
#151300=CARTESIAN_POINT('Ctrl Pts',(7.041677609,1.13384644,-1.770101908));
#151301=CARTESIAN_POINT('Ctrl Pts',(6.92470042800001,1.068610636,-2.147329501));
#151302=CARTESIAN_POINT('',(6.92609816488622,1.06939092015861,-2.14281687848));
#151303=CARTESIAN_POINT('Origin',(-0.176829096809142,0.94654709502762,0.0760326273958178));
#151304=CARTESIAN_POINT('Ctrl Pts',(7.16438135887105,1.1083007626294,-2.2184768961222));
#151305=CARTESIAN_POINT('Ctrl Pts',(7.12459752024626,1.10211922688055,-2.20596074454325));
#151306=CARTESIAN_POINT('Ctrl Pts',(7.08482695982546,1.09579054186779,-2.19339434504393));
#151307=CARTESIAN_POINT('Ctrl Pts',(7.00385935976641,1.08257774698776,-2.16768857502555));
#151308=CARTESIAN_POINT('Ctrl Pts',(6.96449889675582,1.07598454333095,-2.15511422210605));
#151309=CARTESIAN_POINT('Ctrl Pts',(6.92609816709728,1.06939092067094,-2.14281688041309));
#151310=CARTESIAN_POINT('Ctrl Pts',(7.235054212,1.068630405,-1.975851855));
#151311=CARTESIAN_POINT('Ctrl Pts',(7.232699295,1.070029867,-1.984474945));
#151312=CARTESIAN_POINT('Ctrl Pts',(7.230323831,1.071428571,-1.993092396));
#151313=CARTESIAN_POINT('Ctrl Pts',(7.123857894,1.134117105,-2.379317943));
#151314=CARTESIAN_POINT('Ctrl Pts',(6.976852841,1.197973174,-2.752003713));
#151315=CARTESIAN_POINT('Ctrl Pts',(6.92748470000001,1.068630405,-2.138330128));
#151316=CARTESIAN_POINT('Ctrl Pts',(6.924936134,1.070029867,-2.146586641));
#151317=CARTESIAN_POINT('Ctrl Pts',(6.922367894,1.071428571,-2.154837056));
#151318=CARTESIAN_POINT('Ctrl Pts',(6.807261968,1.134117105,-2.524612378));
#151319=CARTESIAN_POINT('Ctrl Pts',(6.65341854999999,1.197973174,-2.88002111));
#151320=CARTESIAN_POINT('Origin',(-0.164722993209007,1.3388535646555,0.096714071594971));
#151321=CARTESIAN_POINT('Ctrl Pts',(6.79374515911296,1.20239769751311,-3.17863770865075));
#151322=CARTESIAN_POINT('Ctrl Pts',(6.78772359020847,1.20018543575654,-3.19138267096105));
#151323=CARTESIAN_POINT('Ctrl Pts',(6.78170202130389,1.197973174,-3.20412763327128));
#151324=CARTESIAN_POINT('Ctrl Pts',(6.60715506895362,1.13384644,-3.57356529384211));
#151325=CARTESIAN_POINT('Ctrl Pts',(6.39350939878208,1.068610636,-3.92185590761168));
#151326=CARTESIAN_POINT('Ctrl Pts',(6.66424349046516,1.20239769751311,-2.85501335574557));
#151327=CARTESIAN_POINT('Ctrl Pts',(6.65883102023257,1.20018543575654,-2.86751723287278));
#151328=CARTESIAN_POINT('Ctrl Pts',(6.65341855,1.197973174,-2.88002111));
#151329=CARTESIAN_POINT('Ctrl Pts',(6.49652751400001,1.13384644,-3.242470445));
#151330=CARTESIAN_POINT('Ctrl Pts',(6.301192412,1.068610636,-3.58573203));
#151331=CARTESIAN_POINT('',(6.30352755149462,1.06939092016514,-3.58162538195189));
#151332=CARTESIAN_POINT('Origin',(-0.156349827179958,0.946547120519208,
0.112267878198516));
#151333=CARTESIAN_POINT('Ctrl Pts',(6.51997514917062,1.10830076264153,-3.70674035357318));
#151334=CARTESIAN_POINT('Ctrl Pts',(6.48381203713835,1.10211922687683,-3.68596447338293));
#151335=CARTESIAN_POINT('Ctrl Pts',(6.44767269474452,1.09579054185558,-3.66514237449989));
#151336=CARTESIAN_POINT('Ctrl Pts',(6.37412364238196,1.08257767322355,-3.62263171337973));
#151337=CARTESIAN_POINT('Ctrl Pts',(6.33838650802529,1.07598446349883,-3.60188999851072));
#151338=CARTESIAN_POINT('Ctrl Pts',(6.30352755295668,1.06939092073101,-3.58162538425232));
#151339=CARTESIAN_POINT('Ctrl Pts',(6.641152922,1.068630405,-3.484980325));
#151340=CARTESIAN_POINT('Ctrl Pts',(6.636999353,1.070029867,-3.492895575));
#151341=CARTESIAN_POINT('Ctrl Pts',(6.632826928,1.071428571,-3.5008009));
#151342=CARTESIAN_POINT('Ctrl Pts',(6.44582303,1.134117105,-3.855109679));
#151343=CARTESIAN_POINT('Ctrl Pts',(6.222138449,1.197973174,-4.187480522));
#151344=CARTESIAN_POINT('Ctrl Pts',(6.30584618800001,1.068630405,-3.577541593));
#151345=CARTESIAN_POINT('Ctrl Pts',(6.3015823,1.070029867,-3.585057207));
#151346=CARTESIAN_POINT('Ctrl Pts',(6.297300509,1.071428571,-3.592562637));
#151347=CARTESIAN_POINT('Ctrl Pts',(6.105394932,1.134117105,-3.928948446));
#151348=CARTESIAN_POINT('Ctrl Pts',(5.878745916,1.197973174,-4.242976131));
#151349=CARTESIAN_POINT('Origin',(-0.14008082696896,1.33885358682711,0.129863289500041));
#151350=CARTESIAN_POINT('Ctrl Pts',(5.95159802469212,1.20239769753535,-4.56477731310792));
#151351=CARTESIAN_POINT('Ctrl Pts',(5.94297744652179,1.20018543576767,-4.57592984602739));
#151352=CARTESIAN_POINT('Ctrl Pts',(5.93435686835148,1.197973174,-4.58708237894685));
#151353=CARTESIAN_POINT('Ctrl Pts',(5.68447255026051,1.13384644,-4.91036035735012));
#151354=CARTESIAN_POINT('Ctrl Pts',(5.40094961069062,1.068610636,-5.20458062606933));
#151355=CARTESIAN_POINT('Ctrl Pts',(5.89469370340292,1.20239769753535,-4.22088008624134));
#151356=CARTESIAN_POINT('Ctrl Pts',(5.88671980970153,1.20018543576767,-4.23192810862066));
#151357=CARTESIAN_POINT('Ctrl Pts',(5.878745916,1.197973174,-4.242976131));
#151358=CARTESIAN_POINT('Ctrl Pts',(5.647607012,1.13384644,-4.563224667));
#151359=CARTESIAN_POINT('Ctrl Pts',(5.383047642,1.068610636,-4.85646971400001));
#151360=CARTESIAN_POINT('',(5.38621099464516,1.06939092021984,-4.85296106368719));
#151361=CARTESIAN_POINT('Origin',(-0.128560173579613,0.946547117492585,
0.143253706418039));
#151362=CARTESIAN_POINT('Ctrl Pts',(5.570702147441,1.10830076265064,-5.02168075233264));
#151363=CARTESIAN_POINT('Ctrl Pts',(5.5398507091389,1.10211922690085,-4.99361660052245));
#151364=CARTESIAN_POINT('Ctrl Pts',(5.50903242037416,1.09579054189062,-4.96551242031142));
#151365=CARTESIAN_POINT('Ctrl Pts',(5.44634166949059,1.0825777217037,-4.90818497254084));
#151366=CARTESIAN_POINT('Ctrl Pts',(5.41589892140718,1.07598451821939,-4.88024577480333));
#151367=CARTESIAN_POINT('Ctrl Pts',(5.38621099577857,1.06939092065068,-4.85296106598922));
#151368=CARTESIAN_POINT('Ctrl Pts',(5.736718702,1.068630405,-4.831154989));
#151369=CARTESIAN_POINT('Ctrl Pts',(5.730960697,1.070029867,-4.83799229));
#151370=CARTESIAN_POINT('Ctrl Pts',(5.72518641,1.071428571,-4.844815845));
#151371=CARTESIAN_POINT('Ctrl Pts',(5.46638864400001,1.134117105,-5.150640772));
#151372=CARTESIAN_POINT('Ctrl Pts',(5.176483778,1.197973174,-5.427155396));
#151373=CARTESIAN_POINT('Ctrl Pts',(5.38935331700001,1.068630405,-4.84947119));
#151374=CARTESIAN_POINT('Ctrl Pts',(5.383573482,1.070029867,-4.855894483));
#151375=CARTESIAN_POINT('Ctrl Pts',(5.377778351,1.071428571,-4.862303981));
#151376=CARTESIAN_POINT('Ctrl Pts',(5.118046414,1.134117105,-5.149571251));
#151377=CARTESIAN_POINT('Ctrl Pts',(4.829189657,1.197973174,-5.407534305));
#151378=CARTESIAN_POINT('Ctrl Pts',(5.38587966315001,1.068630405,-4.84965435201));
#151379=CARTESIAN_POINT('Ctrl Pts',(5.38009960985,1.070029867,-4.85607350493001));
#151380=CARTESIAN_POINT('Ctrl Pts',(5.37430427041,1.071428571,-4.86247886236));
#151381=CARTESIAN_POINT('Ctrl Pts',(5.1145629917,1.134117105,-5.14956055579));
#151382=CARTESIAN_POINT('Ctrl Pts',(4.82571671579,1.197973174,-5.40733809408999));
#151383=CARTESIAN_POINT('Origin',(-0.108889318598229,1.33885360151785,0.156940670213082));
#151384=CARTESIAN_POINT('Ctrl Pts',(4.83116078180512,1.20239769737794,-5.7374730039056));
#151385=CARTESIAN_POINT('Ctrl Pts',(4.82034428343836,1.20018543568896,-5.74651162701026));
#151386=CARTESIAN_POINT('Ctrl Pts',(4.80952778507171,1.197973174,-5.75555025011497));
#151387=CARTESIAN_POINT('Ctrl Pts',(4.49599041422966,1.13384644,-6.01755242754882));
#151388=CARTESIAN_POINT('Ctrl Pts',(4.15584742240734,1.068610636,-6.24394493863673));
#151389=CARTESIAN_POINT('Ctrl Pts',(4.84951458976677,1.20239769737794,-5.38938315709937));
#151390=CARTESIAN_POINT('Ctrl Pts',(4.83935212338343,1.20018543568896,-5.39845873104967));
#151391=CARTESIAN_POINT('Ctrl Pts',(4.829189657,1.197973174,-5.40753430500001));
#151392=CARTESIAN_POINT('Ctrl Pts',(4.53461068300001,1.13384644,-5.670607575));
#151393=CARTESIAN_POINT('Ctrl Pts',(4.213197547,1.068610636,-5.900124272));
#151394=CARTESIAN_POINT('',(4.21704119835776,1.0693909201585,-5.89737767934635));
#151395=CARTESIAN_POINT('Origin',(-0.0947593468883695,0.946547132636281,
0.167541350843304));
#151396=CARTESIAN_POINT('Ctrl Pts',(4.36094930547041,1.10830076259365,-6.10181293976727));
#151397=CARTESIAN_POINT('Ctrl Pts',(4.33685211954456,1.10211922683968,-6.06777276493754));
#151398=CARTESIAN_POINT('Ctrl Pts',(4.31279591317227,1.09579054185722,-6.03370062390097));
#151399=CARTESIAN_POINT('Ctrl Pts',(4.26389471363875,1.08257776763097,-5.96423704338925));
#151400=CARTESIAN_POINT('Ctrl Pts',(4.24016977757793,1.07598455995295,-5.93040672750791));
#151401=CARTESIAN_POINT('Ctrl Pts',(4.21704119895221,1.06939092065416,-5.89737768176648));
#151402=CARTESIAN_POINT('Ctrl Pts',(4.564041892,1.068630405,-5.951430215));
#151403=CARTESIAN_POINT('Ctrl Pts',(4.556948688,1.070029867,-5.956869862));
#151404=CARTESIAN_POINT('Ctrl Pts',(4.549842538,1.071428571,-5.962292586));
#151405=CARTESIAN_POINT('Ctrl Pts',(4.231352001,1.134117105,-6.205333626));
#151406=CARTESIAN_POINT('Ctrl Pts',(3.88878248,1.197973174,-6.413062515));
#151407=CARTESIAN_POINT('Ctrl Pts',(4.220860275,1.068630405,-5.894644903));
#151408=CARTESIAN_POINT('Ctrl Pts',(4.213834751,1.070029867,-5.89967553));
#151409=CARTESIAN_POINT('Ctrl Pts',(4.206797255,1.071428571,-5.904689396));
#151410=CARTESIAN_POINT('Ctrl Pts',(3.891383734,1.134117105,-6.129405827));
#151411=CARTESIAN_POINT('Ctrl Pts',(3.553825856,1.197973174,-6.319242184));
#151412=CARTESIAN_POINT('Origin',(-0.0726058415674252,1.33885357944252,
0.176679306747297));
#151413=CARTESIAN_POINT('Ctrl Pts',(3.48482382869069,1.20239769722685,-6.64189083359813));
#151414=CARTESIAN_POINT('Ctrl Pts',(3.47231717767815,1.20018543561341,-6.64839291107468));
#151415=CARTESIAN_POINT('Ctrl Pts',(3.4598105266656,1.197973174,-6.65489498855133));
#151416=CARTESIAN_POINT('Ctrl Pts',(3.09728076171842,1.13384644,-6.84337043388931));
#151417=CARTESIAN_POINT('Ctrl Pts',(2.71642242712733,1.068610636,-6.99134932534094));
#151418=CARTESIAN_POINT('Ctrl Pts',(3.57757756258052,1.20239769722685,-6.30588466001074));
#151419=CARTESIAN_POINT('Ctrl Pts',(3.56570170929029,1.20018543561341,-6.31256342200547));
#151420=CARTESIAN_POINT('Ctrl Pts',(3.553825856,1.197973174,-6.319242184));
#151421=CARTESIAN_POINT('Ctrl Pts',(3.209580998,1.13384644,-6.512839176));
#151422=CARTESIAN_POINT('Ctrl Pts',(2.846343018,1.068610636,-6.66789557700001));
#151423=CARTESIAN_POINT('',(2.85068724288564,1.06939092013848,-6.66603946941679));
#151424=CARTESIAN_POINT('Origin',(-0.0565274918814662,0.946547102750439,
0.183994782434302));
#151425=CARTESIAN_POINT('Ctrl Pts',(2.94728332000656,1.10830076261339,-6.89663113609631));
#151426=CARTESIAN_POINT('Ctrl Pts',(2.93106714437848,1.10211922686252,-6.85820661904387));
#151427=CARTESIAN_POINT('Ctrl Pts',(2.91489786188007,1.09579054182493,-6.81975969218544));
#151428=CARTESIAN_POINT('Ctrl Pts',(2.88207248594303,1.08257773698977,-6.74140763778961));
#151429=CARTESIAN_POINT('Ctrl Pts',(2.86617475262665,1.07598453111424,-6.70326811364963));
#151430=CARTESIAN_POINT('Ctrl Pts',(2.8506872430964,1.06939092063435,-6.66603947211695));
#151431=CARTESIAN_POINT('Ctrl Pts',(3.177955556,1.068630405,-6.79342317900001));
#151432=CARTESIAN_POINT('Ctrl Pts',(3.169858824,1.070029867,-6.797210821));
#151433=CARTESIAN_POINT('Ctrl Pts',(3.161753086,1.071428571,-6.800979152));
#151434=CARTESIAN_POINT('Ctrl Pts',(2.798462042,1.134117105,-6.969871977));
#151435=CARTESIAN_POINT('Ctrl Pts',(2.419246034,1.197973174,-7.099101959));
#151436=CARTESIAN_POINT('Ctrl Pts',(2.855004498,1.068630405,-6.664191573));
#151437=CARTESIAN_POINT('Ctrl Pts',(2.84706179,1.070029867,-6.667594306));
#151438=CARTESIAN_POINT('Ctrl Pts',(2.839110994,1.071428571,-6.670978097));
#151439=CARTESIAN_POINT('Ctrl Pts',(2.482764276,1.134117105,-6.8226362));
#151440=CARTESIAN_POINT('Ctrl Pts',(2.112289109,1.197973174,-6.935469322));
#151441=CARTESIAN_POINT('Origin',(-0.0329275030577136,1.33885361190165,
0.188156703710749));
#151442=CARTESIAN_POINT('Ctrl Pts',(1.95650203590071,1.19924836941368,-7.24031531054044));
#151443=CARTESIAN_POINT('Ctrl Pts',(1.95257925395036,1.19861077170684,-7.24137077927022));
#151444=CARTESIAN_POINT('Ctrl Pts',(1.948656472,1.197973174,-7.242426248));
#151445=CARTESIAN_POINT('Ctrl Pts',(1.554120557,1.13384644,-7.348580586));
#151446=CARTESIAN_POINT('Ctrl Pts',(1.150387927,1.068610636,-7.411248722));
#151447=CARTESIAN_POINT('Ctrl Pts',(2.11980215310686,1.19924836941368,-6.93318112482194));
#151448=CARTESIAN_POINT('Ctrl Pts',(2.11604563105343,1.19861077170684,-6.93432522341097));
#151449=CARTESIAN_POINT('Ctrl Pts',(2.112289109,1.197973174,-6.93546932199999));
#151450=CARTESIAN_POINT('Ctrl Pts',(1.734474873,1.13384644,-7.050537656));
#151451=CARTESIAN_POINT('Ctrl Pts',(1.346396652,1.068610636,-7.123883495));
#151452=CARTESIAN_POINT('',(1.35103832001002,1.06939092016804,-7.12300466238269));
#151453=CARTESIAN_POINT('Origin',(-0.0156524015825424,0.946547090581574,
0.191844575304695));
#151454=CARTESIAN_POINT('Ctrl Pts',(1.39580564292765,1.10830076261233,-7.36897052522762));
#151455=CARTESIAN_POINT('Ctrl Pts',(1.3882287277522,1.10211922684992,-7.32795835342687));
#151456=CARTESIAN_POINT('Ctrl Pts',(1.38070242688305,1.0957905418705,-7.28693437682775));
#151457=CARTESIAN_POINT('Ctrl Pts',(1.36548790457744,1.08257777103923,-7.20335787924211));
#151458=CARTESIAN_POINT('Ctrl Pts',(1.35816072347702,1.07598456880958,-7.16269250412706));
#151459=CARTESIAN_POINT('Ctrl Pts',(1.35103831922291,1.06939092063558,-7.12300466481012));
#151460=CARTESIAN_POINT('Ctrl Pts',(1.64327155,1.068630405,-7.317763225));
#151461=CARTESIAN_POINT('Ctrl Pts',(1.634549884,1.070029867,-7.319721756));
#151462=CARTESIAN_POINT('Ctrl Pts',(1.625823574,1.071428571,-7.321659491));
#151463=CARTESIAN_POINT('Ctrl Pts',(1.234719107,1.134117105,-7.40850686));
#151464=CARTESIAN_POINT('Ctrl Pts',(0.836588333,1.197973174,-7.453195285));
#151465=CARTESIAN_POINT('Ctrl Pts',(1.355651883,1.068630405,-7.12212805100001));
#151466=CARTESIAN_POINT('Ctrl Pts',(1.347163385,1.070029867,-7.12374378300001));
#151467=CARTESIAN_POINT('Ctrl Pts',(1.338671059,1.071428571,-7.125339276));
#151468=CARTESIAN_POINT('Ctrl Pts',(0.95805352,1.134117105,-7.196847686));
#151469=CARTESIAN_POINT('Ctrl Pts',(0.57198407,1.197973174,-7.227401623));
#151470=CARTESIAN_POINT('Origin',(0.00829042140507816,1.33885358366507,
0.190836349482981));
#151471=CARTESIAN_POINT('Ctrl Pts',(0.356511060962697,1.19962221840631,
-7.49172613854189));
#151472=CARTESIAN_POINT('Ctrl Pts',(0.351263280142558,1.19879769620315,
-7.49196849872099));
#151473=CARTESIAN_POINT('Ctrl Pts',(0.346015499322418,1.197973174,-7.4922108589001));
#151474=CARTESIAN_POINT('Ctrl Pts',(-0.0621275967109266,1.13384644,-7.51106028063581));
#151475=CARTESIAN_POINT('Ctrl Pts',(-0.469903043622183,1.068610636,-7.48546200380075));
#151476=CARTESIAN_POINT('Ctrl Pts',(0.582108670146463,1.19962221840631,
-7.22660035162996));
#151477=CARTESIAN_POINT('Ctrl Pts',(0.577046370073232,1.19879769620315,
-7.22700098731498));
#151478=CARTESIAN_POINT('Ctrl Pts',(0.57198407,1.197973174,-7.227401623));
#151479=CARTESIAN_POINT('Ctrl Pts',(0.178266631,1.13384644,-7.25856083));
#151480=CARTESIAN_POINT('Ctrl Pts',(-0.216505724,1.068610636,-7.246766539));
#151481=CARTESIAN_POINT('',(-0.211783652922205,1.06939092018228,-7.2469060743844));
#151482=CARTESIAN_POINT('Origin',(0.0259544467068482,0.946547088024064,
0.190724426768872));
#151483=CARTESIAN_POINT('Ctrl Pts',(-0.220938355623848,1.10830076264133,
-7.4967450430742));
#151484=CARTESIAN_POINT('Ctrl Pts',(-0.219521722060894,1.10211922691222,
-7.4550629005387));
#151485=CARTESIAN_POINT('Ctrl Pts',(-0.218053119813245,1.09579054189136,
-7.41338010930192));
#151486=CARTESIAN_POINT('Ctrl Pts',(-0.214945473836777,1.08257783683062,
-7.32848733402096));
#151487=CARTESIAN_POINT('Ctrl Pts',(-0.213359497213835,1.07598463444262,
-7.28719754505322));
#151488=CARTESIAN_POINT('Ctrl Pts',(-0.211783654082421,1.06939092059991,
-7.24690607660022));
#151489=CARTESIAN_POINT('Ctrl Pts',(0.031749992,1.068630405,-7.499932796));
#151490=CARTESIAN_POINT('Ctrl Pts',(0.022811208,1.070029867,-7.499970637));
#151491=CARTESIAN_POINT('Ctrl Pts',(0.013872358,1.071428571,-7.499987171));
#151492=CARTESIAN_POINT('Ctrl Pts',(-0.38675792,1.134117105,-7.500728197));
#151493=CARTESIAN_POINT('Ctrl Pts',(-0.785187309,1.197973174,-7.458785484));
#151494=CARTESIAN_POINT('Ctrl Pts',(-0.207089507,1.068630405,-7.247041737));
#151495=CARTESIAN_POINT('Ctrl Pts',(-0.215726884,1.070029867,-7.246794918));
#151496=CARTESIAN_POINT('Ctrl Pts',(-0.224363648,1.071428571,-7.24652751));
#151497=CARTESIAN_POINT('Ctrl Pts',(-0.611454754,1.134117105,-7.234542573));
#151498=CARTESIAN_POINT('Ctrl Pts',(-0.995066308,1.197973174,-7.181388657));
#151499=CARTESIAN_POINT('Ctrl Pts',(-0.20947790199,1.068630405,-7.24451282641));
#151500=CARTESIAN_POINT('Ctrl Pts',(-0.21811226492,1.070029867,-7.24426316081));
#151501=CARTESIAN_POINT('Ctrl Pts',(-0.22674600806,1.071428571,-7.24399291339));
#151502=CARTESIAN_POINT('Ctrl Pts',(-0.61370172234,1.134117105,-7.23188071676));
#151503=CARTESIAN_POINT('Ctrl Pts',(-0.997165097989999,1.197973174,-7.17861468873));
#151504=CARTESIAN_POINT('Origin',(0.049120771256816,1.33885359098496,0.184592545852338));
#151505=CARTESIAN_POINT('Ctrl Pts',(-1.24525698666216,1.20239769734986,
-7.39648876232056));
#151506=CARTESIAN_POINT('Ctrl Pts',(-1.25914833481224,1.20018543567492,
-7.39409631833717));
#151507=CARTESIAN_POINT('Ctrl Pts',(-1.27303968296231,1.197973174,-7.39170387435364));
#151508=CARTESIAN_POINT('Ctrl Pts',(-1.6757075941863,1.13384644,-7.32235420352542));
#151509=CARTESIAN_POINT('Ctrl Pts',(-2.06845928399246,1.068610636,-7.20967352818163));
#151510=CARTESIAN_POINT('Ctrl Pts',(-0.968074109179946,1.20239769734986,
-7.18512874527744));
#151511=CARTESIAN_POINT('Ctrl Pts',(-0.981570208589966,1.20018543567492,
-7.1832587011387));
#151512=CARTESIAN_POINT('Ctrl Pts',(-0.995066308,1.197973174,-7.181388657));
#151513=CARTESIAN_POINT('Ctrl Pts',(-1.386277161,1.13384644,-7.127181768));
#151514=CARTESIAN_POINT('Ctrl Pts',(-1.769284534,1.068610636,-7.030798834));
#151515=CARTESIAN_POINT('',(-1.76470285746994,1.06939092017545,-7.03195021220936));
#151516=CARTESIAN_POINT('Origin',(0.0663477542199706,0.94654708250684,0.180685933335545));
#151517=CARTESIAN_POINT('Ctrl Pts',(-1.82735152120739,1.10830076259602,
-7.27398009430452));
#151518=CARTESIAN_POINT('Ctrl Pts',(-1.81700757923931,1.10211922682501,
-7.23357699113942));
#151519=CARTESIAN_POINT('Ctrl Pts',(-1.80661274423284,1.0957905418318,-7.19318442661767));
#151520=CARTESIAN_POINT('Ctrl Pts',(-1.78532807882825,1.08257768947031,
-7.11094353236947));
#151521=CARTESIAN_POINT('Ctrl Pts',(-1.77490309665638,1.07598448114017,
-7.07096002344486));
#151522=CARTESIAN_POINT('Ctrl Pts',(-1.76470285889488,1.06939092077265,
-7.0319502149922));
#151523=CARTESIAN_POINT('Ctrl Pts',(-1.581256159,1.068630405,-7.331413844));
#151524=CARTESIAN_POINT('Ctrl Pts',(-1.589994095,1.070029867,-7.329529226));
#151525=CARTESIAN_POINT('Ctrl Pts',(-1.598727514,1.071428571,-7.327623785));
#151526=CARTESIAN_POINT('Ctrl Pts',(-1.990150577,1.134117105,-7.242223819));
#151527=CARTESIAN_POINT('Ctrl Pts',(-2.370248465,1.197973174,-7.115611162));
#151528=CARTESIAN_POINT('Ctrl Pts',(-1.760147621,1.068630405,-7.033091806));
#151529=CARTESIAN_POINT('Ctrl Pts',(-1.768530002,1.070029867,-7.030993976));
#151530=CARTESIAN_POINT('Ctrl Pts',(-1.776907359,1.071428571,-7.028876172));
#151531=CARTESIAN_POINT('Ctrl Pts',(-2.152372083,1.134117105,-6.933958291));
#151532=CARTESIAN_POINT('Ctrl Pts',(-2.515588492,1.197973174,-6.799581939));
#151533=CARTESIAN_POINT('Origin',(0.0876542312126244,1.33885357285475,0.169717188211986));
#151534=CARTESIAN_POINT('Ctrl Pts',(-2.80617001522815,1.20239769740834,
-6.95586952263931));
#151535=CARTESIAN_POINT('Ctrl Pts',(-2.81922228681214,1.20018543570416,
-6.95054678334448));
#151536=CARTESIAN_POINT('Ctrl Pts',(-2.83227455839611,1.197973174,-6.94522404404955));
#151537=CARTESIAN_POINT('Ctrl Pts',(-3.21062018829537,1.13384644,-6.79093403112974));
#151538=CARTESIAN_POINT('Ctrl Pts',(-3.56996654686197,1.068610636,-6.59645776536835));
#151539=CARTESIAN_POINT('Ctrl Pts',(-2.49003136393391,1.20239769740834,
-6.80903711112478));
#151540=CARTESIAN_POINT('Ctrl Pts',(-2.50280992796696,1.20018543570416,
-6.80430952506239));
#151541=CARTESIAN_POINT('Ctrl Pts',(-2.515588492,1.197973174,-6.799581939));
#151542=CARTESIAN_POINT('Ctrl Pts',(-2.886000173,1.13384644,-6.662543607));
#151543=CARTESIAN_POINT('Ctrl Pts',(-3.239333565,1.068610636,-6.486078789));
#151544=CARTESIAN_POINT('',(-3.23510651809109,1.06939092015702,-6.48818817439076));
#151545=CARTESIAN_POINT('Origin',(0.103638799473554,0.946547093860595,0.162198973411954));
#151546=CARTESIAN_POINT('Ctrl Pts',(-3.348319761214,1.10830076258882,-6.71109192096732));
#151547=CARTESIAN_POINT('Ctrl Pts',(-3.329532181977,1.10211922683441,-6.6738570618238));
#151548=CARTESIAN_POINT('Ctrl Pts',(-3.31069716493209,1.09579054181929,
-6.63664343517178));
#151549=CARTESIAN_POINT('Ctrl Pts',(-3.2722309301523,1.08257774728062,-6.560901192623));
#151550=CARTESIAN_POINT('Ctrl Pts',(-3.25345441216452,1.07598454419332,
-6.52409355055558));
#151551=CARTESIAN_POINT('Ctrl Pts',(-3.23510652026311,1.06939092068502,
-6.48818817582034));
#151552=CARTESIAN_POINT('Ctrl Pts',(-3.120324531,1.068630405,-6.82008613));
#151553=CARTESIAN_POINT('Ctrl Pts',(-3.128453041,1.070029867,-6.816367176));
#151554=CARTESIAN_POINT('Ctrl Pts',(-3.136572664,1.071428571,-6.812628856));
#151555=CARTESIAN_POINT('Ctrl Pts',(-3.500486005,1.134117105,-6.64508110500001));
#151556=CARTESIAN_POINT('Ctrl Pts',(-3.844479437,1.197973174,-6.43971877199999));
#151557=CARTESIAN_POINT('Ctrl Pts',(-3.23090319,1.068630405,-6.490282319));
#151558=CARTESIAN_POINT('Ctrl Pts',(-3.238638624,1.070029867,-6.486431571));
#151559=CARTESIAN_POINT('Ctrl Pts',(-3.246364857,1.071428571,-6.482562396));
#151560=CARTESIAN_POINT('Ctrl Pts',(-3.592646886,1.134117105,-6.30914982500001));
#151561=CARTESIAN_POINT('Ctrl Pts',(-3.918484554,1.197973174,-6.099834326));
#151562=CARTESIAN_POINT('Origin',(0.122089194624269,1.33885354582984,0.146906389843944));
#151563=CARTESIAN_POINT('Ctrl Pts',(-4.23586965189261,1.2023976974972,-6.19000155562014));
#151564=CARTESIAN_POINT('Ctrl Pts',(-4.24747253727115,1.20018543574859,
-6.18199740627892));
#151565=CARTESIAN_POINT('Ctrl Pts',(-4.25907542264976,1.197973174,-6.17399325693772));
#151566=CARTESIAN_POINT('Ctrl Pts',(-4.59540775076638,1.13384644,-5.9419773320462));
#151567=CARTESIAN_POINT('Ctrl Pts',(-4.90454614294094,1.068610636,-5.67479896766707));
#151568=CARTESIAN_POINT('Ctrl Pts',(-3.89555751945189,1.2023976974972,-6.11456246881635));
#151569=CARTESIAN_POINT('Ctrl Pts',(-3.90702103672596,1.20018543574859,
-6.10719839740816));
#151570=CARTESIAN_POINT('Ctrl Pts',(-3.918484554,1.197973174,-6.099834326));
#151571=CARTESIAN_POINT('Ctrl Pts',(-4.250777025,1.13384644,-5.886372312));
#151572=CARTESIAN_POINT('Ctrl Pts',(-4.557914959,1.068610636,-5.638076909));
#151573=CARTESIAN_POINT('',(-4.5542401936933,1.0693909201846,-5.64104566757719));
#151574=CARTESIAN_POINT('Origin',(0.136083798206407,0.946547087754226,0.136127620145601));
#151575=CARTESIAN_POINT('Ctrl Pts',(-4.71272429052064,1.10830076262936,
-5.83440054806072));
#151576=CARTESIAN_POINT('Ctrl Pts',(-4.68637156050134,1.10211922689068,
-5.80207499348866));
#151577=CARTESIAN_POINT('Ctrl Pts',(-4.65997706604311,1.09579054187506,
-5.76978037268462));
#151578=CARTESIAN_POINT('Ctrl Pts',(-4.60612778559715,1.08257774199474,
-5.70407801871414));
#151579=CARTESIAN_POINT('Ctrl Pts',(-4.57987769066149,1.07598453679128,
-5.67216730677154));
#151580=CARTESIAN_POINT('Ctrl Pts',(-4.55424019597839,1.06939092069683,
-5.64104566923627));
#151581=CARTESIAN_POINT('Ctrl Pts',(-4.513489995,1.068630405,-5.989858769));
#151582=CARTESIAN_POINT('Ctrl Pts',(-4.520629,1.070029867,-5.98447937200001));
#151583=CARTESIAN_POINT('Ctrl Pts',(-4.527755162,1.071428571,-5.979082973));
#151584=CARTESIAN_POINT('Ctrl Pts',(-4.847142598,1.134117105,-5.737221784));
#151585=CARTESIAN_POINT('Ctrl Pts',(-5.138946823,1.197973174,-5.462712289));
#151586=CARTESIAN_POINT('Ctrl Pts',(-4.550585316,1.068630405,-5.643994444));
#151587=CARTESIAN_POINT('Ctrl Pts',(-4.557312103,1.070029867,-5.638570835));
#151588=CARTESIAN_POINT('Ctrl Pts',(-4.564025943,1.071428571,-5.633131207));
#151589=CARTESIAN_POINT('Ctrl Pts',(-4.864933514,1.134117105,-5.389332525));
#151590=CARTESIAN_POINT('Ctrl Pts',(-5.138156632,1.197973174,-5.11486524));
#151591=CARTESIAN_POINT('Origin',(0.150815306188561,1.33885361766223,0.117226161007045));
#151592=CARTESIAN_POINT('Ctrl Pts',(-5.46750473373431,1.20239769723693,
-5.13469599369841));
#151593=CARTESIAN_POINT('Ctrl Pts',(-5.47711569402266,1.20018543561845,
-5.1243847001737));
#151594=CARTESIAN_POINT('Ctrl Pts',(-5.48672665431106,1.197973174,-5.11407340664884));
#151595=CARTESIAN_POINT('Ctrl Pts',(-5.76531915384119,1.13384644,-4.81518037720383));
#151596=CARTESIAN_POINT('Ctrl Pts',(-6.00979461161303,1.068610636,-4.48779287854149));
#151597=CARTESIAN_POINT('Ctrl Pts',(-5.11893173515577,1.20239769723692,
-5.13417768056049));
#151598=CARTESIAN_POINT('Ctrl Pts',(-5.12854418357785,1.20018543561845,
-5.12452146028024));
#151599=CARTESIAN_POINT('Ctrl Pts',(-5.138156632,1.197973174,-5.11486524));
#151600=CARTESIAN_POINT('Ctrl Pts',(-5.416792268,1.13384644,-4.834960791));
#151601=CARTESIAN_POINT('Ctrl Pts',(-5.663373315,1.068610636,-4.526444819));
#151602=CARTESIAN_POINT('',(-5.66042265901186,1.06939092020276,-4.53013413550935));
#151603=CARTESIAN_POINT('Origin',(0.162165348725155,0.946547092345618,0.103690775807711));
#151604=CARTESIAN_POINT('Ctrl Pts',(-5.85676706945754,1.10830076259221,
-4.68489909035697));
#151605=CARTESIAN_POINT('Ctrl Pts',(-5.82408141295832,1.10211922686147,
-4.65899434735455));
#151606=CARTESIAN_POINT('Ctrl Pts',(-5.7913616184495,1.0957905418823,-4.63312879310499));
#151607=CARTESIAN_POINT('Ctrl Pts',(-5.72464727544109,1.08257774895735,
-4.58053855480737));
#151608=CARTESIAN_POINT('Ctrl Pts',(-5.69215102469282,1.07598454214351,
-4.55501688436513));
#151609=CARTESIAN_POINT('Ctrl Pts',(-5.66042266160367,1.06939092069564,
-4.5301341366984));
#151610=CARTESIAN_POINT('Ctrl Pts',(-5.695609683,1.068630405,-4.879552268));
#151611=CARTESIAN_POINT('Ctrl Pts',(-5.701425371,1.070029867,-4.872763963));
#151612=CARTESIAN_POINT('Ctrl Pts',(-5.707224861,1.071428571,-4.865961815));
#151613=CARTESIAN_POINT('Ctrl Pts',(-5.96715219,1.134117105,-4.561096349));
#151614=CARTESIAN_POINT('Ctrl Pts',(-6.193122768,1.197973174,-4.23027545));
#151615=CARTESIAN_POINT('Ctrl Pts',(-5.65748713,1.068630405,-4.533799662));
#151616=CARTESIAN_POINT('Ctrl Pts',(-5.662890733,1.070029867,-4.527056793));
#151617=CARTESIAN_POINT('Ctrl Pts',(-5.668278248,1.071428571,-4.520301063));
#151618=CARTESIAN_POINT('Ctrl Pts',(-5.90974125700001,1.134117105,-4.217516027));
#151619=CARTESIAN_POINT('Ctrl Pts',(-6.11757421800001,1.197973174,-3.89073074));
#151620=CARTESIAN_POINT('Origin',(0.172489465399025,1.33885358243788,0.0820646436682093));
#151621=CARTESIAN_POINT('Ctrl Pts',(-6.44348537030917,1.20239769727684,
-3.83929775550167));
#151622=CARTESIAN_POINT('Ctrl Pts',(-6.45065500842762,1.20018543563844,
-3.82716146182784));
#151623=CARTESIAN_POINT('Ctrl Pts',(-6.45782464654608,1.197973174,-3.81502516815401));
#151624=CARTESIAN_POINT('Ctrl Pts',(-6.66565064167765,1.13384644,-3.46323093972956));
#151625=CARTESIAN_POINT('Ctrl Pts',(-6.83403176425173,1.068610636,-3.09094258099947));
#151626=CARTESIAN_POINT('Ctrl Pts',(-6.10295039234986,1.20239769727684,
-3.91372445118755));
#151627=CARTESIAN_POINT('Ctrl Pts',(-6.11026230517487,1.20018543563845,
-3.90222759559374));
#151628=CARTESIAN_POINT('Ctrl Pts',(-6.11757421800001,1.197973174,-3.89073074));
#151629=CARTESIAN_POINT('Ctrl Pts',(-6.329524324,1.13384644,-3.557471876));
#151630=CARTESIAN_POINT('Ctrl Pts',(-6.504018629,1.068610636,-3.2031612));
#151631=CARTESIAN_POINT('',(-6.50193005203167,1.06939092017978,-3.2073985659925));
#151632=CARTESIAN_POINT('Origin',(0.180664648446098,0.946547090042,0.0664058816374508));
#151633=CARTESIAN_POINT('Ctrl Pts',(-6.72695393012478,1.10830076261049,
-3.31633695786175));
#151634=CARTESIAN_POINT('Ctrl Pts',(-6.68946369205213,1.10211922687114,
-3.29806430321489));
#151635=CARTESIAN_POINT('Ctrl Pts',(-6.65194853850496,1.09579054188135,
-3.27983725979242));
#151636=CARTESIAN_POINT('Ctrl Pts',(-6.57548829285055,1.08257769708028,
-3.24281801837758));
#151637=CARTESIAN_POINT('Ctrl Pts',(-6.53826539480128,1.07598449024056,
-3.22487877187214));
#151638=CARTESIAN_POINT('Ctrl Pts',(-6.50193005463138,1.06939092064217,
-3.20739856646713));
#151639=CARTESIAN_POINT('Ctrl Pts',(-6.611408993,1.068630405,-3.541083327));
#151640=CARTESIAN_POINT('Ctrl Pts',(-6.615629428,1.070029867,-3.533203528));
#151641=CARTESIAN_POINT('Ctrl Pts',(-6.619831069,1.071428571,-3.525313691));
#151642=CARTESIAN_POINT('Ctrl Pts',(-6.808144378,1.134117105,-3.171699118));
#151643=CARTESIAN_POINT('Ctrl Pts',(-6.957715175,1.197973174,-2.800035633));
#151644=CARTESIAN_POINT('Ctrl Pts',(-6.499851134,1.068630405,-3.211609446));
#151645=CARTESIAN_POINT('Ctrl Pts',(-6.503678886,1.070029867,-3.203862607));
#151646=CARTESIAN_POINT('Ctrl Pts',(-6.507488162,1.071428571,-3.196106666));
#151647=CARTESIAN_POINT('Ctrl Pts',(-6.678216068,1.134117105,-2.848493166));
#151648=CARTESIAN_POINT('Ctrl Pts',(-6.810940832,1.197973174,-2.484669994));
#151649=CARTESIAN_POINT('Origin',(0.186098011533374,1.33885358281873,0.0430657848834071));
#151650=CARTESIAN_POINT('Ctrl Pts',(-7.11817579072873,1.20239769742353,
-2.36437822199281));
#151651=CARTESIAN_POINT('Ctrl Pts',(-7.12256886247866,1.20018543571177,
-2.35098440740509));
#151652=CARTESIAN_POINT('Ctrl Pts',(-7.12696193422843,1.197973174,-2.33759059281739));
#151653=CARTESIAN_POINT('Ctrl Pts',(-7.25430371393051,1.13384644,-1.94934467202816));
#151654=CARTESIAN_POINT('Ctrl Pts',(-7.33871718618051,1.068610636,-1.54956324476661));
#151655=CARTESIAN_POINT('Ctrl Pts',(-6.80160187114612,1.20239769742353,
-2.51026981604631));
#151656=CARTESIAN_POINT('Ctrl Pts',(-6.80627135157313,1.20018543571177,
-2.49746990502316));
#151657=CARTESIAN_POINT('Ctrl Pts',(-6.810940832,1.197973174,-2.484669994));
#151658=CARTESIAN_POINT('Ctrl Pts',(-6.946294858,1.13384644,-2.11363953));
#151659=CARTESIAN_POINT('Ctrl Pts',(-7.040543261,1.068610636,-1.730101323));
#151660=CARTESIAN_POINT('',(-7.03941442235458,1.06939092016788,-1.73468860428955));
#151661=CARTESIAN_POINT('Origin',(0.190715988737931,0.946547109884456,0.0260157603669187));
#151662=CARTESIAN_POINT('Ctrl Pts',(-7.28259590116875,1.10830076259209,
-1.79270659508155));
#151663=CARTESIAN_POINT('Ctrl Pts',(-7.24205408327934,1.10211922684959,
-1.78292043793131));
#151664=CARTESIAN_POINT('Ctrl Pts',(-7.20149773745193,1.09579054185039,
-1.77318418171899));
#151665=CARTESIAN_POINT('Ctrl Pts',(-7.118867287594,1.08257773551417,-1.75346717962857));
#151666=CARTESIAN_POINT('Ctrl Pts',(-7.07865822432206,1.07598452917805,
-1.74394916250209));
#151667=CARTESIAN_POINT('Ctrl Pts',(-7.03941442481537,1.06939092068366,
-1.73468860419114));
#151668=CARTESIAN_POINT('Ctrl Pts',(-7.218066166,1.068630405,-2.037037265));
#151669=CARTESIAN_POINT('Ctrl Pts',(-7.220494006,1.070029867,-2.028434422));
#151670=CARTESIAN_POINT('Ctrl Pts',(-7.222901333,1.071428571,-2.019825817));
#151671=CARTESIAN_POINT('Ctrl Pts',(-7.330795302,1.134117105,-1.633996761));
#151672=CARTESIAN_POINT('Ctrl Pts',(-7.396972553,1.197973174,-1.238869262));
#151673=CARTESIAN_POINT('Ctrl Pts',(-7.038289323,1.068630405,-1.739247943));
#151674=CARTESIAN_POINT('Ctrl Pts',(-7.040362243,1.070029867,-1.730859367));
#151675=CARTESIAN_POINT('Ctrl Pts',(-7.042415162,1.071428571,-1.722465874));
#151676=CARTESIAN_POINT('Ctrl Pts',(-7.134424917,1.134117105,-1.346277931));
#151677=CARTESIAN_POINT('Ctrl Pts',(-7.18583542299999,1.197973174,-0.962428841999999));
#151678=CARTESIAN_POINT('Origin',(0.191005223540494,1.33885360436684,0.00205339707159954));
#151679=CARTESIAN_POINT('Ctrl Pts',(-7.46146198490312,1.19924836941368,
-0.759375434223065));
#151680=CARTESIAN_POINT('Ctrl Pts',(-7.46186891395157,1.19861077170684,
-0.755333573111533));
#151681=CARTESIAN_POINT('Ctrl Pts',(-7.462275843,1.197973174,-0.751291712));
#151682=CARTESIAN_POINT('Ctrl Pts',(-7.503202952,1.13384644,-0.344779346));
#151683=CARTESIAN_POINT('Ctrl Pts',(-7.49972886,1.068610636,0.063773298));
#151684=CARTESIAN_POINT('Ctrl Pts',(-7.18479284462103,1.19924836941368,
-0.970213102287846));
#151685=CARTESIAN_POINT('Ctrl Pts',(-7.18531413381051,1.19861077170684,
-0.966320972143922));
#151686=CARTESIAN_POINT('Ctrl Pts',(-7.185835423,1.197973174,-0.962428842));
#151687=CARTESIAN_POINT('Ctrl Pts',(-7.238264365,1.13384644,-0.570975749));
#151688=CARTESIAN_POINT('Ctrl Pts',(-7.24785991500001,1.068610636,-0.176143831));
#151689=CARTESIAN_POINT('',(-7.24774359796863,1.06939092016464,-0.180866531822896));
#151690=CARTESIAN_POINT('Origin',(0.191849688360007,0.946547112772989,-0.0155907848465632));
#151691=CARTESIAN_POINT('Ctrl Pts',(-7.4977117819841,1.10830076263164,-0.185251264675216));
#151692=CARTESIAN_POINT('Ctrl Pts',(-7.4560140745458,1.10211922684026,-0.184409194783553));
#151693=CARTESIAN_POINT('Ctrl Pts',(-7.41431290627305,1.09579054182928,
-0.183618982244394));
#151694=CARTESIAN_POINT('Ctrl Pts',(-7.32937619817292,1.08257780709784,
-0.182126064751401));
#151695=CARTESIAN_POINT('Ctrl Pts',(-7.28806110257299,1.07598460347731,
-0.181474331916232));
#151696=CARTESIAN_POINT('Ctrl Pts',(-7.24774360024735,1.06939092064195,
-0.180866530270857));
#151697=CARTESIAN_POINT('Ctrl Pts',(-7.487214588,1.068630405,-0.437741604));
#151698=CARTESIAN_POINT('Ctrl Pts',(-7.48773631,1.070029867,-0.428817978));
#151699=CARTESIAN_POINT('Ctrl Pts',(-7.488236759,1.071428571,-0.419893133));
#151700=CARTESIAN_POINT('Ctrl Pts',(-7.510666384,1.134117105,-0.019890532));
#151701=CARTESIAN_POINT('Ctrl Pts',(-7.490355716,1.197973174,0.380225258));
#151702=CARTESIAN_POINT('Ctrl Pts',(-7.247624926,1.068630405,-0.185561138));
#151703=CARTESIAN_POINT('Ctrl Pts',(-7.247846087,1.070029867,-0.176923066));
#151704=CARTESIAN_POINT('Ctrl Pts',(-7.248046656,1.071428571,-0.168284491));
#151705=CARTESIAN_POINT('Ctrl Pts',(-7.257035987,1.134117105,0.218887764));
#151706=CARTESIAN_POINT('Ctrl Pts',(-7.224728336,1.197973174,0.604814414000001));
#151707=CARTESIAN_POINT('Origin',(0.186981097361099,1.33885359240906,-0.0390550889411558));
#151708=CARTESIAN_POINT('Ctrl Pts',(-7.45305802788279,1.20239769728737,
0.842992881250072));
#151709=CARTESIAN_POINT('Ctrl Pts',(-7.45142115507788,1.20018543564367,
0.856993380657568));
#151710=CARTESIAN_POINT('Ctrl Pts',(-7.44978428227295,1.197973174,0.870993880065064));
#151711=CARTESIAN_POINT('Ctrl Pts',(-7.402336320024,1.13384644,1.27682575982473));
#151712=CARTESIAN_POINT('Ctrl Pts',(-7.3110840494493,1.068610636,1.67510185406666));
#151713=CARTESIAN_POINT('Ctrl Pts',(-7.22700161094625,1.20239769728737,
0.57765931767797));
#151714=CARTESIAN_POINT('Ctrl Pts',(-7.22586497347307,1.20018543564367,
0.591236865838985));
#151715=CARTESIAN_POINT('Ctrl Pts',(-7.224728336,1.197973174,0.604814414));
#151716=CARTESIAN_POINT('Ctrl Pts',(-7.191780674,1.13384644,0.998386224));
#151717=CARTESIAN_POINT('Ctrl Pts',(-7.116274695,1.068610636,1.38604995));
#151718=CARTESIAN_POINT('',(-7.11717633793565,1.06939092018892,1.38141265923022));
#151719=CARTESIAN_POINT('Origin',(0.184013027001663,0.946547072036405,-0.0564683324673482));
#151720=CARTESIAN_POINT('Ctrl Pts',(-7.36224299279127,1.1083007625811,1.43086620946192));
#151721=CARTESIAN_POINT('Ctrl Pts',(-7.32133913467256,1.10211922683588,
1.4227248176501));
#151722=CARTESIAN_POINT('Ctrl Pts',(-7.2804430444382,1.0957905418693,1.4145320369038));
#151723=CARTESIAN_POINT('Ctrl Pts',(-7.19717121001193,1.08257781249686,
1.39773117588402));
#151724=CARTESIAN_POINT('Ctrl Pts',(-7.1566819324551,1.07598460868545,1.3894861468627));
#151725=CARTESIAN_POINT('Ctrl Pts',(-7.11717634035813,1.0693909206464,1.38141266056319));
#151726=CARTESIAN_POINT('Ctrl Pts',(-7.406269177,1.068630405,1.182022367));
#151727=CARTESIAN_POINT('Ctrl Pts',(-7.404860385,1.070029867,1.190849519));
#151728=CARTESIAN_POINT('Ctrl Pts',(-7.403430556,1.071428571,1.199673288));
#151729=CARTESIAN_POINT('Ctrl Pts',(-7.339347054,1.134117105,1.595145757));
#151730=CARTESIAN_POINT('Ctrl Pts',(-7.233498171,1.197973174,1.981540869));
#151731=CARTESIAN_POINT('Ctrl Pts',(-7.118069642,1.068630405,1.376802299));
#151732=CARTESIAN_POINT('Ctrl Pts',(-7.116428702,1.070029867,1.385285961));
#151733=CARTESIAN_POINT('Ctrl Pts',(-7.114767544,1.071428571,1.393765687));
#151734=CARTESIAN_POINT('Ctrl Pts',(-7.04031611900001,1.134117105,1.77381851));
#151735=CARTESIAN_POINT('Ctrl Pts',(-6.925800981,1.197973174,2.14377722));
#151736=CARTESIAN_POINT('Origin',(0.174213841875577,1.33885354649174,-0.078337391496032));
#151737=CARTESIAN_POINT('Ctrl Pts',(-7.09759112262429,1.20239769754087,
2.42547133988342));
#151738=CARTESIAN_POINT('Ctrl Pts',(-7.09298282519605,1.20018543577042,
2.43879263690317));
#151739=CARTESIAN_POINT('Ctrl Pts',(-7.08837452776767,1.197973174,2.45211393392285));
#151740=CARTESIAN_POINT('Ctrl Pts',(-6.95479401422635,1.13384644,2.83825778088423));
#151741=CARTESIAN_POINT('Ctrl Pts',(-6.78005758344963,1.068610636,3.20760585967038));
#151742=CARTESIAN_POINT('Ctrl Pts',(-6.93385865142889,1.20239769754087,
2.117745680191));
#151743=CARTESIAN_POINT('Ctrl Pts',(-6.92982981621444,1.20018543577042,
2.13076145009547));
#151744=CARTESIAN_POINT('Ctrl Pts',(-6.925800981,1.197973174,2.14377722));
#151745=CARTESIAN_POINT('Ctrl Pts',(-6.809017313,1.13384644,2.521064766));
#151746=CARTESIAN_POINT('Ctrl Pts',(-6.651940379,1.068610636,2.883433576));
#151747=CARTESIAN_POINT('',(-6.65381782292297,1.06939092017145,2.87909852931941));
#151748=CARTESIAN_POINT('Origin',(0.167571566097645,0.946547121045729,-0.0947053690530753));
#151749=CARTESIAN_POINT('Ctrl Pts',(-6.88252390359979,1.10830076262036,
2.9800779698598));
#151750=CARTESIAN_POINT('Ctrl Pts',(-6.84432651353948,1.10211922685067,
2.96333379889362));
#151751=CARTESIAN_POINT('Ctrl Pts',(-6.80614775662968,1.09579054182053,
2.94654111021503));
#151752=CARTESIAN_POINT('Ctrl Pts',(-6.72843428248117,1.08257778223854,
2.91223198284212));
#151753=CARTESIAN_POINT('Ctrl Pts',(-6.69066405871868,1.07598457671899,
2.89547571963673));
#151754=CARTESIAN_POINT('Ctrl Pts',(-6.6538178243887,1.06939092057759,2.87909853129467));
#151755=CARTESIAN_POINT('Ctrl Pts',(-6.979014851,1.068630405,2.746516286));
#151756=CARTESIAN_POINT('Ctrl Pts',(-6.975741419,1.070029867,2.754834216));
#151757=CARTESIAN_POINT('Ctrl Pts',(-6.972448169,1.071428571,2.763144319));
#151758=CARTESIAN_POINT('Ctrl Pts',(-6.824848013,1.134117105,3.135594802));
#151759=CARTESIAN_POINT('Ctrl Pts',(-6.63841029,1.197973174,3.490201831));
#151760=CARTESIAN_POINT('Ctrl Pts',(-6.655681333,1.068630405,2.874787991));
#151761=CARTESIAN_POINT('Ctrl Pts',(-6.652255021,1.070029867,2.882720556));
#151762=CARTESIAN_POINT('Ctrl Pts',(-6.64880981,1.071428571,2.890644931));
#151763=CARTESIAN_POINT('Ctrl Pts',(-6.494398894,1.134117105,3.245807475));
#151764=CARTESIAN_POINT('Ctrl Pts',(-6.30303087,1.197973174,3.582499385));
#151765=CARTESIAN_POINT('Ctrl Pts',(-6.65244799782,1.068630405,2.87607070805));
#151766=CARTESIAN_POINT('Ctrl Pts',(-6.64902015702,1.070029867,2.8839994194));
#151767=CARTESIAN_POINT('Ctrl Pts',(-6.64557342641,1.071428571,2.89191993712));
#151768=CARTESIAN_POINT('Ctrl Pts',(-6.49109440281,1.134117105,3.24690960173));
#151769=CARTESIAN_POINT('Ctrl Pts',(-6.2996770758,1.197973174,3.58342236054));
#151770=CARTESIAN_POINT('Origin',(0.153300462422697,1.33885355272707,-0.11395667019479));
#151771=CARTESIAN_POINT('Ctrl Pts',(-6.41024874438494,1.20239769750625,
3.89453745597396));
#151772=CARTESIAN_POINT('Ctrl Pts',(-6.40288450137365,1.20018543575313,
3.90655666063902));
#151773=CARTESIAN_POINT('Ctrl Pts',(-6.39552025836221,1.197973174,3.91857586530409));
#151774=CARTESIAN_POINT('Ctrl Pts',(-6.18205327054469,1.13384644,4.26697602155056));
#151775=CARTESIAN_POINT('Ctrl Pts',(-5.93200316123656,1.068610636,4.5901257810134));
#151776=CARTESIAN_POINT('Ctrl Pts',(-6.31649616806704,1.20239769750625,
3.55880860922295));
#151777=CARTESIAN_POINT('Ctrl Pts',(-6.3097635190336,1.20018543575313,3.57065399711151));
#151778=CARTESIAN_POINT('Ctrl Pts',(-6.30303087,1.197973174,3.582499385));
#151779=CARTESIAN_POINT('Ctrl Pts',(-6.107871869,1.13384644,3.925861122));
#151780=CARTESIAN_POINT('Ctrl Pts',(-5.876568725,1.068610636,4.245991053));
#151781=CARTESIAN_POINT('',(-5.87933418162948,1.06939092014569,4.24216095191438));
#151782=CARTESIAN_POINT('Origin',(0.143295128420343,0.946547072488477,-0.128514236352059));
#151783=CARTESIAN_POINT('Ctrl Pts',(-6.08098564645011,1.10830076263365,
4.38994459618124));
#151784=CARTESIAN_POINT('Ctrl Pts',(-6.04728079196527,1.10211922686965,
4.36538058482439));
#151785=CARTESIAN_POINT('Ctrl Pts',(-6.01360456489735,1.09579054184488,
4.34077319563695));
#151786=CARTESIAN_POINT('Ctrl Pts',(-5.94508333958708,1.08257776348828,
4.2905600253094));
#151787=CARTESIAN_POINT('Ctrl Pts',(-5.91179827121622,1.07598455844107,
4.26607603671867));
#151788=CARTESIAN_POINT('Ctrl Pts',(-5.87933418351883,1.06939092066381,
4.2421609540683));
#151789=CARTESIAN_POINT('Ctrl Pts',(-6.22542954700001,1.068630405,4.182586157));
#151790=CARTESIAN_POINT('Ctrl Pts',(-6.220444537,1.070029867,4.190005926));
#151791=CARTESIAN_POINT('Ctrl Pts',(-6.215441855,1.071428571,4.197413792));
#151792=CARTESIAN_POINT('Ctrl Pts',(-5.991226664,1.134117105,4.52942692));
#151793=CARTESIAN_POINT('Ctrl Pts',(-5.732917723,1.197973174,4.835664834));
#151794=CARTESIAN_POINT('Ctrl Pts',(-5.882080762,1.068630405,4.238351791));
#151795=CARTESIAN_POINT('Ctrl Pts',(-5.877029288,1.070029867,4.245362341));
#151796=CARTESIAN_POINT('Ctrl Pts',(-5.871961118,1.071428571,4.25236083));
#151797=CARTESIAN_POINT('Ctrl Pts',(-5.64481079600001,1.134117105,4.566026089));
#151798=CARTESIAN_POINT('Ctrl Pts',(-5.385538041,1.197973174,4.853707861));
#151799=CARTESIAN_POINT('Origin',(0.12521894237024,1.33885356109855,-0.144247394630111));
#151800=CARTESIAN_POINT('Ctrl Pts',(-5.42317026021917,1.20239769763789,
5.18149932878505));
#151801=CARTESIAN_POINT('Ctrl Pts',(-5.4133944151325,1.20018543581893,5.19165443686541));
#151802=CARTESIAN_POINT('Ctrl Pts',(-5.40361857004568,1.197973174,5.20180954494577));
#151803=CARTESIAN_POINT('Ctrl Pts',(-5.12024658751617,1.13384644,5.49617520683819));
#151804=CARTESIAN_POINT('Ctrl Pts',(-4.80657486481941,1.068610636,5.75801652210095));
#151805=CARTESIAN_POINT('Ctrl Pts',(-5.40378134486888,1.20239769763789,
4.83346560284931));
#151806=CARTESIAN_POINT('Ctrl Pts',(-5.39465969293444,1.20018543581893,
4.84358673192466));
#151807=CARTESIAN_POINT('Ctrl Pts',(-5.385538041,1.197973174,4.853707861));
#151808=CARTESIAN_POINT('Ctrl Pts',(-5.121129126,1.13384644,5.147088575));
#151809=CARTESIAN_POINT('Ctrl Pts',(-4.826415248,1.068610636,5.410010708));
#151810=CARTESIAN_POINT('',(-4.82993940821834,1.06939092015418,5.40686464364233));
#151811=CARTESIAN_POINT('Origin',(0.112318141206653,0.946547119532799,-0.156313780444191));
#151812=CARTESIAN_POINT('Ctrl Pts',(-4.99510725948456,1.10830076259581,
5.59454229236901));
#151813=CARTESIAN_POINT('Ctrl Pts',(-4.96747094198495,1.10211922681569,
5.56330702642328));
#151814=CARTESIAN_POINT('Ctrl Pts',(-4.93987190779602,1.09579054183511,
5.5320355511299));
#151815=CARTESIAN_POINT('Ctrl Pts',(-4.88374728279049,1.08257782587387,
5.46826659984461));
#151816=CARTESIAN_POINT('Ctrl Pts',(-4.8565037268271,1.07598462233103,5.43719972100207));
#151817=CARTESIAN_POINT('Ctrl Pts',(-4.82993941000098,1.06939092073088,
5.40686464621053));
#151818=CARTESIAN_POINT('Ctrl Pts',(-5.180750076,1.068630405,5.423082947));
#151819=CARTESIAN_POINT('Ctrl Pts',(-5.174286582,1.070029867,5.429257617));
#151820=CARTESIAN_POINT('Ctrl Pts',(-5.167808388,1.071428571,5.435416862));
#151821=CARTESIAN_POINT('Ctrl Pts',(-4.877462215,1.134117105,5.711468069));
#151822=CARTESIAN_POINT('Ctrl Pts',(-4.559360294,1.197973174,5.955017524));
#151823=CARTESIAN_POINT('Ctrl Pts',(-4.833440632,1.068630405,5.403734972));
#151824=CARTESIAN_POINT('Ctrl Pts',(-4.827000198,1.070029867,5.409495702));
#151825=CARTESIAN_POINT('Ctrl Pts',(-4.82054605,1.071428571,5.415241063));
#151826=CARTESIAN_POINT('Ctrl Pts',(-4.531277618,1.134117105,5.672742398));
#151827=CARTESIAN_POINT('Ctrl Pts',(-4.216223439,1.197973174,5.897962352));
#151828=CARTESIAN_POINT('Origin',(0.0912825581236565,1.33885357253129,-0.167793454434852));
#151829=CARTESIAN_POINT('Ctrl Pts',(-4.16592911596048,1.19924836941368,
6.23659367087182));
#151830=CARTESIAN_POINT('Ctrl Pts',(-4.16254869198024,1.19861077170684,
6.23884643943591));
#151831=CARTESIAN_POINT('Ctrl Pts',(-4.159168268,1.197973174,6.241099208));
#151832=CARTESIAN_POINT('Ctrl Pts',(-3.819180299,1.13384644,6.467672624));
#151833=CARTESIAN_POINT('Ctrl Pts',(-3.456591824,1.068610636,6.655972728));
#151834=CARTESIAN_POINT('Ctrl Pts',(-4.22261257419804,1.19924836941368,
5.89339500821418));
#151835=CARTESIAN_POINT('Ctrl Pts',(-4.21941800659903,1.19861077170684,
5.89567868010709));
#151836=CARTESIAN_POINT('Ctrl Pts',(-4.216223439,1.197973174,5.897962352));
#151837=CARTESIAN_POINT('Ctrl Pts',(-3.894928076,1.13384644,6.127643887));
#151838=CARTESIAN_POINT('Ctrl Pts',(-3.550583958,1.068610636,6.321064274));
#151839=CARTESIAN_POINT('',(-3.55470203688038,1.06939092017366,6.3187493536364));
#151840=CARTESIAN_POINT('Origin',(0.0760893310988892,0.946547110468997,
-0.176804295816098));
#151841=CARTESIAN_POINT('Ctrl Pts',(-3.67566320760578,1.10830076262188,
6.53754540923889));
#151842=CARTESIAN_POINT('Ctrl Pts',(-3.65538767083809,1.10211922686063,
6.50109941524943));
#151843=CARTESIAN_POINT('Ctrl Pts',(-3.63515632942574,1.09579054182311,
6.46462607283155));
#151844=CARTESIAN_POINT('Ctrl Pts',(-3.59405206005671,1.08257774660545,
6.39028242294247));
#151845=CARTESIAN_POINT('Ctrl Pts',(-3.57412391075782,1.07598454084017,
6.35408531973988));
#151846=CARTESIAN_POINT('Ctrl Pts',(-3.55470203703904,1.06939092067389,
6.31874935621956));
#151847=CARTESIAN_POINT('Ctrl Pts',(-3.89382449,1.068630405,6.410002406));
#151848=CARTESIAN_POINT('Ctrl Pts',(-3.886184737,1.070029867,6.414643255));
#151849=CARTESIAN_POINT('Ctrl Pts',(-3.878533944,1.071428571,6.419265881));
#151850=CARTESIAN_POINT('Ctrl Pts',(-3.535633054,1.134117105,6.626447319));
#151851=CARTESIAN_POINT('Ctrl Pts',(-3.172612246,1.197973174,6.795920213));
#151852=CARTESIAN_POINT('Ctrl Pts',(-3.558794191,1.068630405,6.316445512));
#151853=CARTESIAN_POINT('Ctrl Pts',(-3.551265944,1.070029867,6.320687056));
#151854=CARTESIAN_POINT('Ctrl Pts',(-3.543727607,1.071428571,6.324910643));
#151855=CARTESIAN_POINT('Ctrl Pts',(-3.205866935,1.134117105,6.514207577));
#151856=CARTESIAN_POINT('Ctrl Pts',(-2.849762915,1.197973174,6.666434679));
#151857=CARTESIAN_POINT('Origin',(0.0530778863023995,1.33885358189054,-0.183493785369463));
#151858=CARTESIAN_POINT('Ctrl Pts',(-2.72784872138814,1.19924836941368,
6.98633719228998));
#151859=CARTESIAN_POINT('Ctrl Pts',(-2.72406305119407,1.19861077170684,
6.98781060114499));
#151860=CARTESIAN_POINT('Ctrl Pts',(-2.720277381,1.197973174,6.98928401));
#151861=CARTESIAN_POINT('Ctrl Pts',(-2.339531555,1.13384644,7.13747290200001));
#151862=CARTESIAN_POINT('Ctrl Pts',(-1.944941241,1.068610636,7.243424851));
#151863=CARTESIAN_POINT('Ctrl Pts',(-2.85698451967887,1.19924836941368,
6.66334759239431));
#151864=CARTESIAN_POINT('Ctrl Pts',(-2.85337371733943,1.19861077170684,
6.66489113569715));
#151865=CARTESIAN_POINT('Ctrl Pts',(-2.849762915,1.197973174,6.666434679));
#151866=CARTESIAN_POINT('Ctrl Pts',(-2.486604518,1.13384644,6.821677381));
#151867=CARTESIAN_POINT('Ctrl Pts',(-2.108731308,1.068610636,6.93655190100001));
#151868=CARTESIAN_POINT('',(-2.1132507478268,1.06939092018769,6.93517636705353));
#151869=CARTESIAN_POINT('Origin',(0.0363027951216388,0.946547113271884,
-0.189027909638053));
#151870=CARTESIAN_POINT('Ctrl Pts',(-2.18434923030014,1.10830076263856,
7.17486016828108));
#151871=CARTESIAN_POINT('Ctrl Pts',(-2.17238253565839,1.1021192268862,7.13490762038882));
#151872=CARTESIAN_POINT('Ctrl Pts',(-2.16046488222171,1.09579054187813,
7.09493786428172));
#151873=CARTESIAN_POINT('Ctrl Pts',(-2.13630354385015,1.08257788288011,
7.01349696441781));
#151874=CARTESIAN_POINT('Ctrl Pts',(-2.1246226002447,1.075984679786,6.97386214325294));
#151875=CARTESIAN_POINT('Ctrl Pts',(-2.11325074774407,1.06939092070939,
6.9351763699027));
#151876=CARTESIAN_POINT('Ctrl Pts',(-2.424827999,1.068630405,7.097197276));
#151877=CARTESIAN_POINT('Ctrl Pts',(-2.416369214,1.070029867,7.100087304));
#151878=CARTESIAN_POINT('Ctrl Pts',(-2.407903564,1.071428571,7.102957161));
#151879=CARTESIAN_POINT('Ctrl Pts',(-2.028481621,1.134117105,7.231581257));
#151880=CARTESIAN_POINT('Ctrl Pts',(-1.637516375,1.197973174,7.319053226));
#151881=CARTESIAN_POINT('Ctrl Pts',(-2.117742488,1.068630405,6.93380608));
#151882=CARTESIAN_POINT('Ctrl Pts',(-2.10947844,1.070029867,6.936330109));
#151883=CARTESIAN_POINT('Ctrl Pts',(-2.1012084,1.071428571,6.938834431));
#151884=CARTESIAN_POINT('Ctrl Pts',(-1.730553477,1.134117105,7.05107565));
#151885=CARTESIAN_POINT('Ctrl Pts',(-1.350050644,1.197973174,7.123191929));
#151886=CARTESIAN_POINT('Origin',(0.0123912359408862,1.3388535675646,-0.190614068400277));
#151887=CARTESIAN_POINT('Ctrl Pts',(-1.16221715234734,1.19924836941368,
7.40940735161141));
#151888=CARTESIAN_POINT('Ctrl Pts',(-1.15820324967367,1.19861077170684,
7.4100325058057));
#151889=CARTESIAN_POINT('Ctrl Pts',(-1.154189347,1.197973174,7.41065766));
#151890=CARTESIAN_POINT('Ctrl Pts',(-0.750488916,1.13384644,7.473532881));
#151891=CARTESIAN_POINT('Ctrl Pts',(-0.342347366,1.068610636,7.492182478));
#151892=CARTESIAN_POINT('Ctrl Pts',(-1.35776704393169,1.19924836941368,
7.12172944830897));
#151893=CARTESIAN_POINT('Ctrl Pts',(-1.35390884396585,1.19861077170684,
7.12246068865448));
#151894=CARTESIAN_POINT('Ctrl Pts',(-1.350050644,1.197973174,7.123191929));
#151895=CARTESIAN_POINT('Ctrl Pts',(-0.962010097,1.13384644,7.196736822));
#151896=CARTESIAN_POINT('Ctrl Pts',(-0.568276727,1.068610636,7.227694069));
#151897=CARTESIAN_POINT('',(-0.572986203455311,1.06939092018801,7.22732224112166));
#151898=CARTESIAN_POINT('Origin',(-0.00518136125522824,0.94654711394043,
-0.19241258054147));
#151899=CARTESIAN_POINT('Ctrl Pts',(-0.590897510175425,1.10830076262937,
7.47668644052261));
#151900=CARTESIAN_POINT('Ctrl Pts',(-0.587799206980913,1.10211922687916,
7.43509547532359));
#151901=CARTESIAN_POINT('Ctrl Pts',(-0.58475249770118,1.09579054188195,
7.39349824672118));
#151902=CARTESIAN_POINT('Ctrl Pts',(-0.578663341299355,1.08257770324263,
7.30876626426851));
#151903=CARTESIAN_POINT('Ctrl Pts',(-0.575775813423528,1.07598449667183,
7.26754705879483));
#151904=CARTESIAN_POINT('Ctrl Pts',(-0.57298620261301,1.06939092059987,
7.22732224306242));
#151905=CARTESIAN_POINT('Ctrl Pts',(-0.842449245,1.068630405,7.45253509));
#151906=CARTESIAN_POINT('Ctrl Pts',(-0.833566951,1.070029867,7.453539162));
#151907=CARTESIAN_POINT('Ctrl Pts',(-0.824682289,1.071428571,7.454522059));
#151908=CARTESIAN_POINT('Ctrl Pts',(-0.426480641,1.134117105,7.498574493));
#151909=CARTESIAN_POINT('Ctrl Pts',(-0.025852058,1.197973174,7.499955445));
#151910=CARTESIAN_POINT('Ctrl Pts',(-0.5776675,1.068630405,7.226949582));
#151911=CARTESIAN_POINT('Ctrl Pts',(-0.56905407,1.070029867,7.22763807400001));
#151912=CARTESIAN_POINT('Ctrl Pts',(-0.560439023,1.071428571,7.228306033));
#151913=CARTESIAN_POINT('Ctrl Pts',(-0.174321262,1.134117105,7.25824326300001));
#151914=CARTESIAN_POINT('Ctrl Pts',(0.212788494,1.197973174,7.246876641));
#151915=CARTESIAN_POINT('Ctrl Pts',(-0.57501968255,1.068630405,7.22469372692));
#151916=CARTESIAN_POINT('Ctrl Pts',(-0.56640894119,1.070029867,7.22537906312));
#151917=CARTESIAN_POINT('Ctrl Pts',(-0.55779659034,1.071428571,7.22604387274));
#151918=CARTESIAN_POINT('Ctrl Pts',(-0.17179966821,1.134117105,7.2558399507));
#151919=CARTESIAN_POINT('Ctrl Pts',(0.21517489952,1.197973174,7.24434585296));
#151920=CARTESIAN_POINT('Origin',(-0.0288748555719699,1.33885357237991,
-0.188821302331477));
#151921=CARTESIAN_POINT('Ctrl Pts',(-1.355629403,4.820162746,7.12213233));
#151922=CARTESIAN_POINT('Ctrl Pts',(-0.969698837,4.755280647,7.195590502));
#151923=CARTESIAN_POINT('Ctrl Pts',(-0.578090317,4.690053947,7.226915773));
#151924=CARTESIAN_POINT('Ctrl Pts',(-0.572170154643126,4.68906787893895,
7.22738933442862));
#151925=CARTESIAN_POINT('Ctrl Pts',(-0.566249992286254,4.68808181087793,
7.22786289585724));
#151926=CARTESIAN_POINT('Ctrl Pts',(-1.64350626427388,4.820162746,7.31794377208008));
#151927=CARTESIAN_POINT('Ctrl Pts',(-1.24696516389368,4.755280647,7.40700127323003));
#151928=CARTESIAN_POINT('Ctrl Pts',(-0.843122611572138,4.690053947,7.45268798177261));
#151929=CARTESIAN_POINT('Ctrl Pts',(-0.837017500589471,4.68906787893895,
7.45337865298712));
#151930=CARTESIAN_POINT('Ctrl Pts',(-0.830912389606805,4.68808181087793,
7.45406932420163));
#151931=CARTESIAN_POINT('',(-1.35103832279166,4.8193909209625,7.12300468390861));
#151932=CARTESIAN_POINT('Origin',(0.0169038419875292,4.69643176852073,-0.198295171745094));
#151933=CARTESIAN_POINT('Origin',(-2.49805601449516,5.70976516819263,14.5140475055271));
#151934=CARTESIAN_POINT('Ctrl Pts',(-2.118148151,4.690053947,6.933682168));
#151935=CARTESIAN_POINT('Ctrl Pts',(-1.7374959,4.755711878,7.049966394));
#151936=CARTESIAN_POINT('Ctrl Pts',(-1.346401839,4.820155008,7.123882515));
#151937=CARTESIAN_POINT('Ctrl Pts',(-1.954774922,4.690053947,7.240777238));
#151938=CARTESIAN_POINT('Ctrl Pts',(-1.557263457,4.755711878,7.348092436));
#151939=CARTESIAN_POINT('Ctrl Pts',(-1.150393323,4.820155008,7.411247884));
#151940=CARTESIAN_POINT('Origin',(0.0771176323196965,4.55371945316075,-0.175153269118729));
#151941=CARTESIAN_POINT('Ctrl Pts',(-2.854983464,4.820162746,6.664200584));
#151942=CARTESIAN_POINT('Ctrl Pts',(-2.493867074,4.755280647,6.818905009));
#151943=CARTESIAN_POINT('Ctrl Pts',(-2.118148151,4.690053947,6.933682168));
#151944=CARTESIAN_POINT('Ctrl Pts',(-2.1124682015092,4.68906787912114,6.93541731740534));
#151945=CARTESIAN_POINT('Ctrl Pts',(-2.10678825201842,4.68808181124226,
6.93715246681066));
#151946=CARTESIAN_POINT('Ctrl Pts',(-3.1782235951834,4.820162746,6.79354904841143));
#151947=CARTESIAN_POINT('Ctrl Pts',(-2.81009813513517,4.755280647,6.96576904967454));
#151948=CARTESIAN_POINT('Ctrl Pts',(-2.4255184898198,4.690053947,7.09720183980452));
#151949=CARTESIAN_POINT('Ctrl Pts',(-2.41970458791905,4.68906787912114,
7.0991887815412));
#151950=CARTESIAN_POINT('Ctrl Pts',(-2.41389068601829,4.68808181124226,
7.1011757232779));
#151951=CARTESIAN_POINT('',(-2.85068725016658,4.81939092091803,6.66603948951303));
#151952=CARTESIAN_POINT('Origin',(0.0591363730587224,4.69643183310118,-0.190025564315469));
#151953=CARTESIAN_POINT('Origin',(-5.55973958744884,5.70977447183052,13.6376944220212));
#151954=CARTESIAN_POINT('Ctrl Pts',(-3.559163733,4.690053947,6.316237292));
#151955=CARTESIAN_POINT('Ctrl Pts',(-3.212408591,4.755711878,6.511631839));
#151956=CARTESIAN_POINT('Ctrl Pts',(-2.846347872,4.820155008,6.667893505));
#151957=CARTESIAN_POINT('Ctrl Pts',(-3.465626441,4.690053947,6.651273064));
#151958=CARTESIAN_POINT('Ctrl Pts',(-3.100478168,4.755711878,6.841532507));
#151959=CARTESIAN_POINT('Ctrl Pts',(-2.716696986,4.820155008,6.99067646800001));
#151960=CARTESIAN_POINT('Origin',(0.112967294143578,4.55371942937115,-0.154479983497169));
#151961=CARTESIAN_POINT('Ctrl Pts',(-4.22084167,4.820162746,5.894658226));
#151962=CARTESIAN_POINT('Ctrl Pts',(-3.90142486,4.755280647,6.123375096));
#151963=CARTESIAN_POINT('Ctrl Pts',(-3.559163733,4.690053947,6.31623729200001));
#151964=CARTESIAN_POINT('Ctrl Pts',(-3.55398958340173,4.68906787912089,
6.31915289583355));
#151965=CARTESIAN_POINT('Ctrl Pts',(-3.54881543380346,4.68808181124179,
6.32206849966711));
#151966=CARTESIAN_POINT('Ctrl Pts',(-4.56433072332386,4.820162746,5.95149552225326));
#151967=CARTESIAN_POINT('Ctrl Pts',(-4.241834042112,4.755280647,6.19882520615937));
#151968=CARTESIAN_POINT('Ctrl Pts',(-3.89449981884596,4.690053947,6.40985842741688));
#151969=CARTESIAN_POINT('Ctrl Pts',(-3.88924897646275,4.68906787912089,
6.41304873262789));
#151970=CARTESIAN_POINT('Ctrl Pts',(-3.88399813407952,4.6880818112418,6.41623903783889));
#151971=CARTESIAN_POINT('',(-4.21704120960913,4.81939092092061,5.89737769746916));
#151972=CARTESIAN_POINT('Origin',(0.0986037219471031,4.69643188759991,-0.172870347922783));
#151973=CARTESIAN_POINT('Origin',(-8.36147418014773,5.70977704265914,12.1237057521521));
#151974=CARTESIAN_POINT('Ctrl Pts',(-4.833756773,4.690053947,5.403452179));
#151975=CARTESIAN_POINT('Ctrl Pts',(-4.537112626,4.755711878,5.668820616));
#151976=CARTESIAN_POINT('Ctrl Pts',(-4.213201843,4.820155008,5.900121205));
#151977=CARTESIAN_POINT('Ctrl Pts',(-4.814429119,4.690053947,5.75076275500001));
#151978=CARTESIAN_POINT('Ctrl Pts',(-4.498717966,4.755711878,6.015070122));
#151979=CARTESIAN_POINT('Ctrl Pts',(-4.155970918,4.820155008,6.24322879));
#151980=CARTESIAN_POINT('Origin',(0.143534806453094,4.5537193991147,-0.126583667889788));
#151981=CARTESIAN_POINT('Ctrl Pts',(-5.389338011,4.820162746,4.8494882));
#151982=CARTESIAN_POINT('Ctrl Pts',(-5.12655635500001,4.755280647,5.14152297));
#151983=CARTESIAN_POINT('Ctrl Pts',(-4.833756773,4.690053947,5.403452179));
#151984=CARTESIAN_POINT('Ctrl Pts',(-4.82933036048759,4.68906787905874,
5.40741190708487));
#151985=CARTESIAN_POINT('Ctrl Pts',(-4.82490394797516,4.68808181111747,
5.41137163516975));
#151986=CARTESIAN_POINT('Ctrl Pts',(-5.73701481973306,4.820162746,4.83115667900776));
#151987=CARTESIAN_POINT('Ctrl Pts',(-5.4752265023282,4.755280647,5.14203118713937));
#151988=CARTESIAN_POINT('Ctrl Pts',(-5.18137866555228,4.690053947,5.42279715860608));
#151989=CARTESIAN_POINT('Ctrl Pts',(-5.17693640599519,4.68906787905874,
5.42704165240171));
#151990=CARTESIAN_POINT('Ctrl Pts',(-5.17249414643811,4.6880818111175,5.43128614619734));
#151991=CARTESIAN_POINT('',(-5.38621100963435,4.81939092093662,4.85296107894373));
#151992=CARTESIAN_POINT('Origin',(0.1334604208639,4.69643183788284,-0.147631864610709));
#151993=CARTESIAN_POINT('Origin',(-10.7723631184045,5.70979140998744,10.0429141545461));
#151994=CARTESIAN_POINT('Ctrl Pts',(-5.88232872,4.690053947,4.238007649));
#151995=CARTESIAN_POINT('Ctrl Pts',(-5.649666317,4.755711878,4.560941642));
#151996=CARTESIAN_POINT('Ctrl Pts',(-5.383051178,4.820155008,4.856465795));
#151997=CARTESIAN_POINT('Ctrl Pts',(-5.938114442,4.690053947,4.58135317));
#151998=CARTESIAN_POINT('Ctrl Pts',(-5.686602712,4.755711878,4.907349744));
#151999=CARTESIAN_POINT('Ctrl Pts',(-5.400916269,4.820155008,5.203854673));
#152000=CARTESIAN_POINT('Origin',(0.16739088947738,4.55371943555998,-0.0927685709538006));
#152001=CARTESIAN_POINT('Ctrl Pts',(-6.305834896,4.820162746,3.577561496));
#152002=CARTESIAN_POINT('Ctrl Pts',(-6.111975772,4.755280647,3.919258944));
#152003=CARTESIAN_POINT('Ctrl Pts',(-5.88232872,4.690053947,4.238007649));
#152004=CARTESIAN_POINT('Ctrl Pts',(-5.87885701914578,4.68906787908345,
4.24282634857307));
#152005=CARTESIAN_POINT('Ctrl Pts',(-5.87538531829157,4.68808181116689,
4.24764504814613));
#152006=CARTESIAN_POINT('Ctrl Pts',(-6.6414424790535,4.820162746,3.48491831938665));
#152007=CARTESIAN_POINT('Ctrl Pts',(-6.45260345686075,4.755280647,3.84480150382246));
#152008=CARTESIAN_POINT('Ctrl Pts',(-6.22598200346879,4.690053947,4.18217192170176));
#152009=CARTESIAN_POINT('Ctrl Pts',(-6.22255604225364,4.68906787908345,
4.18727213595549));
#152010=CARTESIAN_POINT('Ctrl Pts',(-6.21913008103849,4.68808181116689,
4.19237235020922));
#152011=CARTESIAN_POINT('',(-6.3035275691543,4.81939092093462,3.58162539391593));
#152012=CARTESIAN_POINT('Origin',(0.162076923735922,4.69643187830107,-0.115490408366731));
#152013=CARTESIAN_POINT('Origin',(-12.6789187057329,5.70972183643974,7.49205957161615));
#152014=CARTESIAN_POINT('Ctrl Pts',(-6.655849513,4.690053947,2.874398591));
#152015=CARTESIAN_POINT('Ctrl Pts',(-6.49804789100001,4.755711878,3.239798106));
#152016=CARTESIAN_POINT('Ctrl Pts',(-6.301195022,4.820155008,3.585727442));
#152017=CARTESIAN_POINT('Ctrl Pts',(-6.784140134,4.690053947,3.197724603));
#152018=CARTESIAN_POINT('Ctrl Pts',(-6.608588236,4.755711878,3.570167146));
#152019=CARTESIAN_POINT('Ctrl Pts',(-6.393320778,4.820155008,3.921154095));
#152020=CARTESIAN_POINT('Origin',(0.183420107088528,4.55371942284746,-0.0546157082920951));
#152021=CARTESIAN_POINT('Ctrl Pts',(-6.92747795,4.820162746,2.138351993));
#152022=CARTESIAN_POINT('Ctrl Pts',(-6.811605995,4.755280647,2.513734725));
#152023=CARTESIAN_POINT('Ctrl Pts',(-6.655849513,4.690053947,2.874398591));
#152024=CARTESIAN_POINT('Ctrl Pts',(-6.65349485690423,4.68906787923068,
2.87985094431266));
#152025=CARTESIAN_POINT('Ctrl Pts',(-6.65114020080846,4.68808181146138,
2.88530329762533));
#152026=CARTESIAN_POINT('Ctrl Pts',(-7.23532366957013,4.820162746,1.97572905226316));
#152027=CARTESIAN_POINT('Ctrl Pts',(-7.12826384637026,4.755280647,2.36779317546382));
#152028=CARTESIAN_POINT('Ctrl Pts',(-6.97946534366401,4.690053947,2.74599297495909));
#152029=CARTESIAN_POINT('Ctrl Pts',(-6.97721587515433,4.68906787923068,
2.75171042858842));
#152030=CARTESIAN_POINT('Ctrl Pts',(-6.97496640664463,4.68808181146136,
2.75742788221773));
#152031=CARTESIAN_POINT('',(-6.92609818485928,4.81939092094391,2.14281688622834));
#152032=CARTESIAN_POINT('Origin',(0.183114619191084,4.69643185336553,-0.0779485369318891));
#152033=CARTESIAN_POINT('Origin',(-13.993262706542,5.7097470643807,4.59137507535894));
#152034=CARTESIAN_POINT('Ctrl Pts',(-7.118150181,4.690053947,1.376385849));
#152035=CARTESIAN_POINT('Ctrl Pts',(-7.042587967,4.755711878,1.767165211));
#152036=CARTESIAN_POINT('Ctrl Pts',(-6.924701991,4.820155008,2.147324459));
#152037=CARTESIAN_POINT('Ctrl Pts',(-7.312946974,4.690053947,1.664573988));
#152038=CARTESIAN_POINT('Ctrl Pts',(-7.22156351800001,4.755711878,2.0660475));
#152039=CARTESIAN_POINT('Ctrl Pts',(-7.086780713,4.820155008,2.455104709));
#152040=CARTESIAN_POINT('Origin',(0.190872296101794,4.55371947175156,-0.0139088517423921));
#152041=CARTESIAN_POINT('Ctrl Pts',(-7.225199835,4.820162746,0.599155527));
#152042=CARTESIAN_POINT('Ctrl Pts',(-7.192733093,4.755280647,0.990671065));
#152043=CARTESIAN_POINT('Ctrl Pts',(-7.118150181,4.690053947,1.376385849));
#152044=CARTESIAN_POINT('Ctrl Pts',(-7.11702267001631,4.68906787902937,
1.38221691195886));
#152045=CARTESIAN_POINT('Ctrl Pts',(-7.11589515903266,4.68808181105874,
1.38804797491772));
#152046=CARTESIAN_POINT('Ctrl Pts',(-7.49088916700958,4.820162746,0.374156890991696));
#152047=CARTESIAN_POINT('Ctrl Pts',(-7.47061453979235,4.755280647,0.780069469419929));
#152048=CARTESIAN_POINT('Ctrl Pts',(-7.40659664040584,4.690053947,1.18141444721225));
#152049=CARTESIAN_POINT('Ctrl Pts',(-7.40562884654026,4.68906787902937,
1.18748180042454));
#152050=CARTESIAN_POINT('Ctrl Pts',(-7.4046610526747,4.68808181105874,1.19354915363682));
#152051=CARTESIAN_POINT('',(-7.22481214736115,4.81939092093405,0.603812642471597));
#152052=CARTESIAN_POINT('Origin',(0.195589907817557,4.69643185065517,-0.0367618823269955));
#152053=CARTESIAN_POINT('Origin',(-14.6535586857437,5.70979310765313,1.47594165616264));
#152054=CARTESIAN_POINT('Ctrl Pts',(-7.24761405700001,4.690053947,-0.185985165));
#152055=CARTESIAN_POINT('Ctrl Pts',(-7.257824457,4.755711878,0.211901635));
#152056=CARTESIAN_POINT('Ctrl Pts',(-7.224417591,4.820155008,0.608514971));
#152057=CARTESIAN_POINT('Ctrl Pts',(-7.49980854000001,4.690053947,0.053589743));
#152058=CARTESIAN_POINT('Ctrl Pts',(-7.496866517,4.755711878,0.465321769));
#152059=CARTESIAN_POINT('Ctrl Pts',(-7.448870658,4.820155008,0.874257356));
#152060=CARTESIAN_POINT('Origin',(0.189399783009803,4.55371943452198,0.0274482381966176));
#152061=CARTESIAN_POINT('Ctrl Pts',(-7.185079405,4.820162746,-0.968056785));
#152062=CARTESIAN_POINT('Ctrl Pts',(-7.23753598500001,4.755280647,-0.578715273));
#152063=CARTESIAN_POINT('Ctrl Pts',(-7.247614057,4.690053947,-0.185985165));
#152064=CARTESIAN_POINT('Ctrl Pts',(-7.24776641279696,4.6890678788451,-0.18004804641253));
#152065=CARTESIAN_POINT('Ctrl Pts',(-7.24791876859394,4.68808181069019,
-0.174110927825061));
#152066=CARTESIAN_POINT('Ctrl Pts',(-7.39618901257076,4.820162746,-1.2449104313802));
#152067=CARTESIAN_POINT('Ctrl Pts',(-7.46364760078705,4.755280647,-0.844129417606408));
#152068=CARTESIAN_POINT('Ctrl Pts',(-7.48740371130746,4.690053947,-0.438405706039374));
#152069=CARTESIAN_POINT('Ctrl Pts',(-7.48776284558941,4.6890678788451,-0.432272155949239));
#152070=CARTESIAN_POINT('Ctrl Pts',(-7.48812197987134,4.68808181069019,
-0.426138605859105));
#152071=CARTESIAN_POINT('',(-7.18570192408644,4.81939092093424,-0.963425209266199));
#152072=CARTESIAN_POINT('Origin',(0.198919785553169,4.69643189437622,0.00614363754179073));
#152073=CARTESIAN_POINT('Origin',(-14.6279827186348,5.70976925426145,-1.70861569320879));
#152074=CARTESIAN_POINT('Ctrl Pts',(-7.038187555,4.690053947,-1.73965972));
#152075=CARTESIAN_POINT('Ctrl Pts',(-7.133693143,4.755711878,-1.353270226));
#152076=CARTESIAN_POINT('Ctrl Pts',(-7.186327454,4.820155008,-0.958748));
#152077=CARTESIAN_POINT('Ctrl Pts',(-7.335987395,4.690053947,-1.559900299));
#152078=CARTESIAN_POINT('Ctrl Pts',(-7.421624369,4.755711878,-1.157161891));
#152079=CARTESIAN_POINT('Ctrl Pts',(-7.46265969,4.820155008,-0.7474693));
#152080=CARTESIAN_POINT('Origin',(0.179071147294614,4.55371942552132,0.0675218736889965));
#152081=CARTESIAN_POINT('Ctrl Pts',(-6.808992648,4.820162746,-2.490003838));
#152082=CARTESIAN_POINT('Ctrl Pts',(-6.943919739,4.755280647,-2.121041529));
#152083=CARTESIAN_POINT('Ctrl Pts',(-7.038187555,4.690053947,-1.73965972));
#152084=CARTESIAN_POINT('Ctrl Pts',(-7.03961265330949,4.6890678791791,-1.7338941618876));
#152085=CARTESIAN_POINT('Ctrl Pts',(-7.04103775161898,4.68808181135819,
-1.72812860377519));
#152086=CARTESIAN_POINT('Ctrl Pts',(-6.95565128071148,4.820162746,-2.80576712519848));
#152087=CARTESIAN_POINT('Ctrl Pts',(-7.10768879513469,4.755280647,-2.42885775111912));
#152088=CARTESIAN_POINT('Ctrl Pts',(-7.21810810577893,4.690053947,-2.03772649589799));
#152089=CARTESIAN_POINT('Ctrl Pts',(-7.21977737509705,4.6890678791791,-2.03181355005648));
#152090=CARTESIAN_POINT('Ctrl Pts',(-7.22144664441517,4.68808181135819,
-2.02590060421497));
#152091=CARTESIAN_POINT('',(-6.81059626507071,4.819390920953,-2.48561436915926));
#152092=CARTESIAN_POINT('Origin',(0.192948563491753,4.69643189277552,0.0487619033756873));
#152093=CARTESIAN_POINT('Origin',(-13.9185422296696,5.7097552877665,-4.81320545378816));
#152094=CARTESIAN_POINT('Ctrl Pts',(-6.499663225,4.690053947,-3.211989719));
#152095=CARTESIAN_POINT('Ctrl Pts',(-6.675998265,4.755711878,-2.855164676));
#152096=CARTESIAN_POINT('Ctrl Pts',(-6.812212632,4.820155008,-2.481180981));
#152097=CARTESIAN_POINT('Ctrl Pts',(-6.829143632,4.690053947,-3.100451136));
#152098=CARTESIAN_POINT('Ctrl Pts',(-6.999355314,4.755711878,-2.725537947));
#152099=CARTESIAN_POINT('Ctrl Pts',(-7.12750304900001,4.820155008,-2.334245122));
#152100=CARTESIAN_POINT('Origin',(0.160369492462258,4.55371938751372,0.104438319995822));
#152101=CARTESIAN_POINT('Ctrl Pts',(-6.11452496300001,4.820162746,-3.895521079));
#152102=CARTESIAN_POINT('Ctrl Pts',(-6.32561352300001,4.755280647,-3.564190239));
#152103=CARTESIAN_POINT('Ctrl Pts',(-6.499663225,4.690053947,-3.211989719));
#152104=CARTESIAN_POINT('Ctrl Pts',(-6.50229443031012,4.68906787901235,
-3.20666530954798));
#152105=CARTESIAN_POINT('Ctrl Pts',(-6.50492563562025,4.6880818110247,-3.20134090009595));
#152106=CARTESIAN_POINT('Ctrl Pts',(-6.18987502456724,4.820162746,-4.23542926647455));
#152107=CARTESIAN_POINT('Ctrl Pts',(-6.41938236070255,4.755280647,-3.90001539587208));
#152108=CARTESIAN_POINT('Ctrl Pts',(-6.61130178712863,4.690053947,-3.54176546025212));
#152109=CARTESIAN_POINT('Ctrl Pts',(-6.61420313891565,4.68906787901235,
-3.53634959844873));
#152110=CARTESIAN_POINT('Ctrl Pts',(-6.61710449070265,4.68808181102469,
-3.53093373664535));
#152111=CARTESIAN_POINT('',(-6.11703469421881,4.81939092098298,-3.89157896362748));
#152112=CARTESIAN_POINT('Origin',(0.177955156142423,4.69643186978763,0.089100100086858));
#152113=CARTESIAN_POINT('Origin',(-12.5587322634811,5.70978015226369,-7.69292888315619));
#152114=CARTESIAN_POINT('Ctrl Pts',(-5.657221867,4.690053947,-4.534130649));
#152115=CARTESIAN_POINT('Ctrl Pts',(-5.906141128,4.755711878,-4.223554798));
#152116=CARTESIAN_POINT('Ctrl Pts',(-6.119566318,4.820155008,-3.887596697));
#152117=CARTESIAN_POINT('Ctrl Pts',(-6.002976704,4.690053947,-4.496028325));
#152118=CARTESIAN_POINT('Ctrl Pts',(-6.249804185,4.755711878,-4.166470877));
#152119=CARTESIAN_POINT('Ctrl Pts',(-6.459072287,4.820155008,-3.811874236));
#152120=CARTESIAN_POINT('Origin',(0.134168952170949,4.55371938671085,0.136471286468549));
#152121=CARTESIAN_POINT('Ctrl Pts',(-5.134148886,4.820162746,-5.118888084));
#152122=CARTESIAN_POINT('Ctrl Pts',(-5.411528649,4.755280647,-4.840681376));
#152123=CARTESIAN_POINT('Ctrl Pts',(-5.657221867,4.690053947,-4.534130649));
#152124=CARTESIAN_POINT('Ctrl Pts',(-5.66093614652675,4.68906787909637,
-4.52949635303336));
#152125=CARTESIAN_POINT('Ctrl Pts',(-5.66465042605351,4.68808181119276,
-4.52486205706673));
#152126=CARTESIAN_POINT('Ctrl Pts',(-5.13466709208506,4.820162746,-5.46704744287442));
#152127=CARTESIAN_POINT('Ctrl Pts',(-5.43091274263443,4.755280647,-5.18881265472693));
#152128=CARTESIAN_POINT('Ctrl Pts',(-5.69535834553527,4.690053947,-4.880195407032));
#152129=CARTESIAN_POINT('Ctrl Pts',(-5.69935611517983,4.68906787909637,
-4.87552987033527));
#152130=CARTESIAN_POINT('Ctrl Pts',(-5.70335388482441,4.68808181119276,
-4.87086433363855));
#152131=CARTESIAN_POINT('',(-5.13744737884062,4.81939092094632,-5.11557765092014));
#152132=CARTESIAN_POINT('Origin',(0.154640799092037,4.69643183018118,0.125272107351143));
#152133=CARTESIAN_POINT('Origin',(-10.611299383607,5.70977832312957,-10.2127662554641));
#152134=CARTESIAN_POINT('Ctrl Pts',(-4.550255102,4.690053947,-5.644260669));
#152135=CARTESIAN_POINT('Ctrl Pts',(-4.860119396,4.755711878,-5.394456192));
#152136=CARTESIAN_POINT('Ctrl Pts',(-5.14077588500001,4.820155008,-5.112232712));
#152137=CARTESIAN_POINT('Ctrl Pts',(-4.896117256,4.690053947,-5.681376225));
#152138=CARTESIAN_POINT('Ctrl Pts',(-5.208019157,4.755711878,-5.41258426));
#152139=CARTESIAN_POINT('Ctrl Pts',(-5.488622484,4.820155008,-5.11126434800001));
#152140=CARTESIAN_POINT('Origin',(0.101694846917463,4.55371946035496,0.162122973855));
#152141=CARTESIAN_POINT('Ctrl Pts',(-3.913705713,4.820162746,-6.102901571));
#152142=CARTESIAN_POINT('Ctrl Pts',(-4.24440671,4.755280647,-5.890827631));
#152143=CARTESIAN_POINT('Ctrl Pts',(-4.550255102,4.690053947,-5.644260669));
#152144=CARTESIAN_POINT('Ctrl Pts',(-4.55487878052238,4.68906787906646,
-5.6405331804915));
#152145=CARTESIAN_POINT('Ctrl Pts',(-4.55950245904475,4.68808181113291,
-5.63680569198298));
#152146=CARTESIAN_POINT('Ctrl Pts',(-3.83936783390739,4.820162746,-6.44303255698771));
#152147=CARTESIAN_POINT('Ctrl Pts',(-4.18849967985375,4.755280647,-6.23498680147196));
#152148=CARTESIAN_POINT('Ctrl Pts',(-4.51310627696747,4.690053947,-5.99043284123748));
#152149=CARTESIAN_POINT('Ctrl Pts',(-4.5180135336036,4.68906787906646,-5.98673578438489));
#152150=CARTESIAN_POINT('Ctrl Pts',(-4.52292079023975,4.68808181113291,
-5.9830387275323));
#152151=CARTESIAN_POINT('',(-3.91763873447699,4.81939092094378,-6.10037761276723));
#152152=CARTESIAN_POINT('Origin',(0.124095585144508,4.69643185631761,0.155586535597629));
#152153=CARTESIAN_POINT('Origin',(-8.16771175173436,5.70977057295254,-12.2550248833005));
#152154=CARTESIAN_POINT('Ctrl Pts',(-3.230523466,4.690053947,-6.49047133400001));
#152155=CARTESIAN_POINT('Ctrl Pts',(-3.586843883,4.755711878,-6.31311881));
#152156=CARTESIAN_POINT('Ctrl Pts',(-3.921608485,4.820155008,-6.097826407));
#152157=CARTESIAN_POINT('Ctrl Pts',(-3.560320807,4.690053947,-6.601069288));
#152158=CARTESIAN_POINT('Ctrl Pts',(-3.922712942,4.755711878,-6.405611219));
#152159=CARTESIAN_POINT('Ctrl Pts',(-4.261530793,4.820155008,-6.17165741900001));
#152160=CARTESIAN_POINT('Origin',(0.0644657034034357,4.55371945320907,0.180194127272911));
#152161=CARTESIAN_POINT('Ctrl Pts',(-2.510262011,4.820162746,-6.80155016400001));
#152162=CARTESIAN_POINT('Ctrl Pts',(-2.878821031,4.755280647,-6.665525334));
#152163=CARTESIAN_POINT('Ctrl Pts',(-3.230523466,4.690053947,-6.490471334));
#152164=CARTESIAN_POINT('Ctrl Pts',(-3.23584034540781,4.6890678790529,-6.48782494627211));
#152165=CARTESIAN_POINT('Ctrl Pts',(-3.24115722481561,4.68808181110582,
-6.48517855854421));
#152166=CARTESIAN_POINT('Ctrl Pts',(-2.36454400263469,4.820162746,-7.11774863001447));
#152167=CARTESIAN_POINT('Ctrl Pts',(-2.75023702718094,4.755280647,-6.98961989444871));
#152168=CARTESIAN_POINT('Ctrl Pts',(-3.11982637500247,4.690053947,-6.82056429338084));
#152169=CARTESIAN_POINT('Ctrl Pts',(-3.12541366072251,4.6890678790529,-6.81800858675319));
#152170=CARTESIAN_POINT('Ctrl Pts',(-3.13100094644254,4.68808181110579,
-6.81545288012554));
#152171=CARTESIAN_POINT('',(-2.51464565709642,4.81939092092416,-6.79993069751606));
#152172=CARTESIAN_POINT('Origin',(0.087747766164829,4.69643188494964,0.178625850837789));
#152173=CARTESIAN_POINT('Origin',(-5.34229045964354,5.70976774922248,-13.7243426394469));
#152174=CARTESIAN_POINT('Ctrl Pts',(-1.759736143,4.690053947,-7.03319477300001));
#152175=CARTESIAN_POINT('Ctrl Pts',(-2.145851537,4.755711878,-6.936587009));
#152176=CARTESIAN_POINT('Ctrl Pts',(-2.519071031,4.820155008,-6.798292516));
#152177=CARTESIAN_POINT('Ctrl Pts',(-2.058047714,4.690053947,-7.212103688));
#152178=CARTESIAN_POINT('Ctrl Pts',(-2.45398503,4.755711878,-7.099118916));
#152179=CARTESIAN_POINT('Ctrl Pts',(-2.835174659,4.820155008,-6.943470649));
#152180=CARTESIAN_POINT('Origin',(0.0242221099538867,4.55371947014683,0.189839453343754));
#152181=CARTESIAN_POINT('Ctrl Pts',(-0.989441248,4.820162746,-7.182165831));
#152182=CARTESIAN_POINT('Ctrl Pts',(-1.37862488,4.755280647,-7.12855048));
#152183=CARTESIAN_POINT('Ctrl Pts',(-1.759736143,4.690053947,-7.033194773));
#152184=CARTESIAN_POINT('Ctrl Pts',(-1.76549760821494,4.6890678796763,-7.03175322917209));
#152185=CARTESIAN_POINT('Ctrl Pts',(-1.77125907342988,4.68808181235263,
-7.03031168534417));
#152186=CARTESIAN_POINT('Ctrl Pts',(-0.779156721531463,4.820162746,-7.4596466868318));
#152187=CARTESIAN_POINT('Ctrl Pts',(-1.18337634817097,4.755280647,-7.41742612955641));
#152188=CARTESIAN_POINT('Ctrl Pts',(-1.58066685966322,4.690053947,-7.33177373946158));
#152189=CARTESIAN_POINT('Ctrl Pts',(-1.58667291533359,4.6890678796763,-7.33047888592662));
#152190=CARTESIAN_POINT('Ctrl Pts',(-1.59267897100398,4.68808181235263,
-7.32918403239166));
#152191=CARTESIAN_POINT('',(-0.994070543459548,4.81939092091392,-7.18152658034752));
#152192=CARTESIAN_POINT('Origin',(0.0472970145023902,4.69643190404216,0.193313016087062));
#152193=CARTESIAN_POINT('Origin',(-2.26709724430376,5.70979447745367,-14.5520995818287));
#152194=CARTESIAN_POINT('Ctrl Pts',(-0.206665513,4.690053947,-7.24705384000001));
#152195=CARTESIAN_POINT('Ctrl Pts',(-0.604521557,4.755711878,-7.235708109));
#152196=CARTESIAN_POINT('Ctrl Pts',(-0.998744615,4.820155008,-7.180878024));
#152197=CARTESIAN_POINT('Ctrl Pts',(-0.459542598,4.690053947,-7.485908135));
#152198=CARTESIAN_POINT('Ctrl Pts',(-0.870511505,4.755711878,-7.460679703));
#152199=CARTESIAN_POINT('Ctrl Pts',(-1.276248909,4.820155008,-7.390614908));
#152200=CARTESIAN_POINT('Origin',(-0.0171541142577276,4.55371940144747,
0.190607825220247));
#152201=CARTESIAN_POINT('Ctrl Pts',(0.577644689,4.820162746,-7.226951405));
#152202=CARTESIAN_POINT('Ctrl Pts',(0.186034238,4.755280647,-7.25825252900001));
#152203=CARTESIAN_POINT('Ctrl Pts',(-0.206665513,4.690053947,-7.24705384));
#152204=CARTESIAN_POINT('Ctrl Pts',(-0.212602171644338,4.68906787901444,
-7.24688454324418));
#152205=CARTESIAN_POINT('Ctrl Pts',(-0.218538830288674,4.6880818110289,
-7.24671524648837));
#152206=CARTESIAN_POINT('Ctrl Pts',(0.842663062086272,4.820162746,-7.4527399563928));
#152207=CARTESIAN_POINT('Ctrl Pts',(0.438817693973189,4.755280647,-7.49840176325853));
#152208=CARTESIAN_POINT('Ctrl Pts',(0.0324028813005472,4.690053947,-7.5001575948203));
#152209=CARTESIAN_POINT('Ctrl Pts',(0.0262588845073336,4.68906787901444,
-7.50018413869407));
#152210=CARTESIAN_POINT('Ctrl Pts',(0.0201148877141198,4.68808181102888,
-7.50021068256784));
#152211=CARTESIAN_POINT('',(0.572986204252882,4.81939092094349,-7.22732226279767));
#152212=CARTESIAN_POINT('Origin',(0.00463468354769389,4.69643187856393,
0.198960769951227));
#152213=CARTESIAN_POINT('Origin',(0.914164899364814,5.70976303909231,-14.6989833446639));
#152214=CARTESIAN_POINT('Ctrl Pts',(1.356068566,4.690053947,-7.122048725));
#152215=CARTESIAN_POINT('Ctrl Pts',(0.965075178000001,4.755711878,-7.19649554));
#152216=CARTESIAN_POINT('Ctrl Pts',(0.568281989,4.820155008,-7.227693656));
#152217=CARTESIAN_POINT('Ctrl Pts',(1.16045022,4.690053947,-7.409679837));
#152218=CARTESIAN_POINT('Ctrl Pts',(0.75366617,4.755711878,-7.473387399));
#152219=CARTESIAN_POINT('Ctrl Pts',(0.342352821,4.820155008,-7.49218222900001));
#152220=CARTESIAN_POINT('Origin',(-0.057728145566843,4.55371939146095,0.182464146260932));
#152221=CARTESIAN_POINT('Ctrl Pts',(2.117720602,4.820162746,-6.933812764));
#152222=CARTESIAN_POINT('Ctrl Pts',(1.741994603,4.755280647,-7.048566756));
#152223=CARTESIAN_POINT('Ctrl Pts',(1.356068566,4.690053947,-7.122048725));
#152224=CARTESIAN_POINT('Ctrl Pts',(1.35023430029195,4.68906787748777,-7.12315959415833));
#152225=CARTESIAN_POINT('Ctrl Pts',(1.3444000345839,4.68808180797554,-7.12427046331664));
#152226=CARTESIAN_POINT('Ctrl Pts',(2.42508085697513,4.820162746,-7.09735138887713));
#152227=CARTESIAN_POINT('Ctrl Pts',(2.04049310773383,4.755280647,-7.22876046452689));
#152228=CARTESIAN_POINT('Ctrl Pts',(1.64395750021218,4.690053947,-7.31784241626901));
#152229=CARTESIAN_POINT('Ctrl Pts',(1.63796284352882,4.68906787748777,-7.31918911933237));
#152230=CARTESIAN_POINT('Ctrl Pts',(1.63196818684546,4.68808180797554,-7.3205358223957));
#152231=CARTESIAN_POINT('',(2.11325075291932,4.81939092093509,-6.93517638828184));
#152232=CARTESIAN_POINT('Origin',(-0.0382443478991329,4.69643188114676,
0.195305453577753));
#152233=CARTESIAN_POINT('Origin',(4.05250436150527,5.7097037009075,-14.1583157295763));
#152234=CARTESIAN_POINT('Ctrl Pts',(2.855394386,4.690053947,-6.664024527));
#152235=CARTESIAN_POINT('Ctrl Pts',(2.489546071,4.755711878,-6.82078283800001));
#152236=CARTESIAN_POINT('Ctrl Pts',(2.108736358,4.820155008,-6.936550365));
#152237=CARTESIAN_POINT('Ctrl Pts',(2.726181675,4.690053947,-6.986983146));
#152238=CARTESIAN_POINT('Ctrl Pts',(2.342603253,4.755711878,-7.136647807));
#152239=CARTESIAN_POINT('Ctrl Pts',(1.944946514,4.820155008,-7.243423435));
#152240=CARTESIAN_POINT('Origin',(-0.0956029415668058,4.55371945245238,
0.165788556452092));
#152241=CARTESIAN_POINT('Ctrl Pts',(3.558774254,4.820162746,-6.31645674500001));
#152242=CARTESIAN_POINT('Ctrl Pts',(3.216501235,4.755280647,-6.509297835));
#152243=CARTESIAN_POINT('Ctrl Pts',(2.855394386,4.690053947,-6.664024527));
#152244=CARTESIAN_POINT('Ctrl Pts',(2.84993533537919,4.68906787914193,-6.66636361540654));
#152245=CARTESIAN_POINT('Ctrl Pts',(2.84447628475839,4.68808181128384,-6.66870270381308));
#152246=CARTESIAN_POINT('Ctrl Pts',(3.89410456666928,4.820162746,-6.41009855793305));
#152247=CARTESIAN_POINT('Ctrl Pts',(3.54675733240121,4.755280647,-6.62111036091056));
#152248=CARTESIAN_POINT('Ctrl Pts',(3.17864249231939,4.690053947,-6.79335306055965));
#152249=CARTESIAN_POINT('Ctrl Pts',(3.17307749804736,4.68906787914193,-6.79595694807676));
#152250=CARTESIAN_POINT('Ctrl Pts',(3.16751250377533,4.68808181128384,-6.79856083559384));
#152251=CARTESIAN_POINT('',(3.55470204576132,4.81939092093285,-6.31874937272934));
#152252=CARTESIAN_POINT('Origin',(-0.0793350926111663,4.69643185062215,
0.182517857647713));
#152253=CARTESIAN_POINT('Origin',(7.00174251657518,5.70979219759973,-12.9568246707818));
#152254=CARTESIAN_POINT('Ctrl Pts',(4.221205138,4.690053947,-5.894397949));
#152255=CARTESIAN_POINT('Ctrl Pts',(3.897608556,4.755711878,-6.12613791));
#152256=CARTESIAN_POINT('Ctrl Pts',(3.55058856,4.820155008,-6.321061689));
#152257=CARTESIAN_POINT('Ctrl Pts',(4.164439905,4.690053947,-6.237582888));
#152258=CARTESIAN_POINT('Ctrl Pts',(3.822002811,4.755711878,-6.466206494));
#152259=CARTESIAN_POINT('Ctrl Pts',(3.45659667,4.820155008,-6.655970212));
#152260=CARTESIAN_POINT('Origin',(-0.129007324901403,4.5537194263835,0.141360543891498));
#152261=CARTESIAN_POINT('Ctrl Pts',(4.833423576,4.820162746,-5.403750228));
#152262=CARTESIAN_POINT('Ctrl Pts',(4.540607845,4.755280647,-5.665661383));
#152263=CARTESIAN_POINT('Ctrl Pts',(4.221205138,4.690053947,-5.894397949));
#152264=CARTESIAN_POINT('Ctrl Pts',(4.21637655121232,4.68906787902086,-5.89785588575582));
#152265=CARTESIAN_POINT('Ctrl Pts',(4.21154796442465,4.68808181104171,-5.90131382251167));
#152266=CARTESIAN_POINT('Ctrl Pts',(5.18104427449542,4.820162746,-5.4231166428033));
#152267=CARTESIAN_POINT('Ctrl Pts',(4.88717912567789,4.755280647,-5.70386449521244));
#152268=CARTESIAN_POINT('Ctrl Pts',(4.56469769549388,4.690053947,-5.95121406428968));
#152269=CARTESIAN_POINT('Ctrl Pts',(4.55982256595072,4.68906787902086,-5.95495338407317));
#152270=CARTESIAN_POINT('Ctrl Pts',(4.55494743640757,4.68808181104171,-5.95869270385665));
#152271=CARTESIAN_POINT('',(4.82993942138855,4.81939092091076,-5.40686466020919));
#152272=CARTESIAN_POINT('Origin',(-0.116716233036883,4.69643189652617,0.161195976188948));
#152273=CARTESIAN_POINT('Origin',(9.62327638418686,5.70978009376185,-11.1486127013645));
#152274=CARTESIAN_POINT('Ctrl Pts',(5.38963702999999,4.690053947,-4.849155874));
#152275=CARTESIAN_POINT('Ctrl Pts',(5.123423198,4.755711878,-5.145041583));
#152276=CARTESIAN_POINT('Ctrl Pts',(4.826419186,4.820155008,-5.410007194));
#152277=CARTESIAN_POINT('Ctrl Pts',(5.407973553,4.690053947,-5.196520186));
#152278=CARTESIAN_POINT('Ctrl Pts',(5.122689766,4.755711878,-5.493412553));
#152279=CARTESIAN_POINT('Ctrl Pts',(4.806620207,4.820155008,-5.75729121900001));
#152280=CARTESIAN_POINT('Origin',(-0.156379662974808,4.55371942472877,0.110322979267742));
#152281=CARTESIAN_POINT('Ctrl Pts',(5.88206738500001,4.820162746,-4.238370357));
#152282=CARTESIAN_POINT('Ctrl Pts',(5.65240067800001,4.755280647,-4.557104901));
#152283=CARTESIAN_POINT('Ctrl Pts',(5.38963703000001,4.690053947,-4.849155874));
#152284=CARTESIAN_POINT('Ctrl Pts',(5.38566468745547,4.6890678791119,-4.85357096913988));
#152285=CARTESIAN_POINT('Ctrl Pts',(5.38169234491093,4.68808181122383,-4.85798606427976));
#152286=CARTESIAN_POINT('Ctrl Pts',(6.22572411048738,4.820162746,-4.18255582068996));
#152287=CARTESIAN_POINT('Ctrl Pts',(5.99908185506762,4.755280647,-4.51991226473341));
#152288=CARTESIAN_POINT('Ctrl Pts',(5.73731270770339,4.690053947,-4.83080291380854));
#152289=CARTESIAN_POINT('Ctrl Pts',(5.73335539957178,4.6890678791119,-4.83550281869043));
#152290=CARTESIAN_POINT('Ctrl Pts',(5.72939809144017,4.68808181122383,-4.84020272357233));
#152291=CARTESIAN_POINT('',(5.87933419816497,4.81939092091779,-4.24216096526778));
#152292=CARTESIAN_POINT('Origin',(-0.148639930760657,4.69643189193197,0.132336833229253));
#152293=CARTESIAN_POINT('Origin',(11.7947999796108,5.70976647600791,-8.8191591276217));
#152294=CARTESIAN_POINT('Ctrl Pts',(6.306055484,4.690053947,-3.577172659));
#152295=CARTESIAN_POINT('Ctrl Pts',(6.109672265,4.755711878,-3.92336883));
#152296=CARTESIAN_POINT('Ctrl Pts',(5.87657181600001,4.820155008,-4.245986775));
#152297=CARTESIAN_POINT('Ctrl Pts',(6.398636369,4.690053947,-3.912473977));
#152298=CARTESIAN_POINT('Ctrl Pts',(6.183845441,4.755711878,-4.263752746));
#152299=CARTESIAN_POINT('Ctrl Pts',(5.931891526,4.820155008,-4.589407688));
#152300=CARTESIAN_POINT('Origin',(-0.176439461085779,4.55371945041668,0.0741264761620436));
#152301=CARTESIAN_POINT('Ctrl Pts',(6.655672259,4.820162746,-2.874808998));
#152302=CARTESIAN_POINT('Ctrl Pts',(6.49989353800001,4.755280647,-3.235463259));
#152303=CARTESIAN_POINT('Ctrl Pts',(6.306055484,4.690053947,-3.577172659));
#152304=CARTESIAN_POINT('Ctrl Pts',(6.30312512740184,4.68906787905938,-3.58233846816018));
#152305=CARTESIAN_POINT('Ctrl Pts',(6.30019477080367,4.68808181111875,-3.58750427732035));
#152306=CARTESIAN_POINT('Ctrl Pts',(6.9792960067535,4.820162746,-2.74642333683019));
#152307=CARTESIAN_POINT('Ctrl Pts',(6.83047418407916,4.755280647,-3.12461396070996));
#152308=CARTESIAN_POINT('Ctrl Pts',(6.64165735389054,4.69005394700001,-3.48450878786627));
#152309=CARTESIAN_POINT('Ctrl Pts',(6.63880290589765,4.68906787905938,-3.48994951614247));
#152310=CARTESIAN_POINT('Ctrl Pts',(6.63594845790476,4.68808181111875,-3.49539024441867));
#152311=CARTESIAN_POINT('',(6.65381784207734,4.81939092093234,-2.87909853897346));
#152312=CARTESIAN_POINT('Origin',(-0.173613277267033,4.69643187308239,0.0972896797464246));
#152313=CARTESIAN_POINT('Origin',(13.4152092529715,5.70979856953057,-6.07757981371294));
#152314=CARTESIAN_POINT('Ctrl Pts',(6.927609792,4.690053947,-2.137924827));
#152315=CARTESIAN_POINT('Ctrl Pts',(6.81023984700001,4.755711878,-2.518243711));
#152316=CARTESIAN_POINT('Ctrl Pts',(6.651942479,4.820155008,-2.883428734));
#152317=CARTESIAN_POINT('Ctrl Pts',(7.090106059,4.690053947,-2.445484832));
#152318=CARTESIAN_POINT('Ctrl Pts',(6.955851376,4.755711878,-2.8347246));
#152319=CARTESIAN_POINT('Ctrl Pts',(6.779794189,4.820155008,-3.206928554));
#152320=CARTESIAN_POINT('Origin',(-0.188249734327377,4.55371942637612,0.0344642920532923));
#152321=CARTESIAN_POINT('Ctrl Pts',(7.118065296,4.820162746,-1.376824766));
#152322=CARTESIAN_POINT('Ctrl Pts',(7.0434586,4.755280647,-1.762534951));
#152323=CARTESIAN_POINT('Ctrl Pts',(6.927609792,4.690053947,-2.137924827));
#152324=CARTESIAN_POINT('Ctrl Pts',(6.92585844207668,4.68906787922757,-2.14359980149389));
#152325=CARTESIAN_POINT('Ctrl Pts',(6.92410709215334,4.68808181145512,-2.1492747759878));
#152326=CARTESIAN_POINT('Ctrl Pts',(7.4065237781206,4.820162746,-1.18187115117692));
#152327=CARTESIAN_POINT('Ctrl Pts',(7.34248113186987,4.755280647,-1.58321218054904));
#152328=CARTESIAN_POINT('Ctrl Pts',(7.23544548359059,4.690053947,-1.97528290426303));
#152329=CARTESIAN_POINT('Ctrl Pts',(7.23382736703296,4.68906787922757,-1.98121005227403));
#152330=CARTESIAN_POINT('Ctrl Pts',(7.23220925047533,4.68808181145512,-1.98713720028501));
#152331=CARTESIAN_POINT('',(7.11717635827304,4.81939092091954,-1.38141266451028));
#152332=CARTESIAN_POINT('Origin',(-0.190468596064708,4.69643185312465,0.0576933420284076));
#152333=CARTESIAN_POINT('Origin',(14.4079253287426,5.7097819075629,-3.05158571821218));
#152334=CARTESIAN_POINT('Ctrl Pts',(7.225236766,4.690053947,-0.598710006));
#152335=CARTESIAN_POINT('Ctrl Pts',(7.192368183,4.755711878,-0.995368314));
#152336=CARTESIAN_POINT('Ctrl Pts',(7.11627570400001,4.820155008,-1.386044769));
#152337=CARTESIAN_POINT('Ctrl Pts',(7.450050271,4.690053947,-0.864147535));
#152338=CARTESIAN_POINT('Ctrl Pts',(7.402609431,4.755711878,-1.273147882));
#152339=CARTESIAN_POINT('Ctrl Pts',(7.310681212,4.820155008,-1.674497005));
#152340=CARTESIAN_POINT('Origin',(-0.191257348511611,4.55371940857812,-0.00680959593364436));
#152341=CARTESIAN_POINT('Ctrl Pts',(7.24762551100001,4.820162746,0.185538262));
#152342=CARTESIAN_POINT('Ctrl Pts',(7.257679367,4.755280647,-0.207192467));
#152343=CARTESIAN_POINT('Ctrl Pts',(7.225236766,4.690053947,-0.598710006));
#152344=CARTESIAN_POINT('Ctrl Pts',(7.22474631313992,4.68906787866448,-0.604628794594373));
#152345=CARTESIAN_POINT('Ctrl Pts',(7.22425586027986,4.68808181032895,-0.610547583188746));
#152346=CARTESIAN_POINT('Ctrl Pts',(7.48743073003761,4.820162746,0.437944016577193));
#152347=CARTESIAN_POINT('Ctrl Pts',(7.51116182282811,4.755280647,0.0322188422676525));
#152348=CARTESIAN_POINT('Ctrl Pts',(7.49091222439734,4.69005394700001,-0.373694986478134));
#152349=CARTESIAN_POINT('Ctrl Pts',(7.49060609994492,4.68906787866448,-0.37983141179899));
#152350=CARTESIAN_POINT('Ctrl Pts',(7.49029997549253,4.68808181032895,-0.385967837119846));
#152351=CARTESIAN_POINT('',(7.24774361911353,4.81939092094578,0.180866530701085));
#152352=CARTESIAN_POINT('Origin',(-0.198417961527672,4.69643188297084,0.0153993912038071));
#152353=CARTESIAN_POINT('Origin',(14.7269736395706,5.70976965717986,0.117037973839281));
#152354=CARTESIAN_POINT('Ctrl Pts',(7.185019699,4.690053947,0.96849983));
#152355=CARTESIAN_POINT('Ctrl Pts',(7.238189376,4.755711878,0.574049398));
#152356=CARTESIAN_POINT('Ctrl Pts',(7.247859787,4.820155008,0.176149108));
#152357=CARTESIAN_POINT('Ctrl Pts',(7.461638412,4.690053947,0.75759634));
#152358=CARTESIAN_POINT('Ctrl Pts',(7.503229697,4.755711878,0.347959816));
#152359=CARTESIAN_POINT('Ctrl Pts',(7.499728906,4.820155008,-0.063767838));
#152360=CARTESIAN_POINT('Origin',(-0.185321689466242,4.55371943528727,-0.0477650473182711));
#152361=CARTESIAN_POINT('Ctrl Pts',(7.038294813,4.820162746,1.739225727));
#152362=CARTESIAN_POINT('Ctrl Pts',(7.13253911200001,4.755280647,1.357838106));
#152363=CARTESIAN_POINT('Ctrl Pts',(7.18501969900001,4.690053947,0.96849983));
#152364=CARTESIAN_POINT('Ctrl Pts',(7.18581307694984,4.68906787903698,0.962613988761047));
#152365=CARTESIAN_POINT('Ctrl Pts',(7.1866064548997,4.68808181107395,0.956728147522092));
#152366=CARTESIAN_POINT('Ctrl Pts',(7.21823374226126,4.820162746,2.03728140900129));
#152367=CARTESIAN_POINT('Ctrl Pts',(7.3286289343689,4.755280647,1.64614334688791));
#152368=CARTESIAN_POINT('Ctrl Pts',(7.39611223521212,4.690053947,1.24536649294527));
#152369=CARTESIAN_POINT('Ctrl Pts',(7.39713241745345,4.68906787903698,1.23930772842104));
#152370=CARTESIAN_POINT('Ctrl Pts',(7.39815259969477,4.68808181107395,1.23324896389681));
#152371=CARTESIAN_POINT('',(7.03941444328107,4.81939092092237,1.73468860818569));
#152372=CARTESIAN_POINT('Origin',(-0.197089488305159,4.69643185279569,-0.0276146278634712));
#152373=CARTESIAN_POINT('Origin',(14.3578677079183,5.70980883046184,3.28024211300596));
#152374=CARTESIAN_POINT('Ctrl Pts',(6.808839097,4.690053947,2.49042369));
#152375=CARTESIAN_POINT('Ctrl Pts',(6.945560879,4.755711878,2.116625199));
#152376=CARTESIAN_POINT('Ctrl Pts',(7.040542002,4.820155008,1.730106449));
#152377=CARTESIAN_POINT('Ctrl Pts',(7.124328633,4.690053947,2.343915853));
#152378=CARTESIAN_POINT('Ctrl Pts',(7.253007281,4.755711878,1.9527973));
#152379=CARTESIAN_POINT('Ctrl Pts',(7.33809761200001,4.820155008,1.549943043));
#152380=CARTESIAN_POINT('Origin',(-0.170721269218758,4.55371942967028,-0.086487117622841));
#152381=CARTESIAN_POINT('Ctrl Pts',(6.499861271,4.820162746,3.211588931));
#152382=CARTESIAN_POINT('Ctrl Pts',(6.673889256,4.755280647,2.859377679));
#152383=CARTESIAN_POINT('Ctrl Pts',(6.808839097,4.690053947,2.49042369));
#152384=CARTESIAN_POINT('Ctrl Pts',(6.81087920812824,4.68906787902435,2.4848460091877));
#152385=CARTESIAN_POINT('Ctrl Pts',(6.81291931925649,4.68808181104872,2.47926832837541));
#152386=CARTESIAN_POINT('Ctrl Pts',(6.61152016733784,4.820162746,3.54135778708215));
#152387=CARTESIAN_POINT('Ctrl Pts',(6.80341750242848,4.755280647,3.18309601847626));
#152388=CARTESIAN_POINT('Ctrl Pts',(6.95547825829419,4.690053947,2.80619601934055));
#152389=CARTESIAN_POINT('Ctrl Pts',(6.95777704455368,4.68906787902435,2.80049821431333));
#152390=CARTESIAN_POINT('Ctrl Pts',(6.96007583081316,4.68808181104872,2.79480040928613));
#152391=CARTESIAN_POINT('',(6.50193007160717,4.81939092090431,3.20739857423919));
#152392=CARTESIAN_POINT('Origin',(-0.186545351912871,4.69643183132373,-0.0693374519902629));
#152393=CARTESIAN_POINT('Origin',(13.3169049274491,5.709797452772,6.2900119976216));
#152394=CARTESIAN_POINT('Ctrl Pts',(6.114284746,4.690053947,3.895898106));
#152395=CARTESIAN_POINT('Ctrl Pts',(6.328165675,4.755711878,3.560229957));
#152396=CARTESIAN_POINT('Ctrl Pts',(6.50401629700001,4.820155008,3.203165935));
#152397=CARTESIAN_POINT('Ctrl Pts',(6.453893166,4.690053947,3.820636465));
#152398=CARTESIAN_POINT('Ctrl Pts',(6.663642306,4.755711878,3.466324153));
#152399=CARTESIAN_POINT('Ctrl Pts',(6.83334502900001,4.820155008,3.09118031));
#152400=CARTESIAN_POINT('Origin',(-0.148137647083667,4.55371941171401,-0.121165073524416));
#152401=CARTESIAN_POINT('Ctrl Pts',(5.65750144,4.820162746,4.533781805));
#152402=CARTESIAN_POINT('Ctrl Pts',(5.903175755,4.755280647,4.227215929));
#152403=CARTESIAN_POINT('Ctrl Pts',(6.114284746,4.690053947,3.895898106));
#152404=CARTESIAN_POINT('Ctrl Pts',(6.11747619650953,4.68906787916857,3.89088939258605));
#152405=CARTESIAN_POINT('Ctrl Pts',(6.12066764701905,4.68808181133714,3.88588067917208));
#152406=CARTESIAN_POINT('Ctrl Pts',(5.69565925764326,4.820162746,4.87984421090298));
#152407=CARTESIAN_POINT('Ctrl Pts',(5.96008583042904,4.755280647,4.57121065817288));
#152408=CARTESIAN_POINT('Ctrl Pts',(6.18961384778584,4.690053947,4.23581093858657));
#152409=CARTESIAN_POINT('Ctrl Pts',(6.19308374882831,4.68906787916857,4.23074051690108));
#152410=CARTESIAN_POINT('Ctrl Pts',(6.19655364987078,4.68808181133714,4.22567009521558));
#152411=CARTESIAN_POINT('',(5.66042267628095,4.81939092091094,4.53013414754876));
#152412=CARTESIAN_POINT('Origin',(-0.167278715930961,4.69643185358206,-0.107818263156557));
#152413=CARTESIAN_POINT('Origin',(11.6532789256992,5.70978109174142,9.00560699204281));
#152414=CARTESIAN_POINT('Ctrl Pts',(5.133833235,4.690053947,5.119204656));
#152415=CARTESIAN_POINT('Ctrl Pts',(5.414872477,4.755711878,4.83736232));
#152416=CARTESIAN_POINT('Ctrl Pts',(5.663370019,4.820155008,4.526448942));
#152417=CARTESIAN_POINT('Ctrl Pts',(5.481680828,4.690053947,5.11870836300001));
#152418=CARTESIAN_POINT('Ctrl Pts',(5.762692823,4.755711878,4.81776954));
#152419=CARTESIAN_POINT('Ctrl Pts',(6.00907282800001,4.820155008,4.487877421));
#152420=CARTESIAN_POINT('Origin',(-0.118627120782181,4.55371940082309,-0.150177319917639));
#152421=CARTESIAN_POINT('Ctrl Pts',(4.55060313,4.820162746,5.643980081));
#152422=CARTESIAN_POINT('Ctrl Pts',(4.856436318,4.755280647,5.39739426));
#152423=CARTESIAN_POINT('Ctrl Pts',(5.133833235,4.690053947,5.119204656));
#152424=CARTESIAN_POINT('Ctrl Pts',(5.13802679694443,4.68906787905865,5.1149991105697));
#152425=CARTESIAN_POINT('Ctrl Pts',(5.14222035888887,4.68808181111733,5.1107935651394));
#152426=CARTESIAN_POINT('Ctrl Pts',(4.51347565108401,4.820162746,5.99015454228934));
#152427=CARTESIAN_POINT('Ctrl Pts',(4.83806716830898,4.755280647,5.74558056701959));
#152428=CARTESIAN_POINT('Ctrl Pts',(5.13432997385987,4.690053947,5.46736404691458));
#152429=CARTESIAN_POINT('Ctrl Pts',(5.13880874183013,4.68906787905865,5.46315809457868));
#152430=CARTESIAN_POINT('Ctrl Pts',(5.1432875098004,4.68808181111732,5.4589521422428));
#152431=CARTESIAN_POINT('',(4.55424020817694,4.81939092093594,5.64104568324374));
#152432=CARTESIAN_POINT('Origin',(-0.140189866127276,4.69643190112113,-0.141257248052444));
#152433=CARTESIAN_POINT('Origin',(9.44493727481165,5.70978234778588,11.3002261614088));
#152434=CARTESIAN_POINT('Ctrl Pts',(3.913329389,4.690053947,6.103142887));
#152435=CARTESIAN_POINT('Ctrl Pts',(4.24838586,4.755711878,5.888304997));
#152436=CARTESIAN_POINT('Ctrl Pts',(4.557910854,4.820155008,5.638080227));
#152437=CARTESIAN_POINT('Ctrl Pts',(4.253151186,4.690053947,6.177435146));
#152438=CARTESIAN_POINT('Ctrl Pts',(4.592286229,4.755711878,5.943941379));
#152439=CARTESIAN_POINT('Ctrl Pts',(4.903823059,4.820155008,5.674726372));
#152440=CARTESIAN_POINT('Origin',(-0.0835701931440092,4.55371943129,-0.172167829194979));
#152441=CARTESIAN_POINT('Ctrl Pts',(3.230923675,4.820162746,6.490272121));
#152442=CARTESIAN_POINT('Ctrl Pts',(3.582615315,4.755280647,6.315196435));
#152443=CARTESIAN_POINT('Ctrl Pts',(3.913329389,4.690053947,6.10314288700001));
#152444=CARTESIAN_POINT('Ctrl Pts',(3.91832898283825,4.68906787766383,6.09993715221183));
#152445=CARTESIAN_POINT('Ctrl Pts',(3.9233285766765,4.68808180832766,6.09673141742365));
#152446=CARTESIAN_POINT('Ctrl Pts',(3.12024693920707,4.820162746,6.82037190556698));
#152447=CARTESIAN_POINT('Ctrl Pts',(3.48982586236426,4.755280647,6.65129351551268));
#152448=CARTESIAN_POINT('Ctrl Pts',(3.83897053609471,4.690053947,6.44326928801588));
#152449=CARTESIAN_POINT('Ctrl Pts',(3.84424875585212,4.68906787766383,6.44012446677068));
#152450=CARTESIAN_POINT('Ctrl Pts',(3.84952697560952,4.68808180832766,6.4369796455255));
#152451=CARTESIAN_POINT('',(3.23510652906402,4.81939092093346,6.48818819268238));
#152452=CARTESIAN_POINT('Origin',(-0.106546362737626,4.69643187539504,-0.168091752984815));
#152453=CARTESIAN_POINT('Origin',(6.79478071579461,5.70975708926279,13.0661840777453));
#152454=CARTESIAN_POINT('Ctrl Pts',(2.509842609,4.690053947,6.801704939));
#152455=CARTESIAN_POINT('Ctrl Pts',(2.883249442,4.755711878,6.663917077));
#152456=CARTESIAN_POINT('Ctrl Pts',(3.239328843,4.820155008,6.486081147));
#152457=CARTESIAN_POINT('Ctrl Pts',(2.825748922,4.690053947,6.947311928));
#152458=CARTESIAN_POINT('Ctrl Pts',(3.207149434,4.755711878,6.792181124));
#152459=CARTESIAN_POINT('Ctrl Pts',(3.569275975,4.820155008,6.596231425));
#152460=CARTESIAN_POINT('Origin',(-0.0446053174623445,4.55371940454967,
-0.186107667785016));
#152461=CARTESIAN_POINT('Ctrl Pts',(1.76016982,4.820162746,7.03308625));
#152462=CARTESIAN_POINT('Ctrl Pts',(2.141275202,4.755280647,6.93770704300001));
#152463=CARTESIAN_POINT('Ctrl Pts',(2.509842609,4.690053947,6.801704939));
#152464=CARTESIAN_POINT('Ctrl Pts',(2.5154144445643,4.68906787921457,6.79964892062862));
#152465=CARTESIAN_POINT('Ctrl Pts',(2.5209862801286,4.68808181142913,6.79759290225721));
#152466=CARTESIAN_POINT('Ctrl Pts',(1.58111894904948,4.820162746,7.33167625852239));
#152467=CARTESIAN_POINT('Ctrl Pts',(1.97840417808707,4.755280647,7.24599937154038));
#152468=CARTESIAN_POINT('Ctrl Pts',(2.36410510319515,4.690053947,7.11789441891999));
#152469=CARTESIAN_POINT('Ctrl Pts',(2.3699359555464,4.68906787921457,7.11595778611574));
#152470=CARTESIAN_POINT('Ctrl Pts',(2.37576680789764,4.68808181142913,7.1140211533115));
#152471=CARTESIAN_POINT('',(1.76470286420027,4.81939092092281,7.03195023221659));
#152472=CARTESIAN_POINT('Origin',(-0.0679205185731391,4.69643185801115,
-0.187065872027213));
#152473=CARTESIAN_POINT('Origin',(3.8271353988825,5.70978052766214,14.2215713472656));
#152474=CARTESIAN_POINT('Ctrl Pts',(0.988998379000001,4.690053947,7.182226828));
#152475=CARTESIAN_POINT('Ctrl Pts',(1.383295485,4.755711878,7.127931801));
#152476=CARTESIAN_POINT('Ctrl Pts',(1.769279415,4.820155008,7.030800122));
#152477=CARTESIAN_POINT('Ctrl Pts',(1.266217779,4.690053947,7.392340126));
#152478=CARTESIAN_POINT('Ctrl Pts',(1.672049896,4.755711878,7.32282603));
#152479=CARTESIAN_POINT('Ctrl Pts',(2.067833513,4.820155008,7.209304028));
#152480=CARTESIAN_POINT('Origin',(-0.00355486453146994,4.55371941173134,
-0.191345552622352));
#152481=CARTESIAN_POINT('Ctrl Pts',(0.207112381,4.820162746,7.247041083));
#152482=CARTESIAN_POINT('Ctrl Pts',(0.599811441,4.755280647,7.23581818000001));
#152483=CARTESIAN_POINT('Ctrl Pts',(0.988998379000001,4.690053947,7.182226828));
#152484=CARTESIAN_POINT('Ctrl Pts',(0.994881931555155,4.68906787917506,
7.18141665811707));
#152485=CARTESIAN_POINT('Ctrl Pts',(1.00076548411031,4.6880818113501,7.18060648823417));
#152486=CARTESIAN_POINT('Ctrl Pts',(-0.0319404063266016,4.820162746,7.50015957902518));
#152487=CARTESIAN_POINT('Ctrl Pts',(0.374474513060617,4.755280647,7.5018903498288));
#152488=CARTESIAN_POINT('Ctrl Pts',(0.778696743080096,4.690053947,7.45969471738953));
#152489=CARTESIAN_POINT('Ctrl Pts',(0.784807592397145,4.68906787917506,
7.45905682285399));
#152490=CARTESIAN_POINT('Ctrl Pts',(0.790918441714193,4.6880818113501,7.45841892831845));
#152491=CARTESIAN_POINT('',(0.211783654676978,4.81939092020425,7.24690609579801));
#152492=CARTESIAN_POINT('Origin',(-0.0261189597364792,4.69643185026277,
-0.197293460334176));
#152493=CARTESIAN_POINT('Origin',(0.680450293923213,5.7097907178076,14.7119349338605));
#152494=CARTESIAN_POINT('Ctrl Pts',(-0.578090317,4.690053947,7.226915773));
#152495=CARTESIAN_POINT('Ctrl Pts',(-0.181339832,4.755711878,7.258652356));
#152496=CARTESIAN_POINT('Ctrl Pts',(0.216500448,4.820155008,7.246766697));
#152497=CARTESIAN_POINT('Ctrl Pts',(-0.3525203,4.690053947,7.49171071500001));
#152498=CARTESIAN_POINT('Ctrl Pts',(0.058767163,4.755711878,7.511063729));
#152499=CARTESIAN_POINT('Ctrl Pts',(0.469701454000001,4.820155008,7.485277586));
#152500=CARTESIAN_POINT('Origin',(0.0376619171070517,4.55371932361627,-0.187635523132965));
#152501=CARTESIAN_POINT('Ctrl Pts',(0.208106472,1.198733649,7.247012605));
#152502=CARTESIAN_POINT('Ctrl Pts',(0.602872113000001,1.134619049,7.235676446));
#152503=CARTESIAN_POINT('Ctrl Pts',(0.994070541,1.069390921,7.181526562));
#152504=CARTESIAN_POINT('Ctrl Pts',(0.997993468314819,1.06873681508671,
7.1809835484196));
#152505=CARTESIAN_POINT('Ctrl Pts',(1.00191639562964,1.06808270917341,7.18044053483919));
#152506=CARTESIAN_POINT('Ctrl Pts',(-0.030697537,1.198733649,7.499937177));
#152507=CARTESIAN_POINT('Ctrl Pts',(0.377845634,1.134619049,7.50160936));
#152508=CARTESIAN_POINT('Ctrl Pts',(0.784153080000001,1.069390921,7.458894285));
#152509=CARTESIAN_POINT('Ctrl Pts',(0.788227520140971,1.06873681508671,
7.45846593937671));
#152510=CARTESIAN_POINT('Ctrl Pts',(0.792301960281942,1.06808270917341,
7.45803759375342));
#152511=CARTESIAN_POINT('',(0.221348494829952,1.15903910584966,7.4967329445143));
#152512=CARTESIAN_POINT('',(0.784153071897506,1.06939091992727,7.45889428272056));
#152513=CARTESIAN_POINT('Origin',(-0.0390445917594759,0.94650929176938,
-0.183409434795353));
#152514=CARTESIAN_POINT('',(0.889111791278134,1.06939091791718,7.32021042583469));
#152515=CARTESIAN_POINT('Ctrl Pts',(0.221348496723335,1.15903910498851,
7.49673294432665));
#152516=CARTESIAN_POINT('Ctrl Pts',(0.220029630850789,1.16522285270462,
7.45504792860251));
#152517=CARTESIAN_POINT('Ctrl Pts',(0.218659615824573,1.1715546145733,7.41336222418238));
#152518=CARTESIAN_POINT('Ctrl Pts',(0.215810430745453,1.18452221944203,
7.33009059228574));
#152519=CARTESIAN_POINT('Ctrl Pts',(0.214329599541364,1.19116565504539,
7.28845588949761));
#152520=CARTESIAN_POINT('Ctrl Pts',(0.212788495890653,1.19797317326339,
7.24687664196839));
#152521=CARTESIAN_POINT('Ctrl Pts',(0.986271382025894,1.06811592995212,
7.18260612530439));
#152522=CARTESIAN_POINT('Ctrl Pts',(0.990170961512947,1.06875342547606,
7.18206634365219));
#152523=CARTESIAN_POINT('Ctrl Pts',(0.994070541000001,1.069390921,7.18152656200001));
#152524=CARTESIAN_POINT('Ctrl Pts',(1.000303954,1.070409947,7.18066373));
#152525=CARTESIAN_POINT('Ctrl Pts',(1.00653586,1.071428571,7.179790078));
#152526=CARTESIAN_POINT('Ctrl Pts',(1.392414954,1.134501699,7.125693629));
#152527=CARTESIAN_POINT('Ctrl Pts',(1.770273114,1.198754474,7.030549986));
#152528=CARTESIAN_POINT('Ctrl Pts',(1.26341113293498,1.06811592995212,7.39282480932989));
#152529=CARTESIAN_POINT('Ctrl Pts',(1.26742469796749,1.06875342547606,7.39213441616495));
#152530=CARTESIAN_POINT('Ctrl Pts',(1.271438263,1.069390921,7.391444023));
#152531=CARTESIAN_POINT('Ctrl Pts',(1.27785388,1.070409947,7.39034044099999));
#152532=CARTESIAN_POINT('Ctrl Pts',(1.284267572,1.071428571,7.389225724));
#152533=CARTESIAN_POINT('Ctrl Pts',(1.681402823,1.134501699,7.320202535));
#152534=CARTESIAN_POINT('Ctrl Pts',(2.068852438,1.198754474,7.209011693));
#152535=CARTESIAN_POINT('',(1.27143827033051,1.06939091911159,7.39144401914332));
#152536=CARTESIAN_POINT('',(1.82774947115441,1.15903910585546,7.27388011096424));
#152537=CARTESIAN_POINT('Origin',(-0.0717256750925657,1.3383840921539,-0.168465344956257));
#152538=CARTESIAN_POINT('Ctrl Pts',(1.76567788092872,1.19797317330302,7.0317054563247));
#152539=CARTESIAN_POINT('Ctrl Pts',(1.77612131102255,1.19116562418267,7.07198149530744));
#152540=CARTESIAN_POINT('Ctrl Pts',(1.78651780332373,1.18452215733789,7.11232467093176));
#152541=CARTESIAN_POINT('Ctrl Pts',(1.80720121631984,1.17155461457357,7.19303658126377));
#152542=CARTESIAN_POINT('Ctrl Pts',(1.81750039536026,1.16522285269688,7.23345318439212));
#152543=CARTESIAN_POINT('Ctrl Pts',(1.82774947299082,1.15903910498863,7.27388011036608));
#152544=CARTESIAN_POINT('',(1.13275441898507,1.06939091820872,7.28648528985951));
#152545=CARTESIAN_POINT('Origin',(-1.01047642475649E-13,1.16011713399994,
-1.66967134562768E-13));
#152546=CARTESIAN_POINT('',(1.82142216213811,0.979367659149596,7.27546708527639));
#152547=CARTESIAN_POINT('Origin',(-0.0517297820971196,0.94643634185441,
-0.184811503852839));
#152548=CARTESIAN_POINT('',(2.36926179550939,1.06939091992739,7.115939747572));
#152549=CARTESIAN_POINT('Origin',(-0.0169371445751124,0.803756644740858,
-0.182664612580321));
#152550=CARTESIAN_POINT('Origin',(-0.0775593148305506,0.946509321505581,
-0.1707278100195));
#152551=CARTESIAN_POINT('Ctrl Pts',(1.761134548,1.198733649,7.032844738));
#152552=CARTESIAN_POINT('Ctrl Pts',(2.144233849,1.134619049,6.93691066800001));
#152553=CARTESIAN_POINT('Ctrl Pts',(2.51464565,1.069390921,6.79993068));
#152554=CARTESIAN_POINT('Ctrl Pts',(2.51836012957831,1.06873681508671,6.79855704836438));
#152555=CARTESIAN_POINT('Ctrl Pts',(2.52207460915663,1.06808270917341,6.79718341672874));
#152556=CARTESIAN_POINT('Ctrl Pts',(1.582284951,1.198733649,7.331191877));
#152557=CARTESIAN_POINT('Ctrl Pts',(1.981636079,1.134619049,7.24500026));
#152558=CARTESIAN_POINT('Ctrl Pts',(2.369261804,1.069390921,7.115939748));
#152559=CARTESIAN_POINT('Ctrl Pts',(2.37314890434522,1.06873681508671,7.1146455326567));
#152560=CARTESIAN_POINT('Ctrl Pts',(2.37703600469044,1.06808270917341,7.11335131731341));
#152561=CARTESIAN_POINT('',(2.44195370872946,1.06939091791719,6.95793522041222));
#152562=CARTESIAN_POINT('Ctrl Pts',(2.50726090509695,1.06811592995267,6.80266159234607));
#152563=CARTESIAN_POINT('Ctrl Pts',(2.51095327754848,1.06875342547634,6.80129613617304));
#152564=CARTESIAN_POINT('Ctrl Pts',(2.51464565,1.069390921,6.79993068));
#152565=CARTESIAN_POINT('Ctrl Pts',(2.520547846,1.070409947,6.797748021));
#152566=CARTESIAN_POINT('Ctrl Pts',(2.526446244,1.071428571,6.795555119));
#152567=CARTESIAN_POINT('Ctrl Pts',(2.891674563,1.134501699,6.659770816));
#152568=CARTESIAN_POINT('Ctrl Pts',(3.240245538,1.198754474,6.485623243));
#152569=CARTESIAN_POINT('Ctrl Pts',(2.82311208693778,1.06811592995267,6.94838862489811));
#152570=CARTESIAN_POINT('Ctrl Pts',(2.82688340296889,1.06875342547634,6.94685157544905));
#152571=CARTESIAN_POINT('Ctrl Pts',(2.830654719,1.069390921,6.945314526));
#152572=CARTESIAN_POINT('Ctrl Pts',(2.836683105,1.070409947,6.942857578));
#152573=CARTESIAN_POINT('Ctrl Pts',(2.842707217,1.071428571,6.940390168));
#152574=CARTESIAN_POINT('Ctrl Pts',(3.21571972,1.134501699,6.787608363));
#152575=CARTESIAN_POINT('Ctrl Pts',(3.570208235,1.198754474,6.595726886));
#152576=CARTESIAN_POINT('',(2.83065472529928,1.069390919111,6.94531452062289));
#152577=CARTESIAN_POINT('',(3.34868691359671,1.15903910586187,6.71090872772502));
#152578=CARTESIAN_POINT('Origin',(-0.106263825604032,1.33838398565068,-0.149107832000643));
#152579=CARTESIAN_POINT('Ctrl Pts',(3.23600613130859,1.19797317337953,6.48773953814593));
#152580=CARTESIAN_POINT('Ctrl Pts',(3.25486355744072,1.19116562422889,6.52482891711007));
#152581=CARTESIAN_POINT('Ctrl Pts',(3.27368957558313,1.18452215736987,6.56199395330996));
#152582=CARTESIAN_POINT('Ctrl Pts',(3.3112400966168,1.17155461455324,6.63637254212063));
#152583=CARTESIAN_POINT('Ctrl Pts',(3.32998686140786,1.16522285268755,6.67363020853883));
#152584=CARTESIAN_POINT('Ctrl Pts',(3.34868691525358,1.15903910499673,6.71090872675037));
#152585=CARTESIAN_POINT('',(2.67265020052562,1.0693909182078,6.8726225967679));
#152586=CARTESIAN_POINT('Origin',(-4.88758339356465E-13,1.16011713400006,
-7.53303669442928E-13));
#152587=CARTESIAN_POINT('',(3.34284868628286,0.979367659172238,6.71381878362192));
#152588=CARTESIAN_POINT('Origin',(-0.0902493205394439,0.946436353500672,
-0.169370210595567));
#152589=CARTESIAN_POINT('',(3.84358647165651,1.06939091992733,6.440251779367));
#152590=CARTESIAN_POINT('Origin',(-0.0558087578793248,0.803756666233792,
-0.17475322261742));
#152591=CARTESIAN_POINT('Origin',(-0.112447373940797,0.946509336669416,
-0.150063191541521));
#152592=CARTESIAN_POINT('Ctrl Pts',(3.231813931,1.198733649,6.489828867));
#152593=CARTESIAN_POINT('Ctrl Pts',(3.585333593,1.134619049,6.313782657));
#152594=CARTESIAN_POINT('Ctrl Pts',(3.917638724,1.069390921,6.100377597));
#152595=CARTESIAN_POINT('Ctrl Pts',(3.92097107091642,1.06873681508671,6.09823757679778));
#152596=CARTESIAN_POINT('Ctrl Pts',(3.92430341783284,1.06808270917341,6.09609755659557));
#152597=CARTESIAN_POINT('Ctrl Pts',(3.121281553,1.198733649,6.819648192));
#152598=CARTESIAN_POINT('Ctrl Pts',(3.492767424,1.134619049,6.649623));
#152599=CARTESIAN_POINT('Ctrl Pts',(3.84358648,1.069390921,6.440251778));
#152600=CARTESIAN_POINT('Ctrl Pts',(3.84710448405839,1.06873681508671,6.43815220901677));
#152601=CARTESIAN_POINT('Ctrl Pts',(3.85062248811679,1.06808270917341,6.43605264003352));
#152602=CARTESIAN_POINT('',(3.88061258553506,1.06939091791719,6.27031469768993));
#152603=CARTESIAN_POINT('Ctrl Pts',(3.91101369546957,1.06811592995217,6.10463216359967));
#152604=CARTESIAN_POINT('Ctrl Pts',(3.91432620973478,1.06875342547609,6.10250488029983));
#152605=CARTESIAN_POINT('Ctrl Pts',(3.917638724,1.069390921,6.100377597));
#152606=CARTESIAN_POINT('Ctrl Pts',(3.922933723,1.070409947,6.09697717));
#152607=CARTESIAN_POINT('Ctrl Pts',(3.928222811,1.071428571,6.093567555));
#152608=CARTESIAN_POINT('Ctrl Pts',(4.255722683,1.134501699,5.882444522));
#152609=CARTESIAN_POINT('Ctrl Pts',(4.558707681,1.198754474,5.63743596700001));
#152610=CARTESIAN_POINT('Ctrl Pts',(4.2508074552393,1.06811592995217,6.17905351246949));
#152611=CARTESIAN_POINT('Ctrl Pts',(4.25416018011965,1.06875342547609,6.17674167673474));
#152612=CARTESIAN_POINT('Ctrl Pts',(4.257512905,1.069390921,6.17442984100001));
#152613=CARTESIAN_POINT('Ctrl Pts',(4.26287218,1.070409947,6.17073441));
#152614=CARTESIAN_POINT('Ctrl Pts',(4.268225031,1.071428571,6.167029681));
#152615=CARTESIAN_POINT('Ctrl Pts',(4.599673138,1.134501699,5.937633167));
#152616=CARTESIAN_POINT('Ctrl Pts',(4.90462506300001,1.198754474,5.674033221));
#152617=CARTESIAN_POINT('',(4.25751291014559,1.06939091911149,6.17442983448858));
#152618=CARTESIAN_POINT('',(4.71304347805112,1.15903910585152,5.83414271099935));
#152619=CARTESIAN_POINT('Origin',(-0.13583321860543,1.33838405461728,-0.122778182208158));
#152620=CARTESIAN_POINT('Ctrl Pts',(4.55502233005473,1.19797317335072,5.64041413156831));
#152621=CARTESIAN_POINT('Ctrl Pts',(4.58141200040322,1.1911656242053,5.67258259206166));
#152622=CARTESIAN_POINT('Ctrl Pts',(4.60778726111216,1.18452215734081,5.70483169279222));
#152623=CARTESIAN_POINT('Ctrl Pts',(4.66044906985397,1.17155461458284,5.76939909879967));
#152624=CARTESIAN_POINT('Ctrl Pts',(4.68676684286837,1.16522285268912,5.80175570135455));
#152625=CARTESIAN_POINT('Ctrl Pts',(4.71304347948102,1.15903910497747,5.83414270967234));
#152626=CARTESIAN_POINT('',(4.08757582880698,1.06939091820862,6.13740370947139));
#152627=CARTESIAN_POINT('Origin',(-5.95010152260045E-13,1.16011713400006,
-8.0404433111525E-13));
#152628=CARTESIAN_POINT('',(4.70796732118502,0.9793676591462,5.83823977776835));
#152629=CARTESIAN_POINT('Origin',(-0.12454898017964,0.946436321968166,-0.146009561522032));
#152630=CARTESIAN_POINT('',(5.13818931612299,1.06939091992738,5.46342479616291));
#152631=CARTESIAN_POINT('Origin',(-0.0920707914298757,0.80375664195573,
-0.158670405150794));
#152632=CARTESIAN_POINT('Origin',(-0.142077653826491,0.94650933952944,-0.12238203947585));
#152633=CARTESIAN_POINT('Ctrl Pts',(4.551377285,1.198733649,5.643355811));
#152634=CARTESIAN_POINT('Ctrl Pts',(4.858787123,1.134619049,5.395429187));
#152635=CARTESIAN_POINT('Ctrl Pts',(5.137447365,1.069390921,5.115577638));
#152636=CARTESIAN_POINT('Ctrl Pts',(5.14024176241229,1.06873681508671,5.11277129419315));
#152637=CARTESIAN_POINT('Ctrl Pts',(5.14303615982459,1.06808270917341,5.10996495038631));
#152638=CARTESIAN_POINT('Ctrl Pts',(4.51433049900001,1.198733649,5.989225338));
#152639=CARTESIAN_POINT('Ctrl Pts',(4.840580846,1.134619049,5.74331675900001));
#152640=CARTESIAN_POINT('Ctrl Pts',(5.13818932400001,1.069390921,5.463424793));
#152641=CARTESIAN_POINT('Ctrl Pts',(5.14117373381329,1.06873681508671,5.46061804389256));
#152642=CARTESIAN_POINT('Ctrl Pts',(5.1441581436266,1.06808270917341,5.45781129478513));
#152643=CARTESIAN_POINT('',(5.13781833061056,1.06939091791719,5.28950122899115));
#152644=CARTESIAN_POINT('Ctrl Pts',(5.13189183273593,1.06811592995319,5.12115692152758));
#152645=CARTESIAN_POINT('Ctrl Pts',(5.13466959886796,1.06875342547659,5.11836727976378));
#152646=CARTESIAN_POINT('Ctrl Pts',(5.137447365,1.069390921,5.115577638));
#152647=CARTESIAN_POINT('Ctrl Pts',(5.141887578,1.070409947,5.111118442));
#152648=CARTESIAN_POINT('Ctrl Pts',(5.146320044,1.071428571,5.106651545));
#152649=CARTESIAN_POINT('Ctrl Pts',(5.42077794,1.134501699,4.830061659));
#152650=CARTESIAN_POINT('Ctrl Pts',(5.66400972,1.198754474,4.525648449));
#152651=CARTESIAN_POINT('Ctrl Pts',(5.47973979224852,1.06811592995319,5.1207927256041));
#152652=CARTESIAN_POINT('Ctrl Pts',(5.48251715612426,1.06875342547659,5.11781420230205));
#152653=CARTESIAN_POINT('Ctrl Pts',(5.48529452,1.069390921,5.114835679));
#152654=CARTESIAN_POINT('Ctrl Pts',(5.48973409,1.070409947,5.11007455900001));
#152655=CARTESIAN_POINT('Ctrl Pts',(5.494165387,1.071428571,5.10530574));
#152656=CARTESIAN_POINT('Ctrl Pts',(5.768550952,1.134501699,4.810020844));
#152657=CARTESIAN_POINT('Ctrl Pts',(6.009707074,1.198754474,4.487028069));
#152658=CARTESIAN_POINT('',(5.48529452373196,1.06939091911035,5.1148356715626));
#152659=CARTESIAN_POINT('',(5.85702336747576,1.1590391058667,4.68457866535481));
#152660=CARTESIAN_POINT('Origin',(-0.159051194702147,1.33838407973086,-0.0907075657125889));
#152661=CARTESIAN_POINT('Ctrl Pts',(5.66105074778303,1.19797317332967,4.529349227356));
#152662=CARTESIAN_POINT('Ctrl Pts',(5.6937387104184,1.19116562421628,4.55509260821413));
#152663=CARTESIAN_POINT('Ctrl Pts',(5.72642993554067,1.18452215738145,4.58091784158635));
#152664=CARTESIAN_POINT('Ctrl Pts',(5.79174062461541,1.17155461457221,4.63265496589298));
#152665=CARTESIAN_POINT('Ctrl Pts',(5.82439881566446,1.16522285272192,4.65859754577574));
#152666=CARTESIAN_POINT('Ctrl Pts',(5.85702336856875,1.15903910501501,4.68457866377963));
#152667=CARTESIAN_POINT('',(5.31137095443124,1.06939091820696,5.1152066461112));
#152668=CARTESIAN_POINT('Origin',(-9.51062145704284E-13,1.160117134,-8.09248501543181E-13));
#152669=CARTESIAN_POINT('',(5.8529466364323,0.979367659138719,4.68967116858882));
#152670=CARTESIAN_POINT('Origin',(-0.153024751815678,0.9464363304404,-0.115821519499659));
#152671=CARTESIAN_POINT('',(6.19253613899442,1.06939091992736,4.23113414176147));
#152672=CARTESIAN_POINT('Origin',(-0.124027660136634,0.803756642011697,
-0.135168275672048));
#152673=CARTESIAN_POINT('Origin',(-0.165064522538633,0.946509306495977,
-0.0889783519444282));
#152674=CARTESIAN_POINT('Ctrl Pts',(5.658123296,1.198733649,4.53300571));
#152675=CARTESIAN_POINT('Ctrl Pts',(5.90504916800001,1.134619049,4.224791444));
#152676=CARTESIAN_POINT('Ctrl Pts',(6.117034678,1.069390921,3.891578954));
#152677=CARTESIAN_POINT('Ctrl Pts',(6.11916046299299,1.06873681508671,3.88823750811193));
#152678=CARTESIAN_POINT('Ctrl Pts',(6.12128624798599,1.06808270917341,3.88489606222386));
#152679=CARTESIAN_POINT('Ctrl Pts',(5.696294368,1.198733649,4.878752963));
#152680=CARTESIAN_POINT('Ctrl Pts',(5.962054088,1.134619049,4.568459409));
#152681=CARTESIAN_POINT('Ctrl Pts',(6.192536146,1.069390921,4.231134137));
#152682=CARTESIAN_POINT('Ctrl Pts',(6.19484741387888,1.06873681508671,4.22775144824465));
#152683=CARTESIAN_POINT('Ctrl Pts',(6.19715868175776,1.06808270917341,4.22436875948929));
#152684=CARTESIAN_POINT('',(6.15478540133549,1.06939091791719,4.06135656166154));
#152685=CARTESIAN_POINT('Ctrl Pts',(6.11280841197604,1.06811592995216,3.89822207217745));
#152686=CARTESIAN_POINT('Ctrl Pts',(6.11492154498802,1.06875342547608,3.89490051308873));
#152687=CARTESIAN_POINT('Ctrl Pts',(6.117034678,1.069390921,3.891578954));
#152688=CARTESIAN_POINT('Ctrl Pts',(6.120412486,1.070409947,3.886269497));
#152689=CARTESIAN_POINT('Ctrl Pts',(6.123781072,1.071428571,3.880954185));
#152690=CARTESIAN_POINT('Ctrl Pts',(6.332363645,1.134501699,3.551830482));
#152691=CARTESIAN_POINT('Ctrl Pts',(6.50446896,1.198754474,3.202246641));
#152692=CARTESIAN_POINT('Ctrl Pts',(6.4524455879471,1.06811592995216,3.82308936021757));
#152693=CARTESIAN_POINT('Ctrl Pts',(6.45451772397355,1.06875342547608,3.81958342260879));
#152694=CARTESIAN_POINT('Ctrl Pts',(6.45658986,1.069390921,3.816077485));
#152695=CARTESIAN_POINT('Ctrl Pts',(6.45990213500001,1.070409947,3.810473302));
#152696=CARTESIAN_POINT('Ctrl Pts',(6.463204676,1.071428571,3.804863377));
#152697=CARTESIAN_POINT('Ctrl Pts',(6.667697735,1.134501699,3.457497292));
#152698=CARTESIAN_POINT('Ctrl Pts',(6.833781861,1.198754474,3.090214471));
#152699=CARTESIAN_POINT('',(6.45658986212243,1.06939091911146,3.81607747695018));
#152700=CARTESIAN_POINT('',(6.72713535380483,1.15903910586345,3.31596892777236));
#152701=CARTESIAN_POINT('Origin',(-0.174832111025703,1.33838404516078,-0.0543955737960117));
#152702=CARTESIAN_POINT('Ctrl Pts',(6.50237472517852,1.19797317335901,3.20649698852999));
#152703=CARTESIAN_POINT('Ctrl Pts',(6.53983233906171,1.19116565840804,3.22461146673117));
#152704=CARTESIAN_POINT('Ctrl Pts',(6.57731071417596,1.18452222611864,3.24280517092969));
#152705=CARTESIAN_POINT('Ctrl Pts',(6.65221682460398,1.17155461459956,3.27929303559281));
#152706=CARTESIAN_POINT('Ctrl Pts',(6.68968837315633,1.16522285272586,3.29760854664996));
#152707=CARTESIAN_POINT('Ctrl Pts',(6.72713535453218,1.15903910500762,3.31596892600066));
#152708=CARTESIAN_POINT('',(6.28681227798357,1.06939091820867,3.85382820484497));
#152709=CARTESIAN_POINT('Origin',(-5.68121938382404E-13,1.16011713400022,
-2.82326245715225E-13));
#152710=CARTESIAN_POINT('',(6.72424867213753,0.979367659153833,3.32181874799286));
#152711=CARTESIAN_POINT('Origin',(-0.174345382799326,0.946436314050401,
-0.080217914826296));
#152712=CARTESIAN_POINT('',(6.95732685417891,1.06939091992739,2.80100035617951));
#152713=CARTESIAN_POINT('Origin',(-0.150185083090411,0.803756637318066,
-0.105345803537276));
#152714=CARTESIAN_POINT('Origin',(-0.180332952476162,0.946509333178315,
-0.0514140178657779));
#152715=CARTESIAN_POINT('Ctrl Pts',(6.500301751,1.198733649,3.210697299));
#152716=CARTESIAN_POINT('Ctrl Pts',(6.675197676,1.134619049,2.856607148));
#152717=CARTESIAN_POINT('Ctrl Pts',(6.810596247,1.069390921,2.485614363));
#152718=CARTESIAN_POINT('Ctrl Pts',(6.81195402022849,1.06873681508671,2.48189405732976));
#152719=CARTESIAN_POINT('Ctrl Pts',(6.81331179345697,1.06808270917341,2.47817375165952));
#152720=CARTESIAN_POINT('Ctrl Pts',(6.611905843,1.198733649,3.540155522));
#152721=CARTESIAN_POINT('Ctrl Pts',(6.804748307,1.134619049,3.179985975));
#152722=CARTESIAN_POINT('Ctrl Pts',(6.95732686,1.069390921,2.80100035));
#152723=CARTESIAN_POINT('Ctrl Pts',(6.95885691362593,1.06873681508671,2.79719989234521));
#152724=CARTESIAN_POINT('Ctrl Pts',(6.96038696725186,1.06808270917341,2.79339943469041));
#152725=CARTESIAN_POINT('',(6.88396154655908,1.06939091791719,2.64330737457626));
#152726=CARTESIAN_POINT('Ctrl Pts',(6.80789686204117,1.06811592995401,2.49301069012391));
#152727=CARTESIAN_POINT('Ctrl Pts',(6.80924655452058,1.06875342547701,2.48931252656195));
#152728=CARTESIAN_POINT('Ctrl Pts',(6.810596247,1.069390921,2.485614363));
#152729=CARTESIAN_POINT('Ctrl Pts',(6.812753708,1.070409947,2.47970291));
#152730=CARTESIAN_POINT('Ctrl Pts',(6.814900903,1.071428571,2.47378772));
#152731=CARTESIAN_POINT('Ctrl Pts',(6.94785506400001,1.134501699,2.107519659));
#152732=CARTESIAN_POINT('Ctrl Pts',(7.04078646,1.198754474,1.729111338));
#152733=CARTESIAN_POINT('Ctrl Pts',(7.12344219883659,1.06811592995401,2.34662258803516));
#152734=CARTESIAN_POINT('Ctrl Pts',(7.12471221641829,1.06875342547701,2.34275316901758));
#152735=CARTESIAN_POINT('Ctrl Pts',(7.125982234,1.069390921,2.33888375));
#152736=CARTESIAN_POINT('Ctrl Pts',(7.128012336,1.070409947,2.332698548));
#152737=CARTESIAN_POINT('Ctrl Pts',(7.130031697,1.071428571,2.326509831));
#152738=CARTESIAN_POINT('Ctrl Pts',(7.255070382,1.134501699,1.94330501));
#152739=CARTESIAN_POINT('Ctrl Pts',(7.338316604,1.198754474,1.548905879));
#152740=CARTESIAN_POINT('',(7.12598223423462,1.06939091910945,2.33888374168009));
#152741=CARTESIAN_POINT('',(7.28269396775983,1.15903910589433,1.79230816855612));
#152742=CARTESIAN_POINT('Origin',(-0.182438073594617,1.33838404864279,-0.0155400990156312));
#152743=CARTESIAN_POINT('Ctrl Pts',(7.03965488635939,1.19797317331785,1.73371251352998));
#152744=CARTESIAN_POINT('Ctrl Pts',(7.08013084500336,1.19116565746261,1.74335120689549));
#152745=CARTESIAN_POINT('Ctrl Pts',(7.12064411118154,1.18452222427951,1.75306281109334));
#152746=CARTESIAN_POINT('Ctrl Pts',(7.20164275946683,1.17155461460936,1.77259500754028));
#152747=CARTESIAN_POINT('Ctrl Pts',(7.24217553752639,1.16522285275215,1.7824270368528));
#152748=CARTESIAN_POINT('Ctrl Pts',(7.28269396809338,1.15903910505169,1.79230816666107));
#152749=CARTESIAN_POINT('',(6.96828924612935,1.06939091820559,2.41224904023845));
#152750=CARTESIAN_POINT('Origin',(7.94937032866372E-13,1.16011713400011,
2.03287907341032E-13));
#152751=CARTESIAN_POINT('',(7.28113231366877,0.97936765913114,1.79864177447981));
#152752=CARTESIAN_POINT('Origin',(-0.187513717011382,0.946436304846853,
-0.0408633449838341));
#152753=CARTESIAN_POINT('',(7.396800698641,1.06939091992734,1.23989490826094));
#152754=CARTESIAN_POINT('Origin',(-0.169320101023622,0.803756621750654,
-0.0705975350748289));
#152755=CARTESIAN_POINT('Origin',(-0.187169459703335,0.946509334807441,
-0.0114457587835903));
#152756=CARTESIAN_POINT('Ctrl Pts',(7.03853332,1.198733649,1.738260252));
#152757=CARTESIAN_POINT('Ctrl Pts',(7.13322136,1.134619049,1.354851078));
#152758=CARTESIAN_POINT('Ctrl Pts',(7.185701905,1.069390921,0.963425207));
#152759=CARTESIAN_POINT('Ctrl Pts',(7.18622817849381,1.06873681508671,0.959499998892894));
#152760=CARTESIAN_POINT('Ctrl Pts',(7.18675445198762,1.06808270917341,0.955574790785788));
#152761=CARTESIAN_POINT('Ctrl Pts',(7.21835195,1.198733649,2.036024343));
#152762=CARTESIAN_POINT('Ctrl Pts',(7.329260058,1.134619049,1.642819931));
#152763=CARTESIAN_POINT('Ctrl Pts',(7.396800703,1.069390921,1.239894901));
#152764=CARTESIAN_POINT('Ctrl Pts',(7.39747799877158,1.06873681508671,1.23585437963571));
#152765=CARTESIAN_POINT('Ctrl Pts',(7.39815529454315,1.06808270917341,1.23181385827142));
#152766=CARTESIAN_POINT('',(7.29125130110721,1.06939091791719,1.10166007314573));
#152767=CARTESIAN_POINT('Ctrl Pts',(7.18465562199158,1.06811592995212,0.971228900272083));
#152768=CARTESIAN_POINT('Ctrl Pts',(7.1851787634958,1.06875342547606,0.967327053636041));
#152769=CARTESIAN_POINT('Ctrl Pts',(7.18570190500001,1.069390921,0.963425207));
#152770=CARTESIAN_POINT('Ctrl Pts',(7.186538138,1.070409947,0.95718817));
#152771=CARTESIAN_POINT('Ctrl Pts',(7.187363542,1.071428571,0.95094969));
#152772=CARTESIAN_POINT('Ctrl Pts',(7.238472502,1.134501699,0.564663559));
#152773=CARTESIAN_POINT('Ctrl Pts',(7.247884611,1.198754474,0.175124711));
#152774=CARTESIAN_POINT('Ctrl Pts',(7.46135457079931,1.06811592995212,0.760430350372509));
#152775=CARTESIAN_POINT('Ctrl Pts',(7.46176308489966,1.06875342547606,0.756378380186254));
#152776=CARTESIAN_POINT('Ctrl Pts',(7.462171599,1.069390921,0.75232641));
#152777=CARTESIAN_POINT('Ctrl Pts',(7.46282460200001,1.070409947,0.745849403));
#152778=CARTESIAN_POINT('Ctrl Pts',(7.463466361,1.071428571,0.739371272));
#152779=CARTESIAN_POINT('Ctrl Pts',(7.503204002,1.134501699,0.338245945));
#152780=CARTESIAN_POINT('Ctrl Pts',(7.499719818,1.198754474,-0.064827831));
#152781=CARTESIAN_POINT('Ctrl Pts',(7.24776860954439,1.19797317331415,0.179861568603665));
#152782=CARTESIAN_POINT('Ctrl Pts',(7.28937029396337,1.19116565793403,0.180573779781957));
#152783=CARTESIAN_POINT('Ctrl Pts',(7.33102408720557,1.18452222520096,0.181349177264534));
#152784=CARTESIAN_POINT('Ctrl Pts',(7.4143278828079,1.17155461459689,0.183012406879414));
#152785=CARTESIAN_POINT('Ctrl Pts',(7.45602662267977,1.16522285273111,0.183901219767036));
#152786=CARTESIAN_POINT('Ctrl Pts',(7.49772190567691,1.1590391050196,0.184841069551826));
#152787=CARTESIAN_POINT('',(7.32393675399974,1.06939091820872,0.857875791427671));
#152788=CARTESIAN_POINT('Ctrl Pts',(7.247650894,1.198733649,0.184544087));
#152789=CARTESIAN_POINT('Ctrl Pts',(7.257703542,1.134619049,-0.210256324));
#152790=CARTESIAN_POINT('Ctrl Pts',(7.224812129,1.069390921,-0.603812641));
#152791=CARTESIAN_POINT('Ctrl Pts',(7.22448229479504,1.06873681508671,-0.607759213162297));
#152792=CARTESIAN_POINT('Ctrl Pts',(7.22415246059009,1.06808270917341,-0.611705785324593));
#152793=CARTESIAN_POINT('Ctrl Pts',(7.487275942,1.198733649,0.436690929));
#152794=CARTESIAN_POINT('Ctrl Pts',(7.51106375400001,1.134619049,0.028837453));
#152795=CARTESIAN_POINT('Ctrl Pts',(7.490408365,1.069390921,-0.379186656));
#152796=CARTESIAN_POINT('Ctrl Pts',(7.49020123331463,1.06873681508671,-0.383278310791366));
#152797=CARTESIAN_POINT('Ctrl Pts',(7.48999410162926,1.06808270917341,-0.387369965582731));
#152798=CARTESIAN_POINT('',(7.35761024829061,1.06939091791719,-0.491499629180019));
#152799=CARTESIAN_POINT('Ctrl Pts',(7.2254678718203,1.06811592995217,-0.595966473717617));
#152800=CARTESIAN_POINT('Ctrl Pts',(7.22514000041015,1.06875342547609,-0.599889557358809));
#152801=CARTESIAN_POINT('Ctrl Pts',(7.224812129,1.069390921,-0.603812641000001));
#152802=CARTESIAN_POINT('Ctrl Pts',(7.224288032,1.070409947,-0.610083625));
#152803=CARTESIAN_POINT('Ctrl Pts',(7.22375305,1.071428571,-0.616353689));
#152804=CARTESIAN_POINT('Ctrl Pts',(7.190627011,1.134501699,-1.004595582));
#152805=CARTESIAN_POINT('Ctrl Pts',(7.116079733,1.198754474,-1.387050553));
#152806=CARTESIAN_POINT('Ctrl Pts',(7.45038229297622,1.06811592995217,-0.861318764735266));
#152807=CARTESIAN_POINT('Ctrl Pts',(7.44991020298811,1.06875342547609,-0.865363820867633));
#152808=CARTESIAN_POINT('Ctrl Pts',(7.449438113,1.069390921,-0.869408877000001));
#152809=CARTESIAN_POINT('Ctrl Pts',(7.448683485,1.070409947,-0.875874832));
#152810=CARTESIAN_POINT('Ctrl Pts',(7.447917633,1.071428571,-0.882339467));
#152811=CARTESIAN_POINT('Ctrl Pts',(7.400496141,1.134501699,-1.282629125));
#152812=CARTESIAN_POINT('Ctrl Pts',(7.310444469,1.198754474,-1.675530263));
#152813=CARTESIAN_POINT('',(7.44943810973505,1.06939091911148,-0.869408884642924));
#152814=CARTESIAN_POINT('',(7.36216470066823,1.15903910587719,-1.43126898914685));
#152815=CARTESIAN_POINT('Origin',(-0.172101427481555,1.33838407053768,0.0624999501092453));
#152816=CARTESIAN_POINT('Ctrl Pts',(7.11698472793918,1.1979731733218,-1.3823995036554));
#152817=CARTESIAN_POINT('Ctrl Pts',(7.15776689789494,1.19116565700939,-1.39064707706337));
#152818=CARTESIAN_POINT('Ctrl Pts',(7.19861354226323,1.18452222333549,-1.39884414344332));
#152819=CARTESIAN_POINT('Ctrl Pts',(7.28032727466069,1.17155461460988,-1.41512765056565));
#152820=CARTESIAN_POINT('Ctrl Pts',(7.32124218987634,1.16522285270705,-1.42322361423589));
#152821=CARTESIAN_POINT('Ctrl Pts',(7.36216470016111,1.15903910500744,-1.43126899105776));
#152822=CARTESIAN_POINT('',(7.33712511928289,1.06939091820865,-0.736610776103533));
#152823=CARTESIAN_POINT('Origin',(-1.46800974154537E-12,1.16011713399978,
2.62322715632868E-13));
#152824=CARTESIAN_POINT('',(7.36340679369018,0.979367659169459,-1.42486504209286));
#152825=CARTESIAN_POINT('Origin',(-0.18734085634547,0.94643629633262,0.0416483950848034));
#152826=CARTESIAN_POINT('',(7.23377285710191,1.06939091992737,-1.980537857564));
#152827=CARTESIAN_POINT('Origin',(-0.183313845503943,0.803756640188027,
0.00702306772492167));
#152828=CARTESIAN_POINT('Origin',(-0.174676264822841,0.946509290946531,
0.0682025193396724));
#152829=CARTESIAN_POINT('Ctrl Pts',(7.117876367,1.198733649,-1.377801155));
#152830=CARTESIAN_POINT('Ctrl Pts',(7.042823572,1.134619049,-1.765532373));
#152831=CARTESIAN_POINT('Ctrl Pts',(6.926098167,1.069390921,-2.14281688));
#152832=CARTESIAN_POINT('Ctrl Pts',(6.92492764777796,1.06873681508671,-2.14660027888924));
#152833=CARTESIAN_POINT('Ctrl Pts',(6.92375712855592,1.06808270917341,-2.15038367777849));
#152834=CARTESIAN_POINT('Ctrl Pts',(7.406103233,1.198733649,-1.183061667));
#152835=CARTESIAN_POINT('Ctrl Pts',(7.341658458,1.134619049,-1.586493433));
#152836=CARTESIAN_POINT('Ctrl Pts',(7.233772858,1.069390921,-1.980537866));
#152837=CARTESIAN_POINT('Ctrl Pts',(7.23269098410475,1.06873681508671,-1.98448933297642));
#152838=CARTESIAN_POINT('Ctrl Pts',(7.2316091102095,1.06808270917341,-1.98844079995283));
#152839=CARTESIAN_POINT('',(7.07993551791366,1.06939091791719,-2.06167735440915));
#152840=CARTESIAN_POINT('Ctrl Pts',(6.92842527283417,1.06811592995212,-2.13529511646555));
#152841=CARTESIAN_POINT('Ctrl Pts',(6.92726171991709,1.06875342547606,-2.13905599823277));
#152842=CARTESIAN_POINT('Ctrl Pts',(6.926098167,1.069390921,-2.14281688));
#152843=CARTESIAN_POINT('Ctrl Pts',(6.924238247,1.070409947,-2.148828587));
#152844=CARTESIAN_POINT('Ctrl Pts',(6.922367894,1.071428571,-2.154837056));
#152845=CARTESIAN_POINT('Ctrl Pts',(6.806555793,1.134501699,-2.52688095));
#152846=CARTESIAN_POINT('Ctrl Pts',(6.651534875,1.198754474,-2.884368874));
#152847=CARTESIAN_POINT('Ctrl Pts',(7.09103842230696,1.06811592995212,-2.44279357166386));
#152848=CARTESIAN_POINT('Ctrl Pts',(7.08970780165348,1.06875342547606,-2.44664257133193));
#152849=CARTESIAN_POINT('Ctrl Pts',(7.088377181,1.069390921,-2.450491571));
#152850=CARTESIAN_POINT('Ctrl Pts',(7.086250206,1.070409947,-2.456644133));
#152851=CARTESIAN_POINT('Ctrl Pts',(7.084112554,1.071428571,-2.462792993));
#152852=CARTESIAN_POINT('Ctrl Pts',(6.951749306,1.134501699,-2.843529882));
#152853=CARTESIAN_POINT('Ctrl Pts',(6.779340862,1.198754474,-3.207886762));
#152854=CARTESIAN_POINT('',(7.0883771760567,1.06939091911158,-2.45049157765598));
#152855=CARTESIAN_POINT('',(6.88236085655826,1.15903910585907,-2.98045450177495));
#152856=CARTESIAN_POINT('Origin',(-0.154642145265497,1.33838411158198,0.0980354607432685));
#152857=CARTESIAN_POINT('Ctrl Pts',(6.65341854975392,1.19797317333231,-2.88002111080759));
#152858=CARTESIAN_POINT('Ctrl Pts',(6.69147429362735,1.19116565295346,-2.89684283171955));
#152859=CARTESIAN_POINT('Ctrl Pts',(6.72960386502397,1.18452221510443,-2.91362908763632));
#152860=CARTESIAN_POINT('Ctrl Pts',(6.80590665471737,1.17155461461087,-2.94709791120943));
#152861=CARTESIAN_POINT('Ctrl Pts',(6.84412460899343,1.16522285272256,-2.96380009301572));
#152862=CARTESIAN_POINT('Ctrl Pts',(6.88236085568021,1.15903910499693,-2.98045450347072));
#152863=CARTESIAN_POINT('',(7.00723766864643,1.06939091820872,-2.29665424183409));
#152864=CARTESIAN_POINT('Origin',(-9.11163505756818E-13,1.16011713400011,
4.39969241594618E-13));
#152865=CARTESIAN_POINT('',(6.88495056955131,0.979367659115532,-2.97446728926621));
#152866=CARTESIAN_POINT('Origin',(-0.174007811960476,0.946436343448101,
0.0809474406507071));
#152867=CARTESIAN_POINT('',(6.63889417195209,1.0693909199274,-3.48928131855112));
#152868=CARTESIAN_POINT('Origin',(-0.177518215079709,0.803756643672089,
0.0462658936260202));
#152869=CARTESIAN_POINT('Origin',(-0.155930962436405,0.946509332563335,
0.104158238975147));
#152870=CARTESIAN_POINT('Ctrl Pts',(6.655277852,1.198733649,-2.875721945));
#152871=CARTESIAN_POINT('Ctrl Pts',(6.498628999,1.134619049,-3.238254091));
#152872=CARTESIAN_POINT('Ctrl Pts',(6.303527553,1.069390921,-3.581625384));
#152873=CARTESIAN_POINT('Ctrl Pts',(6.30157108094671,1.06873681508671,-3.58506870209134));
#152874=CARTESIAN_POINT('Ctrl Pts',(6.29961460889341,1.06808270917341,-3.58851202018267));
#152875=CARTESIAN_POINT('Ctrl Pts',(6.978629367,1.198733649,-2.747495615));
#152876=CARTESIAN_POINT('Ctrl Pts',(6.828965371,1.134619049,-3.127641648));
#152877=CARTESIAN_POINT('Ctrl Pts',(6.638894171,1.069390921,-3.489281327));
#152878=CARTESIAN_POINT('Ctrl Pts',(6.63698814211831,1.06873681508671,-3.49290783997482));
#152879=CARTESIAN_POINT('Ctrl Pts',(6.63508211323662,1.06808270917341,-3.49653435294964));
#152880=CARTESIAN_POINT('',(6.47121087128357,1.06939091791719,-3.53545333850757));
#152881=CARTESIAN_POINT('Ctrl Pts',(6.30741720870105,1.06811592995355,-3.57477973385255));
#152882=CARTESIAN_POINT('Ctrl Pts',(6.30547238085052,1.06875342547678,-3.57820255892628));
#152883=CARTESIAN_POINT('Ctrl Pts',(6.303527553,1.069390921,-3.581625384));
#152884=CARTESIAN_POINT('Ctrl Pts',(6.300418778,1.070409947,-3.587096713));
#152885=CARTESIAN_POINT('Ctrl Pts',(6.297300509,1.071428571,-3.592562637));
#152886=CARTESIAN_POINT('Ctrl Pts',(6.104217591,1.134501699,-3.931012172));
#152887=CARTESIAN_POINT('Ctrl Pts',(5.875971639,1.198754474,-4.246817313));
#152888=CARTESIAN_POINT('Ctrl Pts',(6.40012547593091,1.06811592995355,-3.91004606779373));
#152889=CARTESIAN_POINT('Ctrl Pts',(6.39799854296545,1.06875342547678,-3.91351903539686));
#152890=CARTESIAN_POINT('Ctrl Pts',(6.39587161,1.069390921,-3.916992003));
#152891=CARTESIAN_POINT('Ctrl Pts',(6.392471743,1.070409947,-3.922543484));
#152892=CARTESIAN_POINT('Ctrl Pts',(6.389062245,1.071428571,-3.928089055));
#152893=CARTESIAN_POINT('Ctrl Pts',(6.1779464,1.134501699,-4.271470342));
#152894=CARTESIAN_POINT('Ctrl Pts',(5.93124281,1.198754474,-4.59024604200001));
#152895=CARTESIAN_POINT('',(6.39587160367231,1.06939091911003,-3.9169920083545));
#152896=CARTESIAN_POINT('',(6.08074546794259,1.15903910585345,-4.39027727503094));
#152897=CARTESIAN_POINT('Origin',(-0.129951979063783,1.33838405798379,0.128986930953131));
#152898=CARTESIAN_POINT('Ctrl Pts',(5.87874591481904,1.19797317339007,-4.24297613254375));
#152899=CARTESIAN_POINT('Ctrl Pts',(5.91229590555161,1.19116562424506,-4.26758553472227));
#152900=CARTESIAN_POINT('Ctrl Pts',(5.94592563809149,1.18452215738926,-4.29217618263442));
#152901=CARTESIAN_POINT('Ctrl Pts',(6.01324940384929,1.17155461456642,-4.34126514960852));
#152902=CARTESIAN_POINT('Ctrl Pts',(6.04698336827264,1.16522285267214,-4.36579257419969));
#152903=CARTESIAN_POINT('Ctrl Pts',(6.0807454666896,1.15903910497335,-4.39027727653642));
#152904=CARTESIAN_POINT('',(6.34969957275281,1.06939091820635,-3.74930870831395));
#152905=CARTESIAN_POINT('Origin',(1.47885176327023E-13,1.16011713399978,
-5.85469173142172E-14));
#152906=CARTESIAN_POINT('',(6.08456170863479,0.979367659166524,-4.38498675147155));
#152907=CARTESIAN_POINT('Origin',(-0.152538369459255,0.946436363046565,
0.116461520105225));
#152908=CARTESIAN_POINT('',(5.73358817473831,1.06939091992739,-4.83486986295877));
#152909=CARTESIAN_POINT('Origin',(-0.163422130638148,0.803756623814009,
0.0833453740518564));
#152910=CARTESIAN_POINT('Origin',(-0.129894276848799,0.946509303917947,
0.135243500605047));
#152911=CARTESIAN_POINT('Ctrl Pts',(5.881485942,1.198733649,-4.239177174));
#152912=CARTESIAN_POINT('Ctrl Pts',(5.650565757,1.134619049,-4.559558646));
#152913=CARTESIAN_POINT('Ctrl Pts',(5.386210996,1.069390921,-4.852961066));
#152914=CARTESIAN_POINT('Ctrl Pts',(5.38356005356643,1.06873681508671,-4.85590329757679));
#152915=CARTESIAN_POINT('Ctrl Pts',(5.38090911113287,1.06808270917341,-4.85884552915358));
#152916=CARTESIAN_POINT('Ctrl Pts',(6.224842549,1.198733649,-4.183459721));
#152917=CARTESIAN_POINT('Ctrl Pts',(5.996957454,1.134619049,-4.522544817));
#152918=CARTESIAN_POINT('Ctrl Pts',(5.733588172,1.069390921,-4.834869871));
#152919=CARTESIAN_POINT('Ctrl Pts',(5.73094711192334,1.06873681508671,-4.83800185824163));
#152920=CARTESIAN_POINT('Ctrl Pts',(5.72830605184669,1.06808270917341,-4.84113384548325));
#152921=CARTESIAN_POINT('',(5.5598995967194,1.06939091791719,-4.84391545390054));
#152922=CARTESIAN_POINT('Ctrl Pts',(5.39148132667974,1.06811592995213,-4.84711162513904));
#152923=CARTESIAN_POINT('Ctrl Pts',(5.38884616133988,1.06875342547606,-4.85003634556952));
#152924=CARTESIAN_POINT('Ctrl Pts',(5.386210996,1.069390921,-4.852961066));
#152925=CARTESIAN_POINT('Ctrl Pts',(5.381998728,1.070409947,-4.857636183));
#152926=CARTESIAN_POINT('Ctrl Pts',(5.377778351,1.071428571,-4.862303981));
#152927=CARTESIAN_POINT('Ctrl Pts',(5.116452959,1.134501699,-5.15133363500001));
#152928=CARTESIAN_POINT('Ctrl Pts',(4.82565450100001,1.198754474,-5.410689294));
#152929=CARTESIAN_POINT('Ctrl Pts',(5.40994977202152,1.06811592995213,-5.19446915376555));
#152930=CARTESIAN_POINT('Ctrl Pts',(5.40712598101076,1.06875342547606,-5.19740369788277));
#152931=CARTESIAN_POINT('Ctrl Pts',(5.40430219,1.069390921,-5.200338242));
#152932=CARTESIAN_POINT('Ctrl Pts',(5.399788407,1.070409947,-5.205029062));
#152933=CARTESIAN_POINT('Ctrl Pts',(5.395266487,1.071428571,-5.209712039));
#152934=CARTESIAN_POINT('Ctrl Pts',(5.115269587,1.134501699,-5.499681596));
#152935=CARTESIAN_POINT('Ctrl Pts',(4.805806437,1.198754474,-5.757970518));
#152936=CARTESIAN_POINT('',(5.40430218280845,1.06939091911149,-5.20033824619054));
#152937=CARTESIAN_POINT('',(4.99480117958429,1.15903910589032,-5.59481556208076));
#152938=CARTESIAN_POINT('Origin',(-0.0991854125737524,1.3383839565782,0.153907115829031));
#152939=CARTESIAN_POINT('Ctrl Pts',(4.82918965631122,1.19797317332657,-5.40753430549404));
#152940=CARTESIAN_POINT('Ctrl Pts',(4.85666484372267,1.1911656561366,-5.43878046336018));
#152941=CARTESIAN_POINT('Ctrl Pts',(4.88422192477404,1.18452222157352,-5.47002543160182));
#152942=CARTESIAN_POINT('Ctrl Pts',(4.93941929418718,1.17155461463316,-5.53243965416407));
#152943=CARTESIAN_POINT('Ctrl Pts',(4.96709190597967,1.16522285273282,-5.56364544646066));
#152944=CARTESIAN_POINT('Ctrl Pts',(4.99480117805053,1.15903910502987,-5.59481556327352));
#152945=CARTESIAN_POINT('',(5.39525658128272,1.06939091820872,-5.02664966657652));
#152946=CARTESIAN_POINT('Origin',(6.0281640790194E-14,1.16011713399972,
1.37476835471162E-13));
#152947=CARTESIAN_POINT('',(4.99966550416853,0.979367659117338,-5.59046910769365));
#152948=CARTESIAN_POINT('Origin',(-0.123936256261242,0.946436354951502,
0.146529879828055));
#152949=CARTESIAN_POINT('',(4.56018596634018,1.06939091992731,-5.95438526676254));
#152950=CARTESIAN_POINT('Origin',(-0.141684595606068,0.803756645137163,
0.116527713010236));
#152951=CARTESIAN_POINT('Origin',(-0.0977841519629702,0.94650933355158,
0.160005103084018));
#152952=CARTESIAN_POINT('Ctrl Pts',(4.832682286,1.198733649,-5.404413189));
#152953=CARTESIAN_POINT('Ctrl Pts',(4.53828834,1.134619049,-5.667663307));
#152954=CARTESIAN_POINT('Ctrl Pts',(4.217041199,1.069390921,-5.897377682));
#152955=CARTESIAN_POINT('Ctrl Pts',(4.2138197413099,1.06873681508671,-5.89968125157441));
#152956=CARTESIAN_POINT('Ctrl Pts',(4.2105982836198,1.06808270917341,-5.90198482114881));
#152957=CARTESIAN_POINT('Ctrl Pts',(5.17998901100001,1.198733649,-5.423809901));
#152958=CARTESIAN_POINT('Ctrl Pts',(4.884538471,1.134619049,-5.705978816));
#152959=CARTESIAN_POINT('Ctrl Pts',(4.560185962,1.069390921,-5.954385274));
#152960=CARTESIAN_POINT('Ctrl Pts',(4.55693336376311,1.06873681508671,-5.95687628728));
#152961=CARTESIAN_POINT('Ctrl Pts',(4.55368076552623,1.06808270917341,-5.95936730056002));
#152962=CARTESIAN_POINT('',(4.38861359606052,1.06939091791719,-5.92588146647613));
#152963=CARTESIAN_POINT('Ctrl Pts',(4.22344576855884,1.06811592995244,-5.89279796219269));
#152964=CARTESIAN_POINT('Ctrl Pts',(4.22024348377942,1.06875342547622,-5.89508782209635));
#152965=CARTESIAN_POINT('Ctrl Pts',(4.217041199,1.069390921,-5.89737768200001));
#152966=CARTESIAN_POINT('Ctrl Pts',(4.2119224,1.070409947,-5.90103798500001));
#152967=CARTESIAN_POINT('Ctrl Pts',(4.206797255,1.071428571,-5.904689396));
#152968=CARTESIAN_POINT('Ctrl Pts',(3.889448673,1.134501699,-6.130784462));
#152969=CARTESIAN_POINT('Ctrl Pts',(3.549695121,1.198754474,-6.321563458));
#152970=CARTESIAN_POINT('Ctrl Pts',(4.16681083229441,1.06811592995244,-6.2360046363775));
#152971=CARTESIAN_POINT('Ctrl Pts',(4.1634222196472,1.06875342547622,-6.23826354068875));
#152972=CARTESIAN_POINT('Ctrl Pts',(4.160033607,1.069390921,-6.240522445));
#152973=CARTESIAN_POINT('Ctrl Pts',(4.154616966,1.070409947,-6.244133266));
#152974=CARTESIAN_POINT('Ctrl Pts',(4.149194064,1.071428571,-6.247734679));
#152975=CARTESIAN_POINT('Ctrl Pts',(3.813408453,1.134501699,-6.470733852));
#152976=CARTESIAN_POINT('Ctrl Pts',(3.455655896,1.198754474,-6.656458693));
#152977=CARTESIAN_POINT('',(4.16003359904353,1.06939091911123,-6.24052244736327));
#152978=CARTESIAN_POINT('',(3.67530553951482,1.15903910585863,-6.53774649177692));
#152979=CARTESIAN_POINT('Origin',(-0.0637810247764503,1.33838400211325,
0.171630786261117));
#152980=CARTESIAN_POINT('Ctrl Pts',(3.55382585549297,1.19797317334867,-6.31924218533958));
#152981=CARTESIAN_POINT('Ctrl Pts',(3.57394168117612,1.19116565846847,-6.35566416603344));
#152982=CARTESIAN_POINT('Ctrl Pts',(3.59413774078712,1.18452222623441,-6.39210258828997));
#152983=CARTESIAN_POINT('Ctrl Pts',(3.63462742819504,1.17155461460377,-6.46492342989095));
#152984=CARTESIAN_POINT('Ctrl Pts',(3.65494474674917,1.16522285272797,-6.50134844137981));
#152985=CARTESIAN_POINT('Ctrl Pts',(3.67530553778319,1.15903910500572,-6.53774649260067));
#152986=CARTESIAN_POINT('',(4.18853738885056,1.06939091820823,-6.06895007326536));
#152987=CARTESIAN_POINT('Origin',(-9.9031026434826E-13,1.16011713399994,
1.74730022117764E-12));
#152988=CARTESIAN_POINT('',(3.68099049779525,0.979367659150468,-6.53454734113609));
#152989=CARTESIAN_POINT('Origin',(-0.0895392482799334,0.946436331401545,
0.169746975250635));
#152990=CARTESIAN_POINT('',(3.1735545308418,1.06939091992736,-6.7954802328553));
#152991=CARTESIAN_POINT('Origin',(-0.113322216432054,0.803756648482305,
0.144261627842868));
#152992=CARTESIAN_POINT('Origin',(-0.0611017779390599,0.94650932016441,
0.177285241390716));
#152993=CARTESIAN_POINT('Ctrl Pts',(3.557907777,1.198733649,-6.31694485100001));
#152994=CARTESIAN_POINT('Ctrl Pts',(3.213805605,1.134619049,-6.510754331));
#152995=CARTESIAN_POINT('Ctrl Pts',(2.850687243,1.069390921,-6.666039472));
#152996=CARTESIAN_POINT('Ctrl Pts',(2.84704590183182,1.06873681508671,-6.6675966672176));
#152997=CARTESIAN_POINT('Ctrl Pts',(2.84340456066365,1.06808270917341,-6.6691538624352));
#152998=CARTESIAN_POINT('Ctrl Pts',(3.892924945,1.198733649,-6.410548758));
#152999=CARTESIAN_POINT('Ctrl Pts',(3.543723898,1.134619049,-6.622607587));
#153000=CARTESIAN_POINT('Ctrl Pts',(3.173554525,1.069390921,-6.795480239));
#153001=CARTESIAN_POINT('Ctrl Pts',(3.16984247648315,1.06873681508671,-6.7972138013049));
#153002=CARTESIAN_POINT('Ctrl Pts',(3.1661304279663,1.06808270917341,-6.79894736360979));
#153003=CARTESIAN_POINT('',(3.01212090167396,1.06939091791719,-6.73075984759063));
#153004=CARTESIAN_POINT('Ctrl Pts',(2.85792658132718,1.06811592995212,-6.66294361747869));
#153005=CARTESIAN_POINT('Ctrl Pts',(2.85430691216359,1.06875342547606,-6.66449154473935));
#153006=CARTESIAN_POINT('Ctrl Pts',(2.850687243,1.069390921,-6.666039472));
#153007=CARTESIAN_POINT('Ctrl Pts',(2.844901262,1.070409947,-6.66851380800001));
#153008=CARTESIAN_POINT('Ctrl Pts',(2.839110994,1.071428571,-6.670978097));
#153009=CARTESIAN_POINT('Ctrl Pts',(2.48057809,1.134501699,-6.823566622));
#153010=CARTESIAN_POINT('Ctrl Pts',(2.107755942,1.198754474,-6.93684834));
#153011=CARTESIAN_POINT('Ctrl Pts',(2.72883644918952,1.06811592995212,-6.98595147272629));
#153012=CARTESIAN_POINT('Ctrl Pts',(2.72504146259476,1.06875342547606,-6.98742911336314));
#153013=CARTESIAN_POINT('Ctrl Pts',(2.721246476,1.069390921,-6.988906754));
#153014=CARTESIAN_POINT('Ctrl Pts',(2.715180253,1.070409947,-6.991268738));
#153015=CARTESIAN_POINT('Ctrl Pts',(2.709109939,1.071428571,-6.993620188));
#153016=CARTESIAN_POINT('Ctrl Pts',(2.333236578,1.134501699,-7.139221784));
#153017=CARTESIAN_POINT('Ctrl Pts',(1.943922727,1.198754474,-7.243698257));
#153018=CARTESIAN_POINT('',(2.72124646772611,1.06939091911157,-6.98890675455456));
#153019=CARTESIAN_POINT('',(2.18395669755006,1.15903910587617,-7.17497966133097));
#153020=CARTESIAN_POINT('Origin',(-0.0253943220334973,1.33838395587535,
0.181329189256539));
#153021=CARTESIAN_POINT('Ctrl Pts',(2.11228910713819,1.19797317338517,-6.93546932305721));
#153022=CARTESIAN_POINT('Ctrl Pts',(2.1241050465527,1.19116562424527,-6.97536428671798));
#153023=CARTESIAN_POINT('Ctrl Pts',(2.13599581747036,1.18452215738752,-7.01529257794451));
#153024=CARTESIAN_POINT('Ctrl Pts',(2.15988442353831,1.17155461460947,-7.09511457081028));
#153025=CARTESIAN_POINT('Ctrl Pts',(2.17189643372923,1.16522285276294,-7.13505560849572));
#153026=CARTESIAN_POINT('Ctrl Pts',(2.18395669573087,1.15903910503581,-7.17497966175034));
#153027=CARTESIAN_POINT('',(2.78596684358495,1.06939091820872,-6.82747311949418));
#153028=CARTESIAN_POINT('Origin',(-1.41271543074861E-13,1.16011713400044,
2.67581096169422E-13));
#153029=CARTESIAN_POINT('',(2.1901964674615,0.979367659171838,-7.17307740322741));
#153030=CARTESIAN_POINT('Origin',(-0.050955182254146,0.946436337456487,
0.185026366150669));
#153031=CARTESIAN_POINT('',(1.63853121200223,1.06939091992734,-7.31882609525481));
#153032=CARTESIAN_POINT('Origin',(-0.0796607088836709,0.803756648666082,
0.165249406374038));
#153033=CARTESIAN_POINT('Origin',(-0.0215621339804298,0.946509307655302,
0.186275393095969));
#153034=CARTESIAN_POINT('Ctrl Pts',(2.116769455,1.198733649,-6.934103192));
#153035=CARTESIAN_POINT('Ctrl Pts',(1.739048891,1.134619049,-7.049409718));
#153036=CARTESIAN_POINT('Ctrl Pts',(1.35103832,1.069390921,-7.123004665));
#153037=CARTESIAN_POINT('Ctrl Pts',(1.34714736042944,1.06873681508671,-7.12374267314921));
#153038=CARTESIAN_POINT('Ctrl Pts',(1.34325640085888,1.06808270917341,-7.1244806812984));
#153039=CARTESIAN_POINT('Ctrl Pts',(2.423832035,1.198733649,-7.097537479));
#153040=CARTESIAN_POINT('Ctrl Pts',(2.037208734,1.134619049,-7.22957058800001));
#153041=CARTESIAN_POINT('Ctrl Pts',(1.638531205,1.069390921,-7.3188261));
#153042=CARTESIAN_POINT('Ctrl Pts',(1.6345332774615,1.06873681508671,-7.31972115187383));
#153043=CARTESIAN_POINT('Ctrl Pts',(1.630535349923,1.06808270917341,-7.32061620374768));
#153044=CARTESIAN_POINT('',(1.49478478146109,1.06939091791719,-7.22091537857491));
#153045=CARTESIAN_POINT('Ctrl Pts',(1.35877392497451,1.06811592995337,-7.12153743298077));
#153046=CARTESIAN_POINT('Ctrl Pts',(1.35490612248726,1.06875342547668,-7.12227104899038));
#153047=CARTESIAN_POINT('Ctrl Pts',(1.35103832,1.069390921,-7.123004665));
#153048=CARTESIAN_POINT('Ctrl Pts',(1.344855702,1.070409947,-7.124177338));
#153049=CARTESIAN_POINT('Ctrl Pts',(1.338671059,1.071428571,-7.125339276));
#153050=CARTESIAN_POINT('Ctrl Pts',(0.955718432,1.134501699,-7.19728639));
#153051=CARTESIAN_POINT('Ctrl Pts',(0.567260438,1.198754474,-7.227773903));
#153052=CARTESIAN_POINT('Ctrl Pts',(1.16326470617094,1.06811592995337,-7.40924298181097));
#153053=CARTESIAN_POINT('Ctrl Pts',(1.15924079508547,1.06875342547668,-7.40987026640548));
#153054=CARTESIAN_POINT('Ctrl Pts',(1.155216884,1.069390921,-7.410497551));
#153055=CARTESIAN_POINT('Ctrl Pts',(1.148784729,1.070409947,-7.411500255));
#153056=CARTESIAN_POINT('Ctrl Pts',(1.142350843,1.071428571,-7.412491791));
#153057=CARTESIAN_POINT('Ctrl Pts',(0.743965153,1.134501699,-7.47388764));
#153058=CARTESIAN_POINT('Ctrl Pts',(0.341293891,1.198754474,-7.492230541));
#153059=CARTESIAN_POINT('',(1.15521687581794,1.06939091911024,-7.41049754966549));
#153060=CARTESIAN_POINT('',(0.590488466701952,1.15903910589274,-7.47671875687175));
#153061=CARTESIAN_POINT('Origin',(0.0141798106748021,1.33838402878226,0.182548839069203));
#153062=CARTESIAN_POINT('Ctrl Pts',(0.571984068188111,1.19797317337619,
-7.22740162320938));
#153063=CARTESIAN_POINT('Ctrl Pts',(0.574947519443085,1.19116562425375,
-7.26890394257768));
#153064=CARTESIAN_POINT('Ctrl Pts',(0.577976888262406,1.18452215740707,
-7.31045489687104));
#153065=CARTESIAN_POINT('Ctrl Pts',(0.584147622817373,1.17155461463842,
-7.39354604020064));
#153066=CARTESIAN_POINT('Ctrl Pts',(0.587292656358846,1.16522285274723,
-7.43513550608413));
#153067=CARTESIAN_POINT('Ctrl Pts',(0.590488464750283,1.15903910503688,
-7.47671875689447));
#153068=CARTESIAN_POINT('',(1.25312758504849,1.06939091820667,-7.26675111092324));
#153069=CARTESIAN_POINT('Origin',(1.5748036555352E-14,1.16011713400006,
7.30318583386236E-13));
#153070=CARTESIAN_POINT('',(0.596991284787135,0.979367659177192,-7.47620233853123));
#153071=CARTESIAN_POINT('Origin',(-0.00998869212352212,0.946436346326042,
0.191654495969603));
#153072=CARTESIAN_POINT('',(0.0268919958833657,1.06939091992737,-7.49995178487649));
#153073=CARTESIAN_POINT('Origin',(-0.042274564920128,0.803756675780424,
0.178510930582303));
#153074=CARTESIAN_POINT('Origin',(0.0189856731973442,0.946509307003066,
0.186555619158163));
#153075=CARTESIAN_POINT('Ctrl Pts',(0.576653346,1.198733649,-7.227030574));
#153076=CARTESIAN_POINT('Ctrl Pts',(0.182976184,1.134619049,-7.258442542));
#153077=CARTESIAN_POINT('Ctrl Pts',(-0.211783654,1.069390921,-7.246906077));
#153078=CARTESIAN_POINT('Ctrl Pts',(-0.215742295038516,1.06873681508671,
-7.24679038963925));
#153079=CARTESIAN_POINT('Ctrl Pts',(-0.219700936077032,1.06808270917341,
-7.24667470227851));
#153080=CARTESIAN_POINT('Ctrl Pts',(0.841403432,1.198733649,-7.452653237));
#153081=CARTESIAN_POINT('Ctrl Pts',(0.435435954,1.134619049,-7.498486904));
#153082=CARTESIAN_POINT('Ctrl Pts',(0.026891988,1.069390921,-7.499951788));
#153083=CARTESIAN_POINT('Ctrl Pts',(0.0227951200966198,1.06873681508671,
-7.49996647781735));
#153084=CARTESIAN_POINT('Ctrl Pts',(0.0186982521932396,1.06808270917341,
-7.49998116763471));
#153085=CARTESIAN_POINT('',(-0.0924458136384814,1.06939091791719,-7.37342893274275));
#153086=CARTESIAN_POINT('Ctrl Pts',(-0.203913492723738,1.06811592995213,
-7.24713607501221));
#153087=CARTESIAN_POINT('Ctrl Pts',(-0.207848573361869,1.06875342547606,
-7.24702107600611));
#153088=CARTESIAN_POINT('Ctrl Pts',(-0.211783654,1.069390921,-7.246906077));
#153089=CARTESIAN_POINT('Ctrl Pts',(-0.218073815,1.070409947,-7.246722253));
#153090=CARTESIAN_POINT('Ctrl Pts',(-0.224363648,1.071428571,-7.24652751));
#153091=CARTESIAN_POINT('Ctrl Pts',(-0.613829558,1.134501699,-7.234469046));
#153092=CARTESIAN_POINT('Ctrl Pts',(-0.999759533999999,1.198754474,-7.180736792));
#153093=CARTESIAN_POINT('Ctrl Pts',(-0.45670000052831,1.06811592995213,
-7.48608652399922));
#153094=CARTESIAN_POINT('Ctrl Pts',(-0.460764682764155,1.06875342547606,
-7.48583412099961));
#153095=CARTESIAN_POINT('Ctrl Pts',(-0.464829365,1.069390921,-7.485581718));
#153096=CARTESIAN_POINT('Ctrl Pts',(-0.471326692,1.070409947,-7.485178256));
#153097=CARTESIAN_POINT('Ctrl Pts',(-0.477823308,1.071428571,-7.484763516));
#153098=CARTESIAN_POINT('Ctrl Pts',(-0.880093255,1.134501699,-7.459082817));
#153099=CARTESIAN_POINT('Ctrl Pts',(-1.277293469,1.198754474,-7.39043445200001));
#153100=CARTESIAN_POINT('',(-0.464829372799176,1.06939091911153,-7.48558171513683));
#153101=CARTESIAN_POINT('',(-1.03059034795361,1.15903910584036,-7.42885479283027));
#153102=CARTESIAN_POINT('Origin',(0.0530909045809279,1.33838406702624,0.175232705328355));
#153103=CARTESIAN_POINT('Ctrl Pts',(-0.995066310316853,1.19797317334389,
-7.18138865679072));
#153104=CARTESIAN_POINT('Ctrl Pts',(-1.0010939147494,1.19116562419481,-7.22255772936614));
#153105=CARTESIAN_POINT('Ctrl Pts',(-1.00706759778314,1.18452215732646,
-7.2637884701795));
#153106=CARTESIAN_POINT('Ctrl Pts',(-1.0189032710843,1.17155461456224,-7.34626351406299));
#153107=CARTESIAN_POINT('Ctrl Pts',(-1.02477227239017,1.16522285266749,
-7.3875567305792));
#153108=CARTESIAN_POINT('Ctrl Pts',(-1.0305903498677,1.15903910495932,-7.42885479242869));
#153109=CARTESIAN_POINT('',(-0.338306526670948,1.06939091820872,-7.3662438967114));
#153110=CARTESIAN_POINT('Origin',(-1.29291109068896E-13,1.16011713399978,
-6.56159154788227E-13));
#153111=CARTESIAN_POINT('',(-1.02412854774879,0.979367659155358,-7.42974836164533));
#153112=CARTESIAN_POINT('Origin',(0.0314449104851384,0.946436323522522,
0.189321198650079));
#153113=CARTESIAN_POINT('',(-1.58600466060697,1.06939091992739,-7.33038806365574));
#153114=CARTESIAN_POINT('Origin',(-0.0029116071295629,0.803756661929236,
0.183425348603111));
#153115=CARTESIAN_POINT('Origin',(0.0586457268839945,0.946509308198984,
0.178112571944439));
#153116=CARTESIAN_POINT('Ctrl Pts',(-0.990426433,1.198733649,-7.182030039));
#153117=CARTESIAN_POINT('Ctrl Pts',(-1.381652286,1.134619049,-7.12807866));
#153118=CARTESIAN_POINT('Ctrl Pts',(-1.764702859,1.069390921,-7.03195021400001));
#153119=CARTESIAN_POINT('Ctrl Pts',(-1.76854407984401,1.06873681508671,
-7.03098624052886));
#153120=CARTESIAN_POINT('Ctrl Pts',(-1.77238530068803,1.06808270917341,
-7.03002226705771));
#153121=CARTESIAN_POINT('Ctrl Pts',(-0.780368259,1.198733649,-7.459291212));
#153122=CARTESIAN_POINT('Ctrl Pts',(-1.186697327,1.134619049,-7.416782306));
#153123=CARTESIAN_POINT('Ctrl Pts',(-1.586004669,1.069390921,-7.330388065));
#153124=CARTESIAN_POINT('Ctrl Pts',(-1.59000891228632,1.06873681508671,
-7.3295217058748));
#153125=CARTESIAN_POINT('Ctrl Pts',(-1.59401315557265,1.06808270917341,
-7.3286553467496));
#153126=CARTESIAN_POINT('',(-1.67535374514333,1.06939091791719,-7.18116914389923));
#153127=CARTESIAN_POINT('Ctrl Pts',(-1.75706614025095,1.06811592995213,
-7.03386668559918));
#153128=CARTESIAN_POINT('Ctrl Pts',(-1.76088449962548,1.06875342547606,
-7.03290844979959));
#153129=CARTESIAN_POINT('Ctrl Pts',(-1.764702859,1.069390921,-7.031950214));
#153130=CARTESIAN_POINT('Ctrl Pts',(-1.770806443,1.070409947,-7.03041849));
#153131=CARTESIAN_POINT('Ctrl Pts',(-1.776907359,1.071428571,-7.028876172));
#153132=CARTESIAN_POINT('Ctrl Pts',(-2.154675559,1.134501699,-6.93337597));
#153133=CARTESIAN_POINT('Ctrl Pts',(-2.52003186,1.198754474,-6.79793640900001));
#153134=CARTESIAN_POINT('Ctrl Pts',(-2.05530992479782,1.06811592995213,
-7.21288898031393));
#153135=CARTESIAN_POINT('Ctrl Pts',(-2.05922531739891,1.06875342547606,
-7.21176869215696));
#153136=CARTESIAN_POINT('Ctrl Pts',(-2.06314071,1.069390921,-7.210648404));
#153137=CARTESIAN_POINT('Ctrl Pts',(-2.0693994,1.070409947,-7.208857642));
#153138=CARTESIAN_POINT('Ctrl Pts',(-2.075654973,1.071428571,-7.207056017));
#153139=CARTESIAN_POINT('Ctrl Pts',(-2.46299948,1.134501699,-7.095499572));
#153140=CARTESIAN_POINT('Ctrl Pts',(-2.836156005,1.198754474,-6.943069863));
#153141=CARTESIAN_POINT('',(-2.06314071700248,1.06939091911153,-7.21064839952851));
#153142=CARTESIAN_POINT('',(-2.60347990315653,1.15903910587584,-7.03362583537486));
#153143=CARTESIAN_POINT('Origin',(0.0895195164046692,1.33838403536281,0.159722890325232));
#153144=CARTESIAN_POINT('Ctrl Pts',(-2.51558849334323,1.19797317341412,
-6.79958193777258));
#153145=CARTESIAN_POINT('Ctrl Pts',(-2.53032530942631,1.19116562429394,
-6.83849274352607));
#153146=CARTESIAN_POINT('Ctrl Pts',(-2.54502272157404,1.18452215744368,
-6.87747536725597));
#153147=CARTESIAN_POINT('Ctrl Pts',(-2.57431138011397,1.17155461460349,
-6.9554778711486));
#153148=CARTESIAN_POINT('Ctrl Pts',(-2.58891998821519,1.16522285277055,
-6.99454401305868));
#153149=CARTESIAN_POINT('Ctrl Pts',(-2.60347990485454,1.15903910504116,
-7.0336258346102));
#153150=CARTESIAN_POINT('',(-1.91392180109997,1.06939091820872,-7.12129930453859));
#153151=CARTESIAN_POINT('Origin',(-4.17634676841416E-13,1.16011713399994,
-1.19002030452009E-12));
#153152=CARTESIAN_POINT('',(-2.59736126722514,0.979367659142584,-7.0358876089964));
#153153=CARTESIAN_POINT('Origin',(0.0714082026105445,0.946436336876394,
0.178135238070495));
#153154=CARTESIAN_POINT('',(-3.12474150253183,1.06939091992737,-6.8180635444769));
#153155=CARTESIAN_POINT('Origin',(0.0365874470695776,0.803756633914609,
0.179762794930365));
#153156=CARTESIAN_POINT('Origin',(0.0955636390219455,0.946509331580637,
0.161341518403026));
#153157=CARTESIAN_POINT('Ctrl Pts',(-2.511194972,1.198733649,-6.80120576200001));
#153158=CARTESIAN_POINT('Ctrl Pts',(-2.881676231,1.134619049,-6.66441374200001));
#153159=CARTESIAN_POINT('Ctrl Pts',(-3.23510652,1.069390921,-6.488188176));
#153160=CARTESIAN_POINT('Ctrl Pts',(-3.23865070943269,1.06873681508671,
-6.48642099076369));
#153161=CARTESIAN_POINT('Ctrl Pts',(-3.24219489886538,1.06808270917341,
-6.48465380552737));
#153162=CARTESIAN_POINT('Ctrl Pts',(-2.365650799,1.198733649,-7.11714102));
#153163=CARTESIAN_POINT('Ctrl Pts',(-2.75334196,1.134619049,-6.98827721));
#153164=CARTESIAN_POINT('Ctrl Pts',(-3.124741511,1.069390921,-6.818063544));
#153165=CARTESIAN_POINT('Ctrl Pts',(-3.12846589570875,1.06873681508671,
-6.8163566459352));
#153166=CARTESIAN_POINT('Ctrl Pts',(-3.1321902804175,1.06808270917341,-6.81464974787039));
#153167=CARTESIAN_POINT('',(-3.17992399802989,1.06939091791719,-6.65312586835001));
#153168=CARTESIAN_POINT('Ctrl Pts',(-3.22806032850427,1.06811592995213,
-6.49170151124601));
#153169=CARTESIAN_POINT('Ctrl Pts',(-3.23158342425213,1.06875342547606,
-6.48994484362301));
#153170=CARTESIAN_POINT('Ctrl Pts',(-3.23510652,1.069390921,-6.488188176));
#153171=CARTESIAN_POINT('Ctrl Pts',(-3.24073813,1.070409947,-6.485380172));
#153172=CARTESIAN_POINT('Ctrl Pts',(-3.246364857,1.071428571,-6.482562396));
#153173=CARTESIAN_POINT('Ctrl Pts',(-3.594771326,1.134501699,-6.308085939));
#153174=CARTESIAN_POINT('Ctrl Pts',(-3.922470298,1.198754474,-6.097272075));
#153175=CARTESIAN_POINT('Ctrl Pts',(-3.55781583914299,1.06811592995213,
-6.6024247660727));
#153176=CARTESIAN_POINT('Ctrl Pts',(-3.5613988635715,1.06875342547606,-6.60048897553635));
#153177=CARTESIAN_POINT('Ctrl Pts',(-3.564981888,1.069390921,-6.598553185));
#153178=CARTESIAN_POINT('Ctrl Pts',(-3.570709293,1.070409947,-6.595458856));
#153179=CARTESIAN_POINT('Ctrl Pts',(-3.576431317,1.071428571,-6.592354589));
#153180=CARTESIAN_POINT('Ctrl Pts',(-3.930738587,1.134501699,-6.400138652));
#153181=CARTESIAN_POINT('Ctrl Pts',(-4.262403038,1.198754474,-6.17105504300001));
#153182=CARTESIAN_POINT('',(-3.56498189383506,1.06939091911155,-6.59855317909549));
#153183=CARTESIAN_POINT('',(-4.05463363206377,1.15903910590348,-6.30951235096862));
#153184=CARTESIAN_POINT('Origin',(0.121762300074483,1.33838403875015,0.136744607366341));
#153185=CARTESIAN_POINT('Ctrl Pts',(-3.91848455494606,1.19797317343746,
-6.09983432463178));
#153186=CARTESIAN_POINT('Ctrl Pts',(-3.94124150543094,1.19116562430746,
-6.13466743758724));
#153187=CARTESIAN_POINT('Ctrl Pts',(-3.96397541200388,1.18452215745755,
-6.1695791600814));
#153188=CARTESIAN_POINT('Ctrl Pts',(-4.00934755051591,1.17155461463885,
-6.23946181284915));
#153189=CARTESIAN_POINT('Ctrl Pts',(-4.03201268338122,1.16522285276633,
-6.27447419137526));
#153190=CARTESIAN_POINT('Ctrl Pts',(-4.05463363359707,1.15903910506087,
-6.30951234983));
#153191=CARTESIAN_POINT('',(-3.40004421925281,1.06939091820872,-6.54337067257439));
#153192=CARTESIAN_POINT('Origin',(3.70580302555545E-13,1.16011713399972,
5.26922255827955E-13));
#153193=CARTESIAN_POINT('',(-4.04914426134537,0.979367659186683,-6.31303657114383));
#153194=CARTESIAN_POINT('Origin',(0.108032464833622,0.946436291803525,0.158619752436514));
#153195=CARTESIAN_POINT('',(-4.51736890386031,1.06939091992732,-5.98693395125204));
#153196=CARTESIAN_POINT('Origin',(0.0743757745959278,0.80375664599575,0.1676948622839));
#153197=CARTESIAN_POINT('Origin',(0.128012932444943,0.946509301500725,0.137025874713763));
#153198=CARTESIAN_POINT('Ctrl Pts',(-3.914542826,1.198733649,-6.102364662));
#153199=CARTESIAN_POINT('Ctrl Pts',(-4.246956198,1.134619049,-5.889128244));
#153200=CARTESIAN_POINT('Ctrl Pts',(-4.554240196,1.069390921,-5.641045669));
#153201=CARTESIAN_POINT('Ctrl Pts',(-4.55732163166763,1.06873681508671,
-5.63855790361001));
#153202=CARTESIAN_POINT('Ctrl Pts',(-4.56040306733527,1.06808270917341,
-5.63607013822001));
#153203=CARTESIAN_POINT('Ctrl Pts',(-3.840318136,1.198733649,-6.442201224));
#153204=CARTESIAN_POINT('Ctrl Pts',(-4.191243384,1.134619049,-6.233008039));
#153205=CARTESIAN_POINT('Ctrl Pts',(-4.517368912,1.069390921,-5.98693394900001));
#153206=CARTESIAN_POINT('Ctrl Pts',(-4.52063929002373,1.06873681508671,
-5.98446632464357));
#153207=CARTESIAN_POINT('Ctrl Pts',(-4.52390966804747,1.06808270917341,
-5.98199870028714));
#153208=CARTESIAN_POINT('',(-4.53580453873334,1.06939091791719,-5.81398982091035));
#153209=CARTESIAN_POINT('Ctrl Pts',(-4.5481140040602,1.06811592995212,-5.64599158717323));
#153210=CARTESIAN_POINT('Ctrl Pts',(-4.5511771000301,1.06875342547606,-5.64351862808662));
#153211=CARTESIAN_POINT('Ctrl Pts',(-4.554240196,1.069390921,-5.64104566900001));
#153212=CARTESIAN_POINT('Ctrl Pts',(-4.559136504,1.070409947,-5.637092685));
#153213=CARTESIAN_POINT('Ctrl Pts',(-4.564025943,1.071428571,-5.633131207));
#153214=CARTESIAN_POINT('Ctrl Pts',(-4.866779581,1.134501699,-5.387836821));
#153215=CARTESIAN_POINT('Ctrl Pts',(-5.141498385,1.198754474,-5.111506076));
#153216=CARTESIAN_POINT('Ctrl Pts',(-4.89396224110399,1.06811592995212,
-5.68323850498272));
#153217=CARTESIAN_POINT('Ctrl Pts',(-4.897045358552,1.06875342547606,-5.68057772849136));
#153218=CARTESIAN_POINT('Ctrl Pts',(-4.900128476,1.069390921,-5.677916952));
#153219=CARTESIAN_POINT('Ctrl Pts',(-4.905056788,1.070409947,-5.673663745));
#153220=CARTESIAN_POINT('Ctrl Pts',(-4.909977709,1.071428571,-5.669401988));
#153221=CARTESIAN_POINT('Ctrl Pts',(-5.214680727,1.134501699,-5.405514363));
#153222=CARTESIAN_POINT('Ctrl Pts',(-5.489344843,1.198754474,-5.110488548));
#153223=CARTESIAN_POINT('',(-4.90012848048504,1.06939091911153,-5.67791694500488));
#153224=CARTESIAN_POINT('',(-5.31619719772624,1.15903910677738,-5.29037308240282));
#153225=CARTESIAN_POINT('Origin',(0.148311690093998,1.33838494836903,0.107372169549576));
#153226=CARTESIAN_POINT('Ctrl Pts',(-5.13815663368765,1.19797317323022,
-5.11486523948492));
#153227=CARTESIAN_POINT('Ctrl Pts',(-5.16786948413822,1.19116565731859,
-5.14399175972748));
#153228=CARTESIAN_POINT('Ctrl Pts',(-5.19757671253684,1.1845222240275,-5.1731999885154));
#153229=CARTESIAN_POINT('Ctrl Pts',(-5.25691108503454,1.17155461463184,
-5.23169545535011));
#153230=CARTESIAN_POINT('Ctrl Pts',(-5.28657294587277,1.16522285281417,
-5.26101693007331));
#153231=CARTESIAN_POINT('Ctrl Pts',(-5.31619719935021,1.15903910507514,
-5.29037308040545));
#153232=CARTESIAN_POINT('',(-4.72718434919243,1.06939091820872,-5.65948129948078));
#153233=CARTESIAN_POINT('Ctrl Pts',(-5.134851007,1.198733649,-5.118183773));
#153234=CARTESIAN_POINT('Ctrl Pts',(-5.413653213,1.134619049,-4.838473655));
#153235=CARTESIAN_POINT('Ctrl Pts',(-5.660422662,1.069390921,-4.530134136));
#153236=CARTESIAN_POINT('Ctrl Pts',(-5.66289725939779,1.06873681508671,
-4.52704211559617));
#153237=CARTESIAN_POINT('Ctrl Pts',(-5.66537185679557,1.06808270917341,
-4.52395009519234));
#153238=CARTESIAN_POINT('Ctrl Pts',(-5.135416465,1.198733649,-5.46603126000001));
#153239=CARTESIAN_POINT('Ctrl Pts',(-5.433166924,1.134619049,-5.18629033999999));
#153240=CARTESIAN_POINT('Ctrl Pts',(-5.698769164,1.069390921,-4.87586197700001));
#153241=CARTESIAN_POINT('Ctrl Pts',(-5.70143261611943,1.06873681508671,
-4.87274900972471));
#153242=CARTESIAN_POINT('Ctrl Pts',(-5.70409606823886,1.06808270917341,
-4.86963604244942));
#153243=CARTESIAN_POINT('',(-5.69876914857299,1.06939091993135,-4.8758619666544));
#153244=CARTESIAN_POINT('Origin',(0.15447204525214,0.946510515245744,0.106299044358358));
#153245=CARTESIAN_POINT('',(-5.67959590065063,1.06939091791719,-4.70299807141377));
#153246=CARTESIAN_POINT('Origin',(-2.07299455379228E-13,1.160117134,-1.76941794549634E-13));
#153247=CARTESIAN_POINT('',(-5.3115937688696,0.979367660225015,-5.29499496096233));
#153248=CARTESIAN_POINT('Origin',(0.139605180174829,0.946436327905003,0.131687433615584));
#153249=CARTESIAN_POINT('Origin',(0.108681843188683,0.803757173971954,0.147781049594621));
#153250=CARTESIAN_POINT('Ctrl Pts',(-5.65550292364228,1.06811592995212,
-4.53628137163686));
#153251=CARTESIAN_POINT('Ctrl Pts',(-5.65796279282114,1.06875342547606,
-4.53320775381843));
#153252=CARTESIAN_POINT('Ctrl Pts',(-5.660422662,1.069390921,-4.530134136));
#153253=CARTESIAN_POINT('Ctrl Pts',(-5.664354722,1.070409947,-4.525221009));
#153254=CARTESIAN_POINT('Ctrl Pts',(-5.668278248,1.071428571,-4.520301063));
#153255=CARTESIAN_POINT('Ctrl Pts',(-5.911222633,1.134501699,-4.215658441));
#153256=CARTESIAN_POINT('Ctrl Pts',(-6.120115721,1.198754474,-3.886731733));
#153257=CARTESIAN_POINT('Ctrl Pts',(-6.00127240686537,1.06811592995212,
-4.49831033178267));
#153258=CARTESIAN_POINT('Ctrl Pts',(-6.00371145443268,1.06875342547606,
-4.49504898289134));
#153259=CARTESIAN_POINT('Ctrl Pts',(-6.006150502,1.069390921,-4.491787634));
#153260=CARTESIAN_POINT('Ctrl Pts',(-6.010049279,1.070409947,-4.486574422));
#153261=CARTESIAN_POINT('Ctrl Pts',(-6.013939,1.071428571,-4.48135445));
#153262=CARTESIAN_POINT('Ctrl Pts',(-6.254790191,1.134501699,-4.158134229));
#153263=CARTESIAN_POINT('Ctrl Pts',(-6.459610984,1.198754474,-3.810961288));
#153264=CARTESIAN_POINT('',(-6.0061505046738,1.0693909191116,-4.4917876261598));
#153265=CARTESIAN_POINT('',(-5.83328659251519,1.06939091820872,-4.51096087140242));
#153266=CARTESIAN_POINT('',(-6.32918129250909,1.15903910586461,-4.02386184692367));
#153267=CARTESIAN_POINT('Origin',(0.167926042615231,1.3383840767741,0.0729793754949004));
#153268=CARTESIAN_POINT('Ctrl Pts',(-6.11757421903209,1.19797317328605,
-3.89073073857305));
#153269=CARTESIAN_POINT('Ctrl Pts',(-6.15285373554259,1.1911656583077,-3.91278890943602));
#153270=CARTESIAN_POINT('Ctrl Pts',(-6.188145325728,1.18452222597648,-3.93492808663254));
#153271=CARTESIAN_POINT('Ctrl Pts',(-6.25866730043927,1.17155461461106,
-3.97930083247413));
#153272=CARTESIAN_POINT('Ctrl Pts',(-6.29393893410434,1.16522285272675,
-4.0015603643175));
#153273=CARTESIAN_POINT('Ctrl Pts',(-6.32918129341782,1.15903910500407,
-4.02386184524901));
#153274=CARTESIAN_POINT('Origin',(-6.17127876578749E-13,1.16011713399983,
-4.562322741819E-13));
#153275=CARTESIAN_POINT('',(-6.61370129654141,1.06939091992739,-3.53680012252872));
#153276=CARTESIAN_POINT('Origin',(0.173717228195296,0.946509319216001,0.0706101781319868));
#153277=CARTESIAN_POINT('',(-6.32567905567461,0.979367659158276,-4.02936527022592));
#153278=CARTESIAN_POINT('Origin',(0.164650191334943,0.946436337767066,0.0985976552067486));
#153279=CARTESIAN_POINT('Origin',(0.137914834916094,0.803756629624046,0.120966140186841));
#153280=CARTESIAN_POINT('Ctrl Pts',(-6.115059263,1.198733649,-3.894682299));
#153281=CARTESIAN_POINT('Ctrl Pts',(-6.327213821,1.134619049,-3.561577415));
#153282=CARTESIAN_POINT('Ctrl Pts',(-6.501930055,1.069390921,-3.207398566));
#153283=CARTESIAN_POINT('Ctrl Pts',(-6.50368210469561,1.06873681508671,
-3.20384687002776));
#153284=CARTESIAN_POINT('Ctrl Pts',(-6.50543415439122,1.06808270917341,
-3.20029517405553));
#153285=CARTESIAN_POINT('Ctrl Pts',(-6.190388428,1.198733649,-4.234275748));
#153286=CARTESIAN_POINT('Ctrl Pts',(-6.42104161800001,1.134619049,-3.897067468));
#153287=CARTESIAN_POINT('Ctrl Pts',(-6.61370130300001,1.069390921,-3.536800117));
#153288=CARTESIAN_POINT('Ctrl Pts',(-6.61563328913966,1.06873681508671,
-3.53318736569346));
#153289=CARTESIAN_POINT('Ctrl Pts',(-6.61756527527932,1.06808270917341,
-3.52957461438691));
#153290=CARTESIAN_POINT('',(-6.55781567014536,1.06939091791719,-3.37209935871988));
#153291=CARTESIAN_POINT('Ctrl Pts',(-6.49844681077687,1.06811592995212,
-3.21445968164217));
#153292=CARTESIAN_POINT('Ctrl Pts',(-6.50018843288844,1.06875342547606,
-3.21092912382109));
#153293=CARTESIAN_POINT('Ctrl Pts',(-6.501930055,1.069390921,-3.207398566));
#153294=CARTESIAN_POINT('Ctrl Pts',(-6.504714009,1.070409947,-3.201755028));
#153295=CARTESIAN_POINT('Ctrl Pts',(-6.507488162,1.071428571,-3.196106666));
#153296=CARTESIAN_POINT('Ctrl Pts',(-6.679263483,1.134501699,-2.846360558));
#153297=CARTESIAN_POINT('Ctrl Pts',(-6.81256324800001,1.198754474,-2.480218134));
#153298=CARTESIAN_POINT('Ctrl Pts',(-6.82796974558505,1.06811592995212,
-3.10304616523142));
#153299=CARTESIAN_POINT('Ctrl Pts',(-6.82965067579253,1.06875342547606,
-3.09933674161571));
#153300=CARTESIAN_POINT('Ctrl Pts',(-6.831331606,1.069390921,-3.095627318));
#153301=CARTESIAN_POINT('Ctrl Pts',(-6.834018545,1.070409947,-3.089697866));
#153302=CARTESIAN_POINT('Ctrl Pts',(-6.836695187,1.071428571,-3.08376376));
#153303=CARTESIAN_POINT('Ctrl Pts',(-7.002432618,1.134501699,-2.716324361));
#153304=CARTESIAN_POINT('Ctrl Pts',(-7.127832894,1.198754474,-2.333237714));
#153305=CARTESIAN_POINT('',(-6.83133160687962,1.06939091911161,-3.09562730976832));
#153306=CARTESIAN_POINT('',(-7.04621990368853,1.15903910588547,-2.56919930445691));
#153307=CARTESIAN_POINT('Origin',(0.179688433322887,1.3383840144886,0.0351740334676576));
#153308=CARTESIAN_POINT('Ctrl Pts',(-6.81094083279843,1.19797317334171,
-2.48466999264094));
#153309=CARTESIAN_POINT('Ctrl Pts',(-6.85013758504179,1.19116562421767,
-2.49862847261659));
#153310=CARTESIAN_POINT('Ctrl Pts',(-6.88936356467505,1.18452215736906,
-2.5126634787143));
#153311=CARTESIAN_POINT('Ctrl Pts',(-6.96777518862747,1.17155461462058,
-2.54083852552382));
#153312=CARTESIAN_POINT('Ctrl Pts',(-7.00700733256815,1.16522285272643,
-2.55499528336012));
#153313=CARTESIAN_POINT('Ctrl Pts',(-7.04621990422763,1.15903910502355,
-2.56919930259339));
#153314=CARTESIAN_POINT('',(-6.6666308378463,1.06939091820872,-3.15151292645983));
#153315=CARTESIAN_POINT('Origin',(9.32413868337534E-14,1.16011713400033,
1.08637057683048E-13));
#153316=CARTESIAN_POINT('',(-7.04398262080491,0.979367659166783,-2.57532693793603));
#153317=CARTESIAN_POINT('Origin',(0.181996628548818,0.946436318537255,0.0608976861711508));
#153318=CARTESIAN_POINT('',(-7.21938411488094,1.06939091992739,-2.03236142178664));
#153319=CARTESIAN_POINT('Origin',(0.160694476192415,0.803756681254556,0.0884903519069058));
#153320=CARTESIAN_POINT('Origin',(0.184834718443735,0.946509311812307,0.0316152163446676));
#153321=CARTESIAN_POINT('Ctrl Pts',(-6.80933414400001,1.198733649,-2.489069809));
#153322=CARTESIAN_POINT('Ctrl Pts',(-6.944920943,1.134619049,-2.118145774));
#153323=CARTESIAN_POINT('Ctrl Pts',(-7.039414425,1.069390921,-1.734688604));
#153324=CARTESIAN_POINT('Ctrl Pts',(-7.04036200309612,1.06873681508671,
-1.73084330581221));
#153325=CARTESIAN_POINT('Ctrl Pts',(-7.04130958119224,1.06808270917341,
-1.72699800762441));
#153326=CARTESIAN_POINT('Ctrl Pts',(-6.955904708,1.198733649,-2.804530209));
#153327=CARTESIAN_POINT('Ctrl Pts',(-7.108675543,1.134619049,-2.425622053));
#153328=CARTESIAN_POINT('Ctrl Pts',(-7.21938412,1.069390921,-2.032361415));
#153329=CARTESIAN_POINT('Ctrl Pts',(-7.22049430263268,1.06873681508671,
-2.02841780789876));
#153330=CARTESIAN_POINT('Ctrl Pts',(-7.22160448526537,1.06808270917341,
-2.02447420079752));
#153331=CARTESIAN_POINT('',(-7.12939926755414,1.06939091791719,-1.88352502822078));
#153332=CARTESIAN_POINT('Ctrl Pts',(-7.03753054804731,1.06811592995241,
-1.7423334291813));
#153333=CARTESIAN_POINT('Ctrl Pts',(-7.03847248652365,1.0687534254762,-1.73851101659065));
#153334=CARTESIAN_POINT('Ctrl Pts',(-7.039414425,1.069390921,-1.734688604));
#153335=CARTESIAN_POINT('Ctrl Pts',(-7.040920098,1.070409947,-1.728578541));
#153336=CARTESIAN_POINT('Ctrl Pts',(-7.042415162,1.071428571,-1.722465874));
#153337=CARTESIAN_POINT('Ctrl Pts',(-7.134989397,1.134501699,-1.343970018));
#153338=CARTESIAN_POINT('Ctrl Pts',(-7.186462889,1.198754474,-0.957732292));
#153339=CARTESIAN_POINT('Ctrl Pts',(-7.33539880555853,1.06811592995241,
-1.56268700810849));
#153340=CARTESIAN_POINT('Ctrl Pts',(-7.33624302077927,1.0687534254762,-1.55870295855425));
#153341=CARTESIAN_POINT('Ctrl Pts',(-7.337087236,1.069390921,-1.554718909));
#153342=CARTESIAN_POINT('Ctrl Pts',(-7.33843670000001,1.070409947,-1.548350472));
#153343=CARTESIAN_POINT('Ctrl Pts',(-7.339775105,1.071428571,-1.541979703));
#153344=CARTESIAN_POINT('Ctrl Pts',(-7.422649079,1.134501699,-1.147502184));
#153345=CARTESIAN_POINT('Ctrl Pts',(-7.462765261,1.198754474,-0.746414538));
#153346=CARTESIAN_POINT('',(-7.33708723535121,1.06939091911119,-1.55471890071167));
#153347=CARTESIAN_POINT('',(-7.43378510362113,1.15903910586694,-0.994403858029308));
#153348=CARTESIAN_POINT('Origin',(0.183048793396375,1.33838406389971,-0.00427602568615876));
#153349=CARTESIAN_POINT('Ctrl Pts',(-7.18583542313158,1.19797317327582,
-0.962428840202223));
#153350=CARTESIAN_POINT('Ctrl Pts',(-7.22711623435964,1.19116565769764,
-0.967634809917467));
#153351=CARTESIAN_POINT('Ctrl Pts',(-7.26844201747691,1.18452222476187,
-0.972909229448894));
#153352=CARTESIAN_POINT('Ctrl Pts',(-7.35107765327792,1.17155461459036,
-0.983569433385695));
#153353=CARTESIAN_POINT('Ctrl Pts',(-7.39243585582729,1.16522285272814,
-0.988961462780946));
#153354=CARTESIAN_POINT('Ctrl Pts',(-7.43378510374658,1.15903910501563,
-0.994403856108894));
#153355=CARTESIAN_POINT('',(-7.18825083433454,1.06939091820823,-1.64470373974097));
#153356=CARTESIAN_POINT('Origin',(-9.86623976961809E-13,1.16011713399994,
-1.70219741080224E-13));
#153357=CARTESIAN_POINT('',(-7.43291738723043,0.97936765919445,-1.0008691806923));
#153358=CARTESIAN_POINT('Origin',(0.190832825435658,0.946436294533378,0.0203500377589748));
#153359=CARTESIAN_POINT('',(-7.4874965564513,1.06939091992734,-0.432891760688444));
#153360=CARTESIAN_POINT('Origin',(0.175960374723034,0.803756653729906,0.0518769504748556));
#153361=CARTESIAN_POINT('Origin',(0.187309731526595,0.946509314557843,-0.00885792245696237));
#153362=CARTESIAN_POINT('Ctrl Pts',(-7.185212128,1.198733649,-0.967071182));
#153363=CARTESIAN_POINT('Ctrl Pts',(-7.23789128,1.134619049,-0.575671991));
#153364=CARTESIAN_POINT('Ctrl Pts',(-7.2477436,1.069390921,-0.180866531));
#153365=CARTESIAN_POINT('Ctrl Pts',(-7.24784239879999,1.06873681508671,
-0.176907432465295));
#153366=CARTESIAN_POINT('Ctrl Pts',(-7.24794119759997,1.06808270917341,
-0.17294833393059));
#153367=CARTESIAN_POINT('Ctrl Pts',(-7.39617061500001,1.198733649,-1.243647954));
#153368=CARTESIAN_POINT('Ctrl Pts',(-7.4639157,1.134619049,-0.840757247));
#153369=CARTESIAN_POINT('Ctrl Pts',(-7.48749656,1.069390921,-0.432891753));
#153370=CARTESIAN_POINT('Ctrl Pts',(-7.48773302822988,1.06873681508671,
-0.428801688795589));
#153371=CARTESIAN_POINT('Ctrl Pts',(-7.48796949645976,1.06808270917341,
-0.424711624591177));
#153372=CARTESIAN_POINT('',(-7.36762007919418,1.06939091791717,-0.306879161346403));
#153373=CARTESIAN_POINT('Ctrl Pts',(-7.2475471775637,1.06811592995236,-0.188737601887027));
#153374=CARTESIAN_POINT('Ctrl Pts',(-7.24764538878185,1.06875342547618,
-0.184802066443513));
#153375=CARTESIAN_POINT('Ctrl Pts',(-7.2477436,1.069390921,-0.180866531));
#153376=CARTESIAN_POINT('Ctrl Pts',(-7.247900589,1.070409947,-0.174575643));
#153377=CARTESIAN_POINT('Ctrl Pts',(-7.248046656,1.071428571,-0.168284491));
#153378=CARTESIAN_POINT('Ctrl Pts',(-7.257091136,1.134501699,0.221263065));
#153379=CARTESIAN_POINT('Ctrl Pts',(-7.224331513,1.198754474,0.609536047));
#153380=CARTESIAN_POINT('Ctrl Pts',(-7.49983277261797,1.06811592995236,
0.0507416564256056));
#153381=CARTESIAN_POINT('Ctrl Pts',(-7.49980079730899,1.06875342547618,
0.0548140422128028));
#153382=CARTESIAN_POINT('Ctrl Pts',(-7.499768822,1.069390921,0.058886428));
#153383=CARTESIAN_POINT('Ctrl Pts',(-7.49971771,1.070409947,0.065396069));
#153384=CARTESIAN_POINT('Ctrl Pts',(-7.499655298,1.071428571,0.071905611));
#153385=CARTESIAN_POINT('Ctrl Pts',(-7.495790718,1.134501699,0.474975919));
#153386=CARTESIAN_POINT('Ctrl Pts',(-7.44874701800001,1.198754474,0.875310152000001));
#153387=CARTESIAN_POINT('',(-7.49976881957978,1.06939091911126,0.0588864359523553));
#153388=CARTESIAN_POINT('',(-7.47375477398927,1.15903910588506,0.626888807520051));
#153389=CARTESIAN_POINT('Origin',(0.177849996470257,1.33838404543367,-0.0435261314210013));
#153390=CARTESIAN_POINT('Ctrl Pts',(-7.22472833593332,1.19797317330152,
0.604814415005951));
#153391=CARTESIAN_POINT('Ctrl Pts',(-7.26616317337376,1.19116565457661,
0.608604313924491));
#153392=CARTESIAN_POINT('Ctrl Pts',(-7.30765664821257,1.18452221845763,
0.612337031058701));
#153393=CARTESIAN_POINT('Ctrl Pts',(-7.39065189683772,1.17155461462232,
0.619690272251385));
#153394=CARTESIAN_POINT('Ctrl Pts',(-7.43220229451985,1.16522285275759,
0.623315096548411));
#153395=CARTESIAN_POINT('Ctrl Pts',(-7.47375477370222,1.15903910504407,
0.626888809402448));
#153396=CARTESIAN_POINT('',(-7.37375621114219,1.06939091820832,-0.0609900343090774));
#153397=CARTESIAN_POINT('Origin',(-1.4658413372004E-13,1.16011713400011,
-1.77097648611929E-13));
#153398=CARTESIAN_POINT('',(-7.47429719740142,0.97936765915432,0.620388107456751));
#153399=CARTESIAN_POINT('Origin',(0.190745673161867,0.946436329317841,-0.0211491355141363));
#153400=CARTESIAN_POINT('',(-7.40550198016269,1.06939091992728,1.18681943978567));
#153401=CARTESIAN_POINT('Origin',(0.182998526930598,0.803756652297692,0.0128378233106978));
#153402=CARTESIAN_POINT('Origin',(0.181026394733831,0.946509328684528,-0.048916885303092));
#153403=CARTESIAN_POINT('Ctrl Pts',(-7.225117579,1.198733649,0.600146619));
#153404=CARTESIAN_POINT('Ctrl Pts',(-7.19242586500001,1.134619049,0.993719575));
#153405=CARTESIAN_POINT('Ctrl Pts',(-7.11717634000001,1.069390921,1.381412661));
#153406=CARTESIAN_POINT('Ctrl Pts',(-7.11642173978711,1.06873681508671,
1.38530043683952));
#153407=CARTESIAN_POINT('Ctrl Pts',(-7.11566713957423,1.06808270917341,
1.38918821267904));
#153408=CARTESIAN_POINT('Ctrl Pts',(-7.490599804,1.198733649,0.375385897));
#153409=CARTESIAN_POINT('Ctrl Pts',(-7.470151454,1.134619049,0.783420434));
#153410=CARTESIAN_POINT('Ctrl Pts',(-7.405501982,1.069390921,1.186819448));
#153411=CARTESIAN_POINT('Ctrl Pts',(-7.40485367883351,1.06873681508671,
1.1908647224631));
#153412=CARTESIAN_POINT('Ctrl Pts',(-7.40420537566703,1.06808270917341,
1.19490999692619));
#153413=CARTESIAN_POINT('',(-7.26133916437191,1.06939091791719,1.28411603543277));
#153414=CARTESIAN_POINT('Ctrl Pts',(-7.11867655828793,1.06811592995212,
1.37368338701899));
#153415=CARTESIAN_POINT('Ctrl Pts',(-7.11792644914396,1.06875342547606,
1.3775480240095));
#153416=CARTESIAN_POINT('Ctrl Pts',(-7.11717634,1.069390921,1.381412661));
#153417=CARTESIAN_POINT('Ctrl Pts',(-7.115977303,1.070409947,1.387590219));
#153418=CARTESIAN_POINT('Ctrl Pts',(-7.114767544,1.071428571,1.393765687));
#153419=CARTESIAN_POINT('Ctrl Pts',(-7.03985936,1.134501699,1.776150134));
#153420=CARTESIAN_POINT('Ctrl Pts',(-6.92439842400001,1.198754474,2.148303159));
#153421=CARTESIAN_POINT('Ctrl Pts',(-7.31358289534331,1.06811592995212,
1.66179769895285));
#153422=CARTESIAN_POINT('Ctrl Pts',(-7.31267622467166,1.06875342547606,
1.66576800047642));
#153423=CARTESIAN_POINT('Ctrl Pts',(-7.311769554,1.069390921,1.669738302));
#153424=CARTESIAN_POINT('Ctrl Pts',(-7.310320256,1.070409947,1.676084763));
#153425=CARTESIAN_POINT('Ctrl Pts',(-7.308859943,1.071428571,1.682428699));
#153426=CARTESIAN_POINT('Ctrl Pts',(-7.218437514,1.134501699,2.075244676));
#153427=CARTESIAN_POINT('Ctrl Pts',(-7.086433643,1.198754474,2.456106313));
#153428=CARTESIAN_POINT('',(-7.3117695495949,1.06939091911166,1.66973830899131));
#153429=CARTESIAN_POINT('',(-7.16425997754007,1.15903910587629,2.2188688494947));
#153430=CARTESIAN_POINT('Origin',(0.16433513636284,1.33838399167333,-0.0807409994602218));
#153431=CARTESIAN_POINT('Ctrl Pts',(-6.92580098057473,1.19797317334101,
2.14377722136203));
#153432=CARTESIAN_POINT('Ctrl Pts',(-6.9654525554008,1.19116562422871,2.15638583603037));
#153433=CARTESIAN_POINT('Ctrl Pts',(-7.0051737095645,1.18452215739093,2.16895121642368));
#153434=CARTESIAN_POINT('Ctrl Pts',(-7.08464747190185,1.17155461458958,
2.19397395012068));
#153435=CARTESIAN_POINT('Ctrl Pts',(-7.12444721430514,1.16522285272146,
2.20644613523128));
#153436=CARTESIAN_POINT('Ctrl Pts',(-7.16425997685052,1.15903910502031,
2.21886885127851));
#153437=CARTESIAN_POINT('',(-7.21447294344383,1.06939091820872,1.52557549831721));
#153438=CARTESIAN_POINT('Origin',(1.20303073058992E-12,1.16011713400017,
-3.39246859770714E-13));
#153439=CARTESIAN_POINT('',(-7.16618717794668,0.979367659170003,2.21263673771568));
#153440=CARTESIAN_POINT('Origin',(0.181740147034324,0.946436360213773,-0.0616594867204892));
#153441=CARTESIAN_POINT('',(-6.97723436100213,1.06939091992733,2.7510362805412));
#153442=CARTESIAN_POINT('Origin',(0.181479818422117,0.803756624957982,-0.0268015869709309));
#153443=CARTESIAN_POINT('Origin',(0.166278516225549,0.94650930964704,-0.0866886107508608));
#153444=CARTESIAN_POINT('Ctrl Pts',(-6.927184563,1.198733649,2.139302231));
#153445=CARTESIAN_POINT('Ctrl Pts',(-6.810650611,1.134619049,2.516645918));
#153446=CARTESIAN_POINT('Ctrl Pts',(-6.653817825,1.069390921,2.879098531));
#153447=CARTESIAN_POINT('Ctrl Pts',(-6.65224511003996,1.06873681508671,
2.88273319605511));
#153448=CARTESIAN_POINT('Ctrl Pts',(-6.65067239507993,1.06808270917341,
2.88636786111022));
#153449=CARTESIAN_POINT('Ctrl Pts',(-7.234776872,1.198733649,1.976867121));
#153450=CARTESIAN_POINT('Ctrl Pts',(-7.127091228,1.134619049,2.370966246));
#153451=CARTESIAN_POINT('Ctrl Pts',(-6.977234361,1.069390921,2.751036289));
#153452=CARTESIAN_POINT('Ctrl Pts',(-6.97573160036808,1.06873681508671,
2.75484762116934));
#153453=CARTESIAN_POINT('Ctrl Pts',(-6.97422883973616,1.06808270917341,
2.75865895333867));
#153454=CARTESIAN_POINT('',(-6.81552610039196,1.06939091791719,2.8150673921034));
#153455=CARTESIAN_POINT('Ctrl Pts',(-6.65694453501886,1.06811592995212,
2.87187246525374));
#153456=CARTESIAN_POINT('Ctrl Pts',(-6.65538118000943,1.06875342547606,
2.87548549812687));
#153457=CARTESIAN_POINT('Ctrl Pts',(-6.653817825,1.069390921,2.879098531));
#153458=CARTESIAN_POINT('Ctrl Pts',(-6.651318828,1.070409947,2.884873904));
#153459=CARTESIAN_POINT('Ctrl Pts',(-6.64880981,1.071428571,2.890644931));
#153460=CARTESIAN_POINT('Ctrl Pts',(-6.49345158400001,1.134501699,3.247986396));
#153461=CARTESIAN_POINT('Ctrl Pts',(-6.300688161,1.198754474,3.586618002));
#153462=CARTESIAN_POINT('Ctrl Pts',(-6.78535800869692,1.06811592995212,
3.19514992667576));
#153463=CARTESIAN_POINT('Ctrl Pts',(-6.78361903784846,1.06875342547606,
3.19883249733788));
#153464=CARTESIAN_POINT('Ctrl Pts',(-6.78188006700001,1.069390921,3.202515068));
#153465=CARTESIAN_POINT('Ctrl Pts',(-6.779100351,1.070409947,3.208401596));
#153466=CARTESIAN_POINT('Ctrl Pts',(-6.776310422,1.071428571,3.21428329));
#153467=CARTESIAN_POINT('Ctrl Pts',(-6.603558194,1.134501699,3.578477299));
#153468=CARTESIAN_POINT('Ctrl Pts',(-6.392766507,1.198754474,3.922057672));
#153469=CARTESIAN_POINT('',(-6.78188006127793,1.06939091911161,3.20251507397874));
#153470=CARTESIAN_POINT('',(-6.51977234700602,1.15903910587942,3.70709705022766));
#153471=CARTESIAN_POINT('Origin',(0.143136145802599,1.3383839765348,-0.11418051460323));
#153472=CARTESIAN_POINT('Ctrl Pts',(-6.30303086913351,1.19797317342552,
3.58249938691693));
#153473=CARTESIAN_POINT('Ctrl Pts',(-6.33904493282402,1.19116562428146,
3.60333713566231));
#153474=CARTESIAN_POINT('Ctrl Pts',(-6.37513624316441,1.18452215742029,
3.62414761846004));
#153475=CARTESIAN_POINT('Ctrl Pts',(-6.44737280500721,1.17155461459444,
3.66566984427696));
#153476=CARTESIAN_POINT('Ctrl Pts',(-6.48356090047984,1.16522285270483,
3.68640620487469));
#153477=CARTESIAN_POINT('Ctrl Pts',(-6.51977234593288,1.15903910501135,
3.70709705184634));
#153478=CARTESIAN_POINT('',(-6.71784893891174,1.06939091820871,3.0408068151596));
#153479=CARTESIAN_POINT('Origin',(4.87023615880489E-13,1.16011713399989,
-2.53703308361608E-13));
#153480=CARTESIAN_POINT('',(-6.5229942104888,0.979367659169073,3.70142493227494));
#153481=CARTESIAN_POINT('Origin',(0.16423608862457,0.946436316923738,-0.0992866306007983));
#153482=CARTESIAN_POINT('',(-6.22271901884537,1.06939091992734,4.18661772371598));
#153483=CARTESIAN_POINT('Origin',(0.171475441864284,0.803756611867204,-0.0651878064944689));
#153484=CARTESIAN_POINT('Origin',(0.143755515321106,0.946509288269899,-0.120406833011424));
#153485=CARTESIAN_POINT('Ctrl Pts',(-6.305344095,1.198733649,3.578426449));
#153486=CARTESIAN_POINT('Ctrl Pts',(-6.110416904,1.134619049,3.921896695));
#153487=CARTESIAN_POINT('Ctrl Pts',(-5.879334183,1.069390921,4.242160954));
#153488=CARTESIAN_POINT('Ctrl Pts',(-5.87701689168871,1.06873681508671,
4.24537255537584));
#153489=CARTESIAN_POINT('Ctrl Pts',(-5.87469960037743,1.06808270917341,
4.24858415675168));
#153490=CARTESIAN_POINT('Ctrl Pts',(-6.64066381400001,1.198733649,3.485912235));
#153491=CARTESIAN_POINT('Ctrl Pts',(-6.450776138,1.134619049,3.847648312));
#153492=CARTESIAN_POINT('Ctrl Pts',(-6.222719017,1.069390921,4.186617732));
#153493=CARTESIAN_POINT('Ctrl Pts',(-6.22043206632414,1.06873681508671,
4.19001690822728));
#153494=CARTESIAN_POINT('Ctrl Pts',(-6.21814511564828,1.06808270917341,
4.19341608445456));
#153495=CARTESIAN_POINT('',(-6.05102661106638,1.06939091791719,4.21438932711088));
#153496=CARTESIAN_POINT('Ctrl Pts',(-5.88394118241394,1.06811592995282,
4.23577597926674));
#153497=CARTESIAN_POINT('Ctrl Pts',(-5.88163768270697,1.06875342547641,
4.23896846663337));
#153498=CARTESIAN_POINT('Ctrl Pts',(-5.879334183,1.069390921,4.242160954));
#153499=CARTESIAN_POINT('Ctrl Pts',(-5.875652077,1.070409947,4.247264092));
#153500=CARTESIAN_POINT('Ctrl Pts',(-5.871961118,1.071428571,4.25236083));
#153501=CARTESIAN_POINT('Ctrl Pts',(-5.643417229,1.134501699,4.567950425));
#153502=CARTESIAN_POINT('Ctrl Pts',(-5.382364723,1.198754474,4.857226574));
#153503=CARTESIAN_POINT('Ctrl Pts',(-5.93985732264725,1.06811592995282,
4.57910049459051));
#153504=CARTESIAN_POINT('Ctrl Pts',(-5.93736736432363,1.06875342547641,
4.58232314179525));
#153505=CARTESIAN_POINT('Ctrl Pts',(-5.934877406,1.069390921,4.585545789));
#153506=CARTESIAN_POINT('Ctrl Pts',(-5.930897249,1.070409947,4.590697137));
#153507=CARTESIAN_POINT('Ctrl Pts',(-5.926908156,1.071428571,4.595841568));
#153508=CARTESIAN_POINT('Ctrl Pts',(-5.679903833,1.134501699,4.9143843));
#153509=CARTESIAN_POINT('Ctrl Pts',(-5.400180715,1.198754474,5.204617973));
#153510=CARTESIAN_POINT('',(-5.93487739907329,1.06939091911089,4.58554579351939));
#153511=CARTESIAN_POINT('',(-5.57042740808656,1.15903910589183,5.02198551255723));
#153512=CARTESIAN_POINT('Origin',(0.115244261096626,1.33838401607545,-0.142281081303194));
#153513=CARTESIAN_POINT('Ctrl Pts',(-5.38553804049224,1.19797317340481,
4.85370786275825));
#153514=CARTESIAN_POINT('Ctrl Pts',(-5.41623061527284,1.1911656242694,4.88180039563952));
#153515=CARTESIAN_POINT('Ctrl Pts',(-5.44700449210093,1.18452215741908,
4.90988290574779));
#153516=CARTESIAN_POINT('Ctrl Pts',(-5.50862615186155,1.17155461463078,
4.96596309029382));
#153517=CARTESIAN_POINT('Ctrl Pts',(-5.53951048516166,1.16522285274509,
4.99399401705785));
#153518=CARTESIAN_POINT('Ctrl Pts',(-5.57042740670401,1.15903910503806,
5.02198551389566));
#153519=CARTESIAN_POINT('',(-5.90710578420689,1.06939091820756,4.41385338527538));
#153520=CARTESIAN_POINT('Origin',(3.86843335142828E-13,1.16011713399978,
-3.00107161343988E-13));
#153521=CARTESIAN_POINT('',(-5.57479328396129,0.979367659167658,5.01713861087021));
#153522=CARTESIAN_POINT('Origin',(0.139052551745913,0.946436336407711,-0.132271185697479));
#153523=CARTESIAN_POINT('',(-5.17723625158196,1.06939091992736,5.42643757430719));
#153524=CARTESIAN_POINT('Origin',(0.153452966466637,0.803756635048499,-0.10052588202717));
#153525=CARTESIAN_POINT('Origin',(0.114510670055927,0.946509351282626,-0.14849495020988));
#153526=CARTESIAN_POINT('Ctrl Pts',(-5.388672745,1.198733649,4.850227423));
#153527=CARTESIAN_POINT('Ctrl Pts',(-5.124466893,1.134619049,5.143763941));
#153528=CARTESIAN_POINT('Ctrl Pts',(-4.829939409,1.069390921,5.40686464600001));
#153529=CARTESIAN_POINT('Ctrl Pts',(-4.82698589531168,1.06873681508671,
5.40950301279372));
#153530=CARTESIAN_POINT('Ctrl Pts',(-4.82403238162336,1.06808270917341,
5.41214137958745));
#153531=CARTESIAN_POINT('Ctrl Pts',(-5.736040696,1.198733649,4.831959968));
#153532=CARTESIAN_POINT('Ctrl Pts',(-5.472829926,1.134619049,5.144418618));
#153533=CARTESIAN_POINT('Ctrl Pts',(-5.17723624800001,1.069390921,5.426437582));
#153534=CARTESIAN_POINT('Ctrl Pts',(-5.17427204254692,1.06873681508671,
5.42926566058618));
#153535=CARTESIAN_POINT('Ctrl Pts',(-5.17130783709384,1.06808270917341,
5.43209373917236));
#153536=CARTESIAN_POINT('',(-5.00358784272335,1.06939091791719,5.4166511008613));
#153537=CARTESIAN_POINT('Ctrl Pts',(-4.83581127987199,1.06811592995214,
5.40161931776984));
#153538=CARTESIAN_POINT('Ctrl Pts',(-4.832875344436,1.06875342547607,5.40424198188491));
#153539=CARTESIAN_POINT('Ctrl Pts',(-4.829939409,1.069390921,5.406864646));
#153540=CARTESIAN_POINT('Ctrl Pts',(-4.82524636499999,1.070409947,5.411056931));
#153541=CARTESIAN_POINT('Ctrl Pts',(-4.82054605,1.071428571,5.415241063));
#153542=CARTESIAN_POINT('Ctrl Pts',(-4.529502956,1.134501699,5.674322168));
#153543=CARTESIAN_POINT('Ctrl Pts',(-4.212367892,1.198754474,5.90071663));
#153544=CARTESIAN_POINT('Ctrl Pts',(-4.81661550888194,1.06811592995214,
5.74893741316851));
#153545=CARTESIAN_POINT('Ctrl Pts',(-4.81349099094096,1.06875342547607,
5.75154944908425));
#153546=CARTESIAN_POINT('Ctrl Pts',(-4.810366473,1.069390921,5.754161485));
#153547=CARTESIAN_POINT('Ctrl Pts',(-4.805371983,1.070409947,5.758336781));
#153548=CARTESIAN_POINT('Ctrl Pts',(-4.800370252,1.071428571,5.762503401));
#153549=CARTESIAN_POINT('Ctrl Pts',(-4.490663482,1.134501699,6.020500154));
#153550=CARTESIAN_POINT('Ctrl Pts',(-4.155088474,1.198754474,6.243816123));
#153551=CARTESIAN_POINT('',(-4.81036646532958,1.06939091911155,5.75416148814387));
#153552=CARTESIAN_POINT('',(-4.36061547464227,1.1590391058868,6.10205151390795));
#153553=CARTESIAN_POINT('Origin',(0.0819636971075782,1.33838395772576,-0.163728735462429));
#153554=CARTESIAN_POINT('Ctrl Pts',(-4.21622343834094,1.19797317332506,
5.89796235369778));
#153555=CARTESIAN_POINT('Ctrl Pts',(-4.24015925230638,1.19116565867653,
5.93199592258888));
#153556=CARTESIAN_POINT('Ctrl Pts',(-4.26417660734966,1.18452222668692,
5.96603716173334));
#153557=CARTESIAN_POINT('Ctrl Pts',(-4.3123022622184,1.17155461461324,6.03405342148723));
#153558=CARTESIAN_POINT('Ctrl Pts',(-4.33643871619161,1.16522285278025,
6.06806821925712));
#153559=CARTESIAN_POINT('Ctrl Pts',(-4.36061547307682,1.15903910505355,
6.10205151487003));
#153560=CARTESIAN_POINT('',(-4.82015292799143,1.06939091820868,5.58051307673611));
#153561=CARTESIAN_POINT('Origin',(-3.27429056090622E-13,1.16011713400039,
3.59521440396193E-13));
#153562=CARTESIAN_POINT('',(-4.36592121873627,0.979367659175133,6.09825646507156));
#153563=CARTESIAN_POINT('Origin',(0.10736725186915,0.946436344476906,-0.159071021017346));
#153564=CARTESIAN_POINT('',(-3.88967167115354,1.06939091992738,6.41252323525665));
#153565=CARTESIAN_POINT('Origin',(0.128255209084623,0.803756677600229,-0.131163488073143));
#153566=CARTESIAN_POINT('Origin',(0.0799114619989633,0.946509291999864,
-0.169639663453076));
#153567=CARTESIAN_POINT('Ctrl Pts',(-4.220033046,1.198733649,5.895237153));
#153568=CARTESIAN_POINT('Ctrl Pts',(-3.898902506,1.134619049,6.125114502));
#153569=CARTESIAN_POINT('Ctrl Pts',(-3.554702037,1.069390921,6.318749356));
#153570=CARTESIAN_POINT('Ctrl Pts',(-3.55125040395404,1.06873681508671,
6.32069112110816));
#153571=CARTESIAN_POINT('Ctrl Pts',(-3.54779877090807,1.06808270917341,
6.32263288621632));
#153572=CARTESIAN_POINT('Ctrl Pts',(-4.563206691,1.198733649,5.95207062200001));
#153573=CARTESIAN_POINT('Ctrl Pts',(-4.238980268,1.134619049,6.200641628));
#153574=CARTESIAN_POINT('Ctrl Pts',(-3.889671666,1.069390921,6.41252324200001));
#153575=CARTESIAN_POINT('Ctrl Pts',(-3.88616880873369,1.06873681508671,
6.4146479851267));
#153576=CARTESIAN_POINT('Ctrl Pts',(-3.88266595146739,1.06808270917341,
6.4167727282534));
#153577=CARTESIAN_POINT('',(-3.72218686821525,1.06939091791719,6.36563628922607));
#153578=CARTESIAN_POINT('Ctrl Pts',(-3.56156421782437,1.06811592995212,
6.31488893800863));
#153579=CARTESIAN_POINT('Ctrl Pts',(-3.55813312741219,1.06875342547606,
6.31681914700431));
#153580=CARTESIAN_POINT('Ctrl Pts',(-3.554702037,1.069390921,6.318749356));
#153581=CARTESIAN_POINT('Ctrl Pts',(-3.549217496,1.070409947,6.321834763));
#153582=CARTESIAN_POINT('Ctrl Pts',(-3.543727607,1.071428571,6.324910643));
#153583=CARTESIAN_POINT('Ctrl Pts',(-3.20379416,1.134501699,6.515368914));
#153584=CARTESIAN_POINT('Ctrl Pts',(-2.84540542,1.198754474,6.668295734));
#153585=CARTESIAN_POINT('Ctrl Pts',(-3.46815410914429,1.06811592995212,
6.64996040604056));
#153586=CARTESIAN_POINT('Ctrl Pts',(-3.46454113007215,1.06875342547606,
6.65183969552028));
#153587=CARTESIAN_POINT('Ctrl Pts',(-3.460928151,1.069390921,6.65371898500001));
#153588=CARTESIAN_POINT('Ctrl Pts',(-3.455152864,1.070409947,6.656722998));
#153589=CARTESIAN_POINT('Ctrl Pts',(-3.44937237,1.071428571,6.65971698));
#153590=CARTESIAN_POINT('Ctrl Pts',(-3.091444697,1.134501699,6.845104111));
#153591=CARTESIAN_POINT('Ctrl Pts',(-2.715708914,1.198754474,6.99106037));
#153592=CARTESIAN_POINT('',(-3.46092814283713,1.06939091911156,6.65371898649407));
#153593=CARTESIAN_POINT('',(-2.94690600790438,1.15903910589172,6.89679236883628));
#153594=CARTESIAN_POINT('Origin',(0.0448505823939493,1.33838402075146,-0.177520621225209));
#153595=CARTESIAN_POINT('Ctrl Pts',(-2.84976291363965,1.19797317337202,
6.6664346795221));
#153596=CARTESIAN_POINT('Ctrl Pts',(-2.8658229917059,1.19116562423472,6.70481824954385));
#153597=CARTESIAN_POINT('Ctrl Pts',(-2.88196106597728,1.18452215738225,
6.74322686101663));
#153598=CARTESIAN_POINT('Ctrl Pts',(-2.91433991138458,1.17155461462031,
6.81999812139951));
#153599=CARTESIAN_POINT('Ctrl Pts',(-2.93059989247976,1.16522285275017,
6.85840629648366));
#153600=CARTESIAN_POINT('Ctrl Pts',(-2.94690600609201,1.15903910504532,
6.89679236946981));
#153601=CARTESIAN_POINT('',(-3.50781507888034,1.06939091820872,6.48623417867685));
#153602=CARTESIAN_POINT('Origin',(8.12934788929631E-13,1.16011713400022,
-1.6531914726059E-12));
#153603=CARTESIAN_POINT('',(-2.95290353040653,0.979367659136253,6.89422662374214));
#153604=CARTESIAN_POINT('Origin',(0.070661430224247,0.946436330066777,-0.17843267214666));
#153605=CARTESIAN_POINT('',(-2.42023036541204,1.06939091992729,7.09876643752802));
#153606=CARTESIAN_POINT('Origin',(0.0970604625441626,0.803756636778403,
-0.155668159303939));
#153607=CARTESIAN_POINT('Origin',(0.0415756801104716,0.946509325067864,
-0.182852213635061));
#153608=CARTESIAN_POINT('Ctrl Pts',(-2.854069293,1.198733649,6.664592146));
#153609=CARTESIAN_POINT('Ctrl Pts',(-2.491029771,1.134619049,6.820061517));
#153610=CARTESIAN_POINT('Ctrl Pts',(-2.113250748,1.069390921,6.93517637));
#153611=CARTESIAN_POINT('Ctrl Pts',(-2.10946239011761,1.06873681508671,
6.93633073864991));
#153612=CARTESIAN_POINT('Ctrl Pts',(-2.10567403223522,1.06808270917341,
6.93748510729981));
#153613=CARTESIAN_POINT('Ctrl Pts',(-3.177002213,1.198733649,6.79386907));
#153614=CARTESIAN_POINT('Ctrl Pts',(-2.806920605,1.134619049,6.966929527));
#153615=CARTESIAN_POINT('Ctrl Pts',(-2.420230359,1.069390921,7.098766443));
#153616=CARTESIAN_POINT('Ctrl Pts',(-2.41635263961303,1.06873681508671,
7.10008850004794));
#153617=CARTESIAN_POINT('Ctrl Pts',(-2.41247492022606,1.06808270917341,
7.10141055709586));
#153618=CARTESIAN_POINT('',(-2.26674057192556,1.06939091791719,7.01697140054787));
#153619=CARTESIAN_POINT('Ctrl Pts',(-2.12078237087665,1.06811592995269,
6.93288137335275));
#153620=CARTESIAN_POINT('Ctrl Pts',(-2.11701655943833,1.06875342547634,
6.93402887167638));
#153621=CARTESIAN_POINT('Ctrl Pts',(-2.113250748,1.069390921,6.93517637));
#153622=CARTESIAN_POINT('Ctrl Pts',(-2.107231161,1.070409947,6.937010627));
#153623=CARTESIAN_POINT('Ctrl Pts',(-2.1012084,1.071428571,6.938834431));
#153624=CARTESIAN_POINT('Ctrl Pts',(-1.728279509,1.134501699,7.05176425));
#153625=CARTESIAN_POINT('Ctrl Pts',(-1.345394953,1.198754474,7.124072741));
#153626=CARTESIAN_POINT('Ctrl Pts',(-1.95752567888414,1.06811592995269,
7.24003864400401));
#153627=CARTESIAN_POINT('Ctrl Pts',(-1.95359317694207,1.06875342547634,
7.241097312502));
#153628=CARTESIAN_POINT('Ctrl Pts',(-1.949660675,1.069390921,7.24215598100001));
#153629=CARTESIAN_POINT('Ctrl Pts',(-1.943374636,1.070409947,7.243848245));
#153630=CARTESIAN_POINT('Ctrl Pts',(-1.93708567,1.071428571,7.245529595));
#153631=CARTESIAN_POINT('Ctrl Pts',(-1.547673393,1.134501699,7.349638609));
#153632=CARTESIAN_POINT('Ctrl Pts',(-1.149345823,1.198754474,7.411410404));
#153633=CARTESIAN_POINT('',(-1.94966066671809,1.06939091911095,7.24215598060968));
#153634=CARTESIAN_POINT('',(-1.39540249131301,1.15903910584932,7.36904687769396));
#153635=CARTESIAN_POINT('Origin',(0.0056402997146246,1.33838410971113,-0.183011834889248));
#153636=CARTESIAN_POINT('Ctrl Pts',(-1.35005064267087,1.19797317333044,
7.12319192941442));
#153637=CARTESIAN_POINT('Ctrl Pts',(-1.35748387767238,1.19116565562259,
7.16413036591661));
#153638=CARTESIAN_POINT('Ctrl Pts',(-1.36498789721534,1.18452222053175,
7.20511000403772));
#153639=CARTESIAN_POINT('Ctrl Pts',(-1.38010626517507,1.17155461459164,
7.28704728882415));
#153640=CARTESIAN_POINT('Ctrl Pts',(-1.38772947465277,1.16522285271402,
7.3280529174482));
#153641=CARTESIAN_POINT('Ctrl Pts',(-1.39540248941714,1.1590391049902,7.36904687791923));
#153642=CARTESIAN_POINT('',(-2.03145569497042,1.06939091820777,7.08866618023702));
#153643=CARTESIAN_POINT('Origin',(-3.19080699362484E-13,1.16011713400028,
1.66403349433075E-12));
#153644=CARTESIAN_POINT('',(-1.40181135465005,0.979367659141008,7.36783040844139));
#153645=CARTESIAN_POINT('Origin',(0.0306516470017276,0.946436331022197,
-0.189451099218505));
#153646=CARTESIAN_POINT('',(-0.837621778443209,1.06939091992729,7.45307921003506));
#153647=CARTESIAN_POINT('Origin',(0.061327216830241,0.80375661447446,-0.172894016761331));
#153648=CARTESIAN_POINT('Origin',(0.00129586030556517,0.946509335692072,
-0.187514887539498));
#153649=CARTESIAN_POINT('Ctrl Pts',(-1.354652431,1.198733649,7.122318217));
#153650=CARTESIAN_POINT('Ctrl Pts',(-0.966679253,1.134619049,7.196110035));
#153651=CARTESIAN_POINT('Ctrl Pts',(-0.572986203,1.069390921,7.227322244));
#153652=CARTESIAN_POINT('Ctrl Pts',(-0.569038259682857,1.06873681508671,
7.22763523919241));
#153653=CARTESIAN_POINT('Ctrl Pts',(-0.565090316365714,1.06808270917341,
7.22794823438482));
#153654=CARTESIAN_POINT('Ctrl Pts',(-1.642244642,1.198733649,7.317993751));
#153655=CARTESIAN_POINT('Ctrl Pts',(-1.243612454,1.134619049,7.407451544));
#153656=CARTESIAN_POINT('Ctrl Pts',(-0.837621771000001,1.069390921,7.453079214));
#153657=CARTESIAN_POINT('Ctrl Pts',(-0.833550507349874,1.06873681508671,
7.45353676704762));
#153658=CARTESIAN_POINT('Ctrl Pts',(-0.829479243699748,1.06808270917341,
7.45399432009523));
#153659=CARTESIAN_POINT('',(-0.705304006274312,1.06939091791719,7.34020072714797));
#153660=CARTESIAN_POINT('Origin',(1.09775469964157E-14,1.16011713400033,
-2.83193607453214E-13));
#153661=CARTESIAN_POINT('',(0.214827962323003,0.979367659150024,7.49692263181167));
#153662=CARTESIAN_POINT('',(-0.347229223939931,1.06939091911043,7.49195780996947));
#153663=CARTESIAN_POINT('Origin',(-0.010791358648808,0.94643631321699,-0.19161089903692));
#153664=CARTESIAN_POINT('Origin',(0.0227263342227098,0.803756637030686,
-0.182035181962791));
#153665=CARTESIAN_POINT('Origin',(-0.0338336897090269,1.33838403136748,
-0.179945622470713));
#153666=CARTESIAN_POINT('Ctrl Pts',(-0.580835096610768,1.06811592995312,
7.22669998041471));
#153667=CARTESIAN_POINT('Ctrl Pts',(-0.576910649805384,1.06875342547656,
7.22701111220736));
#153668=CARTESIAN_POINT('Ctrl Pts',(-0.572986203,1.069390921,7.227322244));
#153669=CARTESIAN_POINT('Ctrl Pts',(-0.56671304,1.070409947,7.227819583));
#153670=CARTESIAN_POINT('Ctrl Pts',(-0.560439023,1.071428571,7.228306033));
#153671=CARTESIAN_POINT('Ctrl Pts',(-0.17195243,1.134501699,7.258426928));
#153672=CARTESIAN_POINT('Ctrl Pts',(0.217524687,1.198754474,7.246736025));
#153673=CARTESIAN_POINT('Ctrl Pts',(-0.355365520528548,1.06811592995312,
7.49158071955915));
#153674=CARTESIAN_POINT('Ctrl Pts',(-0.351297376264274,1.06875342547656,
7.49176926577957));
#153675=CARTESIAN_POINT('Ctrl Pts',(-0.347229232,1.069390921,7.49195781200001));
#153676=CARTESIAN_POINT('Ctrl Pts',(-0.340726371,1.070409947,7.4922592));
#153677=CARTESIAN_POINT('Ctrl Pts',(-0.334222997,1.071428571,7.492549298));
#153678=CARTESIAN_POINT('Ctrl Pts',(0.068465398,1.134501699,7.510512173));
#153679=CARTESIAN_POINT('Ctrl Pts',(0.470759401,1.198754474,7.485211125));
#153680=CARTESIAN_POINT('',(-0.460107700334207,1.06939091820706,7.35964002907317));
#153681=CARTESIAN_POINT('Ctrl Pts',(-1.14050351955613,4.81939092100001,
7.43209880004169));
#153682=CARTESIAN_POINT('Ctrl Pts',(-0.737770323522325,4.754503495,7.49390080806282));
#153683=CARTESIAN_POINT('Ctrl Pts',(-0.330717067503511,4.689276009,7.51182182120226));
#153684=CARTESIAN_POINT('Ctrl Pts',(-1.155216884,4.81939092100001,7.410497551));
#153685=CARTESIAN_POINT('Ctrl Pts',(-0.753654224,4.754503495,7.473096852));
#153686=CARTESIAN_POINT('Ctrl Pts',(-0.347678495,4.689276009,7.491936977));
#153687=CARTESIAN_POINT('Ctrl Pts',(-1.35103832,4.81939092100001,7.123004665));
#153688=CARTESIAN_POINT('Ctrl Pts',(-0.965054425,4.754503495,7.196215207));
#153689=CARTESIAN_POINT('Ctrl Pts',(-0.573419596,4.689276009,7.227287871));
#153690=CARTESIAN_POINT('',(-0.598342121129821,4.73201976879592,7.49397863771111));
#153691=CARTESIAN_POINT('Ctrl Pts',(-0.59831258994097,4.73200270359627,
7.49384481755901));
#153692=CARTESIAN_POINT('Ctrl Pts',(-0.59482195673254,4.72506033663315,
7.44720105427947));
#153693=CARTESIAN_POINT('Ctrl Pts',(-0.59130988361317,4.71792582707077,
7.40055371361005));
#153694=CARTESIAN_POINT('Ctrl Pts',(-0.584568150926036,4.70392125170665,
7.31160013884204));
#153695=CARTESIAN_POINT('Ctrl Pts',(-0.581337570868995,4.69707707070605,
7.26922871111862));
#153696=CARTESIAN_POINT('Ctrl Pts',(-0.578090315740495,4.69005394718278,
7.22691577275115));
#153697=CARTESIAN_POINT('',(-1.2089559129046,4.8193909197054,7.33160125315675));
#153698=CARTESIAN_POINT('Ctrl Pts',(-0.598394674877038,4.73205099219874,
7.49409641631189));
#153699=CARTESIAN_POINT('Ctrl Pts',(-0.701560839128794,4.74662633022798,
7.47123699178965));
#153700=CARTESIAN_POINT('Ctrl Pts',(-0.804232364139554,4.76121922702359,
7.44620705502926));
#153701=CARTESIAN_POINT('Ctrl Pts',(-1.00781309835978,4.79033919834542,
7.39200028864064));
#153702=CARTESIAN_POINT('Ctrl Pts',(-1.10870789696985,4.80486306066967,
7.36285585215043));
#153703=CARTESIAN_POINT('Ctrl Pts',(-1.20895590732316,4.81939092104741,
7.33160125063828));
#153704=CARTESIAN_POINT('',(-1.27957088547711,4.81939091791758,7.22792874414045));
#153705=CARTESIAN_POINT('Ctrl Pts',(-2.4530261316489,4.689268254,7.10774157717197));
#153706=CARTESIAN_POINT('Ctrl Pts',(-2.06279664085677,4.754934719,7.24241770931939));
#153707=CARTESIAN_POINT('Ctrl Pts',(-1.66016901775353,4.819390921,7.33356436923981));
#153708=CARTESIAN_POINT('Ctrl Pts',(-2.429904911,4.689268254,7.09546067));
#153709=CARTESIAN_POINT('Ctrl Pts',(-2.040349667,4.754934719,7.2288674));
#153710=CARTESIAN_POINT('Ctrl Pts',(-1.638531205,4.819390921,7.3188261));
#153711=CARTESIAN_POINT('Ctrl Pts',(-2.122702584,4.689268254,6.932289213));
#153712=CARTESIAN_POINT('Ctrl Pts',(-1.742105785,4.754934719,7.04882990900001));
#153713=CARTESIAN_POINT('Ctrl Pts',(-1.35103832,4.819390921,7.123004665));
#153714=CARTESIAN_POINT('',(-1.55963490183381,4.81939091971443,7.26508708152735));
#153715=CARTESIAN_POINT('',(-1.45491314490615,4.81939091820872,7.19375744735644));
#153716=CARTESIAN_POINT('',(-2.19533721229327,4.7320198238682,7.19014807039892));
#153717=CARTESIAN_POINT('Ctrl Pts',(-1.55963490663822,4.81939092085753,
7.26508707759447));
#153718=CARTESIAN_POINT('Ctrl Pts',(-1.66575655822878,4.80491309558304,
7.25711305448626));
#153719=CARTESIAN_POINT('Ctrl Pts',(-1.77169575683013,4.79041128761736,
7.24690770166126));
#153720=CARTESIAN_POINT('Ctrl Pts',(-1.9836880211467,4.76128647698349,7.22198419719515));
#153721=CARTESIAN_POINT('Ctrl Pts',(-2.08971531443295,4.74666639459473,
7.20724269142357));
#153722=CARTESIAN_POINT('Ctrl Pts',(-2.19539471642952,4.73203683304299,
7.19027205457454));
#153723=CARTESIAN_POINT('Ctrl Pts',(-2.1181481514051,4.6900539473732,6.93368216908028));
#153724=CARTESIAN_POINT('Ctrl Pts',(-2.13041551437734,4.69707706864944,
6.97430777773428));
#153725=CARTESIAN_POINT('Ctrl Pts',(-2.14267916587992,4.70392124758685,
7.0149940936479));
#153726=CARTESIAN_POINT('Ctrl Pts',(-2.1683857367939,4.71792585997149,7.10041893384059));
#153727=CARTESIAN_POINT('Ctrl Pts',(-2.18184357645508,4.72506040970981,
7.14522095253068));
#153728=CARTESIAN_POINT('Ctrl Pts',(-2.19527970815702,4.7320028146934,7.1900240862233));
#153729=CARTESIAN_POINT('Origin',(3.04010289164935E-13,4.93907429999964,
-7.64145691167784E-13));
#153730=CARTESIAN_POINT('',(-2.12995512140554,4.93794662027152,6.99495645510371));
#153731=CARTESIAN_POINT('Ctrl Pts',(-2.12995512205003,4.93794661929206,
6.99495645593132));
#153732=CARTESIAN_POINT('Ctrl Pts',(-2.03687773364896,4.91814186452076,
7.04400094768946));
#153733=CARTESIAN_POINT('Ctrl Pts',(-1.94277951412653,4.89834552796937,
7.09105849203187));
#153734=CARTESIAN_POINT('Ctrl Pts',(-1.80030894915214,4.86872423033274,
7.15854536088304));
#153735=CARTESIAN_POINT('Ctrl Pts',(-1.75268628190587,4.85888055797279,
7.1804867625023));
#153736=CARTESIAN_POINT('Ctrl Pts',(-1.65233933152185,4.83826147072025,
7.22542971669909));
#153737=CARTESIAN_POINT('Ctrl Pts',(-1.60370556157199,4.82833849617245,
7.24647476580251));
#153738=CARTESIAN_POINT('Ctrl Pts',(-1.55963490097094,4.81939092004434,
7.26508707964281));
#153739=CARTESIAN_POINT('',(-2.75676874468984,4.81939091962397,6.90030270497095));
#153740=CARTESIAN_POINT('Ctrl Pts',(-2.75676874432946,4.8193909198592,6.90030270293695));
#153741=CARTESIAN_POINT('Ctrl Pts',(-2.70856221741575,4.82837891575066,
6.90988314681471));
#153742=CARTESIAN_POINT('Ctrl Pts',(-2.65658740037599,4.83808521854872,
6.91969511781252));
#153743=CARTESIAN_POINT('Ctrl Pts',(-2.54838669927649,4.85839508142698,
6.9386041878068));
#153744=CARTESIAN_POINT('Ctrl Pts',(-2.49640727554015,4.86818863447598,
6.94706881560552));
#153745=CARTESIAN_POINT('Ctrl Pts',(-2.33982942837266,4.89780165988493,
6.97071017729041));
#153746=CARTESIAN_POINT('Ctrl Pts',(-2.23501398669613,4.91777478488708,
6.9840524371011));
#153747=CARTESIAN_POINT('Ctrl Pts',(-2.12995512148023,4.93794662119409,
6.99495645411656));
#153748=CARTESIAN_POINT('Ctrl Pts',(-2.19541375170991,4.7320509931869,7.19025143703924));
#153749=CARTESIAN_POINT('Ctrl Pts',(-2.29125384788963,4.74662633122123,
7.14574877728955));
#153750=CARTESIAN_POINT('Ctrl Pts',(-2.38614427324306,4.76121922802501,
7.09923268348006));
#153751=CARTESIAN_POINT('Ctrl Pts',(-2.57331254432414,4.79033919837692,
7.00252940413573));
#153752=CARTESIAN_POINT('Ctrl Pts',(-2.66558328619014,4.80486306068117,
6.95237694925337));
#153753=CARTESIAN_POINT('Ctrl Pts',(-2.75676873810498,4.81939092102955,
6.90030270416342));
#153754=CARTESIAN_POINT('Ctrl Pts',(-2.7115207327671,4.819390921,7.01316591404527));
#153755=CARTESIAN_POINT('Ctrl Pts',(-2.33148881985781,4.754503495,7.16009875803589));
#153756=CARTESIAN_POINT('Ctrl Pts',(-1.93780473105558,4.689276009,7.2651052049765));
#153757=CARTESIAN_POINT('Ctrl Pts',(-2.721246476,4.819390921,6.988906754));
#153758=CARTESIAN_POINT('Ctrl Pts',(-2.342529127,4.754503495,7.13636662));
#153759=CARTESIAN_POINT('Ctrl Pts',(-1.950094955,4.689276009,7.242039054));
#153760=CARTESIAN_POINT('Ctrl Pts',(-2.850687243,4.819390921,6.666039472));
#153761=CARTESIAN_POINT('Ctrl Pts',(-2.48946554,4.754503495,6.82051352));
#153762=CARTESIAN_POINT('Ctrl Pts',(-2.11366662,4.689276009,6.93504963400001));
#153763=CARTESIAN_POINT('',(-2.80344625281137,4.81939091791756,6.78387387063942));
#153764=CARTESIAN_POINT('Ctrl Pts',(-3.92363007934769,4.689268254,6.41423842243658));
#153765=CARTESIAN_POINT('Ctrl Pts',(-3.57147532391773,4.754934719,6.62965370569363));
#153766=CARTESIAN_POINT('Ctrl Pts',(-3.19785474998995,4.819390921,6.80522244558559));
#153767=CARTESIAN_POINT('Ctrl Pts',(-3.898409388,4.689268254,6.407215015));
#153768=CARTESIAN_POINT('Ctrl Pts',(-3.546640232,4.754934719,6.621245631));
#153769=CARTESIAN_POINT('Ctrl Pts',(-3.173554525,4.819390921,6.79548023900001));
#153770=CARTESIAN_POINT('Ctrl Pts',(-3.563312241,4.689268254,6.313897835));
#153771=CARTESIAN_POINT('Ctrl Pts',(-3.216666389,4.754934719,6.509530936));
#153772=CARTESIAN_POINT('Ctrl Pts',(-2.850687243,4.819390921,6.666039472));
#153773=CARTESIAN_POINT('',(-3.08495047229094,4.81939091970353,6.75995798154528));
#153774=CARTESIAN_POINT('',(-2.96734328929225,4.81939091820873,6.71280807683697));
#153775=CARTESIAN_POINT('',(-3.6896807437116,4.73201982384953,6.55011379745764));
#153776=CARTESIAN_POINT('Ctrl Pts',(-3.08495047608777,4.81939092086118,
6.75995797672338));
#153777=CARTESIAN_POINT('Ctrl Pts',(-3.18687688266884,4.80491309566292,
6.72935736384145));
#153778=CARTESIAN_POINT('Ctrl Pts',(-3.28814543198366,4.79041128777397,
6.69661681053702));
#153779=CARTESIAN_POINT('Ctrl Pts',(-3.48982361922147,4.76128647699335,
6.62670393305435));
#153780=CARTESIAN_POINT('Ctrl Pts',(-3.59020306534355,4.7466663945943,6.58951434159313));
#153781=CARTESIAN_POINT('Ctrl Pts',(-3.68976355640026,4.73203683302006,
6.55022252125281));
#153782=CARTESIAN_POINT('Ctrl Pts',(-3.55916373230487,4.69005394749471,
6.31623729329977));
#153783=CARTESIAN_POINT('Ctrl Pts',(-3.57987759641344,4.69707706879228,
6.35327597766147));
#153784=CARTESIAN_POINT('Ctrl Pts',(-3.60060088539638,4.70392124755126,
6.39037474666884));
#153785=CARTESIAN_POINT('Ctrl Pts',(-3.64407026673631,4.7179258599679,6.46827624894677));
#153786=CARTESIAN_POINT('Ctrl Pts',(-3.66684457924855,4.72506040969475,
6.50913778352832));
#153787=CARTESIAN_POINT('Ctrl Pts',(-3.68959793102294,4.732002814679,6.55000507366246));
#153788=CARTESIAN_POINT('Origin',(-3.79904441238921E-13,4.93907429999982,
6.90853624307763E-13));
#153789=CARTESIAN_POINT('',(-3.58386682213069,4.937946620308,6.3735408705598));
#153790=CARTESIAN_POINT('Ctrl Pts',(-3.58386682305503,4.93794661918659,
6.37354087132658));
#153791=CARTESIAN_POINT('Ctrl Pts',(-3.5035086482658,4.9181418644276,6.44144761724973));
#153792=CARTESIAN_POINT('Ctrl Pts',(-3.42172637389743,4.8983455278665,6.50763331800492));
#153793=CARTESIAN_POINT('Ctrl Pts',(-3.29709437357307,4.86872423024352,
6.60416934135374));
#153794=CARTESIAN_POINT('Ctrl Pts',(-3.25530185067192,4.85888055790257,
6.63583523087271));
#153795=CARTESIAN_POINT('Ctrl Pts',(-3.16696236313074,4.83826147072462,
6.70129907166331));
#153796=CARTESIAN_POINT('Ctrl Pts',(-3.1239896871397,4.82833849618614,6.73230692215565));
#153797=CARTESIAN_POINT('Ctrl Pts',(-3.08495047108381,4.81939092001171,
6.75995797994071));
#153798=CARTESIAN_POINT('',(-4.17567813333125,4.81939091958503,6.14635367162492));
#153799=CARTESIAN_POINT('Ctrl Pts',(-4.1756781326346,4.8193909197402,6.14635366996372));
#153800=CARTESIAN_POINT('Ctrl Pts',(-4.13065827124356,4.82837889487366,
6.16607305606045));
#153801=CARTESIAN_POINT('Ctrl Pts',(-4.08200792740075,4.83808518697421,
6.18682866311168));
#153802=CARTESIAN_POINT('Ctrl Pts',(-3.98040163242939,4.8583950812381,6.22855566656678));
#153803=CARTESIAN_POINT('Ctrl Pts',(-3.93145710281929,4.86818863440753,
6.24799643597097));
#153804=CARTESIAN_POINT('Ctrl Pts',(-3.7836221517757,4.89780165995966,6.30474468485385));
#153805=CARTESIAN_POINT('Ctrl Pts',(-3.68412542814874,4.91777478500429,
6.34030723174283));
#153806=CARTESIAN_POINT('Ctrl Pts',(-3.58386682196884,4.93794662138014,
6.3735408694208));
#153807=CARTESIAN_POINT('Ctrl Pts',(-3.68977771447632,4.73205099318326,
6.5501982937046));
#153808=CARTESIAN_POINT('Ctrl Pts',(-3.77381036623843,4.74662633125715,
6.48613329363275));
#153809=CARTESIAN_POINT('Ctrl Pts',(-3.85648272115148,4.76121922808381,
6.42030608363322));
#153810=CARTESIAN_POINT('Ctrl Pts',(-4.01848676156039,4.79033919950061,
6.2856280226034));
#153811=CARTESIAN_POINT('Ctrl Pts',(-4.09781896633792,4.80486306124649,
6.21681262465362));
#153812=CARTESIAN_POINT('Ctrl Pts',(-4.17567812688072,4.81939092105904,
6.14635367227836));
#153813=CARTESIAN_POINT('Ctrl Pts',(-4.15575024852906,4.819390921,6.26630518683826));
#153814=CARTESIAN_POINT('Ctrl Pts',(-3.81618948817902,4.754503495,6.49149844966127));
#153815=CARTESIAN_POINT('Ctrl Pts',(-3.45428279729009,4.689276009,6.67868034729526));
#153816=CARTESIAN_POINT('Ctrl Pts',(-4.160033607,4.819390921,6.240522445));
#153817=CARTESIAN_POINT('Ctrl Pts',(-3.821869971,4.754503495,6.465947816));
#153818=CARTESIAN_POINT('Ctrl Pts',(-3.461327142,4.689276009,6.65351143500001));
#153819=CARTESIAN_POINT('Ctrl Pts',(-4.217041199,4.819390921,5.897377682));
#153820=CARTESIAN_POINT('Ctrl Pts',(-3.897472013,4.754503495,6.125892201));
#153821=CARTESIAN_POINT('Ctrl Pts',(-3.555080941,4.689276009,6.31853618300001));
#153822=CARTESIAN_POINT('',(-4.19623558931448,4.8193909179172,6.02261259398131));
#153823=CARTESIAN_POINT('Ctrl Pts',(-5.21076944541101,4.689268254,5.42081260694443));
#153824=CARTESIAN_POINT('Ctrl Pts',(-4.91315579169461,4.754934719,5.70689446397799));
#153825=CARTESIAN_POINT('Ctrl Pts',(-4.5860123475086,4.819390921,5.95867588311505));
#153826=CARTESIAN_POINT('Ctrl Pts',(-5.184628575,4.689268254,5.419375106));
#153827=CARTESIAN_POINT('Ctrl Pts',(-4.88709384300001,4.754934719,5.704021776));
#153828=CARTESIAN_POINT('Ctrl Pts',(-4.56018596200001,4.819390921,5.954385274));
#153829=CARTESIAN_POINT('Ctrl Pts',(-4.837305378,4.689268254,5.400275611));
#153830=CARTESIAN_POINT('Ctrl Pts',(-4.540819247,4.754934719,5.66585353));
#153831=CARTESIAN_POINT('Ctrl Pts',(-4.217041199,4.819390921,5.897377682));
#153832=CARTESIAN_POINT('',(-4.4660171875858,4.81939091972219,5.93874075956449));
#153833=CARTESIAN_POINT('',(-4.34102375947002,4.81939091820872,5.91797526136406));
#153834=CARTESIAN_POINT('',(-5.01149890497033,4.73201982381453,5.60380348299995));
#153835=CARTESIAN_POINT('Ctrl Pts',(-4.46601719029875,4.81939092087189,
5.93874075396268));
#153836=CARTESIAN_POINT('Ctrl Pts',(-4.55898238578439,4.80491309584948,
5.8869444025433));
#153837=CARTESIAN_POINT('Ctrl Pts',(-4.6508450803644,4.7904112881491,5.83319956134153));
#153838=CARTESIAN_POINT('Ctrl Pts',(-4.83277894394465,4.76128647699006,
5.72156635797227));
#153839=CARTESIAN_POINT('Ctrl Pts',(-4.9228169116799,4.74666639456854,5.66366762468992));
#153840=CARTESIAN_POINT('Ctrl Pts',(-5.01160315398706,4.73203683297963,
5.60389186259176));
#153841=CARTESIAN_POINT('Ctrl Pts',(-4.83375677298044,4.69005394733486,
5.40345218008686));
#153842=CARTESIAN_POINT('Ctrl Pts',(-4.86194858047605,4.69707706858877,
5.43517205187568));
#153843=CARTESIAN_POINT('Ctrl Pts',(-4.89016250998706,4.70392124754382,
5.46694857865637));
#153844=CARTESIAN_POINT('Ctrl Pts',(-4.94936212146285,4.71792585991507,
5.53368415494247));
#153845=CARTESIAN_POINT('Ctrl Pts',(-4.98038800542991,4.72506040965708,
5.56869456572523));
#153846=CARTESIAN_POINT('Ctrl Pts',(-5.01139465595361,4.73200281464944,
5.60371510340813));
#153847=CARTESIAN_POINT('Origin',(-2.94902990916057E-13,4.93907429999893,
3.00107161343988E-13));
#153848=CARTESIAN_POINT('',(-4.8702008953712,4.93794662022304,5.45410559738563));
#153849=CARTESIAN_POINT('Ctrl Pts',(-4.87020089618387,4.93794661936938,
5.45410559780442));
#153850=CARTESIAN_POINT('Ctrl Pts',(-4.80631939369209,4.9181418645925,5.5376993542193));
#153851=CARTESIAN_POINT('Ctrl Pts',(-4.74067711244161,4.89834552799912,
5.61991844185732));
#153852=CARTESIAN_POINT('Ctrl Pts',(-4.63971133011318,4.86872423032248,
5.74098970296878));
#153853=CARTESIAN_POINT('Ctrl Pts',(-4.60570312327546,4.85888055796491,
5.78089941874312));
#153854=CARTESIAN_POINT('Ctrl Pts',(-4.53350175443041,4.83826147078614,
5.86382312992339));
#153855=CARTESIAN_POINT('Ctrl Pts',(-4.4981995269382,4.82833849624498,5.90334388922536));
#153856=CARTESIAN_POINT('Ctrl Pts',(-4.46601718601022,4.81939092005081,
5.93874075821506));
#153857=CARTESIAN_POINT('',(-5.39933745356238,4.81939091961611,5.10500797198601));
#153858=CARTESIAN_POINT('Ctrl Pts',(-5.39933745241095,4.81939091983647,
5.1050079703367));
#153859=CARTESIAN_POINT('Ctrl Pts',(-5.35960920618647,4.8283788969602,5.1339442744892));
#153860=CARTESIAN_POINT('Ctrl Pts',(-5.31655812254176,4.83808518899225,
5.16467301236654));
#153861=CARTESIAN_POINT('Ctrl Pts',(-5.22629740734351,4.85839508126596,
5.22726680555861));
#153862=CARTESIAN_POINT('Ctrl Pts',(-5.18267636485299,4.86818863432646,
5.25677468734867));
#153863=CARTESIAN_POINT('Ctrl Pts',(-5.05049690960121,4.89780165970237,
5.34397633774945));
#153864=CARTESIAN_POINT('Ctrl Pts',(-4.96097126074703,4.91777478468387,
5.40009630635383));
#153865=CARTESIAN_POINT('Ctrl Pts',(-4.8702008950791,4.9379466210003,5.45410559660442));
#153866=CARTESIAN_POINT('Ctrl Pts',(-5.01161177283213,4.7320509931675,5.60386515788382));
#153867=CARTESIAN_POINT('Ctrl Pts',(-5.07990770656187,4.74662633121997,
5.52323342585211));
#153868=CARTESIAN_POINT('Ctrl Pts',(-5.14649632337388,4.76121922804003,
5.44117310698807));
#153869=CARTESIAN_POINT('Ctrl Pts',(-5.27576099365539,4.7903391986696,5.27481766892534));
#153870=CARTESIAN_POINT('Ctrl Pts',(-5.33844518102469,4.80486306082872,
5.19055705554994));
#153871=CARTESIAN_POINT('Ctrl Pts',(-5.39933744725787,4.81939092103739,
5.10500797403888));
#153872=CARTESIAN_POINT('Ctrl Pts',(-5.40566150139869,4.819390921,5.22643899328157));
#153873=CARTESIAN_POINT('Ctrl Pts',(-5.12244937875261,4.754503495,5.51936288912698));
#153874=CARTESIAN_POINT('Ctrl Pts',(-4.80924243929241,4.689276009,5.77996781809004));
#153875=CARTESIAN_POINT('Ctrl Pts',(-5.40430219,4.819390921,5.200338242));
#153876=CARTESIAN_POINT('Ctrl Pts',(-5.122504424,4.754503495,5.493188479));
#153877=CARTESIAN_POINT('Ctrl Pts',(-4.810711519,4.689276009,5.75387301500001));
#153878=CARTESIAN_POINT('Ctrl Pts',(-5.386210996,4.819390921,4.852961066));
#153879=CARTESIAN_POINT('Ctrl Pts',(-5.123237026,4.754503495,5.144830971));
#153880=CARTESIAN_POINT('Ctrl Pts',(-4.830263629,4.689276009,5.406575004));
#153881=CARTESIAN_POINT('',(-5.39281361407602,4.8193909179172,4.97974064683932));
#153882=CARTESIAN_POINT('Ctrl Pts',(-6.25425902407638,4.689268254,4.17391561840196));
#153883=CARTESIAN_POINT('Ctrl Pts',(-6.02510255533609,4.754934719,4.51728717839333));
#153884=CARTESIAN_POINT('Ctrl Pts',(-5.75973310559946,4.819390921,4.83350825853756));
#153885=CARTESIAN_POINT('Ctrl Pts',(-6.22842029200001,4.689268254,4.17813124));
#153886=CARTESIAN_POINT('Ctrl Pts',(-5.999032377,4.754934719,4.520084201));
#153887=CARTESIAN_POINT('Ctrl Pts',(-5.733588172,4.819390921,4.83486987100001));
#153888=CARTESIAN_POINT('Ctrl Pts',(-5.885111492,4.689268254,4.234142502));
#153889=CARTESIAN_POINT('Ctrl Pts',(-5.652648444,4.754934719,4.557247111));
#153890=CARTESIAN_POINT('Ctrl Pts',(-5.38621099600001,4.819390921,4.852961066));
#153891=CARTESIAN_POINT('',(-5.63825790329601,4.81939091975338,4.83983461973514));
#153892=CARTESIAN_POINT('',(-5.51172278325784,4.81939091820872,4.84642449989799));
#153893=CARTESIAN_POINT('',(-6.09898494735702,4.73201982388842,4.39546554549127));
#153894=CARTESIAN_POINT('Ctrl Pts',(-5.63825790479694,4.81939092085883,
4.83983461349765));
#153895=CARTESIAN_POINT('Ctrl Pts',(-5.71791494255591,4.80491309559872,
4.76926446177373));
#153896=CARTESIAN_POINT('Ctrl Pts',(-5.79607638747738,4.79041128765872,
4.69702837984562));
#153897=CARTESIAN_POINT('Ctrl Pts',(-5.94975889685249,4.76128647703165,
4.54889469853867));
#153898=CARTESIAN_POINT('Ctrl Pts',(-6.02524531066462,4.74666639463682,
4.47299410396976));
#153899=CARTESIAN_POINT('Ctrl Pts',(-6.0991057579877,4.73203683307021,4.39552944845035));
#153900=CARTESIAN_POINT('Ctrl Pts',(-5.88232872025789,4.69005394749199,
4.23800765046643));
#153901=CARTESIAN_POINT('Ctrl Pts',(-5.91668025408089,4.6970770688052,4.26292552406789));
#153902=CARTESIAN_POINT('Ctrl Pts',(-5.9510655707326,4.70392124759191,4.28789397167456));
#153903=CARTESIAN_POINT('Ctrl Pts',(-6.02322730468982,4.71792586000582,
4.34034314051077));
#153904=CARTESIAN_POINT('Ctrl Pts',(-6.06105402409859,4.72506040973061,
4.36786537913626));
#153905=CARTESIAN_POINT('Ctrl Pts',(-6.09886413672633,4.73200281470664,
4.39540164253219));
#153906=CARTESIAN_POINT('Origin',(9.65807295250087E-13,4.93907430000018,
-7.16874476447416E-13));
#153907=CARTESIAN_POINT('',(-5.92880978559005,4.93794662022799,4.27964240970281));
#153908=CARTESIAN_POINT('Ctrl Pts',(-5.92880978656371,4.93794661928743,
4.27964240996096));
#153909=CARTESIAN_POINT('Ctrl Pts',(-5.88439198483936,4.91814186452631,
4.37501442529949));
#153910=CARTESIAN_POINT('Ctrl Pts',(-5.83795905720867,4.89834552796916,
4.46942242625393));
#153911=CARTESIAN_POINT('Ctrl Pts',(-5.76538054119186,4.86872423034047,
4.60936776698835));
#153912=CARTESIAN_POINT('Ctrl Pts',(-5.74074683651474,4.85888055798814,
4.65565517495367));
#153913=CARTESIAN_POINT('Ctrl Pts',(-5.68805964221968,4.83826147079414,
4.75216133594935));
#153914=CARTESIAN_POINT('Ctrl Pts',(-5.66207855629228,4.82833849628135,
4.79834705710259));
#153915=CARTESIAN_POINT('Ctrl Pts',(-5.63825790129655,4.81939092014492,
4.83983461867157));
#153916=CARTESIAN_POINT('',(-6.3705297556276,4.81939091962137,3.8249577731703));
#153917=CARTESIAN_POINT('Ctrl Pts',(-6.37052975403151,4.8193909198275,3.82495777170694));
#153918=CARTESIAN_POINT('Ctrl Pts',(-6.33795068445817,4.82837892242052,
3.86175807299039));
#153919=CARTESIAN_POINT('Ctrl Pts',(-6.30251183084649,4.83808522931985,
3.9010231472222));
#153920=CARTESIAN_POINT('Ctrl Pts',(-6.22781732456498,4.85839508129715,
3.98155675809144));
#153921=CARTESIAN_POINT('Ctrl Pts',(-6.19155944002768,4.86818863439397,
4.01975199682512));
#153922=CARTESIAN_POINT('Ctrl Pts',(-6.08121604392898,4.89780165982673,
4.13332959701782));
#153923=CARTESIAN_POINT('Ctrl Pts',(-6.00584758923612,4.91777478480989,
4.20738288023703));
#153924=CARTESIAN_POINT('Ctrl Pts',(-5.92880978508571,4.93794662109296,
4.27964240892365));
#153925=CARTESIAN_POINT('Ctrl Pts',(-6.09910843466592,4.73205099318423,
4.3955015153301));
#153926=CARTESIAN_POINT('Ctrl Pts',(-6.14847420848262,4.74662633121565,
4.30207330148139));
#153927=CARTESIAN_POINT('Ctrl Pts',(-6.19586547756303,4.76121922801461,
4.20761692303707));
#153928=CARTESIAN_POINT('Ctrl Pts',(-6.28634650922938,4.79033919837924,
4.01736270113525));
#153929=CARTESIAN_POINT('Ctrl Pts',(-6.32945163452773,4.80486306068784,
3.92159680566657));
#153930=CARTESIAN_POINT('Ctrl Pts',(-6.37052975011586,4.81939092102897,
3.82495777589447));
#153931=CARTESIAN_POINT('Ctrl Pts',(-6.40281003136325,4.819390921,3.94219032100099));
#153932=CARTESIAN_POINT('Ctrl Pts',(-6.18918922906761,4.754503495,4.28914805360017));
#153933=CARTESIAN_POINT('Ctrl Pts',(-5.93932724980595,4.689276009,4.61099041838498));
#153934=CARTESIAN_POINT('Ctrl Pts',(-6.39587161000001,4.819390921,3.916992003));
#153935=CARTESIAN_POINT('Ctrl Pts',(-6.18361626300001,4.754503495,4.263573754));
#153936=CARTESIAN_POINT('Ctrl Pts',(-5.935152372,4.689276009,4.585189889));
#153937=CARTESIAN_POINT('Ctrl Pts',(-6.303527553,4.819390921,3.581625384));
#153938=CARTESIAN_POINT('Ctrl Pts',(-6.10944517000001,4.754503495,3.923203163));
#153939=CARTESIAN_POINT('Ctrl Pts',(-5.87958855800001,4.689276009,4.241808386));
#153940=CARTESIAN_POINT('',(-6.3372296677262,4.8193909179172,3.70402156085939));
#153941=CARTESIAN_POINT('Ctrl Pts',(-7.00530640168829,4.689268254,2.7318509758169));
#153942=CARTESIAN_POINT('Ctrl Pts',(-6.85532221866109,4.754934719,3.11645656668847));
#153943=CARTESIAN_POINT('Ctrl Pts',(-6.6641351438977,4.819390921,3.48233116048104));
#153944=CARTESIAN_POINT('Ctrl Pts',(-6.980977999,4.689268254,2.741522602));
#153945=CARTESIAN_POINT('Ctrl Pts',(-6.830462824,4.754934719,3.124792514));
#153946=CARTESIAN_POINT('Ctrl Pts',(-6.638894171,4.819390921,3.489281327));
#153947=CARTESIAN_POINT('Ctrl Pts',(-6.657736333,4.689268254,2.870025595));
#153948=CARTESIAN_POINT('Ctrl Pts',(-6.500166082,4.754934719,3.235548881));
#153949=CARTESIAN_POINT('Ctrl Pts',(-6.303527553,4.819390921,3.581625384));
#153950=CARTESIAN_POINT('',(-6.54685994546402,4.81939091973621,3.51462319233795));
#153951=CARTESIAN_POINT('',(-6.4246997757989,4.81939091820872,3.54826031502617));
#153952=CARTESIAN_POINT('',(-6.90128923179587,4.73201982380202,2.98160052488795));
#153953=CARTESIAN_POINT('Ctrl Pts',(-6.54685994559511,4.81939092086963,
3.51462318600688));
#153954=CARTESIAN_POINT('Ctrl Pts',(-6.60948414861081,4.80491309580405,
3.42857901797942));
#153955=CARTESIAN_POINT('Ctrl Pts',(-6.67028959924742,4.79041128806021,
3.34122937663874));
#153956=CARTESIAN_POINT('Ctrl Pts',(-6.78853473591051,4.76128647699977,
3.16352177942524));
#153957=CARTESIAN_POINT('Ctrl Pts',(-6.84593993515113,4.74666639457268,
3.07316835092304));
#153958=CARTESIAN_POINT('Ctrl Pts',(-6.90142095522026,4.73203683297701,
2.98163696307265));
#153959=CARTESIAN_POINT('Ctrl Pts',(-6.65584951415727,4.69005394750498,
2.8743985919351));
#153960=CARTESIAN_POINT('Ctrl Pts',(-6.69475453450432,4.69707706882282,
2.89134933526787));
#153961=CARTESIAN_POINT('Ctrl Pts',(-6.73370341955243,4.70392124757204,
2.90834220782314));
#153962=CARTESIAN_POINT('Ctrl Pts',(-6.8154530731439,4.71792585996462,2.94405250474992));
#153963=CARTESIAN_POINT('Ctrl Pts',(-6.85831189257049,4.72506040967098,
2.96279966231256));
#153964=CARTESIAN_POINT('Ctrl Pts',(-6.90115750837148,4.73200281462704,
2.98156408670324));
#153965=CARTESIAN_POINT('Origin',(8.59555482346508E-13,4.93907430000018,
-3.81856005149395E-13));
#153966=CARTESIAN_POINT('',(-6.71019411999318,4.93794662023874,2.90506789946243));
#153967=CARTESIAN_POINT('Ctrl Pts',(-6.71019412117,4.93794661913889,2.90506789951248));
#153968=CARTESIAN_POINT('Ctrl Pts',(-6.68731694705018,4.91814186443027,
3.00775868445496));
#153969=CARTESIAN_POINT('Ctrl Pts',(-6.6622645250126,4.89834552787458,3.10994118563057));
#153970=CARTESIAN_POINT('Ctrl Pts',(-6.6214669659314,4.86872423024708,3.26221691745863));
#153971=CARTESIAN_POINT('Ctrl Pts',(-6.60735960808125,4.85888055790125,
3.31271766979899));
#153972=CARTESIAN_POINT('Ctrl Pts',(-6.57665018314621,4.83826147076628,
3.41829375935451));
#153973=CARTESIAN_POINT('Ctrl Pts',(-6.56120508540271,4.8283384962618,3.46898484943721));
#153974=CARTESIAN_POINT('Ctrl Pts',(-6.54685994339077,4.81939092009245,
3.51462319175612));
#153975=CARTESIAN_POINT('',(-7.04384316624177,4.81939091957173,2.36605679960635));
#153976=CARTESIAN_POINT('Ctrl Pts',(-7.04384316473025,4.81939091970471,
2.36605679873706));
#153977=CARTESIAN_POINT('Ctrl Pts',(-7.01993684385504,4.82837888959944,
2.40900009757574));
#153978=CARTESIAN_POINT('Ctrl Pts',(-6.99376741163948,4.83808517752402,
2.45496540987332));
#153979=CARTESIAN_POINT('Ctrl Pts',(-6.93813142560118,4.85839508118821,
2.54967354160683));
#153980=CARTESIAN_POINT('Ctrl Pts',(-6.91093207744687,4.86818863432016,
2.59477017043889));
#153981=CARTESIAN_POINT('Ctrl Pts',(-6.82758427512232,4.89780165984243,
2.72941295820832));
#153982=CARTESIAN_POINT('Ctrl Pts',(-6.76989715978556,4.91777478488697,
2.817936906831));
#153983=CARTESIAN_POINT('Ctrl Pts',(-6.71019411921342,4.93794662126058,
2.90506789869156));
#153984=CARTESIAN_POINT('Ctrl Pts',(-6.90141756449681,4.73205099312077,
2.98160910759462));
#153985=CARTESIAN_POINT('Ctrl Pts',(-6.9295448897165,4.74662633118373,2.87975301121524));
#153986=CARTESIAN_POINT('Ctrl Pts',(-6.95552284802293,4.76121922801361,
2.77731724830936));
#153987=CARTESIAN_POINT('Ctrl Pts',(-7.00298945097549,4.79033919925393,
2.57206031116946));
#153988=CARTESIAN_POINT('Ctrl Pts',(-7.02449996483583,4.80486306112818,
2.46926704446389));
#153989=CARTESIAN_POINT('Ctrl Pts',(-7.04384316156922,4.81939092105299,
2.36605680391327));
#153990=CARTESIAN_POINT('Ctrl Pts',(-7.10057027935825,4.819390921,2.47360921065799));
#153991=CARTESIAN_POINT('Ctrl Pts',(-6.96652946959742,4.754503495,2.85837742253879));
#153992=CARTESIAN_POINT('Ctrl Pts',(-6.79169571959383,4.689276009,3.22640823087936));
#153993=CARTESIAN_POINT('Ctrl Pts',(-7.088377181,4.819390921,2.450491571));
#153994=CARTESIAN_POINT('Ctrl Pts',(-6.955589078,4.754503495,2.834599059));
#153995=CARTESIAN_POINT('Ctrl Pts',(-6.78207209700001,4.689276009,3.202108379));
#153996=CARTESIAN_POINT('Ctrl Pts',(-6.926098167,4.819390921,2.14281688));
#153997=CARTESIAN_POINT('Ctrl Pts',(-6.809982448,4.754503495,2.518130736));
#153998=CARTESIAN_POINT('Ctrl Pts',(-6.653990461,4.689276009,2.878699522));
#153999=CARTESIAN_POINT('',(-6.98532390492156,4.8193909179172,2.25510654365763));
#154000=CARTESIAN_POINT('Ctrl Pts',(-7.42879343763473,4.689268254,1.16204801642745));
#154001=CARTESIAN_POINT('Ctrl Pts',(-7.36499463477628,4.754934719,1.56990390823356));
#154002=CARTESIAN_POINT('Ctrl Pts',(-7.25692963095346,4.819390921,1.96832412729405));
#154003=CARTESIAN_POINT('Ctrl Pts',(-7.407112933,4.689268254,1.176723413));
#154004=CARTESIAN_POINT('Ctrl Pts',(-7.342508421,4.754934719,1.583389001));
#154005=CARTESIAN_POINT('Ctrl Pts',(-7.233772858,4.819390921,1.980537866));
#154006=CARTESIAN_POINT('Ctrl Pts',(-7.119052823,4.689268254,1.371709481));
#154007=CARTESIAN_POINT('Ctrl Pts',(-7.043743179,4.754934719,1.762559983));
#154008=CARTESIAN_POINT('Ctrl Pts',(-6.926098167,4.819390921,2.14281688));
#154009=CARTESIAN_POINT('',(-7.14933809287314,4.81939091974536,2.02507189097459));
#154010=CARTESIAN_POINT('',(-7.03726494732171,4.81939091820872,2.08418342172407));
#154011=CARTESIAN_POINT('',(-7.38089690198285,4.73201982388821,1.42831917721988));
#154012=CARTESIAN_POINT('Ctrl Pts',(-7.14933809165179,4.81939092087443,
2.02507188465993));
#154013=CARTESIAN_POINT('Ctrl Pts',(-7.19200122269096,4.80491309589017,
1.9275770295049));
#154014=CARTESIAN_POINT('Ctrl Pts',(-7.2326074846078,4.79041128825026,1.82919820034297));
#154015=CARTESIAN_POINT('Ctrl Pts',(-7.30988623568892,4.76128647706763,
1.63022609776993));
#154016=CARTESIAN_POINT('Ctrl Pts',(-7.34652601697845,4.74666639465519,
1.52964466117206));
#154017=CARTESIAN_POINT('Ctrl Pts',(-7.3810333788971,4.73203683306954,1.42832644690564));
#154018=CARTESIAN_POINT('Ctrl Pts',(-7.11815018181255,4.69005394745638,
1.37638584987177));
#154019=CARTESIAN_POINT('Ctrl Pts',(-7.15978953282356,4.69707706872065,
1.38457686486532));
#154020=CARTESIAN_POINT('Ctrl Pts',(-7.2014807805252,4.70392124759223,1.39279959468546));
#154021=CARTESIAN_POINT('Ctrl Pts',(-7.28899583059621,4.71792585998154,
1.41010124566418));
#154022=CARTESIAN_POINT('Ctrl Pts',(-7.33488271934859,4.72506040971655,
1.41919672582886));
#154023=CARTESIAN_POINT('Ctrl Pts',(-7.38076042506859,4.73200281470688,
1.42831190753412));
#154024=CARTESIAN_POINT('Origin',(-2.94902990916057E-14,4.93907430000053,
-4.98732999343332E-14));
#154025=CARTESIAN_POINT('',(-7.17781723584371,4.93794662022731,1.39465564117819));
#154026=CARTESIAN_POINT('Ctrl Pts',(-7.17781723670216,4.93794661941343,
1.39465564102716));
#154027=CARTESIAN_POINT('Ctrl Pts',(-7.17755040150417,4.91814186461323,
1.49986348894002));
#154028=CARTESIAN_POINT('Ctrl Pts',(-7.17504990843411,4.89834552801126,
1.60504255047927));
#154029=CARTESIAN_POINT('Ctrl Pts',(-7.16794095468464,4.86872423033395,
1.76252842994329));
#154030=CARTESIAN_POINT('Ctrl Pts',(-7.16501958796713,4.85888055797704,
1.81488116780166));
#154031=CARTESIAN_POINT('Ctrl Pts',(-7.157723870727,4.83826147080119,1.9245905659777));
#154032=CARTESIAN_POINT('Ctrl Pts',(-7.15353695671268,4.8283384962796,1.9774167661419));
#154033=CARTESIAN_POINT('Ctrl Pts',(-7.14933809068473,4.81939092011745,
2.02507189085163));
#154034=CARTESIAN_POINT('',(-7.38779429945998,4.81939091967051,0.796521640787532));
#154035=CARTESIAN_POINT('Ctrl Pts',(-7.38779429716093,4.8193909199705,0.796521640040918));
#154036=CARTESIAN_POINT('Ctrl Pts',(-7.37367837789995,4.82837892375171,
0.843600292298873));
#154037=CARTESIAN_POINT('Ctrl Pts',(-7.35800192287268,4.83808523015355,
0.894116694457562));
#154038=CARTESIAN_POINT('Ctrl Pts',(-7.3240262118831,4.85839508130368,0.998570424941728));
#154039=CARTESIAN_POINT('Ctrl Pts',(-7.30715721170585,4.86818863432921,
1.04845977495898));
#154040=CARTESIAN_POINT('Ctrl Pts',(-7.2547022543451,4.89780165967758,1.19787200213601));
#154041=CARTESIAN_POINT('Ctrl Pts',(-7.21739386403372,4.91777478464996,
1.29672733440014));
#154042=CARTESIAN_POINT('Ctrl Pts',(-7.17781723517334,4.93794662096607,
1.3946556407551));
#154043=CARTESIAN_POINT('Ctrl Pts',(-7.38102407937051,4.73205099318476,
1.42829997158409));
#154044=CARTESIAN_POINT('Ctrl Pts',(-7.38659775345975,4.74662633124308,
1.32277867077803));
#154045=CARTESIAN_POINT('Ctrl Pts',(-7.38994770048621,4.76121922805999,
1.21715330607263));
#154046=CARTESIAN_POINT('Ctrl Pts',(-7.39218038646568,4.79033919864747,
1.00649125024579));
#154047=CARTESIAN_POINT('Ctrl Pts',(-7.39109048280139,4.80486306081453,
0.901477106205701));
#154048=CARTESIAN_POINT('Ctrl Pts',(-7.38779429544083,4.81939092103713,
0.796521646044604));
#154049=CARTESIAN_POINT('Ctrl Pts',(-7.46631575272062,4.819390921,0.88936488343584));
#154050=CARTESIAN_POINT('Ctrl Pts',(-7.41812253464388,4.754503495,1.2939522410014));
#154051=CARTESIAN_POINT('Ctrl Pts',(-7.32649204551892,4.689276009,1.69096278051253));
#154052=CARTESIAN_POINT('Ctrl Pts',(-7.44943811300001,4.819390921,0.869408877));
#154053=CARTESIAN_POINT('Ctrl Pts',(-7.40232627800001,4.754503495,1.273081663));
#154054=CARTESIAN_POINT('Ctrl Pts',(-7.311869668,4.689276009,1.66929984));
#154055=CARTESIAN_POINT('Ctrl Pts',(-7.224812129,4.819390921,0.603812641));
#154056=CARTESIAN_POINT('Ctrl Pts',(-7.192092516,4.754503495,0.995313314));
#154057=CARTESIAN_POINT('Ctrl Pts',(-7.117259166,4.689276009,1.380985869));
#154058=CARTESIAN_POINT('',(-7.30679216083989,4.81939091791748,0.700745251315236));
#154059=CARTESIAN_POINT('Ctrl Pts',(-7.5049183491183,4.689268254,-0.462091015612824));
#154060=CARTESIAN_POINT('Ctrl Pts',(-7.53028808736866,4.754934719,-0.0500557111030223));
#154061=CARTESIAN_POINT('Ctrl Pts',(-7.51039815272873,4.819390921,0.362280445934188));
#154062=CARTESIAN_POINT('Ctrl Pts',(-7.48689949900001,4.689268254,-0.443098054));
#154063=CARTESIAN_POINT('Ctrl Pts',(-7.511226485,4.754934719,-0.032052021));
#154064=CARTESIAN_POINT('Ctrl Pts',(-7.49040836500001,4.819390921,0.379186656));
#154065=CARTESIAN_POINT('Ctrl Pts',(-7.247490315,4.689268254,-0.190746244));
#154066=CARTESIAN_POINT('Ctrl Pts',(-7.257962673,4.754934719,0.207155738));
#154067=CARTESIAN_POINT('Ctrl Pts',(-7.224812129,4.819390921,0.603812641));
#154068=CARTESIAN_POINT('',(-7.41752113704197,4.81939091971279,0.440830478443873));
#154069=CARTESIAN_POINT('',(-7.32077543098668,4.81939091820872,0.522652428364941));
#154070=CARTESIAN_POINT('',(-7.51538203638646,4.73201982383859,-0.191748787497206));
#154071=CARTESIAN_POINT('Ctrl Pts',(-7.41752113453922,4.81939092085595,
0.440830472769329));
#154072=CARTESIAN_POINT('Ctrl Pts',(-7.43822831383812,4.80491309553719,
0.336443678595771));
#154073=CARTESIAN_POINT('Ctrl Pts',(-7.45673668403369,4.79041128752491,
0.231635743075057));
#154074=CARTESIAN_POINT('Ctrl Pts',(-7.48943557967304,4.76128647694917,
0.0207028550013527));
#154075=CARTESIAN_POINT('Ctrl Pts',(-7.50359670749935,4.74666639456738,
-0.0854035131269754));
#154076=CARTESIAN_POINT('Ctrl Pts',(-7.51551688532758,4.73203683301208,
-0.191771026338893));
#154077=CARTESIAN_POINT('Ctrl Pts',(-7.24761405796477,4.69005394746672,
-0.185985164613402));
#154078=CARTESIAN_POINT('Ctrl Pts',(-7.2900407301435,4.69707706869655,-0.186936880614835));
#154079=CARTESIAN_POINT('Ctrl Pts',(-7.33252490370272,4.70392124758181,
-0.187868779482321));
#154080=CARTESIAN_POINT('Ctrl Pts',(-7.4217132440767,4.71792585994043,-0.189784780218647));
#154081=CARTESIAN_POINT('Ctrl Pts',(-7.46848258230995,4.72506040967391,
-0.190766271932785));
#154082=CARTESIAN_POINT('Ctrl Pts',(-7.51524718744534,4.7320028146651,-0.19172654865552));
#154083=CARTESIAN_POINT('Origin',(5.52075746229619E-13,4.93907429999911,
4.82198916212928E-14));
#154084=CARTESIAN_POINT('',(-7.30981359479562,4.93794662022752,-0.180969163073113));
#154085=CARTESIAN_POINT('Ctrl Pts',(-7.30981359571788,4.93794661929613,
-0.180969163453093));
#154086=CARTESIAN_POINT('Ctrl Pts',(-7.33216957627644,4.91814186456599,
-0.0781636550505026));
#154087=CARTESIAN_POINT('Ctrl Pts',(-7.35233793245503,4.8983455280094,0.025093910417717));
#154088=CARTESIAN_POINT('Ctrl Pts',(-7.37924999091234,4.86872423035244,
0.180426072259296));
#154089=CARTESIAN_POINT('Ctrl Pts',(-7.38765121524058,4.85888055798396,
0.232182839687074));
#154090=CARTESIAN_POINT('Ctrl Pts',(-7.40411034549692,4.83826147074226,
0.340895656795059));
#154091=CARTESIAN_POINT('Ctrl Pts',(-7.41137739073122,4.82833849619623,
0.393386872495712));
#154092=CARTESIAN_POINT('Ctrl Pts',(-7.4175211349983,4.81939092004165,0.440830478770539));
#154093=CARTESIAN_POINT('',(-7.38630038196097,4.81939091969751,-0.810257984855973));
#154094=CARTESIAN_POINT('Ctrl Pts',(-7.38630037963555,4.81939091994588,
-0.810257985075426));
#154095=CARTESIAN_POINT('Ctrl Pts',(-7.38263500614926,4.82837891042957,
-0.761245578091695));
#154096=CARTESIAN_POINT('Ctrl Pts',(-7.37818459619328,4.83808521117728,
-0.708540272239645));
#154097=CARTESIAN_POINT('Ctrl Pts',(-7.3674576729076,4.85839508126324,-0.599224736206719));
#154098=CARTESIAN_POINT('Ctrl Pts',(-7.36170779607613,4.8681886343682,-0.546875434589808));
#154099=CARTESIAN_POINT('Ctrl Pts',(-7.34259841866334,4.89780165980116,
-0.389680116429263));
#154100=CARTESIAN_POINT('Ctrl Pts',(-7.32741325205991,4.91777478478915,
-0.285115765756162));
#154101=CARTESIAN_POINT('Ctrl Pts',(-7.30981359392888,4.93794662108625,
-0.180969163385907));
#154102=CARTESIAN_POINT('Ctrl Pts',(-7.51550211177187,4.73205099316266,
-0.19179488355814));
#154103=CARTESIAN_POINT('Ctrl Pts',(-7.49826151596717,4.74662633122546,
-0.296047330203138));
#154104=CARTESIAN_POINT('Ctrl Pts',(-7.47882681194459,4.76121922804102,
-0.399923372205497));
#154105=CARTESIAN_POINT('Ctrl Pts',(-7.43572118392055,4.7903391987379,-0.606140228564144));
#154106=CARTESIAN_POINT('Ctrl Pts',(-7.41208182486807,4.80486306086146,
-0.708464902909228));
#154107=CARTESIAN_POINT('Ctrl Pts',(-7.38630037914515,4.81939092103882,
-0.810257979522875));
#154108=CARTESIAN_POINT('Ctrl Pts',(-7.48294460067957,4.819390921,-0.736465157357116));
#154109=CARTESIAN_POINT('Ctrl Pts',(-7.52285243445693,4.754503495,-0.330976710562069));
#154110=CARTESIAN_POINT('Ctrl Pts',(-7.51870974654472,4.689276009,0.0764497902556042));
#154111=CARTESIAN_POINT('Ctrl Pts',(-7.462171599,4.819390921,-0.75232641));
#154112=CARTESIAN_POINT('Ctrl Pts',(-7.502938928,4.754503495,-0.347963618));
#154113=CARTESIAN_POINT('Ctrl Pts',(-7.49977234,4.689276009,0.058436696));
#154114=CARTESIAN_POINT('Ctrl Pts',(-7.185701905,4.819390921,-0.963425207));
#154115=CARTESIAN_POINT('Ctrl Pts',(-7.237908331,4.754503495,-0.574043853));
#154116=CARTESIAN_POINT('Ctrl Pts',(-7.247732742,4.689276009,-0.181301149));
#154117=CARTESIAN_POINT('',(-7.28559392484569,4.81939091791749,-0.887152541784059));
#154118=CARTESIAN_POINT('Ctrl Pts',(-7.23012161980515,4.689268254,-2.0646231853681));
#154119=CARTESIAN_POINT('Ctrl Pts',(-7.34347363819581,4.754934719,-1.66767478139762));
#154120=CARTESIAN_POINT('Ctrl Pts',(-7.41268880490121,4.819390921,-1.26070306624057));
#154121=CARTESIAN_POINT('Ctrl Pts',(-7.21660696600001,4.689268254,-2.042200749));
#154122=CARTESIAN_POINT('Ctrl Pts',(-7.328727947,4.754934719,-1.645994327));
#154123=CARTESIAN_POINT('Ctrl Pts',(-7.396800703,4.819390921,-1.239894901));
#154124=CARTESIAN_POINT('Ctrl Pts',(-7.037043215,4.689268254,-1.744282886));
#154125=CARTESIAN_POINT('Ctrl Pts',(-7.13280789900001,4.754934719,-1.357934879));
#154126=CARTESIAN_POINT('Ctrl Pts',(-7.18570190500001,4.819390921,-0.963425207));
#154127=CARTESIAN_POINT('',(-7.3388691369478,4.81939091972585,-1.16402367686312));
#154128=CARTESIAN_POINT('',(-7.26197459231862,4.81939091820873,-1.06331721224712));
#154129=CARTESIAN_POINT('',(-7.29845625953015,4.73201982380467,-1.80285079211797));
#154130=CARTESIAN_POINT('Ctrl Pts',(-7.33886913323993,4.81939092085855,
-1.16402368197451));
#154131=CARTESIAN_POINT('Ctrl Pts',(-7.33665211510866,4.80491309559566,
-1.27042140196416));
#154132=CARTESIAN_POINT('Ctrl Pts',(-7.33219716189816,4.79041128764499,
-1.37675773825831));
#154133=CARTESIAN_POINT('Ctrl Pts',(-7.31878723969319,4.7612864769747,-1.58978842933262));
#154134=CARTESIAN_POINT('Ctrl Pts',(-7.30980755554305,4.74666639456651,
-1.69645831361357));
#154135=CARTESIAN_POINT('Ctrl Pts',(-7.29858317508326,4.73203683298043,
-1.80290149954302));
#154136=CARTESIAN_POINT('Ctrl Pts',(-7.03818755575372,4.69005394737967,
-1.73965971898629));
#154137=CARTESIAN_POINT('Ctrl Pts',(-7.07941772512982,4.69707706861374,
-1.74970966487086));
#154138=CARTESIAN_POINT('Ctrl Pts',(-7.12070831179316,4.70392124752775,
-1.75975261806698));
#154139=CARTESIAN_POINT('Ctrl Pts',(-7.20739959490221,4.71792585989463,
-1.78079668068838));
#154140=CARTESIAN_POINT('Ctrl Pts',(-7.25286450035518,4.72506040963286,
-1.79180925094483));
#154141=CARTESIAN_POINT('Ctrl Pts',(-7.29832934397703,4.7320028146289,-1.80280008469291));
#154142=CARTESIAN_POINT('Origin',(-8.8037216405823E-13,4.93907430000053,
-2.65304271607203E-13));
#154143=CARTESIAN_POINT('',(-7.10001119460225,4.93794662021071,-1.74813205033564));
#154144=CARTESIAN_POINT('Ctrl Pts',(-7.10001119554104,4.93794661914312,
-1.74813205098826));
#154145=CARTESIAN_POINT('Ctrl Pts',(-7.14394465112064,4.91814186436947,
-1.65253595326797));
#154146=CARTESIAN_POINT('Ctrl Pts',(-7.18583880662247,4.89834552781747,
-1.55602809274632));
#154147=CARTESIAN_POINT('Ctrl Pts',(-7.24551349920576,4.86872423023617,
-1.41011280770722));
#154148=CARTESIAN_POINT('Ctrl Pts',(-7.26484448257846,4.85888055791847,
-1.36137209975618));
#154149=CARTESIAN_POINT('Ctrl Pts',(-7.30428884953336,4.8382614707778,-1.2587391545377));
#154150=CARTESIAN_POINT('Ctrl Pts',(-7.32267005503197,4.82833849625316,
-1.20903735410299));
#154151=CARTESIAN_POINT('Ctrl Pts',(-7.33886913496549,4.81939092007772,
-1.16402367607981));
#154152=CARTESIAN_POINT('',(-7.03943126753197,4.81939091962378,-2.37915084878438));
#154153=CARTESIAN_POINT('Ctrl Pts',(-7.03943126550706,4.81939091985741,
-2.37915084853802));
#154154=CARTESIAN_POINT('Ctrl Pts',(-7.04638780382853,4.82837890877908,
-2.33049638615935));
#154155=CARTESIAN_POINT('Ctrl Pts',(-7.05337152460824,4.83808520858237,
-2.27806659884981));
#154156=CARTESIAN_POINT('Ctrl Pts',(-7.06639500140624,4.85839508132424,
-2.16900081368179));
#154157=CARTESIAN_POINT('Ctrl Pts',(-7.07203310589037,4.86818863440908,
-2.1166393562294));
#154158=CARTESIAN_POINT('Ctrl Pts',(-7.08716284183417,4.89780165986177,
-1.95901122594177));
#154159=CARTESIAN_POINT('Ctrl Pts',(-7.09481094048261,4.91777478488203,
-1.85362716958633));
#154160=CARTESIAN_POINT('Ctrl Pts',(-7.10001119355224,4.93794662119754,
-1.74813205047258));
#154161=CARTESIAN_POINT('Ctrl Pts',(-7.29856361833912,4.73205099311978,
-1.80292162311842));
#154162=CARTESIAN_POINT('Ctrl Pts',(-7.25931490371634,4.74662633119835,
-1.9010304870377));
#154163=CARTESIAN_POINT('Ctrl Pts',(-7.21800429377516,4.76121922803141,
-1.99830007803845));
#154164=CARTESIAN_POINT('Ctrl Pts',(-7.13157592253394,4.79033919889737,
-2.190429264016));
#154165=CARTESIAN_POINT('Ctrl Pts',(-7.08649245851456,4.80486306093905,
-2.28527988030872));
#154166=CARTESIAN_POINT('Ctrl Pts',(-7.03943126641627,4.81939092104429,
-2.37915084214098));
#154167=CARTESIAN_POINT('Ctrl Pts',(-7.1496792742943,4.819390921,-2.32785890618325));
#154168=CARTESIAN_POINT('Ctrl Pts',(-7.27582211625994,4.754503495,-1.94042955853822));
#154169=CARTESIAN_POINT('Ctrl Pts',(-7.35936093581297,4.689276009,-1.54163790783283));
#154170=CARTESIAN_POINT('Ctrl Pts',(-7.125982234,4.819390921,-2.33888375));
#154171=CARTESIAN_POINT('Ctrl Pts',(-7.25272249400001,4.754503495,-1.952738506));
#154172=CARTESIAN_POINT('Ctrl Pts',(-7.33699399300001,4.689276009,-1.555158883));
#154173=CARTESIAN_POINT('Ctrl Pts',(-6.810596247,4.819390921,-2.485614363));
#154174=CARTESIAN_POINT('Ctrl Pts',(-6.945287596,4.754503495,-2.116559367));
#154175=CARTESIAN_POINT('Ctrl Pts',(-7.03931039,4.689276009,-1.735110727));
#154176=CARTESIAN_POINT('',(-6.92454921546238,4.8193909179172,-2.43259874169278));
#154177=CARTESIAN_POINT('Ctrl Pts',(-6.61725243872918,4.689268254,-3.57061587074017));
#154178=CARTESIAN_POINT('Ctrl Pts',(-6.81328652345985,4.754934719,-3.20731523249149));
#154179=CARTESIAN_POINT('Ctrl Pts',(-6.96837036658216,4.819390921,-2.82473750445019));
#154180=CARTESIAN_POINT('Ctrl Pts',(-6.608873911,4.689268254,-3.545812407));
#154181=CARTESIAN_POINT('Ctrl Pts',(-6.803546235,4.754934719,-3.182971767));
#154182=CARTESIAN_POINT('Ctrl Pts',(-6.95732686000001,4.819390921,-2.80100035));
#154183=CARTESIAN_POINT('Ctrl Pts',(-6.49755179600001,4.689268254,-3.216258799));
#154184=CARTESIAN_POINT('Ctrl Pts',(-6.674130955,4.754934719,-2.85952997));
#154185=CARTESIAN_POINT('Ctrl Pts',(-6.810596247,4.819390921,-2.485614363));
#154186=CARTESIAN_POINT('',(-6.9170597724146,4.81939091969098,-2.71444937933755));
#154187=CARTESIAN_POINT('',(-6.86361189254967,4.81939091820872,-2.59956732185072));
#154188=CARTESIAN_POINT('',(-6.74026277951148,4.73201982385666,-3.32965349748354));
#154189=CARTESIAN_POINT('Ctrl Pts',(-6.91705976785379,4.81939092086901,
-2.71444938335613));
#154190=CARTESIAN_POINT('Ctrl Pts',(-6.89202221803927,4.80491309582878,
-2.81788298886713));
#154191=CARTESIAN_POINT('Ctrl Pts',(-6.86481225063187,4.79041128809892,
-2.92077555594569));
#154192=CARTESIAN_POINT('Ctrl Pts',(-6.80592054268088,4.761286477031,-3.12594297386103));
#154193=CARTESIAN_POINT('Ctrl Pts',(-6.77421992653286,4.74666639461734,
-3.22818860897718));
#154194=CARTESIAN_POINT('Ctrl Pts',(-6.74037582725774,4.73203683303548,
-3.32973030246518));
#154195=CARTESIAN_POINT('Ctrl Pts',(-6.4996632263326,4.69005394725939,-3.2119897183158));
#154196=CARTESIAN_POINT('Ctrl Pts',(-6.5377690158468,4.69707706853122,-3.23066796984932));
#154197=CARTESIAN_POINT('Ctrl Pts',(-6.57593531352748,4.70392124749675,
-3.24935238012372));
#154198=CARTESIAN_POINT('Ctrl Pts',(-6.65607595110484,4.71792585990761,
-3.28854050765078));
#154199=CARTESIAN_POINT('Ctrl Pts',(-6.6981105352828,4.72506040966862,-3.30906922090527));
#154200=CARTESIAN_POINT('Ctrl Pts',(-6.74014973176521,4.73200281467784,
-3.32957669250189));
#154201=CARTESIAN_POINT('Origin',(3.63424568217141E-13,4.93907430000018,
1.19479079407903E-13));
#154202=CARTESIAN_POINT('',(-6.55822016129101,4.93794662025088,-3.233554227833));
#154203=CARTESIAN_POINT('Ctrl Pts',(-6.55822016187665,4.93794661944576,
-3.23355422846586));
#154204=CARTESIAN_POINT('Ctrl Pts',(-6.62167681304073,4.91814186463008,
-3.14963750850499));
#154205=CARTESIAN_POINT('Ctrl Pts',(-6.68333784388084,4.89834552804239,
-3.06439195297611));
#154206=CARTESIAN_POINT('Ctrl Pts',(-6.77298484869264,4.86872423034124,
-2.93471638075813));
#154207=CARTESIAN_POINT('Ctrl Pts',(-6.80234169603496,4.85888055795474,
-2.89127079325353));
#154208=CARTESIAN_POINT('Ctrl Pts',(-6.86292692531123,4.83826147067629,
-2.79951672185459));
#154209=CARTESIAN_POINT('Ctrl Pts',(-6.89156280638917,4.8283384961102,-2.75492833775227));
#154210=CARTESIAN_POINT('Ctrl Pts',(-6.91705977081307,4.8193909199736,-2.7144493782663));
#154211=CARTESIAN_POINT('',(-6.36340617132589,4.81939091960603,-3.83679726201069));
#154212=CARTESIAN_POINT('Ctrl Pts',(-6.36340616948724,4.81939091980664,
-3.83679726136057));
#154213=CARTESIAN_POINT('Ctrl Pts',(-6.3806593570124,4.8283789174746,-3.7907757165676));
#154214=CARTESIAN_POINT('Ctrl Pts',(-6.39875066126507,4.83808522135753,
-3.74107298389996));
#154215=CARTESIAN_POINT('Ctrl Pts',(-6.4349155533591,4.85839508125963,-3.63735682436214));
#154216=CARTESIAN_POINT('Ctrl Pts',(-6.45167800761775,4.86818863433314,
-3.5874315745783));
#154217=CARTESIAN_POINT('Ctrl Pts',(-6.50033940714799,4.89780165972296,
-3.43674114880472));
#154218=CARTESIAN_POINT('Ctrl Pts',(-6.53046315438364,4.91777478469678,
-3.33546502858284));
#154219=CARTESIAN_POINT('Ctrl Pts',(-6.5582201605052,4.93794662098598,-3.23355422776447));
#154220=CARTESIAN_POINT('Ctrl Pts',(-6.74035240177763,4.73205099316135,
-3.32974575144665));
#154221=CARTESIAN_POINT('Ctrl Pts',(-6.68093079468288,4.74662633123018,
-3.41712357109346));
#154222=CARTESIAN_POINT('Ctrl Pts',(-6.61967591711042,4.76121922805284,
-3.50323849301328));
#154223=CARTESIAN_POINT('Ctrl Pts',(-6.49396609790326,4.79033919882502,
-3.67229625980263));
#154224=CARTESIAN_POINT('Ctrl Pts',(-6.42954658131606,4.80486306090825,
-3.7552377095359));
#154225=CARTESIAN_POINT('Ctrl Pts',(-6.363406171612,4.81939092104128,-3.83679725544552));
#154226=CARTESIAN_POINT('Ctrl Pts',(-6.48210289236304,4.819390921,-3.81040455899514));
#154227=CARTESIAN_POINT('Ctrl Pts',(-6.68858244194038,4.754503495,-3.45915007679625));
#154228=CARTESIAN_POINT('Ctrl Pts',(-6.8558965873045,4.689276009,-3.08764033017328));
#154229=CARTESIAN_POINT('Ctrl Pts',(-6.45658986,4.819390921,-3.816077485));
#154230=CARTESIAN_POINT('Ctrl Pts',(-6.66337681600001,4.754503495,-3.466205512));
#154231=CARTESIAN_POINT('Ctrl Pts',(-6.831145961,4.689276009,-3.096036961));
#154232=CARTESIAN_POINT('Ctrl Pts',(-6.117034678,4.819390921,-3.891578954));
#154233=CARTESIAN_POINT('Ctrl Pts',(-6.327912933,4.754503495,-3.560106917));
#154234=CARTESIAN_POINT('Ctrl Pts',(-6.501737708,4.689276009,-3.207788456));
#154235=CARTESIAN_POINT('',(-6.24095952935368,4.8193909179172,-3.86402377588778));
#154236=CARTESIAN_POINT('Ctrl Pts',(-5.69496788889646,4.689268254,-4.90965052517024));
#154237=CARTESIAN_POINT('Ctrl Pts',(-5.96451770339228,4.754934719,-4.59698518770047));
#154238=CARTESIAN_POINT('Ctrl Pts',(-6.19821867492906,4.819390921,-4.25669035731628));
#154239=CARTESIAN_POINT('Ctrl Pts',(-5.69211725800001,4.689268254,-4.883625817));
#154240=CARTESIAN_POINT('Ctrl Pts',(-5.960238263,4.754934719,-4.571116985));
#154241=CARTESIAN_POINT('Ctrl Pts',(-6.192536146,4.819390921,-4.231134137));
#154242=CARTESIAN_POINT('Ctrl Pts',(-5.654242076,4.689268254,-4.537846025));
#154243=CARTESIAN_POINT('Ctrl Pts',(-5.903379066,4.754934719,-4.227416618));
#154244=CARTESIAN_POINT('Ctrl Pts',(-6.117034678,4.819390921,-3.891578954));
#154245=CARTESIAN_POINT('',(-6.17181638077985,4.81939091971653,-4.13795044575052));
#154246=CARTESIAN_POINT('',(-6.14431432941737,4.81939091820872,-4.01426455256242));
#154247=CARTESIAN_POINT('',(-5.86690210342724,4.73201982384263,-4.70076530568075));
#154248=CARTESIAN_POINT('Ctrl Pts',(-6.17181637537512,4.81939092084589,
-4.13795044869547));
#154249=CARTESIAN_POINT('Ctrl Pts',(-6.12512902047052,4.80491309537189,
-4.23358350371706));
#154250=CARTESIAN_POINT('Ctrl Pts',(-6.07643634486721,4.79041128718496,
-4.32822116392062));
#154251=CARTESIAN_POINT('Ctrl Pts',(-5.97481656514734,4.76128647695001,
-4.51593189974137));
#154252=CARTESIAN_POINT('Ctrl Pts',(-5.92187730276754,4.74666639456897,
-4.60897239303821));
#154253=CARTESIAN_POINT('Ctrl Pts',(-5.86699599736058,4.73203683301616,
-4.70086461697002));
#154254=CARTESIAN_POINT('Ctrl Pts',(-5.65722186833484,4.6900539472246,-4.53413064874397));
#154255=CARTESIAN_POINT('Ctrl Pts',(-5.6904214938143,4.69707706850835,-4.56056383126527));
#154256=CARTESIAN_POINT('Ctrl Pts',(-5.72367888888419,4.70392124749352,
-4.58701603615188));
#154257=CARTESIAN_POINT('Ctrl Pts',(-5.79352159389577,4.71792585990658,
-4.64251583503509));
#154258=CARTESIAN_POINT('Ctrl Pts',(-5.83016036631121,4.72506040966537,
-4.67160079145656));
#154259=CARTESIAN_POINT('Ctrl Pts',(-5.8668082094939,4.73200281466911,-4.70066599439149));
#154260=CARTESIAN_POINT('Origin',(5.00901403688303E-13,4.93907429999947,
4.46257614195034E-13));
#154261=CARTESIAN_POINT('',(-5.70977404307001,4.93794662017026,-4.56777900150209));
#154262=CARTESIAN_POINT('Ctrl Pts',(-5.70977404358148,4.93794661922554,
-4.56777900237504));
#154263=CARTESIAN_POINT('Ctrl Pts',(-5.78978672754553,4.9181418644839,-4.49946551303395));
#154264=CARTESIAN_POINT('Ctrl Pts',(-5.86833143216554,4.89834552793919,
-4.42946825032602));
#154265=CARTESIAN_POINT('Ctrl Pts',(-5.98375895432666,4.86872423033756,
-4.32209587730957));
#154266=CARTESIAN_POINT('Ctrl Pts',(-6.02176897178718,4.85888055800352,
-4.28597687805401));
#154267=CARTESIAN_POINT('Ctrl Pts',(-6.1006621650845,4.83826147078189,-4.20939199933421));
#154268=CARTESIAN_POINT('Ctrl Pts',(-6.13821373977607,4.82833849622781,
-4.17200193476362));
#154269=CARTESIAN_POINT('Ctrl Pts',(-6.17181637932586,4.81939092005262,
-4.13795044422738));
#154270=CARTESIAN_POINT('',(-5.38983527523063,4.81939091970597,-5.1150393000287));
#154271=CARTESIAN_POINT('Ctrl Pts',(-5.38983527319774,4.81939091997457,
-5.11503929876886));
#154272=CARTESIAN_POINT('Ctrl Pts',(-5.4165784094306,4.82837893202885,-5.07380256711433));
#154273=CARTESIAN_POINT('Ctrl Pts',(-5.44493138418316,4.83808524390011,
-5.02915091937289));
#154274=CARTESIAN_POINT('Ctrl Pts',(-5.50254660586824,4.85839508130118,
-4.93563407236016));
#154275=CARTESIAN_POINT('Ctrl Pts',(-5.52964961625224,4.86818863439001,
-4.89047947924477));
#154276=CARTESIAN_POINT('Ctrl Pts',(-5.6095673266254,4.89780165979951,-4.75377287414642));
#154277=CARTESIAN_POINT('Ctrl Pts',(-5.66076286351395,4.91777664866465,
-4.66133161615084));
#154278=CARTESIAN_POINT('Ctrl Pts',(-5.70977860043483,4.93794849692008,
-4.56777030045401));
#154279=CARTESIAN_POINT('Ctrl Pts',(-5.86696979846174,4.73205099316642,
-4.70087466896192));
#154280=CARTESIAN_POINT('Ctrl Pts',(-5.79015378711476,4.74662633121483,
-4.7734357548079));
#154281=CARTESIAN_POINT('Ctrl Pts',(-5.71181885180552,4.76121922803017,
-4.84436936979641));
#154282=CARTESIAN_POINT('Ctrl Pts',(-5.55270563680197,4.79033919858816,
-4.98245076390519));
#154283=CARTESIAN_POINT('Ctrl Pts',(-5.47196225209423,4.80486306078942,
-5.04960479741087));
#154284=CARTESIAN_POINT('Ctrl Pts',(-5.38983527625753,4.8193909210351,-5.11503929400405));
#154285=CARTESIAN_POINT('Ctrl Pts',(-5.51143058358818,4.819390921,-5.11477993069985));
#154286=CARTESIAN_POINT('Ctrl Pts',(-5.7885920867199,4.754503495,-4.81612458249205));
#154287=CARTESIAN_POINT('Ctrl Pts',(-6.0318581341366,4.689276009,-4.4892681216581));
#154288=CARTESIAN_POINT('Ctrl Pts',(-5.48529452,4.819390921,-5.114835679));
#154289=CARTESIAN_POINT('Ctrl Pts',(-5.762459044,4.754503495,-4.817596601));
#154290=CARTESIAN_POINT('Ctrl Pts',(-6.005881136,4.689276009,-4.492147791));
#154291=CARTESIAN_POINT('Ctrl Pts',(-5.137447365,4.819390921,-5.115577638));
#154292=CARTESIAN_POINT('Ctrl Pts',(-5.414652094,4.754503495,-4.837187824));
#154293=CARTESIAN_POINT('Ctrl Pts',(-5.66015099700001,4.689276009,-4.530473562));
#154294=CARTESIAN_POINT('',(-5.2643984710689,4.81939091791741,-5.11530686482257));
#154295=CARTESIAN_POINT('Ctrl Pts',(-4.50639296980373,4.689268254,-6.01911537846736));
#154296=CARTESIAN_POINT('Ctrl Pts',(-4.83685466449597,4.754934719,-5.771705224826));
#154297=CARTESIAN_POINT('Ctrl Pts',(-5.13824516666925,4.819390921,-5.48960509895427));
#154298=CARTESIAN_POINT('Ctrl Pts',(-4.509203528,4.689268254,-5.993086312));
#154299=CARTESIAN_POINT('Ctrl Pts',(-4.838236174,4.754934719,-5.745521853));
#154300=CARTESIAN_POINT('Ctrl Pts',(-5.138189324,4.819390921,-5.46342479300001));
#154301=CARTESIAN_POINT('Ctrl Pts',(-4.54654628,4.689268254,-5.647248615));
#154302=CARTESIAN_POINT('Ctrl Pts',(-4.85659173300001,4.754934719,-5.397633963));
#154303=CARTESIAN_POINT('Ctrl Pts',(-5.137447365,4.819390921,-5.11557763800001));
#154304=CARTESIAN_POINT('',(-5.13798571439769,4.81939091970502,-5.3679655482769));
#154305=CARTESIAN_POINT('',(-5.13771545634754,4.81939091820872,-5.24125923432883));
#154306=CARTESIAN_POINT('',(-4.71921160543078,4.73201982384171,-5.85207455297479));
#154307=CARTESIAN_POINT('Ctrl Pts',(-5.13798570851046,4.81939092085927,
-5.36796555001529));
#154308=CARTESIAN_POINT('Ctrl Pts',(-5.07183159928317,4.80491309562667,
-5.45132635462913));
#154309=CARTESIAN_POINT('Ctrl Pts',(-5.00393303326813,4.79041128770499,
-5.53328395155443));
#154310=CARTESIAN_POINT('Ctrl Pts',(-4.86433680581298,4.76128647699594,
-5.69476086848324));
#154311=CARTESIAN_POINT('Ctrl Pts',(-4.79263427810061,4.74666639459734,
-5.77424575029438));
#154312=CARTESIAN_POINT('Ctrl Pts',(-4.71928195522053,4.73203683302225,
-5.85219172679468));
#154313=CARTESIAN_POINT('Ctrl Pts',(-4.55025510313446,4.69005394736987,
-5.64426066962907));
#154314=CARTESIAN_POINT('Ctrl Pts',(-4.57699618710132,4.69707706863428,
-5.67721279719471));
#154315=CARTESIAN_POINT('Ctrl Pts',(-4.60378960046422,4.70392124753795,
-5.71019592079278));
#154316=CARTESIAN_POINT('Ctrl Pts',(-4.66006860578606,4.71792585992939,
-5.77941228229491));
#154317=CARTESIAN_POINT('Ctrl Pts',(-4.68959837815049,4.72506040966796,
-5.81569350156484));
#154318=CARTESIAN_POINT('Ctrl Pts',(-4.71914125564104,4.73200281466116,
-5.8519573791549));
#154319=CARTESIAN_POINT('Origin',(-1.53089346754953E-13,4.93907429999875,
-2.01661604082304E-13));
#154320=CARTESIAN_POINT('',(-4.5943452367228,4.93794662024679,-5.68841950581731));
#154321=CARTESIAN_POINT('Ctrl Pts',(-4.59434523707343,4.93794661918462,
-5.68841950689947));
#154322=CARTESIAN_POINT('Ctrl Pts',(-4.68717264971606,4.91814186448087,
-5.63890351089828));
#154323=CARTESIAN_POINT('Ctrl Pts',(-4.77892836507603,4.89834552794767,
-5.58742753507463));
#154324=CARTESIAN_POINT('Ctrl Pts',(-4.91473914215364,4.86872423031433,
-5.5073789738014));
#154325=CARTESIAN_POINT('Ctrl Pts',(-4.9596250237364,4.85888055795239,-5.48027544686202));
#154326=CARTESIAN_POINT('Ctrl Pts',(-5.05313722302055,4.8382614706992,-5.42244078465439));
#154327=CARTESIAN_POINT('Ctrl Pts',(-5.0978486212441,4.82833849615031,-5.39399735769675));
#154328=CARTESIAN_POINT('Ctrl Pts',(-5.13798571334812,4.81939092001646,
-5.36796554655156));
#154329=CARTESIAN_POINT('',(-4.16424167158184,4.81939091970267,-6.15410778547649));
#154330=CARTESIAN_POINT('Ctrl Pts',(-4.16424166989983,4.81939091995633,
-6.15410778383816));
#154331=CARTESIAN_POINT('Ctrl Pts',(-4.19922416010835,4.82837891178309,
-6.11958420957116));
#154332=CARTESIAN_POINT('Ctrl Pts',(-4.23651301091994,4.83808521293132,
-6.08207158245674));
#154333=CARTESIAN_POINT('Ctrl Pts',(-4.31288469475123,4.85839508127127,
-6.00312655673912));
#154334=CARTESIAN_POINT('Ctrl Pts',(-4.3490609546311,4.86818863438469,-5.96485399891931));
#154335=CARTESIAN_POINT('Ctrl Pts',(-4.45649811260519,4.89780165987256,
-5.84852346342451));
#154336=CARTESIAN_POINT('Ctrl Pts',(-4.52636242450352,4.91777478489387,
-5.76925637902194));
#154337=CARTESIAN_POINT('Ctrl Pts',(-4.59434523579166,4.9379466212469,-5.6884195052838));
#154338=CARTESIAN_POINT('Ctrl Pts',(-4.71925420797629,4.7320509931407,-5.8521959118125));
#154339=CARTESIAN_POINT('Ctrl Pts',(-4.62863562367905,4.746626331206,-5.90654738803205));
#154340=CARTESIAN_POINT('Ctrl Pts',(-4.53688348514562,4.76121922803168,
-5.95898291901078));
#154341=CARTESIAN_POINT('Ctrl Pts',(-4.35180682815207,4.79033919897972,
-6.05963141031581));
#154342=CARTESIAN_POINT('Ctrl Pts',(-4.25851504799658,4.80486306098252,
-6.10785797814731));
#154343=CARTESIAN_POINT('Ctrl Pts',(-4.16424167386614,4.81939092104639,
-6.15410777983815));
#154344=CARTESIAN_POINT('Ctrl Pts',(-4.28304990569923,4.819390921,-6.17999387708313));
#154345=CARTESIAN_POINT('Ctrl Pts',(-4.61793359871535,4.754503495,-5.94790245508186));
#154346=CARTESIAN_POINT('Ctrl Pts',(-4.92577669870553,4.689276009,-5.68098272644485));
#154347=CARTESIAN_POINT('Ctrl Pts',(-4.257512905,4.819390921,-6.17442984100001));
#154348=CARTESIAN_POINT('Ctrl Pts',(-4.592095092,4.754503495,-5.943722227));
#154349=CARTESIAN_POINT('Ctrl Pts',(-4.899787985,4.689276009,-5.67821078400001));
#154350=CARTESIAN_POINT('Ctrl Pts',(-3.917638724,4.819390921,-6.100377597));
#154351=CARTESIAN_POINT('Ctrl Pts',(-4.248208141,4.754503495,-5.88808720500001));
#154352=CARTESIAN_POINT('Ctrl Pts',(-4.553901916,4.689276009,-5.64131875900001));
#154353=CARTESIAN_POINT('',(-4.04043957907225,4.81939091791743,-6.1271336267888));
#154354=CARTESIAN_POINT('Ctrl Pts',(-3.10710412312025,4.689268254,-6.84713308652525));
#154355=CARTESIAN_POINT('Ctrl Pts',(-3.48302567743148,4.754934719,-6.67654674054884));
#154356=CARTESIAN_POINT('Ctrl Pts',(-3.8380130251523,4.819390921,-6.4658320075701));
#154357=CARTESIAN_POINT('Ctrl Pts',(-3.115444452,4.689268254,-6.822316752));
#154358=CARTESIAN_POINT('Ctrl Pts',(-3.490003539,4.754934719,-6.651272505));
#154359=CARTESIAN_POINT('Ctrl Pts',(-3.84358648,4.819390921,-6.440251778));
#154360=CARTESIAN_POINT('Ctrl Pts',(-3.226259034,4.689268254,-6.492592136));
#154361=CARTESIAN_POINT('Ctrl Pts',(-3.582715568,4.754934719,-6.315463943));
#154362=CARTESIAN_POINT('Ctrl Pts',(-3.917638724,4.819390921,-6.100377597));
#154363=CARTESIAN_POINT('',(-3.86390854667387,4.81939091970075,-6.34698054757804));
#154364=CARTESIAN_POINT('',(-3.89088271932647,4.81939091820872,-6.22317845909021));
#154365=CARTESIAN_POINT('',(-3.35085601772043,4.73201982388317,-6.72974729825321));
#154366=CARTESIAN_POINT('Ctrl Pts',(-3.86390854051543,4.81939092087177,
-6.34698054805234));
#154367=CARTESIAN_POINT('Ctrl Pts',(-3.78138097004906,4.8049130958697,-6.41417124432607));
#154368=CARTESIAN_POINT('Ctrl Pts',(-3.69745137556109,4.79041128819257,
-6.47961653253445));
#154369=CARTESIAN_POINT('Ctrl Pts',(-3.52640606383257,4.76128647705211,
-6.60730914834069));
#154370=CARTESIAN_POINT('Ctrl Pts',(-3.43929300122602,4.74666639464369,
-6.66952179391214));
#154371=CARTESIAN_POINT('Ctrl Pts',(-3.35089953388808,4.73203683306755,
-6.72987685571895));
#154372=CARTESIAN_POINT('Ctrl Pts',(-3.23052346702925,4.69005394743846,
-6.49047133482806));
#154373=CARTESIAN_POINT('Ctrl Pts',(-3.24955562586843,4.69707706873026,
-6.5284016026402));
#154374=CARTESIAN_POINT('Ctrl Pts',(-3.26863222727741,4.70392124758219,
-6.56637339066714));
#154375=CARTESIAN_POINT('Ctrl Pts',(-3.30871598892618,4.71792585998442,
-6.64606983462008));
#154376=CARTESIAN_POINT('Ctrl Pts',(-3.32975598189518,4.7250604097162,-6.68785084722996));
#154377=CARTESIAN_POINT('Ctrl Pts',(-3.35081250155278,4.73200281469878,
-6.72961774078747));
#154378=CARTESIAN_POINT('Origin',(-4.77048955893622E-15,4.93907430000053,
7.80625564189564E-15));
#154379=CARTESIAN_POINT('',(-3.26408995174312,4.93794662025481,-6.54307583749208));
#154380=CARTESIAN_POINT('Ctrl Pts',(-3.26408995181825,4.93794661952797,
-6.54307583826685));
#154381=CARTESIAN_POINT('Ctrl Pts',(-3.36539158685823,4.9181418646899,-6.51467264853357));
#154382=CARTESIAN_POINT('Ctrl Pts',(-3.46606791803756,4.89834552807624,
-6.48412491890387));
#154383=CARTESIAN_POINT('Ctrl Pts',(-3.61591158944693,4.86872423035731,
-6.43514315094611));
#154384=CARTESIAN_POINT('Ctrl Pts',(-3.66557452130607,4.85888055797118,
-6.41832242708623));
#154385=CARTESIAN_POINT('Ctrl Pts',(-3.76933320020153,4.83826147070826,
-6.38194226575869));
#154386=CARTESIAN_POINT('Ctrl Pts',(-3.81911376685812,4.82833849615013,
-6.36377545925099));
#154387=CARTESIAN_POINT('Ctrl Pts',(-3.86390854603416,4.81939092000138,
-6.34698054571165));
#154388=CARTESIAN_POINT('',(-2.74393275536061,4.81939091966315,-6.90541703078901));
#154389=CARTESIAN_POINT('Ctrl Pts',(-2.74393275405512,4.81939091994474,
-6.90541702881319));
#154390=CARTESIAN_POINT('Ctrl Pts',(-2.78551901199698,4.82837892998224,
-6.8792207421115));
#154391=CARTESIAN_POINT('Ctrl Pts',(-2.83000021338486,4.83808524130702,
-6.85060111088975));
#154392=CARTESIAN_POINT('Ctrl Pts',(-2.92155708880109,4.85839508127528,
-6.78991951522507));
#154393=CARTESIAN_POINT('Ctrl Pts',(-2.9651150362015,4.86818863433114,-6.76031857521332));
#154394=CARTESIAN_POINT('Ctrl Pts',(-3.09504799913575,4.89780165970208,
-6.66980359646244));
#154395=CARTESIAN_POINT('Ctrl Pts',(-3.18031900209256,4.91777478466184,
-6.60740849449519));
#154396=CARTESIAN_POINT('Ctrl Pts',(-3.2640899512144,4.93794662092021,-6.54307583701224));
#154397=CARTESIAN_POINT('Ctrl Pts',(-3.35087153571166,4.7320509931687,-6.72987497807152));
#154398=CARTESIAN_POINT('Ctrl Pts',(-3.25068760284654,4.74662633121048,
-6.7634754300197));
#154399=CARTESIAN_POINT('Ctrl Pts',(-3.14980848920595,4.76121922802042,
-6.79496104980241));
#154400=CARTESIAN_POINT('Ctrl Pts',(-2.94742237247686,4.79033919877432,
-6.85347042449631));
#154401=CARTESIAN_POINT('Ctrl Pts',(-2.8459444151631,4.80486306087506,-6.88051450712535));
#154402=CARTESIAN_POINT('Ctrl Pts',(-2.74393275928622,4.81939092104137,
-6.90541702555452));
#154403=CARTESIAN_POINT('Ctrl Pts',(-2.85439857559013,4.819390921,-6.95623817828906));
#154404=CARTESIAN_POINT('Ctrl Pts',(-3.23134566830383,4.754503495,-6.80156301980523));
#154405=CARTESIAN_POINT('Ctrl Pts',(-3.58937141931755,4.689276009,-6.6070608921574));
#154406=CARTESIAN_POINT('Ctrl Pts',(-2.830654719,4.819390921,-6.945314526));
#154407=CARTESIAN_POINT('Ctrl Pts',(-3.207009877,4.754503495,-6.791926008));
#154408=CARTESIAN_POINT('Ctrl Pts',(-3.564586193,4.689276009,-6.598766951));
#154409=CARTESIAN_POINT('Ctrl Pts',(-2.51464565,4.819390921,-6.79993068));
#154410=CARTESIAN_POINT('Ctrl Pts',(-2.883122697,4.754503495,-6.663666173));
#154411=CARTESIAN_POINT('Ctrl Pts',(-3.234717443,4.689276009,-6.488382161));
#154412=CARTESIAN_POINT('',(-2.62997704800503,4.81939091791719,-6.85299031890594));
#154413=CARTESIAN_POINT('Ctrl Pts',(-1.5625305423085,4.689268254,-7.35498646080462));
#154414=CARTESIAN_POINT('Ctrl Pts',(-1.96633428062159,4.754934719,-7.26920035157733));
#154415=CARTESIAN_POINT('Ctrl Pts',(-2.35831966042307,4.819390921,-7.13972379752685));
#154416=CARTESIAN_POINT('Ctrl Pts',(-1.576010657,4.689268254,-7.332543243));
#154417=CARTESIAN_POINT('Ctrl Pts',(-1.978582217,4.754934719,-7.246017048));
#154418=CARTESIAN_POINT('Ctrl Pts',(-2.369261804,4.819390921,-7.115939748));
#154419=CARTESIAN_POINT('Ctrl Pts',(-1.755115501,4.689268254,-7.034349265));
#154420=CARTESIAN_POINT('Ctrl Pts',(-2.141315605,4.754934719,-6.937989849));
#154421=CARTESIAN_POINT('Ctrl Pts',(-2.51464565,4.819390921,-6.79993068000001));
#154422=CARTESIAN_POINT('',(-2.40915930973851,4.81939091976617,-7.02921779085296));
#154423=CARTESIAN_POINT('',(-2.46211663093204,4.81939091820872,-6.91410877610072));
#154424=CARTESIAN_POINT('',(-1.82581812686482,4.73201982382574,-7.29274453948536));
#154425=CARTESIAN_POINT('Ctrl Pts',(-2.40915930329185,4.81939092085653,
-7.02921778994019));
#154426=CARTESIAN_POINT('Ctrl Pts',(-2.31411716591817,4.80491309552321,
-7.07709661798109));
#154427=CARTESIAN_POINT('Ctrl Pts',(-2.21808099413988,4.7904112875162,-7.12296945072462));
#154428=CARTESIAN_POINT('Ctrl Pts',(-2.02358449302411,4.76128647696444,
-7.21090699632491));
#154429=CARTESIAN_POINT('Ctrl Pts',(-1.92513420577956,4.74666639456743,
-7.25293841133325));
#154430=CARTESIAN_POINT('Ctrl Pts',(-1.8258327745597,4.73203683300157,-7.2928804226923));
#154431=CARTESIAN_POINT('Ctrl Pts',(-1.75973614394115,4.69005394753977,
-7.03319477416654));
#154432=CARTESIAN_POINT('Ctrl Pts',(-1.77016945516759,4.69707706885708,
-7.0743296052304));
#154433=CARTESIAN_POINT('Ctrl Pts',(-1.78063724402955,4.7039212475672,-7.11551453859287));
#154434=CARTESIAN_POINT('Ctrl Pts',(-1.80265148994025,4.71792585997664,
-7.20196454805052));
#154435=CARTESIAN_POINT('Ctrl Pts',(-1.814217896818,4.72506040968594,-7.24729172026223));
#154436=CARTESIAN_POINT('Ctrl Pts',(-1.82580347916994,4.73200281464992,
-7.29260865627842));
#154437=CARTESIAN_POINT('Origin',(6.25584653524136E-14,4.93907430000036,
6.55291793050239E-13));
#154438=CARTESIAN_POINT('',(-1.7812094499623,4.93794662024309,-7.09178521416007));
#154439=CARTESIAN_POINT('Ctrl Pts',(-1.78120944984785,4.93794661935037,
-7.09178521510926));
#154440=CARTESIAN_POINT('Ctrl Pts',(-1.88624855505386,4.91814186459227,
-7.08582293318277));
#154441=CARTESIAN_POINT('Ctrl Pts',(-1.99113798834326,4.89834552802905,
-7.07763182769846));
#154442=CARTESIAN_POINT('Ctrl Pts',(-2.14800803001082,4.86872423039614,
-7.06200718622492));
#154443=CARTESIAN_POINT('Ctrl Pts',(-2.20012582844497,4.85888055804361,
-7.05625578385709));
#154444=CARTESIAN_POINT('Ctrl Pts',(-2.30927934629833,4.83826147084028,
-7.04303121932758));
#154445=CARTESIAN_POINT('Ctrl Pts',(-2.36180139727908,4.82833849632546,
-7.03599049297186));
#154446=CARTESIAN_POINT('Ctrl Pts',(-2.40915930948499,4.81939092018277,
-7.02921778852983));
#154447=CARTESIAN_POINT('',(-1.19532059297275,4.81939091961768,-7.33383665019445));
#154448=CARTESIAN_POINT('Ctrl Pts',(-1.19532059224552,4.81939091984225,
-7.33383664829511));
#154449=CARTESIAN_POINT('Ctrl Pts',(-1.24156587632055,4.82837890505971,
-7.3171926799642));
#154450=CARTESIAN_POINT('Ctrl Pts',(-1.29115944652801,4.83808520204432,
-7.29880433204201));
#154451=CARTESIAN_POINT('Ctrl Pts',(-1.393620720796,4.85839508137039,-7.25922338349757));
#154452=CARTESIAN_POINT('Ctrl Pts',(-1.44252363468209,4.86818863443235,
-7.23967816813496));
#154453=CARTESIAN_POINT('Ctrl Pts',(-1.58887688197419,4.89780165982057,
-7.1792111255017));
#154454=CARTESIAN_POINT('Ctrl Pts',(-1.68556739885766,4.91777478478944,
-7.13660553136001));
#154455=CARTESIAN_POINT('Ctrl Pts',(-1.78120944944539,4.93794662107547,
-7.09178521343167));
#154456=CARTESIAN_POINT('Ctrl Pts',(-1.82580583459438,4.73205099314127,
-7.29287257012552));
#154457=CARTESIAN_POINT('Ctrl Pts',(-1.72074104247871,4.74662633119089,
-7.30415087801442));
#154458=CARTESIAN_POINT('Ctrl Pts',(-1.61545194892915,4.76121922800212,
-7.31321435402907));
#154459=CARTESIAN_POINT('Ctrl Pts',(-1.40521972391614,4.79033919836613,
-7.32684877926749));
#154460=CARTESIAN_POINT('Ctrl Pts',(-1.30030058497591,4.80486306067414,
-7.33144582527584));
#154461=CARTESIAN_POINT('Ctrl Pts',(-1.19532059816352,4.81939092102958,
-7.33383664612755));
#154462=CARTESIAN_POINT('Ctrl Pts',(-1.29227873911615,4.819390921,-7.40721651375988));
#154463=CARTESIAN_POINT('Ctrl Pts',(-1.6936636054524,4.754503495,-7.33719005668571));
#154464=CARTESIAN_POINT('Ctrl Pts',(-2.08513112145502,4.689276009,-7.22420023456691));
#154465=CARTESIAN_POINT('Ctrl Pts',(-1.271438263,4.819390921,-7.391444023));
#154466=CARTESIAN_POINT('Ctrl Pts',(-1.671968444,4.754503495,-7.32254687700001));
#154467=CARTESIAN_POINT('Ctrl Pts',(-2.062708312,4.689276009,-7.21077211));
#154468=CARTESIAN_POINT('Ctrl Pts',(-0.994070541,4.819390921,-7.181526562));
#154469=CARTESIAN_POINT('Ctrl Pts',(-1.38322564,4.754503495,-7.127659516));
#154470=CARTESIAN_POINT('Ctrl Pts',(-1.764281177,4.689276009,-7.03205602400001));
#154471=CARTESIAN_POINT('',(-1.09428701315445,4.81939091791739,-7.25737241764825));
#154472=CARTESIAN_POINT('Ctrl Pts',(0.0551052307094634,4.689268254,-7.5189288428372));
#154473=CARTESIAN_POINT('Ctrl Pts',(-0.35769927843588,4.754934719,-7.5219542327515));
#154474=CARTESIAN_POINT('Ctrl Pts',(-0.768353889884251,4.819390921,-7.47977003953121));
#154475=CARTESIAN_POINT('Ctrl Pts',(0.037115645,4.689268254,-7.499908161));
#154476=CARTESIAN_POINT('Ctrl Pts',(-0.37464459,4.754934719,-7.501945886));
#154477=CARTESIAN_POINT('Ctrl Pts',(-0.78415308,4.819390921,-7.458894285));
#154478=CARTESIAN_POINT('Ctrl Pts',(-0.201904718,4.689268254,-7.24718804));
#154479=CARTESIAN_POINT('Ctrl Pts',(-0.599790104,4.754934719,-7.23610306));
#154480=CARTESIAN_POINT('Ctrl Pts',(-0.994070541000001,4.819390921,-7.18152656200001));
#154481=CARTESIAN_POINT('',(-0.918224705199005,4.81939091820872,-7.28174305106958));
#154482=CARTESIAN_POINT('Ctrl Pts',(-0.206665514464669,4.6900539473239,
-7.24705384062151));
#154483=CARTESIAN_POINT('Ctrl Pts',(-0.208012127751941,4.69707706859336,
-7.28946981548055));
#154484=CARTESIAN_POINT('Ctrl Pts',(-0.209381642204492,4.70392124749239,
-7.33194213439115));
#154485=CARTESIAN_POINT('Ctrl Pts',(-0.212297010587137,4.71792585990076,
-7.42110340287249));
#154486=CARTESIAN_POINT('Ctrl Pts',(-0.213848999159561,4.72506040965179,
-7.4678572868583));
#154487=CARTESIAN_POINT('Ctrl Pts',(-0.215421915432243,4.73200281465868,
-7.51460529612207));
#154488=CARTESIAN_POINT('Ctrl Pts',(0.33026661393265,4.819390921,-7.51184163683667));
#154489=CARTESIAN_POINT('Ctrl Pts',(-0.0767877158185115,4.754503495,-7.52973824160898));
#154490=CARTESIAN_POINT('Ctrl Pts',(-0.483392409605453,4.689276009,-7.50354400259746));
#154491=CARTESIAN_POINT('Ctrl Pts',(0.347229232,4.819390921,-7.491957812));
#154492=CARTESIAN_POINT('Ctrl Pts',(-0.0587476260000001,4.754503495,-7.510773593));
#154493=CARTESIAN_POINT('Ctrl Pts',(-0.464380483,4.689276009,-7.485609579));
#154494=CARTESIAN_POINT('Ctrl Pts',(0.572986203,4.819390921,-7.227322244));
#154495=CARTESIAN_POINT('Ctrl Pts',(0.181349511,4.754503495,-7.25837142200001));
#154496=CARTESIAN_POINT('Ctrl Pts',(-0.211349085,4.689276009,-7.24691876300001));
#154497=CARTESIAN_POINT('',(0.490593424731472,4.8193909179172,-7.32390426471178));
#154498=CARTESIAN_POINT('Ctrl Pts',(1.67016434457945,4.689268254,-7.33129446975108));
#154499=CARTESIAN_POINT('Ctrl Pts',(1.26766134467495,4.754934719,-7.4229898936172));
#154500=CARTESIAN_POINT('Ctrl Pts',(0.857539254896607,4.819390921,-7.47007054607416));
#154501=CARTESIAN_POINT('Ctrl Pts',(1.648506461,4.689268254,-7.31658571));
#154502=CARTESIAN_POINT('Ctrl Pts',(1.246811002,4.754934719,-7.407092072));
#154503=CARTESIAN_POINT('Ctrl Pts',(0.837621771,4.819390921,-7.453079214));
#154504=CARTESIAN_POINT('Ctrl Pts',(1.360746905,4.689268254,-7.121156357));
#154505=CARTESIAN_POINT('Ctrl Pts',(0.969780916,4.754934719,-7.195864134));
#154506=CARTESIAN_POINT('Ctrl Pts',(0.572986203,4.819390921,-7.227322244));
#154507=CARTESIAN_POINT('',(0.764998170628619,4.81939091971407,-7.39112502452024));
#154508=CARTESIAN_POINT('',(0.668602387742703,4.81939091820872,-7.30889111458854));
#154509=CARTESIAN_POINT('',(1.40507629994002,4.73201982382458,-7.38535681886841));
#154510=CARTESIAN_POINT('Ctrl Pts',(0.764998175836196,4.81939092085866,
-7.39112502113075));
#154511=CARTESIAN_POINT('Ctrl Pts',(0.871359881258293,4.80491309562033,
-7.39467151086817));
#154512=CARTESIAN_POINT('Ctrl Pts',(0.977781452401426,4.79041128768559,
-7.3959800244164));
#154513=CARTESIAN_POINT('Ctrl Pts',(1.19122571432888,4.7612864770025,-7.39412301811676));
#154514=CARTESIAN_POINT('Ctrl Pts',(1.29822530834739,4.7466663945937,-7.39093149455899));
#154515=CARTESIAN_POINT('Ctrl Pts',(1.4051200618959,4.73203683300444,-7.38548629353271));
#154516=CARTESIAN_POINT('Ctrl Pts',(1.35606856510726,4.69005394731185,-7.12204872604118));
#154517=CARTESIAN_POINT('Ctrl Pts',(1.36387161560206,4.69707706857266,-7.16376252089336));
#154518=CARTESIAN_POINT('Ctrl Pts',(1.3716644127257,4.70392124750565,-7.20553626584865));
#154519=CARTESIAN_POINT('Ctrl Pts',(1.38798424111399,4.71792585989974,-7.29323971123585));
#154520=CARTESIAN_POINT('Ctrl Pts',(1.39651924019486,4.72506040964578,-7.33923414698756));
#154521=CARTESIAN_POINT('Ctrl Pts',(1.40503253798415,4.73200281464471,-7.3852273442041));
#154522=CARTESIAN_POINT('Origin',(1.3389896830196E-14,4.93907429999875,
-4.15032591627451E-13));
#154523=CARTESIAN_POINT('',(1.361181406915,4.93794662024243,-7.18424037779173));
#154524=CARTESIAN_POINT('Ctrl Pts',(1.36118140755056,4.93794661911314,-7.18424037882069));
#154525=CARTESIAN_POINT('Ctrl Pts',(1.26334700045149,4.91814186435326,-7.22293393378318));
#154526=CARTESIAN_POINT('Ctrl Pts',(1.16471257319447,4.89834552781051,-7.25954181764329));
#154527=CARTESIAN_POINT('Ctrl Pts',(1.0157805627591,4.86872423021828,-7.31122929788308));
#154528=CARTESIAN_POINT('Ctrl Pts',(0.966064778855809,4.85888055788355,
-7.32789316199559));
#154529=CARTESIAN_POINT('Ctrl Pts',(0.861446878623905,4.838261470707,-7.36172324479444));
#154530=CARTESIAN_POINT('Ctrl Pts',(0.810822831831353,4.82833849618497,
-7.37738669142729));
#154531=CARTESIAN_POINT('Ctrl Pts',(0.764998169975832,4.81939092004315,
-7.39112502255717));
#154532=CARTESIAN_POINT('',(1.9945544934734,4.81939091960363,-7.15791196534276));
#154533=CARTESIAN_POINT('Ctrl Pts',(1.99455449333891,4.81939091980167,-7.15791196340296));
#154534=CARTESIAN_POINT('Ctrl Pts',(1.94559476297443,4.82837890968501,-7.1622242001431));
#154535=CARTESIAN_POINT('Ctrl Pts',(1.89286378000787,4.83808520897093,-7.16635918701156));
#154536=CARTESIAN_POINT('Ctrl Pts',(1.78325287452173,4.85839508130526,-7.17345886106996));
#154537=CARTESIAN_POINT('Ctrl Pts',(1.73066296862473,4.86818863442145,-7.17625390465097));
#154538=CARTESIAN_POINT('Ctrl Pts',(1.5724469059283,4.89780165990501,-7.18282763662407));
#154539=CARTESIAN_POINT('Ctrl Pts',(1.46680334461262,4.91777478493161,-7.18475914088505));
#154540=CARTESIAN_POINT('Ctrl Pts',(1.36118140712162,4.93794662129573,-7.18424037668054));
#154541=CARTESIAN_POINT('Ctrl Pts',(1.40514121474242,4.73205099312586,-7.38546785495625));
#154542=CARTESIAN_POINT('Ctrl Pts',(1.50523107615726,4.74662633118788,-7.35158820878161));
#154543=CARTESIAN_POINT('Ctrl Pts',(1.60459452427703,4.76121922800804,-7.31560425391225));
#154544=CARTESIAN_POINT('Ctrl Pts',(1.80112107278766,4.79033919867926,-7.23970430222656));
#154545=CARTESIAN_POINT('Ctrl Pts',(1.89827335282728,4.80486306083143,-7.19982206555386));
#154546=CARTESIAN_POINT('Ctrl Pts',(1.99455448709657,4.81939092103824,-7.15791196385871));
#154547=CARTESIAN_POINT('Ctrl Pts',(1.93736906818931,4.819390921,-7.26522139449432));
#154548=CARTESIAN_POINT('Ctrl Pts',(1.54367868338508,4.754503495,-7.37020423461234));
#154549=CARTESIAN_POINT('Ctrl Pts',(1.14094919361909,4.689276009,-7.43203039289954));
#154550=CARTESIAN_POINT('Ctrl Pts',(1.949660675,4.819390921,-7.242155981));
#154551=CARTESIAN_POINT('Ctrl Pts',(1.557220167,4.754503495,-7.34780488300001));
#154552=CARTESIAN_POINT('Ctrl Pts',(1.155661261,4.689276009,-7.410428264));
#154553=CARTESIAN_POINT('Ctrl Pts',(2.113250748,4.819390921,-6.93517637));
#154554=CARTESIAN_POINT('Ctrl Pts',(1.73744496,4.754503495,-7.04968994800001));
#154555=CARTESIAN_POINT('Ctrl Pts',(1.351465456,4.689276009,-7.122923636));
#154556=CARTESIAN_POINT('',(2.05354654700379,4.81939091791738,-7.04721236860803));
#154557=CARTESIAN_POINT('Ctrl Pts',(3.20712842978384,4.689268254,-6.80085691434977));
#154558=CARTESIAN_POINT('Ctrl Pts',(2.83374753197936,4.754934719,-6.97693479805095));
#154559=CARTESIAN_POINT('Ctrl Pts',(2.44333481731984,4.819390921,-7.11107885687941));
#154560=CARTESIAN_POINT('Ctrl Pts',(3.182814947,4.689268254,-6.79114784200001));
#154561=CARTESIAN_POINT('Ctrl Pts',(2.809967097,4.754934719,-6.965890866));
#154562=CARTESIAN_POINT('Ctrl Pts',(2.420230359,4.819390921,-7.098766443));
#154563=CARTESIAN_POINT('Ctrl Pts',(2.859771516,4.689268254,-6.662147317));
#154564=CARTESIAN_POINT('Ctrl Pts',(2.494006057,4.754934719,-6.819154599));
#154565=CARTESIAN_POINT('Ctrl Pts',(2.113250748,4.819390921,-6.93517637));
#154566=CARTESIAN_POINT('',(2.33598633845085,4.81939091972229,-7.0538726353531));
#154567=CARTESIAN_POINT('',(2.22416637565606,4.81939091820872,-6.99428355248962));
#154568=CARTESIAN_POINT('',(2.95985980325624,4.73201982382998,-6.91064140985388));
#154569=CARTESIAN_POINT('Ctrl Pts',(2.33598634279356,4.81939092086852,-7.05387263091369));
#154570=CARTESIAN_POINT('Ctrl Pts',(2.44062375986601,4.80491309579386,-7.03447158329896));
#154571=CARTESIAN_POINT('Ctrl Pts',(2.54483854424275,4.79041128804214,-7.0128720128882));
#154572=CARTESIAN_POINT('Ctrl Pts',(2.75289339897587,4.76128647701724,-6.96517421484957));
#154573=CARTESIAN_POINT('Ctrl Pts',(2.85670531885606,4.74666639459917,-6.93905555747064));
#154574=CARTESIAN_POINT('Ctrl Pts',(2.95993037533596,4.73203683300646,-6.91075844994129));
#154575=CARTESIAN_POINT('Ctrl Pts',(2.85539438564915,4.69005394748178,-6.66402452836791));
#154576=CARTESIAN_POINT('Ctrl Pts',(2.87198223804774,4.69707706875983,-6.70308565294994));
#154577=CARTESIAN_POINT('Ctrl Pts',(2.88857296395198,4.70392124756544,-6.74220752936085));
#154578=CARTESIAN_POINT('Ctrl Pts',(2.92336489211045,4.71792585995299,-6.82435223648));
#154579=CARTESIAN_POINT('Ctrl Pts',(2.94158779172578,4.72506040967516,-6.86743657534881));
#154580=CARTESIAN_POINT('Ctrl Pts',(2.95978923117651,4.73200281465349,-6.91052436976648));
#154581=CARTESIAN_POINT('Origin',(6.13658429626796E-14,4.93907429999947,
-3.72098185597025E-13));
#154582=CARTESIAN_POINT('',(2.87375706009855,4.93794662024794,-6.72366306323252));
#154583=CARTESIAN_POINT('Ctrl Pts',(2.87375706070915,4.9379466194289,-6.72366306386225));
#154584=CARTESIAN_POINT('Ctrl Pts',(2.78652793794651,4.91814186461107,-6.78248349077825));
#154585=CARTESIAN_POINT('Ctrl Pts',(2.69806914139962,4.89834552800437,-6.83943898910689));
#154586=CARTESIAN_POINT('Ctrl Pts',(2.56373035855149,4.86872423031914,-6.92193402490032));
#154587=CARTESIAN_POINT('Ctrl Pts',(2.51875914010647,4.85888055795341,-6.94889572116907));
#154588=CARTESIAN_POINT('Ctrl Pts',(2.42385961591318,4.83826147075346,-7.00442463156618));
#154589=CARTESIAN_POINT('Ctrl Pts',(2.3777863091507,4.82833849621868,-7.03060454918325));
#154590=CARTESIAN_POINT('Ctrl Pts',(2.33598633738469,4.81939092005231,-7.0538726335647));
#154591=CARTESIAN_POINT('',(3.4866624037102,4.8193909195952,-6.56179370394099));
#154592=CARTESIAN_POINT('Ctrl Pts',(3.48666240317772,4.8193909197725,-6.56179370213862));
#154593=CARTESIAN_POINT('Ctrl Pts',(3.43977429249229,4.82837891588597,-6.57653002753051));
#154594=CARTESIAN_POINT('Ctrl Pts',(3.38916501125661,4.83808521941846,-6.59190394743572));
#154595=CARTESIAN_POINT('Ctrl Pts',(3.28364302290187,4.85839508118745,-6.62240072374302));
#154596=CARTESIAN_POINT('Ctrl Pts',(3.23288349162489,4.86818863429477,-6.63643569594599));
#154597=CARTESIAN_POINT('Ctrl Pts',(3.07977959098872,4.89780165972668,-6.67686751425433));
#154598=CARTESIAN_POINT('Ctrl Pts',(2.97702113403897,4.91777478470248,-6.70146410384215));
#154599=CARTESIAN_POINT('Ctrl Pts',(2.87375706007209,4.93794662099952,-6.72366306242647));
#154600=CARTESIAN_POINT('Ctrl Pts',(2.95994706988585,4.73205099314337,-6.91073589519746));
#154601=CARTESIAN_POINT('Ctrl Pts',(3.05041376349921,4.74662633121276,-6.8561319747512));
#154602=CARTESIAN_POINT('Ctrl Pts',(3.13971866278778,4.76121922803844,-6.79962910056749));
#154603=CARTESIAN_POINT('Ctrl Pts',(3.31533428564133,4.79033919902709,-6.68325624768655));
#154604=CARTESIAN_POINT('Ctrl Pts',(3.40164169634223,4.80486306101155,-6.62342156777488));
#154605=CARTESIAN_POINT('Ctrl Pts',(3.4866623972128,4.81939092104663,-6.56179370386531));
#154606=CARTESIAN_POINT('Ctrl Pts',(3.45388229713187,4.819390921,-6.67888747440437));
#154607=CARTESIAN_POINT('Ctrl Pts',(3.09196438218115,4.754503495,-6.86604766914545));
#154608=CARTESIAN_POINT('Ctrl Pts',(2.71194128065134,4.689276009,-7.01300330203434));
#154609=CARTESIAN_POINT('Ctrl Pts',(3.460928151,4.819390921,-6.653718985));
#154610=CARTESIAN_POINT('Ctrl Pts',(3.100374075,4.754503495,-6.841260983));
#154611=CARTESIAN_POINT('Ctrl Pts',(2.721665569,4.689276009,-6.988743559));
#154612=CARTESIAN_POINT('Ctrl Pts',(3.554702037,4.819390921,-6.318749356));
#154613=CARTESIAN_POINT('Ctrl Pts',(3.212299413,4.754503495,-6.511372807));
#154614=CARTESIAN_POINT('Ctrl Pts',(2.851086974,4.689276009,-6.665868515));
#154615=CARTESIAN_POINT('',(3.52082035429869,4.81939091791742,-6.43977814068551));
#154616=CARTESIAN_POINT('Ctrl Pts',(4.59413075429447,4.689268254,-5.95241884841558));
#154617=CARTESIAN_POINT('Ctrl Pts',(4.26733083418468,4.754934719,-6.20464598542213));
#154618=CARTESIAN_POINT('Ctrl Pts',(3.91488275966786,4.819390921,-6.41958102282211));
#154619=CARTESIAN_POINT('Ctrl Pts',(4.568298544,4.689268254,-5.948163449));
#154620=CARTESIAN_POINT('Ctrl Pts',(4.241732254,4.754934719,-6.198972345));
#154621=CARTESIAN_POINT('Ctrl Pts',(3.889671666,4.819390921,-6.412523242));
#154622=CARTESIAN_POINT('Ctrl Pts',(4.225076389,4.689268254,-5.891623674));
#154623=CARTESIAN_POINT('Ctrl Pts',(3.901614248,4.754934719,-6.123588974));
#154624=CARTESIAN_POINT('Ctrl Pts',(3.554702037,4.819390921,-6.318749356));
#154625=CARTESIAN_POINT('',(3.79774638263754,4.81939091972637,-6.38678900096167));
#154626=CARTESIAN_POINT('',(3.67573081612178,4.81939091820872,-6.35263106417826));
#154627=CARTESIAN_POINT('',(4.37624355193186,4.73201982384556,-6.11279208909231));
#154628=CARTESIAN_POINT('Ctrl Pts',(3.79774638599498,4.81939092085526,-6.38678899563233));
#154629=CARTESIAN_POINT('Ctrl Pts',(3.89576678816968,4.80491309551935,-6.34534758150289));
#154630=CARTESIAN_POINT('Ctrl Pts',(3.99290182116961,4.79041128749769,-6.30184989818854));
#154631=CARTESIAN_POINT('Ctrl Pts',(4.18583884888006,4.76128647695171,-6.21054160612787));
#154632=CARTESIAN_POINT('Ctrl Pts',(4.2816089641817,4.74666639456629,-6.1627170944889));
#154633=CARTESIAN_POINT('Ctrl Pts',(4.37633763423928,4.73203683302124,-6.11289122193341));
#154634=CARTESIAN_POINT('Ctrl Pts',(4.22120513800341,4.69005394745124,-5.8943979506271));
#154635=CARTESIAN_POINT('Ctrl Pts',(4.24580216290519,4.69707706874209,-5.92897994972898));
#154636=CARTESIAN_POINT('Ctrl Pts',(4.27041505393711,4.70392124756459,-5.96362066268045));
#154637=CARTESIAN_POINT('Ctrl Pts',(4.32205225002897,4.71792585996443,-6.03636563588632));
#154638=CARTESIAN_POINT('Ctrl Pts',(4.34911096763941,4.72506040969101,-6.0745253020366));
#154639=CARTESIAN_POINT('Ctrl Pts',(4.37614946962444,4.73200281466989,-6.1126929562512));
#154640=CARTESIAN_POINT('Origin',(1.6978606021123E-13,4.93907429999947,
-5.68121938382404E-14));
#154641=CARTESIAN_POINT('',(4.2519590248966,4.93794662024346,-5.94869473742009));
#154642=CARTESIAN_POINT('Ctrl Pts',(4.25195902576348,4.9379466192731,-5.94869473799322));
#154643=CARTESIAN_POINT('Ctrl Pts',(4.1794139247583,4.9181418644975,-6.02489165867405));
#154644=CARTESIAN_POINT('Ctrl Pts',(4.1052669945485,4.89834552794473,-6.09953159527505));
#154645=CARTESIAN_POINT('Ctrl Pts',(3.99180297237013,4.86872423032577,-6.20897680991753));
#154646=CARTESIAN_POINT('Ctrl Pts',(3.95367912386868,4.85888055797775,-6.24497563923672));
#154647=CARTESIAN_POINT('Ctrl Pts',(3.87293537213586,4.83826147073724,-6.31960690711586));
#154648=CARTESIAN_POINT('Ctrl Pts',(3.83356714218467,4.82833849620036,-6.35507915179506));
#154649=CARTESIAN_POINT('Ctrl Pts',(3.79774638116995,4.81939092007985,-6.38678899940356));
#154650=CARTESIAN_POINT('',(4.81573785503565,4.8193909195985,-5.65885326212327));
#154651=CARTESIAN_POINT('Ctrl Pts',(4.81573785412003,4.81939091978043,-5.65885326046163));
#154652=CARTESIAN_POINT('Ctrl Pts',(4.77311389288525,4.82837890454499,-5.68332458283608));
#154653=CARTESIAN_POINT('Ctrl Pts',(4.72699279340066,4.83808520180399,-5.70921855673414));
#154654=CARTESIAN_POINT('Ctrl Pts',(4.63049367195276,4.85839508124016,-5.7616864892933));
#154655=CARTESIAN_POINT('Ctrl Pts',(4.58393797450878,4.86818863433821,-5.7863051303968));
#154656=CARTESIAN_POINT('Ctrl Pts',(4.44310520378661,4.89780165977954,-5.85870448813445));
#154657=CARTESIAN_POINT('Ctrl Pts',(4.3480367221006,4.91777478478945,-5.90481605383178));
#154658=CARTESIAN_POINT('Ctrl Pts',(4.25195902465804,4.9379466211439,-5.9486947364838));
#154659=CARTESIAN_POINT('Ctrl Pts',(4.37634908987473,4.7320509931612,-6.11286560566984));
#154660=CARTESIAN_POINT('Ctrl Pts',(4.45296249357072,4.74662633122668,-6.04009062964906));
#154661=CARTESIAN_POINT('Ctrl Pts',(4.52803304613346,4.76121922804461,-5.96571084781629));
#154662=CARTESIAN_POINT('Ctrl Pts',(4.67452614959537,4.7903391989875,-5.81430656012054));
#154663=CARTESIAN_POINT('Ctrl Pts',(4.74595305356124,4.80486306098948,-5.7373172396589));
#154664=CARTESIAN_POINT('Ctrl Pts',(4.81573784867121,4.8193909210453,-5.65885326343773));
#154665=CARTESIAN_POINT('Ctrl Pts',(4.80889582853022,4.819390921,-5.7802561994388));
#154666=CARTESIAN_POINT('Ctrl Pts',(4.4956732629108,4.754503495,-6.04084234557442));
#154667=CARTESIAN_POINT('Ctrl Pts',(4.15612600775738,4.689276009,-6.26605597125353));
#154668=CARTESIAN_POINT('Ctrl Pts',(4.810366473,4.819390921,-5.754161485));
#154669=CARTESIAN_POINT('Ctrl Pts',(4.498557937,4.754503495,-6.014827323));
#154670=CARTESIAN_POINT('Ctrl Pts',(4.16040782,4.689276009,-6.240272973));
#154671=CARTESIAN_POINT('Ctrl Pts',(4.829939409,4.819390921,-5.406864646));
#154672=CARTESIAN_POINT('Ctrl Pts',(4.536950317,4.754503495,-5.66859111));
#154673=CARTESIAN_POINT('Ctrl Pts',(4.217394834,4.689276009,-5.89712479200001));
#154674=CARTESIAN_POINT('',(4.82279603852955,4.81939091791738,-5.53361490783684));
#154675=CARTESIAN_POINT('Ctrl Pts',(5.76631663010193,4.689268254,-4.82565229291977));
#154676=CARTESIAN_POINT('Ctrl Pts',(5.50137849007381,4.754934719,-5.1422348217962));
#154677=CARTESIAN_POINT('Ctrl Pts',(5.20337513502365,4.819390921,-5.42791071594587));
#154678=CARTESIAN_POINT('Ctrl Pts',(5.74017357700001,4.689268254,-4.827049544));
#154679=CARTESIAN_POINT('Ctrl Pts',(5.475158725,4.754934719,-5.142196766));
#154680=CARTESIAN_POINT('Ctrl Pts',(5.177236248,4.819390921,-5.426437582));
#154681=CARTESIAN_POINT('Ctrl Pts',(5.392821385,4.689268254,-4.845614255));
#154682=CARTESIAN_POINT('Ctrl Pts',(5.126787292,4.754934719,-5.141691134));
#154683=CARTESIAN_POINT('Ctrl Pts',(4.829939409,4.819390921,-5.406864646));
#154684=CARTESIAN_POINT('',(5.08192802541004,4.81939091972029,-5.42106621189636));
#154685=CARTESIAN_POINT('',(4.95542216813492,4.81939091820872,-5.41393660870127));
#154686=CARTESIAN_POINT('',(5.58799901600127,4.73201982386544,-5.02911540404799));
#154687=CARTESIAN_POINT('Ctrl Pts',(5.08192802756682,4.81939092086455,-5.4210662059747));
#154688=CARTESIAN_POINT('Ctrl Pts',(5.16874808717188,4.80491309572286,-5.35952218075136));
#154689=CARTESIAN_POINT('Ctrl Pts',(5.25426143996334,4.79041128789788,-5.29616028910016));
#154690=CARTESIAN_POINT('Ctrl Pts',(5.42305912547235,4.76128647702865,-5.16551097479791));
#154691=CARTESIAN_POINT('Ctrl Pts',(5.50630933252438,4.74666639462265,-5.09821682969789));
#154692=CARTESIAN_POINT('Ctrl Pts',(5.58811220930506,4.73203683304752,-5.02919199433367));
#154693=CARTESIAN_POINT('Ctrl Pts',(5.38963703028743,4.69005394753149,-4.84915587539731));
#154694=CARTESIAN_POINT('Ctrl Pts',(5.42109309802439,4.69707706884286,-4.87764173344675));
#154695=CARTESIAN_POINT('Ctrl Pts',(5.45257728229003,4.7039212475901,-4.906181521479));
#154696=CARTESIAN_POINT('Ctrl Pts',(5.51864524839433,4.71792585999831,-4.96612528693495));
#154697=CARTESIAN_POINT('Ctrl Pts',(5.55327454843862,4.72506040971483,-4.99757597681861));
#154698=CARTESIAN_POINT('Ctrl Pts',(5.58788582269747,4.73200281468336,-5.02903881376231));
#154699=CARTESIAN_POINT('Origin',(2.52402265754625E-13,4.93907430000018,
-1.57859836313889E-13));
#154700=CARTESIAN_POINT('',(5.43134411168424,4.93794662030685,-4.89557205727329));
#154701=CARTESIAN_POINT('Ctrl Pts',(5.43134411273164,4.93794661925887,-4.89557205767653));
#154702=CARTESIAN_POINT('Ctrl Pts',(5.37687516145781,4.9181418644691,-4.98558258899984));
#154703=CARTESIAN_POINT('Ctrl Pts',(5.32050712531743,4.89834552788478,-5.07441688360505));
#154704=CARTESIAN_POINT('Ctrl Pts',(5.23322331493081,4.86872423024933,-5.20569474071468));
#154705=CARTESIAN_POINT('Ctrl Pts',(5.2037294650359,4.85888055790566,-5.24904743786462));
#154706=CARTESIAN_POINT('Ctrl Pts',(5.14091697406473,4.83826147074124,-5.33929138771099));
#154707=CARTESIAN_POINT('Ctrl Pts',(5.11009463552047,4.82833849622207,-5.38239731671222));
#154708=CARTESIAN_POINT('Ctrl Pts',(5.08192802368369,4.81939092006014,-5.42106621071751));
#154709=CARTESIAN_POINT('',(5.91963475744616,4.81939091962027,-4.49131113040391));
#154710=CARTESIAN_POINT('Ctrl Pts',(5.9196347561068,4.81939091985038,-4.49131112886811));
#154711=CARTESIAN_POINT('Ctrl Pts',(5.88326785870452,4.82837892128484,-4.52437328388305));
#154712=CARTESIAN_POINT('Ctrl Pts',(5.84379145345502,4.83808522668422,-4.5595765661234));
#154713=CARTESIAN_POINT('Ctrl Pts',(5.76082758369809,4.85839508134986,-4.63156219823851));
#154714=CARTESIAN_POINT('Ctrl Pts',(5.72065261291011,4.86818863441021,-4.66561336776986));
#154715=CARTESIAN_POINT('Ctrl Pts',(5.59867615593021,4.89780165987564,-4.76659495141481));
#154716=CARTESIAN_POINT('Ctrl Pts',(5.51574294592142,4.91777478493435,-4.83206536780779));
#154717=CARTESIAN_POINT('Ctrl Pts',(5.43134411120292,4.93794662130489,-4.89557205631661));
#154718=CARTESIAN_POINT('Ctrl Pts',(5.58811789039565,4.73205099315931,-5.02916451435992));
#154719=CARTESIAN_POINT('Ctrl Pts',(5.64729564669879,4.74662633121721,-4.94162135968071));
#154720=CARTESIAN_POINT('Ctrl Pts',(5.70462163705322,4.76121922803165,-4.85284258604163));
#154721=CARTESIAN_POINT('Ctrl Pts',(5.81514236548186,4.79033919860815,-4.67348636165991));
#154722=CARTESIAN_POINT('Ctrl Pts',(5.86834892079121,4.80486306079293,-4.58294233458863));
#154723=CARTESIAN_POINT('Ctrl Pts',(5.91963475136461,4.81939092103644,-4.49131113315614));
#154724=CARTESIAN_POINT('Ctrl Pts',(5.93905073662225,4.819390921,-4.61134656846007));
#154725=CARTESIAN_POINT('Ctrl Pts',(5.68916945885119,4.754503495,-4.9331739483148));
#154726=CARTESIAN_POINT('Ctrl Pts',(5.40597490160482,4.689276009,-5.22611482698729));
#154727=CARTESIAN_POINT('Ctrl Pts',(5.934877406,4.819390921,-4.585545789));
#154728=CARTESIAN_POINT('Ctrl Pts',(5.68639423,4.754503495,-4.907147023));
#154729=CARTESIAN_POINT('Ctrl Pts',(5.404614025,4.689276009,-5.200014158));
#154730=CARTESIAN_POINT('Ctrl Pts',(5.879334183,4.819390921,-4.242160954));
#154731=CARTESIAN_POINT('Ctrl Pts',(5.649458466,4.754503495,-4.560752393));
#154732=CARTESIAN_POINT('Ctrl Pts',(5.386501999,4.689276009,-4.852638067));
#154733=CARTESIAN_POINT('',(5.89960538046836,4.8193909179172,-4.36748347900853));
#154734=CARTESIAN_POINT('Ctrl Pts',(6.66887594922512,4.689268254,-3.47324360036106));
#154735=CARTESIAN_POINT('Ctrl Pts',(6.47818780120644,4.754934719,-3.83937847364755));
#154736=CARTESIAN_POINT('Ctrl Pts',(6.24856347140929,4.819390921,-4.18243733692546));
#154737=CARTESIAN_POINT('Ctrl Pts',(6.643644474,4.689268254,-3.480228168));
#154738=CARTESIAN_POINT('Ctrl Pts',(6.452572859,4.754934719,-3.844977782));
#154739=CARTESIAN_POINT('Ctrl Pts',(6.222719017,4.819390921,-4.186617732));
#154740=CARTESIAN_POINT('Ctrl Pts',(6.308404047,4.689268254,-3.573029299));
#154741=CARTESIAN_POINT('Ctrl Pts',(6.112237461,4.754934719,-3.919373532));
#154742=CARTESIAN_POINT('Ctrl Pts',(5.879334183,4.819390921,-4.242160954));
#154743=CARTESIAN_POINT('',(6.12848436209898,4.81939091971738,-4.20186039183531));
#154744=CARTESIAN_POINT('',(6.00340348775815,4.81939091820872,-4.22209249434916));
#154745=CARTESIAN_POINT('',(6.53846585632056,4.73201982386532,-3.71028287274101));
#154746=CARTESIAN_POINT('Ctrl Pts',(6.12848436286711,4.81939092087191,-4.2018603856999));
#154747=CARTESIAN_POINT('Ctrl Pts',(6.20004447082737,4.80491309586707,-4.12309147994593));
#154748=CARTESIAN_POINT('Ctrl Pts',(6.26993763454746,4.79041128819051,-4.04282811188466));
#154749=CARTESIAN_POINT('Ctrl Pts',(6.40670318462008,4.76128647705193,-3.87894679171586));
#154750=CARTESIAN_POINT('Ctrl Pts',(6.47354079612634,4.74666639463727,-3.79532961265998));
#154751=CARTESIAN_POINT('Ctrl Pts',(6.53859286789724,4.73203683304325,-3.71033333914916));
#154752=CARTESIAN_POINT('Ctrl Pts',(6.30605548406717,4.69005394743836,-3.57717266011216));
#154753=CARTESIAN_POINT('Ctrl Pts',(6.3428997435947,4.69707706869056,-3.59823040999787));
#154754=CARTESIAN_POINT('Ctrl Pts',(6.37978305655066,4.70392124755452,-3.61933478523539));
#154755=CARTESIAN_POINT('Ctrl Pts',(6.4571925278355,4.71792585994776,-3.66367443923128));
#154756=CARTESIAN_POINT('Ctrl Pts',(6.49777318281428,4.72506040968754,-3.68694555374012));
#154757=CARTESIAN_POINT('Ctrl Pts',(6.53833884474388,4.7320028146874,-3.71023240633286));
#154758=CARTESIAN_POINT('Origin',(5.41233724504764E-13,4.93907429999964,
-3.14201789586299E-13));
#154759=CARTESIAN_POINT('',(6.35676558561064,4.9379466202581,-3.61353786721423));
#154760=CARTESIAN_POINT('Ctrl Pts',(6.35676558641561,4.93794661949784,-3.61353786733658));
#154761=CARTESIAN_POINT('Ctrl Pts',(6.3229196923951,4.91814186467107,-3.71315321718136));
#154762=CARTESIAN_POINT('Ctrl Pts',(6.28696625694172,4.8983455280375,-3.8120280771608));
#154763=CARTESIAN_POINT('Ctrl Pts',(6.22994395212096,4.86872423032536,-3.95900017046747));
#154764=CARTESIAN_POINT('Ctrl Pts',(6.21045920039375,4.85888055795967,-4.00767961165742));
#154765=CARTESIAN_POINT('Ctrl Pts',(6.16851501210557,4.83826147076072,-4.10931653712138));
#154766=CARTESIAN_POINT('Ctrl Pts',(6.14767978318993,4.82833849621905,-4.15804056525908));
#154767=CARTESIAN_POINT('Ctrl Pts',(6.12848436019905,4.81939092003673,-4.20186039106825));
#154768=CARTESIAN_POINT('',(6.74673611732405,4.81939091966401,-3.11376028273081));
#154769=CARTESIAN_POINT('Ctrl Pts',(6.74673611541487,4.81939091994905,-3.11376028131458));
#154770=CARTESIAN_POINT('Ctrl Pts',(6.71832675655188,4.82837894707265,-3.15386739304371));
#154771=CARTESIAN_POINT('Ctrl Pts',(6.68734090682483,4.83808526753276,-3.19673395510896));
#154772=CARTESIAN_POINT('Ctrl Pts',(6.62179160131477,4.85839508125913,-3.28487120529323));
#154773=CARTESIAN_POINT('Ctrl Pts',(6.58987589384118,4.86818863433174,-3.32676270870871));
#154774=CARTESIAN_POINT('Ctrl Pts',(6.49245923422682,4.89780165972544,-3.45160473170117));
#154775=CARTESIAN_POINT('Ctrl Pts',(6.42553916100857,4.91777478469304,-3.5333726746681));
#154776=CARTESIAN_POINT('Ctrl Pts',(6.3567655851381,4.93794662095604,-3.61353786663321));
#154777=CARTESIAN_POINT('Ctrl Pts',(6.53859250876927,4.73205099317319,-3.71030528036639));
#154778=CARTESIAN_POINT('Ctrl Pts',(6.57756753156013,4.74662633124687,-3.61208736757819));
#154779=CARTESIAN_POINT('Ctrl Pts',(6.6144684601147,4.7612192280688,-3.51306079885455));
#154780=CARTESIAN_POINT('Ctrl Pts',(6.68384898913673,4.79033919873798,-3.31413913287888));
#154781=CARTESIAN_POINT('Ctrl Pts',(6.71634731529611,4.80486306086017,-3.21427413852161));
#154782=CARTESIAN_POINT('Ctrl Pts',(6.74673611187852,4.81939092103915,-3.11376028637559));
#154783=CARTESIAN_POINT('Ctrl Pts',(6.79150223242666,4.819390921,-3.22681549701117));
#154784=CARTESIAN_POINT('Ctrl Pts',(6.61664641316176,4.754503495,-3.59483582030978));
#154785=CARTESIAN_POINT('Ctrl Pts',(6.40304641741186,4.689276009,-3.94180636280658));
#154786=CARTESIAN_POINT('Ctrl Pts',(6.781880067,4.819390921,-3.202515068));
#154787=CARTESIAN_POINT('Ctrl Pts',(6.60834104800001,4.754503495,-3.570013982));
#154788=CARTESIAN_POINT('Ctrl Pts',(6.396106485,4.689276009,-3.916608461));
#154789=CARTESIAN_POINT('Ctrl Pts',(6.65381782500001,4.819390921,-2.879098531));
#154790=CARTESIAN_POINT('Ctrl Pts',(6.497804216,4.754503495,-3.239657963));
#154791=CARTESIAN_POINT('Ctrl Pts',(6.303742317,4.689276009,-3.58124738));
#154792=CARTESIAN_POINT('',(6.70055573136945,4.81939091791743,-2.99713337640664));
#154793=CARTESIAN_POINT('Ctrl Pts',(7.25960604149006,4.689268254,-1.95842989642778));
#154794=CARTESIAN_POINT('Ctrl Pts',(7.15208425107236,4.754934719,-2.35699705509661));
#154795=CARTESIAN_POINT('Ctrl Pts',(7.0015759247285,4.819390921,-2.74139783555722));
#154796=CARTESIAN_POINT('Ctrl Pts',(7.23646594,4.689268254,-1.97067519));
#154797=CARTESIAN_POINT('Ctrl Pts',(7.128271858,4.754934719,-2.36797191));
#154798=CARTESIAN_POINT('Ctrl Pts',(6.977234361,4.819390921,-2.751036289));
#154799=CARTESIAN_POINT('Ctrl Pts',(6.929012748,4.689268254,-2.133373465));
#154800=CARTESIAN_POINT('Ctrl Pts',(6.811886199,4.754934719,-2.513790379));
#154801=CARTESIAN_POINT('Ctrl Pts',(6.653817825,4.819390921,-2.879098531));
#154802=CARTESIAN_POINT('',(6.88847958175789,4.81939091976399,-2.78618024947188));
#154803=CARTESIAN_POINT('',(6.77067233276658,4.81939091820872,-2.83282802776268));
#154804=CARTESIAN_POINT('',(7.18320130066625,4.73201982383894,-2.21796163729291));
#154805=CARTESIAN_POINT('Ctrl Pts',(6.88847958119671,4.81939092085773,-2.78618024299713));
#154806=CARTESIAN_POINT('Ctrl Pts',(6.94143366829728,4.80491309556365,-2.69386960074661));
#154807=CARTESIAN_POINT('Ctrl Pts',(6.99243851802072,4.79041128758828,-2.60045777954763));
#154808=CARTESIAN_POINT('Ctrl Pts',(7.09077692407315,4.7612864769949,-2.41100736677257));
#154809=CARTESIAN_POINT('Ctrl Pts',(7.13807668749975,4.74666639459136,-2.31497700028956));
#154810=CARTESIAN_POINT('Ctrl Pts',(7.18333619157649,4.73203683301509,-2.21798362007685));
#154811=CARTESIAN_POINT('Ctrl Pts',(6.92760979322192,4.69005394737233,-2.13792482796009));
#154812=CARTESIAN_POINT('Ctrl Pts',(6.96811944820875,4.69707706867108,-2.15056983262706));
#154813=CARTESIAN_POINT('Ctrl Pts',(7.00867726644626,4.70392124753095,-2.16325197718333));
#154814=CARTESIAN_POINT('Ctrl Pts',(7.09380866214356,4.71792585994454,-2.18991424646924));
#154815=CARTESIAN_POINT('Ctrl Pts',(7.13844316561336,4.72506040967912,-2.20391765390694));
#154816=CARTESIAN_POINT('Ctrl Pts',(7.18306640975602,4.73200281466279,-2.21793965450897));
#154817=CARTESIAN_POINT('Origin',(6.57026516526216E-13,4.93907430000125,
-1.80844922370582E-13));
#154818=CARTESIAN_POINT('',(6.98495176460664,4.93794662022521,-2.16253866434672));
#154819=CARTESIAN_POINT('Ctrl Pts',(6.98495285287821,4.93794846925664,-2.16252889722076));
#154820=CARTESIAN_POINT('Ctrl Pts',(6.97331261263774,4.91814371449703,-2.26709116209391));
#154821=CARTESIAN_POINT('Ctrl Pts',(6.95945383338078,4.89834552799468,-2.37139307551936));
#154822=CARTESIAN_POINT('Ctrl Pts',(6.935359333946,4.86872423037574,-2.52718715267149));
#154823=CARTESIAN_POINT('Ctrl Pts',(6.92679476578634,4.85888055803537,-2.57891714116587));
#154824=CARTESIAN_POINT('Ctrl Pts',(6.90768014386894,4.83826147081477,-2.68719461261355));
#154825=CARTESIAN_POINT('Ctrl Pts',(6.89780625681373,4.82833849629522,-2.73925845828388));
#154826=CARTESIAN_POINT('Ctrl Pts',(6.88847957946565,4.8193909201761,-2.78618024909484));
#154827=CARTESIAN_POINT('',(7.25836759455823,4.81939091960755,-1.59061346457017));
#154828=CARTESIAN_POINT('Ctrl Pts',(7.25836759274682,4.81939091981385,-1.59061346376413));
#154829=CARTESIAN_POINT('Ctrl Pts',(7.2392443413621,4.82837891576264,-1.63588989669372));
#154830=CARTESIAN_POINT('Ctrl Pts',(7.21819800562684,4.83808521910493,-1.68441523451707));
#154831=CARTESIAN_POINT('Ctrl Pts',(7.17312800219686,4.85839508139569,-1.78458328712413));
#154832=CARTESIAN_POINT('Ctrl Pts',(7.1509639011611,4.86818863447246,-1.83235632410635));
#154833=CARTESIAN_POINT('Ctrl Pts',(7.08266213355276,4.89780165987253,-1.9752213120985));
#154834=CARTESIAN_POINT('Ctrl Pts',(7.03488430515766,4.91777478482829,-2.0694634035917));
#154835=CARTESIAN_POINT('Ctrl Pts',(6.98495176389734,4.93794662106943,-2.16253866378324));
#154836=CARTESIAN_POINT('Ctrl Pts',(7.18332980902812,4.73205099315307,-2.21795629449247));
#154837=CARTESIAN_POINT('Ctrl Pts',(7.20027966947563,4.74662633120077,-2.11365618425764));
#154838=CARTESIAN_POINT('Ctrl Pts',(7.21503008972912,4.7612192280067,-2.0090121929705));
#154839=CARTESIAN_POINT('Ctrl Pts',(7.24002626209827,4.79033919833949,-1.79982644475022));
#154840=CARTESIAN_POINT('Ctrl Pts',(7.25029677383234,4.80486306066114,-1.69531005772086));
#154841=CARTESIAN_POINT('Ctrl Pts',(7.25836759025581,4.81939092102856,-1.59061346945665));
#154842=CARTESIAN_POINT('Ctrl Pts',(7.32639063248861,4.819390921,-1.69140211925593));
#154843=CARTESIAN_POINT('Ctrl Pts',(7.23473633580764,4.754503495,-2.08840716336033));
#154844=CARTESIAN_POINT('Ctrl Pts',(7.10071859964245,4.689276009,-2.47318341352876));
#154845=CARTESIAN_POINT('Ctrl Pts',(7.311769554,4.819390921,-1.669738302));
#154846=CARTESIAN_POINT('Ctrl Pts',(7.221289184,4.754503495,-2.065951054));
#154847=CARTESIAN_POINT('Ctrl Pts',(7.08852411500001,4.689276009,-2.450066505));
#154848=CARTESIAN_POINT('Ctrl Pts',(7.11717634000001,4.819390921,-1.381412661));
#154849=CARTESIAN_POINT('Ctrl Pts',(7.04231986300001,4.754503495,-1.767080728));
#154850=CARTESIAN_POINT('Ctrl Pts',(6.926226651,4.689276009,-2.142401545));
#154851=CARTESIAN_POINT('',(7.18819554290371,4.81939091791719,-1.48664064912483));
#154852=CARTESIAN_POINT('Ctrl Pts',(7.51088502287621,4.689268254,-0.352042186526741));
#154853=CARTESIAN_POINT('Ctrl Pts',(7.49155719048726,4.754934719,-0.764405074307319));
#154854=CARTESIAN_POINT('Ctrl Pts',(7.42720247132914,4.819390921,-1.17217361937048));
#154855=CARTESIAN_POINT('Ctrl Pts',(7.4909183,4.689268254,-0.36897563));
#154856=CARTESIAN_POINT('Ctrl Pts',(7.470660787,4.754934719,-0.780242304));
#154857=CARTESIAN_POINT('Ctrl Pts',(7.405501982,4.819390921,-1.186819448));
#154858=CARTESIAN_POINT('Ctrl Pts',(7.22562851299999,4.689268254,-0.593963458000001));
#154859=CARTESIAN_POINT('Ctrl Pts',(7.193018709,4.754934719,-0.990665182));
#154860=CARTESIAN_POINT('Ctrl Pts',(7.11717634,4.819390921,-1.381412661));
#154861=CARTESIAN_POINT('',(7.22135206436877,4.81939091820872,-1.31110367082324));
#154862=CARTESIAN_POINT('Ctrl Pts',(7.2252367670457,4.69005394743003,-0.598710006737396));
#154863=CARTESIAN_POINT('Ctrl Pts',(7.26751763097446,4.69707706870792,-0.6023509997094));
#154864=CARTESIAN_POINT('Ctrl Pts',(7.30985351641467,4.7039212475935,-0.606017910678717));
#154865=CARTESIAN_POINT('Ctrl Pts',(7.39872618716097,4.71792585997227,-0.613756097271705));
#154866=CARTESIAN_POINT('Ctrl Pts',(7.44532747948944,4.72506040969926,-0.617837014015916));
#154867=CARTESIAN_POINT('Ctrl Pts',(7.49192177268656,4.73200281467246,-0.62193850969841));
#154868=CARTESIAN_POINT('Ctrl Pts',(7.51870514809341,4.819390921,-0.076900657597555));
#154869=CARTESIAN_POINT('Ctrl Pts',(7.51453802865909,4.754503495,-0.484326909943372));
#154870=CARTESIAN_POINT('Ctrl Pts',(7.46636907136083,4.689276009,-0.888917156273409));
#154871=CARTESIAN_POINT('Ctrl Pts',(7.499768822,4.819390921,-0.058886428));
#154872=CARTESIAN_POINT('Ctrl Pts',(7.496577864,4.754503495,-0.465286552));
#154873=CARTESIAN_POINT('Ctrl Pts',(7.449490235,4.689276009,-0.868962162));
#154874=CARTESIAN_POINT('Ctrl Pts',(7.2477436,4.819390921,0.180866531));
#154875=CARTESIAN_POINT('Ctrl Pts',(7.25754446000001,4.754503495,-0.211876761));
#154876=CARTESIAN_POINT('Ctrl Pts',(7.22484832400001,4.689276009,-0.603379396));
#154877=CARTESIAN_POINT('',(7.33880352304753,4.81939091791719,0.0942407518356453));
#154878=CARTESIAN_POINT('Ctrl Pts',(7.41096336896773,4.689268254,1.27080662387004));
#154879=CARTESIAN_POINT('Ctrl Pts',(7.48073324162791,4.754934719,0.86392963883171));
#154880=CARTESIAN_POINT('Ctrl Pts',(7.50554128344012,4.819390921,0.451860133748774));
#154881=CARTESIAN_POINT('Ctrl Pts',(7.39510364700001,4.689268254,1.24997682));
#154882=CARTESIAN_POINT('Ctrl Pts',(7.463729921,4.754934719,0.843970566));
#154883=CARTESIAN_POINT('Ctrl Pts',(7.48749656,4.819390921,0.432891753));
#154884=CARTESIAN_POINT('Ctrl Pts',(7.18438192,4.689268254,0.97321962));
#154885=CARTESIAN_POINT('Ctrl Pts',(7.23781366,4.754934719,0.578782418));
#154886=CARTESIAN_POINT('Ctrl Pts',(7.2477436,4.819390921,0.180866531));
#154887=CARTESIAN_POINT('',(7.42170146897581,4.81939091973662,0.363728793212368));
#154888=CARTESIAN_POINT('',(7.33436939906887,4.81939091820872,0.271926436703321));
#154889=CARTESIAN_POINT('',(7.4505948541799,4.73201982386191,1.00318047675999));
#154890=CARTESIAN_POINT('Ctrl Pts',(7.42170146582378,4.81939092087145,0.363728798718234));
#154891=CARTESIAN_POINT('Ctrl Pts',(7.43100106085642,4.80491309582812,0.469742510757373));
#154892=CARTESIAN_POINT('Ctrl Pts',(7.43806920306258,4.79041128812343,0.575937162154928));
#154893=CARTESIAN_POINT('Ctrl Pts',(7.44777055976193,4.76128647702322,0.789168928915151));
#154894=CARTESIAN_POINT('Ctrl Pts',(7.45037655808387,4.74666639461449,0.896184384460626));
#154895=CARTESIAN_POINT('Ctrl Pts',(7.45072650818383,4.7320368330397,1.00321716493418));
#154896=CARTESIAN_POINT('Ctrl Pts',(7.18501969993772,4.69005394736277,0.968499828836364));
#154897=CARTESIAN_POINT('Ctrl Pts',(7.22709476672504,4.69707706864331,0.974033096195835));
#154898=CARTESIAN_POINT('Ctrl Pts',(7.26922914014701,4.70392124752637,0.979552879507885));
#154899=CARTESIAN_POINT('Ctrl Pts',(7.35768749876934,4.71792585994092,0.991100604633074));
#154900=CARTESIAN_POINT('Ctrl Pts',(7.40407655527288,4.72506040968585,0.997132997816654));
#154901=CARTESIAN_POINT('Ctrl Pts',(7.45046320017597,4.73200281468412,1.00314378858579));
#154902=CARTESIAN_POINT('Origin',(9.94430232603705E-13,4.9390743,9.72800399262619E-14));
#154903=CARTESIAN_POINT('',(7.24739694618749,4.93794662020714,0.970238183641761));
#154904=CARTESIAN_POINT('Ctrl Pts',(7.24739694729143,4.93794661905671,0.970238184238935));
#154905=CARTESIAN_POINT('Ctrl Pts',(7.28073710674728,4.91814186433868,0.870452432924917));
#154906=CARTESIAN_POINT('Ctrl Pts',(7.31195134176256,4.89834552778171,0.769980750653622));
#154907=CARTESIAN_POINT('Ctrl Pts',(7.35550000134278,4.86872423018959,0.618468858201964));
#154908=CARTESIAN_POINT('Ctrl Pts',(7.36944786817102,4.85888055785931,0.567923823437499));
#154909=CARTESIAN_POINT('Ctrl Pts',(7.39756443723973,4.83826147072286,0.461627830901946));
#154910=CARTESIAN_POINT('Ctrl Pts',(7.41046418140696,4.82833849622491,0.41023002688005));
#154911=CARTESIAN_POINT('Ctrl Pts',(7.4217014669009,4.81939092009302,0.363728792642376));
#154912=CARTESIAN_POINT('',(7.25539727428587,4.81939091962013,1.60410776566287));
#154913=CARTESIAN_POINT('Ctrl Pts',(7.25539727225668,4.81939091984757,1.6041077656361));
#154914=CARTESIAN_POINT('Ctrl Pts',(7.25705256066902,4.82837891800305,1.55498633038954));
#154915=CARTESIAN_POINT('Ctrl Pts',(7.25832668383295,4.83808522200181,1.50210879657953));
#154916=CARTESIAN_POINT('Ctrl Pts',(7.25948173003012,4.85839508137762,1.39227434661416));
#154917=CARTESIAN_POINT('Ctrl Pts',(7.25942551431641,4.86818863450141,1.33961024775736));
#154918=CARTESIAN_POINT('Ctrl Pts',(7.25742400178274,4.89780104726198,1.18127360416032));
#154919=CARTESIAN_POINT('Ctrl Pts',(7.2536330114369,4.9177754105084,1.07567386289559));
#154920=CARTESIAN_POINT('Ctrl Pts',(7.24739694504265,4.93794662132742,0.9702381839238));
#154921=CARTESIAN_POINT('Ctrl Pts',(7.45070924183244,4.73205099316992,1.00323928500142));
#154922=CARTESIAN_POINT('Ctrl Pts',(7.4222980389261,4.74662633124793,1.10501656302923));
#154923=CARTESIAN_POINT('Ctrl Pts',(7.39174628626538,4.76121922807228,1.20618241809027));
#154924=CARTESIAN_POINT('Ctrl Pts',(7.32659738124921,4.79033919874295,1.40652988402164));
#154925=CARTESIAN_POINT('Ctrl Pts',(7.29203335377851,4.80486306086565,1.50569886250131));
#154926=CARTESIAN_POINT('Ctrl Pts',(7.2553972724486,4.81939092103895,1.60410775924929));
#154927=CARTESIAN_POINT('Ctrl Pts',(7.35945336807604,4.819390921,1.54119659248567));
#154928=CARTESIAN_POINT('Ctrl Pts',(7.44296827404257,4.754503495,1.14239993157747));
#154929=CARTESIAN_POINT('Ctrl Pts',(7.48290042445847,4.689276009,0.736913879334189));
#154930=CARTESIAN_POINT('Ctrl Pts',(7.337087236,4.819390921,1.554718909));
#154931=CARTESIAN_POINT('Ctrl Pts',(7.421334894,4.754503495,1.157134232));
#154932=CARTESIAN_POINT('Ctrl Pts',(7.462126472,4.689276009,0.752773886));
#154933=CARTESIAN_POINT('Ctrl Pts',(7.039414425,4.819390921,1.734688604));
#154934=CARTESIAN_POINT('Ctrl Pts',(7.133414344,4.754503495,1.353234327));
#154935=CARTESIAN_POINT('Ctrl Pts',(7.185644119,4.689276009,0.963856104));
#154936=CARTESIAN_POINT('',(7.14805379311779,4.81939091791745,1.6690064577682));
#154937=CARTESIAN_POINT('Ctrl Pts',(6.9645133045181,4.689268254,2.83423392936511));
#154938=CARTESIAN_POINT('Ctrl Pts',(7.12011852097099,4.754934719,2.45186796138366));
#154939=CARTESIAN_POINT('Ctrl Pts',(7.23292932676832,4.819390921,2.05476540792949));
#154940=CARTESIAN_POINT('Ctrl Pts',(6.953502166,4.689268254,2.810481743));
#154941=CARTESIAN_POINT('Ctrl Pts',(7.107803339,4.754934719,2.428720309));
#154942=CARTESIAN_POINT('Ctrl Pts',(7.21938412,4.819390921,2.032361415));
#154943=CARTESIAN_POINT('Ctrl Pts',(6.807201613,4.689268254,2.49489603));
#154944=CARTESIAN_POINT('Ctrl Pts',(6.94417648700001,4.754934719,2.121166795));
#154945=CARTESIAN_POINT('Ctrl Pts',(7.039414425,4.819390921,1.734688604));
#154946=CARTESIAN_POINT('',(7.16999527406823,4.81939091970922,1.95067144827473));
#154947=CARTESIAN_POINT('',(7.10443977264433,4.81939091820872,1.8422415662143));
#154948=CARTESIAN_POINT('',(7.06074993823213,4.73201982385919,2.58138433013341));
#154949=CARTESIAN_POINT('Ctrl Pts',(7.16999526991829,4.81939092084721,1.95067145274065));
#154950=CARTESIAN_POINT('Ctrl Pts',(7.15628763084189,4.80491309538955,2.05620576419138));
#154951=CARTESIAN_POINT('Ctrl Pts',(7.14036181216804,4.79041128722461,2.16143708857166));
#154952=CARTESIAN_POINT('Ctrl Pts',(7.10399783077811,4.76128647693571,2.3717691141358));
#154953=CARTESIAN_POINT('Ctrl Pts',(7.08353774277662,4.74666639456533,2.47684282010996));
#154954=CARTESIAN_POINT('Ctrl Pts',(7.0608706273649,4.73203683303586,2.58144846228725));
#154955=CARTESIAN_POINT('Ctrl Pts',(6.80883909823081,4.69005394741873,2.49042368960527));
#154956=CARTESIAN_POINT('Ctrl Pts',(6.84874098442337,4.69707706872806,2.50487248769431));
#154957=CARTESIAN_POINT('Ctrl Pts',(6.88870368909124,4.70392124757714,2.51932086608864));
#154958=CARTESIAN_POINT('Ctrl Pts',(6.97261152078471,4.71792585998271,2.54961454381537));
#154959=CARTESIAN_POINT('Ctrl Pts',(7.01661924063605,4.72506040971095,2.56547817877681));
#154960=CARTESIAN_POINT('Ctrl Pts',(7.06062924909937,4.73200281468252,2.58132019797957));
#154961=CARTESIAN_POINT('Origin',(1.04300248993106E-12,4.93907430000018,
3.03468188078693E-13));
#154962=CARTESIAN_POINT('',(6.86938430310311,4.93794662027974,2.50553066717595));
#154963=CARTESIAN_POINT('Ctrl Pts',(6.86938430382193,4.93794661939022,2.50553066780109));
#154964=CARTESIAN_POINT('Ctrl Pts',(6.92339597581209,4.91814186465082,2.41524500063482));
#154965=CARTESIAN_POINT('Ctrl Pts',(6.97547888113087,4.89834552808515,2.32383242836538));
#154966=CARTESIAN_POINT('Ctrl Pts',(7.05057997558024,4.86872423042573,2.18522447423273));
#154967=CARTESIAN_POINT('Ctrl Pts',(7.07506743745908,4.8588805580645,2.13885953332533));
#154968=CARTESIAN_POINT('Ctrl Pts',(7.12537715336372,4.83826147078332,2.04109291284144));
#154969=CARTESIAN_POINT('Ctrl Pts',(7.14902431737564,4.82833849620866,1.99366982439162));
#154970=CARTESIAN_POINT('Ctrl Pts',(7.16999527224034,4.81939092003057,1.95067144731637));
#154971=CARTESIAN_POINT('',(6.74093436535114,4.81939091956886,3.12630056326878));
#154972=CARTESIAN_POINT('Ctrl Pts',(6.74093436364107,4.81939091970027,3.1263005628563));
#154973=CARTESIAN_POINT('Ctrl Pts',(6.75311058856627,4.82837890461987,3.07868347282228));
#154974=CARTESIAN_POINT('Ctrl Pts',(6.76572202560481,4.83808520173977,3.02731611672858));
#154975=CARTESIAN_POINT('Ctrl Pts',(6.79046125202133,4.85839508123233,2.92029772999924));
#154976=CARTESIAN_POINT('Ctrl Pts',(6.80172757514065,4.86818863438586,2.86885280366468));
#154977=CARTESIAN_POINT('Ctrl Pts',(6.83381121865547,4.8978016598734,2.71378450832141));
#154978=CARTESIAN_POINT('Ctrl Pts',(6.85280850453319,4.91777478484511,2.60984512293696));
#154979=CARTESIAN_POINT('Ctrl Pts',(6.86938430221194,4.93794662111043,2.50553066719498));
#154980=CARTESIAN_POINT('Ctrl Pts',(7.06084900952567,4.73205099317129,2.58146635344278));
#154981=CARTESIAN_POINT('Ctrl Pts',(7.01122293851196,4.74662633122357,2.67475656650648));
#154982=CARTESIAN_POINT('Ctrl Pts',(6.95963780046243,4.76121922803318,2.76698949640077));
#154983=CARTESIAN_POINT('Ctrl Pts',(6.85294325765045,4.79033919870283,2.94864786124386));
#154984=CARTESIAN_POINT('Ctrl Pts',(6.79786891886765,4.80486306085235,3.03806808008998));
#154985=CARTESIAN_POINT('Ctrl Pts',(6.74093436486265,4.81939092103708,3.12630055704499));
#154986=CARTESIAN_POINT('Ctrl Pts',(6.85608172884453,4.819390921,3.08722920296354));
#154987=CARTESIAN_POINT('Ctrl Pts',(7.0233735958105,4.754503495,2.71570942253431));
#154988=CARTESIAN_POINT('Ctrl Pts',(7.14953966970884,4.689276009,2.32828764003355));
#154989=CARTESIAN_POINT('Ctrl Pts',(6.831331606,4.819390921,3.095627318));
#154990=CARTESIAN_POINT('Ctrl Pts',(6.999078553,4.754503495,2.725448706));
#154991=CARTESIAN_POINT('Ctrl Pts',(7.12584196800001,4.689276009,2.339311063));
#154992=CARTESIAN_POINT('Ctrl Pts',(6.501930055,4.819390921,3.207398566));
#154993=CARTESIAN_POINT('Ctrl Pts',(6.675733702,4.754503495,2.855069682));
#154994=CARTESIAN_POINT('Ctrl Pts',(6.81044718200001,4.689276009,2.486022764));
#154995=CARTESIAN_POINT('',(6.62214921468494,4.81939091791719,3.16660628438882));
#154996=CARTESIAN_POINT('Ctrl Pts',(6.19241033836026,4.689268254,4.26513560605128));
#154997=CARTESIAN_POINT('Ctrl Pts',(6.4265749708741,4.754934719,3.92515966456883));
#154998=CARTESIAN_POINT('Ctrl Pts',(6.62211363423336,4.819390921,3.56159213646275));
#154999=CARTESIAN_POINT('Ctrl Pts',(6.186762652,4.689268254,4.239571663));
#155000=CARTESIAN_POINT('Ctrl Pts',(6.419523772,4.754934719,3.899905791));
#155001=CARTESIAN_POINT('Ctrl Pts',(6.61370130300001,4.819390921,3.536800117));
#155002=CARTESIAN_POINT('Ctrl Pts',(6.111724124,4.689268254,3.899913875));
#155003=CARTESIAN_POINT('Ctrl Pts',(6.32583734,4.754934719,3.564367771));
#155004=CARTESIAN_POINT('Ctrl Pts',(6.501930055,4.819390921,3.207398566));
#155005=CARTESIAN_POINT('',(6.58302806924343,4.8193909197456,3.44640287397763));
#155006=CARTESIAN_POINT('',(6.542314438764,4.81939091820872,3.32641552756463));
#155007=CARTESIAN_POINT('',(6.3407522023859,4.73201982388303,4.03888552173727));
#155008=CARTESIAN_POINT('Ctrl Pts',(6.5830280640492,4.81939092085899,3.44640287763249));
#155009=CARTESIAN_POINT('Ctrl Pts',(6.54695414499058,4.80491309561722,3.54652311704798));
#155010=CARTESIAN_POINT('Ctrl Pts',(6.50877903958484,4.79041128768656,3.64587060988582));
#155011=CARTESIAN_POINT('Ctrl Pts',(6.42805005867109,4.76128647704054,3.8434680110759));
#155012=CARTESIAN_POINT('Ctrl Pts',(6.38548057524206,4.74666639463987,3.94168683827164));
#155013=CARTESIAN_POINT('Ctrl Pts',(6.34085628336632,4.7320368330631,4.03897409908925));
#155014=CARTESIAN_POINT('Ctrl Pts',(6.11428474712324,4.69005394750855,3.89589810638951));
#155015=CARTESIAN_POINT('Ctrl Pts',(6.15014768491915,4.69707706880471,3.91858682551975));
#155016=CARTESIAN_POINT('Ctrl Pts',(6.18607010944633,4.70392124763845,3.94128820901256));
#155017=CARTESIAN_POINT('Ctrl Pts',(6.26150397730438,4.71792586002178,3.98891134089339));
#155018=CARTESIAN_POINT('Ctrl Pts',(6.30107260842563,4.72506040973843,4.01386445183326));
#155019=CARTESIAN_POINT('Ctrl Pts',(6.34064812140549,4.73200281470297,4.03879694438529));
#155020=CARTESIAN_POINT('Origin',(1.01047642475649E-13,4.93907430000125,
1.22731685925359E-13));
#155021=CARTESIAN_POINT('',(6.17016688530534,4.93794662024516,3.92366731972341));
#155022=CARTESIAN_POINT('Ctrl Pts',(6.17016688596748,4.93794661920754,3.92366732061585));
#155023=CARTESIAN_POINT('Ctrl Pts',(6.24232454472163,4.91814186446448,3.84710339503515));
#155024=CARTESIAN_POINT('Ctrl Pts',(6.31284078157814,4.89834552790831,3.7690242829255));
#155025=CARTESIAN_POINT('Ctrl Pts',(6.41598266705498,4.86872423030126,3.64980142099868));
#155026=CARTESIAN_POINT('Ctrl Pts',(6.44986471740306,4.85888055796827,3.6097845471039));
#155027=CARTESIAN_POINT('Ctrl Pts',(6.52001515335497,4.83826147078904,3.52511875777889));
#155028=CARTESIAN_POINT('Ctrl Pts',(6.55330402191576,4.82833849627079,3.48388783610231));
#155029=CARTESIAN_POINT('Ctrl Pts',(6.58302806754595,4.81939092012227,3.44640287254168));
#155030=CARTESIAN_POINT('',(5.91127285763218,4.81939091960316,4.50231102143997));
#155031=CARTESIAN_POINT('Ctrl Pts',(5.91127285587575,4.81939091979814,4.5023110205943));
#155032=CARTESIAN_POINT('Ctrl Pts',(5.93340068110552,4.82837890717549,4.45842470701994));
#155033=CARTESIAN_POINT('Ctrl Pts',(5.9567597358703,4.83808520599485,4.4109693698699));
#155034=CARTESIAN_POINT('Ctrl Pts',(6.0039263530434,4.85839508132317,4.31177123615426));
#155035=CARTESIAN_POINT('Ctrl Pts',(6.02598841424333,4.86818863446027,4.26395099008268));
#155036=CARTESIAN_POINT('Ctrl Pts',(6.09065705974093,4.89780165993548,4.11940514025462));
#155037=CARTESIAN_POINT('Ctrl Pts',(6.13155409507273,4.91777478492038,4.02197965479997));
#155038=CARTESIAN_POINT('Ctrl Pts',(6.17016688427914,4.93794662122005,3.92366731952039));
#155039=CARTESIAN_POINT('Ctrl Pts',(6.34083132488251,4.73205099318433,4.03898692477078));
#155040=CARTESIAN_POINT('Ctrl Pts',(6.27231084572381,4.74662633121309,4.11942792610098));
#155041=CARTESIAN_POINT('Ctrl Pts',(6.20210438604712,4.7612192280144,4.19841522144427));
#155042=CARTESIAN_POINT('Ctrl Pts',(6.05885312475774,4.79033919848783,4.35289034064804));
#155043=CARTESIAN_POINT('Ctrl Pts',(5.98584368919382,4.80486306074136,4.42838061007477));
#155044=CARTESIAN_POINT('Ctrl Pts',(5.91127285856016,4.81939092103213,4.50231101503326));
#155045=CARTESIAN_POINT('Ctrl Pts',(6.03212732728657,4.819390921,4.48890640701289));
#155046=CARTESIAN_POINT('Ctrl Pts',(6.27537377440064,4.754503495,4.16203535965215));
#155047=CARTESIAN_POINT('Ctrl Pts',(6.48187438570106,4.689276009,3.81079325888398));
#155048=CARTESIAN_POINT('Ctrl Pts',(6.006150502,4.819390921,4.491787634));
#155049=CARTESIAN_POINT('Ctrl Pts',(6.249553078,4.754503495,4.166324228));
#155050=CARTESIAN_POINT('Ctrl Pts',(6.456361013,4.689276009,3.816464655));
#155051=CARTESIAN_POINT('Ctrl Pts',(5.660422662,4.819390921,4.530134136));
#155052=CARTESIAN_POINT('Ctrl Pts',(5.905903171,4.754503495,4.223405152));
#155053=CARTESIAN_POINT('Ctrl Pts',(6.116801304,4.689276009,3.891945762));
#155054=CARTESIAN_POINT('',(5.7866002991413,4.81939091791719,4.51613912119474));
#155055=CARTESIAN_POINT('Ctrl Pts',(5.13075714752225,4.689268254,5.49660428171978));
#155056=CARTESIAN_POINT('Ctrl Pts',(5.43253191840415,4.754934719,5.21491526319109));
#155057=CARTESIAN_POINT('Ctrl Pts',(5.70165526825467,4.819390921,4.90188277526916));
#155058=CARTESIAN_POINT('Ctrl Pts',(5.130736993,4.689268254,5.47042392400001));
#155059=CARTESIAN_POINT('Ctrl Pts',(5.431074409,4.754934719,5.188736012));
#155060=CARTESIAN_POINT('Ctrl Pts',(5.698769164,4.819390921,4.875861977));
#155061=CARTESIAN_POINT('Ctrl Pts',(5.130469208,4.689268254,5.12257608100001));
#155062=CARTESIAN_POINT('Ctrl Pts',(5.41170907,4.754934719,4.840902871));
#155063=CARTESIAN_POINT('Ctrl Pts',(5.660422662,4.819390921,4.530134136));
#155064=CARTESIAN_POINT('',(5.68824578838242,4.81939091971947,4.78098433171713));
#155065=CARTESIAN_POINT('',(5.67427775255105,4.81939091820873,4.6550499957781));
#155066=CARTESIAN_POINT('',(5.32426794103522,4.73201982384579,5.30753291487205));
#155067=CARTESIAN_POINT('Ctrl Pts',(5.68824578258985,4.81939092086497,4.78098433419026));
#155068=CARTESIAN_POINT('Ctrl Pts',(5.63149236024124,4.80491309574013,4.87100899105073));
#155069=CARTESIAN_POINT('Ctrl Pts',(5.5728529938489,4.79041128793007,4.95982727479803));
#155070=CARTESIAN_POINT('Ctrl Pts',(5.45153381034727,4.76128647704277,5.1354506154349));
#155071=CARTESIAN_POINT('Ctrl Pts',(5.38884543321955,4.74666639462687,5.22222196051445));
#155072=CARTESIAN_POINT('Ctrl Pts',(5.32435054716052,4.7320368330288,5.30764179564587));
#155073=CARTESIAN_POINT('Ctrl Pts',(5.13383323629967,4.69005394740914,5.11920465603329));
#155074=CARTESIAN_POINT('Ctrl Pts',(5.16398031443929,4.69707706865119,5.14907239726348));
#155075=CARTESIAN_POINT('Ctrl Pts',(5.19418276648921,4.70392124753492,5.17896529492946));
#155076=CARTESIAN_POINT('Ctrl Pts',(5.25761546681946,4.71792585991741,5.24169107654769));
#155077=CARTESIAN_POINT('Ctrl Pts',(5.29089482417904,4.72506040965878,5.274566883803));
#155078=CARTESIAN_POINT('Ctrl Pts',(5.32418533490993,4.73200281466277,5.30742403409823));
#155079=CARTESIAN_POINT('Origin',(-4.33680868994202E-13,4.93907430000142,
-5.08707659330199E-13));
#155080=CARTESIAN_POINT('',(5.18243932173717,4.93794662023057,5.15833764936207));
#155081=CARTESIAN_POINT('Ctrl Pts',(5.18243932225554,4.93794661907332,5.15833765050919));
#155082=CARTESIAN_POINT('Ctrl Pts',(5.26936895578191,4.91814186434841,5.09907551064492));
#155083=CARTESIAN_POINT('Ctrl Pts',(5.35502126333883,4.89834552778627,5.03798075123464));
#155084=CARTESIAN_POINT('Ctrl Pts',(5.48138113989073,4.86872423019759,4.94371771012989));
#155085=CARTESIAN_POINT('Ctrl Pts',(5.52307349170308,4.85888055787091,4.91192004780149));
#155086=CARTESIAN_POINT('Ctrl Pts',(5.60978449120292,4.83826147075238,4.84431396785914));
#155087=CARTESIAN_POINT('Ctrl Pts',(5.65115851388493,4.8283384962394,4.81120312496045));
#155088=CARTESIAN_POINT('Ctrl Pts',(5.6882457871148,4.81939092005774,4.78098433006123));
#155089=CARTESIAN_POINT('',(4.80520680109334,4.81939091959657,5.66779841993978));
#155090=CARTESIAN_POINT('Ctrl Pts',(4.80520679962465,4.81939091977378,5.66779841878496));
#155091=CARTESIAN_POINT('Ctrl Pts',(4.83625148209303,4.82837888943184,5.62969505090097));
#155092=CARTESIAN_POINT('Ctrl Pts',(4.86926588559444,4.83808517869205,5.58837073655554));
#155093=CARTESIAN_POINT('Ctrl Pts',(4.93665453039515,4.8583950812876,5.50163111211332));
#155094=CARTESIAN_POINT('Ctrl Pts',(4.96848073234918,4.86818863446822,5.45967156764961));
#155095=CARTESIAN_POINT('Ctrl Pts',(5.06270859626848,4.89780104727634,5.3324095996632));
#155096=CARTESIAN_POINT('Ctrl Pts',(5.12359685564863,4.91777541052763,5.24604816832737));
#155097=CARTESIAN_POINT('Ctrl Pts',(5.18243932064061,4.93794662136248,5.15833764888674));
#155098=CARTESIAN_POINT('Ctrl Pts',(5.32432341505984,4.73205099313603,5.3076489561436));
#155099=CARTESIAN_POINT('Ctrl Pts',(5.2401124691097,4.74662633120553,5.3714794139907));
#155100=CARTESIAN_POINT('Ctrl Pts',(5.15456746375139,4.76121922803258,5.43352771672791));
#155101=CARTESIAN_POINT('Ctrl Pts',(4.98145774809673,4.79033919935161,5.55359651013127));
#155102=CARTESIAN_POINT('Ctrl Pts',(4.89392705868379,4.80486306117032,5.61162698657165));
#155103=CARTESIAN_POINT('Ctrl Pts',(4.80520680348237,4.81939092105607,5.66779841383323));
#155104=CARTESIAN_POINT('Ctrl Pts',(4.92611735566809,4.819390921,5.68068733594333));
#155105=CARTESIAN_POINT('Ctrl Pts',(5.23394444927887,4.754503495,5.41374914837397));
#155106=CARTESIAN_POINT('Ctrl Pts',(5.51112386023993,4.689276009,5.11511042105134));
#155107=CARTESIAN_POINT('Ctrl Pts',(4.900128476,4.819390921,5.677916952));
#155108=CARTESIAN_POINT('Ctrl Pts',(5.207805447,4.754503495,5.412387059));
#155109=CARTESIAN_POINT('Ctrl Pts',(5.48498779400001,4.689276009,5.115164602));
#155110=CARTESIAN_POINT('Ctrl Pts',(4.554240196,4.819390921,5.641045669));
#155111=CARTESIAN_POINT('Ctrl Pts',(4.859919172,4.754503495,5.394258892));
#155112=CARTESIAN_POINT('Ctrl Pts',(5.13714059500001,4.689276009,5.11588570100001));
#155113=CARTESIAN_POINT('',(4.68047638465216,4.8193909179172,5.65450231179019));
#155114=CARTESIAN_POINT('Ctrl Pts',(3.82919545430357,4.689268254,6.47105785099436));
#155115=CARTESIAN_POINT('Ctrl Pts',(4.18446971154184,4.754934719,6.26082722012167));
#155116=CARTESIAN_POINT('Ctrl Pts',(4.51459383830672,4.819390921,6.01296682235049));
#155117=CARTESIAN_POINT('Ctrl Pts',(3.834803774,4.689268254,6.44548524300001));
#155118=CARTESIAN_POINT('Ctrl Pts',(4.188674043,4.754934719,6.234946704));
#155119=CARTESIAN_POINT('Ctrl Pts',(4.517368912,4.819390921,5.98693394900001));
#155120=CARTESIAN_POINT('Ctrl Pts',(3.909319254,4.689268254,6.105712323));
#155121=CARTESIAN_POINT('Ctrl Pts',(4.244535298,4.754934719,5.891082733));
#155122=CARTESIAN_POINT('Ctrl Pts',(4.554240196,4.819390921,5.64104566900001));
#155123=CARTESIAN_POINT('',(4.5274874560285,4.81939091970524,5.89201227629259));
#155124=CARTESIAN_POINT('',(4.54091814475076,4.81939091820872,5.76601949987998));
#155125=CARTESIAN_POINT('',(4.0588268284519,4.73201982389532,6.32800596761535));
#155126=CARTESIAN_POINT('Ctrl Pts',(4.52748745002682,4.8193909208755,5.89201227736476));
#155127=CARTESIAN_POINT('Ctrl Pts',(4.45270825217731,4.80491309595357,5.96773189845441));
#155128=CARTESIAN_POINT('Ctrl Pts',(4.37634653726941,4.79041128835246,6.04186792862038));
#155129=CARTESIAN_POINT('Ctrl Pts',(4.22010990001682,4.76128647707316,6.18730525675326));
#155130=CARTESIAN_POINT('Ctrl Pts',(4.14023386809453,4.74666639465908,6.2585717879563));
#155131=CARTESIAN_POINT('Ctrl Pts',(4.05888409709935,4.7320368330706,6.3281300607384));
#155132=CARTESIAN_POINT('Ctrl Pts',(3.91332938999963,4.69005394748938,6.10314288784437));
#155133=CARTESIAN_POINT('Ctrl Pts',(3.93635096493821,4.69707706879331,6.13879306848366));
#155134=CARTESIAN_POINT('Ctrl Pts',(3.95942121082128,4.70392124759608,6.17447972053153));
#155135=CARTESIAN_POINT('Ctrl Pts',(4.00788670113755,4.71792586001038,6.24937516349814));
#155136=CARTESIAN_POINT('Ctrl Pts',(4.03332067884046,4.72506040973901,6.28863643055456));
#155137=CARTESIAN_POINT('Ctrl Pts',(4.05876955980445,4.73200281472003,6.3278818744923));
#155138=CARTESIAN_POINT('Origin',(1.51571463713474E-13,4.93907430000036,
2.61509564003504E-13));
#155139=CARTESIAN_POINT('',(3.95238665404255,4.93794662023081,6.15180984471564));
#155140=CARTESIAN_POINT('Ctrl Pts',(3.95238665422766,4.93794661938177,6.15180984560589));
#155141=CARTESIAN_POINT('Ctrl Pts',(4.05002352969431,4.91814186458453,6.11262052322142));
#155142=CARTESIAN_POINT('Ctrl Pts',(4.14680690131411,4.89834552798455,6.07136683959648));
#155143=CARTESIAN_POINT('Ctrl Pts',(4.29047632194858,4.86872423028554,6.00647125421571));
#155144=CARTESIAN_POINT('Ctrl Pts',(4.33802948738522,4.85888055790745,5.98437962672833));
#155145=CARTESIAN_POINT('Ctrl Pts',(4.43724654087929,4.83826147070269,5.93699444105603));
#155146=CARTESIAN_POINT('Ctrl Pts',(4.48477111437587,4.82833849616324,5.91355190316687));
#155147=CARTESIAN_POINT('Ctrl Pts',(4.52748745518786,4.81939092000006,5.89201227450301));
#155148=CARTESIAN_POINT('',(3.4744546152313,4.81939091970674,6.56826586411545));
#155149=CARTESIAN_POINT('Ctrl Pts',(3.47445461370284,4.81939091997752,6.56826586226773));
#155150=CARTESIAN_POINT('Ctrl Pts',(3.51296474936782,4.82837892459898,6.537726893308));
#155151=CARTESIAN_POINT('Ctrl Pts',(3.55409086076293,4.83808523213118,6.504465780003));
#155152=CARTESIAN_POINT('Ctrl Pts',(3.63855022943076,4.85839508128673,6.43424083121638));
#155153=CARTESIAN_POINT('Ctrl Pts',(3.67865241365108,4.86818863433627,6.40010397069764));
#155154=CARTESIAN_POINT('Ctrl Pts',(3.79803731333291,4.89780165972223,6.29607137019479));
#155155=CARTESIAN_POINT('Ctrl Pts',(3.8760623568951,4.91777478470677,6.22482261377889));
#155156=CARTESIAN_POINT('Ctrl Pts',(3.95238665336921,4.93794662100664,6.1518098442261));
#155157=CARTESIAN_POINT('Ctrl Pts',(4.05885606001792,4.73205099321256,6.32813122119888));
#155158=CARTESIAN_POINT('Ctrl Pts',(3.96289225747811,4.74662633126892,6.37236649436752));
#155159=CARTESIAN_POINT('Ctrl Pts',(3.86600869576448,4.76121922808055,6.41457449488229));
#155160=CARTESIAN_POINT('Ctrl Pts',(3.67113495261786,4.79033919859532,6.49462267289275));
#155161=CARTESIAN_POINT('Ctrl Pts',(3.5731758422539,4.80486306079332,6.53247991950132));
#155162=CARTESIAN_POINT('Ctrl Pts',(3.47445461813372,4.81939092103448,6.56826585872816));
#155163=CARTESIAN_POINT('Ctrl Pts',(3.58976761215825,4.819390921,6.60684564007593));
#155164=CARTESIAN_POINT('Ctrl Pts',(3.94778169971128,4.754503495,6.41232204349741));
#155165=CARTESIAN_POINT('Ctrl Pts',(4.2826793086101,4.689276009,6.18025070349683));
#155166=CARTESIAN_POINT('Ctrl Pts',(3.564981888,4.819390921,6.598553185));
#155167=CARTESIAN_POINT('Ctrl Pts',(3.922546621,4.754503495,6.405372686));
#155168=CARTESIAN_POINT('Ctrl Pts',(4.257142641,4.689276009,6.174685136));
#155169=CARTESIAN_POINT('Ctrl Pts',(3.23510652,4.819390921,6.48818817600001));
#155170=CARTESIAN_POINT('Ctrl Pts',(3.586690754,4.754503495,6.31288308));
#155171=CARTESIAN_POINT('Ctrl Pts',(3.917272901,4.689276009,6.100612512));
#155172=CARTESIAN_POINT('',(3.35549859635726,4.8193909179172,6.52846725931102));
#155173=CARTESIAN_POINT('Ctrl Pts',(2.34858483786858,4.689268254,7.14293194666788));
#155174=CARTESIAN_POINT('Ctrl Pts',(2.74074635153136,4.754934719,7.01398985508504));
#155175=CARTESIAN_POINT('Ctrl Pts',(3.11643501878727,4.819390921,6.84289122444231));
#155176=CARTESIAN_POINT('Ctrl Pts',(2.359559393,4.689268254,7.119162835));
#155177=CARTESIAN_POINT('Ctrl Pts',(2.750415934,4.754934719,6.98961821800001));
#155178=CARTESIAN_POINT('Ctrl Pts',(3.124741511,4.819390921,6.818063544));
#155179=CARTESIAN_POINT('Ctrl Pts',(2.505373877,4.689268254,6.803352243));
#155180=CARTESIAN_POINT('Ctrl Pts',(2.878891773,4.754934719,6.665802114));
#155181=CARTESIAN_POINT('Ctrl Pts',(3.23510652,4.819390921,6.488188176));
#155182=CARTESIAN_POINT('',(3.15502884264767,4.81939091970705,6.72753627497528));
#155183=CARTESIAN_POINT('',(3.19523025164699,4.81939091820872,6.60737634111682));
#155184=CARTESIAN_POINT('',(2.60359948408427,4.73201982384173,7.05258849478579));
#155185=CARTESIAN_POINT('Ctrl Pts',(3.15502883653014,4.81939092085369,6.72753627472605));
#155186=CARTESIAN_POINT('Ctrl Pts',(3.0657204519689,4.80491309551931,6.78541029771323));
#155187=CARTESIAN_POINT('Ctrl Pts',(2.9752069736963,4.79041128748405,6.84139755873418));
#155188=CARTESIAN_POINT('Ctrl Pts',(2.79135834054187,4.76128647696698,6.94984838141895));
#155189=CARTESIAN_POINT('Ctrl Pts',(2.69802956840313,4.74666639457685,7.0022777548983));
#155190=CARTESIAN_POINT('Ctrl Pts',(2.60362873745907,4.73203683301562,7.05272199775456));
#155191=CARTESIAN_POINT('Ctrl Pts',(2.50984261070199,4.69005394735047,6.80170493940382));
#155192=CARTESIAN_POINT('Ctrl Pts',(2.52466221878368,4.69707706866363,6.84147059689012));
#155193=CARTESIAN_POINT('Ctrl Pts',(2.5395215197407,4.70392124749718,6.88128233602919));
#155194=CARTESIAN_POINT('Ctrl Pts',(2.57075360727919,4.71792585993317,6.96484541325419));
#155195=CARTESIAN_POINT('Ctrl Pts',(2.587152940809,4.72506040967556,7.00865632725573));
#155196=CARTESIAN_POINT('Ctrl Pts',(2.60357023070946,4.73200281466784,7.05245499181701));
#155197=CARTESIAN_POINT('Origin',(2.7527893159407E-13,4.93907429999929,
6.93022028652734E-13));
#155198=CARTESIAN_POINT('',(2.5375247805209,4.93794662024614,6.85763024787807));
#155199=CARTESIAN_POINT('Ctrl Pts',(2.53751508663611,4.9379484691976,6.85763186342078));
#155200=CARTESIAN_POINT('Ctrl Pts',(2.64129381194683,4.91814371445961,6.84034780770094));
#155201=CARTESIAN_POINT('Ctrl Pts',(2.74469245836587,4.89834552797129,6.82086256179474));
#155202=CARTESIAN_POINT('Ctrl Pts',(2.89895360012165,4.86872423033738,6.78836887775632));
#155203=CARTESIAN_POINT('Ctrl Pts',(2.95014404579079,4.85888055797823,6.77701626516097));
#155204=CARTESIAN_POINT('Ctrl Pts',(3.0572278742593,4.83826147071546,6.75206765238496));
#155205=CARTESIAN_POINT('Ctrl Pts',(3.10868080240164,4.82833849616026,6.73938956646646));
#155206=CARTESIAN_POINT('Ctrl Pts',(3.15502884219955,4.81939092002354,6.72753627298416));
#155207=CARTESIAN_POINT('',(1.98124079272459,4.81939091960563,7.16160849615506));
#155208=CARTESIAN_POINT('Ctrl Pts',(1.98124079184273,4.81939091980114,7.16160849442862));
#155209=CARTESIAN_POINT('Ctrl Pts',(2.02541538625655,4.82837889211582,7.14006213131342));
#155210=CARTESIAN_POINT('Ctrl Pts',(2.07273008306626,4.83808518301028,7.11641958361174));
#155211=CARTESIAN_POINT('Ctrl Pts',(2.17031136292566,4.85839508131333,7.0659926007449));
#155212=CARTESIAN_POINT('Ctrl Pts',(2.21681439661171,4.86818863443092,7.04127462508136));
#155213=CARTESIAN_POINT('Ctrl Pts',(2.35577207790842,4.89780165988963,6.9653384732215));
#155214=CARTESIAN_POINT('Ctrl Pts',(2.44728931581958,4.91777478487672,6.91252855109724));
#155215=CARTESIAN_POINT('Ctrl Pts',(2.53752477986336,4.9379466211697,6.85763024713663));
#155216=CARTESIAN_POINT('Ctrl Pts',(2.60360110640195,4.73205099316428,7.05271710393411));
#155217=CARTESIAN_POINT('Ctrl Pts',(2.50037160818322,4.74662633122825,7.07528880007722));
#155218=CARTESIAN_POINT('Ctrl Pts',(2.39667965795009,4.76121922804818,7.09568289904169));
#155219=CARTESIAN_POINT('Ctrl Pts',(2.18915396030579,4.79033919892996,7.13196750112894));
#155220=CARTESIAN_POINT('Ctrl Pts',(2.08534689191287,4.80486306096256,7.14788135295602));
#155221=CARTESIAN_POINT('Ctrl Pts',(1.98124079742037,4.81939092104364,7.16160849159641));
#155222=CARTESIAN_POINT('Ctrl Pts',(2.08556432488194,4.819390921,7.22407518407912));
#155223=CARTESIAN_POINT('Ctrl Pts',(2.47702506393543,4.754503495,7.1110618872917));
#155224=CARTESIAN_POINT('Ctrl Pts',(2.85398143190021,4.689276009,6.95640933332439));
#155225=CARTESIAN_POINT('Ctrl Pts',(2.06314071,4.819390921,7.210648404));
#155226=CARTESIAN_POINT('Ctrl Pts',(2.453873874,4.754503495,7.098850206));
#155227=CARTESIAN_POINT('Ctrl Pts',(2.83023823,4.689276009,6.945484257));
#155228=CARTESIAN_POINT('Ctrl Pts',(1.764702859,4.819390921,7.031950214));
#155229=CARTESIAN_POINT('Ctrl Pts',(2.145752663,4.754503495,6.936323872));
#155230=CARTESIAN_POINT('Ctrl Pts',(2.51423788,4.689276009,6.800081461));
#155231=CARTESIAN_POINT('',(1.87253223753566,4.8193909179172,7.09651615128198));
#155232=CARTESIAN_POINT('Ctrl Pts',(0.758157004557344,4.689268254,7.48081048409299));
#155233=CARTESIAN_POINT('Ctrl Pts',(1.16886873855041,4.754934719,7.4391861192906));
#155234=CARTESIAN_POINT('Ctrl Pts',(1.57255516057675,4.819390921,7.35284963772685));
#155235=CARTESIAN_POINT('Ctrl Pts',(0.773984637,4.689268254,7.45995628600001));
#155236=CARTESIAN_POINT('Ctrl Pts',(1.183551433,4.754934719,7.417462952));
#155237=CARTESIAN_POINT('Ctrl Pts',(1.586004669,4.819390921,7.330388065));
#155238=CARTESIAN_POINT('Ctrl Pts',(0.984280001000001,4.689268254,7.182874973));
#155239=CARTESIAN_POINT('Ctrl Pts',(1.378634468,4.754934719,7.128835996));
#155240=CARTESIAN_POINT('Ctrl Pts',(1.764702859,4.819390921,7.03195021400001));
#155241=CARTESIAN_POINT('',(1.63504458650614,4.81939091971965,7.24848815472403));
#155242=CARTESIAN_POINT('',(1.70013694327804,4.81939091820872,7.13977960720693));
#155243=CARTESIAN_POINT('',(1.0266307218224,4.732019823845,7.44739982217204));
#155244=CARTESIAN_POINT('Ctrl Pts',(1.6350445805021,4.81939092087202,7.24848815316613));
#155245=CARTESIAN_POINT('Ctrl Pts',(1.53538297452666,4.80491309586785,7.28581045002857));
#155246=CARTESIAN_POINT('Ctrl Pts',(1.43495004754048,4.79041128818367,7.32103103698584));
#155247=CARTESIAN_POINT('Ctrl Pts',(1.2320859680399,4.76128647702923,7.38742431950823));
#155248=CARTESIAN_POINT('Ctrl Pts',(1.12966840519222,4.74666639460951,7.41856499618032));
#155249=CARTESIAN_POINT('Ctrl Pts',(1.02663059207865,4.73203683301885,7.44753649252512));
#155250=CARTESIAN_POINT('Ctrl Pts',(0.988998379597802,4.69005394744881,
7.18222682902306));
#155251=CARTESIAN_POINT('Ctrl Pts',(0.994923072737245,4.69707706871718,
7.22424856495182));
#155252=CARTESIAN_POINT('Ctrl Pts',(1.00087662460663,4.703921247592,7.26632383850002));
#155253=CARTESIAN_POINT('Ctrl Pts',(1.01341493203483,4.71792585996633,7.35464723268727));
#155254=CARTESIAN_POINT('Ctrl Pts',(1.02001280689968,4.72506040969293,7.40095924373872));
#155255=CARTESIAN_POINT('Ctrl Pts',(1.02663085156615,4.73200281467114,7.44726315181896));
#155256=CARTESIAN_POINT('Origin',(1.85940672581264E-14,4.93907429999982,
-2.15105711021124E-13));
#155257=CARTESIAN_POINT('',(1.0040110691062,4.93794662027172,7.2427954824852));
#155258=CARTESIAN_POINT('Ctrl Pts',(1.00401106883361,4.93794661914717,7.24279548365829));
#155259=CARTESIAN_POINT('Ctrl Pts',(1.10907906612687,4.91814186439149,7.24822487784654));
#155260=CARTESIAN_POINT('Ctrl Pts',(1.21423924707293,4.89834552782296,7.2514223315788));
#155261=CARTESIAN_POINT('Ctrl Pts',(1.37187903032445,4.86872423019335,7.252849917406));
#155262=CARTESIAN_POINT('Ctrl Pts',(1.42431314780498,4.85888055784907,7.25276715523505));
#155263=CARTESIAN_POINT('Ctrl Pts',(1.53425662938434,4.83826147072032,7.25142168492364));
#155264=CARTESIAN_POINT('Ctrl Pts',(1.58723203015921,4.82833849621078,7.25010086423123));
#155265=CARTESIAN_POINT('Ctrl Pts',(1.63504458649721,4.8193909200433,7.24848815266336));
#155266=CARTESIAN_POINT('',(0.395386352630777,4.81939091962198,7.42008227473765));
#155267=CARTESIAN_POINT('Ctrl Pts',(0.39538635210853,4.81939091985495,7.42008227275818));
#155268=CARTESIAN_POINT('Ctrl Pts',(0.443160188367102,4.82837892523183,
7.40853584051378));
#155269=CARTESIAN_POINT('Ctrl Pts',(0.494451219908121,4.83808523378702,
7.39561727616033));
#155270=CARTESIAN_POINT('Ctrl Pts',(0.600591149699864,4.85839508140899,
7.36734640934662));
#155271=CARTESIAN_POINT('Ctrl Pts',(0.651320602397542,4.86818863451005,
7.35320310385632));
#155272=CARTESIAN_POINT('Ctrl Pts',(0.803353558541045,4.89780165997746,
7.30891409091188));
#155273=CARTESIAN_POINT('Ctrl Pts',(0.904083746722127,4.91777478499841,
7.27701233627068));
#155274=CARTESIAN_POINT('Ctrl Pts',(1.00401106855046,4.93794662133483,7.24279548148896));
#155275=CARTESIAN_POINT('Ctrl Pts',(1.02660465904708,4.73205099316698,7.44752577325948));
#155276=CARTESIAN_POINT('Ctrl Pts',(0.920936361614114,4.74662633123541,
7.44737846502169));
#155277=CARTESIAN_POINT('Ctrl Pts',(0.81528454305873,4.76121922805836,7.44500505710333));
#155278=CARTESIAN_POINT('Ctrl Pts',(0.604810566195762,4.79033919861928,
7.43582945489426));
#155279=CARTESIAN_POINT('Ctrl Pts',(0.500009440448111,4.80486306080291,
7.42905579852791));
#155280=CARTESIAN_POINT('Ctrl Pts',(0.395386358326975,4.81939092103597,
7.42008227124413));
#155281=CARTESIAN_POINT('Ctrl Pts',(0.483842367355651,4.819390921,7.50351500170055));
#155282=CARTESIAN_POINT('Ctrl Pts',(0.890445490471756,4.754503495,7.47729638044081));
#155283=CARTESIAN_POINT('Ctrl Pts',(1.29183455551508,4.689276009,7.40729399359796));
#155284=CARTESIAN_POINT('Ctrl Pts',(0.464829365,4.819390921,7.485581718));
#155285=CARTESIAN_POINT('Ctrl Pts',(0.870460713,4.754503495,7.46039338));
#155286=CARTESIAN_POINT('Ctrl Pts',(1.270995025,4.689276009,7.391520253));
#155287=CARTESIAN_POINT('Ctrl Pts',(0.211783654,4.819390921,7.246906077));
#155288=CARTESIAN_POINT('Ctrl Pts',(0.604481562,4.754503495,7.23542986900001));
#155289=CARTESIAN_POINT('Ctrl Pts',(0.993639891,4.689276009,7.18158616));
#155290=CARTESIAN_POINT('',(0.304135795242029,4.8193909179172,7.33401370379861));
#155291=CARTESIAN_POINT('Origin',(7.74696333558783E-14,4.93907430000071,
1.65666091955785E-13));
#155292=CARTESIAN_POINT('',(0.0386074640004457,4.81939091973237,7.43050878427183));
#155293=CARTESIAN_POINT('Ctrl Pts',(0.0386074583560088,4.81939092087357,
7.43050878143317));
#155294=CARTESIAN_POINT('Ctrl Pts',(-0.0667473027758887,4.80491309622522,
7.44553420406776));
#155295=CARTESIAN_POINT('Ctrl Pts',(-0.172403546298225,4.79041128890658,
7.45834124249127));
#155296=CARTESIAN_POINT('Ctrl Pts',(-0.384797367802654,4.76128647803856,
7.47957250648728));
#155297=CARTESIAN_POINT('Ctrl Pts',(-0.491514790303439,4.74666639559778,
7.4879683829733));
#155298=CARTESIAN_POINT('Ctrl Pts',(-0.598371652318673,4.73203683399558,
7.49411245786321));
#155299=CARTESIAN_POINT('',(-0.576449089007819,4.93794662013209,7.28929565003906));
#155300=CARTESIAN_POINT('Ctrl Pts',(-0.576449089233835,4.93794661980761,
7.28929565063075));
#155301=CARTESIAN_POINT('Ctrl Pts',(-0.47500468183286,4.91814186494119,
7.317184622455));
#155302=CARTESIAN_POINT('Ctrl Pts',(-0.372990444739158,4.89834552828498,
7.34291365205627));
#155303=CARTESIAN_POINT('Ctrl Pts',(-0.219342958828865,4.86872420722662,
7.37819578327224));
#155304=CARTESIAN_POINT('Ctrl Pts',(-0.168116808705067,4.8588805115865,
7.3893867665824));
#155305=CARTESIAN_POINT('Ctrl Pts',(-0.0604545170709904,4.83826142650624,
7.41170734373942));
#155306=CARTESIAN_POINT('Ctrl Pts',(-0.00843383585907548,4.8283384752577,
7.421805523601));
#155307=CARTESIAN_POINT('Ctrl Pts',(0.0386074644507542,4.8193909200799,
7.43050878219518));
#155308=CARTESIAN_POINT('Ctrl Pts',(-1.20895591300036,4.81939091996494,
7.33160125079922));
#155309=CARTESIAN_POINT('Ctrl Pts',(-1.15981566191495,4.82837914487869,
7.33059470553182));
#155310=CARTESIAN_POINT('Ctrl Pts',(-1.1069453862108,4.83808569120533,7.32900417473453));
#155311=CARTESIAN_POINT('Ctrl Pts',(-0.997209430183357,4.8583955671125,
7.32421114410252));
#155312=CARTESIAN_POINT('Ctrl Pts',(-0.944626917499339,4.86818887849713,
7.32130389107535));
#155313=CARTESIAN_POINT('Ctrl Pts',(-0.786632152526621,4.89780104677615,
7.31073322814866));
#155314=CARTESIAN_POINT('Ctrl Pts',(-0.681392523108954,4.91777540990695,
7.30123074296795));
#155315=CARTESIAN_POINT('Ctrl Pts',(-0.576449089121962,4.93794662060687,
7.28929564983784));
#155316=CARTESIAN_POINT('Ctrl Pts',(-0.867721406319706,4.689268254,7.46889463457454));
#155317=CARTESIAN_POINT('Ctrl Pts',(-0.457663876072064,4.754934719,7.51653430751444));
#155318=CARTESIAN_POINT('Ctrl Pts',(-0.0448556267016637,4.819390921,7.51899697287651));
#155319=CARTESIAN_POINT('Ctrl Pts',(-0.847780781,4.689268254,7.451930471));
#155320=CARTESIAN_POINT('Ctrl Pts',(-0.438654618,4.754934719,7.498475363));
#155321=CARTESIAN_POINT('Ctrl Pts',(-0.026891988,4.819390921,7.499951788));
#155322=CARTESIAN_POINT('Ctrl Pts',(-0.582837713,4.689268254,7.226534453));
#155323=CARTESIAN_POINT('Ctrl Pts',(-0.186086252,4.754934719,7.258533431));
#155324=CARTESIAN_POINT('Ctrl Pts',(0.211783654,4.819390921,7.246906077));
#155325=CARTESIAN_POINT('',(0.124676045108029,4.81939091820872,7.33925823720938));
#155326=CARTESIAN_POINT('Ctrl Pts',(-0.037115645,0.939268254,7.499908161));
#155327=CARTESIAN_POINT('Ctrl Pts',(0.37464459,1.004934719,7.501945886));
#155328=CARTESIAN_POINT('Ctrl Pts',(0.78415308,1.069390921,7.458894285));
#155329=CARTESIAN_POINT('Ctrl Pts',(0.201904718,0.939268254,7.24718804));
#155330=CARTESIAN_POINT('Ctrl Pts',(0.599790104,1.004934719,7.23610306));
#155331=CARTESIAN_POINT('Ctrl Pts',(0.994070541000001,1.069390921,7.18152656200001));
#155332=CARTESIAN_POINT('',(0.206665520798754,0.940053947693287,7.24705384020318));
#155333=CARTESIAN_POINT('Origin',(0.0171543106145804,0.803719061399266,
-0.190604237663627));
#155334=CARTESIAN_POINT('Ctrl Pts',(0.20666551447053,0.940053947354557,
7.24705384080662));
#155335=CARTESIAN_POINT('Ctrl Pts',(0.20798572187948,0.946939351516512,
7.28863807645421));
#155336=CARTESIAN_POINT('Ctrl Pts',(0.209327926431948,0.953652683633494,
7.33027599541269));
#155337=CARTESIAN_POINT('Ctrl Pts',(0.212049360335663,0.96674613250779,
7.41355144745307));
#155338=CARTESIAN_POINT('Ctrl Pts',(0.213430188150455,0.973133921158012,
7.45523782159286));
#155339=CARTESIAN_POINT('Ctrl Pts',(0.214827964027396,0.979367659147288,
7.49692263175492));
#155340=CARTESIAN_POINT('Ctrl Pts',(1.271438263,1.069390921,7.391444023));
#155341=CARTESIAN_POINT('Ctrl Pts',(1.671968444,1.004503495,7.32254687700001));
#155342=CARTESIAN_POINT('Ctrl Pts',(2.062708312,0.939276009000001,7.21077211));
#155343=CARTESIAN_POINT('Ctrl Pts',(0.994070541,1.069390921,7.181526562));
#155344=CARTESIAN_POINT('Ctrl Pts',(1.38322564,1.004503495,7.127659516));
#155345=CARTESIAN_POINT('Ctrl Pts',(1.764281177,0.939276009000001,7.03205602400001));
#155346=CARTESIAN_POINT('',(1.75973614927377,0.940053948104567,7.03319478739377));
#155347=CARTESIAN_POINT('Origin',(-0.0472960242995052,0.946431379382763,
-0.193309116276293));
#155348=CARTESIAN_POINT('Ctrl Pts',(1.82142216389955,0.979367659138093,
7.27546708476632));
#155349=CARTESIAN_POINT('Ctrl Pts',(1.81109607941231,0.973133929663875,
7.23505737799103));
#155350=CARTESIAN_POINT('Ctrl Pts',(1.80078618995315,0.966746137351372,
7.19464242018625));
#155351=CARTESIAN_POINT('Ctrl Pts',(1.7802265873758,0.953652667115658,7.11389879786013));
#155352=CARTESIAN_POINT('Ctrl Pts',(1.76996485896721,0.946939346100155,
7.07352295524683));
#155353=CARTESIAN_POINT('Ctrl Pts',(1.75973614734533,0.940053949831287,
7.03319478758808));
#155354=CARTESIAN_POINT('Ctrl Pts',(1.576010657,0.939268254,7.332543243));
#155355=CARTESIAN_POINT('Ctrl Pts',(1.978582217,1.004934719,7.246017048));
#155356=CARTESIAN_POINT('Ctrl Pts',(2.369261804,1.069390921,7.115939748));
#155357=CARTESIAN_POINT('Ctrl Pts',(1.755115501,0.939268254,7.034349265));
#155358=CARTESIAN_POINT('Ctrl Pts',(2.141315605,1.004934719,6.937989849));
#155359=CARTESIAN_POINT('Ctrl Pts',(2.51464565,1.069390921,6.79993068000001));
#155360=CARTESIAN_POINT('Origin',(-0.0242212355237648,0.803718937193291,
-0.189835864139434));
#155361=CARTESIAN_POINT('Ctrl Pts',(2.830654719,1.069390921,6.945314526));
#155362=CARTESIAN_POINT('Ctrl Pts',(3.207009877,1.004503495,6.79192600800001));
#155363=CARTESIAN_POINT('Ctrl Pts',(3.564586193,0.939276009000001,6.598766951));
#155364=CARTESIAN_POINT('Ctrl Pts',(2.51464565,1.069390921,6.79993068));
#155365=CARTESIAN_POINT('Ctrl Pts',(2.883122697,1.004503495,6.663666173));
#155366=CARTESIAN_POINT('Ctrl Pts',(3.234717443,0.939276009000001,6.488382161));
#155367=CARTESIAN_POINT('',(3.23052347474322,0.940053947055572,6.49047134645543));
#155368=CARTESIAN_POINT('Origin',(-0.0877460033529154,0.946431378272004,
-0.178622367929185));
#155369=CARTESIAN_POINT('Ctrl Pts',(3.34284868775709,0.979367659169516,
6.71381878287936));
#155370=CARTESIAN_POINT('Ctrl Pts',(3.32407710461605,0.973133921631213,
6.6765735873877));
#155371=CARTESIAN_POINT('Ctrl Pts',(3.30532024644803,0.966746133471279,
6.6393198563039));
#155372=CARTESIAN_POINT('Ctrl Pts',(3.26788383502628,0.953652667121443,
6.56488370404856));
#155373=CARTESIAN_POINT('Ctrl Pts',(3.24918240690816,0.946939345899294,
6.52765779341606));
#155374=CARTESIAN_POINT('Ctrl Pts',(3.23052347304827,0.940053949659564,
6.49047134682375));
#155375=CARTESIAN_POINT('Ctrl Pts',(3.115444452,0.939268254,6.822316752));
#155376=CARTESIAN_POINT('Ctrl Pts',(3.490003539,1.004934719,6.651272505));
#155377=CARTESIAN_POINT('Ctrl Pts',(3.84358648,1.069390921,6.440251778));
#155378=CARTESIAN_POINT('Ctrl Pts',(3.226259034,0.939268254,6.492592136));
#155379=CARTESIAN_POINT('Ctrl Pts',(3.582715568,1.004934719,6.315463943));
#155380=CARTESIAN_POINT('Ctrl Pts',(3.917638724,1.069390921,6.100377597));
#155381=CARTESIAN_POINT('Origin',(-0.0644639989330614,0.803719114066693,
-0.180190601896159));
#155382=CARTESIAN_POINT('Ctrl Pts',(4.257512905,1.069390921,6.174429841));
#155383=CARTESIAN_POINT('Ctrl Pts',(4.592095092,1.004503495,5.94372222700001));
#155384=CARTESIAN_POINT('Ctrl Pts',(4.899787985,0.939276009000001,5.67821078400001));
#155385=CARTESIAN_POINT('Ctrl Pts',(3.917638724,1.069390921,6.100377597));
#155386=CARTESIAN_POINT('Ctrl Pts',(4.248208141,1.004503495,5.888087205));
#155387=CARTESIAN_POINT('Ctrl Pts',(4.553901916,0.939276009000001,5.64131875900001));
#155388=CARTESIAN_POINT('',(4.55025511321812,0.940053947070528,5.64426067931356));
#155389=CARTESIAN_POINT('Origin',(-0.124093184552952,0.946431366950847,
-0.15558361214484));
#155390=CARTESIAN_POINT('Ctrl Pts',(4.70796732248974,0.979367659143468,
5.83823977670622));
#155391=CARTESIAN_POINT('Ctrl Pts',(4.68162799240347,0.973133921597488,
5.80590068860478));
#155392=CARTESIAN_POINT('Ctrl Pts',(4.65530120807522,0.966746133420276,
5.77355009899131));
#155393=CARTESIAN_POINT('Ctrl Pts',(4.60273846663385,0.953652667081854,
5.70890194445239));
#155394=CARTESIAN_POINT('Ctrl Pts',(4.57647179682449,0.946939345811367,
5.67656660889873));
#155395=CARTESIAN_POINT('Ctrl Pts',(4.55025511161339,0.940053949596736,
5.6442606800774));
#155396=CARTESIAN_POINT('Ctrl Pts',(4.509203528,0.939268254,5.993086312));
#155397=CARTESIAN_POINT('Ctrl Pts',(4.838236174,1.004934719,5.745521853));
#155398=CARTESIAN_POINT('Ctrl Pts',(5.138189324,1.069390921,5.46342479300001));
#155399=CARTESIAN_POINT('Ctrl Pts',(4.54654628,0.939268254,5.647248615));
#155400=CARTESIAN_POINT('Ctrl Pts',(4.85659173300001,1.004934719,5.397633963));
#155401=CARTESIAN_POINT('Ctrl Pts',(5.137447365,1.069390921,5.11557763800001));
#155402=CARTESIAN_POINT('Origin',(-0.101692449550215,0.80371912530934,-0.162119920180928));
#155403=CARTESIAN_POINT('Ctrl Pts',(5.48529452,1.069390921,5.114835679));
#155404=CARTESIAN_POINT('Ctrl Pts',(5.762459044,1.004503495,4.817596601));
#155405=CARTESIAN_POINT('Ctrl Pts',(6.005881136,0.939276009000001,4.492147791));
#155406=CARTESIAN_POINT('Ctrl Pts',(5.137447365,1.069390921,5.115577638));
#155407=CARTESIAN_POINT('Ctrl Pts',(5.414652094,1.004503495,4.837187824));
#155408=CARTESIAN_POINT('Ctrl Pts',(5.660150997,0.939276009000001,4.530473562));
#155409=CARTESIAN_POINT('',(5.65722188060532,0.940053948044077,4.53413065603272));
#155410=CARTESIAN_POINT('Origin',(-0.154637863350217,0.946431349422814,
-0.125269808525206));
#155411=CARTESIAN_POINT('Ctrl Pts',(5.8529466375557,0.979367659130068,4.68967116711043));
#155412=CARTESIAN_POINT('Ctrl Pts',(5.82027120160593,0.973133929826048,
4.66375036058833));
#155413=CARTESIAN_POINT('Ctrl Pts',(5.78760547892972,0.9667461373603,4.63781557159902));
#155414=CARTESIAN_POINT('Ctrl Pts',(5.72237416328795,0.953652667030445,
4.58597827493679));
#155415=CARTESIAN_POINT('Ctrl Pts',(5.68977045243928,0.94693934575306,4.56004547916225));
#155416=CARTESIAN_POINT('Ctrl Pts',(5.65722187920481,0.940053949524057,
4.53413065739852));
#155417=CARTESIAN_POINT('Ctrl Pts',(5.69211725800001,0.939268254,4.883625817));
#155418=CARTESIAN_POINT('Ctrl Pts',(5.960238263,1.004934719,4.571116985));
#155419=CARTESIAN_POINT('Ctrl Pts',(6.192536146,1.069390921,4.231134137));
#155420=CARTESIAN_POINT('Ctrl Pts',(5.654242076,0.939268254,4.537846025));
#155421=CARTESIAN_POINT('Ctrl Pts',(5.903379066,1.004934719,4.227416618));
#155422=CARTESIAN_POINT('Ctrl Pts',(6.117034678,1.069390921,3.891578954));
#155423=CARTESIAN_POINT('Origin',(-0.134165992850455,0.803718955617848,
-0.136468870569669));
#155424=CARTESIAN_POINT('Ctrl Pts',(6.45658986,1.069390921,3.816077485));
#155425=CARTESIAN_POINT('Ctrl Pts',(6.66337681600001,1.004503495,3.466205512));
#155426=CARTESIAN_POINT('Ctrl Pts',(6.831145961,0.939276009000001,3.096036961));
#155427=CARTESIAN_POINT('Ctrl Pts',(6.117034678,1.069390921,3.891578954));
#155428=CARTESIAN_POINT('Ctrl Pts',(6.327912933,1.004503495,3.560106917));
#155429=CARTESIAN_POINT('Ctrl Pts',(6.501737708,0.939276009000001,3.207788456));
#155430=CARTESIAN_POINT('',(6.49966323932527,0.940053947076377,3.21198972307322));
#155431=CARTESIAN_POINT('Origin',(-0.177951791258012,0.946431387463854,
-0.0890984797086419));
#155432=CARTESIAN_POINT('Ctrl Pts',(6.72424867288718,0.979367659151059,
3.32181874645751));
#155433=CARTESIAN_POINT('Ctrl Pts',(6.68676491361813,0.973133921588396,
3.30352818266222));
#155434=CARTESIAN_POINT('Ctrl Pts',(6.64928771115034,0.96674613337873,3.28522191245718));
#155435=CARTESIAN_POINT('Ctrl Pts',(6.57443800366579,0.953652667026606,
3.2486193585997));
#155436=CARTESIAN_POINT('Ctrl Pts',(6.53702176458215,0.946939345686209,
3.23030169093364));
#155437=CARTESIAN_POINT('Ctrl Pts',(6.49966323833265,0.940053949471073,
3.21198972419785));
#155438=CARTESIAN_POINT('Ctrl Pts',(6.608873911,0.939268254,3.545812407));
#155439=CARTESIAN_POINT('Ctrl Pts',(6.803546235,1.004934719,3.182971767));
#155440=CARTESIAN_POINT('Ctrl Pts',(6.95732686000001,1.069390921,2.80100035));
#155441=CARTESIAN_POINT('Ctrl Pts',(6.49755179600001,0.939268254,3.216258799));
#155442=CARTESIAN_POINT('Ctrl Pts',(6.674130955,1.004934719,2.85952997));
#155443=CARTESIAN_POINT('Ctrl Pts',(6.810596247,1.069390921,2.485614363));
#155444=CARTESIAN_POINT('Origin',(-0.160366188329994,0.80371906941477,-0.104436620283826));
#155445=CARTESIAN_POINT('Ctrl Pts',(7.125982234,1.069390921,2.33888375));
#155446=CARTESIAN_POINT('Ctrl Pts',(7.252722494,1.004503495,1.952738506));
#155447=CARTESIAN_POINT('Ctrl Pts',(7.33699399300001,0.939276009000001,
1.555158883));
#155448=CARTESIAN_POINT('Ctrl Pts',(6.810596247,1.069390921,2.485614363));
#155449=CARTESIAN_POINT('Ctrl Pts',(6.945287596,1.004503495,2.116559367));
#155450=CARTESIAN_POINT('Ctrl Pts',(7.03931039,0.939276009000001,1.735110727));
#155451=CARTESIAN_POINT('',(7.03818757051311,0.940053948728594,1.73965971993727));
#155452=CARTESIAN_POINT('Origin',(-0.192944911291157,0.946431408256025,
-0.0487610407518779));
#155453=CARTESIAN_POINT('Ctrl Pts',(7.2811323139677,0.9793676591109,1.79864177274421));
#155454=CARTESIAN_POINT('Ctrl Pts',(7.24059302186394,0.973133928980762,
1.78883674406157));
#155455=CARTESIAN_POINT('Ctrl Pts',(7.20005668258872,0.966746136965024,
1.77901494874504));
#155456=CARTESIAN_POINT('Ctrl Pts',(7.11908843034966,0.953652667076533,
1.75935861156909));
#155457=CARTESIAN_POINT('Ctrl Pts',(7.078609206097,0.946939345946012,1.74951258654573));
#155458=CARTESIAN_POINT('Ctrl Pts',(7.03818756973805,0.94005394976175,1.73965972239499));
#155459=CARTESIAN_POINT('Ctrl Pts',(7.21660696600001,0.939268254,2.042200749));
#155460=CARTESIAN_POINT('Ctrl Pts',(7.328727947,1.004934719,1.645994327));
#155461=CARTESIAN_POINT('Ctrl Pts',(7.396800703,1.069390921,1.239894901));
#155462=CARTESIAN_POINT('Ctrl Pts',(7.037043215,0.939268254,1.744282886));
#155463=CARTESIAN_POINT('Ctrl Pts',(7.13280789900001,1.004934719,1.357934879));
#155464=CARTESIAN_POINT('Ctrl Pts',(7.18570190500001,1.069390921,0.963425207));
#155465=CARTESIAN_POINT('Origin',(-0.17906743711432,0.803719095684063,-0.0675208998158564));
#155466=CARTESIAN_POINT('Ctrl Pts',(7.462171599,1.069390921,0.75232641));
#155467=CARTESIAN_POINT('Ctrl Pts',(7.502938928,1.004503495,0.347963618));
#155468=CARTESIAN_POINT('Ctrl Pts',(7.49977234,0.939276009000001,-0.058436696));
#155469=CARTESIAN_POINT('Ctrl Pts',(7.185701905,1.069390921,0.963425207));
#155470=CARTESIAN_POINT('Ctrl Pts',(7.237908331,1.004503495,0.574043853));
#155471=CARTESIAN_POINT('Ctrl Pts',(7.247732742,0.939276009000001,0.181301149));
#155472=CARTESIAN_POINT('',(7.2476140724582,0.94005394809245,0.185985162743354));
#155473=CARTESIAN_POINT('Origin',(-0.198915958460675,0.946431400007768,
-0.00614357805642111));
#155474=CARTESIAN_POINT('Ctrl Pts',(7.49755829989574,0.979367659085542,
0.191362308830966));
#155475=CARTESIAN_POINT('Ctrl Pts',(7.45585900341291,0.973133929072959,
0.190501265756741));
#155476=CARTESIAN_POINT('Ctrl Pts',(7.41415898547609,0.966746137041716,
0.18962321328262));
#155477=CARTESIAN_POINT('Ctrl Pts',(7.3308581944993,0.953652667140489,0.187832211268411));
#155478=CARTESIAN_POINT('Ctrl Pts',(7.28920874762298,0.946939345996497,
0.186918217560852));
#155479=CARTESIAN_POINT('Ctrl Pts',(7.2476140721247,0.940053949810692,0.185985164931034));
#155480=CARTESIAN_POINT('Ctrl Pts',(7.48689949900001,0.939268254,0.443098054));
#155481=CARTESIAN_POINT('Ctrl Pts',(7.511226485,1.004934719,0.032052021));
#155482=CARTESIAN_POINT('Ctrl Pts',(7.49040836500001,1.069390921,-0.379186656));
#155483=CARTESIAN_POINT('Ctrl Pts',(7.247490315,0.939268254,0.190746244));
#155484=CARTESIAN_POINT('Ctrl Pts',(7.257962673,1.004934719,-0.207155738));
#155485=CARTESIAN_POINT('Ctrl Pts',(7.224812129,1.069390921,-0.603812641));
#155486=CARTESIAN_POINT('Origin',(-0.189396225307447,0.803718964998261,
-0.0274481071492917));
#155487=CARTESIAN_POINT('Ctrl Pts',(7.449438113,1.069390921,-0.869408877000001));
#155488=CARTESIAN_POINT('Ctrl Pts',(7.402326278,1.004503495,-1.273081663));
#155489=CARTESIAN_POINT('Ctrl Pts',(7.311869668,0.939276009000001,-1.66929984));
#155490=CARTESIAN_POINT('Ctrl Pts',(7.224812129,1.069390921,-0.603812640999999));
#155491=CARTESIAN_POINT('Ctrl Pts',(7.192092516,1.004503495,-0.995313314));
#155492=CARTESIAN_POINT('Ctrl Pts',(7.117259166,0.939276009000001,-1.380985869));
#155493=CARTESIAN_POINT('',(7.11815019522468,0.940053947080983,-1.37638585417308));
#155494=CARTESIAN_POINT('Origin',(-0.195586225751974,0.946431364602441,
0.0367611360511885));
#155495=CARTESIAN_POINT('Ctrl Pts',(7.36340679335851,0.979367659166656,
-1.42486504376531));
#155496=CARTESIAN_POINT('Ctrl Pts',(7.32249725512431,0.973133921633095,
-1.41674183026556));
#155497=CARTESIAN_POINT('Ctrl Pts',(7.28158343164316,0.966746133459874,
-1.40863508849938));
#155498=CARTESIAN_POINT('Ctrl Pts',(7.19984517687634,0.95365266713448,-1.39247701472651));
#155499=CARTESIAN_POINT('Ctrl Pts',(7.15897298894388,0.946939345913326,
-1.38441623981205));
#155500=CARTESIAN_POINT('Ctrl Pts',(7.11815019511434,0.940053949699928,
-1.37638585248842));
#155501=CARTESIAN_POINT('Ctrl Pts',(7.407112933,0.939268254,-1.176723413));
#155502=CARTESIAN_POINT('Ctrl Pts',(7.342508421,1.004934719,-1.583389001));
#155503=CARTESIAN_POINT('Ctrl Pts',(7.233772858,1.069390921,-1.980537866));
#155504=CARTESIAN_POINT('Ctrl Pts',(7.119052823,0.939268254,-1.371709481));
#155505=CARTESIAN_POINT('Ctrl Pts',(7.043743179,1.004934719,-1.762559983));
#155506=CARTESIAN_POINT('Ctrl Pts',(6.926098167,1.069390921,-2.14281688));
#155507=CARTESIAN_POINT('Origin',(-0.19086840065011,0.80371912887615,0.0139081448841));
#155508=CARTESIAN_POINT('Ctrl Pts',(7.08837718100001,1.069390921,-2.450491571));
#155509=CARTESIAN_POINT('Ctrl Pts',(6.955589078,1.004503495,-2.834599059));
#155510=CARTESIAN_POINT('Ctrl Pts',(6.78207209700001,0.939276009000001,
-3.202108379));
#155511=CARTESIAN_POINT('Ctrl Pts',(6.926098167,1.069390921,-2.14281688));
#155512=CARTESIAN_POINT('Ctrl Pts',(6.809982448,1.004503495,-2.518130736));
#155513=CARTESIAN_POINT('Ctrl Pts',(6.653990461,0.939276009000001,-2.878699522));
#155514=CARTESIAN_POINT('',(6.65584952602707,0.940053947074734,-2.87439859900565));
#155515=CARTESIAN_POINT('Origin',(-0.183110903818539,0.946431324714851,
0.0779469181040487));
#155516=CARTESIAN_POINT('Ctrl Pts',(6.88495056874341,0.979367659097039,
-2.97446729084826));
#155517=CARTESIAN_POINT('Ctrl Pts',(6.84674376983869,0.973133929140185,
-2.95773967239493));
#155518=CARTESIAN_POINT('Ctrl Pts',(6.80852917359771,0.966746137080596,
-2.94102718811594));
#155519=CARTESIAN_POINT('Ctrl Pts',(6.73217540049579,0.953652667102936,
-2.90767556313915));
#155520=CARTESIAN_POINT('Ctrl Pts',(6.69399161031049,0.946939345963208,
-2.89101693261409));
#155521=CARTESIAN_POINT('Ctrl Pts',(6.65584952632392,0.940053949701299,
-2.87439859723607));
#155522=CARTESIAN_POINT('Ctrl Pts',(6.980977999,0.939268254,-2.741522602));
#155523=CARTESIAN_POINT('Ctrl Pts',(6.830462824,1.004934719,-3.124792514));
#155524=CARTESIAN_POINT('Ctrl Pts',(6.638894171,1.069390921,-3.489281327));
#155525=CARTESIAN_POINT('Ctrl Pts',(6.657736333,0.939268254,-2.870025595));
#155526=CARTESIAN_POINT('Ctrl Pts',(6.500166082,1.004934719,-3.235548881));
#155527=CARTESIAN_POINT('Ctrl Pts',(6.303527553,1.069390921,-3.581625384));
#155528=CARTESIAN_POINT('Origin',(-0.183416398185337,0.803719072608364,
0.0546141480222323));
#155529=CARTESIAN_POINT('Ctrl Pts',(6.39587161,1.069390921,-3.916992003));
#155530=CARTESIAN_POINT('Ctrl Pts',(6.183616263,1.004503495,-4.263573754));
#155531=CARTESIAN_POINT('Ctrl Pts',(5.935152372,0.939276009000001,-4.585189889));
#155532=CARTESIAN_POINT('Ctrl Pts',(6.303527553,1.069390921,-3.581625384));
#155533=CARTESIAN_POINT('Ctrl Pts',(6.10944517,1.004503495,-3.923203163));
#155534=CARTESIAN_POINT('Ctrl Pts',(5.87958855800001,0.939276009000001,
-4.241808386));
#155535=CARTESIAN_POINT('',(5.88232873095194,0.940053948109766,-4.23800766024314));
#155536=CARTESIAN_POINT('Origin',(-0.162073690401495,0.946431358264443,
0.115488049280784));
#155537=CARTESIAN_POINT('Ctrl Pts',(6.08456170750433,0.979367659144574,
-4.38498675280478));
#155538=CARTESIAN_POINT('Ctrl Pts',(6.05084410437289,0.973133928914535,
-4.36043688345674));
#155539=CARTESIAN_POINT('Ctrl Pts',(6.01711563512004,0.966746137004887,
-4.33590011995558));
#155540=CARTESIAN_POINT('Ctrl Pts',(5.9497165849654,0.953652667153041,-4.28691443395892));
#155541=CARTESIAN_POINT('Ctrl Pts',(5.91600662413242,0.946939346097956,
-4.26243688720522));
#155542=CARTESIAN_POINT('Ctrl Pts',(5.88232873168166,0.940053949827562,
-4.238007658753));
#155543=CARTESIAN_POINT('Ctrl Pts',(6.22842029200001,0.939268254,-4.17813124));
#155544=CARTESIAN_POINT('Ctrl Pts',(5.999032377,1.004934719,-4.520084201));
#155545=CARTESIAN_POINT('Ctrl Pts',(5.733588172,1.069390921,-4.83486987100001));
#155546=CARTESIAN_POINT('Ctrl Pts',(5.885111492,0.939268254,-4.234142502));
#155547=CARTESIAN_POINT('Ctrl Pts',(5.652648444,1.004934719,-4.557247111));
#155548=CARTESIAN_POINT('Ctrl Pts',(5.38621099600001,1.069390921,-4.852961066));
#155549=CARTESIAN_POINT('Origin',(-0.167387900493161,0.803718943983406,
0.0927664531750083));
#155550=CARTESIAN_POINT('Ctrl Pts',(5.40430219,1.069390921,-5.200338242));
#155551=CARTESIAN_POINT('Ctrl Pts',(5.122504424,1.004503495,-5.493188479));
#155552=CARTESIAN_POINT('Ctrl Pts',(4.810711519,0.939276009000001,-5.753873015));
#155553=CARTESIAN_POINT('Ctrl Pts',(5.386210996,1.069390921,-4.852961066));
#155554=CARTESIAN_POINT('Ctrl Pts',(5.123237026,1.004503495,-5.144830971));
#155555=CARTESIAN_POINT('Ctrl Pts',(4.830263629,0.939276009000001,-5.406575004));
#155556=CARTESIAN_POINT('',(4.83375678100282,0.940053947060246,-5.40345219171606));
#155557=CARTESIAN_POINT('Origin',(-0.133457977517737,0.946431359286523,
0.147629070274841));
#155558=CARTESIAN_POINT('Ctrl Pts',(4.99966550307941,0.979367659095725,
-5.59046910848041));
#155559=CARTESIAN_POINT('Ctrl Pts',(4.97201370358805,0.973133930785602,
-5.559244922896));
#155560=CARTESIAN_POINT('Ctrl Pts',(4.94434846128487,0.96674613782819,-5.52803118575712));
#155561=CARTESIAN_POINT('Ctrl Pts',(4.88905563426153,0.953652667068031,
-5.46570194974581));
#155562=CARTESIAN_POINT('Ctrl Pts',(4.86139574168978,0.946939345779763,
-5.43455002807549));
#155563=CARTESIAN_POINT('Ctrl Pts',(4.83375678201755,0.940053949586176,
-5.40345219025493));
#155564=CARTESIAN_POINT('Ctrl Pts',(5.184628575,0.939268254,-5.419375106));
#155565=CARTESIAN_POINT('Ctrl Pts',(4.88709384300001,1.004934719,-5.704021776));
#155566=CARTESIAN_POINT('Ctrl Pts',(4.56018596200001,1.069390921,-5.954385274));
#155567=CARTESIAN_POINT('Ctrl Pts',(4.837305378,0.939268254,-5.400275611));
#155568=CARTESIAN_POINT('Ctrl Pts',(4.540819247,1.004934719,-5.66585353));
#155569=CARTESIAN_POINT('Ctrl Pts',(4.217041199,1.069390921,-5.897377682));
#155570=CARTESIAN_POINT('Origin',(-0.143532263022791,0.803719077910381,
0.126580913646047));
#155571=CARTESIAN_POINT('Ctrl Pts',(4.160033607,1.069390921,-6.24052244500001));
#155572=CARTESIAN_POINT('Ctrl Pts',(3.821869971,1.004503495,-6.46594781600001));
#155573=CARTESIAN_POINT('Ctrl Pts',(3.461327142,0.939276009000001,-6.65351143500001));
#155574=CARTESIAN_POINT('Ctrl Pts',(4.217041199,1.069390921,-5.897377682));
#155575=CARTESIAN_POINT('Ctrl Pts',(3.897472013,1.004503495,-6.125892201));
#155576=CARTESIAN_POINT('Ctrl Pts',(3.555080941,0.939276009000001,-6.31853618300001));
#155577=CARTESIAN_POINT('',(3.55916373788445,0.940053947075642,-6.31623730607955));
#155578=CARTESIAN_POINT('Origin',(-0.0986017871388895,0.946431370250801,
0.172866876304308));
#155579=CARTESIAN_POINT('Ctrl Pts',(3.68099049666104,0.979367659141269,
-6.53454734171104));
#155580=CARTESIAN_POINT('Ctrl Pts',(3.66069745649746,0.973133930415714,
-6.49810883838615));
#155581=CARTESIAN_POINT('Ctrl Pts',(3.64038904380532,0.966746137680773,
-6.46167765320151));
#155582=CARTESIAN_POINT('Ctrl Pts',(3.59978787616403,0.953652667071589,
-6.38891931766773));
#155583=CARTESIAN_POINT('Ctrl Pts',(3.57947139933411,0.946939345954821,
-6.35254965228124));
#155584=CARTESIAN_POINT('Ctrl Pts',(3.55916373886498,0.940053949718943,
-6.31623730502998));
#155585=CARTESIAN_POINT('Ctrl Pts',(3.898409388,0.939268254,-6.407215015));
#155586=CARTESIAN_POINT('Ctrl Pts',(3.546640232,1.004934719,-6.621245631));
#155587=CARTESIAN_POINT('Ctrl Pts',(3.173554525,1.069390921,-6.79548023900001));
#155588=CARTESIAN_POINT('Ctrl Pts',(3.563312241,0.939268254,-6.313897835));
#155589=CARTESIAN_POINT('Ctrl Pts',(3.216666389,1.004934719,-6.509530936));
#155590=CARTESIAN_POINT('Ctrl Pts',(2.850687243,1.069390921,-6.666039472));
#155591=CARTESIAN_POINT('Origin',(-0.112965338103565,0.803719091406703,
0.154476604966692));
#155592=CARTESIAN_POINT('Ctrl Pts',(2.721246476,1.069390921,-6.988906754));
#155593=CARTESIAN_POINT('Ctrl Pts',(2.342529127,1.004503495,-7.13636662));
#155594=CARTESIAN_POINT('Ctrl Pts',(1.950094955,0.939276009000001,-7.242039054));
#155595=CARTESIAN_POINT('Ctrl Pts',(2.850687243,1.069390921,-6.666039472));
#155596=CARTESIAN_POINT('Ctrl Pts',(2.48946554,1.004503495,-6.82051352));
#155597=CARTESIAN_POINT('Ctrl Pts',(2.11366662,0.939276009000001,-6.935049634));
#155598=CARTESIAN_POINT('',(2.11814815318168,0.940053947040107,-6.93368218303118));
#155599=CARTESIAN_POINT('Origin',(-0.0591353114936999,0.946431348139323,
0.190021965440267));
#155600=CARTESIAN_POINT('Ctrl Pts',(2.19019646628857,0.979367659164797,
-7.1730774035426));
#155601=CARTESIAN_POINT('Ctrl Pts',(2.17821106626055,0.97313392993309,-7.13312840511824));
#155602=CARTESIAN_POINT('Ctrl Pts',(2.1662090814254,0.96674613745119,-7.09318325406989));
#155603=CARTESIAN_POINT('Ctrl Pts',(2.14219803858705,0.953652667117197,
-7.01339791887875));
#155604=CARTESIAN_POINT('Ctrl Pts',(2.13017495246056,0.946939345817816,
-6.97351111311087));
#155605=CARTESIAN_POINT('Ctrl Pts',(2.11814815529179,0.940053949598351,
-6.93368218195176));
#155606=CARTESIAN_POINT('Ctrl Pts',(2.429904911,0.939268254,-7.09546067));
#155607=CARTESIAN_POINT('Ctrl Pts',(2.040349667,1.004934719,-7.2288674));
#155608=CARTESIAN_POINT('Ctrl Pts',(1.638531205,1.069390921,-7.3188261));
#155609=CARTESIAN_POINT('Ctrl Pts',(2.122702584,0.939268254,-6.932289213));
#155610=CARTESIAN_POINT('Ctrl Pts',(1.742105785,1.004934719,-7.04882990900001));
#155611=CARTESIAN_POINT('Ctrl Pts',(1.35103832,1.069390921,-7.123004665));
#155612=CARTESIAN_POINT('Origin',(-0.0771164253396961,0.803719107667327,
0.175149470351337));
#155613=CARTESIAN_POINT('Ctrl Pts',(1.155216884,1.069390921,-7.410497551));
#155614=CARTESIAN_POINT('Ctrl Pts',(0.753654224,1.004503495,-7.473096852));
#155615=CARTESIAN_POINT('Ctrl Pts',(0.347678495,0.939276009000001,-7.491936977));
#155616=CARTESIAN_POINT('Ctrl Pts',(1.35103832,1.069390921,-7.123004665));
#155617=CARTESIAN_POINT('Ctrl Pts',(0.965054424999999,1.004503495,-7.196215207));
#155618=CARTESIAN_POINT('Ctrl Pts',(0.573419596,0.939276009000001,-7.227287871));
#155619=CARTESIAN_POINT('',(0.578090315769932,0.940053947054566,-7.22691578804911));
#155620=CARTESIAN_POINT('Origin',(-0.0169036609396048,0.946431334859754,
0.198291733152491));
#155621=CARTESIAN_POINT('Ctrl Pts',(0.596991283107538,0.97936765917447,
-7.47620233865752));
#155622=CARTESIAN_POINT('Ctrl Pts',(0.593873944611415,0.973133921644323,
-7.43461076353645));
#155623=CARTESIAN_POINT('Ctrl Pts',(0.590739588336705,0.966746133474978,
-7.3930194660492));
#155624=CARTESIAN_POINT('Ctrl Pts',(0.584441400587957,0.953652667122777,
-7.30993782852173));
#155625=CARTESIAN_POINT('Ctrl Pts',(0.581273891583116,0.946939345895764,
-7.26839894647513));
#155626=CARTESIAN_POINT('Ctrl Pts',(0.578090316875115,0.940053949636729,
-7.2269157875357));
#155627=CARTESIAN_POINT('Ctrl Pts',(0.847780781,0.939268254,-7.451930471));
#155628=CARTESIAN_POINT('Ctrl Pts',(0.438654618,1.004934719,-7.498475363));
#155629=CARTESIAN_POINT('Ctrl Pts',(0.026891988,1.069390921,-7.499951788));
#155630=CARTESIAN_POINT('Ctrl Pts',(0.582837713,0.939268254,-7.226534453));
#155631=CARTESIAN_POINT('Ctrl Pts',(0.186086252,1.004934719,-7.258533431));
#155632=CARTESIAN_POINT('Ctrl Pts',(-0.211783654,1.069390921,-7.246906077));
#155633=CARTESIAN_POINT('Origin',(-0.0376615330110996,0.803719054725182,
0.187632234918865));
#155634=CARTESIAN_POINT('Ctrl Pts',(-0.464829365,1.069390921,-7.485581718));
#155635=CARTESIAN_POINT('Ctrl Pts',(-0.870460713,1.004503495,-7.46039338));
#155636=CARTESIAN_POINT('Ctrl Pts',(-1.270995025,0.939276009000001,-7.391520253));
#155637=CARTESIAN_POINT('Ctrl Pts',(-0.211783654,1.069390921,-7.246906077));
#155638=CARTESIAN_POINT('Ctrl Pts',(-0.604481562,1.004503495,-7.23542986900001));
#155639=CARTESIAN_POINT('Ctrl Pts',(-0.993639891,0.939276009000001,-7.18158616));
#155640=CARTESIAN_POINT('',(-0.988998383218434,0.940053947070287,-7.18222684270956));
#155641=CARTESIAN_POINT('Origin',(0.0261184061910333,0.946431356628239,
0.197289686170977));
#155642=CARTESIAN_POINT('Ctrl Pts',(-1.02412854958253,0.979367659146776,
-7.42974836134486));
#155643=CARTESIAN_POINT('Ctrl Pts',(-1.0182320549564,0.973133929868704,
-7.38845909318597));
#155644=CARTESIAN_POINT('Ctrl Pts',(-1.01235222786181,0.966746137434024,
-7.34716635363524));
#155645=CARTESIAN_POINT('Ctrl Pts',(-1.00064306753657,0.953652667137174,
-7.26467316949527));
#155646=CARTESIAN_POINT('Ctrl Pts',(-0.994806890059517,0.946939345921978,
-7.22342452261311));
#155647=CARTESIAN_POINT('Ctrl Pts',(-0.9889983814996,0.940053949703201,
-7.18222684251186));
#155648=CARTESIAN_POINT('Ctrl Pts',(-0.773984637,0.939268254,-7.45995628600001));
#155649=CARTESIAN_POINT('Ctrl Pts',(-1.183551433,1.004934719,-7.417462952));
#155650=CARTESIAN_POINT('Ctrl Pts',(-1.586004669,1.069390921,-7.330388065));
#155651=CARTESIAN_POINT('Ctrl Pts',(-0.984280001000001,0.939268254,-7.182874973));
#155652=CARTESIAN_POINT('Ctrl Pts',(-1.378634468,1.004934719,-7.128835996));
#155653=CARTESIAN_POINT('Ctrl Pts',(-1.764702859,1.069390921,-7.03195021400001));
#155654=CARTESIAN_POINT('Origin',(0.00355437245078333,0.803719069914868,
0.191341631743444));
#155655=CARTESIAN_POINT('Ctrl Pts',(-2.06314071,1.069390921,-7.210648404));
#155656=CARTESIAN_POINT('Ctrl Pts',(-2.453873874,1.004503495,-7.098850206));
#155657=CARTESIAN_POINT('Ctrl Pts',(-2.83023823,0.939276009000001,-6.945484257));
#155658=CARTESIAN_POINT('Ctrl Pts',(-1.764702859,1.069390921,-7.03195021400001));
#155659=CARTESIAN_POINT('Ctrl Pts',(-2.145752663,1.004503495,-6.936323872));
#155660=CARTESIAN_POINT('Ctrl Pts',(-2.51423788,0.939276009000001,-6.800081461));
#155661=CARTESIAN_POINT('',(-2.50984261641908,0.940053947041797,-6.80170495217655));
#155662=CARTESIAN_POINT('Origin',(0.0679191305552662,0.946431346107127,
0.187062182692088));
#155663=CARTESIAN_POINT('Ctrl Pts',(-2.59736126895321,0.979367659134186,
-7.0358876083094));
#155664=CARTESIAN_POINT('Ctrl Pts',(-2.58272665904198,0.973133929858945,
-6.99683123235415));
#155665=CARTESIAN_POINT('Ctrl Pts',(-2.56810758069108,0.966746137396923,
-6.95776788295547));
#155666=CARTESIAN_POINT('Ctrl Pts',(-2.53893857804772,0.953652667032495,
-6.87972046655708));
#155667=CARTESIAN_POINT('Ctrl Pts',(-2.52437160761352,0.946939345850515,
-6.84069079594145));
#155668=CARTESIAN_POINT('Ctrl Pts',(-2.50984261543138,0.940053949591765,
-6.80170495209428));
#155669=CARTESIAN_POINT('Ctrl Pts',(-2.359559393,0.939268254,-7.119162835));
#155670=CARTESIAN_POINT('Ctrl Pts',(-2.750415934,1.004934719,-6.98961821800001));
#155671=CARTESIAN_POINT('Ctrl Pts',(-3.124741511,1.069390921,-6.818063544));
#155672=CARTESIAN_POINT('Ctrl Pts',(-2.505373877,0.939268254,-6.803352243));
#155673=CARTESIAN_POINT('Ctrl Pts',(-2.878891773,1.004934719,-6.665802114));
#155674=CARTESIAN_POINT('Ctrl Pts',(-3.23510652,1.069390921,-6.488188176));
#155675=CARTESIAN_POINT('Origin',(0.0446040535888903,0.803719077786697,
0.186104077523978));
#155676=CARTESIAN_POINT('Ctrl Pts',(-3.564981888,1.069390921,-6.59855318500001));
#155677=CARTESIAN_POINT('Ctrl Pts',(-3.922546621,1.004503495,-6.405372686));
#155678=CARTESIAN_POINT('Ctrl Pts',(-4.257142641,0.939276009000001,-6.174685136));
#155679=CARTESIAN_POINT('Ctrl Pts',(-3.23510652,1.069390921,-6.488188176));
#155680=CARTESIAN_POINT('Ctrl Pts',(-3.586690754,1.004503495,-6.31288308));
#155681=CARTESIAN_POINT('Ctrl Pts',(-3.917272901,0.939276009000001,-6.100612512));
#155682=CARTESIAN_POINT('',(-3.91332939950011,0.940053948078126,-6.10314289857884));
#155683=CARTESIAN_POINT('Origin',(0.106544188480028,0.946431356239456,0.168088403438719));
#155684=CARTESIAN_POINT('Ctrl Pts',(-4.04914426237965,0.979367659183749,
-6.31303657046451));
#155685=CARTESIAN_POINT('Ctrl Pts',(-4.02645583639741,0.973133930248886,
-6.27803932140032));
#155686=CARTESIAN_POINT('Ctrl Pts',(-4.00378107790911,0.966746137632722,
-6.24303192029114));
#155687=CARTESIAN_POINT('Ctrl Pts',(-3.95851614221157,0.95365266713256,
-6.17307968194312));
#155688=CARTESIAN_POINT('Ctrl Pts',(-3.93589951412828,0.946939346036999,
-6.13809397195536));
#155689=CARTESIAN_POINT('Ctrl Pts',(-3.91332939753396,0.940053949787857,
-6.10314289951169));
#155690=CARTESIAN_POINT('Ctrl Pts',(-3.834803774,0.939268254,-6.44548524300001));
#155691=CARTESIAN_POINT('Ctrl Pts',(-4.188674043,1.004934719,-6.234946704));
#155692=CARTESIAN_POINT('Ctrl Pts',(-4.517368912,1.069390921,-5.98693394900001));
#155693=CARTESIAN_POINT('Ctrl Pts',(-3.909319254,0.939268254,-6.105712323));
#155694=CARTESIAN_POINT('Ctrl Pts',(-4.244535298,1.004934719,-5.891082733));
#155695=CARTESIAN_POINT('Ctrl Pts',(-4.554240196,1.069390921,-5.64104566900001));
#155696=CARTESIAN_POINT('Origin',(0.08356823025853,0.80371894377527,0.172164714886629));
#155697=CARTESIAN_POINT('Ctrl Pts',(-4.900128476,1.069390921,-5.677916952));
#155698=CARTESIAN_POINT('Ctrl Pts',(-5.207805447,1.004503495,-5.412387059));
#155699=CARTESIAN_POINT('Ctrl Pts',(-5.484987794,0.939276009000001,-5.115164602));
#155700=CARTESIAN_POINT('Ctrl Pts',(-4.554240196,1.069390921,-5.641045669));
#155701=CARTESIAN_POINT('Ctrl Pts',(-4.859919172,1.004503495,-5.394258892));
#155702=CARTESIAN_POINT('Ctrl Pts',(-5.137140595,0.939276009000001,-5.115885701));
#155703=CARTESIAN_POINT('',(-5.13383324781926,0.940053948082874,-5.11920466472028));
#155704=CARTESIAN_POINT('Origin',(0.140187158168336,0.9464314117376,0.141254600293041));
#155705=CARTESIAN_POINT('Ctrl Pts',(-5.31159377033098,0.979367659185378,
-5.29499495970319));
#155706=CARTESIAN_POINT('Ctrl Pts',(-5.28191237207512,0.973133921633951,
-5.26569322721615));
#155707=CARTESIAN_POINT('Ctrl Pts',(-5.2522422024183,0.966746133433956,
-5.23637870407356));
#155708=CARTESIAN_POINT('Ctrl Pts',(-5.1929978910845,0.953652667097977,
-5.17779255156783));
#155709=CARTESIAN_POINT('Ctrl Pts',(-5.16338913336467,0.946939345930828,
-5.14848669395025));
#155710=CARTESIAN_POINT('Ctrl Pts',(-5.13383324626273,0.940053949730156,
-5.11920466590403));
#155711=CARTESIAN_POINT('Ctrl Pts',(-5.130736993,0.939268254,-5.47042392400001));
#155712=CARTESIAN_POINT('Ctrl Pts',(-5.431074409,1.004934719,-5.188736012));
#155713=CARTESIAN_POINT('Ctrl Pts',(-5.698769164,1.069390921,-4.875861977));
#155714=CARTESIAN_POINT('Ctrl Pts',(-5.130469208,0.939268254,-5.12257608100001));
#155715=CARTESIAN_POINT('Ctrl Pts',(-5.41170907,1.004934719,-4.840902871));
#155716=CARTESIAN_POINT('Ctrl Pts',(-5.660422662,1.069390921,-4.530134136));
#155717=CARTESIAN_POINT('Origin',(0.11862458411581,0.80371897769967,0.15017473186036));
#155718=CARTESIAN_POINT('Ctrl Pts',(-6.006150502,1.069390921,-4.491787634));
#155719=CARTESIAN_POINT('Ctrl Pts',(-6.249553078,1.004503495,-4.166324228));
#155720=CARTESIAN_POINT('Ctrl Pts',(-6.456361013,0.939276009000001,-3.816464655));
#155721=CARTESIAN_POINT('Ctrl Pts',(-5.660422662,1.069390921,-4.530134136));
#155722=CARTESIAN_POINT('Ctrl Pts',(-5.905903171,1.004503495,-4.223405152));
#155723=CARTESIAN_POINT('Ctrl Pts',(-6.116801304,0.939276009000001,-3.891945762));
#155724=CARTESIAN_POINT('',(-6.11428476024431,0.940053948058558,-3.89589811155744));
#155725=CARTESIAN_POINT('Origin',(0.16727548068703,0.946431357451162,0.107816230720738));
#155726=CARTESIAN_POINT('Ctrl Pts',(-6.32567905648818,0.979367659135639,
-4.02936526868395));
#155727=CARTESIAN_POINT('Ctrl Pts',(-6.29039262764721,0.973133928858821,
-4.00712924358955));
#155728=CARTESIAN_POINT('Ctrl Pts',(-6.25511435220885,0.966746136961554,
-3.98487827339719));
#155729=CARTESIAN_POINT('Ctrl Pts',(-6.18466083040325,0.953652667160767,
-3.94039759680165));
#155730=CARTESIAN_POINT('Ctrl Pts',(-6.14944441594141,0.94693934598928,
-3.91814190177741));
#155731=CARTESIAN_POINT('Ctrl Pts',(-6.11428475859154,0.940053949754415,
-3.89589811364495));
#155732=CARTESIAN_POINT('Ctrl Pts',(-6.186762652,0.939268254,-4.239571663));
#155733=CARTESIAN_POINT('Ctrl Pts',(-6.419523772,1.004934719,-3.899905791));
#155734=CARTESIAN_POINT('Ctrl Pts',(-6.61370130300001,1.069390921,-3.536800117));
#155735=CARTESIAN_POINT('Ctrl Pts',(-6.111724124,0.939268254,-3.899913875));
#155736=CARTESIAN_POINT('Ctrl Pts',(-6.32583734,1.004934719,-3.564367771));
#155737=CARTESIAN_POINT('Ctrl Pts',(-6.501930055,1.069390921,-3.207398566));
#155738=CARTESIAN_POINT('Origin',(0.148134494418555,0.80371897014872,0.121163037150532));
#155739=CARTESIAN_POINT('Ctrl Pts',(-6.831331606,1.069390921,-3.095627318));
#155740=CARTESIAN_POINT('Ctrl Pts',(-6.999078553,1.004503495,-2.725448706));
#155741=CARTESIAN_POINT('Ctrl Pts',(-7.12584196800001,0.939276009000001,
-2.339311063));
#155742=CARTESIAN_POINT('Ctrl Pts',(-6.501930055,1.069390921,-3.207398566));
#155743=CARTESIAN_POINT('Ctrl Pts',(-6.675733702,1.004503495,-2.855069682));
#155744=CARTESIAN_POINT('Ctrl Pts',(-6.81044718200001,0.939276009000001,
-2.486022764));
#155745=CARTESIAN_POINT('',(-6.80883911175379,0.940053947055498,-2.49042369268793));
#155746=CARTESIAN_POINT('Origin',(0.186541774058421,0.946431338254617,0.0693361714653745));
#155747=CARTESIAN_POINT('Ctrl Pts',(-7.043982621342,0.979367659152127,-2.57532693620972));
#155748=CARTESIAN_POINT('Ctrl Pts',(-7.00474108494745,0.973133929429406,
-2.5611963175052));
#155749=CARTESIAN_POINT('Ctrl Pts',(-6.96550429303653,0.966746137216144,
-2.5470493483575));
#155750=CARTESIAN_POINT('Ctrl Pts',(-6.88713590294071,0.95365266710452,
-2.51875402924264));
#155751=CARTESIAN_POINT('Ctrl Pts',(-6.84795851182924,0.946939345877625,
-2.50458914798822));
#155752=CARTESIAN_POINT('Ctrl Pts',(-6.808839110773,0.940053949626277,-2.49042369414692));
#155753=CARTESIAN_POINT('Ctrl Pts',(-6.953502166,0.939268254,-2.810481743));
#155754=CARTESIAN_POINT('Ctrl Pts',(-7.107803339,1.004934719,-2.428720309));
#155755=CARTESIAN_POINT('Ctrl Pts',(-7.21938412,1.069390921,-2.032361415));
#155756=CARTESIAN_POINT('Ctrl Pts',(-6.807201613,0.939268254,-2.49489603));
#155757=CARTESIAN_POINT('Ctrl Pts',(-6.94417648700001,1.004934719,-2.121166795));
#155758=CARTESIAN_POINT('Ctrl Pts',(-7.039414425,1.069390921,-1.734688604));
#155759=CARTESIAN_POINT('Origin',(0.170717629805586,0.803719092771659,0.0864857378840431));
#155760=CARTESIAN_POINT('Ctrl Pts',(-7.337087236,1.069390921,-1.554718909));
#155761=CARTESIAN_POINT('Ctrl Pts',(-7.421334894,1.004503495,-1.157134232));
#155762=CARTESIAN_POINT('Ctrl Pts',(-7.462126472,0.939276009000001,-0.752773886));
#155763=CARTESIAN_POINT('Ctrl Pts',(-7.039414425,1.069390921,-1.734688604));
#155764=CARTESIAN_POINT('Ctrl Pts',(-7.133414344,1.004503495,-1.353234327));
#155765=CARTESIAN_POINT('Ctrl Pts',(-7.185644119,0.939276009000001,-0.963856104));
#155766=CARTESIAN_POINT('',(-7.18501971399297,0.940053947079714,-0.9684998294504));
#155767=CARTESIAN_POINT('Origin',(0.197085704960005,0.946431359289948,0.027614151461707));
#155768=CARTESIAN_POINT('Ctrl Pts',(-7.4329173874246,0.979367659184994,
-1.0008691788516));
#155769=CARTESIAN_POINT('Ctrl Pts',(-7.3915556332617,0.973133929796456,
-0.995504696752814));
#155770=CARTESIAN_POINT('Ctrl Pts',(-7.35019499413787,0.966746137377657,
-0.990123226044648));
#155771=CARTESIAN_POINT('Ctrl Pts',(-7.26757615490654,0.953652667071922,
-0.979336322679543));
#155772=CARTESIAN_POINT('Ctrl Pts',(-7.2262696785515,0.94693934584413,-0.973924589329538));
#155773=CARTESIAN_POINT('Ctrl Pts',(-7.18501971341776,0.94005394961285,
-0.968499830609128));
#155774=CARTESIAN_POINT('Ctrl Pts',(-7.39510364700001,0.939268254,-1.24997682));
#155775=CARTESIAN_POINT('Ctrl Pts',(-7.463729921,1.004934719,-0.843970566000001));
#155776=CARTESIAN_POINT('Ctrl Pts',(-7.48749656,1.069390921,-0.432891753));
#155777=CARTESIAN_POINT('Ctrl Pts',(-7.18438192,0.939268254,-0.97321962));
#155778=CARTESIAN_POINT('Ctrl Pts',(-7.23781366,1.004934719,-0.578782418));
#155779=CARTESIAN_POINT('Ctrl Pts',(-7.2477436,1.069390921,-0.180866531));
#155780=CARTESIAN_POINT('Origin',(0.185317934167133,0.803719109795523,0.0477644810006672));
#155781=CARTESIAN_POINT('Ctrl Pts',(-7.499768822,1.069390921,0.058886428));
#155782=CARTESIAN_POINT('Ctrl Pts',(-7.496577864,1.004503495,0.465286552));
#155783=CARTESIAN_POINT('Ctrl Pts',(-7.449490235,0.939276009000001,0.868962162));
#155784=CARTESIAN_POINT('Ctrl Pts',(-7.24774360000001,1.069390921,-0.180866531));
#155785=CARTESIAN_POINT('Ctrl Pts',(-7.25754446,1.004503495,0.211876761));
#155786=CARTESIAN_POINT('Ctrl Pts',(-7.22484832400001,0.939276009000001,
0.603379396));
#155787=CARTESIAN_POINT('',(-7.22523678108189,0.940053948086643,0.598710009952622));
#155788=CARTESIAN_POINT('Origin',(0.198414091245139,0.946431379860457,-0.0153990371398191));
#155789=CARTESIAN_POINT('Ctrl Pts',(-7.47429719712509,0.979367659133194,
0.62038810919019));
#155790=CARTESIAN_POINT('Ctrl Pts',(-7.43274924742846,0.973133928964554,
0.616735617683767));
#155791=CARTESIAN_POINT('Ctrl Pts',(-7.39119874306821,0.966746137007537,
0.613099958047034));
#155792=CARTESIAN_POINT('Ctrl Pts',(-7.30819262379929,0.95365266714958,
0.605874061569174));
#155793=CARTESIAN_POINT('Ctrl Pts',(-7.2666885075572,0.946939345977453,
0.602279600214168));
#155794=CARTESIAN_POINT('Ctrl Pts',(-7.22523678098003,0.940053949744611,
0.598710007937336));
#155795=CARTESIAN_POINT('Ctrl Pts',(-7.4909183,0.939268254,0.36897563));
#155796=CARTESIAN_POINT('Ctrl Pts',(-7.470660787,1.004934719,0.780242304));
#155797=CARTESIAN_POINT('Ctrl Pts',(-7.405501982,1.069390921,1.186819448));
#155798=CARTESIAN_POINT('Ctrl Pts',(-7.22562851299999,0.939268254,0.593963458000001));
#155799=CARTESIAN_POINT('Ctrl Pts',(-7.193018709,1.004934719,0.990665182));
#155800=CARTESIAN_POINT('Ctrl Pts',(-7.11717634,1.069390921,1.381412661));
#155801=CARTESIAN_POINT('Origin',(0.191253352313244,0.803718922848623,0.00680992009186643));
#155802=CARTESIAN_POINT('Ctrl Pts',(-7.311769554,1.069390921,1.669738302));
#155803=CARTESIAN_POINT('Ctrl Pts',(-7.221289184,1.004503495,2.065951054));
#155804=CARTESIAN_POINT('Ctrl Pts',(-7.08852411500001,0.939276009000001,
2.450066505));
#155805=CARTESIAN_POINT('Ctrl Pts',(-7.11717634,1.069390921,1.381412661));
#155806=CARTESIAN_POINT('Ctrl Pts',(-7.04231986300001,1.004503495,1.767080728));
#155807=CARTESIAN_POINT('Ctrl Pts',(-6.926226651,0.939276009000001,2.142401545));
#155808=CARTESIAN_POINT('',(-6.92760980555269,0.94005394704967,2.13792483369844));
#155809=CARTESIAN_POINT('Origin',(0.190464918460538,0.946431351991406,-0.057692183818133));
#155810=CARTESIAN_POINT('Ctrl Pts',(-7.16618717754861,0.979367659162817,
2.21263673886222));
#155811=CARTESIAN_POINT('Ctrl Pts',(-7.12639577943535,0.973133929903967,
2.20013806146995));
#155812=CARTESIAN_POINT('Ctrl Pts',(-7.08659825869256,0.966746137413077,
2.18765527027077));
#155813=CARTESIAN_POINT('Ctrl Pts',(-7.00708612763533,0.953652667044357,
2.16275444828855));
#155814=CARTESIAN_POINT('Ctrl Pts',(-6.96732505701767,0.946939345769651,
2.15032186507112));
#155815=CARTESIAN_POINT('Ctrl Pts',(-6.92760980569742,0.940053949535198,
2.13792483185428));
#155816=CARTESIAN_POINT('Ctrl Pts',(-7.23646594,0.939268254,1.97067519));
#155817=CARTESIAN_POINT('Ctrl Pts',(-7.128271858,1.004934719,2.36797191));
#155818=CARTESIAN_POINT('Ctrl Pts',(-6.977234361,1.069390921,2.751036289));
#155819=CARTESIAN_POINT('Ctrl Pts',(-6.929012748,0.939268254,2.133373465));
#155820=CARTESIAN_POINT('Ctrl Pts',(-6.811886199,1.004934719,2.513790379));
#155821=CARTESIAN_POINT('Ctrl Pts',(-6.653817825,1.069390921,2.879098531));
#155822=CARTESIAN_POINT('Origin',(0.188246019438175,0.803719090896389,-0.034463192469657));
#155823=CARTESIAN_POINT('Ctrl Pts',(-6.781880067,1.069390921,3.202515068));
#155824=CARTESIAN_POINT('Ctrl Pts',(-6.60834104800001,1.004503495,3.570013982));
#155825=CARTESIAN_POINT('Ctrl Pts',(-6.396106485,0.939276009000001,3.916608461));
#155826=CARTESIAN_POINT('Ctrl Pts',(-6.653817825,1.069390921,2.879098531));
#155827=CARTESIAN_POINT('Ctrl Pts',(-6.497804216,1.004503495,3.239657963));
#155828=CARTESIAN_POINT('Ctrl Pts',(-6.303742317,0.939276009000001,3.58124738));
#155829=CARTESIAN_POINT('',(-6.30605549550746,0.94005394707995,3.57717266853147));
#155830=CARTESIAN_POINT('Origin',(0.173609964766765,0.94643137782079,-0.0972877614143342));
#155831=CARTESIAN_POINT('Ctrl Pts',(-6.52299420951791,0.979367659152604,
3.70142493378223));
#155832=CARTESIAN_POINT('Ctrl Pts',(-6.48681995481761,0.973133929282097,
3.68066449204472));
#155833=CARTESIAN_POINT('Ctrl Pts',(-6.45063631116856,0.966746137137303,
3.65991825214105));
#155834=CARTESIAN_POINT('Ctrl Pts',(-6.37833607187544,0.953652667104105,
3.61850684058575));
#155835=CARTESIAN_POINT('Ctrl Pts',(-6.34217723114372,0.946939345906579,
3.59781746951572));
#155836=CARTESIAN_POINT('Ctrl Pts',(-6.30605549594103,0.940053949701714,
3.57717266689846));
#155837=CARTESIAN_POINT('Ctrl Pts',(-6.643644474,0.939268254,3.480228168));
#155838=CARTESIAN_POINT('Ctrl Pts',(-6.452572859,1.004934719,3.844977782));
#155839=CARTESIAN_POINT('Ctrl Pts',(-6.222719017,1.069390921,4.186617732));
#155840=CARTESIAN_POINT('Ctrl Pts',(-6.308404047,0.939268254,3.573029299));
#155841=CARTESIAN_POINT('Ctrl Pts',(-6.112237461,1.004934719,3.919373532));
#155842=CARTESIAN_POINT('Ctrl Pts',(-5.879334183,1.069390921,4.242160954));
#155843=CARTESIAN_POINT('Origin',(0.176436100079234,0.803719120296965,-0.0741246307396093));
#155844=CARTESIAN_POINT('Ctrl Pts',(-5.934877406,1.069390921,4.585545789));
#155845=CARTESIAN_POINT('Ctrl Pts',(-5.68639423,1.004503495,4.907147023));
#155846=CARTESIAN_POINT('Ctrl Pts',(-5.404614025,0.939276009000001,5.200014158));
#155847=CARTESIAN_POINT('Ctrl Pts',(-5.879334183,1.069390921,4.242160954));
#155848=CARTESIAN_POINT('Ctrl Pts',(-5.649458466,1.004503495,4.560752393));
#155849=CARTESIAN_POINT('Ctrl Pts',(-5.386501999,0.939276009000001,4.852638067));
#155850=CARTESIAN_POINT('',(-5.3896370399433,0.940053947055203,4.8491558857356));
#155851=CARTESIAN_POINT('Origin',(0.148636968835451,0.946431371091245,-0.132334142889854));
#155852=CARTESIAN_POINT('Ctrl Pts',(-5.5747932828214,0.979367659164909,
5.01713861212506));
#155853=CARTESIAN_POINT('Ctrl Pts',(-5.54392760548416,0.973133921651111,
4.98908710816583));
#155854=CARTESIAN_POINT('Ctrl Pts',(-5.51304976423055,0.966746133499498,
4.96104750887767));
#155855=CARTESIAN_POINT('Ctrl Pts',(-5.45134211096734,0.953652667146328,
4.90506187481743));
#155856=CARTESIAN_POINT('Ctrl Pts',(-5.42047624750108,0.946939346057015,
4.87708312846141));
#155857=CARTESIAN_POINT('Ctrl Pts',(-5.38963704040107,0.94005394978954,
4.84915588455596));
#155858=CARTESIAN_POINT('Ctrl Pts',(-5.74017357700001,0.939268254,4.827049544));
#155859=CARTESIAN_POINT('Ctrl Pts',(-5.475158725,1.004934719,5.142196766));
#155860=CARTESIAN_POINT('Ctrl Pts',(-5.177236248,1.069390921,5.426437582));
#155861=CARTESIAN_POINT('Ctrl Pts',(-5.392821385,0.939268254,4.845614255));
#155862=CARTESIAN_POINT('Ctrl Pts',(-5.126787292,1.004934719,5.141691134));
#155863=CARTESIAN_POINT('Ctrl Pts',(-4.829939409,1.069390921,5.406864646));
#155864=CARTESIAN_POINT('Origin',(0.156376705074808,0.803719083698706,-0.110320379162943));
#155865=CARTESIAN_POINT('Ctrl Pts',(-4.810366473,1.069390921,5.754161485));
#155866=CARTESIAN_POINT('Ctrl Pts',(-4.498557937,1.004503495,6.014827323));
#155867=CARTESIAN_POINT('Ctrl Pts',(-4.16040782,0.939276009000001,6.240272973));
#155868=CARTESIAN_POINT('Ctrl Pts',(-4.829939409,1.069390921,5.406864646));
#155869=CARTESIAN_POINT('Ctrl Pts',(-4.536950317,1.004503495,5.66859111));
#155870=CARTESIAN_POINT('Ctrl Pts',(-4.217394834,0.939276009000001,5.89712479200001));
#155871=CARTESIAN_POINT('',(-4.22120514517481,0.940053948808827,5.89439796322484));
#155872=CARTESIAN_POINT('Origin',(0.116713988276355,0.946431391368445,-0.161192793784344));
#155873=CARTESIAN_POINT('Ctrl Pts',(-4.36592121772472,0.979367659169013,
6.09825646575288));
#155874=CARTESIAN_POINT('Ctrl Pts',(-4.34180743928535,0.973133930010902,
6.06422562774249));
#155875=CARTESIAN_POINT('Ctrl Pts',(-4.31767917226086,0.966746137510712,
6.03020373075736));
#155876=CARTESIAN_POINT('Ctrl Pts',(-4.26944945116904,0.953652667121064,
5.96226166741486));
#155877=CARTESIAN_POINT('Ctrl Pts',(-4.24531981791811,0.946939346056006,
5.92830180049019));
#155878=CARTESIAN_POINT('Ctrl Pts',(-4.22120514626669,0.940053949810634,
5.89439796224477));
#155879=CARTESIAN_POINT('Ctrl Pts',(-4.568298544,0.939268254,5.948163449));
#155880=CARTESIAN_POINT('Ctrl Pts',(-4.241732254,1.004934719,6.198972345));
#155881=CARTESIAN_POINT('Ctrl Pts',(-3.889671666,1.069390921,6.412523242));
#155882=CARTESIAN_POINT('Ctrl Pts',(-4.225076389,0.939268254,5.891623674));
#155883=CARTESIAN_POINT('Ctrl Pts',(-3.901614248,1.004934719,6.123588974));
#155884=CARTESIAN_POINT('Ctrl Pts',(-3.554702037,1.069390921,6.318749356));
#155885=CARTESIAN_POINT('Origin',(0.129005056016377,0.803719098892777,-0.141357475233095));
#155886=CARTESIAN_POINT('Ctrl Pts',(-3.460928151,1.069390921,6.653718985));
#155887=CARTESIAN_POINT('Ctrl Pts',(-3.100374075,1.004503495,6.841260983));
#155888=CARTESIAN_POINT('Ctrl Pts',(-2.721665569,0.939276009000001,6.988743559));
#155889=CARTESIAN_POINT('Ctrl Pts',(-3.554702037,1.069390921,6.318749356));
#155890=CARTESIAN_POINT('Ctrl Pts',(-3.212299413,1.004503495,6.511372807));
#155891=CARTESIAN_POINT('Ctrl Pts',(-2.851086974,0.939276009000001,6.665868515));
#155892=CARTESIAN_POINT('',(-2.85539438941291,0.940053948098198,6.66402454208368));
#155893=CARTESIAN_POINT('Origin',(0.0793335642571924,0.94643133914452,-0.1825142284368));
#155894=CARTESIAN_POINT('Ctrl Pts',(-2.9529035287323,0.979367659117687,
6.89422662433445));
#155895=CARTESIAN_POINT('Ctrl Pts',(-2.93666913907019,0.97313392913207,
6.85580765366883));
#155896=CARTESIAN_POINT('Ctrl Pts',(-2.92041868086989,0.966746137072281,
6.81739430829125));
#155897=CARTESIAN_POINT('Ctrl Pts',(-2.8879220802227,0.953652667109427,
6.74067273051987));
#155898=CARTESIAN_POINT('Ctrl Pts',(-2.87165695187532,0.946939345996193,
6.70231966810689));
#155899=CARTESIAN_POINT('Ctrl Pts',(-2.85539439105084,0.940053949768782,
6.66402454108775));
#155900=CARTESIAN_POINT('Ctrl Pts',(-3.182814947,0.939268254,6.79114784200001));
#155901=CARTESIAN_POINT('Ctrl Pts',(-2.809967097,1.004934719,6.965890866));
#155902=CARTESIAN_POINT('Ctrl Pts',(-2.420230359,1.069390921,7.098766443));
#155903=CARTESIAN_POINT('Ctrl Pts',(-2.859771516,0.939268254,6.662147317));
#155904=CARTESIAN_POINT('Ctrl Pts',(-2.494006057,1.004934719,6.819154599));
#155905=CARTESIAN_POINT('Ctrl Pts',(-2.113250748,1.069390921,6.93517637));
#155906=CARTESIAN_POINT('Origin',(0.095601296301798,0.803718949325442,-0.165784735215747));
#155907=CARTESIAN_POINT('Ctrl Pts',(-1.949660675,1.069390921,7.24215598100001));
#155908=CARTESIAN_POINT('Ctrl Pts',(-1.557220167,1.004503495,7.347804883));
#155909=CARTESIAN_POINT('Ctrl Pts',(-1.155661261,0.939276009000001,7.410428264));
#155910=CARTESIAN_POINT('Ctrl Pts',(-2.113250748,1.069390921,6.93517637));
#155911=CARTESIAN_POINT('Ctrl Pts',(-1.73744496,1.004503495,7.049689948));
#155912=CARTESIAN_POINT('Ctrl Pts',(-1.351465456,0.939276009000001,7.122923636));
#155913=CARTESIAN_POINT('',(-1.35606856648097,0.940053947035547,7.1220487401457));
#155914=CARTESIAN_POINT('Origin',(0.0382436804210429,0.946431393530997,
-0.195301735553574));
#155915=CARTESIAN_POINT('Ctrl Pts',(-1.40181135298697,0.979367659138296,
7.36783040874983));
#155916=CARTESIAN_POINT('Ctrl Pts',(-1.3942154481657,0.973133921591531,
7.32681968872295));
#155917=CARTESIAN_POINT('Ctrl Pts',(-1.38660265533696,0.966746133408986,
7.28581108465508));
#155918=CARTESIAN_POINT('Ctrl Pts',(-1.37135868269623,0.953652667065727,
7.20389742909375));
#155919=CARTESIAN_POINT('Ctrl Pts',(-1.36371859852421,0.946939345797094,
7.162944517369));
#155920=CARTESIAN_POINT('Ctrl Pts',(-1.35606856762555,0.940053949578423,
7.12204873950346));
#155921=CARTESIAN_POINT('Ctrl Pts',(-1.648506461,0.939268254,7.31658571));
#155922=CARTESIAN_POINT('Ctrl Pts',(-1.246811002,1.004934719,7.407092072));
#155923=CARTESIAN_POINT('Ctrl Pts',(-0.837621771,1.069390921,7.453079214));
#155924=CARTESIAN_POINT('Ctrl Pts',(-1.360746905,0.939268254,7.121156357));
#155925=CARTESIAN_POINT('Ctrl Pts',(-0.969780916,1.004934719,7.195864134));
#155926=CARTESIAN_POINT('Ctrl Pts',(-0.572986203,1.069390921,7.227322244));
#155927=CARTESIAN_POINT('Origin',(0.0577273861487002,0.803719070356922,
-0.182460475737256));
#155928=CARTESIAN_POINT('Ctrl Pts',(-0.347229232,1.069390921,7.491957812));
#155929=CARTESIAN_POINT('Ctrl Pts',(0.058747626,1.004503495,7.510773593));
#155930=CARTESIAN_POINT('Ctrl Pts',(0.464380483,0.939276009000001,7.485609579));
#155931=CARTESIAN_POINT('Ctrl Pts',(-0.572986203,1.069390921,7.227322244));
#155932=CARTESIAN_POINT('Ctrl Pts',(-0.181349511,1.004503495,7.258371422));
#155933=CARTESIAN_POINT('Ctrl Pts',(0.211349085,0.939276009000001,7.24691876300001));
#155934=CARTESIAN_POINT('Origin',(-0.00463470785240436,0.946431364356144,
-0.198957029881124));
#155935=CARTESIAN_POINT('Ctrl Pts',(-1.35877392498063,4.81811592995236,
7.12153743297961));
#155936=CARTESIAN_POINT('Ctrl Pts',(-1.35490612249032,4.81875342547618,
7.1222710489898));
#155937=CARTESIAN_POINT('Ctrl Pts',(-1.35103832,4.819390921,7.123004665));
#155938=CARTESIAN_POINT('Ctrl Pts',(-1.344855702,4.820409947,7.12417733800001));
#155939=CARTESIAN_POINT('Ctrl Pts',(-1.338671059,4.821428571,7.125339276));
#155940=CARTESIAN_POINT('Ctrl Pts',(-0.955718432,4.884501699,7.19728639));
#155941=CARTESIAN_POINT('Ctrl Pts',(-0.567260438,4.948754474,7.227773903));
#155942=CARTESIAN_POINT('Ctrl Pts',(-1.21606691400034,4.81811592995236,
7.33154082511742));
#155943=CARTESIAN_POINT('Ctrl Pts',(-1.21208516350017,4.81875342547618,
7.33219682755871));
#155944=CARTESIAN_POINT('Ctrl Pts',(-1.208103413,4.819390921,7.33285283));
#155945=CARTESIAN_POINT('Ctrl Pts',(-1.201738651,4.820409947,7.333901439));
#155946=CARTESIAN_POINT('Ctrl Pts',(-1.195372079,4.821428571,7.334938996));
#155947=CARTESIAN_POINT('Ctrl Pts',(-0.801154479,4.884501699,7.399184481));
#155948=CARTESIAN_POINT('Ctrl Pts',(-0.402321868,4.948754474,7.420807342));
#155949=CARTESIAN_POINT('',(-0.57198312172941,4.94797310013266,7.22740172850988));
#155950=CARTESIAN_POINT('Origin',(-0.00829022335223695,5.08885443639218,
-0.190840199381178));
#155951=CARTESIAN_POINT('Ctrl Pts',(-0.571982217557311,4.94797287193578,
7.22740176977812));
#155952=CARTESIAN_POINT('Ctrl Pts',(-0.573456838245926,4.94458997048659,
7.24802737088461));
#155953=CARTESIAN_POINT('Ctrl Pts',(-0.574945447045747,4.94124830640299,
7.26865888388256));
#155954=CARTESIAN_POINT('Ctrl Pts',(-0.576449088949175,4.93794661992768,
7.28929564968059));
#155955=CARTESIAN_POINT('Ctrl Pts',(-2.16235458594344,4.95685569181143,
6.91814254814242));
#155956=CARTESIAN_POINT('Ctrl Pts',(-1.76154032246365,4.88876675985096,
7.04342220983006));
#155957=CARTESIAN_POINT('Ctrl Pts',(-1.34893983835,4.819390921,7.12157531593001));
#155958=CARTESIAN_POINT('Ctrl Pts',(-1.3218087413993,4.8148290198817,7.12671437800155));
#155959=CARTESIAN_POINT('Ctrl Pts',(-1.2946776444487,4.81026711876327,7.13185344007204));
#155960=CARTESIAN_POINT('Ctrl Pts',(-2.16460409637423,4.95685569181143,
6.91931998895273));
#155961=CARTESIAN_POINT('Ctrl Pts',(-1.76372161586533,4.88876675985096,
7.04472997983171));
#155962=CARTESIAN_POINT('Ctrl Pts',(-1.35103832,4.819390921,7.123004665));
#155963=CARTESIAN_POINT('Ctrl Pts',(-1.32390177765177,4.8148290198817,7.12815172166587));
#155964=CARTESIAN_POINT('Ctrl Pts',(-1.29676523530354,4.81026711876327,
7.13329877833112));
#155965=CARTESIAN_POINT('Ctrl Pts',(-2.38955513945283,4.95685569181143,
7.03706406998286));
#155966=CARTESIAN_POINT('Ctrl Pts',(-1.98185095603346,4.88876675985096,
7.17550697999575));
#155967=CARTESIAN_POINT('Ctrl Pts',(-1.560886485,4.819390921,7.265939572));
#155968=CARTESIAN_POINT('Ctrl Pts',(-1.53320540289719,4.8148290198817,7.27188608809886));
#155969=CARTESIAN_POINT('Ctrl Pts',(-1.50552432079462,4.81026711876327,
7.27783260419724));
#155970=CARTESIAN_POINT('',(-2.11228819893379,4.94797311771878,6.93546962696871));
#155971=CARTESIAN_POINT('Origin',(0.0156522182859661,4.69654718398349,-0.1918471612771));
#155972=CARTESIAN_POINT('Ctrl Pts',(-2.12995512149651,4.93794661942987,
6.9949564549365));
#155973=CARTESIAN_POINT('Ctrl Pts',(-2.12405034199266,4.94124830642815,
6.97512540270629));
#155974=CARTESIAN_POINT('Ctrl Pts',(-2.11816137081836,4.94458997052876,
6.95529624952042));
#155975=CARTESIAN_POINT('Ctrl Pts',(-2.1122872006493,4.94797287203487,6.93546979394767));
#155976=CARTESIAN_POINT('Ctrl Pts',(-2.85886884210992,4.81811592995234,
6.66058590328662));
#155977=CARTESIAN_POINT('Ctrl Pts',(-2.85525045263496,4.81875342547617,
6.6621343435833));
#155978=CARTESIAN_POINT('Ctrl Pts',(-2.85163206316,4.81939092100001,6.66368278388));
#155979=CARTESIAN_POINT('Ctrl Pts',(-2.84584812772,4.820409947,6.66615793995999));
#155980=CARTESIAN_POINT('Ctrl Pts',(-2.84005990385,4.821428571,6.66862305261));
#155981=CARTESIAN_POINT('Ctrl Pts',(-2.48165357213,4.884501699,6.82126257693001));
#155982=CARTESIAN_POINT('Ctrl Pts',(-2.10895180115,4.948754474,6.93460856659));
#155983=CARTESIAN_POINT('Ctrl Pts',(-2.85792658132591,4.81811592995234,
6.66294361747922));
#155984=CARTESIAN_POINT('Ctrl Pts',(-2.85430691216296,4.81875342547617,
6.66449154473961));
#155985=CARTESIAN_POINT('Ctrl Pts',(-2.850687243,4.81939092100001,6.666039472));
#155986=CARTESIAN_POINT('Ctrl Pts',(-2.844901262,4.820409947,6.668513808));
#155987=CARTESIAN_POINT('Ctrl Pts',(-2.839110994,4.821428571,6.670978097));
#155988=CARTESIAN_POINT('Ctrl Pts',(-2.48057809,4.884501699,6.823566622));
#155989=CARTESIAN_POINT('Ctrl Pts',(-2.107755942,4.948754474,6.93684834));
#155990=CARTESIAN_POINT('Ctrl Pts',(-2.76370050292588,4.81811592995234,
6.89871503673933));
#155991=CARTESIAN_POINT('Ctrl Pts',(-2.75995286496294,4.81875342547617,
6.90021166036967));
#155992=CARTESIAN_POINT('Ctrl Pts',(-2.756205227,4.81939092100001,6.901708284));
#155993=CARTESIAN_POINT('Ctrl Pts',(-2.75021469,4.820409947,6.904100612));
#155994=CARTESIAN_POINT('Ctrl Pts',(-2.744220009,4.821428571,6.906482536));
#155995=CARTESIAN_POINT('Ctrl Pts',(-2.373029877,4.884501699,7.053971129));
#155996=CARTESIAN_POINT('Ctrl Pts',(-1.988170027,4.948754474,7.160825681));
#155997=CARTESIAN_POINT('Origin',(0.0329293447624329,5.08885503540763,-0.188162932465979));
#155998=CARTESIAN_POINT('Ctrl Pts',(-3.59899609457623,4.95685569337321,
6.29155789759412));
#155999=CARTESIAN_POINT('Ctrl Pts',(-3.23448406651575,4.88876676064928,
6.50007181265036));
#156000=CARTESIAN_POINT('Ctrl Pts',(-2.84833055488,4.819390921,6.66509465184));
#156001=CARTESIAN_POINT('Ctrl Pts',(-2.82293850999083,4.81482901910993,
6.67594595116572));
#156002=CARTESIAN_POINT('Ctrl Pts',(-2.79754646510191,4.81026711721972,
6.6867972504915));
#156003=CARTESIAN_POINT('Ctrl Pts',(-3.60144612767277,4.95685569337321,
6.29222423224807));
#156004=CARTESIAN_POINT('Ctrl Pts',(-3.23689549438232,4.88876676064928,
6.50088009410198));
#156005=CARTESIAN_POINT('Ctrl Pts',(-2.850687243,4.819390921,6.666039472));
#156006=CARTESIAN_POINT('Ctrl Pts',(-2.82529159862497,4.81482901910993,
6.67689974961262));
#156007=CARTESIAN_POINT('Ctrl Pts',(-2.79989595425014,4.81026711721972,
6.68776002722526));
#156008=CARTESIAN_POINT('Ctrl Pts',(-3.84644943732711,4.95685569337321,
6.35885769764247));
#156009=CARTESIAN_POINT('Ctrl Pts',(-3.47803828103868,4.88876676064928,
6.58170823926466));
#156010=CARTESIAN_POINT('Ctrl Pts',(-3.086356055,4.819390921,6.76052148800001));
#156011=CARTESIAN_POINT('Ctrl Pts',(-3.06060046203974,4.81482901910993,
6.77227959430188));
#156012=CARTESIAN_POINT('Ctrl Pts',(-3.03484486907951,4.81026711721972,
6.78403770060382));
#156013=CARTESIAN_POINT('',(-3.55382503325055,4.9479731176806,6.31924267752363));
#156014=CARTESIAN_POINT('Origin',(0.0565277989466323,4.69654717972231,-0.18399723361456));
#156015=CARTESIAN_POINT('Ctrl Pts',(-3.58386682219125,4.93794661934438,
6.37354087035044));
#156016=CARTESIAN_POINT('Ctrl Pts',(-3.57383700388081,4.94124830645077,
6.35544280984233));
#156017=CARTESIAN_POINT('Ctrl Pts',(-3.56382303182418,4.9445899705472,6.3373432059445));
#156018=CARTESIAN_POINT('Ctrl Pts',(-3.55382409446741,4.9479728720179,6.31924305487698));
#156019=CARTESIAN_POINT('Ctrl Pts',(-4.22385916096707,4.81811592995213,
5.89029281182821));
#156020=CARTESIAN_POINT('Ctrl Pts',(-4.22065823623853,4.81875342547606,
5.89258289768411));
#156021=CARTESIAN_POINT('Ctrl Pts',(-4.21745731151,4.819390921,5.89487298353999));
#156022=CARTESIAN_POINT('Ctrl Pts',(-4.21234068653,4.820409947,5.89853364772001));
#156023=CARTESIAN_POINT('Ctrl Pts',(-4.20721771493,4.821428571,5.90218542367));
#156024=CARTESIAN_POINT('Ctrl Pts',(-3.89000370937,4.884501699,6.12830308735));
#156025=CARTESIAN_POINT('Ctrl Pts',(-3.55038153655001,4.948754474,6.31911897488));
#156026=CARTESIAN_POINT('Ctrl Pts',(-4.22344576856042,4.81811592995213,
5.89279796219157));
#156027=CARTESIAN_POINT('Ctrl Pts',(-4.22024348378021,4.81875342547606,
5.89508782209578));
#156028=CARTESIAN_POINT('Ctrl Pts',(-4.217041199,4.819390921,5.897377682));
#156029=CARTESIAN_POINT('Ctrl Pts',(-4.2119224,4.820409947,5.90103798500001));
#156030=CARTESIAN_POINT('Ctrl Pts',(-4.206797255,4.821428571,5.904689396));
#156031=CARTESIAN_POINT('Ctrl Pts',(-3.889448673,4.884501699,6.130784462));
#156032=CARTESIAN_POINT('Ctrl Pts',(-3.549695121,4.948754474,6.321563458));
#156033=CARTESIAN_POINT('Ctrl Pts',(-4.18210652789557,4.81811592995213,
6.14331299852691));
#156034=CARTESIAN_POINT('Ctrl Pts',(-4.17876823794779,4.81875342547606,
6.14558026326346));
#156035=CARTESIAN_POINT('Ctrl Pts',(-4.175429948,4.819390921,6.147847528));
#156036=CARTESIAN_POINT('Ctrl Pts',(-4.170093747,4.820409947,6.151471713));
#156037=CARTESIAN_POINT('Ctrl Pts',(-4.164751262,4.821428571,6.155086629));
#156038=CARTESIAN_POINT('Ctrl Pts',(-3.833945036,4.884501699,6.378921927));
#156039=CARTESIAN_POINT('Ctrl Pts',(-3.481053566,4.948754474,6.56601177));
#156040=CARTESIAN_POINT('Origin',(0.0726090705661236,5.08885504255354,-0.176685151946212));
#156041=CARTESIAN_POINT('Ctrl Pts',(-4.86735251457583,4.95685568844401,
5.37078701507674));
#156042=CARTESIAN_POINT('Ctrl Pts',(-4.55618691247175,4.88876675812967,
5.65278529087343));
#156043=CARTESIAN_POINT('Ctrl Pts',(-4.21453650053,4.819390921,5.89696156949));
#156044=CARTESIAN_POINT('Ctrl Pts',(-4.19207081821782,4.81482901952818,
5.91301770907552));
#156045=CARTESIAN_POINT('Ctrl Pts',(-4.1696051359056,4.81026711805618,5.92907384866106));
#156046=CARTESIAN_POINT('Ctrl Pts',(-4.86988850951164,4.95685568844401,
5.3709110865213));
#156047=CARTESIAN_POINT('Ctrl Pts',(-4.55871571911483,4.88876675812967,
5.6530562894507));
#156048=CARTESIAN_POINT('Ctrl Pts',(-4.217041199,4.819390921,5.897377682));
#156049=CARTESIAN_POINT('Ctrl Pts',(-4.19457393142246,4.81482901952818,
5.91344336374728));
#156050=CARTESIAN_POINT('Ctrl Pts',(-4.17210666384516,4.81026711805618,
5.92950904549473));
#156051=CARTESIAN_POINT('Ctrl Pts',(-5.12348800309282,4.95685568844401,
5.38331823097723));
#156052=CARTESIAN_POINT('Ctrl Pts',(-4.81159638342372,4.88876675812967,
5.68015614717736));
#156053=CARTESIAN_POINT('Ctrl Pts',(-4.467511046,4.819390921,5.938988933));
#156054=CARTESIAN_POINT('Ctrl Pts',(-4.44488525188809,4.81482901952818,
5.95600883092791));
#156055=CARTESIAN_POINT('Ctrl Pts',(-4.42225945777601,4.81026711805618,
5.9730287288553));
#156056=CARTESIAN_POINT('',(-4.82918895415257,4.94797309993411,5.40753499076431));
#156057=CARTESIAN_POINT('Origin',(0.094760193322927,4.69654721337739,-0.167543692837909));
#156058=CARTESIAN_POINT('Ctrl Pts',(-4.87020089538197,4.9379466194895,5.45410559722007));
#156059=CARTESIAN_POINT('Ctrl Pts',(-4.8565150415706,4.94124830103405,5.43858679968498));
#156060=CARTESIAN_POINT('Ctrl Pts',(-4.84284433309257,4.94458995962699,
5.42306308763061));
#156061=CARTESIAN_POINT('Ctrl Pts',(-4.82918818983745,4.94797285533979,
5.40753560967742));
#156062=CARTESIAN_POINT('Ctrl Pts',(-5.39134652093208,4.81811592995213,
4.84457617665));
#156063=CARTESIAN_POINT('Ctrl Pts',(-5.38871273241604,4.81875342547607,
4.847500825375));
#156064=CARTESIAN_POINT('Ctrl Pts',(-5.3860789439,4.819390921,4.85042547409999));
#156065=CARTESIAN_POINT('Ctrl Pts',(-5.38186887673,4.820409947,4.85510047648001));
#156066=CARTESIAN_POINT('Ctrl Pts',(-5.37765070077,4.821428571,4.85976816369));
#156067=CARTESIAN_POINT('Ctrl Pts',(-5.11646159673,4.884501699,5.14879095710001));
#156068=CARTESIAN_POINT('Ctrl Pts',(-4.82579937693,4.948754474,5.40815440248));
#156069=CARTESIAN_POINT('Ctrl Pts',(-5.39148132667972,4.81811592995213,
4.84711162513907));
#156070=CARTESIAN_POINT('Ctrl Pts',(-5.38884616133986,4.81875342547607,
4.85003634556953));
#156071=CARTESIAN_POINT('Ctrl Pts',(-5.386210996,4.819390921,4.852961066));
#156072=CARTESIAN_POINT('Ctrl Pts',(-5.381998728,4.820409947,4.857636183));
#156073=CARTESIAN_POINT('Ctrl Pts',(-5.377778351,4.821428571,4.862303981));
#156074=CARTESIAN_POINT('Ctrl Pts',(-5.116452959,4.884501699,5.151333635));
#156075=CARTESIAN_POINT('Ctrl Pts',(-4.825654501,4.948754474,5.410689294));
#156076=CARTESIAN_POINT('Ctrl Pts',(-5.4049619014445,4.81811592995213,5.10065647404533));
#156077=CARTESIAN_POINT('Ctrl Pts',(-5.40218905372225,4.81875342547607,
5.10358836502267));
#156078=CARTESIAN_POINT('Ctrl Pts',(-5.399416206,4.819390921,5.10652025600001));
#156079=CARTESIAN_POINT('Ctrl Pts',(-5.394983855,4.820409947,5.111206835));
#156080=CARTESIAN_POINT('Ctrl Pts',(-5.390543374,4.821428571,5.115885712));
#156081=CARTESIAN_POINT('Ctrl Pts',(-5.115589186,4.884501699,5.405601425));
#156082=CARTESIAN_POINT('Ctrl Pts',(-4.811166908,4.948754474,5.664178446));
#156083=CARTESIAN_POINT('Origin',(0.108891420928572,5.08885434269428,-0.156943200427216));
#156084=CARTESIAN_POINT('Ctrl Pts',(-5.90811696378675,4.95685568770243,
4.19888409086371));
#156085=CARTESIAN_POINT('Ctrl Pts',(-5.66484753557328,4.88876675775061,
4.54118080731132));
#156086=CARTESIAN_POINT('Ctrl Pts',(-5.38367540411,4.819390921,4.85309311810001));
#156087=CARTESIAN_POINT('Ctrl Pts',(-5.36518655435748,4.81482902001977,
4.87360332947881));
#156088=CARTESIAN_POINT('Ctrl Pts',(-5.34669770460441,4.81026711903938,
4.89411354085806));
#156089=CARTESIAN_POINT('Ctrl Pts',(-5.91062034026415,4.95685568770243,
4.19846009763442));
#156090=CARTESIAN_POINT('Ctrl Pts',(-5.66737547681082,4.88876675775061,
4.54090185142077));
#156091=CARTESIAN_POINT('Ctrl Pts',(-5.386210996,4.819390921,4.852961066));
#156092=CARTESIAN_POINT('Ctrl Pts',(-5.36772264932633,4.81482902001977,
4.87348093723415));
#156093=CARTESIAN_POINT('Ctrl Pts',(-5.34923430265263,4.81026711903938,
4.89400080846849));
#156094=CARTESIAN_POINT('Ctrl Pts',(-6.16095798800407,4.95685568770243,
4.15606077470563));
#156095=CARTESIAN_POINT('Ctrl Pts',(-5.92016960056519,4.88876675775061,
4.51300626236517));
#156096=CARTESIAN_POINT('Ctrl Pts',(-5.63977018500001,4.819390921,4.839755856));
#156097=CARTESIAN_POINT('Ctrl Pts',(-5.6213321462153,4.81482902001977,4.86124171276682));
#156098=CARTESIAN_POINT('Ctrl Pts',(-5.6028941074302,4.81026711903938,4.8827275695335));
#156099=CARTESIAN_POINT('',(-5.87874536368429,4.94797309819258,4.24297694153243));
#156100=CARTESIAN_POINT('Origin',(0.128561535844363,4.69654720238666,-0.143255839490103));
#156101=CARTESIAN_POINT('Ctrl Pts',(-5.92880978556242,4.93794661941978,
4.27964240952211));
#156102=CARTESIAN_POINT('Ctrl Pts',(-5.91210778970961,4.94124830639064,
4.267428466771));
#156103=CARTESIAN_POINT('Ctrl Pts',(-5.89541952835817,4.94458997046672,
4.25520646896433));
#156104=CARTESIAN_POINT('Ctrl Pts',(-5.878744682587,4.94797287194661,4.24297766149803));
#156105=CARTESIAN_POINT('Ctrl Pts',(-6.306740508148,4.81811592995213,3.57233254198123));
#156106=CARTESIAN_POINT('Ctrl Pts',(-6.30479700952399,4.81875342547606,
3.57575500105562));
#156107=CARTESIAN_POINT('Ctrl Pts',(-6.3028535109,4.819390921,3.57917746013));
#156108=CARTESIAN_POINT('Ctrl Pts',(-6.29974686065001,4.820409947,3.58464820408));
#156109=CARTESIAN_POINT('Ctrl Pts',(-6.2966307174,4.821428571,3.59011354672));
#156110=CARTESIAN_POINT('Ctrl Pts',(-6.10367942619001,4.884501699,3.92852708364));
#156111=CARTESIAN_POINT('Ctrl Pts',(-5.87556820104999,4.948754474,4.2443105418));
#156112=CARTESIAN_POINT('Ctrl Pts',(-6.30741720870541,4.81811592995213,
3.57477973384487));
#156113=CARTESIAN_POINT('Ctrl Pts',(-6.30547238085271,4.81875342547606,
3.57820255892243));
#156114=CARTESIAN_POINT('Ctrl Pts',(-6.303527553,4.819390921,3.581625384));
#156115=CARTESIAN_POINT('Ctrl Pts',(-6.300418778,4.820409947,3.587096713));
#156116=CARTESIAN_POINT('Ctrl Pts',(-6.297300509,4.821428571,3.592562637));
#156117=CARTESIAN_POINT('Ctrl Pts',(-6.104217591,4.884501699,3.931012172));
#156118=CARTESIAN_POINT('Ctrl Pts',(-5.875971639,4.948754474,4.246817313));
#156119=CARTESIAN_POINT('Ctrl Pts',(-6.37508726444723,4.81811592995213,
3.81949892020891));
#156120=CARTESIAN_POINT('Ctrl Pts',(-6.37300951372361,4.81875342547606,
3.82295834560446));
#156121=CARTESIAN_POINT('Ctrl Pts',(-6.370931763,4.819390921,3.826417771));
#156122=CARTESIAN_POINT('Ctrl Pts',(-6.367610513,4.820409947,3.831947605));
#156123=CARTESIAN_POINT('Ctrl Pts',(-6.364279669,4.821428571,3.837471665));
#156124=CARTESIAN_POINT('Ctrl Pts',(-6.158034072,4.884501699,4.179521008));
#156125=CARTESIAN_POINT('Ctrl Pts',(-5.916315434,4.948754474,4.497494433));
#156126=CARTESIAN_POINT('Origin',(0.140086370307819,5.0888550933578,-0.129867356607448));
#156127=CARTESIAN_POINT('Ctrl Pts',(-6.67262443499624,4.95685568835189,
2.83064600545431));
#156128=CARTESIAN_POINT('Ctrl Pts',(-6.50862618644082,4.88876675808259,
3.21723575405344));
#156129=CARTESIAN_POINT('Ctrl Pts',(-6.30107962914,4.819390921,3.5822994261));
#156130=CARTESIAN_POINT('Ctrl Pts',(-6.28743212615761,4.81482901953652,
3.60630467879053));
#156131=CARTESIAN_POINT('Ctrl Pts',(-6.27378462317401,4.81026711807287,
3.6303099314808));
#156132=CARTESIAN_POINT('Ctrl Pts',(-6.67497813791429,4.95685568835189,
2.82969377301616));
#156133=CARTESIAN_POINT('Ctrl Pts',(-6.51103505853922,4.88876675808259,
3.21641988734669));
#156134=CARTESIAN_POINT('Ctrl Pts',(-6.303527553,4.819390921,3.581625384));
#156135=CARTESIAN_POINT('Ctrl Pts',(-6.28988261791864,4.81482901953652,
3.60563996255826));
#156136=CARTESIAN_POINT('Ctrl Pts',(-6.27623768283663,4.81026711807287,
3.62965454111647));
#156137=CARTESIAN_POINT('Ctrl Pts',(-6.91034842971931,4.95685568835189,
2.73447052920114));
#156138=CARTESIAN_POINT('Ctrl Pts',(-6.75192226837977,4.88876675808259,
3.13483321667203));
#156139=CARTESIAN_POINT('Ctrl Pts',(-6.548319939,4.819390921,3.514221174));
#156140=CARTESIAN_POINT('Ctrl Pts',(-6.53493179402859,4.81482901953652,
3.5391683393324));
#156141=CARTESIAN_POINT('Ctrl Pts',(-6.52154364905773,4.81026711807287,
3.56411550466487));
#156142=CARTESIAN_POINT('',(-6.65341820032519,4.94797309994886,2.88002202749723));
#156143=CARTESIAN_POINT('Origin',(0.156351623027657,4.69654720595462,-0.112269673876696));
#156144=CARTESIAN_POINT('Ctrl Pts',(-6.71019411991621,4.93794661929365,
2.90506789926301));
#156145=CARTESIAN_POINT('Ctrl Pts',(-6.69125700190066,4.94124830104398,
2.8967299597595));
#156146=CARTESIAN_POINT('Ctrl Pts',(-6.67233156532678,4.94458995962745,
2.88838120181602));
#156147=CARTESIAN_POINT('Ctrl Pts',(-6.65341776657222,4.94797285537006,
2.88002291003781));
#156148=CARTESIAN_POINT('Ctrl Pts',(-6.92723831926984,4.81811592995213,
2.13305060920743));
#156149=CARTESIAN_POINT('Ctrl Pts',(-6.92607598581492,4.81875342547607,
2.13681084778371));
#156150=CARTESIAN_POINT('Ctrl Pts',(-6.92491365236001,4.819390921,2.14057108636));
#156151=CARTESIAN_POINT('Ctrl Pts',(-6.92305568165001,4.820409947,2.14658176523));
#156152=CARTESIAN_POINT('Ctrl Pts',(-6.92118727974,4.821428571,2.15258920948));
#156153=CARTESIAN_POINT('Ctrl Pts',(-6.80549598965,4.884501699,2.52456965116));
#156154=CARTESIAN_POINT('Ctrl Pts',(-6.6506019875,4.948754474,2.88200743695));
#156155=CARTESIAN_POINT('Ctrl Pts',(-6.92842527283416,4.81811592995213,
2.13529511646558));
#156156=CARTESIAN_POINT('Ctrl Pts',(-6.92726171991708,4.81875342547607,
2.13905599823279));
#156157=CARTESIAN_POINT('Ctrl Pts',(-6.926098167,4.819390921,2.14281688));
#156158=CARTESIAN_POINT('Ctrl Pts',(-6.924238247,4.820409947,2.148828587));
#156159=CARTESIAN_POINT('Ctrl Pts',(-6.922367894,4.821428571,2.154837056));
#156160=CARTESIAN_POINT('Ctrl Pts',(-6.806555793,4.884501699,2.52688095));
#156161=CARTESIAN_POINT('Ctrl Pts',(-6.651534875,4.948754474,2.884368874));
#156162=CARTESIAN_POINT('Ctrl Pts',(-7.04712062926671,4.81811592995213,
2.35974584228107));
#156163=CARTESIAN_POINT('Ctrl Pts',(-7.04583513013336,4.81875342547607,
2.36357104314054));
#156164=CARTESIAN_POINT('Ctrl Pts',(-7.04454963100001,4.819390921,2.367396244));
#156165=CARTESIAN_POINT('Ctrl Pts',(-7.042494782,4.820409947,2.373510764));
#156166=CARTESIAN_POINT('Ctrl Pts',(-7.04042932,4.821428571,2.379621708));
#156167=CARTESIAN_POINT('Ctrl Pts',(-6.91253612799999,4.884501699,2.758010834));
#156168=CARTESIAN_POINT('Ctrl Pts',(-6.744823625,4.948754474,3.120512579));
#156169=CARTESIAN_POINT('Origin',(0.164726360945872,5.08885438716697,-0.0967156443673012));
#156170=CARTESIAN_POINT('Ctrl Pts',(-7.12512740838388,4.95685569400282,
1.33005002914295));
#156171=CARTESIAN_POINT('Ctrl Pts',(-7.04806871480836,4.88876676097111,
1.74285631658049));
#156172=CARTESIAN_POINT('Ctrl Pts',(-6.92385237336,4.819390921,2.14400139464));
#156173=CARTESIAN_POINT('Ctrl Pts',(-6.91568435966481,4.81482901872219,
2.17037923231526));
#156174=CARTESIAN_POINT('Ctrl Pts',(-6.90751634597049,4.81026711644424,
2.19675706999057));
#156175=CARTESIAN_POINT('Ctrl Pts',(-7.12722138118998,4.95685569400282,
1.32861408279614));
#156176=CARTESIAN_POINT('Ctrl Pts',(-7.05024588158478,4.88876676097111,
1.74154168808874));
#156177=CARTESIAN_POINT('Ctrl Pts',(-6.926098167,4.819390921,2.14281688));
#156178=CARTESIAN_POINT('Ctrl Pts',(-6.91793466595719,4.81482901872219,
2.16920327348772));
#156179=CARTESIAN_POINT('Ctrl Pts',(-6.90977116491436,4.81026711644424,
2.19558966697542));
#156180=CARTESIAN_POINT('Ctrl Pts',(-7.3366186618006,4.95685569400282,1.18501944811523));
#156181=CARTESIAN_POINT('Ctrl Pts',(-7.26796255922654,4.88876676097111,
1.61007883891379));
#156182=CARTESIAN_POINT('Ctrl Pts',(-7.150677531,4.819390921,2.024365416));
#156183=CARTESIAN_POINT('Ctrl Pts',(-7.14296529518933,4.81482901872219,
2.05160739073463));
#156184=CARTESIAN_POINT('Ctrl Pts',(-7.13525305937811,4.81026711644424,
2.07884936546924));
#156185=CARTESIAN_POINT('',(-7.11698457125967,4.94797311770983,1.38240044863595));
#156186=CARTESIAN_POINT('Origin',(0.17683115899466,4.69654717205242,-0.0760339757490586));
#156187=CARTESIAN_POINT('Ctrl Pts',(-7.17781723575636,4.93794661952795,
1.39465564104632));
#156188=CARTESIAN_POINT('Ctrl Pts',(-7.15753041337576,4.94124830639808,
1.39058355349331));
#156189=CARTESIAN_POINT('Ctrl Pts',(-7.13725267401122,4.94458997048373,
1.38649838771534));
#156190=CARTESIAN_POINT('Ctrl Pts',(-7.11698425112877,4.94797287196985,
1.38240140852592));
#156191=CARTESIAN_POINT('Ctrl Pts',(-7.22382616583707,4.8181159299523,0.594029601741248));
#156192=CARTESIAN_POINT('Ctrl Pts',(-7.22349934711854,4.81875342547615,
0.597951795075624));
#156193=CARTESIAN_POINT('Ctrl Pts',(-7.22317252840001,4.819390921,0.60187398841));
#156194=CARTESIAN_POINT('Ctrl Pts',(-7.22265011411001,4.820409947,0.60814354927));
#156195=CARTESIAN_POINT('Ctrl Pts',(-7.22211681729,4.821428571,0.61441219304));
#156196=CARTESIAN_POINT('Ctrl Pts',(-7.18909512433,4.884501699,1.00256614643));
#156197=CARTESIAN_POINT('Ctrl Pts',(-7.11466101674,4.948754474,1.38494486827));
#156198=CARTESIAN_POINT('Ctrl Pts',(-7.22546787182024,4.8181159299523,0.595966473718428));
#156199=CARTESIAN_POINT('Ctrl Pts',(-7.22514000041012,4.81875342547615,
0.599889557359214));
#156200=CARTESIAN_POINT('Ctrl Pts',(-7.22481212900001,4.819390921,0.603812641));
#156201=CARTESIAN_POINT('Ctrl Pts',(-7.224288032,4.820409947,0.610083625));
#156202=CARTESIAN_POINT('Ctrl Pts',(-7.22375305,4.821428571,0.616353689));
#156203=CARTESIAN_POINT('Ctrl Pts',(-7.190627011,4.884501699,1.004595582));
#156204=CARTESIAN_POINT('Ctrl Pts',(-7.116079733,4.948754474,1.387050553));
#156205=CARTESIAN_POINT('Ctrl Pts',(-7.3896384701368,4.8181159299523,0.789653671436417));
#156206=CARTESIAN_POINT('Ctrl Pts',(-7.3892053295684,4.81875342547615,0.793665785718209));
#156207=CARTESIAN_POINT('Ctrl Pts',(-7.388772189,4.819390921,0.7976779));
#156208=CARTESIAN_POINT('Ctrl Pts',(-7.388079821,4.820409947,0.804091198));
#156209=CARTESIAN_POINT('Ctrl Pts',(-7.387376321,4.821428571,0.810503285));
#156210=CARTESIAN_POINT('Ctrl Pts',(-7.343815678,4.884501699,1.207539139));
#156211=CARTESIAN_POINT('Ctrl Pts',(-7.257951359,4.948754474,1.597619026));
#156212=CARTESIAN_POINT('Origin',(0.181669057018288,5.08885504760921,-0.0590436952889718));
#156213=CARTESIAN_POINT('Ctrl Pts',(-7.24446733055631,4.95685568893944,
-0.232737546559316));
#156214=CARTESIAN_POINT('Ctrl Pts',(-7.25795137311849,4.88876675838292,
0.186982886110066));
#156215=CARTESIAN_POINT('Ctrl Pts',(-7.22287347641,4.819390921,0.605452241600001));
#156216=CARTESIAN_POINT('Ctrl Pts',(-7.22056688208267,4.81482901940451,
0.632969257502106));
#156217=CARTESIAN_POINT('Ctrl Pts',(-7.21826028775529,4.81026711780884,
0.660486273404169));
#156218=CARTESIAN_POINT('Ctrl Pts',(-7.24620366143262,4.95685568893944,
-0.234590063517152));
#156219=CARTESIAN_POINT('Ctrl Pts',(-7.25979503268815,4.88876675838292,
0.185230966400782));
#156220=CARTESIAN_POINT('Ctrl Pts',(-7.224812129,4.819390921,0.603812641));
#156221=CARTESIAN_POINT('Ctrl Pts',(-7.22251178106663,4.81482901940451,
0.631337042596366));
#156222=CARTESIAN_POINT('Ctrl Pts',(-7.2202114331332,4.81026711780884,0.658861444192682));
#156223=CARTESIAN_POINT('Ctrl Pts',(-7.41983674906335,4.95685568893944,
-0.419841759300748));
#156224=CARTESIAN_POINT('Ctrl Pts',(-7.44416098965419,4.88876675838292,
0.0100389954723747));
#156225=CARTESIAN_POINT('Ctrl Pts',(-7.418677388,4.819390921,0.439852581));
#156226=CARTESIAN_POINT('Ctrl Pts',(-7.41700167946185,4.81482901940451,
0.468115552022235));
#156227=CARTESIAN_POINT('Ctrl Pts',(-7.41532597092326,4.81026711780884,
0.496378523044461));
#156228=CARTESIAN_POINT('',(-7.24776867689946,4.94797309998237,-0.179860590483462));
#156229=CARTESIAN_POINT('Origin',(0.18904191733669,4.69654715983599,-0.0362428711872403));
#156230=CARTESIAN_POINT('Ctrl Pts',(-7.30981359466555,4.93794661942718,
-0.180969163199008));
#156231=CARTESIAN_POINT('Ctrl Pts',(-7.28912572194307,4.94124830104116,
-0.180584981752446));
#156232=CARTESIAN_POINT('Ctrl Pts',(-7.26844390838857,4.94458995964329,
-0.180215524655243));
#156233=CARTESIAN_POINT('Ctrl Pts',(-7.24776865382235,4.94797285551049,
-0.179859607395719));
#156234=CARTESIAN_POINT('Ctrl Pts',(-7.18263592795554,4.81811592995231,
-0.972767571003609));
#156235=CARTESIAN_POINT('Ctrl Pts',(-7.18315990615277,4.81875342547615,
-0.968866820156804));
#156236=CARTESIAN_POINT('Ctrl Pts',(-7.18368388435,4.819390921,-0.96496606931));
#156237=CARTESIAN_POINT('Ctrl Pts',(-7.18452145479,4.82040994700001,-0.95873078391));
#156238=CARTESIAN_POINT('Ctrl Pts',(-7.18534819926,4.821428571,-0.95249405318));
#156239=CARTESIAN_POINT('Ctrl Pts',(-7.23654016133,4.884501699,-0.566316237149999));
#156240=CARTESIAN_POINT('Ctrl Pts',(-7.24604640355999,4.948754474,-0.17687618393));
#156241=CARTESIAN_POINT('Ctrl Pts',(-7.18465562199173,4.81811592995231,
-0.971228900270977));
#156242=CARTESIAN_POINT('Ctrl Pts',(-7.18517876349587,4.81875342547615,
-0.967327053635489));
#156243=CARTESIAN_POINT('Ctrl Pts',(-7.185701905,4.819390921,-0.963425207));
#156244=CARTESIAN_POINT('Ctrl Pts',(-7.186538138,4.82040994700001,-0.95718817));
#156245=CARTESIAN_POINT('Ctrl Pts',(-7.187363542,4.821428571,-0.95094969));
#156246=CARTESIAN_POINT('Ctrl Pts',(-7.238472502,4.884501699,-0.564663559));
#156247=CARTESIAN_POINT('Ctrl Pts',(-7.247884611,4.948754474,-0.175124711));
#156248=CARTESIAN_POINT('Ctrl Pts',(-7.38662502560986,4.81811592995231,
-0.817361827007792));
#156249=CARTESIAN_POINT('Ctrl Pts',(-7.38706449780493,4.81875342547615,
-0.813350401503896));
#156250=CARTESIAN_POINT('Ctrl Pts',(-7.38750397,4.819390921,-0.809338976));
#156251=CARTESIAN_POINT('Ctrl Pts',(-7.388206459,4.82040994700001,-0.802926779000001));
#156252=CARTESIAN_POINT('Ctrl Pts',(-7.388897816,4.821428571,-0.796513372));
#156253=CARTESIAN_POINT('Ctrl Pts',(-7.431706569,4.884501699,-0.399395744));
#156254=CARTESIAN_POINT('Ctrl Pts',(-7.431705355,4.948754474,2.2582E-5));
#156255=CARTESIAN_POINT('Origin',(0.190112165852048,5.08885462582407,-0.0186099193378765));
#156256=CARTESIAN_POINT('Ctrl Pts',(-7.02506401246283,4.95685569218473,
-1.78464262253522));
#156257=CARTESIAN_POINT('Ctrl Pts',(-7.12846029442096,4.88876676004178,
-1.37763368220099));
#156258=CARTESIAN_POINT('Ctrl Pts',(-7.18416104268,4.819390921,-0.96140718635));
#156259=CARTESIAN_POINT('Ctrl Pts',(-7.18782372009859,4.81482901964336,
-0.934037654790715));
#156260=CARTESIAN_POINT('Ctrl Pts',(-7.1914863975165,4.81026711828654,-0.90666812323139));
#156261=CARTESIAN_POINT('Ctrl Pts',(-7.0263615124981,4.95685569218473,-1.78682508849492));
#156262=CARTESIAN_POINT('Ctrl Pts',(-7.12988423930301,4.88876676004178,
-1.37974097530298));
#156263=CARTESIAN_POINT('Ctrl Pts',(-7.185701905,4.819390921,-0.963425207));
#156264=CARTESIAN_POINT('Ctrl Pts',(-7.1893722704815,4.81482901964336,-0.936049805210888));
#156265=CARTESIAN_POINT('Ctrl Pts',(-7.19304263596297,4.81026711828654,
-0.908674403421743));
#156266=CARTESIAN_POINT('Ctrl Pts',(-7.15611151602414,4.95685569218473,
-2.0050716844652));
#156267=CARTESIAN_POINT('Ctrl Pts',(-7.27227872750701,4.88876676004178,
-1.59047028550176));
#156268=CARTESIAN_POINT('Ctrl Pts',(-7.339788137,4.819390921,-1.165227272));
#156269=CARTESIAN_POINT('Ctrl Pts',(-7.34422730877804,4.81482901964336,
-1.13726484722787));
#156270=CARTESIAN_POINT('Ctrl Pts',(-7.34866648055661,4.81026711828654,
-1.10930242245574));
#156271=CARTESIAN_POINT('',(-7.03965514124212,4.94797311768998,-1.7337115899803));
#156272=CARTESIAN_POINT('Origin',(0.192413371046692,4.69654719529238,0.00524289899331731));
#156273=CARTESIAN_POINT('Ctrl Pts',(-7.10001119442563,4.93794661929334,
-1.74813205044452));
#156274=CARTESIAN_POINT('Ctrl Pts',(-7.07988954751257,4.94124830637727,
-1.74330956268131));
#156275=CARTESIAN_POINT('Ctrl Pts',(-7.05977065306694,4.9445899704517,-1.73850275691499));
#156276=CARTESIAN_POINT('Ctrl Pts',(-7.03965525371808,4.94797287189028,
-1.73371058431184));
#156277=CARTESIAN_POINT('Ctrl Pts',(-6.80559361859715,4.81811592995213,
-2.49407921308506));
#156278=CARTESIAN_POINT('Ctrl Pts',(-6.80694389264858,4.81875342547607,
-2.49038229955253));
#156279=CARTESIAN_POINT('Ctrl Pts',(-6.80829416670001,4.819390921,-2.48668538602));
#156280=CARTESIAN_POINT('Ctrl Pts',(-6.81045255733,4.820409947,-2.48077593118));
#156281=CARTESIAN_POINT('Ctrl Pts',(-6.81260068542,4.821428571,-2.47486273772));
#156282=CARTESIAN_POINT('Ctrl Pts',(-6.94561262344,4.884501699,-2.10871830233));
#156283=CARTESIAN_POINT('Ctrl Pts',(-7.03861471392,4.948754474,-1.7304267022));
#156284=CARTESIAN_POINT('Ctrl Pts',(-6.80789686203718,4.81811592995213,
-2.49301069013484));
#156285=CARTESIAN_POINT('Ctrl Pts',(-6.80924655451859,4.81875342547607,
-2.48931252656742));
#156286=CARTESIAN_POINT('Ctrl Pts',(-6.810596247,4.819390921,-2.485614363));
#156287=CARTESIAN_POINT('Ctrl Pts',(-6.81275370800001,4.820409947,-2.47970291));
#156288=CARTESIAN_POINT('Ctrl Pts',(-6.814900903,4.821428571,-2.47378772));
#156289=CARTESIAN_POINT('Ctrl Pts',(-6.947855064,4.884501699,-2.107519659));
#156290=CARTESIAN_POINT('Ctrl Pts',(-7.04078646,4.948754474,-1.729111338));
#156291=CARTESIAN_POINT('Ctrl Pts',(-7.03822120603974,4.81811592995213,
-2.38615839511329));
#156292=CARTESIAN_POINT('Ctrl Pts',(-7.03951274151988,4.81875342547607,
-2.38233522805665));
#156293=CARTESIAN_POINT('Ctrl Pts',(-7.040804277,4.819390921,-2.378512061));
#156294=CARTESIAN_POINT('Ctrl Pts',(-7.042868775,4.820409947,-2.372400792));
#156295=CARTESIAN_POINT('Ctrl Pts',(-7.044922661,4.821428571,-2.366285948));
#156296=CARTESIAN_POINT('Ctrl Pts',(-7.17209912,4.884501699,-1.987655326));
#156297=CARTESIAN_POINT('Ctrl Pts',(-7.257961068,4.948754474,-1.597574918));
#156298=CARTESIAN_POINT('Origin',(0.189670017113995,5.08885506248735,0.0226941950227263));
#156299=CARTESIAN_POINT('Ctrl Pts',(-6.47717652379903,4.95685568712946,
-3.25309974465563));
#156300=CARTESIAN_POINT('Ctrl Pts',(-6.66565034037312,4.88876675745772,
-2.87783360445593));
#156301=CARTESIAN_POINT('Ctrl Pts',(-6.80952522398,4.819390921,-2.4833122827));
#156302=CARTESIAN_POINT('Ctrl Pts',(-6.81898590893967,4.81482902029794,
-2.45737000673472));
#156303=CARTESIAN_POINT('Ctrl Pts',(-6.82844659389913,4.81026711959574,
-2.43142773077));
#156304=CARTESIAN_POINT('Ctrl Pts',(-6.47797452333863,4.95685568712946,
-3.25551010993541));
#156305=CARTESIAN_POINT('Ctrl Pts',(-6.6665879885029,4.88876675745772,-2.88019773628271));
#156306=CARTESIAN_POINT('Ctrl Pts',(-6.810596247,4.819390921,-2.485614363));
#156307=CARTESIAN_POINT('Ctrl Pts',(-6.82006570220355,4.81482902029794,
-2.45966800675379));
#156308=CARTESIAN_POINT('Ctrl Pts',(-6.82953515740693,4.81026711959574,
-2.4337216505078));
#156309=CARTESIAN_POINT('Ctrl Pts',(-6.55777447729816,4.95685568712946,
-3.49654663791317));
#156310=CARTESIAN_POINT('Ctrl Pts',(-6.76035280148079,4.88876675745772,
-3.11661091896105));
#156311=CARTESIAN_POINT('Ctrl Pts',(-6.917698549,4.819390921,-2.715822393));
#156312=CARTESIAN_POINT('Ctrl Pts',(-6.92804502859184,4.81482902029794,
-2.68946800865921));
#156313=CARTESIAN_POINT('Ctrl Pts',(-6.93839150818421,4.81026711959574,
-2.66311362431852));
#156314=CARTESIAN_POINT('',(-6.50237519691556,4.9479731000183,-3.20649612919631));
#156315=CARTESIAN_POINT('Origin',(0.186787698060051,4.69654717645868,0.0464834694545685));
#156316=CARTESIAN_POINT('Ctrl Pts',(-6.55822016114327,4.93794661955904,
-3.23355422788455));
#156317=CARTESIAN_POINT('Ctrl Pts',(-6.53960567031831,4.94124830107305,
-3.22451894133828));
#156318=CARTESIAN_POINT('Ctrl Pts',(-6.52099049576717,4.94458995968661,
-3.21549956301667));
#156319=CARTESIAN_POINT('Ctrl Pts',(-6.50237558887183,4.94797285554171,
-3.20649522704559));
#156320=CARTESIAN_POINT('Ctrl Pts',(-6.11032931624113,4.81811592995213,
-3.89877048441623));
#156321=CARTESIAN_POINT('Ctrl Pts',(-6.11244274850557,4.81875342547607,
-3.89545027115312));
#156322=CARTESIAN_POINT('Ctrl Pts',(-6.11455618077,4.819390921,-3.89213005789));
#156323=CARTESIAN_POINT('Ctrl Pts',(-6.11793446712,4.820409947,-3.88682275217));
#156324=CARTESIAN_POINT('Ctrl Pts',(-6.1213035352,4.821428571,-3.88150959062));
#156325=CARTESIAN_POINT('Ctrl Pts',(-6.32991595857,4.884501699,-3.55251904328));
#156326=CARTESIAN_POINT('Ctrl Pts',(-6.50206522372001,4.948754474,-3.20306439151));
#156327=CARTESIAN_POINT('Ctrl Pts',(-6.11280841197595,4.81811592995213,
-3.89822207217761));
#156328=CARTESIAN_POINT('Ctrl Pts',(-6.11492154498798,4.81875342547607,
-3.89490051308881));
#156329=CARTESIAN_POINT('Ctrl Pts',(-6.117034678,4.819390921,-3.891578954));
#156330=CARTESIAN_POINT('Ctrl Pts',(-6.120412486,4.820409947,-3.886269497));
#156331=CARTESIAN_POINT('Ctrl Pts',(-6.123781072,4.821428571,-3.880954185));
#156332=CARTESIAN_POINT('Ctrl Pts',(-6.332363645,4.884501699,-3.551830482));
#156333=CARTESIAN_POINT('Ctrl Pts',(-6.50446896,4.948754474,-3.202246641));
#156334=CARTESIAN_POINT('Ctrl Pts',(-6.36071798545746,4.81811592995213,
-3.84338084831584));
#156335=CARTESIAN_POINT('Ctrl Pts',(-6.36280119322874,4.81875342547607,
-3.83992470665792));
#156336=CARTESIAN_POINT('Ctrl Pts',(-6.364884401,4.819390921,-3.836468565));
#156337=CARTESIAN_POINT('Ctrl Pts',(-6.368214374,4.820409947,-3.83094398));
#156338=CARTESIAN_POINT('Ctrl Pts',(-6.371534752,4.821428571,-3.825413623));
#156339=CARTESIAN_POINT('Ctrl Pts',(-6.577132288,4.884501699,-3.482974354));
#156340=CARTESIAN_POINT('Ctrl Pts',(-6.74484258800001,4.948754474,-3.12047159));
#156341=CARTESIAN_POINT('Origin',(0.180357139429196,5.08885511133933,0.0629370989123257));
#156342=CARTESIAN_POINT('Ctrl Pts',(-5.62642342793858,4.95685569311866,
-4.56944559844393));
#156343=CARTESIAN_POINT('Ctrl Pts',(-5.89116197315354,4.88876676051917,
-4.24346925844328));
#156344=CARTESIAN_POINT('Ctrl Pts',(-6.11648357412,4.819390921,-3.88910045677));
#156345=CARTESIAN_POINT('Ctrl Pts',(-6.13129989983707,4.81482901911934,
-3.86579845835072));
#156346=CARTESIAN_POINT('Ctrl Pts',(-6.14611622555393,4.81026711723851,
-3.84249645993146));
#156347=CARTESIAN_POINT('Ctrl Pts',(-5.6266846134028,4.95685569311866,-4.57197115702515));
#156348=CARTESIAN_POINT('Ctrl Pts',(-5.8915694811121,4.88876676051917,-4.24597968480163));
#156349=CARTESIAN_POINT('Ctrl Pts',(-6.117034678,4.819390921,-3.891578954));
#156350=CARTESIAN_POINT('Ctrl Pts',(-6.13186044606048,4.81482901911934,
-3.86827485603784));
#156351=CARTESIAN_POINT('Ctrl Pts',(-6.14668621412129,4.81026711723851,
-3.84497075807568));
#156352=CARTESIAN_POINT('Ctrl Pts',(-5.65280315982447,4.95685569311866,
-4.82452701514691));
#156353=CARTESIAN_POINT('Ctrl Pts',(-5.93232027696772,4.88876676051917,
-4.49702232063717));
#156354=CARTESIAN_POINT('Ctrl Pts',(-6.172145066,4.819390921,-4.139428677));
#156355=CARTESIAN_POINT('Ctrl Pts',(-6.18791506840579,4.81482901911934,
-4.11591462474872));
#156356=CARTESIAN_POINT('Ctrl Pts',(-6.20368507081199,4.81026711723851,
-4.09240057249751));
#156357=CARTESIAN_POINT('',(-5.66105136716546,4.94797311770236,-4.52934849656686));
#156358=CARTESIAN_POINT('Origin',(0.172428333552543,4.69654718770639,0.085550693991383));
#156359=CARTESIAN_POINT('Ctrl Pts',(-5.7097740428877,4.93794661935847,-4.56777900152391));
#156360=CARTESIAN_POINT('Ctrl Pts',(-5.69353704127715,4.94124830632178,
-4.5549533693698));
#156361=CARTESIAN_POINT('Ctrl Pts',(-5.67729595263904,4.94458997037757,
-4.5421431261003));
#156362=CARTESIAN_POINT('Ctrl Pts',(-5.66105189175548,4.9479728717964,-4.52934763110827));
#156363=CARTESIAN_POINT('Ctrl Pts',(-5.12935280446128,4.81811592995225,
-5.12115957988297));
#156364=CARTESIAN_POINT('Ctrl Pts',(-5.13213057353563,4.81875342547613,
-5.11837131681149));
#156365=CARTESIAN_POINT('Ctrl Pts',(-5.13490834261001,4.819390921,-5.11558305374));
#156366=CARTESIAN_POINT('Ctrl Pts',(-5.13934856031,4.82040994700001,-5.11112606156001));
#156367=CARTESIAN_POINT('Ctrl Pts',(-5.14378103484,4.821428571,-5.10666136836));
#156368=CARTESIAN_POINT('Ctrl Pts',(-5.4182394588,4.884501699,-4.83020794186));
#156369=CARTESIAN_POINT('Ctrl Pts',(-5.66148638954,4.948754474,-4.5259303487));
#156370=CARTESIAN_POINT('Ctrl Pts',(-5.13189183273185,4.81811592995225,
-5.12115692153167));
#156371=CARTESIAN_POINT('Ctrl Pts',(-5.13466959886593,4.81875342547613,
-5.11836727976584));
#156372=CARTESIAN_POINT('Ctrl Pts',(-5.13744736500001,4.819390921,-5.115577638));
#156373=CARTESIAN_POINT('Ctrl Pts',(-5.141887578,4.82040994700001,-5.11111844200001));
#156374=CARTESIAN_POINT('Ctrl Pts',(-5.146320044,4.821428571,-5.106651545));
#156375=CARTESIAN_POINT('Ctrl Pts',(-5.42077794,4.884501699,-4.830061659));
#156376=CARTESIAN_POINT('Ctrl Pts',(-5.66400972,4.948754474,-4.525648449));
#156377=CARTESIAN_POINT('Ctrl Pts',(-5.38579465978926,4.81811592995225,
-5.12089108640102));
#156378=CARTESIAN_POINT('Ctrl Pts',(-5.38857213189463,4.81875342547613,
-5.11796357520052));
#156379=CARTESIAN_POINT('Ctrl Pts',(-5.391349604,4.819390921,-5.115036064));
#156380=CARTESIAN_POINT('Ctrl Pts',(-5.395789347,4.82040994700001,-5.110356486));
#156381=CARTESIAN_POINT('Ctrl Pts',(-5.40022096,4.821428571,-5.105669209));
#156382=CARTESIAN_POINT('Ctrl Pts',(-5.67462606,4.884501699,-4.815433373));
#156383=CARTESIAN_POINT('Ctrl Pts',(-5.916342766,4.948754474,-4.497458479));
#156384=CARTESIAN_POINT('Origin',(0.162609572644723,5.08885473206602,0.100236046809242));
#156385=CARTESIAN_POINT('Ctrl Pts',(-4.51258505800762,4.95685569008051,
-5.67212920879434));
#156386=CARTESIAN_POINT('Ctrl Pts',(-4.84120943276726,4.88876675896619,
-5.41068498147605));
#156387=CARTESIAN_POINT('Ctrl Pts',(-5.13744194926001,4.819390921,-5.11303861561001));
#156388=CARTESIAN_POINT('Ctrl Pts',(-5.15692112007753,4.81482901869991,
-5.09346647520961));
#156389=CARTESIAN_POINT('Ctrl Pts',(-5.17640029089601,4.81026711639968,
-5.07389433480971));
#156390=CARTESIAN_POINT('Ctrl Pts',(-4.51229721666626,4.95685569008051,
-5.67465186837979));
#156391=CARTESIAN_POINT('Ctrl Pts',(-4.84106774596149,4.88876675896619,
-5.41322431763507));
#156392=CARTESIAN_POINT('Ctrl Pts',(-5.137447365,4.819390921,-5.115577638));
#156393=CARTESIAN_POINT('Ctrl Pts',(-5.15693620874494,4.81482901869991,
-5.09600547696734));
#156394=CARTESIAN_POINT('Ctrl Pts',(-5.17642505249043,4.81026711639968,
-5.07643331593493));
#156395=CARTESIAN_POINT('Ctrl Pts',(-4.48351308253065,4.95685569008051,
-5.92691782692511));
#156396=CARTESIAN_POINT('Ctrl Pts',(-4.82689906538418,4.88876675896619,
-5.66715793353732));
#156397=CARTESIAN_POINT('Ctrl Pts',(-5.13798893900001,4.819390921,-5.369479877));
#156398=CARTESIAN_POINT('Ctrl Pts',(-5.15844507548202,4.81482901869991,
-5.34990565273664));
#156399=CARTESIAN_POINT('Ctrl Pts',(-5.17890121196401,4.81026711639968,
-5.33033142847279));
#156400=CARTESIAN_POINT('',(-4.55502311951874,4.94797310000155,-5.64041354953503));
#156401=CARTESIAN_POINT('Origin',(0.150006191366085,4.69654718716523,0.120617561408115));
#156402=CARTESIAN_POINT('Ctrl Pts',(-4.59434523651735,4.93794661933408,
-5.6884195057972));
#156403=CARTESIAN_POINT('Ctrl Pts',(-4.58124499947238,4.9412483010484,-5.67240328103802));
#156404=CARTESIAN_POINT('Ctrl Pts',(-4.56813746317855,4.94458995965945,
-5.6564012061072));
#156405=CARTESIAN_POINT('Ctrl Pts',(-4.55502385387762,4.94797285546293,
-5.64041289547318));
#156406=CARTESIAN_POINT('Ctrl Pts',(-3.90853345679646,4.81811592995226,
-6.10408894376807));
#156407=CARTESIAN_POINT('Ctrl Pts',(-3.91184567755823,4.81875342547613,
-6.10196300756403));
#156408=CARTESIAN_POINT('Ctrl Pts',(-3.91515789832001,4.819390921,-6.09983707136));
#156409=CARTESIAN_POINT('Ctrl Pts',(-3.92045242816,4.820409947,-6.09643879767));
#156410=CARTESIAN_POINT('Ctrl Pts',(-3.92574105073,4.821428571,-6.09303133678));
#156411=CARTESIAN_POINT('Ctrl Pts',(-4.25321210359,4.884501699,-5.88204168643));
#156412=CARTESIAN_POINT('Ctrl Pts',(-4.5561827445,4.948754474,-5.6371688346));
#156413=CARTESIAN_POINT('Ctrl Pts',(-3.91101369547004,4.81811592995226,
-6.10463216359936));
#156414=CARTESIAN_POINT('Ctrl Pts',(-3.91432620973502,4.81875342547613,
-6.10250488029968));
#156415=CARTESIAN_POINT('Ctrl Pts',(-3.917638724,4.819390921,-6.100377597));
#156416=CARTESIAN_POINT('Ctrl Pts',(-3.922933723,4.820409947,-6.09697717));
#156417=CARTESIAN_POINT('Ctrl Pts',(-3.928222811,4.821428571,-6.093567555));
#156418=CARTESIAN_POINT('Ctrl Pts',(-4.255722683,4.884501699,-5.882444522));
#156419=CARTESIAN_POINT('Ctrl Pts',(-4.558707681,4.948754474,-5.637435967));
#156420=CARTESIAN_POINT('Ctrl Pts',(-4.15903756282845,4.81811592995226,
-6.15895414672832));
#156421=CARTESIAN_POINT('Ctrl Pts',(-4.16237942741423,4.81875342547613,
-6.15669215386416));
#156422=CARTESIAN_POINT('Ctrl Pts',(-4.165721292,4.819390921,-6.154430161));
#156423=CARTESIAN_POINT('Ctrl Pts',(-4.171063207,4.820409947,-6.150814403));
#156424=CARTESIAN_POINT('Ctrl Pts',(-4.176398838,4.821428571,-6.147189377));
#156425=CARTESIAN_POINT('Ctrl Pts',(-4.506780624,4.884501699,-5.922728079));
#156426=CARTESIAN_POINT('Ctrl Pts',(-4.811201331,4.948754474,-5.664149207));
#156427=CARTESIAN_POINT('Origin',(0.137261010202675,5.08885510563361,0.132850046849201));
#156428=CARTESIAN_POINT('Ctrl Pts',(-3.18774320373244,4.95685569209715,
-6.50959038225223));
#156429=CARTESIAN_POINT('Ctrl Pts',(-3.56488730825351,4.88876675999702,
-6.32490309878235));
#156430=CARTESIAN_POINT('Ctrl Pts',(-3.91817924964,4.819390921,-6.09789677132001));
#156431=CARTESIAN_POINT('Ctrl Pts',(-3.94141043440046,4.81482901979346,
-6.08296966623404));
#156432=CARTESIAN_POINT('Ctrl Pts',(-3.96464161916139,4.81026711858739,
-6.06804256114847));
#156433=CARTESIAN_POINT('Ctrl Pts',(-3.18691979471379,4.95685569209715,
-6.51199218607273));
#156434=CARTESIAN_POINT('Ctrl Pts',(-3.56420305179831,4.88876675999702,
-6.32735260820541));
#156435=CARTESIAN_POINT('Ctrl Pts',(-3.917638724,4.819390921,-6.100377597));
#156436=CARTESIAN_POINT('Ctrl Pts',(-3.94087935997272,4.81482901979346,
-6.08545255115646));
#156437=CARTESIAN_POINT('Ctrl Pts',(-3.96411999594573,4.81026711858739,
-6.07052750531346));
#156438=CARTESIAN_POINT('Ctrl Pts',(-3.10457889284941,4.95685569209715,
-6.75217256812281));
#156439=CARTESIAN_POINT('Ctrl Pts',(-3.49577740627834,4.88876675999702,
-6.5723035505118));
#156440=CARTESIAN_POINT('Ctrl Pts',(-3.86358616,4.819390921,-6.348460165));
#156441=CARTESIAN_POINT('Ctrl Pts',(-3.88777191719758,4.81482901979346,
-6.33374104339812));
#156442=CARTESIAN_POINT('Ctrl Pts',(-3.91195767439497,4.81026711858739,
-6.3190219217962));
#156443=CARTESIAN_POINT('',(-3.23600699950429,4.9479731176986,-6.48773913498767));
#156444=CARTESIAN_POINT('Origin',(0.120569870483082,4.69654718513396,0.150044397100799));
#156445=CARTESIAN_POINT('Ctrl Pts',(-3.26408995160878,4.93794661963025,
-6.54307583744842));
#156446=CARTESIAN_POINT('Ctrl Pts',(-3.25473899234202,4.94124830639095,
-6.52461786857059));
#156447=CARTESIAN_POINT('Ctrl Pts',(-3.24537786108337,4.94458997045841,
-6.50617215046991));
#156448=CARTESIAN_POINT('Ctrl Pts',(-3.23600783896611,4.94797287203117,
-6.4877385697174));
#156449=CARTESIAN_POINT('Ctrl Pts',(-2.50495542924116,4.81811592995212,
-6.80159789469528));
#156450=CARTESIAN_POINT('Ctrl Pts',(-2.50864722546058,4.81875342547606,
-6.80023369102764));
#156451=CARTESIAN_POINT('Ctrl Pts',(-2.51233902168,4.819390921,-6.79886948736));
#156452=CARTESIAN_POINT('Ctrl Pts',(-2.51824029658,4.820409947,-6.79668883047));
#156453=CARTESIAN_POINT('Ctrl Pts',(-2.52413777697,4.821428571,-6.79449793217));
#156454=CARTESIAN_POINT('Ctrl Pts',(-2.88930927728,4.884501699,-6.65883769814));
#156455=CARTESIAN_POINT('Ctrl Pts',(-3.2378370587,4.948754474,-6.48481956928001));
#156456=CARTESIAN_POINT('Ctrl Pts',(-2.50726090509375,4.81811592995212,
-6.80266159234725));
#156457=CARTESIAN_POINT('Ctrl Pts',(-2.51095327754687,4.81875342547606,
-6.80129613617363));
#156458=CARTESIAN_POINT('Ctrl Pts',(-2.51464565,4.819390921,-6.79993068000001));
#156459=CARTESIAN_POINT('Ctrl Pts',(-2.520547846,4.820409947,-6.797748021));
#156460=CARTESIAN_POINT('Ctrl Pts',(-2.526446244,4.821428571,-6.795555119));
#156461=CARTESIAN_POINT('Ctrl Pts',(-2.891674563,4.884501699,-6.659770816));
#156462=CARTESIAN_POINT('Ctrl Pts',(-3.240245538,4.948754474,-6.485623243));
#156463=CARTESIAN_POINT('Ctrl Pts',(-2.73780849035282,4.81811592995212,
-6.90903135754417));
#156464=CARTESIAN_POINT('Ctrl Pts',(-2.74155848617641,4.81875342547606,
-6.90754065077208));
#156465=CARTESIAN_POINT('Ctrl Pts',(-2.745308482,4.819390921,-6.906049944));
#156466=CARTESIAN_POINT('Ctrl Pts',(-2.751302788,4.820409947,-6.903667074));
#156467=CARTESIAN_POINT('Ctrl Pts',(-2.757292947,4.821428571,-6.901273802));
#156468=CARTESIAN_POINT('Ctrl Pts',(-3.128203135,4.884501699,-6.753082602));
#156469=CARTESIAN_POINT('Ctrl Pts',(-3.481093468,4.948754474,-6.565990615));
#156470=CARTESIAN_POINT('Origin',(0.10549315056409,5.08885506891935,0.159251289995697));
#156471=CARTESIAN_POINT('Ctrl Pts',(-1.71384602885931,4.9568556919657,-7.04267033616501));
#156472=CARTESIAN_POINT('Ctrl Pts',(-2.12187502117099,4.88876675992982,
-6.94337577306025));
#156473=CARTESIAN_POINT('Ctrl Pts',(-2.51570684263,4.819390921,-6.79762405168));
#156474=CARTESIAN_POINT('Ctrl Pts',(-2.54160378198105,4.81482901971299,
-6.78803995186074));
#156475=CARTESIAN_POINT('Ctrl Pts',(-2.56750072133154,4.8102671184258,-6.7784558520405));
#156476=CARTESIAN_POINT('Ctrl Pts',(-1.71252555387243,4.9568556919657,-7.04483897854714));
#156477=CARTESIAN_POINT('Ctrl Pts',(-2.12068019013151,4.88876675992982,
-6.9456209194025));
#156478=CARTESIAN_POINT('Ctrl Pts',(-2.51464565,4.819390921,-6.79993068));
#156479=CARTESIAN_POINT('Ctrl Pts',(-2.54055137692377,4.81482901971299,
-6.79035062301057));
#156480=CARTESIAN_POINT('Ctrl Pts',(-2.56645710384759,4.8102671184258,-6.78077056602059));
#156481=CARTESIAN_POINT('Ctrl Pts',(-1.58047805518487,4.9568556919657,-7.26170321676013));
#156482=CARTESIAN_POINT('Ctrl Pts',(-2.00119708618366,4.88876675992982,
-7.1701355536279));
#156483=CARTESIAN_POINT('Ctrl Pts',(-2.408526387,4.819390921,-7.03059351200001));
#156484=CARTESIAN_POINT('Ctrl Pts',(-2.43531087119952,4.81482901971299,
-7.02141773799681));
#156485=CARTESIAN_POINT('Ctrl Pts',(-2.46209535539906,4.8102671184258,-7.01224196399419));
#156486=CARTESIAN_POINT('',(-1.76567881676234,4.94797311766291,-7.03170524848912));
#156487=CARTESIAN_POINT('Origin',(0.0854958773501102,4.69654720986263,0.172455336006564));
#156488=CARTESIAN_POINT('Ctrl Pts',(-1.78120944981267,4.93794661947598,
-7.09178521407223));
#156489=CARTESIAN_POINT('Ctrl Pts',(-1.77604502744539,4.9412483063804,-7.07174860270665));
#156490=CARTESIAN_POINT('Ctrl Pts',(-1.7708680381815,4.94458997045698,-7.05172176875845));
#156491=CARTESIAN_POINT('Ctrl Pts',(-1.76567975786171,4.94797287184847,
-7.03170487683643));
#156492=CARTESIAN_POINT('Ctrl Pts',(-0.984248470461467,4.81811592995224,
-7.18107168715767));
#156493=CARTESIAN_POINT('Ctrl Pts',(-0.988147217940733,4.81875342547613,
-7.18053300485384));
#156494=CARTESIAN_POINT('Ctrl Pts',(-0.99204596542,4.819390921,-7.17999432255));
#156495=CARTESIAN_POINT('Ctrl Pts',(-0.998278048469998,4.820409947,-7.17913324784));
#156496=CARTESIAN_POINT('Ctrl Pts',(-1.00450862757,4.821428571,-7.17826135544));
#156497=CARTESIAN_POINT('Ctrl Pts',(-1.3903055601,4.884501699,-7.1242738604));
#156498=CARTESIAN_POINT('Ctrl Pts',(-1.76809370969,4.948754474,-7.02924734988));
#156499=CARTESIAN_POINT('Ctrl Pts',(-0.986271382026669,4.81811592995224,
-7.18260612530429));
#156500=CARTESIAN_POINT('Ctrl Pts',(-0.990170961513334,4.81875342547613,
-7.18206634365215));
#156501=CARTESIAN_POINT('Ctrl Pts',(-0.994070541,4.819390921,-7.181526562));
#156502=CARTESIAN_POINT('Ctrl Pts',(-1.000303954,4.820409947,-7.18066373));
#156503=CARTESIAN_POINT('Ctrl Pts',(-1.00653586,4.821428571,-7.179790078));
#156504=CARTESIAN_POINT('Ctrl Pts',(-1.392414954,4.884501699,-7.125693629));
#156505=CARTESIAN_POINT('Ctrl Pts',(-1.770273114,4.948754474,-7.030549986));
#156506=CARTESIAN_POINT('Ctrl Pts',(-1.18856253854683,4.81811592995224,
-7.33604993996594));
#156507=CARTESIAN_POINT('Ctrl Pts',(-1.19254531877341,4.81875342547613,
-7.33540022348297));
#156508=CARTESIAN_POINT('Ctrl Pts',(-1.196528099,4.819390921,-7.33475050700001));
#156509=CARTESIAN_POINT('Ctrl Pts',(-1.202894507,4.820409947,-7.33371194600001));
#156510=CARTESIAN_POINT('Ctrl Pts',(-1.209259103,4.821428571,-7.332662334));
#156511=CARTESIAN_POINT('Ctrl Pts',(-1.603354344,4.884501699,-7.267670489));
#156512=CARTESIAN_POINT('Ctrl Pts',(-1.988213545,4.948754474,-7.160813598));
#156513=CARTESIAN_POINT('Origin',(0.0687924138857683,5.08885501609288,0.178205812545522));
#156514=CARTESIAN_POINT('Ctrl Pts',(-0.159811349130863,4.95685568709043,
-7.24644285164568));
#156515=CARTESIAN_POINT('Ctrl Pts',(-0.579646230555093,4.88876675743777,
-7.23718391136641));
#156516=CARTESIAN_POINT('Ctrl Pts',(-0.99560278045,4.819390921,-7.17950198642001));
#156517=CARTESIAN_POINT('Ctrl Pts',(-1.02295455786329,4.81482902039626,
-7.17570903455444));
#156518=CARTESIAN_POINT('Ctrl Pts',(-1.05030633527657,4.81026711979238,
-7.17191608268926));
#156519=CARTESIAN_POINT('Ctrl Pts',(-0.158055552108266,4.95685568709043,
-7.24827692929834));
#156520=CARTESIAN_POINT('Ctrl Pts',(-0.577996693906887,4.88876675743777,
-7.23911971407556));
#156521=CARTESIAN_POINT('Ctrl Pts',(-0.994070541,4.819390921,-7.181526562));
#156522=CARTESIAN_POINT('Ctrl Pts',(-1.02143003144691,4.81482902039626,
-7.17773944751295));
#156523=CARTESIAN_POINT('Ctrl Pts',(-1.04878952189387,4.81026711979238,
-7.17395233302586));
#156524=CARTESIAN_POINT('Ctrl Pts',(0.0175241501514,4.95685568709043,-7.43168469456425));
#156525=CARTESIAN_POINT('Ctrl Pts',(-0.41304302908634,4.88876675743777,
-7.43269998499101));
#156526=CARTESIAN_POINT('Ctrl Pts',(-0.840846596,4.819390921,-7.38398412));
#156527=CARTESIAN_POINT('Ctrl Pts',(-0.868977389809564,4.81482902039626,
-7.38078074335875));
#156528=CARTESIAN_POINT('Ctrl Pts',(-0.897108183619176,4.81026711979238,
-7.37757736671704));
#156529=CARTESIAN_POINT('',(-0.212789476047507,4.94797309998795,-7.24687665554507));
#156530=CARTESIAN_POINT('Origin',(0.0464242208071746,4.69654713733818,0.186802261620559));
#156531=CARTESIAN_POINT('Ctrl Pts',(-0.215041574107111,4.93794661934344,
-7.3088905962304));
#156532=CARTESIAN_POINT('Ctrl Pts',(-0.214305172576142,4.94124830105344,
-7.28821226501762));
#156533=CARTESIAN_POINT('Ctrl Pts',(-0.213554397023954,4.94458995967662,
-7.26754078098889));
#156534=CARTESIAN_POINT('Ctrl Pts',(-0.212790456728527,4.94797285555638,
-7.2468765792746));
#156535=CARTESIAN_POINT('Ctrl Pts',(0.58248085480347,4.81811592995213,-7.22476655041542));
#156536=CARTESIAN_POINT('Ctrl Pts',(0.578557456876735,4.81875342547606,
-7.22507857698772));
#156537=CARTESIAN_POINT('Ctrl Pts',(0.574634058950001,4.819390921,-7.22539060356));
#156538=CARTESIAN_POINT('Ctrl Pts',(0.56836257257,4.820409947,-7.22588937285));
#156539=CARTESIAN_POINT('Ctrl Pts',(0.5620902297,4.821428571,-7.22637725608));
#156540=CARTESIAN_POINT('Ctrl Pts',(0.17370729917,4.884501699,-7.25658689547));
#156541=CARTESIAN_POINT('Ctrl Pts',(-0.21567626421,4.948754474,-7.24499533628));
#156542=CARTESIAN_POINT('Ctrl Pts',(0.580835096616913,4.81811592995213,
-7.22669998041422));
#156543=CARTESIAN_POINT('Ctrl Pts',(0.576910649808457,4.81875342547606,
-7.22701111220712));
#156544=CARTESIAN_POINT('Ctrl Pts',(0.572986203000001,4.819390921,-7.227322244));
#156545=CARTESIAN_POINT('Ctrl Pts',(0.56671304,4.820409947,-7.227819583));
#156546=CARTESIAN_POINT('Ctrl Pts',(0.560439023,4.821428571,-7.228306033));
#156547=CARTESIAN_POINT('Ctrl Pts',(0.17195243,4.884501699,-7.258426928));
#156548=CARTESIAN_POINT('Ctrl Pts',(-0.217524687,4.948754474,-7.246736025));
#156549=CARTESIAN_POINT('Ctrl Pts',(0.416259277961255,4.81811592995213,
-7.42004298029423));
#156550=CARTESIAN_POINT('Ctrl Pts',(0.412229942980628,4.81875342547606,
-7.42026463414712));
#156551=CARTESIAN_POINT('Ctrl Pts',(0.408200608,4.819390921,-7.420486288));
#156552=CARTESIAN_POINT('Ctrl Pts',(0.401759783,4.820409947,-7.42084059800001));
#156553=CARTESIAN_POINT('Ctrl Pts',(0.395318353,4.821428571,-7.421183725));
#156554=CARTESIAN_POINT('Ctrl Pts',(-0.003534487,4.884501699,-7.442430181));
#156555=CARTESIAN_POINT('Ctrl Pts',(-0.402366966,4.948754474,-7.420804897));
#156556=CARTESIAN_POINT('Origin',(0.0288751199735729,5.08885504792801,0.18882771706922));
#156557=CARTESIAN_POINT('Ctrl Pts',(1.40169596736114,4.95685568822406,-7.11137975895541));
#156558=CARTESIAN_POINT('Ctrl Pts',(0.98968619117965,4.88876675801725,-7.19258937817722));
#156559=CARTESIAN_POINT('Ctrl Pts',(0.571054562559999,4.819390921,-7.22567438806));
#156560=CARTESIAN_POINT('Ctrl Pts',(0.543526877900215,4.81482901971525,
-7.22784993729411));
#156561=CARTESIAN_POINT('Ctrl Pts',(0.515999193240412,4.81026711843093,
-7.23002548652851));
#156562=CARTESIAN_POINT('Ctrl Pts',(1.40380498731083,4.95685568822406,-7.11279351242862));
#156563=CARTESIAN_POINT('Ctrl Pts',(0.991713302934894,4.88876675801725,
-7.19412532127777));
#156564=CARTESIAN_POINT('Ctrl Pts',(0.572986203,4.819390921,-7.227322244));
#156565=CARTESIAN_POINT('Ctrl Pts',(0.54545224049573,4.81482901971525,-7.2295051522131));
#156566=CARTESIAN_POINT('Ctrl Pts',(0.517918277991468,4.81026711843093,
-7.23168806042634));
#156567=CARTESIAN_POINT('Ctrl Pts',(1.61470698227998,4.95685568822406,-7.25416885975011));
#156568=CARTESIAN_POINT('Ctrl Pts',(1.19442447845929,4.88876675801725,-7.34771963133292));
#156569=CARTESIAN_POINT('Ctrl Pts',(0.766150247,4.819390921,-7.392107838));
#156570=CARTESIAN_POINT('Ctrl Pts',(0.737988500047442,4.81482901971525,
-7.39502664411069));
#156571=CARTESIAN_POINT('Ctrl Pts',(0.709826753094835,4.81026711843093,
-7.39794545022136));
#156572=CARTESIAN_POINT('',(1.3500496883036,4.9479730999751,-7.123192154401));
#156573=CARTESIAN_POINT('Origin',(0.00518181707668791,4.69654721187571,
0.1924151738053));
#156574=CARTESIAN_POINT('Ctrl Pts',(1.36118140704012,4.93794661927204,-7.18424037761141));
#156575=CARTESIAN_POINT('Ctrl Pts',(1.35745536226788,4.94124830104824,-7.16388718961221));
#156576=CARTESIAN_POINT('Ctrl Pts',(1.35374482708709,4.9445899596398,-7.14353759904923));
#156577=CARTESIAN_POINT('Ctrl Pts',(1.35004871438277,4.94797285546353,-7.12319229067635));
#156578=CARTESIAN_POINT('Ctrl Pts',(2.1219740218502,4.81811592995224,-6.93063935649274));
#156579=CARTESIAN_POINT('Ctrl Pts',(2.1182094271201,4.81875342547612,-6.93178750320637));
#156580=CARTESIAN_POINT('Ctrl Pts',(2.11444483239,4.819390921,-6.93293564992));
#156581=CARTESIAN_POINT('Ctrl Pts',(2.10842719028,4.820409947,-6.93477094336));
#156582=CARTESIAN_POINT('Ctrl Pts',(2.10240637238,4.821428571,-6.93659578717));
#156583=CARTESIAN_POINT('Ctrl Pts',(1.72959779769,4.884501699,-7.04958999141));
#156584=CARTESIAN_POINT('Ctrl Pts',(1.34682596407,4.948754474,-7.12197539235));
#156585=CARTESIAN_POINT('Ctrl Pts',(2.1207823708793,4.81811592995224,-6.93288137335194));
#156586=CARTESIAN_POINT('Ctrl Pts',(2.11701655943965,4.81875342547612,-6.93402887167597));
#156587=CARTESIAN_POINT('Ctrl Pts',(2.113250748,4.819390921,-6.93517637000001));
#156588=CARTESIAN_POINT('Ctrl Pts',(2.107231161,4.820409947,-6.937010627));
#156589=CARTESIAN_POINT('Ctrl Pts',(2.1012084,4.821428571,-6.938834431));
#156590=CARTESIAN_POINT('Ctrl Pts',(1.728279509,4.884501699,-7.05176425));
#156591=CARTESIAN_POINT('Ctrl Pts',(1.345394953,4.948754474,-7.12407274100001));
#156592=CARTESIAN_POINT('Ctrl Pts',(2.00161727379,4.81811592995224,-7.15708305927198));
#156593=CARTESIAN_POINT('Ctrl Pts',(1.997729791395,4.81875342547612,-7.15816571863599));
#156594=CARTESIAN_POINT('Ctrl Pts',(1.993842309,4.819390921,-7.159248378));
#156595=CARTESIAN_POINT('Ctrl Pts',(1.987628233,4.820409947,-7.160978991));
#156596=CARTESIAN_POINT('Ctrl Pts',(1.981411162,4.821428571,-7.162698814));
#156597=CARTESIAN_POINT('Ctrl Pts',(1.59645064,4.884501699,-7.269190109));
#156598=CARTESIAN_POINT('Ctrl Pts',(1.202293846,4.948754474,-7.333807606));
#156599=CARTESIAN_POINT('Origin',(-0.0123919794028246,5.08885456115538,
0.190618511251751));
#156600=CARTESIAN_POINT('Ctrl Pts',(2.89766155263498,4.95685569176659,-6.64379644459623));
#156601=CARTESIAN_POINT('Ctrl Pts',(2.51274199308637,4.88876675982804,-6.81167735636691));
#156602=CARTESIAN_POINT('Ctrl Pts',(2.11101002792,4.819390921,-6.93398228561));
#156603=CARTESIAN_POINT('Ctrl Pts',(2.08459360491011,4.81482901987171,-6.94202460991387));
#156604=CARTESIAN_POINT('Ctrl Pts',(2.0581771819,4.81026711874384,-6.95006693421685));
#156605=CARTESIAN_POINT('Ctrl Pts',(2.90002518007121,4.95685569176659,-6.64472376834042));
#156606=CARTESIAN_POINT('Ctrl Pts',(2.51505189446649,4.88876675982804,-6.81274162086169));
#156607=CARTESIAN_POINT('Ctrl Pts',(2.113250748,4.819390921,-6.93517637));
#156608=CARTESIAN_POINT('Ctrl Pts',(2.08682977588114,4.81482901987171,-6.94322723078481));
#156609=CARTESIAN_POINT('Ctrl Pts',(2.06040880376209,4.81026711874384,-6.9512780915691));
#156610=CARTESIAN_POINT('Ctrl Pts',(3.13638792369391,4.95685569176659,-6.73745614275944));
#156611=CARTESIAN_POINT('Ctrl Pts',(2.74604203247821,4.88876675982804,-6.91916807033975));
#156612=CARTESIAN_POINT('Ctrl Pts',(2.337322756,4.819390921,-7.054584809));
#156613=CARTESIAN_POINT('Ctrl Pts',(2.31044687298363,4.81482901987171,-7.06348931787967));
#156614=CARTESIAN_POINT('Ctrl Pts',(2.28357098996724,4.81026711874384,-7.0723938267588));
#156615=CARTESIAN_POINT('',(2.84976204342522,4.94797311766865,-6.66643508049058));
#156616=CARTESIAN_POINT('Origin',(-0.0363028520273356,4.69654719454111,
0.189030396997524));
#156617=CARTESIAN_POINT('Ctrl Pts',(2.87375706015906,4.93794661954414,-6.72366306308529));
#156618=CARTESIAN_POINT('Ctrl Pts',(2.86574277996985,4.94124830641424,-6.7045866805003));
#156619=CARTESIAN_POINT('Ctrl Pts',(2.85774442166727,4.944589970506,-6.68551047643368));
#156620=CARTESIAN_POINT('Ctrl Pts',(2.84976106911649,4.94797287194898,-6.66643535407212));
#156621=CARTESIAN_POINT('Ctrl Pts',(3.56224604129919,4.81811592995226,-6.31244316851444));
#156622=CARTESIAN_POINT('Ctrl Pts',(3.55881627853959,4.81875342547613,-6.31437374918723));
#156623=CARTESIAN_POINT('Ctrl Pts',(3.55538651578,4.819390921,-6.31630432986));
#156624=CARTESIAN_POINT('Ctrl Pts',(3.54990409701001,4.82040994700001,-6.31939033098));
#156625=CARTESIAN_POINT('Ctrl Pts',(3.5444163292,4.821428571,-6.32246680877));
#156626=CARTESIAN_POINT('Ctrl Pts',(3.20461422651,4.884501699,-6.51296209527));
#156627=CARTESIAN_POINT('Ctrl Pts',(2.84635210687,4.948754474,-6.66593979512));
#156628=CARTESIAN_POINT('Ctrl Pts',(3.56156421782362,4.81811592995226,-6.31488893800906));
#156629=CARTESIAN_POINT('Ctrl Pts',(3.55813312741181,4.81875342547613,-6.31681914700453));
#156630=CARTESIAN_POINT('Ctrl Pts',(3.554702037,4.819390921,-6.318749356));
#156631=CARTESIAN_POINT('Ctrl Pts',(3.549217496,4.82040994700001,-6.321834763));
#156632=CARTESIAN_POINT('Ctrl Pts',(3.543727607,4.821428571,-6.324910643));
#156633=CARTESIAN_POINT('Ctrl Pts',(3.20379416,4.884501699,-6.515368914));
#156634=CARTESIAN_POINT('Ctrl Pts',(2.84540542,4.948754474,-6.668295734));
#156635=CARTESIAN_POINT('Ctrl Pts',(3.49338187026653,4.81811592995226,-6.55946588747069));
#156636=CARTESIAN_POINT('Ctrl Pts',(3.48981801463327,4.81875342547613,-6.56135892873535));
#156637=CARTESIAN_POINT('Ctrl Pts',(3.486254159,4.819390921,-6.56325197));
#156638=CARTESIAN_POINT('Ctrl Pts',(3.480557395,4.82040994700001,-6.56627796500001));
#156639=CARTESIAN_POINT('Ctrl Pts',(3.474855387,4.821428571,-6.569294066));
#156640=CARTESIAN_POINT('Ctrl Pts',(3.121787509,4.884501699,-6.756050787));
#156641=CARTESIAN_POINT('Ctrl Pts',(2.750736733,4.948754474,-6.90388962200001));
#156642=CARTESIAN_POINT('Origin',(-0.0530789841776808,5.088854266967,0.183496663322691));
#156643=CARTESIAN_POINT('Ctrl Pts',(4.25813567976833,4.95685569138745,-5.86555659771945));
#156644=CARTESIAN_POINT('Ctrl Pts',(3.91830476069365,4.88876675963424,-6.11225887305368));
#156645=CARTESIAN_POINT('Ctrl Pts',(3.55225701086,4.819390921,-6.31806487721999));
#156646=CARTESIAN_POINT('Ctrl Pts',(3.52818705236385,4.81482902010773,-6.33159792579308));
#156647=CARTESIAN_POINT('Ctrl Pts',(3.50411709386742,4.81026711921589,-6.34513097436566));
#156648=CARTESIAN_POINT('Ctrl Pts',(4.26064339410638,4.95685569138745,-5.86595413111433));
#156649=CARTESIAN_POINT('Ctrl Pts',(3.92078944326703,4.88876675963424,-6.11280169512173));
#156650=CARTESIAN_POINT('Ctrl Pts',(3.554702037,4.819390921,-6.318749356));
#156651=CARTESIAN_POINT('Ctrl Pts',(3.53062947084212,4.81482902010773,-6.33229171939924));
#156652=CARTESIAN_POINT('Ctrl Pts',(3.50655690468406,4.81026711921589,-6.34583408279862));
#156653=CARTESIAN_POINT('Ctrl Pts',(4.51141482791148,4.95685569138745,-5.9057074706027));
#156654=CARTESIAN_POINT('Ctrl Pts',(4.16925770060524,4.88876675963424,-6.16708390192625));
#156655=CARTESIAN_POINT('Ctrl Pts',(3.799204651,4.819390921,-6.387197234));
#156656=CARTESIAN_POINT('Ctrl Pts',(3.77487131866991,4.81482902010773,-6.40167108002116));
#156657=CARTESIAN_POINT('Ctrl Pts',(3.75053798634005,4.81026711921589,-6.41614492604184));
#156658=CARTESIAN_POINT('',(4.21622267410172,4.94797311771113,-5.89796293161155));
#156659=CARTESIAN_POINT('Origin',(-0.0760899040411644,4.69654718804145,
0.176806699785292));
#156660=CARTESIAN_POINT('Ctrl Pts',(4.25195902492911,4.93794661940964,-5.94869473723432));
#156661=CARTESIAN_POINT('Ctrl Pts',(4.24003125643147,4.94124830642766,-5.93178718271987));
#156662=CARTESIAN_POINT('Ctrl Pts',(4.2281190752871,4.94458997053798,-5.91487638029457));
#156663=CARTESIAN_POINT('Ctrl Pts',(4.21622178143906,4.9479728720019,-5.89796340846924));
#156664=CARTESIAN_POINT('Ctrl Pts',(4.83595139454949,4.81811592995224,-5.39908415713318));
#156665=CARTESIAN_POINT('Ctrl Pts',(4.83301683562474,4.81875342547612,-5.40170689882159));
#156666=CARTESIAN_POINT('Ctrl Pts',(4.8300822767,4.819390921,-5.40432964051));
#156667=CARTESIAN_POINT('Ctrl Pts',(4.82539143303,4.820409947,-5.40852204951));
#156668=CARTESIAN_POINT('Ctrl Pts',(4.82069331814,4.821428571,-5.41270630934));
#156669=CARTESIAN_POINT('Ctrl Pts',(4.52978645493,4.884501699,-5.67179532928999));
#156670=CARTESIAN_POINT('Ctrl Pts',(4.21278598864,4.948754474,-5.89821226196999));
#156671=CARTESIAN_POINT('Ctrl Pts',(4.83581127987154,4.81811592995224,-5.40161931777024));
#156672=CARTESIAN_POINT('Ctrl Pts',(4.83287534443577,4.81875342547612,-5.40424198188512));
#156673=CARTESIAN_POINT('Ctrl Pts',(4.829939409,4.819390921,-5.406864646));
#156674=CARTESIAN_POINT('Ctrl Pts',(4.825246365,4.820409947,-5.411056931));
#156675=CARTESIAN_POINT('Ctrl Pts',(4.82054605,4.821428571,-5.415241063));
#156676=CARTESIAN_POINT('Ctrl Pts',(4.529502956,4.884501699,-5.674322168));
#156677=CARTESIAN_POINT('Ctrl Pts',(4.212367892,4.948754474,-5.90071663));
#156678=CARTESIAN_POINT('Ctrl Pts',(4.82179981207699,4.81811592995224,-5.65513538147644));
#156679=CARTESIAN_POINT('Ctrl Pts',(4.81872622553849,4.81875342547612,-5.65775028823822));
#156680=CARTESIAN_POINT('Ctrl Pts',(4.815652639,4.819390921,-5.660365195));
#156681=CARTESIAN_POINT('Ctrl Pts',(4.81073956200001,4.820409947,-5.66454508));
#156682=CARTESIAN_POINT('Ctrl Pts',(4.805819236,4.821428571,-5.668716429));
#156683=CARTESIAN_POINT('Ctrl Pts',(4.501153063,4.884501699,-5.927006039));
#156684=CARTESIAN_POINT('Ctrl Pts',(4.170558228,4.948754474,-6.151153433));
#156685=CARTESIAN_POINT('Origin',(-0.0912841262940889,5.08885421242553,
0.167795861051647));
#156686=CARTESIAN_POINT('Ctrl Pts',(5.41950410049451,4.95685568701706,-4.81304986278409));
#156687=CARTESIAN_POINT('Ctrl Pts',(5.14065194348953,4.88876675740027,-5.12703796729849));
#156688=CARTESIAN_POINT('Ctrl Pts',(4.82740440351001,4.819390921,-5.4067217783));
#156689=CARTESIAN_POINT('Ctrl Pts',(4.8068063940441,4.81482902041816,-5.42511276003547));
#156690=CARTESIAN_POINT('Ctrl Pts',(4.78620838457831,4.81026711983679,-5.44350374177202));
#156691=CARTESIAN_POINT('Ctrl Pts',(5.42203864379239,4.95685568701706,-4.81289901763019));
#156692=CARTESIAN_POINT('Ctrl Pts',(5.14319522626593,4.88876675740027,-5.12703396517967));
#156693=CARTESIAN_POINT('Ctrl Pts',(4.829939409,4.819390921,-5.40686464600001));
#156694=CARTESIAN_POINT('Ctrl Pts',(4.80934085525011,4.81482902041816,-5.42526528535617));
#156695=CARTESIAN_POINT('Ctrl Pts',(4.78874230150022,4.81026711983679,-5.44366592471281));
#156696=CARTESIAN_POINT('Ctrl Pts',(5.67549297358001,4.95685568701706,-4.79781450224067));
#156697=CARTESIAN_POINT('Ctrl Pts',(5.39752350390582,4.88876675740026,-5.12663375329746));
#156698=CARTESIAN_POINT('Ctrl Pts',(5.083439958,4.819390921,-5.421151416));
#156699=CARTESIAN_POINT('Ctrl Pts',(5.06278697585029,4.81482902041816,-5.44051781742368));
#156700=CARTESIAN_POINT('Ctrl Pts',(5.04213399370004,4.81026711983679,-5.4598842188474));
#156701=CARTESIAN_POINT('',(5.38553741667845,4.94797309998007,-4.8537086189417));
#156702=CARTESIAN_POINT('Origin',(-0.112319138838276,4.69654718411941,0.156315944691232));
#156703=CARTESIAN_POINT('Ctrl Pts',(5.43134411167541,4.93794661940633,-4.89557205706981));
#156704=CARTESIAN_POINT('Ctrl Pts',(5.41606060857847,4.94124830110674,-4.88162393184319));
#156705=CARTESIAN_POINT('Ctrl Pts',(5.40079162965653,4.9445899597274,-4.86766928403193));
#156706=CARTESIAN_POINT('Ctrl Pts',(5.3855367237962,4.94797285563725,-4.85370931688512));
#156707=CARTESIAN_POINT('Ctrl Pts',(5.88353303667876,4.81811592995213,-4.23326996873311));
#156708=CARTESIAN_POINT('Ctrl Pts',(5.88123089797938,4.81875342547606,-4.23646223596155));
#156709=CARTESIAN_POINT('Ctrl Pts',(5.87892875928001,4.819390921,-4.23965450319));
#156710=CARTESIAN_POINT('Ctrl Pts',(5.87524882883,4.820409947,-4.2447572893));
#156711=CARTESIAN_POINT('Ctrl Pts',(5.87156004599,4.821428571,-4.24985367917));
#156712=CARTESIAN_POINT('Ctrl Pts',(5.64315090426,4.884501699,-4.56542171849));
#156713=CARTESIAN_POINT('Ctrl Pts',(5.38223467966999,4.948754474,-4.85469087829));
#156714=CARTESIAN_POINT('Ctrl Pts',(5.88394118241643,4.81811592995213,-4.23577597926327));
#156715=CARTESIAN_POINT('Ctrl Pts',(5.88163768270821,4.81875342547606,-4.23896846663164));
#156716=CARTESIAN_POINT('Ctrl Pts',(5.879334183,4.819390921,-4.242160954));
#156717=CARTESIAN_POINT('Ctrl Pts',(5.875652077,4.820409947,-4.247264092));
#156718=CARTESIAN_POINT('Ctrl Pts',(5.871961118,4.821428571,-4.25236083));
#156719=CARTESIAN_POINT('Ctrl Pts',(5.643417229,4.884501699,-4.567950425));
#156720=CARTESIAN_POINT('Ctrl Pts',(5.382364723,4.948754474,-4.857226574));
#156721=CARTESIAN_POINT('Ctrl Pts',(5.92475575618305,4.81811592995213,-4.4863770322797));
#156722=CARTESIAN_POINT('Ctrl Pts',(5.92231615559152,4.81875342547606,-4.48959153363985));
#156723=CARTESIAN_POINT('Ctrl Pts',(5.919876555,4.819390921,-4.492806035));
#156724=CARTESIAN_POINT('Ctrl Pts',(5.91597689399999,4.820409947,-4.497944362));
#156725=CARTESIAN_POINT('Ctrl Pts',(5.912068319,4.821428571,-4.503075913));
#156726=CARTESIAN_POINT('Ctrl Pts',(5.670049703,4.884501699,-4.820821076));
#156727=CARTESIAN_POINT('Ctrl Pts',(5.395369056,4.948754474,-5.110796145));
#156728=CARTESIAN_POINT('Origin',(-0.125223862622925,5.08885502181064,0.144251894682397));
#156729=CARTESIAN_POINT('Ctrl Pts',(6.32746257224836,4.95685569308826,-3.53549021668554));
#156730=CARTESIAN_POINT('Ctrl Pts',(6.12262797809732,4.88876676050363,-3.90208244265041));
#156731=CARTESIAN_POINT('Ctrl Pts',(5.8768277322,4.819390921,-4.24256637770999));
#156732=CARTESIAN_POINT('Ctrl Pts',(5.86066480615082,4.81482901928418,-4.26495535719707));
#156733=CARTESIAN_POINT('Ctrl Pts',(5.84450188010154,4.81026711756876,-4.28734433668393));
#156734=CARTESIAN_POINT('Ctrl Pts',(6.32990543207855,4.95685569308826,-3.53479804630303));
#156735=CARTESIAN_POINT('Ctrl Pts',(6.12511093998675,4.88876676050363,-3.90153180347262));
#156736=CARTESIAN_POINT('Ctrl Pts',(5.879334183,4.819390921,-4.242160954));
#156737=CARTESIAN_POINT('Ctrl Pts',(5.86317280149572,4.81482901928418,-4.26455948232562));
#156738=CARTESIAN_POINT('Ctrl Pts',(5.84701141999185,4.81026711756876,-4.28695801065105));
#156739=CARTESIAN_POINT('Ctrl Pts',(6.57419141509754,4.95685569308826,-3.46558100805243));
#156740=CARTESIAN_POINT('Ctrl Pts',(6.37340712892996,4.88876676050363,-3.84646788569382));
#156741=CARTESIAN_POINT('Ctrl Pts',(6.129979263,4.819390921,-4.201618583));
#156742=CARTESIAN_POINT('Ctrl Pts',(6.11397233598914,4.81482901928418,-4.22497199518201));
#156743=CARTESIAN_POINT('Ctrl Pts',(6.09796540897784,4.81026711756876,-4.24832540736376));
#156744=CARTESIAN_POINT('',(6.3030304192409,4.94797311771796,-3.58250023232274));
#156745=CARTESIAN_POINT('Origin',(-0.143296611127498,4.6965471432477,0.128516156270087));
#156746=CARTESIAN_POINT('Ctrl Pts',(6.35676558557265,4.93794661960481,-3.61353786707144));
#156747=CARTESIAN_POINT('Ctrl Pts',(6.33884093764623,4.94124830641803,-3.60320132726921));
#156748=CARTESIAN_POINT('Ctrl Pts',(6.32092907315555,4.94458997050698,-3.59285529378713));
#156749=CARTESIAN_POINT('Ctrl Pts',(6.30302980933956,4.94797287201421,-3.58250104001691));
#156750=CARTESIAN_POINT('Ctrl Pts',(6.65600721331838,4.81811592995226,-2.86951278315679));
#156751=CARTESIAN_POINT('Ctrl Pts',(6.6544451401742,4.81875342547613,-2.87312530844839));
#156752=CARTESIAN_POINT('Ctrl Pts',(6.65288306703001,4.819390921,-2.87673783374));
#156753=CARTESIAN_POINT('Ctrl Pts',(6.65038611907,4.820409947,-2.88251239538));
#156754=CARTESIAN_POINT('Ctrl Pts',(6.64787915151,4.821428571,-2.8882826146));
#156755=CARTESIAN_POINT('Ctrl Pts',(6.49264788863,4.884501699,-3.24557406119));
#156756=CARTESIAN_POINT('Ctrl Pts',(6.30001605838,4.948754474,-3.58416954491));
#156757=CARTESIAN_POINT('Ctrl Pts',(6.65694453501851,4.81811592995226,-2.87187246525453));
#156758=CARTESIAN_POINT('Ctrl Pts',(6.65538118000926,4.81875342547613,-2.87548549812727));
#156759=CARTESIAN_POINT('Ctrl Pts',(6.653817825,4.819390921,-2.879098531));
#156760=CARTESIAN_POINT('Ctrl Pts',(6.651318828,4.820409947,-2.884873904));
#156761=CARTESIAN_POINT('Ctrl Pts',(6.64880981,4.821428571,-2.890644931));
#156762=CARTESIAN_POINT('Ctrl Pts',(6.493451584,4.884501699,-3.247986396));
#156763=CARTESIAN_POINT('Ctrl Pts',(6.300688161,4.948754474,-3.586618002));
#156764=CARTESIAN_POINT('Ctrl Pts',(6.75067670503122,4.81811592995226,-3.1078406750286));
#156765=CARTESIAN_POINT('Ctrl Pts',(6.74898516351561,4.81875342547613,-3.1115044660143));
#156766=CARTESIAN_POINT('Ctrl Pts',(6.747293622,4.819390921,-3.115168257));
#156767=CARTESIAN_POINT('Ctrl Pts',(6.744589721,4.820409947,-3.121024766));
#156768=CARTESIAN_POINT('Ctrl Pts',(6.741875659,4.821428571,-3.126876571));
#156769=CARTESIAN_POINT('Ctrl Pts',(6.573821121,4.884501699,-3.489219877));
#156770=CARTESIAN_POINT('Ctrl Pts',(6.36789842300001,4.948754474,-3.831463711));
#156771=CARTESIAN_POINT('Origin',(-0.153306328492075,5.08885506698253,0.11396006920804));
#156772=CARTESIAN_POINT('Ctrl Pts',(6.93955589199911,4.9568556875656,-2.09261503770074));
#156773=CARTESIAN_POINT('Ctrl Pts',(6.81831671158644,4.88876675768066,-2.49466990755172));
#156774=CARTESIAN_POINT('Ctrl Pts',(6.65145712774,4.819390921,-2.88003328896));
#156775=CARTESIAN_POINT('Ctrl Pts',(6.6404850525028,4.81482902001618,-2.90537337382057));
#156776=CARTESIAN_POINT('Ctrl Pts',(6.62951297726621,4.81026711903278,-2.93071345868095));
#156777=CARTESIAN_POINT('Ctrl Pts',(6.9417928429581,4.9568556875656,-2.09141390723561));
#156778=CARTESIAN_POINT('Ctrl Pts',(6.82062325206529,4.88876675768066,-2.49359837861227));
#156779=CARTESIAN_POINT('Ctrl Pts',(6.653817825,4.819390921,-2.879098531));
#156780=CARTESIAN_POINT('Ctrl Pts',(6.64284931091445,4.81482902001618,-2.90444760941933));
#156781=CARTESIAN_POINT('Ctrl Pts',(6.63188079682888,4.81026711903278,-2.92979668783863));
#156782=CARTESIAN_POINT('Ctrl Pts',(7.16548793885633,4.9568556875656,-1.9713008607217));
#156783=CARTESIAN_POINT('Ctrl Pts',(7.0512772999503,4.88876675768066,-2.38644548466673));
#156784=CARTESIAN_POINT('Ctrl Pts',(6.889887551,4.819390921,-2.785622735));
#156785=CARTESIAN_POINT('Ctrl Pts',(6.87927515207644,4.81482902001618,-2.81187116929824));
#156786=CARTESIAN_POINT('Ctrl Pts',(6.86866275315322,4.81026711903278,-2.83811960359658));
#156787=CARTESIAN_POINT('',(6.92580073240705,4.94797309995735,-2.14377816991343));
#156788=CARTESIAN_POINT('Origin',(-0.167573576195836,4.69654721101772,0.0947069641933204));
#156789=CARTESIAN_POINT('Ctrl Pts',(6.98495176452533,4.93794661944175,-2.16253866418928));
#156790=CARTESIAN_POINT('Ctrl Pts',(6.96522416660578,4.94124830102568,-2.1562970657359));
#156791=CARTESIAN_POINT('Ctrl Pts',(6.94550701213803,4.94458995962433,-2.1500434483145));
#156792=CARTESIAN_POINT('Ctrl Pts',(6.92580039661835,4.94797285546969,-2.14377909421981));
#156793=CARTESIAN_POINT('Ctrl Pts',(7.11725388874147,4.81811592995212,-1.37158036941615));
#156794=CARTESIAN_POINT('Ctrl Pts',(7.11650492238074,4.81875342547606,-1.37544423513808));
#156795=CARTESIAN_POINT('Ctrl Pts',(7.11575595602,4.819390921,-1.37930810086));
#156796=CARTESIAN_POINT('Ctrl Pts',(7.11455874574,4.820409947,-1.385484426));
#156797=CARTESIAN_POINT('Ctrl Pts',(7.11335081559,4.821428571,-1.39165866431));
#156798=CARTESIAN_POINT('Ctrl Pts',(7.03855587389999,4.884501699,-1.77396696899));
#156799=CARTESIAN_POINT('Ctrl Pts',(6.92321568887,4.948754474,-2.14605642768));
#156800=CARTESIAN_POINT('Ctrl Pts',(7.11867655828793,4.81811592995212,-1.373683387019));
#156801=CARTESIAN_POINT('Ctrl Pts',(7.11792644914396,4.81875342547606,-1.3775480240095));
#156802=CARTESIAN_POINT('Ctrl Pts',(7.11717634,4.819390921,-1.381412661));
#156803=CARTESIAN_POINT('Ctrl Pts',(7.115977303,4.820409947,-1.387590219));
#156804=CARTESIAN_POINT('Ctrl Pts',(7.114767544,4.821428571,-1.393765687));
#156805=CARTESIAN_POINT('Ctrl Pts',(7.03985936,4.884501699,-1.776150134));
#156806=CARTESIAN_POINT('Ctrl Pts',(6.92439842400001,4.948754474,-2.148303159));
#156807=CARTESIAN_POINT('Ctrl Pts',(7.26094351293389,4.81811592995212,-1.58398514730385));
#156808=CARTESIAN_POINT('Ctrl Pts',(7.26007912546694,4.81875342547606,-1.58792691115193));
#156809=CARTESIAN_POINT('Ctrl Pts',(7.259214738,4.819390921,-1.591868675));
#156810=CARTESIAN_POINT('Ctrl Pts',(7.257833029,4.820409947,-1.598169519));
#156811=CARTESIAN_POINT('Ctrl Pts',(7.256440385,4.821428571,-1.604467956));
#156812=CARTESIAN_POINT('Ctrl Pts',(7.17020797,4.884501699,-1.994466635));
#156813=CARTESIAN_POINT('Ctrl Pts',(7.042671937,4.948754474,-2.372976291));
#156814=CARTESIAN_POINT('Origin',(-0.174217518094983,5.08885440428902,0.0783386349219456));
#156815=CARTESIAN_POINT('Ctrl Pts',(7.22716330708476,4.95685568851546,-0.551891470492521));
#156816=CARTESIAN_POINT('Ctrl Pts',(7.19518854433772,4.88876675816619,-0.970609363519733));
#156817=CARTESIAN_POINT('Ctrl Pts',(7.11507177985001,4.819390921,-1.38283304498));
#156818=CARTESIAN_POINT('Ctrl Pts',(7.10980359427104,4.81482901954,-1.40993936745616));
#156819=CARTESIAN_POINT('Ctrl Pts',(7.10453540869258,4.81026711808047,-1.43704568993249));
#156820=CARTESIAN_POINT('Ctrl Pts',(7.2290897518345,4.95685568851546,-0.550237543452612));
#156821=CARTESIAN_POINT('Ctrl Pts',(7.19721081214112,4.88876675816619,-0.96906704830979));
#156822=CARTESIAN_POINT('Ctrl Pts',(7.11717634000001,4.819390921,-1.381412661));
#156823=CARTESIAN_POINT('Ctrl Pts',(7.11191356566496,4.81482901954,-1.40852700122815));
#156824=CARTESIAN_POINT('Ctrl Pts',(7.10665079133035,4.81026711808047,-1.43564134145638));
#156825=CARTESIAN_POINT('Ctrl Pts',(7.42173422680767,4.95685568851546,-0.384844839461617));
#156826=CARTESIAN_POINT('Ctrl Pts',(7.39943759248132,4.88876675816619,-0.814835527315462));
#156827=CARTESIAN_POINT('Ctrl Pts',(7.327632355,4.819390921,-1.239374263));
#156828=CARTESIAN_POINT('Ctrl Pts',(7.32291070505559,4.81482901954,-1.26729037842628));
#156829=CARTESIAN_POINT('Ctrl Pts',(7.31818905511107,4.81026711808047,-1.2952064938526));
#156830=CARTESIAN_POINT('',(7.22472829738214,4.94797309996594,-0.604815395171998));
#156831=CARTESIAN_POINT('Origin',(-0.18401515634942,4.69654714103903,0.0564694460061609));
#156832=CARTESIAN_POINT('Ctrl Pts',(7.28652936242152,4.93794661929278,-0.610421556976864));
#156833=CARTESIAN_POINT('Ctrl Pts',(7.26592122571832,4.94124830102619,-0.608566733030478));
#156834=CARTESIAN_POINT('Ctrl Pts',(7.24532070465871,4.94458995961649,-0.606697926929616));
#156835=CARTESIAN_POINT('Ctrl Pts',(7.22472816812392,4.94797285536847,-0.604816370059737));
#156836=CARTESIAN_POINT('Ctrl Pts',(7.24570568262718,4.81811592995212,0.190485620212301));
#156837=CARTESIAN_POINT('Ctrl Pts',(7.24580484410859,4.81875342547606,0.186551083671151));
#156838=CARTESIAN_POINT('Ctrl Pts',(7.24590400559,4.819390921,0.18261654713));
#156839=CARTESIAN_POINT('Ctrl Pts',(7.24606251356999,4.820409947,0.17632725586));
#156840=CARTESIAN_POINT('Ctrl Pts',(7.24621010232,4.821428571,0.17003769794));
#156841=CARTESIAN_POINT('Ctrl Pts',(7.25534880874,4.884501699,-0.21941115215));
#156842=CARTESIAN_POINT('Ctrl Pts',(7.22269344875,4.948754474,-0.60759609609));
#156843=CARTESIAN_POINT('Ctrl Pts',(7.24754717756366,4.81811592995212,0.188737601888497));
#156844=CARTESIAN_POINT('Ctrl Pts',(7.24764538878184,4.81875342547606,0.184802066444248));
#156845=CARTESIAN_POINT('Ctrl Pts',(7.2477436,4.819390921,0.180866531));
#156846=CARTESIAN_POINT('Ctrl Pts',(7.247900589,4.820409947,0.174575643));
#156847=CARTESIAN_POINT('Ctrl Pts',(7.248046656,4.821428571,0.168284491));
#156848=CARTESIAN_POINT('Ctrl Pts',(7.257091136,4.884501699,-0.221263065));
#156849=CARTESIAN_POINT('Ctrl Pts',(7.224331513,4.948754474,-0.609536047));
#156850=CARTESIAN_POINT('Ctrl Pts',(7.43169667121216,4.81811592995212,0.0139357695080179));
#156851=CARTESIAN_POINT('Ctrl Pts',(7.43169985610608,4.81875342547606,0.00990034375400896));
#156852=CARTESIAN_POINT('Ctrl Pts',(7.431703041,4.819390921,0.005864918));
#156853=CARTESIAN_POINT('Ctrl Pts',(7.431708132,4.820409947,-0.000585643));
#156854=CARTESIAN_POINT('Ctrl Pts',(7.431702024,4.821428571,-0.007036203));
#156855=CARTESIAN_POINT('Ctrl Pts',(7.431323862,4.884501699,-0.40645435));
#156856=CARTESIAN_POINT('Ctrl Pts',(7.388137938,4.948754474,-0.803531138));
#156857=CARTESIAN_POINT('Origin',(-0.186981779434326,5.08885376242707,0.0390553085750223));
#156858=CARTESIAN_POINT('Ctrl Pts',(7.17683659769354,4.95685568833166,1.01463792187901));
#156859=CARTESIAN_POINT('Ctrl Pts',(7.23562135714399,4.88876675807225,0.59883579236326));
#156860=CARTESIAN_POINT('Ctrl Pts',(7.24599358387,4.819390921,0.1790269366));
#156861=CARTESIAN_POINT('Ctrl Pts',(7.24667562358123,4.81482901957461,0.151421840960049));
#156862=CARTESIAN_POINT('Ctrl Pts',(7.24735766329251,4.81026711814964,0.123816745320095));
#156863=CARTESIAN_POINT('Ctrl Pts',(7.1783624578197,4.95685568833166,1.01666730969899));
#156864=CARTESIAN_POINT('Ctrl Pts',(7.23726479326338,4.88876675807225,0.600776776901795));
#156865=CARTESIAN_POINT('Ctrl Pts',(7.2477436,4.819390921,0.180866531));
#156866=CARTESIAN_POINT('Ctrl Pts',(7.24843264802317,4.81482901957461,0.153254768315198));
#156867=CARTESIAN_POINT('Ctrl Pts',(7.2491216960458,4.81026711814964,0.125643005630368));
#156868=CARTESIAN_POINT('Ctrl Pts',(7.33094847043569,4.95685568833166,1.21960609169697));
#156869=CARTESIAN_POINT('Ctrl Pts',(7.40160840520117,4.88876675807225,0.794875230755259));
#156870=CARTESIAN_POINT('Ctrl Pts',(7.422745213,4.819390921,0.364825971));
#156871=CARTESIAN_POINT('Ctrl Pts',(7.42413509221002,4.81482901957461,0.336547503829866));
#156872=CARTESIAN_POINT('Ctrl Pts',(7.42552497141996,4.81026711814964,0.3082690366597));
#156873=CARTESIAN_POINT('',(7.18583559604642,4.94797309996092,0.962427875205284));
#156874=CARTESIAN_POINT('Origin',(-0.191852051531565,4.69654718848674,0.0155914013782869));
#156875=CARTESIAN_POINT('Ctrl Pts',(7.24739694602179,4.93794661920552,0.970238183677667));
#156876=CARTESIAN_POINT('Ctrl Pts',(7.2268718837182,4.94124830101889,0.967619503186338));
#156877=CARTESIAN_POINT('Ctrl Pts',(7.20635125317722,4.94458995960823,0.965016114428145));
#156878=CARTESIAN_POINT('Ctrl Pts',(7.18583567941776,4.94797285540608,0.962426895097326));
#156879=CARTESIAN_POINT('Ctrl Pts',(7.03535633396982,4.81811592995228,1.74364471283293));
#156880=CARTESIAN_POINT('Ctrl Pts',(7.03629898575991,4.81875342547614,1.73982348006647));
#156881=CARTESIAN_POINT('Ctrl Pts',(7.03724163755,4.819390921,1.7360022473));
#156882=CARTESIAN_POINT('Ctrl Pts',(7.03874845077001,4.820409947,1.72989407023));
#156883=CARTESIAN_POINT('Ctrl Pts',(7.04024465825,4.821428571,1.72378328719));
#156884=CARTESIAN_POINT('Ctrl Pts',(7.13288969786,4.884501699,1.34540408529));
#156885=CARTESIAN_POINT('Ctrl Pts',(7.18444608966999,4.948754474,0.95927475253));
#156886=CARTESIAN_POINT('Ctrl Pts',(7.03753054804711,4.81811592995228,1.74233342918212));
#156887=CARTESIAN_POINT('Ctrl Pts',(7.03847248652355,4.81875342547614,1.73851101659106));
#156888=CARTESIAN_POINT('Ctrl Pts',(7.039414425,4.819390921,1.734688604));
#156889=CARTESIAN_POINT('Ctrl Pts',(7.040920098,4.820409947,1.728578541));
#156890=CARTESIAN_POINT('Ctrl Pts',(7.042415162,4.821428571,1.722465874));
#156891=CARTESIAN_POINT('Ctrl Pts',(7.134989397,4.884501699,1.343970018));
#156892=CARTESIAN_POINT('Ctrl Pts',(7.186462889,4.948754474,0.957732292));
#156893=CARTESIAN_POINT('Ctrl Pts',(7.25495195577528,4.81811592995228,1.61120506410024));
#156894=CARTESIAN_POINT('Ctrl Pts',(7.25582256288765,4.81875342547614,1.60726466905012));
#156895=CARTESIAN_POINT('Ctrl Pts',(7.25669317,4.819390921,1.603324274));
#156896=CARTESIAN_POINT('Ctrl Pts',(7.258084821,4.820409947,1.597025618));
#156897=CARTESIAN_POINT('Ctrl Pts',(7.259465537,4.821428571,1.590724555));
#156898=CARTESIAN_POINT('Ctrl Pts',(7.344959311,4.884501699,1.200563289));
#156899=CARTESIAN_POINT('Ctrl Pts',(7.388142822,4.948754474,0.803486239));
#156900=CARTESIAN_POINT('Origin',(-0.191011727371936,5.08885504122789,-0.00205421031792302));
#156901=CARTESIAN_POINT('Ctrl Pts',(6.79092898502783,4.95685568875588,2.5337239759622));
#156902=CARTESIAN_POINT('Ctrl Pts',(6.93772455677668,4.88876675828909,2.14028005350535));
#156903=CARTESIAN_POINT('Ctrl Pts',(7.0381007817,4.819390921,1.73251581655));
#156904=CARTESIAN_POINT('Ctrl Pts',(7.04470115542056,4.81482901947769,1.70570273052457));
#156905=CARTESIAN_POINT('Ctrl Pts',(7.05130152914082,4.81026711795524,1.67888964449888));
#156906=CARTESIAN_POINT('Ctrl Pts',(6.79198291299492,4.95685568875588,2.53603393264285));
#156907=CARTESIAN_POINT('Ctrl Pts',(6.9389123159695,4.88876675828909,2.14252894909245));
#156908=CARTESIAN_POINT('Ctrl Pts',(7.039414425,4.819390921,1.734688604));
#156909=CARTESIAN_POINT('Ctrl Pts',(7.04602307639943,4.81482901947769,1.70787051338158));
#156910=CARTESIAN_POINT('Ctrl Pts',(7.0526317277983,4.81026711795524,1.68105242276316));
#156911=CARTESIAN_POINT('Ctrl Pts',(6.89737570970381,4.95685568875588,2.76702960070795));
#156912=CARTESIAN_POINT('Ctrl Pts',(7.05768823525181,4.88876675828909,2.36741850780217));
#156913=CARTESIAN_POINT('Ctrl Pts',(7.170778755,4.819390921,1.951967349));
#156914=CARTESIAN_POINT('Ctrl Pts',(7.17821517428315,4.81482901947769,1.92464879908613));
#156915=CARTESIAN_POINT('Ctrl Pts',(7.18565159356626,4.81026711795524,1.89733024917257));
#156916=CARTESIAN_POINT('',(6.81094120886271,4.94797309996511,2.48466908736485));
#156917=CARTESIAN_POINT('Origin',(-0.190718463343362,4.69654718882403,-0.0260156744271445));
#156918=CARTESIAN_POINT('Ctrl Pts',(6.869384302947,4.93794661951538,2.50553066725023));
#156919=CARTESIAN_POINT('Ctrl Pts',(6.84990204463961,4.9412483010766,2.49856092685401));
#156920=CARTESIAN_POINT('Ctrl Pts',(6.83042082661489,4.94458995967786,2.49160707485885));
#156921=CARTESIAN_POINT('Ctrl Pts',(6.81094150090676,4.94797285556573,2.48466814837251));
#156922=CARTESIAN_POINT('Ctrl Pts',(6.49604154141455,4.81811592995212,3.21527291645958));
#156923=CARTESIAN_POINT('Ctrl Pts',(6.49778360652728,4.81875342547606,3.21174366421979));
#156924=CARTESIAN_POINT('Ctrl Pts',(6.49952567164,4.819390921,3.20821441198));
#156925=CARTESIAN_POINT('Ctrl Pts',(6.50231033377,4.820409947,3.20257296093));
#156926=CARTESIAN_POINT('Ctrl Pts',(6.50508519853,4.821428571,3.19692668465));
#156927=CARTESIAN_POINT('Ctrl Pts',(6.67690459158,4.884501699,2.84730972435));
#156928=CARTESIAN_POINT('Ctrl Pts',(6.81026201690001,4.948754474,2.48129098042));
#156929=CARTESIAN_POINT('Ctrl Pts',(6.49844681077687,4.81811592995212,3.21445968164217));
#156930=CARTESIAN_POINT('Ctrl Pts',(6.50018843288844,4.81875342547606,3.21092912382109));
#156931=CARTESIAN_POINT('Ctrl Pts',(6.501930055,4.819390921,3.207398566));
#156932=CARTESIAN_POINT('Ctrl Pts',(6.504714009,4.820409947,3.201755028));
#156933=CARTESIAN_POINT('Ctrl Pts',(6.507488162,4.821428571,3.196106666));
#156934=CARTESIAN_POINT('Ctrl Pts',(6.679263483,4.884501699,2.846360558));
#156935=CARTESIAN_POINT('Ctrl Pts',(6.81256324800001,4.948754474,2.480218134));
#156936=CARTESIAN_POINT('Ctrl Pts',(6.73897374700992,4.81811592995212,3.13313619990097));
#156937=CARTESIAN_POINT('Ctrl Pts',(6.74067106900496,4.81875342547606,3.12947508395048));
#156938=CARTESIAN_POINT('Ctrl Pts',(6.742368391,4.819390921,3.125813968));
#156939=CARTESIAN_POINT('Ctrl Pts',(6.745081532,4.820409947,3.119961735));
#156940=CARTESIAN_POINT('Ctrl Pts',(6.747784509,4.821428571,3.114104801));
#156941=CARTESIAN_POINT('Ctrl Pts',(6.91515262499999,4.884501699,2.751443923));
#156942=CARTESIAN_POINT('Ctrl Pts',(7.042686358,4.948754474,2.372933492));
#156943=CARTESIAN_POINT('Origin',(-0.186104172907255,5.08885501602928,-0.0430679738727974));
#156944=CARTESIAN_POINT('Ctrl Pts',(6.08748506749854,4.95685569264032,3.93433593143617));
#156945=CARTESIAN_POINT('Ctrl Pts',(6.31542746113433,4.88876676027466,3.58164720780548));
#156946=CARTESIAN_POINT('Ctrl Pts',(6.50111420902001,4.819390921,3.20499418263));
#156947=CARTESIAN_POINT('Ctrl Pts',(6.51332429053711,4.81482901950453,3.18022685704854));
#156948=CARTESIAN_POINT('Ctrl Pts',(6.52553437205403,4.8102671180095,3.1554595314668));
#156949=CARTESIAN_POINT('Ctrl Pts',(6.08801778279943,4.95685569264032,3.93681844597466));
#156950=CARTESIAN_POINT('Ctrl Pts',(6.3161040050993,4.88876676027466,3.58409885859014));
#156951=CARTESIAN_POINT('Ctrl Pts',(6.501930055,4.819390921,3.207398566));
#156952=CARTESIAN_POINT('Ctrl Pts',(6.51414929650819,4.81482901950453,3.18262813228619));
#156953=CARTESIAN_POINT('Ctrl Pts',(6.52636853801631,4.8102671180095,3.15785769857232));
#156954=CARTESIAN_POINT('Ctrl Pts',(6.14128931288863,4.95685569264032,4.18506989982365));
#156955=CARTESIAN_POINT('Ctrl Pts',(6.38375840159689,4.88876676027466,3.82926393705604));
#156956=CARTESIAN_POINT('Ctrl Pts',(6.583514653,4.819390921,3.447836903));
#156957=CARTESIAN_POINT('Ctrl Pts',(6.59664989361871,4.81482901950453,3.42275565605227));
#156958=CARTESIAN_POINT('Ctrl Pts',(6.60978513423729,4.8102671180095,3.3976744091045));
#156959=CARTESIAN_POINT('',(6.11757475519473,4.94797311771029,3.89072994474234));
#156960=CARTESIAN_POINT('Origin',(-0.180667002327166,4.69654715766115,-0.0664062771459656));
#156961=CARTESIAN_POINT('Ctrl Pts',(6.17016688510887,4.93794661935354,3.92366731976889));
#156962=CARTESIAN_POINT('Ctrl Pts',(6.15263837057492,4.94124830638632,3.91267240131556));
#156963=CARTESIAN_POINT('Ctrl Pts',(6.13510745688151,4.94458997046307,3.90169322281712));
#156964=CARTESIAN_POINT('Ctrl Pts',(6.11757518297218,4.94797287189733,3.89072902756295));
#156965=CARTESIAN_POINT('Ctrl Pts',(5.65297906669916,4.81811592995212,4.53655853165158));
#156966=CARTESIAN_POINT('Ctrl Pts',(5.65543908785958,4.81875342547607,4.53348628412579));
#156967=CARTESIAN_POINT('Ctrl Pts',(5.65789910902,4.819390921,4.53041403660001));
#156968=CARTESIAN_POINT('Ctrl Pts',(5.66183141196,4.820409947,4.52550309999));
#156969=CARTESIAN_POINT('Ctrl Pts',(5.66575518471,4.821428571,4.52058534395));
#156970=CARTESIAN_POINT('Ctrl Pts',(5.90871484845,4.884501699,4.21607832444));
#156971=CARTESIAN_POINT('Ctrl Pts',(6.11763766114001,4.948754474,3.88728480021));
#156972=CARTESIAN_POINT('Ctrl Pts',(5.65550292364228,4.81811592995212,4.53628137163685));
#156973=CARTESIAN_POINT('Ctrl Pts',(5.65796279282114,4.81875342547607,4.53320775381843));
#156974=CARTESIAN_POINT('Ctrl Pts',(5.660422662,4.819390921,4.530134136));
#156975=CARTESIAN_POINT('Ctrl Pts',(5.664354722,4.820409947,4.525221009));
#156976=CARTESIAN_POINT('Ctrl Pts',(5.668278248,4.821428571,4.520301063));
#156977=CARTESIAN_POINT('Ctrl Pts',(5.911222633,4.884501699,4.215658441));
#156978=CARTESIAN_POINT('Ctrl Pts',(6.120115721,4.948754474,3.886731733));
#156979=CARTESIAN_POINT('Ctrl Pts',(5.90788861795456,4.81811592995212,4.50856537016347));
#156980=CARTESIAN_POINT('Ctrl Pts',(5.91033328897728,4.81875342547607,4.50535472308173));
#156981=CARTESIAN_POINT('Ctrl Pts',(5.91277796,4.819390921,4.50214407600001));
#156982=CARTESIAN_POINT('Ctrl Pts',(5.916685726,4.820409947,4.49701191));
#156983=CARTESIAN_POINT('Ctrl Pts',(5.920584577,4.821428571,4.491872968));
#156984=CARTESIAN_POINT('Ctrl Pts',(6.162001088,4.884501699,4.173670097));
#156985=CARTESIAN_POINT('Ctrl Pts',(6.367921707,4.948754474,3.831425012));
#156986=CARTESIAN_POINT('Origin',(-0.172494949443869,5.08885499938439,-0.0820680645597976));
#156987=CARTESIAN_POINT('Ctrl Pts',(5.09939714484627,4.95685568743367,5.15098266598226));
#156988=CARTESIAN_POINT('Ctrl Pts',(5.39782800952324,4.88876675761323,4.85554049568293));
#156989=CARTESIAN_POINT('Ctrl Pts',(5.6601427614,4.819390921,4.52761058301));
#156990=CARTESIAN_POINT('Ctrl Pts',(5.6773916183094,4.81482902019137,4.50604711355382));
#156991=CARTESIAN_POINT('Ctrl Pts',(5.6946404752189,4.81026711938254,4.48448364409787));
#156992=CARTESIAN_POINT('Ctrl Pts',(5.09938373833295,4.95685568743367,5.15352165875207));
#156993=CARTESIAN_POINT('Ctrl Pts',(5.39796170382317,4.88876675761323,4.85808026518442));
#156994=CARTESIAN_POINT('Ctrl Pts',(5.660422662,4.819390921,4.530134136));
#156995=CARTESIAN_POINT('Ctrl Pts',(5.67768113289997,4.81482902019137,4.50856960020544));
#156996=CARTESIAN_POINT('Ctrl Pts',(5.69493960379982,4.81026711938254,4.48700506441108));
#156997=CARTESIAN_POINT('Ctrl Pts',(5.09804308700086,4.95685568743367,5.40742093573342));
#156998=CARTESIAN_POINT('Ctrl Pts',(5.41133113381643,4.88876675761323,5.11205721533326));
#156999=CARTESIAN_POINT('Ctrl Pts',(5.688412722,4.819390921,4.782489435));
#157000=CARTESIAN_POINT('Ctrl Pts',(5.70663259195628,4.81482902019137,4.76081826536794));
#157001=CARTESIAN_POINT('Ctrl Pts',(5.72485246191249,4.81026711938254,4.73914709573632));
#157002=CARTESIAN_POINT('',(5.13815735487595,4.94797309995233,5.11486457517324));
#157003=CARTESIAN_POINT('Origin',(-0.162167537007684,4.69654715563134,-0.10369164188563));
#157004=CARTESIAN_POINT('Ctrl Pts',(5.18243932158301,4.93794661922244,5.15833764928942));
#157005=CARTESIAN_POINT('Ctrl Pts',(5.1676842196987,4.94124830104337,5.14383169758156));
#157006=CARTESIAN_POINT('Ctrl Pts',(5.15292339167731,4.94458995965422,5.12934060138166));
#157007=CARTESIAN_POINT('Ctrl Pts',(5.13815801437043,4.94797285546854,5.11486384540008));
#157008=CARTESIAN_POINT('Ctrl Pts',(4.54558957227979,4.81811592995213,5.64571971271425));
#157009=CARTESIAN_POINT('Ctrl Pts',(4.54865252210489,4.81875342547607,5.64324812455213));
#157010=CARTESIAN_POINT('Ctrl Pts',(4.55171547193,4.819390921,5.64077653638999));
#157011=CARTESIAN_POINT('Ctrl Pts',(4.55661154632,4.820409947,5.63682574379));
#157012=CARTESIAN_POINT('Ctrl Pts',(4.56150075553,4.821428571,5.6328664576));
#157013=CARTESIAN_POINT('Ctrl Pts',(4.86424016452,4.884501699,5.38770778825));
#157014=CARTESIAN_POINT('Ctrl Pts',(5.1389593677,4.948754474,5.11151350319));
#157015=CARTESIAN_POINT('Ctrl Pts',(4.54811400406023,4.81811592995213,5.64599158717321));
#157016=CARTESIAN_POINT('Ctrl Pts',(4.55117710003011,4.81875342547607,5.64351862808661));
#157017=CARTESIAN_POINT('Ctrl Pts',(4.554240196,4.819390921,5.641045669));
#157018=CARTESIAN_POINT('Ctrl Pts',(4.559136504,4.820409947,5.637092685));
#157019=CARTESIAN_POINT('Ctrl Pts',(4.564025943,4.821428571,5.633131207));
#157020=CARTESIAN_POINT('Ctrl Pts',(4.866779581,4.884501699,5.387836821));
#157021=CARTESIAN_POINT('Ctrl Pts',(5.141498385,4.948754474,5.111506076));
#157022=CARTESIAN_POINT('Ctrl Pts',(4.80055718210447,4.81811592995213,5.67317903306961));
#157023=CARTESIAN_POINT('Ctrl Pts',(4.80363489255224,4.81875342547607,5.67056898153481));
#157024=CARTESIAN_POINT('Ctrl Pts',(4.806712603,4.819390921,5.66795893));
#157025=CARTESIAN_POINT('Ctrl Pts',(4.811632272,4.820409947,5.663786806));
#157026=CARTESIAN_POINT('Ctrl Pts',(4.81654469,4.821428571,5.659606147));
#157027=CARTESIAN_POINT('Ctrl Pts',(5.120721229,4.884501699,5.400740096));
#157028=CARTESIAN_POINT('Ctrl Pts',(5.39540011500001,4.948754474,5.110763357));
#157029=CARTESIAN_POINT('Origin',(-0.150820013878292,5.08885506147785,-0.117230767712908));
#157030=CARTESIAN_POINT('Ctrl Pts',(3.87286705614322,4.95685568876092,6.12677520712686));
#157031=CARTESIAN_POINT('Ctrl Pts',(4.22783210957198,4.88876675829167,5.9023941230321));
#157032=CARTESIAN_POINT('Ctrl Pts',(4.55450932862001,4.819390921,5.63852094492999));
#157033=CARTESIAN_POINT('Ctrl Pts',(4.57599042881487,4.8148290194499,5.62116960897195));
#157034=CARTESIAN_POINT('Ctrl Pts',(4.59747152901017,4.81026711789965,5.60381827301339));
#157035=CARTESIAN_POINT('Ctrl Pts',(3.87230815465685,4.95685568876092,6.12925195764689));
#157036=CARTESIAN_POINT('Ctrl Pts',(4.22741670280422,4.88876675829167,5.90490325445912));
#157037=CARTESIAN_POINT('Ctrl Pts',(4.554240196,4.819390921,5.641045669));
#157038=CARTESIAN_POINT('Ctrl Pts',(4.57573091464835,4.8148290194499,5.62369535835715));
#157039=CARTESIAN_POINT('Ctrl Pts',(4.59722163329677,4.81026711789965,5.60634504771392));
#157040=CARTESIAN_POINT('Ctrl Pts',(3.81641800601945,4.95685568876092,6.3769270096507));
#157041=CARTESIAN_POINT('Ctrl Pts',(4.1858760260283,4.88876675829167,6.15581639716052));
#157042=CARTESIAN_POINT('Ctrl Pts',(4.527326934,4.819390921,5.893518076));
#157043=CARTESIAN_POINT('Ctrl Pts',(4.54977949799321,4.8148290194499,5.87627029687959));
#157044=CARTESIAN_POINT('Ctrl Pts',(4.57223206198565,4.81026711789965,5.85902251775936));
#157045=CARTESIAN_POINT('',(3.91848540259602,4.94797309996321,6.09983383216804));
#157046=CARTESIAN_POINT('Origin',(-0.136085764728019,4.69654715609852,-0.13612896908482));
#157047=CARTESIAN_POINT('Ctrl Pts',(3.95238665388103,4.93794661950124,6.15180984468191));
#157048=CARTESIAN_POINT('Ctrl Pts',(3.9410948705015,4.94124830105337,6.13447112212709));
#157049=CARTESIAN_POINT('Ctrl Pts',(3.92979429991244,4.9445899596633,6.11714567805156));
#157050=CARTESIAN_POINT('Ctrl Pts',(3.91848620333279,4.94797285553905,6.09983326138289));
#157051=CARTESIAN_POINT('Ctrl Pts',(3.22565336150107,4.81811592995213,6.49089331482735));
#157052=CARTESIAN_POINT('Ctrl Pts',(3.22917601981553,4.81875342547607,6.48913795466867));
#157053=CARTESIAN_POINT('Ctrl Pts',(3.23269867813,4.819390921,6.48738259451));
#157054=CARTESIAN_POINT('Ctrl Pts',(3.2383295889,4.820409947,6.48457668047));
#157055=CARTESIAN_POINT('Ctrl Pts',(3.2439556203,4.821428571,6.48176099564));
#157056=CARTESIAN_POINT('Ctrl Pts',(3.59231901789,4.884501699,6.30741402349));
#157057=CARTESIAN_POINT('Ctrl Pts',(3.91998904488,4.948754474,6.09673351488));
#157058=CARTESIAN_POINT('Ctrl Pts',(3.22806032850429,4.81811592995213,6.491701511246));
#157059=CARTESIAN_POINT('Ctrl Pts',(3.23158342425215,4.81875342547607,6.489944843623));
#157060=CARTESIAN_POINT('Ctrl Pts',(3.23510652,4.819390921,6.48818817600001));
#157061=CARTESIAN_POINT('Ctrl Pts',(3.24073813,4.820409947,6.485380172));
#157062=CARTESIAN_POINT('Ctrl Pts',(3.246364857,4.821428571,6.482562396));
#157063=CARTESIAN_POINT('Ctrl Pts',(3.594771326,4.884501699,6.308085939));
#157064=CARTESIAN_POINT('Ctrl Pts',(3.922470298,4.948754474,6.097272075));
#157065=CARTESIAN_POINT('Ctrl Pts',(3.46875702882678,4.81811592995213,6.57252115311178));
#157066=CARTESIAN_POINT('Ctrl Pts',(3.47232386791339,4.81875342547607,6.57063373905589));
#157067=CARTESIAN_POINT('Ctrl Pts',(3.475890707,4.819390921,6.568746325));
#157068=CARTESIAN_POINT('Ctrl Pts',(3.48159224,4.820409947,6.565729325));
#157069=CARTESIAN_POINT('Ctrl Pts',(3.487288527,4.821428571,6.562702432));
#157070=CARTESIAN_POINT('Ctrl Pts',(3.840002137,4.884501699,6.37527749));
#157071=CARTESIAN_POINT('Ctrl Pts',(4.17059561,4.948754474,6.151128087));
#157072=CARTESIAN_POINT('Origin',(-0.122092848167099,5.08885500771978,-0.14691196824937));
#157073=CARTESIAN_POINT('Ctrl Pts',(2.4652460103968,4.95685568917762,6.81608654441024));
#157074=CARTESIAN_POINT('Ctrl Pts',(2.86014748013306,4.88876675850466,6.67325835902554));
#157075=CARTESIAN_POINT('Ctrl Pts',(3.23591210149,4.819390921,6.48578033413));
#157076=CARTESIAN_POINT('Ctrl Pts',(3.26062101125556,4.81482901918335,6.47345246360451));
#157077=CARTESIAN_POINT('Ctrl Pts',(3.28532992102107,4.81026711736656,6.46112459307846));
#157078=CARTESIAN_POINT('Ctrl Pts',(2.46416774756807,4.95685568917762,6.81838524258134));
#157079=CARTESIAN_POINT('Ctrl Pts',(2.85920239626229,4.88876675850466,6.67561952817654));
#157080=CARTESIAN_POINT('Ctrl Pts',(3.23510652,4.819390921,6.488188176));
#157081=CARTESIAN_POINT('Ctrl Pts',(3.25982460293285,4.81482901918335,6.47586337450206));
#157082=CARTESIAN_POINT('Ctrl Pts',(3.2845426858658,4.81026711736656,6.46353857300428));
#157083=CARTESIAN_POINT('Ctrl Pts',(2.35634146469517,4.95685568917762,7.04825505969156));
#157084=CARTESIAN_POINT('Ctrl Pts',(2.76469400918577,4.88876675850466,6.91173644327635));
#157085=CARTESIAN_POINT('Ctrl Pts',(3.154548371,4.819390921,6.728972363));
#157086=CARTESIAN_POINT('Ctrl Pts',(3.1801837706632,4.81482901918335,6.71695446426431));
#157087=CARTESIAN_POINT('Ctrl Pts',(3.20581917032638,4.81026711736656,6.7049365655283));
#157088=CARTESIAN_POINT('',(2.51558942704793,4.9479730999938,6.79958163914524));
#157089=CARTESIAN_POINT('Origin',(-0.103640466394893,4.69654717413986,-0.162200810867108));
#157090=CARTESIAN_POINT('Ctrl Pts',(2.53752478034511,4.93794661939396,6.85763024779903));
#157091=CARTESIAN_POINT('Ctrl Pts',(2.53022430469866,4.94124830104487,6.83826949569286));
#157092=CARTESIAN_POINT('Ctrl Pts',(2.52291239351571,4.9445899596398,6.81891982227765));
#157093=CARTESIAN_POINT('Ctrl Pts',(2.51559033183994,4.94797285549285,6.79958125379799));
#157094=CARTESIAN_POINT('Ctrl Pts',(1.75488918513372,4.81811592995213,7.03255995761173));
#157095=CARTESIAN_POINT('Ctrl Pts',(1.75870683623686,4.81875342547607,7.03160290467086));
#157096=CARTESIAN_POINT('Ctrl Pts',(1.76252448734,4.819390921,7.03064585173001));
#157097=CARTESIAN_POINT('Ctrl Pts',(1.76862693918,4.820409947,7.02911601851));
#157098=CARTESIAN_POINT('Ctrl Pts',(1.77472672631,4.821428571,7.02757559326));
#157099=CARTESIAN_POINT('Ctrl Pts',(2.15242502647,4.884501699,6.93219258975));
#157100=CARTESIAN_POINT('Ctrl Pts',(2.51772439171,4.948754474,6.79687704404));
#157101=CARTESIAN_POINT('Ctrl Pts',(1.75706614025099,4.81811592995213,7.03386668559916));
#157102=CARTESIAN_POINT('Ctrl Pts',(1.76088449962549,4.81875342547607,7.03290844979959));
#157103=CARTESIAN_POINT('Ctrl Pts',(1.764702859,4.819390921,7.031950214));
#157104=CARTESIAN_POINT('Ctrl Pts',(1.770806443,4.820409947,7.03041849));
#157105=CARTESIAN_POINT('Ctrl Pts',(1.776907359,4.821428571,7.028876172));
#157106=CARTESIAN_POINT('Ctrl Pts',(2.154675559,4.884501699,6.93337597));
#157107=CARTESIAN_POINT('Ctrl Pts',(2.52003186,4.948754474,6.79793640900001));
#157108=CARTESIAN_POINT('Ctrl Pts',(1.9747616519787,4.81811592995213,7.16453948434252));
#157109=CARTESIAN_POINT('Ctrl Pts',(1.97865083848935,4.81875342547607,7.16346296267127));
#157110=CARTESIAN_POINT('Ctrl Pts',(1.982540025,4.819390921,7.162386441));
#157111=CARTESIAN_POINT('Ctrl Pts',(1.988756825,4.820409947,7.160665639));
#157112=CARTESIAN_POINT('Ctrl Pts',(1.994970628,4.821428571,7.158934046));
#157113=CARTESIAN_POINT('Ctrl Pts',(2.379728812,4.884501699,7.051713995));
#157114=CARTESIAN_POINT('Ctrl Pts',(2.750778689,4.948754474,6.90387290500001));
#157115=CARTESIAN_POINT('Origin',(-0.0876565393637996,5.08885494092209,
-0.169723292818464));
#157116=CARTESIAN_POINT('Ctrl Pts',(0.9423528081216,4.95685568855937,7.18668524794689));
#157117=CARTESIAN_POINT('Ctrl Pts',(1.35872553599178,4.88876675818864,7.13208844931892));
#157118=CARTESIAN_POINT('Ctrl Pts',(1.76600722127,4.819390921,7.02977184234001));
#157119=CARTESIAN_POINT('Ctrl Pts',(1.79278857613182,4.81482901954031,7.02304387626926));
#157120=CARTESIAN_POINT('Ctrl Pts',(1.81956993099389,4.81026711808049,7.01631591019912));
#157121=CARTESIAN_POINT('Ctrl Pts',(0.940805602326207,4.95685568855937,
7.18869840920379));
#157122=CARTESIAN_POINT('Ctrl Pts',(1.35729496608203,4.88876675818864,7.13419125054935));
#157123=CARTESIAN_POINT('Ctrl Pts',(1.764702859,4.819390921,7.03195021400001));
#157124=CARTESIAN_POINT('Ctrl Pts',(1.79149251281487,4.81482901954031,7.02522721716447));
#157125=CARTESIAN_POINT('Ctrl Pts',(1.81828216663001,4.81026711808049,7.01850422032941));
#157126=CARTESIAN_POINT('Ctrl Pts',(0.786085022786937,4.95685568855937,
7.39001453489349));
#157127=CARTESIAN_POINT('Ctrl Pts',(1.21423797510712,4.88876675818864,7.34447137359237));
#157128=CARTESIAN_POINT('Ctrl Pts',(1.634266632,4.819390921,7.24978738));
#157129=CARTESIAN_POINT('Ctrl Pts',(1.66188618112043,4.81482901954031,7.24356130668562));
#157130=CARTESIAN_POINT('Ctrl Pts',(1.68950573024058,4.81026711808049,7.23733523337184));
#157131=CARTESIAN_POINT('',(0.995067285914387,4.94797309999901,7.18138856534732));
#157132=CARTESIAN_POINT('Origin',(-0.0663489787352659,4.69654714665182,
-0.180687961604724));
#157133=CARTESIAN_POINT('Ctrl Pts',(1.00401106893079,4.9379466193054,7.24279548235482));
#157134=CARTESIAN_POINT('Ctrl Pts',(1.00104326306824,4.94124830106007,7.22231798754459));
#157135=CARTESIAN_POINT('Ctrl Pts',(0.998061908143027,4.94458995965412,
7.20184885391167));
#157136=CARTESIAN_POINT('Ctrl Pts',(0.995068252627058,4.94797285554153,
7.18138838348548));
#157137=CARTESIAN_POINT('Ctrl Pts',(0.202068341494658,4.81811592995213,
7.24539191659084));
#157138=CARTESIAN_POINT('Ctrl Pts',(0.206002476142329,4.81875342547607,
7.24527792053542));
#157139=CARTESIAN_POINT('Ctrl Pts',(0.20993661079,4.819390921,7.24516392448001));
#157140=CARTESIAN_POINT('Ctrl Pts',(0.21622525964,4.820409947,7.24498170368));
#157141=CARTESIAN_POINT('Ctrl Pts',(0.22251358328,4.821428571,7.24478856649));
#157142=CARTESIAN_POINT('Ctrl Pts',(0.61188603345,4.884501699,7.23282953454999));
#157143=CARTESIAN_POINT('Ctrl Pts',(0.9977337452,4.948754474,7.17920615693));
#157144=CARTESIAN_POINT('Ctrl Pts',(0.203913492723773,4.81811592995213,
7.24713607501221));
#157145=CARTESIAN_POINT('Ctrl Pts',(0.207848573361887,4.81875342547607,
7.24702107600611));
#157146=CARTESIAN_POINT('Ctrl Pts',(0.211783654,4.819390921,7.246906077));
#157147=CARTESIAN_POINT('Ctrl Pts',(0.218073815,4.820409947,7.246722253));
#157148=CARTESIAN_POINT('Ctrl Pts',(0.224363648,4.821428571,7.24652751));
#157149=CARTESIAN_POINT('Ctrl Pts',(0.613829558,4.884501699,7.234469046));
#157150=CARTESIAN_POINT('Ctrl Pts',(0.999759534,4.948754474,7.180736792));
#157151=CARTESIAN_POINT('Ctrl Pts',(0.388428615635301,4.81811592995213,
7.42155191714905));
#157152=CARTESIAN_POINT('Ctrl Pts',(0.39245829531765,4.81875342547607,7.42133662307452));
#157153=CARTESIAN_POINT('Ctrl Pts',(0.396487975,4.819390921,7.421121329));
#157154=CARTESIAN_POINT('Ctrl Pts',(0.402929351,4.820409947,7.420777185));
#157155=CARTESIAN_POINT('Ctrl Pts',(0.40937012,4.821428571,7.420421861));
#157156=CARTESIAN_POINT('Ctrl Pts',(0.808182013,4.884501699,7.398420191));
#157157=CARTESIAN_POINT('Ctrl Pts',(1.202338414,4.948754474,7.333800299));
#157158=CARTESIAN_POINT('Origin',(-0.0491212403127217,5.08885412658079,
-0.18459499834712));
#157159=CARTESIAN_POINT('Ctrl Pts',(-0.576653346,4.948733649,7.227030574));
#157160=CARTESIAN_POINT('Ctrl Pts',(-0.182976184,4.884619049,7.258442542));
#157161=CARTESIAN_POINT('Ctrl Pts',(0.211783654,4.819390921,7.246906077));
#157162=CARTESIAN_POINT('Ctrl Pts',(0.215742295038516,4.81873681508671,
7.24679038963925));
#157163=CARTESIAN_POINT('Ctrl Pts',(0.219700936077032,4.81808270917342,
7.24667470227851));
#157164=CARTESIAN_POINT('Ctrl Pts',(-0.769900980000001,4.948733649,7.391718134));
#157165=CARTESIAN_POINT('Ctrl Pts',(-0.367252812,4.884619049,7.433656857));
#157166=CARTESIAN_POINT('Ctrl Pts',(0.037568402,4.819390921,7.431610398));
#157167=CARTESIAN_POINT('Ctrl Pts',(0.0416279382464466,4.81873681508671,
7.43158987616418));
#157168=CARTESIAN_POINT('Ctrl Pts',(0.0456874744928932,4.81808270917342,
7.43156935432838));
#157169=CARTESIAN_POINT('Origin',(-0.0259541685259539,4.69654854547677,
-0.190718431943377));
#157170=CARTESIAN_POINT('Ctrl Pts',(0.206665513,0.940053947,7.24705384000001));
#157171=CARTESIAN_POINT('Ctrl Pts',(0.604521557,1.005711878,7.235708109));
#157172=CARTESIAN_POINT('Ctrl Pts',(0.998744615,1.070155008,7.180878024));
#157173=CARTESIAN_POINT('Ctrl Pts',(0.459542598,0.940053947,7.485908135));
#157174=CARTESIAN_POINT('Ctrl Pts',(0.870511505,1.005711878,7.46067970300001));
#157175=CARTESIAN_POINT('Ctrl Pts',(1.276248909,1.070155008,7.390614908));
#157176=CARTESIAN_POINT('',(0.459542605383732,0.940053946884193,7.48590813582171));
#157177=CARTESIAN_POINT('',(1.0261937944465,1.03040248140644,7.42946339183112));
#157178=CARTESIAN_POINT('Origin',(0.0103931857568756,0.803673959797629,
-0.186267928095857));
#157179=CARTESIAN_POINT('Ctrl Pts',(0.994070540727961,1.06939092128209,
7.18152656204117));
#157180=CARTESIAN_POINT('Ctrl Pts',(0.999368724668876,1.06258635416255,
7.22279958838759));
#157181=CARTESIAN_POINT('Ctrl Pts',(1.0046992679533,1.05593965772069,7.26411847661544));
#157182=CARTESIAN_POINT('Ctrl Pts',(1.01540706332824,1.04295320028424,7.34675130349826));
#157183=CARTESIAN_POINT('Ctrl Pts',(1.02079005965345,1.03660648770934,7.38810953196721));
#157184=CARTESIAN_POINT('Ctrl Pts',(1.02619379318487,1.03040248141801,7.42946339193619));
#157185=CARTESIAN_POINT('',(0.333104057544598,0.940053946665902,7.36648098740755));
#157186=CARTESIAN_POINT('Origin',(1.29020058525775E-14,1.03148891300017,
-5.85469173142172E-14));
#157187=CARTESIAN_POINT('',(1.02255389523182,0.849330499810774,7.42996524430959));
#157188=CARTESIAN_POINT('Origin',(-0.0107703989177524,0.946426667970798,
-0.19229223055656));
#157189=CARTESIAN_POINT('',(1.58082723656417,0.940053948012009,7.33150634364829));
#157190=CARTESIAN_POINT('Origin',(-0.018799123902504,0.803583936067687,
-0.190543498808742));
#157191=CARTESIAN_POINT('Origin',(-0.0396491737200962,0.946429284259858,
-0.188708477980701));
#157192=CARTESIAN_POINT('Ctrl Pts',(0.989441248,1.070162746,7.182165831));
#157193=CARTESIAN_POINT('Ctrl Pts',(1.37862488,1.005280647,7.12855048));
#157194=CARTESIAN_POINT('Ctrl Pts',(1.759736143,0.940053947,7.033194773));
#157195=CARTESIAN_POINT('Ctrl Pts',(1.77283532249515,0.937812039362714,
7.02991730092518));
#157196=CARTESIAN_POINT('Ctrl Pts',(1.78593450199029,0.935570131725414,
7.02663982885036));
#157197=CARTESIAN_POINT('Ctrl Pts',(0.778916875456521,1.070162746,7.45996317561611));
#157198=CARTESIAN_POINT('Ctrl Pts',(1.1831536518329,1.005280647,7.41775561500099));
#157199=CARTESIAN_POINT('Ctrl Pts',(1.58046261703313,0.940053947,7.3321142923038));
#157200=CARTESIAN_POINT('Ctrl Pts',(1.59411852793229,0.937812039362713,
7.32917071344081));
#157201=CARTESIAN_POINT('Ctrl Pts',(1.60777443883138,0.935570131725414,
7.32622713457786));
#157202=CARTESIAN_POINT('',(1.67028170264392,0.940053949937996,7.18235055439685));
#157203=CARTESIAN_POINT('Ctrl Pts',(1.759736143,0.940053947,7.03319477300001));
#157204=CARTESIAN_POINT('Ctrl Pts',(2.145851537,1.005711878,6.936587009));
#157205=CARTESIAN_POINT('Ctrl Pts',(2.519071031,1.070155008,6.798292516));
#157206=CARTESIAN_POINT('Ctrl Pts',(2.058047714,0.940053947,7.212103688));
#157207=CARTESIAN_POINT('Ctrl Pts',(2.45398503,1.005711878,7.099118916));
#157208=CARTESIAN_POINT('Ctrl Pts',(2.835174659,1.070155008,6.943470649));
#157209=CARTESIAN_POINT('',(2.05804772140884,0.940053946884192,7.21210368721667));
#157210=CARTESIAN_POINT('',(2.59931696986772,1.03040248142397,7.03516533471204));
#157211=CARTESIAN_POINT('Origin',(-0.0298918993812045,0.803673986466962,
-0.184147321042287));
#157212=CARTESIAN_POINT('Ctrl Pts',(2.51464564999319,1.06939092119121,6.79993067959644));
#157213=CARTESIAN_POINT('Ctrl Pts',(2.52869245150643,1.06258635149592,6.83909982773586));
#157214=CARTESIAN_POINT('Ctrl Pts',(2.54278071547496,1.05593965239104,6.87830681115066));
#157215=CARTESIAN_POINT('Ctrl Pts',(2.57100176913631,1.0429532017803,6.95670582817617));
#157216=CARTESIAN_POINT('Ctrl Pts',(2.58514970700579,1.03660649073983,6.99593992918472));
#157217=CARTESIAN_POINT('Ctrl Pts',(2.59931696867331,1.03040248144127,7.03516533503894));
#157218=CARTESIAN_POINT('',(1.90889193047692,0.940053946665902,7.12264922997018));
#157219=CARTESIAN_POINT('Origin',(-6.26452015262124E-13,1.03148891300033,
-1.8253627775966E-12));
#157220=CARTESIAN_POINT('',(2.59587005224225,0.849330499783684,7.03643792502342));
#157221=CARTESIAN_POINT('Origin',(-0.0518557823053684,0.946426648330426,
-0.18548135075145));
#157222=CARTESIAN_POINT('',(3.11992552026395,0.940053948012017,6.82026867260148));
#157223=CARTESIAN_POINT('Origin',(-0.0593208284644847,0.803583927461065,
-0.182047421518711));
#157224=CARTESIAN_POINT('Origin',(-0.0792889380638379,0.946429283724577,
-0.175773157664761));
#157225=CARTESIAN_POINT('Ctrl Pts',(2.510262011,1.070162746,6.80155016400001));
#157226=CARTESIAN_POINT('Ctrl Pts',(2.878821031,1.005280647,6.665525334));
#157227=CARTESIAN_POINT('Ctrl Pts',(3.230523466,0.940053947,6.490471334));
#157228=CARTESIAN_POINT('Ctrl Pts',(3.24261183409407,0.937812039407971,
6.48445455112403));
#157229=CARTESIAN_POINT('Ctrl Pts',(3.2547002021882,0.935570131815929,6.47843776824816));
#157230=CARTESIAN_POINT('Ctrl Pts',(2.36437779987387,1.070162746,7.11810927904205));
#157231=CARTESIAN_POINT('Ctrl Pts',(2.75009036708949,1.005280647,6.98998954958823));
#157232=CARTESIAN_POINT('Ctrl Pts',(3.11970011633105,0.940053947,6.82094079016248));
#157233=CARTESIAN_POINT('Ctrl Pts',(3.13240397691135,0.937812039407971,
6.81513041347349));
#157234=CARTESIAN_POINT('Ctrl Pts',(3.14510783749165,0.935570131815929,
6.80932003678452));
#157235=CARTESIAN_POINT('',(3.17522450484935,0.940053949937996,6.65536999669985));
#157236=CARTESIAN_POINT('Ctrl Pts',(3.230523466,0.940053947,6.49047133400001));
#157237=CARTESIAN_POINT('Ctrl Pts',(3.586843883,1.005711878,6.31311881000001));
#157238=CARTESIAN_POINT('Ctrl Pts',(3.921608485,1.070155008,6.097826407));
#157239=CARTESIAN_POINT('Ctrl Pts',(3.560320807,0.940053947,6.601069288));
#157240=CARTESIAN_POINT('Ctrl Pts',(3.922712942,1.005711878,6.405611219));
#157241=CARTESIAN_POINT('Ctrl Pts',(4.261530793,1.070155008,6.171657419));
#157242=CARTESIAN_POINT('',(3.56032081408952,0.940053946884188,6.60106928563899));
#157243=CARTESIAN_POINT('',(4.05089897255837,1.03040248143616,6.31191076539481));
#157244=CARTESIAN_POINT('Origin',(-0.0687791674829624,0.80367396202427,
-0.173416020060584));
#157245=CARTESIAN_POINT('Ctrl Pts',(3.9176387235532,1.06939092116972,6.10037759740578));
#157246=CARTESIAN_POINT('Ctrl Pts',(3.93977731881556,1.06258635418866,6.13561133127413));
#157247=CARTESIAN_POINT('Ctrl Pts',(3.96196453935034,1.0559396579215,6.17087310068767));
#157248=CARTESIAN_POINT('Ctrl Pts',(4.00637928790532,1.04295320259416,6.24137252538175));
#157249=CARTESIAN_POINT('Ctrl Pts',(4.02863062364503,1.03660649242267,6.2766479612956));
#157250=CARTESIAN_POINT('Ctrl Pts',(4.05089897146474,1.03040248145668,6.31191076594333));
#157251=CARTESIAN_POINT('',(3.39542213831681,0.940053946665902,6.54577031005759));
#157252=CARTESIAN_POINT('Origin',(-3.6949610038306E-13,1.03148891300017,
-5.41667405373758E-13));
#157253=CARTESIAN_POINT('',(4.04780621136812,0.849330499792421,6.31389458847702));
#157254=CARTESIAN_POINT('Origin',(-0.0905162729480125,0.946426679995198,
-0.169997196421141));
#157255=CARTESIAN_POINT('',(4.51313955453792,0.940053948012019,5.99012281865662));
#157256=CARTESIAN_POINT('Origin',(-0.0970687103584039,0.803583922662045,
-0.165038982853876));
#157257=CARTESIAN_POINT('Origin',(-0.1152210911026,0.946429287942322,-0.154618692676783));
#157258=CARTESIAN_POINT('Ctrl Pts',(3.913705713,1.070162746,6.102901571));
#157259=CARTESIAN_POINT('Ctrl Pts',(4.24440671,1.005280647,5.890827631));
#157260=CARTESIAN_POINT('Ctrl Pts',(4.550255102,0.940053947,5.644260669));
#157261=CARTESIAN_POINT('Ctrl Pts',(4.56076742050196,0.937812039364825,
5.63578591319158));
#157262=CARTESIAN_POINT('Ctrl Pts',(4.5712797390039,0.935570131729636,5.62731115738306));
#157263=CARTESIAN_POINT('Ctrl Pts',(3.83928304573905,1.070162746,6.44342050299382));
#157264=CARTESIAN_POINT('Ctrl Pts',(4.18843591351092,1.005280647,6.23537934193769));
#157265=CARTESIAN_POINT('Ctrl Pts',(4.51306390582548,0.940053947,5.99082767768925));
#157266=CARTESIAN_POINT('Ctrl Pts',(4.52422169817986,0.937812039364825,
5.98242218970237));
#157267=CARTESIAN_POINT('Ctrl Pts',(4.53537949053428,0.935570131729636,
5.97401670171551));
#157268=CARTESIAN_POINT('',(4.53169733829032,0.940053949937996,5.81719173486759));
#157269=CARTESIAN_POINT('Ctrl Pts',(4.550255102,0.940053947,5.644260669));
#157270=CARTESIAN_POINT('Ctrl Pts',(4.860119396,1.005711878,5.394456192));
#157271=CARTESIAN_POINT('Ctrl Pts',(5.14077588500001,1.070155008,5.112232712));
#157272=CARTESIAN_POINT('Ctrl Pts',(4.896117256,0.940053947,5.681376225));
#157273=CARTESIAN_POINT('Ctrl Pts',(5.208019157,1.005711878,5.41258426));
#157274=CARTESIAN_POINT('Ctrl Pts',(5.488622484,1.070155008,5.11126434800001));
#157275=CARTESIAN_POINT('',(4.89611726241347,0.94005394688418,5.68137622117121));
#157276=CARTESIAN_POINT('',(5.31306544163784,1.03040248139847,5.29351826402951));
#157277=CARTESIAN_POINT('Origin',(-0.104450594516354,0.803673959972207,
-0.154576303251013));
#157278=CARTESIAN_POINT('Ctrl Pts',(5.13744736507667,1.0693909212065,5.11557763819519));
#157279=CARTESIAN_POINT('Ctrl Pts',(5.16664259530524,1.06258635144726,5.14522849550555));
#157280=CARTESIAN_POINT('Ctrl Pts',(5.19589134248179,1.05593965230488,5.17489628147042));
#157281=CARTESIAN_POINT('Ctrl Pts',(5.25442297546138,1.04295320044881,5.23419959482863));
#157282=CARTESIAN_POINT('Ctrl Pts',(5.2837372741119,1.03660648808713,5.26386694208382));
#157283=CARTESIAN_POINT('Ctrl Pts',(5.31306544069633,1.03040248141083,5.2935182648699));
#157284=CARTESIAN_POINT('',(4.72318618057174,0.940053946665902,5.66281844568906));
#157285=CARTESIAN_POINT('Origin',(-1.31101726696947E-12,1.03148891300044,
-1.34310965127504E-12));
#157286=CARTESIAN_POINT('',(5.31047145089205,0.849330499771562,5.29612055861479));
#157287=CARTESIAN_POINT('Origin',(-0.124944554379689,0.946426703525078,
-0.14656457946748));
#157288=CARTESIAN_POINT('',(5.69532420086373,0.940053948010709,4.87988547605802));
#157289=CARTESIAN_POINT('Origin',(-0.130277934429539,0.803583951405237,
-0.140313671440268));
#157290=CARTESIAN_POINT('Origin',(-0.14576573591514,0.946429263697512,-0.12623466299575));
#157291=CARTESIAN_POINT('Ctrl Pts',(5.13414888600001,1.070162746,5.118888084));
#157292=CARTESIAN_POINT('Ctrl Pts',(5.411528649,1.005280647,4.840681376));
#157293=CARTESIAN_POINT('Ctrl Pts',(5.657221867,0.940053947,4.534130649));
#157294=CARTESIAN_POINT('Ctrl Pts',(5.66566659185461,0.937812039229164,
4.52359418989632));
#157295=CARTESIAN_POINT('Ctrl Pts',(5.6741113167094,0.935570131458313,4.51305773079268));
#157296=CARTESIAN_POINT('Ctrl Pts',(5.13466768313965,1.070162746,5.46744454586968));
#157297=CARTESIAN_POINT('Ctrl Pts',(5.4309348517102,1.005280647,5.1892097256946));
#157298=CARTESIAN_POINT('Ctrl Pts',(5.69540184317356,0.940053947,4.88059012097109));
#157299=CARTESIAN_POINT('Ctrl Pts',(5.70449184164491,0.937812039229164,
4.86998255244376));
#157300=CARTESIAN_POINT('Ctrl Pts',(5.71358184011627,0.935570131458314,
4.85937498391645));
#157301=CARTESIAN_POINT('',(5.67627304106311,0.940053949938004,4.70700805305583));
#157302=CARTESIAN_POINT('Ctrl Pts',(5.657221867,0.940053947,4.534130649));
#157303=CARTESIAN_POINT('Ctrl Pts',(5.906141128,1.005711878,4.223554798));
#157304=CARTESIAN_POINT('Ctrl Pts',(6.119566318,1.070155008,3.887596697));
#157305=CARTESIAN_POINT('Ctrl Pts',(6.002976704,0.940053947,4.496028325));
#157306=CARTESIAN_POINT('Ctrl Pts',(6.249804185,1.005711878,4.166470877));
#157307=CARTESIAN_POINT('Ctrl Pts',(6.459072287,1.070155008,3.811874236));
#157308=CARTESIAN_POINT('',(6.00297670939691,0.9400539468842,4.49602831991059));
#157309=CARTESIAN_POINT('',(6.3267988756447,1.03040248135818,4.02760673190842));
#157310=CARTESIAN_POINT('Origin',(-0.135237854469713,0.803673991008168,
-0.128508530935612));
#157311=CARTESIAN_POINT('Ctrl Pts',(6.11703467735814,1.06939092122838,3.89157895396036));
#157312=CARTESIAN_POINT('Ctrl Pts',(6.15192139724256,1.06258635146732,3.91426047917283));
#157313=CARTESIAN_POINT('Ctrl Pts',(6.18686402201107,1.05593965231519,3.9369470327545));
#157314=CARTESIAN_POINT('Ctrl Pts',(6.25677568131884,1.04295319969706,3.98228129938604));
#157315=CARTESIAN_POINT('Ctrl Pts',(6.29178223507313,1.03660648657069,4.00495333581444));
#157316=CARTESIAN_POINT('Ctrl Pts',(6.3267988749145,1.03040248136766,4.02760673295417));
#157317=CARTESIAN_POINT('',(5.83009928675315,0.940053946665909,4.51507948538187));
#157318=CARTESIAN_POINT('Origin',(4.10695782937509E-13,1.03148891299983,
2.1467203015213E-13));
#157319=CARTESIAN_POINT('',(6.32482494729382,0.849330499764723,4.03070581740142));
#157320=CARTESIAN_POINT('Origin',(-0.153530836941408,0.946426677340838,
-0.116278825077462));
#157321=CARTESIAN_POINT('',(6.61120181473465,0.940053948010707,3.54147011535873));
#157322=CARTESIAN_POINT('Origin',(-0.157395227955885,0.803583957882191,
-0.109027212856986));
#157323=CARTESIAN_POINT('Origin',(-0.169494640360354,0.946429293361835,
-0.0919481097987146));
#157324=CARTESIAN_POINT('Ctrl Pts',(6.114524963,1.070162746,3.895521079));
#157325=CARTESIAN_POINT('Ctrl Pts',(6.32561352300001,1.005280647,3.564190239));
#157326=CARTESIAN_POINT('Ctrl Pts',(6.499663225,0.940053947,3.211989719));
#157327=CARTESIAN_POINT('Ctrl Pts',(6.50564548947943,0.937812039280326,
3.19988423053191));
#157328=CARTESIAN_POINT('Ctrl Pts',(6.51162775395894,0.93557013156064,3.18777874206383));
#157329=CARTESIAN_POINT('Ctrl Pts',(6.1899609672,1.070162746,4.2358169583214));
#157330=CARTESIAN_POINT('Ctrl Pts',(6.41948931138866,1.005280647,3.90039843070349));
#157331=CARTESIAN_POINT('Ctrl Pts',(6.61142911963172,0.940053947,3.54214159525235));
#157332=CARTESIAN_POINT('Ctrl Pts',(6.6180262851761,0.937812039280326,3.52982794509029));
#157333=CARTESIAN_POINT('Ctrl Pts',(6.62462345072036,0.93557013156064,3.5175142949283));
#157334=CARTESIAN_POINT('',(6.55543252479518,0.940053949938004,3.37672990639611));
#157335=CARTESIAN_POINT('Ctrl Pts',(6.499663225,0.940053947,3.211989719));
#157336=CARTESIAN_POINT('Ctrl Pts',(6.675998265,1.005711878,2.855164676));
#157337=CARTESIAN_POINT('Ctrl Pts',(6.812212632,1.070155008,2.481180981));
#157338=CARTESIAN_POINT('Ctrl Pts',(6.829143632,0.940053947,3.100451136));
#157339=CARTESIAN_POINT('Ctrl Pts',(6.999355314,1.005711878,2.725537947));
#157340=CARTESIAN_POINT('Ctrl Pts',(7.127503049,1.070155008,2.334245122));
#157341=CARTESIAN_POINT('',(6.82914363621652,0.940053946884184,3.10045112982859));
#157342=CARTESIAN_POINT('',(7.04469822610831,1.03040248142797,2.5733687845793));
#157343=CARTESIAN_POINT('Origin',(-0.159701616024189,0.803673941611579,
-0.0964319565452881));
#157344=CARTESIAN_POINT('Ctrl Pts',(6.81059624699143,1.06939092111156,2.48561436359438));
#157345=CARTESIAN_POINT('Ctrl Pts',(6.84954319235847,1.06258635136358,2.5002659938163));
#157346=CARTESIAN_POINT('Ctrl Pts',(6.88854581641247,1.05593965223858,2.51491051690288));
#157347=CARTESIAN_POINT('Ctrl Pts',(6.96656848502177,1.04295320336159,2.54415594493735));
#157348=CARTESIAN_POINT('Ctrl Pts',(7.00563039808937,1.03660649398555,2.55877253825662));
#157349=CARTESIAN_POINT('Ctrl Pts',(7.04469822533426,1.03040248145228,2.57336878626287));
#157350=CARTESIAN_POINT('',(6.664403429376,0.940053946665909,3.15622042565031));
#157351=CARTESIAN_POINT('Origin',(1.58206781009085E-12,1.03148891299961,
5.70507183161872E-13));
#157352=CARTESIAN_POINT('',(7.04343665848193,0.849330499775803,2.57681975219681));
#157353=CARTESIAN_POINT('Origin',(-0.174937395364666,0.946426703968627,
-0.080555512952542));
#157354=CARTESIAN_POINT('',(7.217946980252,0.940053948011585,2.0374595491609));
#157355=CARTESIAN_POINT('Origin',(-0.177153273325414,0.803583973570313,
-0.0726429733030526));
#157356=CARTESIAN_POINT('Origin',(-0.185298049236705,0.946429317162114,
-0.0533620738118479));
#157357=CARTESIAN_POINT('Ctrl Pts',(6.80899264800001,1.070162746,2.490003838));
#157358=CARTESIAN_POINT('Ctrl Pts',(6.943919739,1.005280647,2.121041529));
#157359=CARTESIAN_POINT('Ctrl Pts',(7.038187555,0.940053947,1.73965972));
#157360=CARTESIAN_POINT('Ctrl Pts',(7.04142763503705,0.937812039448509,
1.7265512420669));
#157361=CARTESIAN_POINT('Ctrl Pts',(7.0446677150741,0.935570131897005,1.7134427641338));
#157362=CARTESIAN_POINT('Ctrl Pts',(6.95581855636277,1.070162746,2.80612727794603));
#157363=CARTESIAN_POINT('Ctrl Pts',(7.10787558656333,1.005280647,2.42920883961683));
#157364=CARTESIAN_POINT('Ctrl Pts',(7.21831331925159,0.940053947,2.03806646438908));
#157365=CARTESIAN_POINT('Ctrl Pts',(7.22210917565524,0.937812039448509,
2.02462250593755));
#157366=CARTESIAN_POINT('Ctrl Pts',(7.22590503205889,0.935570131897005,
2.01117854748595));
#157367=CARTESIAN_POINT('',(7.12806727013939,0.940053949938004,1.88855962198939));
#157368=CARTESIAN_POINT('Ctrl Pts',(7.038187555,0.940053947,1.73965972));
#157369=CARTESIAN_POINT('Ctrl Pts',(7.133693143,1.005711878,1.353270226));
#157370=CARTESIAN_POINT('Ctrl Pts',(7.186327454,1.070155008,0.958748));
#157371=CARTESIAN_POINT('Ctrl Pts',(7.335987395,0.940053947,1.559900299));
#157372=CARTESIAN_POINT('Ctrl Pts',(7.421624369,1.005711878,1.157161891));
#157373=CARTESIAN_POINT('Ctrl Pts',(7.46265969,1.070155008,0.7474693));
#157374=CARTESIAN_POINT('',(7.33598739777246,0.940053946884192,1.55990029209667));
#157375=CARTESIAN_POINT('',(7.43319531680987,1.03040248137726,0.998802974411074));
#157376=CARTESIAN_POINT('Origin',(-0.176697923435072,0.803673966896485,
-0.0598462981616252));
#157377=CARTESIAN_POINT('Ctrl Pts',(7.18570190537006,1.06939092111547,0.963425207554627));
#157378=CARTESIAN_POINT('Ctrl Pts',(7.22688794226064,1.06258635431296,0.969361846302531));
#157379=CARTESIAN_POINT('Ctrl Pts',(7.26812682594864,1.05593965822805,0.975279574506992));
#157380=CARTESIAN_POINT('Ctrl Pts',(7.35061233071141,1.04295319985269,0.987068702007152));
#157381=CARTESIAN_POINT('Ctrl Pts',(7.39190315818797,1.03660648691664,0.992946414394434));
#157382=CARTESIAN_POINT('Ctrl Pts',(7.43319531658188,1.03040248138745,0.99880297566297));
#157383=CARTESIAN_POINT('',(7.1870874754579,0.940053946665909,1.64978000750524));
#157384=CARTESIAN_POINT('Origin',(2.90566182226115E-13,1.03148891300033,
-6.53773910008759E-14));
#157385=CARTESIAN_POINT('',(7.43270510019514,0.849330500339288,1.00244445928462));
#157386=CARTESIAN_POINT('Origin',(-0.188164822754386,0.946426684333019,
-0.0410658480806596));
#157387=CARTESIAN_POINT('',(7.48718896703835,0.940053948011584,0.438179637481235));
#157388=CARTESIAN_POINT('Origin',(-0.188627616963447,0.803583944653875,
-0.0328619031245316));
#157389=CARTESIAN_POINT('Origin',(-0.192437196061649,0.946429297142976,
-0.0122808963513313));
#157390=CARTESIAN_POINT('Ctrl Pts',(7.185079405,1.070162746,0.968056785));
#157391=CARTESIAN_POINT('Ctrl Pts',(7.23753598500001,1.005280647,0.578715273));
#157392=CARTESIAN_POINT('Ctrl Pts',(7.247614057,0.940053947,0.185985165));
#157393=CARTESIAN_POINT('Ctrl Pts',(7.24796045053153,0.937812039325257,
0.17248663382751));
#157394=CARTESIAN_POINT('Ctrl Pts',(7.24830684406306,0.935570131650501,
0.158988102655022));
#157395=CARTESIAN_POINT('Ctrl Pts',(7.39642979953016,1.070162746,1.24522620453934));
#157396=CARTESIAN_POINT('Ctrl Pts',(7.46390549870593,1.005280647,0.844432143122291));
#157397=CARTESIAN_POINT('Ctrl Pts',(7.48767721009522,0.940053947,0.438693611337785));
#157398=CARTESIAN_POINT('Ctrl Pts',(7.48849426786764,0.937812039325257,
0.424747967478025));
#157399=CARTESIAN_POINT('Ctrl Pts',(7.48931132564014,0.935570131650498,
0.41080232361826));
#157400=CARTESIAN_POINT('',(7.36740151176666,0.940053949938004,0.312082388401445));
#157401=CARTESIAN_POINT('Ctrl Pts',(7.24761405700001,0.940053947,0.185985165));
#157402=CARTESIAN_POINT('Ctrl Pts',(7.257824457,1.005711878,-0.211901635));
#157403=CARTESIAN_POINT('Ctrl Pts',(7.224417591,1.070155008,-0.608514971));
#157404=CARTESIAN_POINT('Ctrl Pts',(7.49980854000001,0.940053947,-0.053589743));
#157405=CARTESIAN_POINT('Ctrl Pts',(7.496866517,1.005711878,-0.465321769));
#157406=CARTESIAN_POINT('Ctrl Pts',(7.448870658,1.070155008,-0.874257356));
#157407=CARTESIAN_POINT('',(7.49980854123035,0.940053946884195,-0.05358975035691));
#157408=CARTESIAN_POINT('',(7.47412445611645,1.03040248135761,-0.62246575367252));
#157409=CARTESIAN_POINT('Origin',(-0.185431817958654,0.803673979949119,
-0.0204623074656415));
#157410=CARTESIAN_POINT('Ctrl Pts',(7.22481212868082,1.06939092120208,-0.603812640052707));
#157411=CARTESIAN_POINT('Ctrl Pts',(7.26631147867449,1.06258635144333,-0.606868578566119));
#157412=CARTESIAN_POINT('Ctrl Pts',(7.30785837722625,1.05593965229337,-0.609954346170825));
#157413=CARTESIAN_POINT('Ctrl Pts',(7.39094942006576,1.04295324244345,-0.616172764027325));
#157414=CARTESIAN_POINT('Ctrl Pts',(7.43253811868122,1.03660657331793,-0.619308753071964));
#157415=CARTESIAN_POINT('Ctrl Pts',(7.47412445621601,1.03040248136036,-0.62246575236655));
#157416=CARTESIAN_POINT('',(7.37371129851838,0.940053946665909,0.0661977089534413));
#157417=CARTESIAN_POINT('Origin',(-1.32099192695634E-12,1.03148891300011,
1.23267010748024E-13));
#157418=CARTESIAN_POINT('',(7.47442851198712,0.849330499786397,-0.618804022598348));
#157419=CARTESIAN_POINT('Origin',(-0.192593390699098,0.946426691613029,
0.000344107344360314));
#157420=CARTESIAN_POINT('',(7.40633831793416,0.940053948010714,-1.18158906852439));
#157421=CARTESIAN_POINT('Origin',(-0.191281893020457,0.803583929448492,
0.00845574576009325));
#157422=CARTESIAN_POINT('Origin',(-0.190578083564067,0.946429301495116,
0.02937453071876));
#157423=CARTESIAN_POINT('Ctrl Pts',(7.225199835,1.070162746,-0.599155527));
#157424=CARTESIAN_POINT('Ctrl Pts',(7.192733093,1.005280647,-0.990671065));
#157425=CARTESIAN_POINT('Ctrl Pts',(7.118150181,0.940053947,-1.376385849));
#157426=CARTESIAN_POINT('Ctrl Pts',(7.11558669079624,0.937812039276247,
-1.38964325667839));
#157427=CARTESIAN_POINT('Ctrl Pts',(7.11302320059262,0.935570131552479,
-1.40290066435676));
#157428=CARTESIAN_POINT('Ctrl Pts',(7.49119220641564,1.070162746,-0.373900262498168));
#157429=CARTESIAN_POINT('Ctrl Pts',(7.47093148525627,1.005280647,-0.779829261873931));
#157430=CARTESIAN_POINT('Ctrl Pts',(7.40692563609068,0.940053947,-1.18119206712137));
#157431=CARTESIAN_POINT('Ctrl Pts',(7.40472569024625,0.937812039276248,
-1.19498731313431));
#157432=CARTESIAN_POINT('Ctrl Pts',(7.40252574440196,0.935570131552477,
-1.20878255914725));
#157433=CARTESIAN_POINT('',(7.26224424685807,0.940053949938004,-1.27898747034023));
#157434=CARTESIAN_POINT('Ctrl Pts',(7.118150181,0.940053947,-1.376385849));
#157435=CARTESIAN_POINT('Ctrl Pts',(7.042587967,1.005711878,-1.767165211));
#157436=CARTESIAN_POINT('Ctrl Pts',(6.924701991,1.070155008,-2.147324459));
#157437=CARTESIAN_POINT('Ctrl Pts',(7.312946974,0.940053947,-1.664573988));
#157438=CARTESIAN_POINT('Ctrl Pts',(7.221563518,1.005711878,-2.0660475));
#157439=CARTESIAN_POINT('Ctrl Pts',(7.086780713,1.070155008,-2.455104709));
#157440=CARTESIAN_POINT('',(7.31294697361584,0.940053946884197,-1.66457399541545));
#157441=CARTESIAN_POINT('',(7.16557184278519,1.03040248136924,-2.21462867485676));
#157442=CARTESIAN_POINT('Origin',(-0.185495574279347,0.803673981046612,
0.0198785268233517));
#157443=CARTESIAN_POINT('Ctrl Pts',(6.92609816677978,1.06939092119062,-2.14281687978802));
#157444=CARTESIAN_POINT('Ctrl Pts',(6.96597033263714,1.06258635417184,-2.15472250079013));
#157445=CARTESIAN_POINT('Ctrl Pts',(7.00588252084771,1.05593965785563,-2.16666747443939));
#157446=CARTESIAN_POINT('Ctrl Pts',(7.08569446013349,1.04295320004583,-2.19060271567495));
#157447=CARTESIAN_POINT('Ctrl Pts',(7.12563698639577,1.03660648728853,-2.20260581656275));
#157448=CARTESIAN_POINT('Ctrl Pts',(7.16557184309803,1.03040248138017,-2.21462867362724));
#157449=CARTESIAN_POINT('',(7.215548577078,0.940053946665909,-1.52047992050266));
#157450=CARTESIAN_POINT('Origin',(-6.3274038786254E-13,1.03148891299978,
1.57968256531138E-13));
#157451=CARTESIAN_POINT('',(7.16665595397576,0.849330499759727,-2.21111791586516));
#157452=CARTESIAN_POINT('Origin',(-0.188016845225611,0.946426674270018,
0.0417380006194687));
#157453=CARTESIAN_POINT('',(6.9791755234254,0.940053948011584,-2.74610798041312));
#157454=CARTESIAN_POINT('Origin',(-0.18499204033991,0.803583928938046,0.0493779806989719));
#157455=CARTESIAN_POINT('Origin',(-0.179807836070603,0.946429282548676,
0.0696564257744658));
#157456=CARTESIAN_POINT('Ctrl Pts',(6.92747795,1.070162746,-2.138351993));
#157457=CARTESIAN_POINT('Ctrl Pts',(6.811605995,1.005280647,-2.513734725));
#157458=CARTESIAN_POINT('Ctrl Pts',(6.655849513,0.940053947,-2.874398591));
#157459=CARTESIAN_POINT('Ctrl Pts',(6.6504960051112,0.937812039321254,-2.88679497301278));
#157460=CARTESIAN_POINT('Ctrl Pts',(6.64514249722251,0.935570131642496,
-2.8991913550255));
#157461=CARTESIAN_POINT('Ctrl Pts',(7.23567479171325,1.070162746,-1.97554356806818));
#157462=CARTESIAN_POINT('Ctrl Pts',(7.12862501943956,1.005280647,-2.36762671770142));
#157463=CARTESIAN_POINT('Ctrl Pts',(6.97983445285341,0.940053947,-2.74584651830165));
#157464=CARTESIAN_POINT('Ctrl Pts',(6.97472037052588,0.937812039321253,
-2.75884631555064));
#157465=CARTESIAN_POINT('Ctrl Pts',(6.9696062881982,0.935570131642497,-2.77184611279955));
#157466=CARTESIAN_POINT('',(6.81751251259641,0.940053949938004,-2.81025329724772));
#157467=CARTESIAN_POINT('Ctrl Pts',(6.655849513,0.940053947,-2.874398591));
#157468=CARTESIAN_POINT('Ctrl Pts',(6.49804789100001,1.005711878,-3.239798106));
#157469=CARTESIAN_POINT('Ctrl Pts',(6.301195022,1.070155008,-3.585727442));
#157470=CARTESIAN_POINT('Ctrl Pts',(6.784140134,0.940053947,-3.197724603));
#157471=CARTESIAN_POINT('Ctrl Pts',(6.608588236,1.005711878,-3.570167146));
#157472=CARTESIAN_POINT('Ctrl Pts',(6.393320778,1.070155008,-3.921154095));
#157473=CARTESIAN_POINT('',(6.78414013202652,0.940053946884191,-3.19772461020444));
#157474=CARTESIAN_POINT('',(6.52196505392216,1.03040248138268,-3.70323802043655));
#157475=CARTESIAN_POINT('Origin',(-0.176885230900306,0.803673982213261,
0.0592896936848697));
#157476=CARTESIAN_POINT('Ctrl Pts',(6.30352755236845,1.06939092115757,-3.58162538384938));
#157477=CARTESIAN_POINT('Ctrl Pts',(6.33990818722998,1.06258635142359,-3.60182400325982));
#157478=CARTESIAN_POINT('Ctrl Pts',(6.37631945100853,1.05593965229467,-3.62206965996145));
#157479=CARTESIAN_POINT('Ctrl Pts',(6.44911979335023,1.04295324246494,-3.66260236648865));
#157480=CARTESIAN_POINT('Ctrl Pts',(6.485547906345,1.03660657334913,-3.68291115436475));
#157481=CARTESIAN_POINT('Ctrl Pts',(6.52196505456613,1.03040248138544,-3.70323801928368));
#157482=CARTESIAN_POINT('',(6.71999482265735,0.940053946665909,-3.03606159886512));
#157483=CARTESIAN_POINT('Origin',(-1.33400235302616E-12,1.03148891300006,
7.94937032866372E-13));
#157484=CARTESIAN_POINT('',(6.5237785286103,0.849330499784263,-3.70004239307047));
#157485=CARTESIAN_POINT('Origin',(-0.174648438018141,0.946426696792022,
0.0811801132268097));
#157486=CARTESIAN_POINT('',(6.22567423713443,0.940053948012022,-4.18222193475387));
#157487=CARTESIAN_POINT('Origin',(-0.170052142850048,0.803583965490886,
0.0879913438511026));
#157488=CARTESIAN_POINT('Origin',(-0.160630037195878,0.946429248627739,
0.106681332694981));
#157489=CARTESIAN_POINT('Ctrl Pts',(6.305834896,1.070162746,-3.577561496));
#157490=CARTESIAN_POINT('Ctrl Pts',(6.111975772,1.005280647,-3.919258944));
#157491=CARTESIAN_POINT('Ctrl Pts',(5.88232872,0.940053947,-4.238007649));
#157492=CARTESIAN_POINT('Ctrl Pts',(5.87443551850391,0.937812039335438,
-4.24896336444796));
#157493=CARTESIAN_POINT('Ctrl Pts',(5.86654231700796,0.935570131670863,
-4.25991907989585));
#157494=CARTESIAN_POINT('Ctrl Pts',(6.64182526572518,1.070162746,-3.4848126526049));
#157495=CARTESIAN_POINT('Ctrl Pts',(6.4529919693508,1.005280647,-3.84471657929409));
#157496=CARTESIAN_POINT('Ctrl Pts',(6.22637396689046,0.940053947,-4.18210823669196));
#157497=CARTESIAN_POINT('Ctrl Pts',(6.21858487689136,0.937812039335437,
-4.19370472927367));
#157498=CARTESIAN_POINT('Ctrl Pts',(6.21079578689226,0.935570131670863,
-4.20530122185541));
#157499=CARTESIAN_POINT('',(6.05400147015755,0.940053949938004,-4.21011480237209));
#157500=CARTESIAN_POINT('Ctrl Pts',(5.88232872,0.940053947,-4.238007649));
#157501=CARTESIAN_POINT('Ctrl Pts',(5.649666317,1.005711878,-4.560941642));
#157502=CARTESIAN_POINT('Ctrl Pts',(5.383051178,1.070155008,-4.856465795));
#157503=CARTESIAN_POINT('Ctrl Pts',(5.938114442,0.940053947,-4.58135317));
#157504=CARTESIAN_POINT('Ctrl Pts',(5.686602712,1.005711878,-4.907349744));
#157505=CARTESIAN_POINT('Ctrl Pts',(5.400916269,1.070155008,-5.203854673));
#157506=CARTESIAN_POINT('',(5.93811443852413,0.940053946884183,-4.58135317661113));
#157507=CARTESIAN_POINT('',(5.57339842761695,1.03040248139026,-5.01868807215372));
#157508=CARTESIAN_POINT('Origin',(-0.160004360491645,0.80367397061341,0.095928749465683));
#157509=CARTESIAN_POINT('Ctrl Pts',(5.38621099635172,1.0693909211544,-4.85296106572622));
#157510=CARTESIAN_POINT('Ctrl Pts',(5.4173989531335,1.06258635419649,-4.88050820243491));
#157511=CARTESIAN_POINT('Ctrl Pts',(5.44860670944017,1.05593965794799,-4.90810785948304));
#157512=CARTESIAN_POINT('Ctrl Pts',(5.51099190624788,1.0429532023085,-4.96334305032409));
#157513=CARTESIAN_POINT('Ctrl Pts',(5.54220277780223,1.03660649187402,-4.99100819024458));
#157514=CARTESIAN_POINT('Ctrl Pts',(5.57339842834238,1.03040248140988,-5.01868807116424));
#157515=CARTESIAN_POINT('',(5.91022157977611,0.940053946665909,-4.40968041114037));
#157516=CARTESIAN_POINT('Origin',(-5.79831321845248E-13,1.03148891300033,
5.99346960949987E-13));
#157517=CARTESIAN_POINT('',(5.57585647005732,0.849330499761024,-5.01595699988355));
#157518=CARTESIAN_POINT('Origin',(-0.153113955485447,0.94642670548866,0.116826443368859));
#157519=CARTESIAN_POINT('',(5.18106734053611,0.940053948010703,-5.42277984334141));
#157520=CARTESIAN_POINT('Origin',(-0.147161145078586,0.803583943981683,
0.122490578603415));
#157521=CARTESIAN_POINT('Origin',(-0.13394123761439,0.946429246866666,0.138717858777231));
#157522=CARTESIAN_POINT('Ctrl Pts',(5.389338011,1.070162746,-4.8494882));
#157523=CARTESIAN_POINT('Ctrl Pts',(5.12655635500001,1.005280647,-5.14152297));
#157524=CARTESIAN_POINT('Ctrl Pts',(4.833756773,0.940053947,-5.403452179));
#157525=CARTESIAN_POINT('Ctrl Pts',(4.82369295517009,0.937812039337555,
-5.41245495088139));
#157526=CARTESIAN_POINT('Ctrl Pts',(4.81362913734007,0.935570131675098,
-5.4214577227628));
#157527=CARTESIAN_POINT('Ctrl Pts',(5.73741137229587,1.070162746,-4.83113577047591));
#157528=CARTESIAN_POINT('Ctrl Pts',(5.47562418787128,1.005280647,-5.14203176680072));
#157529=CARTESIAN_POINT('Ctrl Pts',(5.18177515547889,0.940053947,-5.42281922306667));
#157530=CARTESIAN_POINT('Ctrl Pts',(5.17167526697736,0.937812039337554,
-5.43247017198359));
#157531=CARTESIAN_POINT('Ctrl Pts',(5.16157537847578,0.9355701316751,-5.44212112090062));
#157532=CARTESIAN_POINT('',(5.00741204770229,0.940053949938004,-5.41311601880107));
#157533=CARTESIAN_POINT('Ctrl Pts',(4.833756773,0.940053947,-5.403452179));
#157534=CARTESIAN_POINT('Ctrl Pts',(4.537112626,1.005711878,-5.668820616));
#157535=CARTESIAN_POINT('Ctrl Pts',(4.213201843,1.070155008,-5.900121205));
#157536=CARTESIAN_POINT('Ctrl Pts',(4.814429119,0.940053947,-5.75076275500001));
#157537=CARTESIAN_POINT('Ctrl Pts',(4.498717966,1.005711878,-6.015070122));
#157538=CARTESIAN_POINT('Ctrl Pts',(4.155970918,1.070155008,-6.24322879));
#157539=CARTESIAN_POINT('',(4.81442911420674,0.940053946884196,-5.75076276067055));
#157540=CARTESIAN_POINT('',(4.36422588487778,1.0304024813986,-6.09946984755704));
#157541=CARTESIAN_POINT('Origin',(-0.135641776486256,0.803673954689217,
0.128082311223656));
#157542=CARTESIAN_POINT('Ctrl Pts',(4.21704119950274,1.06939092120473,-5.89737768206881));
#157543=CARTESIAN_POINT('Ctrl Pts',(4.24157817909531,1.06258635425499,-5.93098527065094));
#157544=CARTESIAN_POINT('Ctrl Pts',(4.26612320501677,1.05593965799867,-5.96464840807458));
#157545=CARTESIAN_POINT('Ctrl Pts',(4.3151759308655,1.04295320406734,-6.03200319497704));
#157546=CARTESIAN_POINT('Ctrl Pts',(4.33970991495528,1.03660649541051,-6.0657309438879));
#157547=CARTESIAN_POINT('Ctrl Pts',(4.3642258862629,1.03040248142576,-6.09946984635852));
#157548=CARTESIAN_POINT('',(4.82409294445209,0.940053946665909,-5.57710746833892));
#157549=CARTESIAN_POINT('Origin',(-2.55871712706579E-14,1.03148891300033,
5.63785129692462E-15));
#157550=CARTESIAN_POINT('',(4.36721355993799,0.849330499767501,-6.09733103257099));
#157551=CARTESIAN_POINT('Origin',(-0.124420020460023,0.946426691654718,
0.147010116000383));
#157552=CARTESIAN_POINT('',(3.89419949472767,0.940053948010701,-6.40977459130316));
#157553=CARTESIAN_POINT('Origin',(-0.117388650912164,0.803583922843219,
0.151261955103784));
#157554=CARTESIAN_POINT('Origin',(-0.100989597831267,0.946429327963876,
0.164268201422029));
#157555=CARTESIAN_POINT('Ctrl Pts',(4.22084167,1.070162746,-5.894658226));
#157556=CARTESIAN_POINT('Ctrl Pts',(3.90142486,1.005280647,-6.123375096));
#157557=CARTESIAN_POINT('Ctrl Pts',(3.559163733,0.940053947,-6.316237292));
#157558=CARTESIAN_POINT('Ctrl Pts',(3.54739987259014,0.93781203948184,-6.32286616034962));
#157559=CARTESIAN_POINT('Ctrl Pts',(3.53563601218029,0.935570131963667,
-6.32949502869939));
#157560=CARTESIAN_POINT('Ctrl Pts',(4.564722499399,1.070162746,-5.95156034962586));
#157561=CARTESIAN_POINT('Ctrl Pts',(4.24222230535363,1.005280647,-6.19891126289899));
#157562=CARTESIAN_POINT('Ctrl Pts',(3.89488229582533,0.940053947,-6.40996520962909));
#157563=CARTESIAN_POINT('Ctrl Pts',(3.88294386909641,0.93781203948184,-6.41721934681388));
#157564=CARTESIAN_POINT('Ctrl Pts',(3.8710054423675,0.93557013196367,-6.42447348399874));
#157565=CARTESIAN_POINT('',(3.72668160336882,0.940053949938004,-6.36300594715486));
#157566=CARTESIAN_POINT('Ctrl Pts',(3.559163733,0.940053947,-6.316237292));
#157567=CARTESIAN_POINT('Ctrl Pts',(3.212408591,1.005711878,-6.511631839));
#157568=CARTESIAN_POINT('Ctrl Pts',(2.846347872,1.070155008,-6.667893505));
#157569=CARTESIAN_POINT('Ctrl Pts',(3.465626441,0.940053947,-6.651273064));
#157570=CARTESIAN_POINT('Ctrl Pts',(3.100478168,1.005711878,-6.841532507));
#157571=CARTESIAN_POINT('Ctrl Pts',(2.716696986,1.070155008,-6.99067646800001));
#157572=CARTESIAN_POINT('',(3.46562643508481,0.940053946884187,-6.65127306852387));
#157573=CARTESIAN_POINT('',(2.95098699066175,1.03040248141321,-6.89504719174915));
#157574=CARTESIAN_POINT('Origin',(-0.104936565028214,0.803673979513478,
0.154246636087574));
#157575=CARTESIAN_POINT('Ctrl Pts',(2.85068724327674,1.06939092112309,-6.66603947209202));
#157576=CARTESIAN_POINT('Ctrl Pts',(2.86742593070085,1.06258635140717,-6.70413607482185));
#157577=CARTESIAN_POINT('Ctrl Pts',(2.88416053581012,1.05593965229657,-6.74228865949464));
#157578=CARTESIAN_POINT('Ctrl Pts',(2.91758713608327,1.04295320302106,-6.81861358783656));
#157579=CARTESIAN_POINT('Ctrl Pts',(2.9342970631903,1.03660649331213,-6.85682688896462));
#157580=CARTESIAN_POINT('Ctrl Pts',(2.95098699231288,1.03040248143631,-6.89504719088899));
#157581=CARTESIAN_POINT('',(3.51239508520041,0.940053946665902,-6.48375517897489));
#157582=CARTESIAN_POINT('Origin',(3.30464822173582E-13,1.03148891299967,
-9.38051719634458E-13));
#157583=CARTESIAN_POINT('',(2.95436459746952,0.84933049977548,-6.89360064298541));
#157584=CARTESIAN_POINT('Origin',(-0.0899083695330682,0.94642667139641,
0.170319820844224));
#157585=CARTESIAN_POINT('',(2.42524320939457,0.940053948010701,-7.09705540292411));
#157586=CARTESIAN_POINT('Origin',(-0.0821273225261276,0.803583927069448,
0.172960628750021));
#157587=CARTESIAN_POINT('Origin',(-0.0633156235864346,0.946429243334707,
0.182137290076859));
#157588=CARTESIAN_POINT('Ctrl Pts',(2.854983464,1.070162746,-6.664200584));
#157589=CARTESIAN_POINT('Ctrl Pts',(2.493867074,1.005280647,-6.818905009));
#157590=CARTESIAN_POINT('Ctrl Pts',(2.118148151,0.940053947,-6.933682168));
#157591=CARTESIAN_POINT('Ctrl Pts',(2.10523431145353,0.937812039322795,
-6.93762717508959));
#157592=CARTESIAN_POINT('Ctrl Pts',(2.09232047190712,0.935570131645578,
-6.94157218217907));
#157593=CARTESIAN_POINT('Ctrl Pts',(3.17859227582898,1.070162746,-6.79369658044958));
#157594=CARTESIAN_POINT('Ctrl Pts',(2.81045882138829,1.005280647,-6.96593655959706));
#157595=CARTESIAN_POINT('Ctrl Pts',(2.42586906972625,0.940053947,-7.09738834677674));
#157596=CARTESIAN_POINT('Ctrl Pts',(2.41265033082292,0.937812039322796,
-7.10190647770869));
#157597=CARTESIAN_POINT('Ctrl Pts',(2.39943159191954,0.935570131645576,
-7.10642460864078));
#157598=CARTESIAN_POINT('',(2.27169566876624,0.940053949938004,-7.01536878858059));
#157599=CARTESIAN_POINT('Ctrl Pts',(2.118148151,0.940053947,-6.933682168));
#157600=CARTESIAN_POINT('Ctrl Pts',(1.7374959,1.005711878,-7.049966394));
#157601=CARTESIAN_POINT('Ctrl Pts',(1.346401839,1.070155008,-7.123882515));
#157602=CARTESIAN_POINT('Ctrl Pts',(1.954774922,0.940053947,-7.240777238));
#157603=CARTESIAN_POINT('Ctrl Pts',(1.557263457,1.005711878,-7.348092436));
#157604=CARTESIAN_POINT('Ctrl Pts',(1.150393323,1.070155008,-7.411247884));
#157605=CARTESIAN_POINT('',(1.95477491526828,0.940053946884195,-7.24077724113414));
#157606=CARTESIAN_POINT('',(1.39976322578504,1.03040248139436,-7.36821979250953));
#157607=CARTESIAN_POINT('Origin',(-0.0693247149754145,0.80367397856932,
0.173198591715785));
#157608=CARTESIAN_POINT('Ctrl Pts',(1.35103831954935,1.06939092127104,-7.12300466507705));
#157609=CARTESIAN_POINT('Ctrl Pts',(1.35919602246169,1.06258635152761,-7.16380891331529));
#157610=CARTESIAN_POINT('Ctrl Pts',(1.36733770403458,1.05593965239,-7.20466695716615));
#157611=CARTESIAN_POINT('Ctrl Pts',(1.38357520950748,1.04295320012166,-7.28639320066194));
#157612=CARTESIAN_POINT('Ctrl Pts',(1.39167974182571,1.03660648740826,-7.32730525705295));
#157613=CARTESIAN_POINT('Ctrl Pts',(1.39976322701735,1.03040248140542,-7.36821979220919));
#157614=CARTESIAN_POINT('',(2.03646153453295,0.940053946665909,-7.08722970356521));
#157615=CARTESIAN_POINT('Origin',(-1.22081164621868E-13,1.03148891300022,
7.35522753814166E-13));
#157616=CARTESIAN_POINT('',(1.40337283012418,0.849330499797391,-7.36753314876967));
#157617=CARTESIAN_POINT('Origin',(-0.0511926721854314,0.946426678719604,
0.185665675650389));
#157618=CARTESIAN_POINT('',(0.842885249819145,0.940053948012019,-7.45248579171939));
#157619=CARTESIAN_POINT('Origin',(-0.0430257937312871,0.803583941878107,
0.186571820443324));
#157620=CARTESIAN_POINT('Origin',(-0.022681201455298,0.946429259171787,
0.191490017379453));
#157621=CARTESIAN_POINT('Ctrl Pts',(1.355629403,1.070162746,-7.12213233));
#157622=CARTESIAN_POINT('Ctrl Pts',(0.969698837,1.005280647,-7.195590502));
#157623=CARTESIAN_POINT('Ctrl Pts',(0.578090316999999,0.940053947,-7.226915773));
#157624=CARTESIAN_POINT('Ctrl Pts',(0.564630335631451,0.937812039273551,
-7.22799245428371));
#157625=CARTESIAN_POINT('Ctrl Pts',(0.551170354262883,0.935570131547088,
-7.22906913556744));
#157626=CARTESIAN_POINT('Ctrl Pts',(1.64383461035206,1.070162746,-7.31816711034626));
#157627=CARTESIAN_POINT('Ctrl Pts',(1.24728140782744,1.005280647,-7.40724240375129));
#157628=CARTESIAN_POINT('Ctrl Pts',(0.843424901635076,0.940053947,-7.45294549263674));
#157629=CARTESIAN_POINT('Ctrl Pts',(0.82954394457899,0.937812039273551,
-7.45451635407991));
#157630=CARTESIAN_POINT('Ctrl Pts',(0.815662987522898,0.935570131547088,
-7.45608721552305));
#157631=CARTESIAN_POINT('',(0.710487769969494,0.940053949938004,-7.33970078274537));
#157632=CARTESIAN_POINT('Ctrl Pts',(0.578090317,0.940053947,-7.226915773));
#157633=CARTESIAN_POINT('Ctrl Pts',(0.181339832,1.005711878,-7.258652356));
#157634=CARTESIAN_POINT('Ctrl Pts',(-0.216500448,1.070155008,-7.246766697));
#157635=CARTESIAN_POINT('Ctrl Pts',(0.3525203,0.940053947,-7.49171071500001));
#157636=CARTESIAN_POINT('Ctrl Pts',(-0.058767163,1.005711878,-7.51106372900001));
#157637=CARTESIAN_POINT('Ctrl Pts',(-0.469701454,1.070155008,-7.485277586));
#157638=CARTESIAN_POINT('Ctrl Pts',(-0.211783653451336,1.06939092118085,
-7.246906076998));
#157639=CARTESIAN_POINT('Ctrl Pts',(-0.212588380605611,1.06258635139668,
-7.28851000993393));
#157640=CARTESIAN_POINT('Ctrl Pts',(-0.213420318916879,1.05593965224487,
-7.33016303650157));
#157641=CARTESIAN_POINT('Ctrl Pts',(-0.215131163835453,1.04295320260911,
-7.41346913277568));
#157642=CARTESIAN_POINT('Ctrl Pts',(-0.216010993470867,1.03660649245927,
-7.45516690495362));
#157643=CARTESIAN_POINT('Ctrl Pts',(-0.216911912134888,1.03040248144745,
-7.49686262505193));
#157644=CARTESIAN_POINT('',(0.465305306457437,0.940053946665909,-7.35931324412915));
#157645=CARTESIAN_POINT('Ctrl Pts',(-0.207112381,1.070162746,-7.247041083));
#157646=CARTESIAN_POINT('Ctrl Pts',(-0.599811441,1.005280647,-7.23581818000001));
#157647=CARTESIAN_POINT('Ctrl Pts',(-0.988998379000001,0.940053947,-7.182226828));
#157648=CARTESIAN_POINT('Ctrl Pts',(-1.00237512739108,0.937812039399596,
-7.18038483906961));
#157649=CARTESIAN_POINT('Ctrl Pts',(-1.01575187578216,0.935570131799181,
-7.17854285013935));
#157650=CARTESIAN_POINT('Ctrl Pts',(0.0322130647155368,1.070162746,-7.5004482804543));
#157651=CARTESIAN_POINT('Ctrl Pts',(-0.37421749868138,1.005280647,-7.50219382593539));
#157652=CARTESIAN_POINT('Ctrl Pts',(-0.778456877626605,0.940053947,-7.46001119120499));
#157653=CARTESIAN_POINT('Ctrl Pts',(-0.792350993625732,0.937812039399596,
-7.4585613314174));
#157654=CARTESIAN_POINT('Ctrl Pts',(-0.806245109624853,0.93557013179918,
-7.45711147162981));
#157655=CARTESIAN_POINT('',(-0.883941747984165,0.940053949938004,-7.32083652582854));
#157656=CARTESIAN_POINT('Ctrl Pts',(-0.988998379000001,0.940053947,-7.182226828));
#157657=CARTESIAN_POINT('Ctrl Pts',(-1.383295485,1.005711878,-7.127931801));
#157658=CARTESIAN_POINT('Ctrl Pts',(-1.769279415,1.070155008,-7.030800122));
#157659=CARTESIAN_POINT('Ctrl Pts',(-1.266217779,0.940053947,-7.392340126));
#157660=CARTESIAN_POINT('Ctrl Pts',(-1.672049896,1.005711878,-7.32282603));
#157661=CARTESIAN_POINT('Ctrl Pts',(-2.067833513,1.070155008,-7.209304028));
#157662=CARTESIAN_POINT('',(-1.26621778643958,0.940053946884194,-7.39234012602042));
#157663=CARTESIAN_POINT('',(-1.82344449210477,1.03040248140051,-7.27496049378735));
#157664=CARTESIAN_POINT('Origin',(0.00980681374477876,0.803673982828573,
0.186299599692954));
#157665=CARTESIAN_POINT('Ctrl Pts',(-1.76470285870304,1.0693909211237,-7.03195021484481));
#157666=CARTESIAN_POINT('Ctrl Pts',(-1.77443238319902,1.06258635439378,
-7.0724084603665));
#157667=CARTESIAN_POINT('Ctrl Pts',(-1.78419903575377,1.05593965838706,
-7.11290879976689));
#157668=CARTESIAN_POINT('Ctrl Pts',(-1.80377824443044,1.04295319938803,
-7.19389952326287));
#157669=CARTESIAN_POINT('Ctrl Pts',(-1.81360129805581,1.03660648596745,
-7.23443330970032));
#157670=CARTESIAN_POINT('Ctrl Pts',(-1.8234444908508,1.03040248140673,-7.27496049406823));
#157671=CARTESIAN_POINT('',(-1.12760808102257,0.940053946665909,-7.28728347668704));
#157672=CARTESIAN_POINT('Origin',(1.82688066063807E-13,1.03148891300028,
1.05688027773887E-12));
#157673=CARTESIAN_POINT('',(-1.81988018947365,0.849330499782048,-7.27585294622769));
#157674=CARTESIAN_POINT('Origin',(0.0314977611362444,0.946426717532798,
0.190000801711974));
#157675=CARTESIAN_POINT('',(-2.36423563052596,0.940053948011583,-7.11761125000035));
#157676=CARTESIAN_POINT('Origin',(0.0392903192037833,0.80358394884751,0.18739407073207));
#157677=CARTESIAN_POINT('Origin',(0.0598196617767915,0.946429284061458,
0.183315221226698));
#157678=CARTESIAN_POINT('Ctrl Pts',(-1.76016982,1.070162746,-7.03308625));
#157679=CARTESIAN_POINT('Ctrl Pts',(-2.141275202,1.005280647,-6.93770704300001));
#157680=CARTESIAN_POINT('Ctrl Pts',(-2.509842609,0.940053947,-6.801704939));
#157681=CARTESIAN_POINT('Ctrl Pts',(-2.5225106438222,0.937812039302131,
-6.7970304090317));
#157682=CARTESIAN_POINT('Ctrl Pts',(-2.53517867864446,0.935570131604248,
-6.79235587906328));
#157683=CARTESIAN_POINT('Ctrl Pts',(-1.58091472751367,1.070162746,-7.33201682380305));
#157684=CARTESIAN_POINT('Ctrl Pts',(-1.9782184109335,1.005280647,-7.2463510030766));
#157685=CARTESIAN_POINT('Ctrl Pts',(-2.36393887816032,0.940053947,-7.11825505777561));
#157686=CARTESIAN_POINT('Ctrl Pts',(-2.37719648102391,0.937812039302131,
-7.11385227048396));
#157687=CARTESIAN_POINT('Ctrl Pts',(-2.39045408388743,0.935570131604251,
-7.10944948319232));
#157688=CARTESIAN_POINT('',(-2.4370391315969,0.940053949938004,-6.95965808951324));
#157689=CARTESIAN_POINT('Ctrl Pts',(-2.509842609,0.940053947,-6.801704939));
#157690=CARTESIAN_POINT('Ctrl Pts',(-2.883249442,1.005711878,-6.663917077));
#157691=CARTESIAN_POINT('Ctrl Pts',(-3.239328843,1.070155008,-6.486081147));
#157692=CARTESIAN_POINT('Ctrl Pts',(-2.825748922,0.940053947,-6.947311928));
#157693=CARTESIAN_POINT('Ctrl Pts',(-3.207149434,1.005711878,-6.792181124));
#157694=CARTESIAN_POINT('Ctrl Pts',(-3.569275975,1.070155008,-6.596231425));
#157695=CARTESIAN_POINT('',(-2.82574892929789,0.940053946884188,-6.94731192641957));
#157696=CARTESIAN_POINT('',(-3.34471483303188,1.03040248138734,-6.71288929457019));
#157697=CARTESIAN_POINT('Origin',(0.0496264431287224,0.803673994692571,
0.179835839121838));
#157698=CARTESIAN_POINT('Ctrl Pts',(-3.23510652003408,1.06939092112879,
-6.48818817562549));
#157699=CARTESIAN_POINT('Ctrl Pts',(-3.25330590091125,1.06258635422436,
-6.5256089706994));
#157700=CARTESIAN_POINT('Ctrl Pts',(-3.27155059089123,1.05593965801357,
-6.56306289431301));
#157701=CARTESIAN_POINT('Ctrl Pts',(-3.308082654659,1.04295320088744,-6.63795113776892));
#157702=CARTESIAN_POINT('Ctrl Pts',(-3.32638961188595,1.03660648899569,
-6.67542559096316));
#157703=CARTESIAN_POINT('Ctrl Pts',(-3.34471483187464,1.03040248140146,
-6.71288929505088));
#157704=CARTESIAN_POINT('',(-2.66779576740801,0.940053946665909,-6.87450843275956));
#157705=CARTESIAN_POINT('Origin',(-4.28693539000768E-13,1.03148891300006,
-1.08116640640255E-12));
#157706=CARTESIAN_POINT('',(-3.34142571261753,0.849330499763146,-6.71452710230813));
#157707=CARTESIAN_POINT('Origin',(0.0716058869507563,0.946426693350637,
0.1787875325584));
#157708=CARTESIAN_POINT('',(-3.83903714025104,0.940053948010709,-6.44296467836105));
#157709=CARTESIAN_POINT('Origin',(0.0786558872479498,0.803583953786049,
0.174566560624118));
#157710=CARTESIAN_POINT('Origin',(0.0978284994784367,0.946429275126823,
0.166170014912738));
#157711=CARTESIAN_POINT('Ctrl Pts',(-3.230923675,1.070162746,-6.490272121));
#157712=CARTESIAN_POINT('Ctrl Pts',(-3.582615315,1.005280647,-6.315196435));
#157713=CARTESIAN_POINT('Ctrl Pts',(-3.913329389,0.940053947,-6.10314288700001));
#157714=CARTESIAN_POINT('Ctrl Pts',(-3.92469636653137,0.937812039286857,
-6.09585439187666));
#157715=CARTESIAN_POINT('Ctrl Pts',(-3.93606334406277,0.9355701315737,-6.08856589675335));
#157716=CARTESIAN_POINT('Ctrl Pts',(-3.12012070378108,1.070162746,-6.82074841004759));
#157717=CARTESIAN_POINT('Ctrl Pts',(-3.48972002877604,1.005280647,-6.6516768603758));
#157718=CARTESIAN_POINT('Ctrl Pts',(-3.83888572403908,0.940053947,-6.44365722863245));
#157719=CARTESIAN_POINT('Ctrl Pts',(-3.85088690247331,0.937812039286857,
-6.4365073832947));
#157720=CARTESIAN_POINT('Ctrl Pts',(-3.86288808090748,0.935570131573697,
-6.42935753795705));
#157721=CARTESIAN_POINT('',(-3.87618327441021,0.940053949938004,-6.27305377597788));
#157722=CARTESIAN_POINT('Ctrl Pts',(-3.913329389,0.940053947,-6.103142887));
#157723=CARTESIAN_POINT('Ctrl Pts',(-4.24838586,1.005711878,-5.888304997));
#157724=CARTESIAN_POINT('Ctrl Pts',(-4.557910854,1.070155008,-5.638080227));
#157725=CARTESIAN_POINT('Ctrl Pts',(-4.253151186,0.940053947,-6.177435146));
#157726=CARTESIAN_POINT('Ctrl Pts',(-4.592286229,1.005711878,-5.943941379));
#157727=CARTESIAN_POINT('Ctrl Pts',(-4.903823059,1.070155008,-5.674726372));
#157728=CARTESIAN_POINT('',(-4.25315119279166,0.940053946884186,-6.1774351428866));
#157729=CARTESIAN_POINT('',(-4.70959002624101,1.03040248143653,-5.83693085285918));
#157730=CARTESIAN_POINT('Origin',(0.0871253604258709,0.803673999127675,
0.164962849378982));
#157731=CARTESIAN_POINT('Ctrl Pts',(-4.55424019564849,1.06939092116492,
-5.6410456689495));
#157732=CARTESIAN_POINT('Ctrl Pts',(-4.58005845053803,1.06258635411618,
-5.67367925829113));
#157733=CARTESIAN_POINT('Ctrl Pts',(-4.60592807690455,1.05593965775849,
-5.70633546168935));
#157734=CARTESIAN_POINT('Ctrl Pts',(-4.65770463307133,1.04295324250708,
-5.77161933531371));
#157735=CARTESIAN_POINT('Ctrl Pts',(-4.68363929647117,1.03660657338509,
-5.80428196715605));
#157736=CARTESIAN_POINT('Ctrl Pts',(-4.70959002478975,1.03040248144053,
-5.83693085401346));
#157737=CARTESIAN_POINT('',(-4.08324028920423,0.940053946665909,-6.14028901536671));
#157738=CARTESIAN_POINT('Ctrl Pts',(-4.55060313,1.070162746,-5.643980081));
#157739=CARTESIAN_POINT('Ctrl Pts',(-4.856436318,1.005280647,-5.39739426));
#157740=CARTESIAN_POINT('Ctrl Pts',(-5.133833235,0.940053947,-5.119204656));
#157741=CARTESIAN_POINT('Ctrl Pts',(-5.14336764735008,0.937812039408671,
-5.10964299819672));
#157742=CARTESIAN_POINT('Ctrl Pts',(-5.15290205970014,0.93557013181733,
-5.10008134039349));
#157743=CARTESIAN_POINT('Ctrl Pts',(-4.51343330428368,1.070162746,-5.99054938140099));
#157744=CARTESIAN_POINT('Ctrl Pts',(-4.8380462168537,1.005280647,-5.74597770079901));
#157745=CARTESIAN_POINT('Ctrl Pts',(-5.13433054042948,0.940053947,-5.46776114999407));
#157746=CARTESIAN_POINT('Ctrl Pts',(-5.1445141320295,0.937812039408671,
-5.4581985660019));
#157747=CARTESIAN_POINT('Ctrl Pts',(-5.15469772362943,0.93557013181733,
-5.44863598200959));
#157748=CARTESIAN_POINT('',(-5.1343295360762,0.940053947994143,-5.46705224605016));
#157749=CARTESIAN_POINT('Origin',(0.131263079631537,0.946429252240351,0.141254971903578));
#157750=CARTESIAN_POINT('',(-5.13408139500295,0.940053949938004,-5.29312843988776));
#157751=CARTESIAN_POINT('Origin',(3.29163779566599E-13,1.03148891300067,
2.43294967505747E-13));
#157752=CARTESIAN_POINT('',(-4.70672988344602,0.84933049976998,-5.83923743366367));
#157753=CARTESIAN_POINT('Origin',(0.108365671171387,0.946426717023636,0.159214253106947));
#157754=CARTESIAN_POINT('Origin',(0.114343691470368,0.803583965489527,0.153576714676756));
#157755=CARTESIAN_POINT('Ctrl Pts',(-5.133833235,0.940053947,-5.119204656));
#157756=CARTESIAN_POINT('Ctrl Pts',(-5.414872477,1.005711878,-4.83736232));
#157757=CARTESIAN_POINT('Ctrl Pts',(-5.663370019,1.070155008,-4.526448942));
#157758=CARTESIAN_POINT('Ctrl Pts',(-5.48168082800001,0.940053947,-5.118708363));
#157759=CARTESIAN_POINT('Ctrl Pts',(-5.762692823,1.005711878,-4.81776954000001));
#157760=CARTESIAN_POINT('Ctrl Pts',(-6.00907282800001,1.070155008,-4.487877421));
#157761=CARTESIAN_POINT('',(-5.48168083392426,0.940053946884176,-5.11870835851933));
#157762=CARTESIAN_POINT('',(-5.30775703292102,0.940053946665848,-5.11895650802657));
#157763=CARTESIAN_POINT('',(-5.85425002368675,1.03040248140204,-4.6880440119527));
#157764=CARTESIAN_POINT('Origin',(0.12055094137318,0.803673950252423,0.142377062403563));
#157765=CARTESIAN_POINT('Ctrl Pts',(-5.66042266110811,1.06939092119514,
-4.5301341364565));
#157766=CARTESIAN_POINT('Ctrl Pts',(-5.69265256937191,1.06258635144978,
-4.55645461935443));
#157767=CARTESIAN_POINT('Ctrl Pts',(-5.72493751116658,1.05593965231105,
-4.58278614556));
#157768=CARTESIAN_POINT('Ctrl Pts',(-5.78953782558348,1.04295320444697,
-4.63541342140573));
#157769=CARTESIAN_POINT('Ctrl Pts',(-5.8218878647054,1.03660649618985,-4.66173740606064));
#157770=CARTESIAN_POINT('Ctrl Pts',(-5.85425002241471,1.03040248143066,
-4.68804401325544));
#157771=CARTESIAN_POINT('Origin',(-7.68482499857726E-13,1.03148891300006,
-6.66133814775094E-13));
#157772=CARTESIAN_POINT('',(-6.18954639384257,0.94005394801071,-4.23550651616131));
#157773=CARTESIAN_POINT('Origin',(0.158559547460965,0.946429307724211,0.109734571990215));
#157774=CARTESIAN_POINT('',(-5.85195259583044,0.849330499752317,-4.69091151220864));
#157775=CARTESIAN_POINT('Origin',(0.140058776211579,0.946426676654599,0.132196708814087));
#157776=CARTESIAN_POINT('Origin',(0.144684649935504,0.80358397165336,0.125405500795563));
#157777=CARTESIAN_POINT('Ctrl Pts',(-5.65750144,1.070162746,-4.533781805));
#157778=CARTESIAN_POINT('Ctrl Pts',(-5.903175755,1.005280647,-4.227215929));
#157779=CARTESIAN_POINT('Ctrl Pts',(-6.114284746,0.940053947,-3.895898106));
#157780=CARTESIAN_POINT('Ctrl Pts',(-6.12154077546899,0.937812039371516,
-3.8845103774343));
#157781=CARTESIAN_POINT('Ctrl Pts',(-6.12879680493797,0.935570131743017,
-3.87312264886852));
#157782=CARTESIAN_POINT('Ctrl Pts',(-5.69570277961804,1.070162746,-4.88023892213736));
#157783=CARTESIAN_POINT('Ctrl Pts',(-5.96015074082017,1.005280647,-4.57160301106027));
#157784=CARTESIAN_POINT('Ctrl Pts',(-6.18969976651681,0.940053947,-4.23619863575172));
#157785=CARTESIAN_POINT('Ctrl Pts',(-6.19758959862271,0.937812039371516,
-4.22467044825133));
#157786=CARTESIAN_POINT('Ctrl Pts',(-6.20547943072859,0.935570131743017,
-4.21314226075093));
#157787=CARTESIAN_POINT('',(-6.15191557598767,0.940053949937996,-4.06570230088741));
#157788=CARTESIAN_POINT('Ctrl Pts',(-6.114284746,0.940053947,-3.895898106));
#157789=CARTESIAN_POINT('Ctrl Pts',(-6.328165675,1.005711878,-3.560229957));
#157790=CARTESIAN_POINT('Ctrl Pts',(-6.504016297,1.070155008,-3.203165935));
#157791=CARTESIAN_POINT('Ctrl Pts',(-6.453893166,0.940053947,-3.820636465));
#157792=CARTESIAN_POINT('Ctrl Pts',(-6.663642306,1.005711878,-3.466324153));
#157793=CARTESIAN_POINT('Ctrl Pts',(-6.833345029,1.070155008,-3.09118031));
#157794=CARTESIAN_POINT('',(-6.45389317085123,0.940053946884177,-3.82063645932707));
#157795=CARTESIAN_POINT('',(-6.72517179580522,1.03040248141041,-3.3199494442733));
#157796=CARTESIAN_POINT('Origin',(0.148339177973227,0.803673947869585,0.11313337249165));
#157797=CARTESIAN_POINT('Ctrl Pts',(-6.50193005456292,1.06939092119945,
-3.2073985664642));
#157798=CARTESIAN_POINT('Ctrl Pts',(-6.53906455727252,1.06258635401515,
-3.22617520648721));
#157799=CARTESIAN_POINT('Ctrl Pts',(-6.57625517898209,1.05593965751181,
-3.24495080022106));
#157800=CARTESIAN_POINT('Ctrl Pts',(-6.65065852245689,1.04295320266092,
-3.2824605419063));
#157801=CARTESIAN_POINT('Ctrl Pts',(-6.68791112565472,1.03660649256361,
-3.30121479015096));
#157802=CARTESIAN_POINT('Ctrl Pts',(-6.72517179514983,1.03040248143128,
-3.31994944530406));
#157803=CARTESIAN_POINT('',(-6.28408895707088,0.940053946665902,-3.85826728375583));
#157804=CARTESIAN_POINT('Origin',(-1.09461051334137E-12,1.03148891300011,
-5.60966204044E-13));
#157805=CARTESIAN_POINT('',(-6.72354450891251,0.849330499744447,-3.32324378227747));
#157806=CARTESIAN_POINT('Origin',(0.165202437536132,0.946426669462313,0.0989974117800008));
#157807=CARTESIAN_POINT('',(-6.95534693954528,0.940053948010697,-2.8059132146749));
#157808=CARTESIAN_POINT('Origin',(0.168260764014773,0.803583930496838,0.0913708078726105));
#157809=CARTESIAN_POINT('Origin',(0.178442577358902,0.946429305675131,0.0730836020607856));
#157810=CARTESIAN_POINT('Ctrl Pts',(-6.499861271,1.070162746,-3.211588931));
#157811=CARTESIAN_POINT('Ctrl Pts',(-6.673889256,1.005280647,-2.859377679));
#157812=CARTESIAN_POINT('Ctrl Pts',(-6.808839097,0.940053947,-2.49042369));
#157813=CARTESIAN_POINT('Ctrl Pts',(-6.81347745935914,0.93781203943013,
-2.4777423686872));
#157814=CARTESIAN_POINT('Ctrl Pts',(-6.8181158217183,0.935570131860246,
-2.46506104737443));
#157815=CARTESIAN_POINT('Ctrl Pts',(-6.61164752301968,1.070162746,-3.54173391418792));
#157816=CARTESIAN_POINT('Ctrl Pts',(-6.80356523949808,1.005280647,-3.18346524449584));
#157817=CARTESIAN_POINT('Ctrl Pts',(-6.95564551169704,0.940053947,-2.8065561823157));
#157818=CARTESIAN_POINT('Ctrl Pts',(-6.96087266428134,0.93781203943013,
-2.79360143710162));
#157819=CARTESIAN_POINT('Ctrl Pts',(-6.96609981686578,0.935570131860243,
-2.78064669188749));
#157820=CARTESIAN_POINT('',(-6.88209302200538,0.940053949937988,-2.64816844109373));
#157821=CARTESIAN_POINT('Ctrl Pts',(-6.808839097,0.940053947,-2.49042369));
#157822=CARTESIAN_POINT('Ctrl Pts',(-6.945560879,1.005711878,-2.116625199));
#157823=CARTESIAN_POINT('Ctrl Pts',(-7.040542002,1.070155008,-1.730106449));
#157824=CARTESIAN_POINT('Ctrl Pts',(-7.124328633,0.940053947,-2.343915853));
#157825=CARTESIAN_POINT('Ctrl Pts',(-7.253007281,1.005711878,-1.9527973));
#157826=CARTESIAN_POINT('Ctrl Pts',(-7.33809761200001,1.070155008,-1.549943043));
#157827=CARTESIAN_POINT('',(-7.12432863651568,0.940053946884185,-2.34391584642018));
#157828=CARTESIAN_POINT('',(-7.28163201009094,1.03040248138348,-1.79661772960873));
#157829=CARTESIAN_POINT('Origin',(0.16919157413491,0.803673975598803,0.0785998784174352));
#157830=CARTESIAN_POINT('Ctrl Pts',(-7.039414425409,1.06939092121324,-1.73468860427594));
#157831=CARTESIAN_POINT('Ctrl Pts',(-7.07971716454285,1.06258635436219,
-1.74504343605081));
#157832=CARTESIAN_POINT('Ctrl Pts',(-7.12007448535464,1.05593965822046,
-1.75538518191534));
#157833=CARTESIAN_POINT('Ctrl Pts',(-7.20080181548591,1.04295320175447,
-1.77602344967893));
#157834=CARTESIAN_POINT('Ctrl Pts',(-7.241215088716,1.03660649073035,-1.78633102704174));
#157835=CARTESIAN_POINT('Ctrl Pts',(-7.28163200969059,1.03040248140093,
-1.79661773077921));
#157836=CARTESIAN_POINT('',(-6.9665838656709,0.940053946665902,-2.41716976956639));
#157837=CARTESIAN_POINT('Origin',(-1.03866568124111E-12,1.03148891300022,
-2.78531538111526E-13));
#157838=CARTESIAN_POINT('',(-7.2807509534696,0.849330499739627,-1.80018486640627));
#157839=CARTESIAN_POINT('Origin',(0.182621432084888,0.946426675897866,0.0611692177252093));
#157840=CARTESIAN_POINT('',(-7.39592319216369,0.940053948011588,-1.24511853176423));
#157841=CARTESIAN_POINT('Origin',(0.183968884429788,0.803583937744143,0.0530635059579526));
#157842=CARTESIAN_POINT('Origin',(0.189981445166029,0.946429293144479,0.0330150515353095));
#157843=CARTESIAN_POINT('Ctrl Pts',(-7.038294813,1.070162746,-1.739225727));
#157844=CARTESIAN_POINT('Ctrl Pts',(-7.13253911200001,1.005280647,-1.357838106));
#157845=CARTESIAN_POINT('Ctrl Pts',(-7.185019699,0.940053947,-0.96849983));
#157846=CARTESIAN_POINT('Ctrl Pts',(-7.18682350978693,0.937812039434179,
-0.955117880175332));
#157847=CARTESIAN_POINT('Ctrl Pts',(-7.1886273205737,0.935570131868345,
-0.941735930350652));
#157848=CARTESIAN_POINT('Ctrl Pts',(-7.21843897667503,1.070162746,-2.03762136480417));
#157849=CARTESIAN_POINT('Ctrl Pts',(-7.32885259013869,1.005280647,-1.64647218155056));
#157850=CARTESIAN_POINT('Ctrl Pts',(-7.39635300274975,0.940053947,-1.24568228101568));
#157851=CARTESIAN_POINT('Ctrl Pts',(-7.39867306011474,0.937812039434179,
-1.23190672728822));
#157852=CARTESIAN_POINT('Ctrl Pts',(-7.40099311747971,0.935570131868342,
-1.21813117356077));
#157853=CARTESIAN_POINT('',(-7.29047144671895,0.940053949937996,-1.10680916809047));
#157854=CARTESIAN_POINT('Ctrl Pts',(-7.185019699,0.940053947,-0.96849983));
#157855=CARTESIAN_POINT('Ctrl Pts',(-7.238189376,1.005711878,-0.574049398));
#157856=CARTESIAN_POINT('Ctrl Pts',(-7.247859787,1.070155008,-0.176149108));
#157857=CARTESIAN_POINT('Ctrl Pts',(-7.461638412,0.940053947,-0.75759634));
#157858=CARTESIAN_POINT('Ctrl Pts',(-7.503229697,1.005711878,-0.347959816));
#157859=CARTESIAN_POINT('Ctrl Pts',(-7.499728906,1.070155008,0.063767838));
#157860=CARTESIAN_POINT('',(-7.46163841400411,0.940053946884194,-0.757596332849195));
#157861=CARTESIAN_POINT('',(-7.49761120468137,1.0304024813601,-0.189278166809903));
#157862=CARTESIAN_POINT('Origin',(0.182132582553779,0.803673978539305,0.0403910626042792));
#157863=CARTESIAN_POINT('Ctrl Pts',(-7.24774360045422,1.06939092115902,
-0.180866531000679));
#157864=CARTESIAN_POINT('Ctrl Pts',(-7.28933006618477,1.06258635442796,
-0.18231537485848));
#157865=CARTESIAN_POINT('Ctrl Pts',(-7.33096702426481,1.0559396584134,-0.183739705341759));
#157866=CARTESIAN_POINT('Ctrl Pts',(-7.41424361053092,1.04295320219039,
-0.186541472070499));
#157867=CARTESIAN_POINT('Ctrl Pts',(-7.4559278651807,1.03660649163244,-0.187920404768487));
#157868=CARTESIAN_POINT('Ctrl Pts',(-7.49761120453003,1.03040248137935,
-0.189278168028761));
#157869=CARTESIAN_POINT('',(-7.32332905573954,0.940053946665902,-0.863048082967379));
#157870=CARTESIAN_POINT('Origin',(-1.02782365951626E-13,1.03148891300017,
-9.97465998686664E-14));
#157871=CARTESIAN_POINT('',(-7.49751757547009,0.849330500331513,-0.192951307338575));
#157872=CARTESIAN_POINT('Origin',(0.191501740654354,0.946426720742303,0.0204809236977732));
#157873=CARTESIAN_POINT('',(-7.49067429688827,0.940053948011587,0.373896511679711));
#157874=CARTESIAN_POINT('Origin',(0.191074840971184,0.80358395566385,0.012275030548928));
#157875=CARTESIAN_POINT('Origin',(0.192636884694252,0.946429308031184,-0.00859721590453562));
#157876=CARTESIAN_POINT('Ctrl Pts',(-7.24762551100001,1.070162746,-0.185538262));
#157877=CARTESIAN_POINT('Ctrl Pts',(-7.257679367,1.005280647,0.207192467));
#157878=CARTESIAN_POINT('Ctrl Pts',(-7.225236766,0.940053947,0.598710006));
#157879=CARTESIAN_POINT('Ctrl Pts',(-7.22412168102199,0.937812039412696,
0.612166859424246));
#157880=CARTESIAN_POINT('Ctrl Pts',(-7.2230065960441,0.935570131825379,
0.62562371284849));
#157881=CARTESIAN_POINT('Ctrl Pts',(-7.48770424676855,1.070162746,-0.438231905210894));
#157882=CARTESIAN_POINT('Ctrl Pts',(-7.51145093952435,1.005280647,-0.0324919097134924));
#157883=CARTESIAN_POINT('Ctrl Pts',(-7.4912152481729,0.940053947,0.373438339134095));
#157884=CARTESIAN_POINT('Ctrl Pts',(-7.49051972701397,0.937812039412696,
0.387390571959122));
#157885=CARTESIAN_POINT('Ctrl Pts',(-7.48982420585515,0.93557013182538,
0.401342804784149));
#157886=CARTESIAN_POINT('',(-7.35795552980536,0.940053949937996,0.486303271575305));
#157887=CARTESIAN_POINT('Ctrl Pts',(-7.225236766,0.940053947,0.598710006));
#157888=CARTESIAN_POINT('Ctrl Pts',(-7.192368183,1.005711878,0.995368314));
#157889=CARTESIAN_POINT('Ctrl Pts',(-7.116275704,1.070155008,1.386044769));
#157890=CARTESIAN_POINT('Ctrl Pts',(-7.450050271,0.940053947,0.864147535));
#157891=CARTESIAN_POINT('Ctrl Pts',(-7.402609431,1.005711878,1.273147882));
#157892=CARTESIAN_POINT('Ctrl Pts',(-7.310681212,1.070155008,1.674497005));
#157893=CARTESIAN_POINT('',(-7.45005027142285,0.940053946884191,0.864147542426273));
#157894=CARTESIAN_POINT('',(-7.36301043203333,1.0304024814159,1.426911832604));
#157895=CARTESIAN_POINT('Origin',(0.186557358451386,0.803674007595516,0.000293611196806182));
#157896=CARTESIAN_POINT('Ctrl Pts',(-7.11717634030228,1.06939092119072,
1.38141266024738));
#157897=CARTESIAN_POINT('Ctrl Pts',(-7.15810199822856,1.06258635413951,
1.38893755060872));
#157898=CARTESIAN_POINT('Ctrl Pts',(-7.19907169867902,1.05593965777816,
1.39649723575846));
#157899=CARTESIAN_POINT('Ctrl Pts',(-7.28100362967791,1.04295320030069,
1.4116629786443));
#157900=CARTESIAN_POINT('Ctrl Pts',(-7.32200977315745,1.03660648775052,
1.41927716981832));
#157901=CARTESIAN_POINT('Ctrl Pts',(-7.36301043220623,1.03040248142752,
1.42691183134996));
#157902=CARTESIAN_POINT('',(-7.33764351829699,0.940053946665902,0.731428772536595));
#157903=CARTESIAN_POINT('Origin',(-5.11743425413158E-13,1.03148891299978,
6.89552581700781E-14));
#157904=CARTESIAN_POINT('',(-7.36370860840547,0.84933050033943,1.42330444080272));
#157905=CARTESIAN_POINT('Origin',(0.191427338004395,0.946426677476739,-0.0211651271497584));
#157906=CARTESIAN_POINT('',(-7.23516979657277,0.94005394801158,1.97542857061911));
#157907=CARTESIAN_POINT('Origin',(0.189246193072801,0.803583945876243,-0.0290873467451794));
#157908=CARTESIAN_POINT('Origin',(0.186285059628298,0.94642927109937,-0.0498074733912154));
#157909=CARTESIAN_POINT('Ctrl Pts',(-7.118065296,1.070162746,1.376824766));
#157910=CARTESIAN_POINT('Ctrl Pts',(-7.0434586,1.005280647,1.762534951));
#157911=CARTESIAN_POINT('Ctrl Pts',(-6.927609792,0.940053947,2.137924827));
#157912=CARTESIAN_POINT('Ctrl Pts',(-6.92362795126682,0.93781203933228,
2.15082735681355));
#157913=CARTESIAN_POINT('Ctrl Pts',(-6.91964611053353,0.935570131664546,
2.16372988662716));
#157914=CARTESIAN_POINT('Ctrl Pts',(-7.40685278759771,1.070162746,1.18164879131978));
#157915=CARTESIAN_POINT('Ctrl Pts',(-7.3428221904726,1.005280647,1.58300764889336));
#157916=CARTESIAN_POINT('Ctrl Pts',(-7.2357965942918,0.940053947,1.97509739841982));
#157917=CARTESIAN_POINT('Ctrl Pts',(-7.23211801627514,0.93781203933228,
1.98857391978146));
#157918=CARTESIAN_POINT('Ctrl Pts',(-7.22843943825845,0.935570131664544,
2.00205044114303));
#157919=CARTESIAN_POINT('',(-7.08138978994764,0.940053949937996,2.0566767108959));
#157920=CARTESIAN_POINT('Ctrl Pts',(-6.927609792,0.940053947,2.137924827));
#157921=CARTESIAN_POINT('Ctrl Pts',(-6.81023984700001,1.005711878,2.518243711));
#157922=CARTESIAN_POINT('Ctrl Pts',(-6.65194247900001,1.070155008,2.883428734));
#157923=CARTESIAN_POINT('Ctrl Pts',(-7.090106059,0.940053947,2.445484832));
#157924=CARTESIAN_POINT('Ctrl Pts',(-6.955851376,1.005711878,2.8347246));
#157925=CARTESIAN_POINT('Ctrl Pts',(-6.779794189,1.070155008,3.206928554));
#157926=CARTESIAN_POINT('',(-7.09010605781718,0.940053946884182,2.44548483938707));
#157927=CARTESIAN_POINT('',(-6.88412347496954,1.03040248139212,2.97638102061096));
#157928=CARTESIAN_POINT('Origin',(0.182258551121615,0.803674002173012,-0.0398174380776881));
#157929=CARTESIAN_POINT('Ctrl Pts',(-6.65381782566217,1.06939092107355,
2.87909853088944));
#157930=CARTESIAN_POINT('Ctrl Pts',(-6.69216903288866,1.06258635444552,
2.89524529923536));
#157931=CARTESIAN_POINT('Ctrl Pts',(-6.73055577275058,1.05593965854339,
2.91143551651327));
#157932=CARTESIAN_POINT('Ctrl Pts',(-6.80731199029965,1.04295320173078,
2.94385963439241));
#157933=CARTESIAN_POINT('Ctrl Pts',(-6.84572259686926,1.03660649073646,
2.96011091445485));
#157934=CARTESIAN_POINT('Ctrl Pts',(-6.88412347535908,1.03040248140959,
2.97638101943679));
#157935=CARTESIAN_POINT('',(-7.00885792486393,0.940053946665902,2.29170483144534));
#157936=CARTESIAN_POINT('Origin',(-1.03866568124111E-12,1.03148891299989,
4.40836603332606E-13));
#157937=CARTESIAN_POINT('',(-6.88558081090655,0.849330499781311,2.97300805498949));
#157938=CARTESIAN_POINT('Origin',(0.182401896620048,0.946426692996323,-0.0618214724555677));
#157939=CARTESIAN_POINT('',(-6.64135679832037,0.940053948011584,3.48459178406726));
#157940=CARTESIAN_POINT('Origin',(0.178568934923994,0.803583974132988,-0.0690897062119694));
#157941=CARTESIAN_POINT('Origin',(0.171222606441985,0.9464292487965,-0.088688748689485));
#157942=CARTESIAN_POINT('Ctrl Pts',(-6.65567225900001,1.070162746,2.874808998));
#157943=CARTESIAN_POINT('Ctrl Pts',(-6.49989353800001,1.005280647,3.235463259));
#157944=CARTESIAN_POINT('Ctrl Pts',(-6.306055484,0.940053947,3.577172659));
#157945=CARTESIAN_POINT('Ctrl Pts',(-6.29939307402217,0.937812039345993,
3.58891755670764));
#157946=CARTESIAN_POINT('Ctrl Pts',(-6.29273066404431,0.935570131691972,
3.60066245441528));
#157947=CARTESIAN_POINT('Ctrl Pts',(-6.97966512496644,1.070162746,2.74627690293544));
#157948=CARTESIAN_POINT('Ctrl Pts',(-6.83085123717913,1.005280647,3.12448752840956));
#157949=CARTESIAN_POINT('Ctrl Pts',(-6.64204013408926,0.940053947,3.48440309746884));
#157950=CARTESIAN_POINT('Ctrl Pts',(-6.63555050549884,0.937812039345993,
3.49677375962209));
#157951=CARTESIAN_POINT('Ctrl Pts',(-6.62906087690843,0.935570131691969,
3.50914442177529));
#157952=CARTESIAN_POINT('',(-6.47370613432616,0.940053949937996,3.53088223240309));
#157953=CARTESIAN_POINT('Ctrl Pts',(-6.306055484,0.940053947,3.577172659));
#157954=CARTESIAN_POINT('Ctrl Pts',(-6.109672265,1.005711878,3.92336883));
#157955=CARTESIAN_POINT('Ctrl Pts',(-5.876571816,1.070155008,4.245986775));
#157956=CARTESIAN_POINT('Ctrl Pts',(-6.398636369,0.940053947,3.912473977));
#157957=CARTESIAN_POINT('Ctrl Pts',(-6.183845441,1.005711878,4.263752746));
#157958=CARTESIAN_POINT('Ctrl Pts',(-5.93189152599999,1.070155008,4.589407688));
#157959=CARTESIAN_POINT('',(-6.39863636626611,0.940053946884198,3.91247398391473));
#157960=CARTESIAN_POINT('',(-6.08334255562739,1.03040248140864,4.38667794022568));
#157961=CARTESIAN_POINT('Origin',(0.169438150914281,0.803673962997426,-0.0780669157412039));
#157962=CARTESIAN_POINT('Ctrl Pts',(-5.87933418335156,1.06939092119007,
4.2421609543172));
#157963=CARTESIAN_POINT('Ctrl Pts',(-5.91331768376038,1.06258635438258,
4.26617459658952));
#157964=CARTESIAN_POINT('Ctrl Pts',(-5.94732654606767,1.05593965826363,
4.29023831069015));
#157965=CARTESIAN_POINT('Ctrl Pts',(-6.01531802142512,1.04295320100036,
4.33840469011669));
#157966=CARTESIAN_POINT('Ctrl Pts',(-6.0493370692213,1.0366064891846,4.36253317257371));
#157967=CARTESIAN_POINT('Ctrl Pts',(-6.08334255628681,1.03040248142303,
4.38667793916132));
#157968=CARTESIAN_POINT('',(-6.35234592546061,0.940053946665902,3.74482331976312));
#157969=CARTESIAN_POINT('Origin',(4.90059381963448E-14,1.03148891299983,
-1.29236898960272E-13));
#157970=CARTESIAN_POINT('',(-6.08549090775791,0.849330500325969,4.38369711683369));
#157971=CARTESIAN_POINT('Origin',(0.164847907881348,0.946426697543599,-0.0995873118847546));
#157972=CARTESIAN_POINT('',(-5.73700133724396,0.94005394801159,4.83081935903908));
#157973=CARTESIAN_POINT('Origin',(0.15954181886888,0.803583967399387,-0.105861446646613));
#157974=CARTESIAN_POINT('Origin',(0.148154021637887,0.94642927363567,-0.123423023477816));
#157975=CARTESIAN_POINT('Ctrl Pts',(-5.882067385,1.070162746,4.238370357));
#157976=CARTESIAN_POINT('Ctrl Pts',(-5.65240067800001,1.005280647,4.557104901));
#157977=CARTESIAN_POINT('Ctrl Pts',(-5.38963703,0.940053947,4.849155874));
#157978=CARTESIAN_POINT('Ctrl Pts',(-5.38060557750435,0.937812039312306,
4.85919396149436));
#157979=CARTESIAN_POINT('Ctrl Pts',(-5.37157412500868,0.935570131624597,
4.86923204898861));
#157980=CARTESIAN_POINT('Ctrl Pts',(-6.22611607790624,1.070162746,4.18249215983857));
#157981=CARTESIAN_POINT('Ctrl Pts',(-5.99947727211045,1.005280647,4.51986984361793));
#157982=CARTESIAN_POINT('Ctrl Pts',(-5.73770925905211,0.940053947,4.83078198081959));
#157983=CARTESIAN_POINT('Ctrl Pts',(-5.72871202753696,0.937812039312306,
4.84146834561484));
#157984=CARTESIAN_POINT('Ctrl Pts',(-5.7197147960219,0.935570131624597,
4.85215471041007));
#157985=CARTESIAN_POINT('',(-5.56331917461025,0.940053949937996,4.83998762566666));
#157986=CARTESIAN_POINT('Ctrl Pts',(-5.38963702999999,0.940053947,4.849155874));
#157987=CARTESIAN_POINT('Ctrl Pts',(-5.123423198,1.005711878,5.145041583));
#157988=CARTESIAN_POINT('Ctrl Pts',(-4.826419186,1.070155008,5.410007194));
#157989=CARTESIAN_POINT('Ctrl Pts',(-5.407973553,0.940053947,5.196520186));
#157990=CARTESIAN_POINT('Ctrl Pts',(-5.122689766,1.005711878,5.493412553));
#157991=CARTESIAN_POINT('Ctrl Pts',(-4.806620207,1.070155008,5.75729121900001));
#157992=CARTESIAN_POINT('',(-5.40797354882796,0.940053946884182,5.19652019220046));
#157993=CARTESIAN_POINT('',(-4.99811129844124,1.03040248142711,5.59185867529939));
#157994=CARTESIAN_POINT('Origin',(0.148694582446472,0.803673986557815,-0.112665824199406));
#157995=CARTESIAN_POINT('Ctrl Pts',(-4.8299394093612,1.06939092113262,5.40686464598623));
#157996=CARTESIAN_POINT('Ctrl Pts',(-4.85796618327951,1.06258635138517,
5.43762232415357));
#157997=CARTESIAN_POINT('Ctrl Pts',(-4.88600696365171,1.05593965225773,
5.46843435718009));
#157998=CARTESIAN_POINT('Ctrl Pts',(-4.94205445198269,1.04295320341478,
5.53009075102171));
#157999=CARTESIAN_POINT('Ctrl Pts',(-4.97009123117722,1.03660649407792,
5.56096819981129));
#158000=CARTESIAN_POINT('Ctrl Pts',(-4.99811129971693,1.0304024814516,5.5918586739572));
#158001=CARTESIAN_POINT('',(-5.39880529010589,0.940053946665902,5.02283803149846));
#158002=CARTESIAN_POINT('Origin',(-2.32019264911898E-13,1.03148891299983,
2.66713734431434E-13));
#158003=CARTESIAN_POINT('',(-5.00085021307736,0.849330499754917,5.58940937371024));
#158004=CARTESIAN_POINT('Origin',(0.139585301709059,0.9464267015393,-0.132696195866576));
#158005=CARTESIAN_POINT('',(-4.56439006760893,0.940053948010712,5.95116319036083));
#158006=CARTESIAN_POINT('Origin',(0.133054720215192,0.803583963958215,-0.137683229263514));
#158007=CARTESIAN_POINT('Origin',(0.118157849674241,0.946429283675318,-0.152386068274454));
#158008=CARTESIAN_POINT('Ctrl Pts',(-4.833423576,1.070162746,5.403750228));
#158009=CARTESIAN_POINT('Ctrl Pts',(-4.540607845,1.005280647,5.665661383));
#158010=CARTESIAN_POINT('Ctrl Pts',(-4.221205138,0.940053947,5.894397949));
#158011=CARTESIAN_POINT('Ctrl Pts',(-4.21022694371415,0.937812039309391,
5.90225985626249));
#158012=CARTESIAN_POINT('Ctrl Pts',(-4.19924874942829,0.935570131618771,
5.91012176352508));
#158013=CARTESIAN_POINT('Ctrl Pts',(-5.18144076305731,1.070162746,5.42313873171225));
#158014=CARTESIAN_POINT('Ctrl Pts',(-4.88757441729678,1.005280647,5.70390806884625));
#158015=CARTESIAN_POINT('Ctrl Pts',(-4.56508947558847,0.940053947,5.9512788675075));
#158016=CARTESIAN_POINT('Ctrl Pts',(-4.55400534177636,0.937812039309391,
5.95978125220506));
#158017=CARTESIAN_POINT('Ctrl Pts',(-4.54292120796426,0.935570131618772,
5.96828363690254));
#158018=CARTESIAN_POINT('',(-4.3927975929503,0.940053949937996,5.9227805762912));
#158019=CARTESIAN_POINT('Ctrl Pts',(-4.221205138,0.940053947,5.894397949));
#158020=CARTESIAN_POINT('Ctrl Pts',(-3.897608556,1.005711878,6.12613791));
#158021=CARTESIAN_POINT('Ctrl Pts',(-3.55058856,1.070155008,6.321061689));
#158022=CARTESIAN_POINT('Ctrl Pts',(-4.164439905,0.940053947,6.237582888));
#158023=CARTESIAN_POINT('Ctrl Pts',(-3.822002811,1.005711878,6.466206494));
#158024=CARTESIAN_POINT('Ctrl Pts',(-3.45659667,1.070155008,6.655970212));
#158025=CARTESIAN_POINT('',(-4.1644398996237,0.940053946884196,6.2375828931164));
#158026=CARTESIAN_POINT('',(-3.67917391284191,1.03040248141186,6.53557031310756));
#158027=CARTESIAN_POINT('Origin',(0.120998550274901,0.803673961062085,-0.141997014740639));
#158028=CARTESIAN_POINT('Ctrl Pts',(-3.55470203693565,1.06939092122075,
6.31874935624554));
#158029=CARTESIAN_POINT('Ctrl Pts',(-3.5754615686637,1.06258635149433,6.35481286461373));
#158030=CARTESIAN_POINT('Ctrl Pts',(-3.59622309476572,1.05593965237264,
6.39093246815098));
#158031=CARTESIAN_POINT('Ctrl Pts',(-3.63770592193111,1.0429532034737,6.46319592317457));
#158032=CARTESIAN_POINT('Ctrl Pts',(-3.65844947780599,1.03660649420318,
6.49937855271611));
#158033=CARTESIAN_POINT('Ctrl Pts',(-3.67917391437289,1.03040248143664,
6.53557031207056));
#158034=CARTESIAN_POINT('',(-4.19282251981636,0.940053946665902,6.06599041966374));
#158035=CARTESIAN_POINT('Origin',(1.95373231481888E-13,1.03148891300056,
-4.58400678526871E-13));
#158036=CARTESIAN_POINT('',(-3.68237532060303,0.849330499766696,6.53376706031241));
#158037=CARTESIAN_POINT('Origin',(0.107796101383926,0.946426683836144,-0.159600559127751));
#158038=CARTESIAN_POINT('',(-3.17835299299454,0.940053948010695,6.79323724514997));
#158039=CARTESIAN_POINT('Origin',(0.100346144483314,0.80358391676753,-0.163067062224314));
#158040=CARTESIAN_POINT('Origin',(0.0826369660285103,0.94642931938388,-0.174223943159391));
#158041=CARTESIAN_POINT('Ctrl Pts',(-3.558774254,1.070162746,6.316456745));
#158042=CARTESIAN_POINT('Ctrl Pts',(-3.216501235,1.005280647,6.509297835));
#158043=CARTESIAN_POINT('Ctrl Pts',(-2.855394386,0.940053947,6.664024527));
#158044=CARTESIAN_POINT('Ctrl Pts',(-2.84298277861454,0.937812039393734,
6.66934263979257));
#158045=CARTESIAN_POINT('Ctrl Pts',(-2.83057117122915,0.935570131787453,
6.67466075258513));
#158046=CARTESIAN_POINT('Ctrl Pts',(-3.89448703709711,1.070162746,6.41020536373886));
#158047=CARTESIAN_POINT('Ctrl Pts',(-3.54713401528997,1.005280647,6.62123789183456));
#158048=CARTESIAN_POINT('Ctrl Pts',(-3.17901118204665,0.940053947,6.79350056985927));
#158049=CARTESIAN_POINT('Ctrl Pts',(-3.16635842819142,0.937812039393734,
6.79942141221586));
#158050=CARTESIAN_POINT('Ctrl Pts',(-3.15370567433618,0.935570131787455,
6.80534225457233));
#158051=CARTESIAN_POINT('',(-3.01687367847068,0.940053949937996,6.72863089041115));
#158052=CARTESIAN_POINT('Ctrl Pts',(-2.855394386,0.940053947,6.664024527));
#158053=CARTESIAN_POINT('Ctrl Pts',(-2.489546071,1.005711878,6.82078283800001));
#158054=CARTESIAN_POINT('Ctrl Pts',(-2.108736358,1.070155008,6.936550365));
#158055=CARTESIAN_POINT('Ctrl Pts',(-2.726181675,0.940053947,6.986983146));
#158056=CARTESIAN_POINT('Ctrl Pts',(-2.342603253,1.005711878,7.136647807));
#158057=CARTESIAN_POINT('Ctrl Pts',(-1.944946514,1.070155008,7.243423435));
#158058=CARTESIAN_POINT('',(-2.72618166865117,0.940053946884198,6.98698314983959));
#158059=CARTESIAN_POINT('',(-2.18820244488194,1.03040248138689,7.17368594663709));
#158060=CARTESIAN_POINT('Origin',(0.087644423473624,0.803673967492884,-0.16468805624954));
#158061=CARTESIAN_POINT('Ctrl Pts',(-2.11325074753863,1.06939092118773,
6.93517636918274));
#158062=CARTESIAN_POINT('Ctrl Pts',(-2.12577234001398,1.06258635408308,
6.97485940334765));
#158063=CARTESIAN_POINT('Ctrl Pts',(-2.13828382082693,1.05593965766241,
7.01459764785347));
#158064=CARTESIAN_POINT('Ctrl Pts',(-2.16326231440692,1.04295319922269,
7.09408926356511));
#158065=CARTESIAN_POINT('Ctrl Pts',(-2.17574271090272,1.03660648558926,
7.13388524388851));
#158066=CARTESIAN_POINT('Ctrl Pts',(-2.18820244610799,1.03040248139184,
7.1736859462382));
#158067=CARTESIAN_POINT('',(-2.79078802860556,0.940053946665902,6.8255038372746));
#158068=CARTESIAN_POINT('Origin',(-4.74880551548651E-14,1.03148891299972,
3.08780778723872E-13));
#158069=CARTESIAN_POINT('',(-2.19171665066048,0.849330499771342,7.17261306109147));
#158070=CARTESIAN_POINT('Origin',(0.0709664804794227,0.946426656566132,
-0.179042142893574));
#158071=CARTESIAN_POINT('',(-1.64369966596779,0.940053948010708,7.31766707464516));
#158072=CARTESIAN_POINT('Origin',(0.0629454791960926,0.803583969908237,
-0.180826038645768));
#158073=CARTESIAN_POINT('Origin',(0.0432520105150996,0.94642927386581,-0.187915429956872));
#158074=CARTESIAN_POINT('Ctrl Pts',(-2.117720602,1.070162746,6.933812764));
#158075=CARTESIAN_POINT('Ctrl Pts',(-1.741994603,1.005280647,7.048566756));
#158076=CARTESIAN_POINT('Ctrl Pts',(-1.356068566,0.940053947,7.122048725));
#158077=CARTESIAN_POINT('Ctrl Pts',(-1.34280389759946,0.937812039319745,
7.12457437462911));
#158078=CARTESIAN_POINT('Ctrl Pts',(-1.32953922919893,0.935570131639477,
7.12710002425809));
#158079=CARTESIAN_POINT('Ctrl Pts',(-2.42543142519539,1.070162746,7.0975379173685));
#158080=CARTESIAN_POINT('Ctrl Pts',(-2.04083356844032,1.005280647,7.2289659894335));
#158081=CARTESIAN_POINT('Ctrl Pts',(-1.64428585988024,0.940053947,7.31806573416641));
#158082=CARTESIAN_POINT('Ctrl Pts',(-1.63065611388038,0.937812039319745,
7.32112818255068));
#158083=CARTESIAN_POINT('Ctrl Pts',(-1.61702636788052,0.935570131639477,
7.32419063093486));
#158084=CARTESIAN_POINT('',(-1.49988410426394,0.940053949937996,7.21985790168456));
#158085=CARTESIAN_POINT('Ctrl Pts',(-1.356068566,0.940053947,7.122048725));
#158086=CARTESIAN_POINT('Ctrl Pts',(-0.965075178000001,1.005711878,7.19649554));
#158087=CARTESIAN_POINT('Ctrl Pts',(-0.568281989,1.070155008,7.227693656));
#158088=CARTESIAN_POINT('Ctrl Pts',(-1.16045022,0.940053947,7.409679837));
#158089=CARTESIAN_POINT('Ctrl Pts',(-0.75366617,1.005711878,7.473387399));
#158090=CARTESIAN_POINT('Ctrl Pts',(-0.342352821,1.070155008,7.49218222900001));
#158091=CARTESIAN_POINT('',(-1.16045021294829,0.940053946884191,7.40967983939926));
#158092=CARTESIAN_POINT('',(-0.594913062081684,1.03040248135913,7.4763679983408));
#158093=CARTESIAN_POINT('Origin',(0.0501923127855627,0.803673966063474,
-0.179678925408648));
#158094=CARTESIAN_POINT('Ctrl Pts',(-0.572986203044213,1.06939092119402,
7.22732224375387));
#158095=CARTESIAN_POINT('Ctrl Pts',(-0.576684369626288,1.06258635141026,
7.26876929900361));
#158096=CARTESIAN_POINT('Ctrl Pts',(-0.580360792552439,1.05593965225368,
7.31026810206519));
#158097=CARTESIAN_POINT('Ctrl Pts',(-0.587666952126212,1.04295319907133,
7.39327085176534));
#158098=CARTESIAN_POINT('Ctrl Pts',(-0.591300604526767,1.0366064853031,
7.43481934128274));
#158099=CARTESIAN_POINT('Ctrl Pts',(-0.59491306336725,1.03040248136352,
7.47636799821832));
#158100=CARTESIAN_POINT('',(-1.25825939098333,0.940053946665902,7.26586428134924));
#158101=CARTESIAN_POINT('Origin',(2.16764201531848E-13,1.03148891300033,
-1.72735090120391E-12));
#158102=CARTESIAN_POINT('',(-0.598575745926003,0.849330499809727,7.4760756466581));
#158103=CARTESIAN_POINT('Origin',(0.0308185621203441,0.946426654691962,
-0.190111958654687));
#158104=CARTESIAN_POINT('',(-0.0321887715705101,0.940053948012013,7.49993092670776));
#158105=CARTESIAN_POINT('Origin',(0.0226016159826436,0.803583929116596,
-0.190129976591281));
#158106=CARTESIAN_POINT('Origin',(0.00184455323367208,0.946429300663522,
-0.192820044683663));
#158107=CARTESIAN_POINT('Ctrl Pts',(-0.577644689000001,1.070162746,7.226951405));
#158108=CARTESIAN_POINT('Ctrl Pts',(-0.186034238,1.005280647,7.25825252900001));
#158109=CARTESIAN_POINT('Ctrl Pts',(0.206665513,0.940053947,7.24705384));
#158110=CARTESIAN_POINT('Ctrl Pts',(0.220163000300406,0.937812039403535,
7.24666892974179));
#158111=CARTESIAN_POINT('Ctrl Pts',(0.233660487600805,0.935570131807057,
7.24628401948363));
#158112=CARTESIAN_POINT('Ctrl Pts',(-0.842965336257744,1.070162746,7.45299748588597));
#158113=CARTESIAN_POINT('Ctrl Pts',(-0.439106013265268,1.005280647,7.4986756722331));
#158114=CARTESIAN_POINT('Ctrl Pts',(-0.0326755574926569,0.940053947,7.50044627943826));
#158115=CARTESIAN_POINT('Ctrl Pts',(-0.0187061319931008,0.937812039403535,
7.50050713699725));
#158116=CARTESIAN_POINT('Ctrl Pts',(-0.00473670649354516,0.935570131807057,
7.50056799455627));
#158117=CARTESIAN_POINT('',(0.0872383841134713,0.940053949937996,7.37349238228569));
#158118=CARTESIAN_POINT('Ctrl Pts',(-0.575145653352384,4.94745154526473,
7.22714282422102));
#158119=CARTESIAN_POINT('Ctrl Pts',(-0.57356878941999,4.94771235963237,
7.22726762074545));
#158120=CARTESIAN_POINT('Ctrl Pts',(-0.571991925487597,4.947973174,7.22739241726988));
#158121=CARTESIAN_POINT('Ctrl Pts',(-0.414102629595647,4.97408817100001,
7.23988812788054));
#158122=CARTESIAN_POINT('Ctrl Pts',(-0.255818264017313,5.00031307,7.24547672211003));
#158123=CARTESIAN_POINT('Ctrl Pts',(-0.527285648139283,4.94745154526473,
7.28327884871706));
#158124=CARTESIAN_POINT('Ctrl Pts',(-0.525696541069641,4.94771235963237,
7.28339319785853));
#158125=CARTESIAN_POINT('Ctrl Pts',(-0.524107434,4.947973174,7.28350754700001));
#158126=CARTESIAN_POINT('Ctrl Pts',(-0.364992249,4.97408817100001,7.294957175));
#158127=CARTESIAN_POINT('Ctrl Pts',(-0.205528848,5.00031307,7.299447149));
#158128=CARTESIAN_POINT('Origin',(-0.0077921681403096,5.08925695568899,
-0.196936015308897));
#158129=CARTESIAN_POINT('',(-0.500739504532107,4.94797317561532,7.31089209031288));
#158130=CARTESIAN_POINT('Ctrl Pts',(-0.622179465,4.94766207,7.268458786));
#158131=CARTESIAN_POINT('Ctrl Pts',(-0.462446769,4.973931887,7.282131892));
#158132=CARTESIAN_POINT('Ctrl Pts',(-0.30226761,5.00031307,7.288774568));
#158133=CARTESIAN_POINT('Ctrl Pts',(-0.573864989,4.94766207,7.227252519));
#158134=CARTESIAN_POINT('Ctrl Pts',(-0.415037848,4.973931887,7.239863859));
#158135=CARTESIAN_POINT('Ctrl Pts',(-0.255810014,5.00031307,7.24548557600001));
#158136=CARTESIAN_POINT('Ctrl Pts',(-0.571982121404791,4.94797287213543,
7.22740188220303));
#158137=CARTESIAN_POINT('Ctrl Pts',(-0.572436165542444,4.94882769742138,
7.23260489888446));
#158138=CARTESIAN_POINT('Ctrl Pts',(-0.572889190404426,4.94967947054502,
7.23780850677221));
#158139=CARTESIAN_POINT('Ctrl Pts',(-0.573343134511853,4.9505285274177,
7.24301247656969));
#158140=CARTESIAN_POINT('Ctrl Pts',(-0.573764558557747,4.95131675878061,
7.24784363963775));
#158141=CARTESIAN_POINT('Ctrl Pts',(-0.574186775096978,4.95210264917475,
7.25267511613723));
#158142=CARTESIAN_POINT('Ctrl Pts',(-0.574609775307212,4.95288622030903,
7.25750689950655));
#158143=CARTESIAN_POINT('Ctrl Pts',(-0.575032775944805,4.95366979223496,
7.26233868775745));
#158144=CARTESIAN_POINT('Ctrl Pts',(-0.575456560362438,4.95445104509375,
7.26717078409749));
#158145=CARTESIAN_POINT('Ctrl Pts',(-0.575881119919221,4.95523000034009,
7.27200318231908));
#158146=CARTESIAN_POINT('Ctrl Pts',(-0.853730891,5.000313899,7.244911592));
#158147=CARTESIAN_POINT('Ctrl Pts',(-0.742882782,4.98224132,7.257973788));
#158148=CARTESIAN_POINT('Ctrl Pts',(-0.631686945,4.964285714,7.267638682));
#158149=CARTESIAN_POINT('Ctrl Pts',(-0.580289944,4.955986264,7.27210599500001));
#158150=CARTESIAN_POINT('Ctrl Pts',(-0.528834902,4.947660853,7.275845934));
#158151=CARTESIAN_POINT('Ctrl Pts',(-0.892761299,5.000313899,7.194822949));
#158152=CARTESIAN_POINT('Ctrl Pts',(-0.782679553,4.98224132,7.20848231500001));
#158153=CARTESIAN_POINT('Ctrl Pts',(-0.672231452,4.964285714,7.218767545));
#158154=CARTESIAN_POINT('Ctrl Pts',(-0.621180069,4.955986264,7.22352159));
#158155=CARTESIAN_POINT('Ctrl Pts',(-0.570066555,4.947660853,7.227553121));
#158156=CARTESIAN_POINT('Ctrl Pts',(-0.571983137701933,4.94797303766448,
7.22740180177));
#158157=CARTESIAN_POINT('Ctrl Pts',(-0.605444395477702,4.95342302831041,
7.22475356782426));
#158158=CARTESIAN_POINT('Ctrl Pts',(-0.638862058334151,4.95886083424197,
7.22187499458713));
#158159=CARTESIAN_POINT('Ctrl Pts',(-0.672231451656842,4.96428571396197,
7.21876754515345));
#158160=CARTESIAN_POINT('Ctrl Pts',(-0.745099376405782,4.97613189093767,
7.21198188447502));
#158161=CARTESIAN_POINT('Ctrl Pts',(-0.817988928543339,4.98803923900258,
7.20408107381268));
#158162=CARTESIAN_POINT('Ctrl Pts',(-0.890849230764476,5.00000000015126,
7.19505994779791));
#158163=CARTESIAN_POINT('Ctrl Pts',(-0.892761299,5.000313899,7.194822949));
#158164=CARTESIAN_POINT('Ctrl Pts',(-0.782679553,4.98224132,7.20848231500001));
#158165=CARTESIAN_POINT('Ctrl Pts',(-0.672231452,4.964285714,7.218767545));
#158166=CARTESIAN_POINT('Ctrl Pts',(-0.622137718,4.95614194999999,7.223432411));
#158167=CARTESIAN_POINT('Ctrl Pts',(-0.57198407,4.947973174,7.227401623));
#158168=CARTESIAN_POINT('Ctrl Pts',(-0.950940418,5.000313899,7.240157672));
#158169=CARTESIAN_POINT('Ctrl Pts',(-0.840165045,4.98224132,7.254707187));
#158170=CARTESIAN_POINT('Ctrl Pts',(-0.728996408,4.964285714,7.265860928));
#158171=CARTESIAN_POINT('Ctrl Pts',(-0.678575876,4.95614194999999,7.270919708));
#158172=CARTESIAN_POINT('Ctrl Pts',(-0.628089994,4.947973174,7.27527826));
#158173=CARTESIAN_POINT('',(-0.655474541515816,4.94797317334227,7.29864619863935));
#158174=CARTESIAN_POINT('Ctrl Pts',(-1.537156899,4.81863040500001,7.245585413));
#158175=CARTESIAN_POINT('Ctrl Pts',(-1.528521258,4.820029867,7.247417471));
#158176=CARTESIAN_POINT('Ctrl Pts',(-1.519881274,4.821428571,7.24922894));
#158177=CARTESIAN_POINT('Ctrl Pts',(-1.132645864,4.884117105,7.33041714000001));
#158178=CARTESIAN_POINT('Ctrl Pts',(-0.738965005000001,4.947973174,7.369890775));
#158179=CARTESIAN_POINT('Ctrl Pts',(-1.355651883,4.81863040500001,7.12212805100001));
#158180=CARTESIAN_POINT('Ctrl Pts',(-1.347163385,4.820029867,7.12374378300001));
#158181=CARTESIAN_POINT('Ctrl Pts',(-1.338671059,4.821428571,7.125339276));
#158182=CARTESIAN_POINT('Ctrl Pts',(-0.95805352,4.884117105,7.196847686));
#158183=CARTESIAN_POINT('Ctrl Pts',(-0.57198407,4.947973174,7.227401623));
#158184=CARTESIAN_POINT('Ctrl Pts',(-1.35103832261869,4.81939091791739,
7.12300468506627));
#158185=CARTESIAN_POINT('Ctrl Pts',(-1.35423171894372,4.82234724740109,
7.14079909641026));
#158186=CARTESIAN_POINT('Ctrl Pts',(-1.3574262227148,4.82527010320382,7.15859892100757));
#158187=CARTESIAN_POINT('Ctrl Pts',(-1.36063744721484,4.82816321756001,
7.17640053315189));
#158188=CARTESIAN_POINT('Ctrl Pts',(-1.36364364406067,4.83087161470014,
7.19306556241983));
#158189=CARTESIAN_POINT('Ctrl Pts',(-1.36666047782763,4.83355328556713,
7.20973303985136));
#158190=CARTESIAN_POINT('Ctrl Pts',(-1.36968750153964,4.83620904390085,
7.22640277020807));
#158191=CARTESIAN_POINT('Ctrl Pts',(-1.37271455775148,4.83886483074828,
7.24307267954037));
#158192=CARTESIAN_POINT('Ctrl Pts',(-1.37575181232463,4.84149471141675,
7.25974488617966));
#158193=CARTESIAN_POINT('Ctrl Pts',(-1.37879884640616,4.84409946429526,
7.27641920768044));
#158194=CARTESIAN_POINT('Ctrl Pts',(-2.01675012375466,4.94924836941368,
7.12700095619442));
#158195=CARTESIAN_POINT('Ctrl Pts',(-2.01288868187733,4.94861077170684,
7.12808912409721));
#158196=CARTESIAN_POINT('Ctrl Pts',(-2.00902724,4.94797317400001,7.129177292));
#158197=CARTESIAN_POINT('Ctrl Pts',(-1.620660636,4.88384644,7.238620367));
#158198=CARTESIAN_POINT('Ctrl Pts',(-1.222703557,4.818610636,7.30522794400001));
#158199=CARTESIAN_POINT('Ctrl Pts',(-2.11980215310686,4.94924836941368,
6.93318112482194));
#158200=CARTESIAN_POINT('Ctrl Pts',(-2.11604563105343,4.94861077170684,
6.93432522341097));
#158201=CARTESIAN_POINT('Ctrl Pts',(-2.112289109,4.94797317400001,6.935469322));
#158202=CARTESIAN_POINT('Ctrl Pts',(-1.734474873,4.88384644,7.050537656));
#158203=CARTESIAN_POINT('Ctrl Pts',(-1.346396652,4.818610636,7.123883495));
#158204=CARTESIAN_POINT('',(-2.09494101683223,4.94797317334255,6.96801245134783));
#158205=CARTESIAN_POINT('Ctrl Pts',(-2.1153154539966,4.94745154526473,6.93454760851299));
#158206=CARTESIAN_POINT('Ctrl Pts',(-2.1138022814983,4.94771235963237,6.93500846525649));
#158207=CARTESIAN_POINT('Ctrl Pts',(-2.112289109,4.947973174,6.935469322));
#158208=CARTESIAN_POINT('Ctrl Pts',(-1.960777152,4.974088171,6.981614297));
#158209=CARTESIAN_POINT('Ctrl Pts',(-1.807394542,5.00031307,7.021098559));
#158210=CARTESIAN_POINT('Ctrl Pts',(-2.0806476628918,4.94745154526474,6.99964900947169));
#158211=CARTESIAN_POINT('Ctrl Pts',(-2.0791202899459,4.94771235963237,7.00010229623584));
#158212=CARTESIAN_POINT('Ctrl Pts',(-2.077592917,4.947973174,7.00055558299999));
#158213=CARTESIAN_POINT('Ctrl Pts',(-1.924659088,4.974088171,7.04594258599999));
#158214=CARTESIAN_POINT('Ctrl Pts',(-1.769889065,5.00031307,7.084607504));
#158215=CARTESIAN_POINT('Origin',(0.0347258367496797,5.08925692701997,-0.194008213182874));
#158216=CARTESIAN_POINT('Ctrl Pts',(-2.17013704,4.94766207,6.964776065));
#158217=CARTESIAN_POINT('Ctrl Pts',(-2.017078119,4.973931887,7.012467309));
#158218=CARTESIAN_POINT('Ctrl Pts',(-1.862071839,5.00031307,7.053388468));
#158219=CARTESIAN_POINT('Ctrl Pts',(-2.114094,4.94766207,6.934919362));
#158220=CARTESIAN_POINT('Ctrl Pts',(-1.961691214,4.973931887,6.981378996));
#158221=CARTESIAN_POINT('Ctrl Pts',(-1.807394542,5.00031307,7.021098559));
#158222=CARTESIAN_POINT('Ctrl Pts',(-2.11228726159542,4.94797287202588,
6.93546999405279));
#158223=CARTESIAN_POINT('Ctrl Pts',(-2.11384918555808,4.94882769739943,
6.94045376112391));
#158224=CARTESIAN_POINT('Ctrl Pts',(-2.11541024084986,4.94967947054799,
6.94543832469033));
#158225=CARTESIAN_POINT('Ctrl Pts',(-2.11697227168855,4.95052852744352,
6.95042304407898));
#158226=CARTESIAN_POINT('Ctrl Pts',(-2.11842240029988,4.9513167588064,6.95505066347414));
#158227=CARTESIAN_POINT('Ctrl Pts',(-2.11987337024825,4.95210264919842,
6.95967841859454));
#158228=CARTESIAN_POINT('Ctrl Pts',(-2.12132517151473,4.95288622033075,
6.96430630494391));
#158229=CARTESIAN_POINT('Ctrl Pts',(-2.12277697424796,4.95366979225473,
6.96893419596886));
#158230=CARTESIAN_POINT('Ctrl Pts',(-2.12422960866792,4.95445104511177,
6.97356221939012));
#158231=CARTESIAN_POINT('Ctrl Pts',(-2.12568306502001,4.95523000036473,
6.97819037105365));
#158232=CARTESIAN_POINT('Ctrl Pts',(-2.391212971,5.000313899,6.89200268));
#158233=CARTESIAN_POINT('Ctrl Pts',(-2.285764415,4.98224132,6.928588556));
#158234=CARTESIAN_POINT('Ctrl Pts',(-2.179245942,4.964285714,6.961931308));
#158235=CARTESIAN_POINT('Ctrl Pts',(-2.130010915,4.955986264,6.977343013));
#158236=CARTESIAN_POINT('Ctrl Pts',(-2.080562839,4.947660853,6.992056828));
#158237=CARTESIAN_POINT('Ctrl Pts',(-2.418563293,5.000313899,6.834694697));
#158238=CARTESIAN_POINT('Ctrl Pts',(-2.313991557,4.98224132,6.871699036));
#158239=CARTESIAN_POINT('Ctrl Pts',(-2.208336691,4.964285714,6.905486881));
#158240=CARTESIAN_POINT('Ctrl Pts',(-2.159500841,4.955986264,6.921104317));
#158241=CARTESIAN_POINT('Ctrl Pts',(-2.110448992,4.947660853,6.936029488));
#158242=CARTESIAN_POINT('Ctrl Pts',(-2.112289109,4.947973174,6.93546932199999));
#158243=CARTESIAN_POINT('Ctrl Pts',(-2.14439727935191,4.9534229210678,6.92569035367246));
#158244=CARTESIAN_POINT('Ctrl Pts',(-2.17641514247988,4.95886077964643,
6.91569521664372));
#158245=CARTESIAN_POINT('Ctrl Pts',(-2.20833669130953,4.9642857140526,6.90548688090102));
#158246=CARTESIAN_POINT('Ctrl Pts',(-2.27804228996723,4.97613189126059,
6.88319541385734));
#158247=CARTESIAN_POINT('Ctrl Pts',(-2.34752928232983,4.98803923902554,
6.85981022134622));
#158248=CARTESIAN_POINT('Ctrl Pts',(-2.41674687579387,5.00000000018585,
6.83533719297713));
#158249=CARTESIAN_POINT('Ctrl Pts',(-2.418563293,5.000313899,6.834694697));
#158250=CARTESIAN_POINT('Ctrl Pts',(-2.313991557,4.98224132,6.871699036));
#158251=CARTESIAN_POINT('Ctrl Pts',(-2.208336691,4.964285714,6.905486881));
#158252=CARTESIAN_POINT('Ctrl Pts',(-2.16041693,4.95614194999999,6.920811357));
#158253=CARTESIAN_POINT('Ctrl Pts',(-2.112289109,4.947973174,6.93546932199999));
#158254=CARTESIAN_POINT('Ctrl Pts',(-2.485127842,5.000313899,6.866462729));
#158255=CARTESIAN_POINT('Ctrl Pts',(-2.380070051,4.98224132,6.904485514));
#158256=CARTESIAN_POINT('Ctrl Pts',(-2.2738982,4.964285714,6.939276459));
#158257=CARTESIAN_POINT('Ctrl Pts',(-2.22574396,4.95614194999999,6.95505589100001));
#158258=CARTESIAN_POINT('Ctrl Pts',(-2.177375369,4.947973174,6.970165514));
#158259=CARTESIAN_POINT('',(-2.20914309734462,4.94797317334223,6.98710025528443));
#158260=CARTESIAN_POINT('Ctrl Pts',(-3.058805711,4.81863040500001,6.745744357));
#158261=CARTESIAN_POINT('Ctrl Pts',(-3.050765805,4.820029867,6.749389991));
#158262=CARTESIAN_POINT('Ctrl Pts',(-3.042717231,4.821428571,6.753016449));
#158263=CARTESIAN_POINT('Ctrl Pts',(-2.681988233,4.884117105,6.915550681));
#158264=CARTESIAN_POINT('Ctrl Pts',(-2.305997078,4.947973174,7.03873119100001));
#158265=CARTESIAN_POINT('Ctrl Pts',(-2.855004498,4.81863040500001,6.664191573));
#158266=CARTESIAN_POINT('Ctrl Pts',(-2.84706179,4.820029867,6.667594306));
#158267=CARTESIAN_POINT('Ctrl Pts',(-2.839110994,4.821428571,6.670978097));
#158268=CARTESIAN_POINT('Ctrl Pts',(-2.482764276,4.884117105,6.82263620000001));
#158269=CARTESIAN_POINT('Ctrl Pts',(-2.112289109,4.947973174,6.935469322));
#158270=CARTESIAN_POINT('Ctrl Pts',(-2.85068725011375,4.81939091791738,
6.66603949042913));
#158271=CARTESIAN_POINT('Ctrl Pts',(-2.85763125915416,4.82234724729619,
6.68273139310464));
#158272=CARTESIAN_POINT('Ctrl Pts',(-2.8645775133876,4.82527010313846,6.69942834382324));
#158273=CARTESIAN_POINT('Ctrl Pts',(-2.87154048165056,4.8281632175241,6.71612344585626));
#158274=CARTESIAN_POINT('Ctrl Pts',(-2.87805888394757,4.83087161468242,
6.73175261251785));
#158275=CARTESIAN_POINT('Ctrl Pts',(-2.88458820076314,4.83355328556657,
6.74738188348297));
#158276=CARTESIAN_POINT('Ctrl Pts',(-2.8911279536013,4.83620904391647,6.76301116416415));
#158277=CARTESIAN_POINT('Ctrl Pts',(-2.89766777665392,4.8388648307801,6.77864061265008));
#158278=CARTESIAN_POINT('Ctrl Pts',(-2.90421805348943,4.8414947114638,6.79427011238702));
#158279=CARTESIAN_POINT('Ctrl Pts',(-2.91077833579864,4.84409946434516,
6.80989957516688));
#158280=CARTESIAN_POINT('Ctrl Pts',(-3.50169415916581,4.94924836941368,
6.52683397198676));
#158281=CARTESIAN_POINT('Ctrl Pts',(-3.49815691958291,4.94861077170685,
6.52872679499338));
#158282=CARTESIAN_POINT('Ctrl Pts',(-3.49461968,4.947973174,6.530619618));
#158283=CARTESIAN_POINT('Ctrl Pts',(-3.138859897,4.88384644,6.72099131500001));
#158284=CARTESIAN_POINT('Ctrl Pts',(-2.764525494,4.818610636,6.871590653));
#158285=CARTESIAN_POINT('Ctrl Pts',(-3.56067135454208,4.94924836941368,
6.31539240121984));
#158286=CARTESIAN_POINT('Ctrl Pts',(-3.55724860527104,4.94861077170685,
6.31731729260992));
#158287=CARTESIAN_POINT('Ctrl Pts',(-3.553825856,4.947973174,6.319242184));
#158288=CARTESIAN_POINT('Ctrl Pts',(-3.209580998,4.88384644,6.51283917600001));
#158289=CARTESIAN_POINT('Ctrl Pts',(-2.846343018,4.818610636,6.66789557700001));
#158290=CARTESIAN_POINT('',(-3.54387916349532,4.94797317334249,6.35475380005075));
#158291=CARTESIAN_POINT('Ctrl Pts',(-3.55658330557724,4.94745154526473,
6.31769144495039));
#158292=CARTESIAN_POINT('Ctrl Pts',(-3.55520458078862,4.94771235963237,
6.31846681447519));
#158293=CARTESIAN_POINT('Ctrl Pts',(-3.553825856,4.947973174,6.319242184));
#158294=CARTESIAN_POINT('Ctrl Pts',(-3.41577597,4.97408817100001,6.396878907));
#158295=CARTESIAN_POINT('Ctrl Pts',(-3.27446731,5.00031307,6.468412776));
#158296=CARTESIAN_POINT('Ctrl Pts',(-3.53672090509896,4.94745154526473,
6.38872336160057));
#158297=CARTESIAN_POINT('Ctrl Pts',(-3.53532668454948,4.94771235963237,
6.38949439080029));
#158298=CARTESIAN_POINT('Ctrl Pts',(-3.533932464,4.947973174,6.39026542));
#158299=CARTESIAN_POINT('Ctrl Pts',(-3.394331008,4.97408817100001,6.467467552));
#158300=CARTESIAN_POINT('Ctrl Pts',(-3.251491236,5.00031307,6.538499487));
#158301=CARTESIAN_POINT('Origin',(0.075620165187994,5.08925701702758,-0.182007724103123));
#158302=CARTESIAN_POINT('Ctrl Pts',(-3.616621419,4.94766207,6.33542815600001));
#158303=CARTESIAN_POINT('Ctrl Pts',(-3.477393138,4.973931887,6.414907549));
#158304=CARTESIAN_POINT('Ctrl Pts',(-3.334807658,5.00031307,6.488193762));
#158305=CARTESIAN_POINT('Ctrl Pts',(-3.555470326,4.94766207,6.318317083));
#158306=CARTESIAN_POINT('Ctrl Pts',(-3.41661808,4.973931887,6.39645261100001));
#158307=CARTESIAN_POINT('Ctrl Pts',(-3.27446731,5.00031307,6.468412776));
#158308=CARTESIAN_POINT('Ctrl Pts',(-3.55382419701178,4.94797287199161,
6.31924323720788));
#158309=CARTESIAN_POINT('Ctrl Pts',(-3.55642096691804,4.94882769743475,
6.32377471888897));
#158310=CARTESIAN_POINT('Ctrl Pts',(-3.55901705931681,4.94967947057971,
6.32830716537846));
#158311=CARTESIAN_POINT('Ctrl Pts',(-3.56161413796261,4.95052852746963,
6.33283955432302));
#158312=CARTESIAN_POINT('Ctrl Pts',(-3.56402516469487,4.95131675883958,
6.33704724781126));
#158313=CARTESIAN_POINT('Ctrl Pts',(-3.56643704228009,4.95210264923673,
6.34125489297957));
#158314=CARTESIAN_POINT('Ctrl Pts',(-3.56884975996899,4.95288622037288,
6.34546248759392));
#158315=CARTESIAN_POINT('Ctrl Pts',(-3.57126248009547,4.95366979230068,
6.34967008645925));
#158316=CARTESIAN_POINT('Ctrl Pts',(-3.57367604093657,4.95445104516023,
6.35387763583144));
#158317=CARTESIAN_POINT('Ctrl Pts',(-3.57609043208675,4.9552300004188,6.35808513377476));
#158318=CARTESIAN_POINT('Ctrl Pts',(-3.816884591,5.000313899,6.216831382));
#158319=CARTESIAN_POINT('Ctrl Pts',(-3.721766245,4.98224132,6.275230223));
#158320=CARTESIAN_POINT('Ctrl Pts',(-3.624905821,4.964285714,6.330691763));
#158321=CARTESIAN_POINT('Ctrl Pts',(-3.580134942,4.955986264,6.356327227));
#158322=CARTESIAN_POINT('Ctrl Pts',(-3.53500597,4.947660853,6.381326915));
#158323=CARTESIAN_POINT('Ctrl Pts',(-3.831275955,5.000313899,6.154983717));
#158324=CARTESIAN_POINT('Ctrl Pts',(-3.737103887,4.98224132,6.213602748));
#158325=CARTESIAN_POINT('Ctrl Pts',(-3.641182561,4.964285714,6.269313324));
#158326=CARTESIAN_POINT('Ctrl Pts',(-3.596845753,4.955986264,6.295063898));
#158327=CARTESIAN_POINT('Ctrl Pts',(-3.55214918,4.947660853,6.320184824));
#158328=CARTESIAN_POINT('Ctrl Pts',(-3.55382585665352,4.9479731737983,6.31924218509526));
#158329=CARTESIAN_POINT('Ctrl Pts',(-3.60037619299507,4.95664467837811,
6.29306313140172));
#158330=CARTESIAN_POINT('Ctrl Pts',(-3.64659716777283,4.9652738833346,6.26639280945056));
#158331=CARTESIAN_POINT('Ctrl Pts',(-3.7385464658405,4.98260085400305,6.21197461326868));
#158332=CARTESIAN_POINT('Ctrl Pts',(-3.7842501153838,4.99129109054103,6.18423872841419));
#158333=CARTESIAN_POINT('Ctrl Pts',(-3.82964012287192,5.00000000030332,
6.15600166741685));
#158334=CARTESIAN_POINT('Ctrl Pts',(-3.831275955,5.000313899,6.154983717));
#158335=CARTESIAN_POINT('Ctrl Pts',(-3.737103887,4.98224132,6.213602748));
#158336=CARTESIAN_POINT('Ctrl Pts',(-3.641182561,4.964285714,6.269313324));
#158337=CARTESIAN_POINT('Ctrl Pts',(-3.597677446,4.95614194999999,6.294580855));
#158338=CARTESIAN_POINT('Ctrl Pts',(-3.553825856,4.947973174,6.319242184));
#158339=CARTESIAN_POINT('Ctrl Pts',(-3.903113449,5.000313899,6.17169962));
#158340=CARTESIAN_POINT('Ctrl Pts',(-3.808685626,4.98224132,6.231417774));
#158341=CARTESIAN_POINT('Ctrl Pts',(-3.712475039,4.964285714,6.288219134));
#158342=CARTESIAN_POINT('Ctrl Pts',(-3.668838729,4.95614194999999,6.31398139));
#158343=CARTESIAN_POINT('Ctrl Pts',(-3.624849092,4.947973174,6.339135576));
#158344=CARTESIAN_POINT('',(-3.65951457699334,4.94797317334225,6.34884527048642));
#158345=CARTESIAN_POINT('Ctrl Pts',(-4.437428167,4.81863040500001,5.930479793));
#158346=CARTESIAN_POINT('Ctrl Pts',(-4.430359933,4.820029867,5.935768535));
#158347=CARTESIAN_POINT('Ctrl Pts',(-4.423279112,4.821428571,5.941040415));
#158348=CARTESIAN_POINT('Ctrl Pts',(-4.105923812,4.884117105,6.177320758));
#158349=CARTESIAN_POINT('Ctrl Pts',(-3.765203291,4.947973174,6.378448361));
#158350=CARTESIAN_POINT('Ctrl Pts',(-4.220860275,4.81863040500001,5.894644903));
#158351=CARTESIAN_POINT('Ctrl Pts',(-4.213834751,4.820029867,5.89967553000001));
#158352=CARTESIAN_POINT('Ctrl Pts',(-4.206797255,4.821428571,5.904689396));
#158353=CARTESIAN_POINT('Ctrl Pts',(-3.891383734,4.884117105,6.129405827));
#158354=CARTESIAN_POINT('Ctrl Pts',(-3.553825856,4.947973174,6.319242184));
#158355=CARTESIAN_POINT('Ctrl Pts',(-4.21704120998609,4.8193909177524,5.89737769849005));
#158356=CARTESIAN_POINT('Ctrl Pts',(-4.2274111371836,4.82234724726756,5.91218659723742));
#158357=CARTESIAN_POINT('Ctrl Pts',(-4.23778434295171,4.82527010313881,
5.92699994298082));
#158358=CARTESIAN_POINT('Ctrl Pts',(-4.24817347433187,4.82816321750719,
5.94180789041483));
#158359=CARTESIAN_POINT('Ctrl Pts',(-4.2578992888877,4.83087161465861,5.95567039204521));
#158360=CARTESIAN_POINT('Ctrl Pts',(-4.26763578520111,4.83355328553615,
5.96953064924705));
#158361=CARTESIAN_POINT('Ctrl Pts',(-4.2773824756305,4.83620904387986,5.98338867250614));
#158362=CARTESIAN_POINT('Ctrl Pts',(-4.28712927070582,4.83886483073728,
5.99724684455274));
#158363=CARTESIAN_POINT('Ctrl Pts',(-4.29688628617097,4.84149471141519,
6.01110281940253));
#158364=CARTESIAN_POINT('Ctrl Pts',(-4.30665306526583,4.84409946429903,
6.0249566073236));
#158365=CARTESIAN_POINT('Ctrl Pts',(-4.82290286777507,4.94924836941368,
5.62147948639974));
#158366=CARTESIAN_POINT('Ctrl Pts',(-4.81985522788753,4.94861077170684,
5.62408845819987));
#158367=CARTESIAN_POINT('Ctrl Pts',(-4.816807588,4.94797317400001,5.62669743));
#158368=CARTESIAN_POINT('Ctrl Pts',(-4.510289559,4.88384644,5.889096179));
#158369=CARTESIAN_POINT('Ctrl Pts',(-4.177081292,4.818610636,6.116645419));
#158370=CARTESIAN_POINT('Ctrl Pts',(-4.83504752209277,4.94924836941368,
5.40230294817827));
#158371=CARTESIAN_POINT('Ctrl Pts',(-4.83211858954639,4.94861077170684,
5.40491862658914));
#158372=CARTESIAN_POINT('Ctrl Pts',(-4.829189657,4.94797317400001,5.40753430500001));
#158373=CARTESIAN_POINT('Ctrl Pts',(-4.53461068300001,4.88384644,5.670607575));
#158374=CARTESIAN_POINT('Ctrl Pts',(-4.213197547,4.818610636,5.900124272));
#158375=CARTESIAN_POINT('',(-4.82710945999426,4.94797317334255,5.44435392384521));
#158376=CARTESIAN_POINT('Ctrl Pts',(-4.83154927588509,4.94745154526473,
5.40542705122461));
#158377=CARTESIAN_POINT('Ctrl Pts',(-4.83036946644255,4.94771235963237,
5.4064806781123));
#158378=CARTESIAN_POINT('Ctrl Pts',(-4.829189657,4.947973174,5.40753430500001));
#158379=CARTESIAN_POINT('Ctrl Pts',(-4.711056901,4.974088171,5.51303256900001));
#158380=CARTESIAN_POINT('Ctrl Pts',(-4.588429626,5.00031307,5.613271201));
#158381=CARTESIAN_POINT('Ctrl Pts',(-4.82742100891798,4.94745154526473,
5.47906810964861));
#158382=CARTESIAN_POINT('Ctrl Pts',(-4.82622513295899,4.94771235963237,
5.4801208288243));
#158383=CARTESIAN_POINT('Ctrl Pts',(-4.825029257,4.947973174,5.481173548));
#158384=CARTESIAN_POINT('Ctrl Pts',(-4.705287782,4.974088171,5.586580924));
#158385=CARTESIAN_POINT('Ctrl Pts',(-4.581057291,5.00031307,5.6866585));
#158386=CARTESIAN_POINT('Origin',(0.11297875860618,5.08925694774986,-0.161496694229351));
#158387=CARTESIAN_POINT('Ctrl Pts',(-4.893996599,4.94766207,5.409842668));
#158388=CARTESIAN_POINT('Ctrl Pts',(-4.775109118,4.97393188700001,5.517393842));
#158389=CARTESIAN_POINT('Ctrl Pts',(-4.651611577,5.00031307,5.619618328));
#158390=CARTESIAN_POINT('Ctrl Pts',(-4.83059681,4.94766207,5.40627732));
#158391=CARTESIAN_POINT('Ctrl Pts',(-4.711787681,4.97393188700001,5.512435211));
#158392=CARTESIAN_POINT('Ctrl Pts',(-4.588429626,5.00031307,5.613271201));
#158393=CARTESIAN_POINT('Ctrl Pts',(-4.82918826277984,4.94797287201526,
5.40753569026454));
#158394=CARTESIAN_POINT('Ctrl Pts',(-4.83269845602471,4.94882769741037,
5.41140299956885));
#158395=CARTESIAN_POINT('Ctrl Pts',(-4.83620819522548,4.94967947055171,
5.41527139680809));
#158396=CARTESIAN_POINT('Ctrl Pts',(-4.83971888527368,4.95052852743952,
5.41913952584698));
#158397=CARTESIAN_POINT('Ctrl Pts',(-4.84297807326694,4.9513167588061,5.42273054628652));
#158398=CARTESIAN_POINT('Ctrl Pts',(-4.84623808186077,4.95210264920189,
5.42632133664188));
#158399=CARTESIAN_POINT('Ctrl Pts',(-4.84949890005566,4.95288622033443,
5.42991189702264));
#158400=CARTESIAN_POINT('Ctrl Pts',(-4.85275972154501,4.95366979225863,
5.433502461031));
#158401=CARTESIAN_POINT('Ctrl Pts',(-4.8560213534601,4.95445104511235,5.43709279596945));
#158402=CARTESIAN_POINT('Ctrl Pts',(-4.8592837852266,4.95523000036476,5.44068290219272));
#158403=CARTESIAN_POINT('Ctrl Pts',(-5.064082929,5.000313899,5.250967958));
#158404=CARTESIAN_POINT('Ctrl Pts',(-4.983742422,4.98224132,5.328449099));
#158405=CARTESIAN_POINT('Ctrl Pts',(-4.901069133,4.964285714,5.403436108));
#158406=CARTESIAN_POINT('Ctrl Pts',(-4.862855839,4.955986264,5.438096644));
#158407=CARTESIAN_POINT('Ctrl Pts',(-4.824156151,4.947660853,5.472213249));
#158408=CARTESIAN_POINT('Ctrl Pts',(-5.064842411,5.000313899,5.18747254));
#158409=CARTESIAN_POINT('Ctrl Pts',(-4.985473393,4.98224132,5.264965301));
#158410=CARTESIAN_POINT('Ctrl Pts',(-4.903770781,4.964285714,5.339993645));
#158411=CARTESIAN_POINT('Ctrl Pts',(-4.866006155,4.955986264,5.374673287));
#158412=CARTESIAN_POINT('Ctrl Pts',(-4.82775482,4.947660853,5.408815342));
#158413=CARTESIAN_POINT('Ctrl Pts',(-4.82918900301269,4.94797303315607,
5.40753502919794));
#158414=CARTESIAN_POINT('Ctrl Pts',(-4.85422464232958,4.95342302537021,
5.3851768922145));
#158415=CARTESIAN_POINT('Ctrl Pts',(-4.87908618026873,4.95886083280405,
5.36266176634008));
#158416=CARTESIAN_POINT('Ctrl Pts',(-4.90377078123183,4.9642857140524,5.33999364493616));
#158417=CARTESIAN_POINT('Ctrl Pts',(-4.95767392528497,4.97613189121847,
5.29049383644634));
#158418=CARTESIAN_POINT('Ctrl Pts',(-5.01091942444511,4.98803923906662,
5.24009317944469));
#158419=CARTESIAN_POINT('Ctrl Pts',(-5.06346365273142,5.00000000024774,
5.18881834708339));
#158420=CARTESIAN_POINT('Ctrl Pts',(-5.064842411,5.000313899,5.18747254));
#158421=CARTESIAN_POINT('Ctrl Pts',(-4.985473393,4.98224132,5.264965301));
#158422=CARTESIAN_POINT('Ctrl Pts',(-4.903770781,4.964285714,5.339993645));
#158423=CARTESIAN_POINT('Ctrl Pts',(-4.866714564,4.95614194999999,5.374022748));
#158424=CARTESIAN_POINT('Ctrl Pts',(-4.829189657,4.947973174,5.40753430500001));
#158425=CARTESIAN_POINT('Ctrl Pts',(-5.13859381,5.000313899,5.188354696));
#158426=CARTESIAN_POINT('Ctrl Pts',(-5.059211294,4.98224132,5.266975863));
#158427=CARTESIAN_POINT('Ctrl Pts',(-4.977460671,4.964285714,5.343131672));
#158428=CARTESIAN_POINT('Ctrl Pts',(-4.940382678,4.95614194999999,5.377672137));
#158429=CARTESIAN_POINT('Ctrl Pts',(-4.9028289,4.947973174,5.41169470400001));
#158430=CARTESIAN_POINT('',(-4.93877122247881,4.94797317334225,5.41372533678253));
#158431=CARTESIAN_POINT('Ctrl Pts',(-5.608561414,4.818630405,4.83791258399999));
#158432=CARTESIAN_POINT('Ctrl Pts',(-5.602795355,4.820029867,4.844597141));
#158433=CARTESIAN_POINT('Ctrl Pts',(-5.597013377,4.821428571,4.851267933));
#158434=CARTESIAN_POINT('Ctrl Pts',(-5.337870958,4.884117105,5.150246182));
#158435=CARTESIAN_POINT('Ctrl Pts',(-5.048352782,4.947973174,5.419916374));
#158436=CARTESIAN_POINT('Ctrl Pts',(-5.389353317,4.818630405,4.84947119));
#158437=CARTESIAN_POINT('Ctrl Pts',(-5.383573482,4.820029867,4.855894483));
#158438=CARTESIAN_POINT('Ctrl Pts',(-5.377778351,4.821428571,4.862303981));
#158439=CARTESIAN_POINT('Ctrl Pts',(-5.118046414,4.884117105,5.14957125100001));
#158440=CARTESIAN_POINT('Ctrl Pts',(-4.829189657,4.947973174,5.407534305));
#158441=CARTESIAN_POINT('Ctrl Pts',(-5.38621101020249,4.8193909179172,4.85296107987876));
#158442=CARTESIAN_POINT('Ctrl Pts',(-5.39952197013658,4.82234724738473,
4.86519452629106));
#158443=CARTESIAN_POINT('Ctrl Pts',(-5.41283708726114,4.82527010318465,
4.87743161198874));
#158444=CARTESIAN_POINT('Ctrl Pts',(-5.42616659749074,4.82816321755476,
4.88966000170456));
#158445=CARTESIAN_POINT('Ctrl Pts',(-5.43864505593992,4.8308716147002,4.90110764309131));
#158446=CARTESIAN_POINT('Ctrl Pts',(-5.45113346393274,4.83355328557171,
4.91255079625502));
#158447=CARTESIAN_POINT('Ctrl Pts',(-5.46363134748182,4.83620904390926,
4.92398957626564));
#158448=CARTESIAN_POINT('Ctrl Pts',(-5.47612936521519,4.83886483076053,
4.93542847908943));
#158449=CARTESIAN_POINT('Ctrl Pts',(-5.48863689206368,4.84149471143217,
4.94686303899888));
#158450=CARTESIAN_POINT('Ctrl Pts',(-5.50115348427103,4.8440994643342,4.9582933643208));
#158451=CARTESIAN_POINT('Ctrl Pts',(-5.91859799888375,4.94924836941368,
4.45327086703888));
#158452=CARTESIAN_POINT('Ctrl Pts',(-5.91618246294187,4.94861077170684,
4.45647399501944));
#158453=CARTESIAN_POINT('Ctrl Pts',(-5.913766927,4.94797317400001,4.459677123));
#158454=CARTESIAN_POINT('Ctrl Pts',(-5.670823094,4.88384644,4.781833451));
#158455=CARTESIAN_POINT('Ctrl Pts',(-5.394321411,4.818610636,5.07569264400001));
#158456=CARTESIAN_POINT('Ctrl Pts',(-5.88334224037081,4.94924836941368,
4.23660781253323));
#158457=CARTESIAN_POINT('Ctrl Pts',(-5.8810440781854,4.94861077170684,4.23979197176662));
#158458=CARTESIAN_POINT('Ctrl Pts',(-5.878745916,4.94797317400001,4.242976131));
#158459=CARTESIAN_POINT('Ctrl Pts',(-5.647607012,4.88384644,4.563224667));
#158460=CARTESIAN_POINT('Ctrl Pts',(-5.383047642,4.818610636,4.85646971400001));
#158461=CARTESIAN_POINT('',(-5.88462948285355,4.94797317334255,4.2793821087636));
#158462=CARTESIAN_POINT('Ctrl Pts',(-5.88059737102393,4.94745154526473,
4.24041089533189));
#158463=CARTESIAN_POINT('Ctrl Pts',(-5.87967164351197,4.94771235963237,
4.24169351316595));
#158464=CARTESIAN_POINT('Ctrl Pts',(-5.878745916,4.947973174,4.242976131));
#158465=CARTESIAN_POINT('Ctrl Pts',(-5.786054047,4.974088171,4.371402955));
#158466=CARTESIAN_POINT('Ctrl Pts',(-5.687842072,5.00031307,4.495659303));
#158467=CARTESIAN_POINT('Ctrl Pts',(-5.8923962720813,4.94745154526473,4.31321772265892));
#158468=CARTESIAN_POINT('Ctrl Pts',(-5.89145465854065,4.94771235963237,
4.31450290782946));
#158469=CARTESIAN_POINT('Ctrl Pts',(-5.890513045,4.947973174,4.315788093));
#158470=CARTESIAN_POINT('Ctrl Pts',(-5.796230529,4.974088171,4.444471981));
#158471=CARTESIAN_POINT('Ctrl Pts',(-5.696418198,5.00031307,4.568915682));
#158472=CARTESIAN_POINT('Origin',(0.145053772061448,5.08925682528172,-0.133433391065872));
#158473=CARTESIAN_POINT('Ctrl Pts',(-5.942533939,4.94766207,4.23129895));
#158474=CARTESIAN_POINT('Ctrl Pts',(-5.849546304,4.97393188700001,4.361892931));
#158475=CARTESIAN_POINT('Ctrl Pts',(-5.750911309,5.00031307,4.488275785));
#158476=CARTESIAN_POINT('Ctrl Pts',(-5.879849956,4.94766207,4.241446038));
#158477=CARTESIAN_POINT('Ctrl Pts',(-5.786639328,4.97393188700001,4.370662467));
#158478=CARTESIAN_POINT('Ctrl Pts',(-5.687842072,5.00031307,4.495659303));
#158479=CARTESIAN_POINT('Ctrl Pts',(-5.87874485221915,4.94797287197443,
4.24297778393543));
#158480=CARTESIAN_POINT('Ctrl Pts',(-5.88300433631815,4.94882769735767,
4.24600009009462));
#158481=CARTESIAN_POINT('Ctrl Pts',(-5.88726361083142,4.94967947049228,
4.2490235562089));
#158482=CARTESIAN_POINT('Ctrl Pts',(-5.89152375628648,4.9505285273734,4.25204655598669));
#158483=CARTESIAN_POINT('Ctrl Pts',(-5.89547870958579,4.95131675874924,
4.25485299137045));
#158484=CARTESIAN_POINT('Ctrl Pts',(-5.89943441481983,4.95210264915382,
4.2576590256409));
#158485=CARTESIAN_POINT('Ctrl Pts',(-5.90339086128714,4.95288622029679,
4.26046466127556));
#158486=CARTESIAN_POINT('Ctrl Pts',(-5.90734731175169,4.9536697922314,4.2632702997448));
#158487=CARTESIAN_POINT('Ctrl Pts',(-5.91130450444941,4.95445104509708,
4.2660755402845));
#158488=CARTESIAN_POINT('Ctrl Pts',(-5.9152624289547,4.95523000032746,4.26888038538439));
#158489=CARTESIAN_POINT('Ctrl Pts',(-6.07333975212726,5.00000000006602,
4.04081843272464));
#158490=CARTESIAN_POINT('Ctrl Pts',(-6.01205174514958,4.98208534611668,
4.13293414918722));
#158491=CARTESIAN_POINT('Ctrl Pts',(-5.94799829406127,4.964285714,4.2231487833414));
#158492=CARTESIAN_POINT('Ctrl Pts',(-5.91869173970455,4.9561417990393,4.26442493549441));
#158493=CARTESIAN_POINT('Ctrl Pts',(-5.88881516434955,4.94797287197443,
4.30529038626618));
#158494=CARTESIAN_POINT('Ctrl Pts',(-6.06052525045423,5.00000000006602,
3.97901164806512));
#158495=CARTESIAN_POINT('Ctrl Pts',(-6.00017468145858,4.98208534611668,
4.07093300385634));
#158496=CARTESIAN_POINT('Ctrl Pts',(-5.93706413,4.964285714,4.160981797));
#158497=CARTESIAN_POINT('Ctrl Pts',(-5.90818898457355,4.9561417990393,4.2021820712548));
#158498=CARTESIAN_POINT('Ctrl Pts',(-5.87874482871382,4.94797287197443,
4.24297763849028));
#158499=CARTESIAN_POINT('Ctrl Pts',(-5.87874535042468,4.94797301671685,
4.24297691564759));
#158500=CARTESIAN_POINT('Ctrl Pts',(-5.90818924040026,4.95614187119239,
4.20218170623045));
#158501=CARTESIAN_POINT('Ctrl Pts',(-5.93706413,4.964285714,4.160981797));
#158502=CARTESIAN_POINT('Ctrl Pts',(-6.00017468145858,4.98208534611668,
4.07093300385634));
#158503=CARTESIAN_POINT('Ctrl Pts',(-6.06052525045423,5.00000000006602,
3.97901164806513));
#158504=CARTESIAN_POINT('Ctrl Pts',(-6.061582466,5.000313899,3.977400912));
#158505=CARTESIAN_POINT('Ctrl Pts',(-6.000727704,4.98224132,4.07014392800001));
#158506=CARTESIAN_POINT('Ctrl Pts',(-5.93706413,4.964285714,4.160981797));
#158507=CARTESIAN_POINT('Ctrl Pts',(-5.908189518,4.95614194999999,4.20218131));
#158508=CARTESIAN_POINT('Ctrl Pts',(-5.878745916,4.947973174,4.242976131));
#158509=CARTESIAN_POINT('Ctrl Pts',(-6.133799235,5.000313899,3.96240807299999));
#158510=CARTESIAN_POINT('Ctrl Pts',(-6.073173866,4.98224132,4.056256015));
#158511=CARTESIAN_POINT('Ctrl Pts',(-6.009705774,4.964285714,4.148205311));
#158512=CARTESIAN_POINT('Ctrl Pts',(-5.980919823,4.95614194999999,4.189908912));
#158513=CARTESIAN_POINT('Ctrl Pts',(-5.951557878,4.947973174,4.231209003));
#158514=CARTESIAN_POINT('',(-5.98709641432499,4.94797317334225,4.2254656227057));
#158515=CARTESIAN_POINT('Ctrl Pts',(-6.51744456300001,4.81863040500001,
3.51912996));
#158516=CARTESIAN_POINT('Ctrl Pts',(-6.513250293,4.820029867,3.526897768));
#158517=CARTESIAN_POINT('Ctrl Pts',(-6.509037518,4.821428571,3.534655555));
#158518=CARTESIAN_POINT('Ctrl Pts',(-6.32022519,4.884117105,3.882351818));
#158519=CARTESIAN_POINT('Ctrl Pts',(-6.095446908,4.947973174,4.207955121));
#158520=CARTESIAN_POINT('Ctrl Pts',(-6.30584618800001,4.81863040500001,
3.577541593));
#158521=CARTESIAN_POINT('Ctrl Pts',(-6.3015823,4.820029867,3.585057207));
#158522=CARTESIAN_POINT('Ctrl Pts',(-6.297300509,4.821428571,3.592562637));
#158523=CARTESIAN_POINT('Ctrl Pts',(-6.105394932,4.884117105,3.928948446));
#158524=CARTESIAN_POINT('Ctrl Pts',(-5.878745916,4.947973174,4.242976131));
#158525=CARTESIAN_POINT('Ctrl Pts',(-6.30352756992369,4.8193909179172,3.58162539475427));
#158526=CARTESIAN_POINT('Ctrl Pts',(-6.31915715586046,4.82234724729902,
3.59071136724813));
#158527=CARTESIAN_POINT('Ctrl Pts',(-6.3347915846792,4.82527010310562,3.59979999996221));
#158528=CARTESIAN_POINT('Ctrl Pts',(-6.35043820069919,4.82816321747808,
3.60887704594857));
#158529=CARTESIAN_POINT('Ctrl Pts',(-6.36508582432909,4.83087161464152,
3.61737454809917));
#158530=CARTESIAN_POINT('Ctrl Pts',(-6.37974220004758,4.83355328553194,
3.62586552810932));
#158531=CARTESIAN_POINT('Ctrl Pts',(-6.39440688968605,4.83620904388884,
3.63435020025117));
#158532=CARTESIAN_POINT('Ctrl Pts',(-6.40907173677283,4.83886483075945,
3.6428349634892));
#158533=CARTESIAN_POINT('Ctrl Pts',(-6.4237449370543,4.84149471145087,3.65131344117656));
#158534=CARTESIAN_POINT('Ctrl Pts',(-6.43842608023093,4.84409946433625,
3.65978583438252));
#158535=CARTESIAN_POINT('Ctrl Pts',(-6.73754606545279,4.94924836941368,
3.07683225208978));
#158536=CARTESIAN_POINT('Ctrl Pts',(-6.73587558122639,4.94861077170684,
3.08047976154489));
#158537=CARTESIAN_POINT('Ctrl Pts',(-6.734205097,4.94797317400001,3.084127271));
#158538=CARTESIAN_POINT('Ctrl Pts',(-6.566195243,4.88384644,3.450977506));
#158539=CARTESIAN_POINT('Ctrl Pts',(-6.359329057,4.818610636,3.797406123));
#158540=CARTESIAN_POINT('Ctrl Pts',(-6.65653841463485,4.94924836941368,
2.87281360540941));
#158541=CARTESIAN_POINT('Ctrl Pts',(-6.65497848231742,4.94861077170684,
2.87641735770471));
#158542=CARTESIAN_POINT('Ctrl Pts',(-6.65341855,4.94797317400001,2.88002111));
#158543=CARTESIAN_POINT('Ctrl Pts',(-6.496527514,4.88384644,3.242470445));
#158544=CARTESIAN_POINT('Ctrl Pts',(-6.301192412,4.818610636,3.58573203));
#158545=CARTESIAN_POINT('',(-6.6669907716028,4.94797317334255,2.91431114283332));
#158546=CARTESIAN_POINT('Ctrl Pts',(-6.65467526919907,4.94745154526473,
2.87711784001687));
#158547=CARTESIAN_POINT('Ctrl Pts',(-6.65404690959953,4.94771235963237,
2.87856947500844));
#158548=CARTESIAN_POINT('Ctrl Pts',(-6.65341854999999,4.947973174,2.88002111));
#158549=CARTESIAN_POINT('Ctrl Pts',(-6.59050173599999,4.974088171,3.025371398));
#158550=CARTESIAN_POINT('Ctrl Pts',(-6.521297344,5.00031307,3.167835372));
#158551=CARTESIAN_POINT('Ctrl Pts',(-6.68184963465255,4.94745154526473,
2.94568606831802));
#158552=CARTESIAN_POINT('Ctrl Pts',(-6.68120631232628,4.94771235963237,
2.94714362565901));
#158553=CARTESIAN_POINT('Ctrl Pts',(-6.68056299,4.947973174,2.948601183));
#158554=CARTESIAN_POINT('Ctrl Pts',(-6.616147978,4.974088171,3.094544468));
#158555=CARTESIAN_POINT('Ctrl Pts',(-6.54542092200001,5.00031307,3.237535444));
#158556=CARTESIAN_POINT('Origin',(0.170346293524872,5.08925697390287,-0.0991313731653343));
#158557=CARTESIAN_POINT('Ctrl Pts',(-6.71320499500001,4.94766207,2.854904395));
#158558=CARTESIAN_POINT('Ctrl Pts',(-6.65046520500001,4.973931887,3.002434754));
#158559=CARTESIAN_POINT('Ctrl Pts',(-6.58130482,5.00031307,3.147066456));
#158560=CARTESIAN_POINT('Ctrl Pts',(-6.654167854,4.94766207,2.878289453));
#158561=CARTESIAN_POINT('Ctrl Pts',(-6.59091415,4.973931887,3.024522403));
#158562=CARTESIAN_POINT('Ctrl Pts',(-6.521297344,5.00031307,3.167835372));
#158563=CARTESIAN_POINT('Ctrl Pts',(-6.65341786670797,4.94797287202618,
2.88002295259182));
#158564=CARTESIAN_POINT('Ctrl Pts',(-6.6582274728443,4.9488276973978,2.88205893561886));
#158565=CARTESIAN_POINT('Ctrl Pts',(-6.66303712369621,4.94967947052343,
2.88409609656622));
#158566=CARTESIAN_POINT('Ctrl Pts',(-6.66784752488418,4.95052852739581,
2.88613261486336));
#158567=CARTESIAN_POINT('Ctrl Pts',(-6.67231331419332,4.95131675876267,
2.88802323921752));
#158568=CARTESIAN_POINT('Ctrl Pts',(-6.67677975163519,4.95210264915868,
2.88991331020176));
#158569=CARTESIAN_POINT('Ctrl Pts',(-6.68124682727894,4.9528862202939,2.89180283254273));
#158570=CARTESIAN_POINT('Ctrl Pts',(-6.6857139074358,4.95366979222076,2.8936923567927));
#158571=CARTESIAN_POINT('Ctrl Pts',(-6.69018162692286,4.95445104507959,
2.89558133287419));
#158572=CARTESIAN_POINT('Ctrl Pts',(-6.69464997632219,4.95523000034612,
2.89746976556783));
#158573=CARTESIAN_POINT('Ctrl Pts',(-6.800861408,5.000313899,2.639296217));
#158574=CARTESIAN_POINT('Ctrl Pts',(-6.760479825,4.98224132,2.743350299));
#158575=CARTESIAN_POINT('Ctrl Pts',(-6.716933807,4.964285714,2.846120278));
#158576=CARTESIAN_POINT('Ctrl Pts',(-6.696805943,4.955986264,2.893622674));
#158577=CARTESIAN_POINT('Ctrl Pts',(-6.676008248,4.947660853,2.940835644));
#158578=CARTESIAN_POINT('Ctrl Pts',(-6.774889661,5.000313899,2.581350438));
#158579=CARTESIAN_POINT('Ctrl Pts',(-6.735394657,4.98224132,2.685007149));
#158580=CARTESIAN_POINT('Ctrl Pts',(-6.692746959,4.964285714,2.787407065));
#158581=CARTESIAN_POINT('Ctrl Pts',(-6.673034316,4.955986264,2.834738411));
#158582=CARTESIAN_POINT('Ctrl Pts',(-6.652654221,4.947660853,2.88178622));
#158583=CARTESIAN_POINT('Ctrl Pts',(-6.65341826090931,4.94797303315017,
2.88002204190334));
#158584=CARTESIAN_POINT('Ctrl Pts',(-6.66675205370264,4.95342302528965,
2.84921815417841));
#158585=CARTESIAN_POINT('Ctrl Pts',(-6.67986191870764,4.95886083272511,
2.81834489018571));
#158586=CARTESIAN_POINT('Ctrl Pts',(-6.69274695880392,4.96428571390858,
2.78740706557253));
#158587=CARTESIAN_POINT('Ctrl Pts',(-6.72088369664955,4.97613189090849,
2.71984891517555));
#158588=CARTESIAN_POINT('Ctrl Pts',(-6.74804531683569,4.98803923904378,
2.65174931160051));
#158589=CARTESIAN_POINT('Ctrl Pts',(-6.77420342353812,5.00000000021333,
2.58315078520084));
#158590=CARTESIAN_POINT('Ctrl Pts',(-6.774889661,5.000313899,2.581350438));
#158591=CARTESIAN_POINT('Ctrl Pts',(-6.735394657,4.98224132,2.685007149));
#158592=CARTESIAN_POINT('Ctrl Pts',(-6.692746959,4.964285714,2.787407065));
#158593=CARTESIAN_POINT('Ctrl Pts',(-6.673404096,4.95614194999999,2.833850545));
#158594=CARTESIAN_POINT('Ctrl Pts',(-6.65341855,4.947973174,2.88002111));
#158595=CARTESIAN_POINT('Ctrl Pts',(-6.842195025,5.000313899,2.551183652));
#158596=CARTESIAN_POINT('Ctrl Pts',(-6.803161577,4.98224132,2.655870144));
#158597=CARTESIAN_POINT('Ctrl Pts',(-6.760943714,4.964285714,2.759313481));
#158598=CARTESIAN_POINT('Ctrl Pts',(-6.74179580400001,4.95614194999999,
2.806230203));
#158599=CARTESIAN_POINT('Ctrl Pts',(-6.721998624,4.947973174,2.852876671));
#158600=CARTESIAN_POINT('',(-6.75547163206247,4.94797317334224,2.83962783278288));
#158601=CARTESIAN_POINT('Ctrl Pts',(-7.121579248,4.818630405,2.035796731));
#158602=CARTESIAN_POINT('Ctrl Pts',(-7.119152886,4.820029867,2.044284575));
#158603=CARTESIAN_POINT('Ctrl Pts',(-7.116706299,4.821428571,2.052766612));
#158604=CARTESIAN_POINT('Ctrl Pts',(-7.007052717,4.884117105,2.432922999));
#158605=CARTESIAN_POINT('Ctrl Pts',(-6.857524711,4.947973174,2.799234563));
#158606=CARTESIAN_POINT('Ctrl Pts',(-6.92748470000001,4.818630405,2.138330128));
#158607=CARTESIAN_POINT('Ctrl Pts',(-6.924936134,4.820029867,2.146586641));
#158608=CARTESIAN_POINT('Ctrl Pts',(-6.922367894,4.821428571,2.154837056));
#158609=CARTESIAN_POINT('Ctrl Pts',(-6.80726196800001,4.884117105,2.524612378));
#158610=CARTESIAN_POINT('Ctrl Pts',(-6.65341855,4.947973174,2.88002111));
#158611=CARTESIAN_POINT('Ctrl Pts',(-6.92609818576639,4.81939091801858,
2.14281688688501));
#158612=CARTESIAN_POINT('Ctrl Pts',(-6.94331557651135,4.82234724733196,
2.1483305351867));
#158613=CARTESIAN_POINT('Ctrl Pts',(-6.96053826846024,4.82527010314683,
2.15384574070213));
#158614=CARTESIAN_POINT('Ctrl Pts',(-6.97777037186197,4.82816321751424,
2.1593470105455));
#158615=CARTESIAN_POINT('Ctrl Pts',(-6.99390225394218,4.83087161466876,
2.16449703978662));
#158616=CARTESIAN_POINT('Ctrl Pts',(-7.01004128142858,4.83355328554812,
2.1696388179197));
#158617=CARTESIAN_POINT('Ctrl Pts',(-7.02618707245826,4.83620904389281,
2.17477264840198));
#158618=CARTESIAN_POINT('Ctrl Pts',(-7.04233303683825,4.83886483075122,
2.17990653400395));
#158619=CARTESIAN_POINT('Ctrl Pts',(-7.05848580791564,4.84149471142928,
2.18503248530806));
#158620=CARTESIAN_POINT('Ctrl Pts',(-7.0746450282201,4.8440994643031,2.19015078689032));
#158621=CARTESIAN_POINT('Ctrl Pts',(-7.24145396603117,4.94924836941368,
1.55652438013174));
#158622=CARTESIAN_POINT('Ctrl Pts',(-7.24060664351559,4.94861077170684,
1.56044571756587));
#158623=CARTESIAN_POINT('Ctrl Pts',(-7.239759321,4.94797317400001,1.564367055));
#158624=CARTESIAN_POINT('Ctrl Pts',(-7.154539401,4.88384644,1.958757687));
#158625=CARTESIAN_POINT('Ctrl Pts',(-7.026981543,4.818610636,2.341557111));
#158626=CARTESIAN_POINT('Ctrl Pts',(-7.11848225152531,4.94924836941368,
1.37468982618827));
#158627=CARTESIAN_POINT('Ctrl Pts',(-7.11773348976265,4.94861077170684,
1.37854466409414));
#158628=CARTESIAN_POINT('Ctrl Pts',(-7.11698472800001,4.94797317400001,
1.382399502));
#158629=CARTESIAN_POINT('Ctrl Pts',(-7.041677609,4.88384644,1.770101908));
#158630=CARTESIAN_POINT('Ctrl Pts',(-6.92470042800001,4.818610636,2.147329501));
#158631=CARTESIAN_POINT('',(-7.1376109817771,4.94797317334255,1.41297022657449));
#158632=CARTESIAN_POINT('Ctrl Pts',(-7.11758794858711,4.94745154526474,
1.3792939513611));
#158633=CARTESIAN_POINT('Ctrl Pts',(-7.11728633829356,4.94771235963237,
1.38084672668055));
#158634=CARTESIAN_POINT('Ctrl Pts',(-7.11698472799999,4.947973174,1.382399502));
#158635=CARTESIAN_POINT('Ctrl Pts',(-7.086784889,4.974088171,1.537876837));
#158636=CARTESIAN_POINT('Ctrl Pts',(-7.049824001,5.00031307,1.691886981));
#158637=CARTESIAN_POINT('Ctrl Pts',(-7.15886713411728,4.94745154526474,
1.44041740752365));
#158638=CARTESIAN_POINT('Ctrl Pts',(-7.15855218405864,4.94771235963237,
1.44197918326182));
#158639=CARTESIAN_POINT('Ctrl Pts',(-7.158237234,4.947973174,1.443540959));
#158640=CARTESIAN_POINT('Ctrl Pts',(-7.126701702,4.974088171,1.599919494));
#158641=CARTESIAN_POINT('Ctrl Pts',(-7.088367037,5.00031307,1.754771648));
#158642=CARTESIAN_POINT('Origin',(0.187674271491483,5.0892572792628,-0.0601944222287432));
#158643=CARTESIAN_POINT('Ctrl Pts',(-7.169974048,4.94766207,1.345017684));
#158644=CARTESIAN_POINT('Ctrl Pts',(-7.140415745,4.97393188700001,1.502586065));
#158645=CARTESIAN_POINT('Ctrl Pts',(-7.103963832,5.00031307,1.658703797));
#158646=CARTESIAN_POINT('Ctrl Pts',(-7.117344258,4.94766207,1.380547252));
#158647=CARTESIAN_POINT('Ctrl Pts',(-7.087005153,4.97393188700001,1.536959034));
#158648=CARTESIAN_POINT('Ctrl Pts',(-7.049824001,5.00031307,1.691886981));
#158649=CARTESIAN_POINT('Ctrl Pts',(-7.11698445645141,4.94797287217653,
1.38240144844194));
#158650=CARTESIAN_POINT('Ctrl Pts',(-7.12211929286213,4.94882769748685,
1.38335590857904));
#158651=CARTESIAN_POINT('Ctrl Pts',(-7.12725442627626,4.94967947061876,
1.38431150914361));
#158652=CARTESIAN_POINT('Ctrl Pts',(-7.1323901543448,4.95052852750091,1.38526632077196));
#158653=CARTESIAN_POINT('Ctrl Pts',(-7.13715796428302,4.9513167588455,1.3861527307045));
#158654=CARTESIAN_POINT('Ctrl Pts',(-7.14192628825405,4.95210264922268,
1.38703846086629));
#158655=CARTESIAN_POINT('Ctrl Pts',(-7.1466951175664,4.95288622034009,1.38792351800371));
#158656=CARTESIAN_POINT('Ctrl Pts',(-7.15146395169674,4.95366979224915,
1.3888085760353));
#158657=CARTESIAN_POINT('Ctrl Pts',(-7.15623329237243,4.9544510450911,1.38969296126365));
#158658=CARTESIAN_POINT('Ctrl Pts',(-7.16100313117102,4.95523000029981,
1.39057668033257));
#158659=CARTESIAN_POINT('Ctrl Pts',(-7.209231717,5.000313899,1.115606768));
#158660=CARTESIAN_POINT('Ctrl Pts',(-7.192162786,4.98224132,1.22590897));
#158661=CARTESIAN_POINT('Ctrl Pts',(-7.171727357,4.964285714,1.33563735));
#158662=CARTESIAN_POINT('Ctrl Pts',(-7.16228168200001,4.955986264,1.386356063));
#158663=CARTESIAN_POINT('Ctrl Pts',(-7.152119618,4.947660853,1.436936109));
#158664=CARTESIAN_POINT('Ctrl Pts',(-7.171410545,5.000313899,1.064598886));
#158665=CARTESIAN_POINT('Ctrl Pts',(-7.155122041,4.98224132,1.174322419));
#158666=CARTESIAN_POINT('Ctrl Pts',(-7.135484378,4.964285714,1.283496277));
#158667=CARTESIAN_POINT('Ctrl Pts',(-7.126407446,4.955986264,1.333958678));
#158668=CARTESIAN_POINT('Ctrl Pts',(-7.116617714,4.947660853,1.384287653));
#158669=CARTESIAN_POINT('Ctrl Pts',(-7.11698472847237,4.94797317392425,
1.38239950207922));
#158670=CARTESIAN_POINT('Ctrl Pts',(-7.12716810933566,4.9566446894656,1.32997257504285));
#158671=CARTESIAN_POINT('Ctrl Pts',(-7.13676381742098,4.96527388632384,
1.27747875017038));
#158672=CARTESIAN_POINT('Ctrl Pts',(-7.15481559698884,4.98260138485293,
1.17216568210234));
#158673=CARTESIAN_POINT('Ctrl Pts',(-7.1632632328562,4.99129054983285,1.1193827722584));
#158674=CARTESIAN_POINT('Ctrl Pts',(-7.17112737309111,5.0000000005155,1.0665046610168));
#158675=CARTESIAN_POINT('Ctrl Pts',(-7.171410545,5.000313899,1.064598886));
#158676=CARTESIAN_POINT('Ctrl Pts',(-7.155122041,4.98224132,1.174322419));
#158677=CARTESIAN_POINT('Ctrl Pts',(-7.135484378,4.964285714,1.283496277));
#158678=CARTESIAN_POINT('Ctrl Pts',(-7.126577716,4.95614194999999,1.333012078));
#158679=CARTESIAN_POINT('Ctrl Pts',(-7.116984728,4.947973174,1.382399502));
#158680=CARTESIAN_POINT('Ctrl Pts',(-7.230657381,5.000313899,1.02066872));
#158681=CARTESIAN_POINT('Ctrl Pts',(-7.215041014,4.98224132,1.131298737));
#158682=CARTESIAN_POINT('Ctrl Pts',(-7.196047441,4.964285714,1.241399218));
#158683=CARTESIAN_POINT('Ctrl Pts',(-7.187432907,4.95614194999999,1.291335288));
#158684=CARTESIAN_POINT('Ctrl Pts',(-7.178126185,4.947973174,1.341146996));
#158685=CARTESIAN_POINT('',(-7.20796850522684,4.94797317334227,1.32101220153407));
#158686=CARTESIAN_POINT('Ctrl Pts',(-7.39271680200001,4.818630405,0.457271909));
#158687=CARTESIAN_POINT('Ctrl Pts',(-7.392171803,4.820029867,0.466082908));
#158688=CARTESIAN_POINT('Ctrl Pts',(-7.391605803,4.821428571,0.474892584));
#158689=CARTESIAN_POINT('Ctrl Pts',(-7.366238246,4.884117105,0.869733404));
#158690=CARTESIAN_POINT('Ctrl Pts',(-7.29895228100001,4.947973174,1.259624909));
#158691=CARTESIAN_POINT('Ctrl Pts',(-7.225201726,4.818630405,0.599132722));
#158692=CARTESIAN_POINT('Ctrl Pts',(-7.22448765,4.820029867,0.607744069));
#158693=CARTESIAN_POINT('Ctrl Pts',(-7.22375305,4.821428571,0.616353689));
#158694=CARTESIAN_POINT('Ctrl Pts',(-7.19082900000001,4.884117105,1.002228242));
#158695=CARTESIAN_POINT('Ctrl Pts',(-7.116984728,4.947973174,1.382399502));
#158696=CARTESIAN_POINT('Ctrl Pts',(-7.22481214832045,4.81939091801871,
0.603812642716627));
#158697=CARTESIAN_POINT('Ctrl Pts',(-7.24281227785518,4.82234724740094,
0.605496154954794));
#158698=CARTESIAN_POINT('Ctrl Pts',(-7.26081791900121,4.82527010320758,
0.607180048451803));
#158699=CARTESIAN_POINT('Ctrl Pts',(-7.27882975580833,4.82816321756723,
0.608848308897013));
#158700=CARTESIAN_POINT('Ctrl Pts',(-7.29569158745309,4.83087161470539,
0.610410055601027));
#158701=CARTESIAN_POINT('Ctrl Pts',(-7.31255862370503,4.83355328557064,
0.611962208038663));
#158702=CARTESIAN_POINT('Ctrl Pts',(-7.3294305568632,4.83620904390283,0.613505144663772));
#158703=CARTESIAN_POINT('Ctrl Pts',(-7.34630267116798,4.83886483074873,
0.61504809785472));
#158704=CARTESIAN_POINT('Ctrl Pts',(-7.36317972739467,4.8414947114159,0.616581838997027));
#158705=CARTESIAN_POINT('Ctrl Pts',(-7.38006143768145,4.84409946429152,
0.618106722867779));
#158706=CARTESIAN_POINT('Ctrl Pts',(-7.40675952790616,4.94924836941368,
-0.0365648420981692));
#158707=CARTESIAN_POINT('Ctrl Pts',(-7.40677498695308,4.94861077170685,
-0.0325530340490846));
#158708=CARTESIAN_POINT('Ctrl Pts',(-7.406790446,4.947973174,-0.028541226));
#158709=CARTESIAN_POINT('Ctrl Pts',(-7.408345248,4.88384644,0.374948537));
#158710=CARTESIAN_POINT('Ctrl Pts',(-7.366060182,4.818610636,0.776219491));
#158711=CARTESIAN_POINT('Ctrl Pts',(-7.24757376884405,4.94924836941368,
-0.187712921172618));
#158712=CARTESIAN_POINT('Ctrl Pts',(-7.24767118892203,4.94861077170685,
-0.183787245586309));
#158713=CARTESIAN_POINT('Ctrl Pts',(-7.247768609,4.947973174,-0.17986157));
#158714=CARTESIAN_POINT('Ctrl Pts',(-7.257566686,4.88384644,0.214965374));
#158715=CARTESIAN_POINT('Ctrl Pts',(-7.224417148,4.818610636,0.608520231));
#158716=CARTESIAN_POINT('',(-7.27448443441505,4.94797317334249,-0.154439607001196));
#158717=CARTESIAN_POINT('Ctrl Pts',(-7.24769012502909,4.94745154526473,
-0.183024189166083));
#158718=CARTESIAN_POINT('Ctrl Pts',(-7.24772936701454,4.94771235963237,
-0.181442879583041));
#158719=CARTESIAN_POINT('Ctrl Pts',(-7.247768609,4.947973174,-0.17986157));
#158720=CARTESIAN_POINT('Ctrl Pts',(-7.251697857,4.97408817100001,-0.021527137));
#158721=CARTESIAN_POINT('Ctrl Pts',(-7.248708723,5.00031307,0.136827835));
#158722=CARTESIAN_POINT('Ctrl Pts',(-7.30114396216113,4.94745154526473,
-0.132203570485143));
#158723=CARTESIAN_POINT('Ctrl Pts',(-7.30117211108056,4.94771235963237,
-0.130610603242571));
#158724=CARTESIAN_POINT('Ctrl Pts',(-7.30120026,4.947973174,-0.129017636));
#158725=CARTESIAN_POINT('Ctrl Pts',(-7.304018774,4.97408817100001,0.030484063));
#158726=CARTESIAN_POINT('Ctrl Pts',(-7.299868989,5.00031307,0.18995668));
#158727=CARTESIAN_POINT('Origin',(0.196226351021154,5.08925695299974,-0.0184426163327351));
#158728=CARTESIAN_POINT('Ctrl Pts',(-7.291483082,4.94766207,-0.22776056));
#158729=CARTESIAN_POINT('Ctrl Pts',(-7.296488381,4.97393188700001,-0.067521878));
#158730=CARTESIAN_POINT('Ctrl Pts',(-7.294449391,5.00031307,0.092781992));
#158731=CARTESIAN_POINT('Ctrl Pts',(-7.247721555,4.94766207,-0.181747804));
#158732=CARTESIAN_POINT('Ctrl Pts',(-7.251715671,4.97393188700001,-0.022470832));
#158733=CARTESIAN_POINT('Ctrl Pts',(-7.248708723,5.00031307,0.136827835));
#158734=CARTESIAN_POINT('Ctrl Pts',(-7.24776876254565,4.94797287209048,
-0.179859610832122));
#158735=CARTESIAN_POINT('Ctrl Pts',(-7.25298873007889,4.94882769744435,
-0.180031303752704));
#158736=CARTESIAN_POINT('Ctrl Pts',(-7.25820923271784,4.94967947057355,
-0.180201946555563));
#158737=CARTESIAN_POINT('Ctrl Pts',(-7.26343014649147,4.95052852744933,
-0.180373487663704));
#158738=CARTESIAN_POINT('Ctrl Pts',(-7.26827703965157,4.95131675880924,
-0.180532739752471));
#158739=CARTESIAN_POINT('Ctrl Pts',(-7.27312428867693,4.95210264919798,
-0.180692766204615));
#158740=CARTESIAN_POINT('Ctrl Pts',(-7.27797188654918,4.95288622032569,
-0.180853558570527));
#158741=CARTESIAN_POINT('Ctrl Pts',(-7.28281948931899,4.95366979224505,
-0.181014351098888));
#158742=CARTESIAN_POINT('Ctrl Pts',(-7.2876674421591,4.95445104509613,-0.181175909583881));
#158743=CARTESIAN_POINT('Ctrl Pts',(-7.29251573846638,4.95523000034311,
-0.18133822573945));
#158744=CARTESIAN_POINT('Ctrl Pts',(-7.28050636400001,5.000313899,-0.460247214));
#158745=CARTESIAN_POINT('Ctrl Pts',(-7.287548207,4.98224132,-0.348854501));
#158746=CARTESIAN_POINT('Ctrl Pts',(-7.291178906,4.964285714,-0.237298496));
#158747=CARTESIAN_POINT('Ctrl Pts',(-7.292857089,4.955986264,-0.185735018));
#158748=CARTESIAN_POINT('Ctrl Pts',(-7.29380582399999,4.947660853,-0.134152962));
#158749=CARTESIAN_POINT('Ctrl Pts',(-7.232604243,5.000313899,-0.501932126));
#158750=CARTESIAN_POINT('Ctrl Pts',(-7.240283871,4.98224132,-0.391272321));
#158751=CARTESIAN_POINT('Ctrl Pts',(-7.244574478,4.964285714,-0.28042937));
#158752=CARTESIAN_POINT('Ctrl Pts',(-7.246557685,4.955986264,-0.22919548));
#158753=CARTESIAN_POINT('Ctrl Pts',(-7.247816073,4.947660853,-0.177938666));
#158754=CARTESIAN_POINT('Ctrl Pts',(-7.24776873792564,4.94797303320985,
-0.179860602843012));
#158755=CARTESIAN_POINT('Ctrl Pts',(-7.24693594426172,4.95342302542251,
-0.213416168512296));
#158756=CARTESIAN_POINT('Ctrl Pts',(-7.24587078836578,4.95886083283933,
-0.246940673114338));
#158757=CARTESIAN_POINT('Ctrl Pts',(-7.24457447817704,4.96428571406034,
-0.280429370195282));
#158758=CARTESIAN_POINT('Ctrl Pts',(-7.24174375852354,4.97613189122118,
-0.353557797662088));
#158759=CARTESIAN_POINT('Ctrl Pts',(-7.23780069553802,4.98803923920819,
-0.42676819201584));
#158760=CARTESIAN_POINT('Ctrl Pts',(-7.23273737682363,5.00000000046251,
-0.500010033005965));
#158761=CARTESIAN_POINT('Ctrl Pts',(-7.232604243,5.000313899,-0.501932126));
#158762=CARTESIAN_POINT('Ctrl Pts',(-7.240283871,4.98224132,-0.391272321));
#158763=CARTESIAN_POINT('Ctrl Pts',(-7.244574478,4.964285714,-0.28042937));
#158764=CARTESIAN_POINT('Ctrl Pts',(-7.246520483,4.95614194999999,-0.230156553));
#158765=CARTESIAN_POINT('Ctrl Pts',(-7.247768609,4.947973174,-0.17986157));
#158766=CARTESIAN_POINT('Ctrl Pts',(-7.281022233,5.000313899,-0.557571548));
#158767=CARTESIAN_POINT('Ctrl Pts',(-7.289553152,4.98224132,-0.446170941));
#158768=CARTESIAN_POINT('Ctrl Pts',(-7.294671987,4.964285714,-0.334561492));
#158769=CARTESIAN_POINT('Ctrl Pts',(-7.296993635,4.95614194999999,-0.283941029));
#158770=CARTESIAN_POINT('Ctrl Pts',(-7.298612544,4.947973174,-0.233293221));
#158771=CARTESIAN_POINT('',(-7.32342878135728,4.94797317334223,-0.259372492529681));
#158772=CARTESIAN_POINT('Ctrl Pts',(-7.318179135,4.818630405,-1.14263444));
#158773=CARTESIAN_POINT('Ctrl Pts',(-7.319540982,4.820029867,-1.133912278));
#158774=CARTESIAN_POINT('Ctrl Pts',(-7.320882034,4.821428571,-1.125186894));
#158775=CARTESIAN_POINT('Ctrl Pts',(-7.380986662,4.884117105,-0.734123958));
#158776=CARTESIAN_POINT('Ctrl Pts',(-7.399088954,4.947973174,-0.338883407));
#158777=CARTESIAN_POINT('Ctrl Pts',(-7.18507635000001,4.818630405,-0.968079464000001));
#158778=CARTESIAN_POINT('Ctrl Pts',(-7.186230154,4.820029867,-0.95951594));
#158779=CARTESIAN_POINT('Ctrl Pts',(-7.187363542,4.821428571,-0.95094969));
#158780=CARTESIAN_POINT('Ctrl Pts',(-7.238160861,4.884117105,-0.567018973000001));
#158781=CARTESIAN_POINT('Ctrl Pts',(-7.247768609,4.947973174,-0.17986157));
#158782=CARTESIAN_POINT('Ctrl Pts',(-7.18570192502524,4.81939091775255,
-0.96342520897109));
#158783=CARTESIAN_POINT('Ctrl Pts',(-7.20364312653454,4.82234724727576,
-0.965650551686533));
#158784=CARTESIAN_POINT('Ctrl Pts',(-7.22158979302488,4.82527010313215,
-0.96787670764295));
#158785=CARTESIAN_POINT('Ctrl Pts',(-7.23953914972131,4.82816321749835,
-0.970119462776279));
#158786=CARTESIAN_POINT('Ctrl Pts',(-7.25634249050191,4.83087161465345,
-0.972219024305425));
#158787=CARTESIAN_POINT('Ctrl Pts',(-7.27314885172646,4.83355328553458,
-0.974329074620028));
#158788=CARTESIAN_POINT('Ctrl Pts',(-7.28995801424419,4.83620904388172,
-0.976449177968326));
#158789=CARTESIAN_POINT('Ctrl Pts',(-7.30676735723456,4.83886483074258,
-0.978569304079248));
#158790=CARTESIAN_POINT('Ctrl Pts',(-7.32357954629048,4.84149471142377,
-0.98069948922502));
#158791=CARTESIAN_POINT('Ctrl Pts',(-7.34039437668646,4.84409946433426,
-0.982839325059756));
#158792=CARTESIAN_POINT('Ctrl Pts',(-7.22573324546067,4.94924836941368,
-1.62794433293449));
#158793=CARTESIAN_POINT('Ctrl Pts',(-7.22661076323034,4.94861077170684,
-1.62402964196724));
#158794=CARTESIAN_POINT('Ctrl Pts',(-7.227488281,4.94797317400001,-1.620114951));
#158795=CARTESIAN_POINT('Ctrl Pts',(-7.315745105,4.88384644,-1.226392791));
#158796=CARTESIAN_POINT('Ctrl Pts',(-7.360710034,4.818610636,-0.825413289));
#158797=CARTESIAN_POINT('Ctrl Pts',(-7.03777679268802,4.94924836941368,
-1.74133842106059));
#158798=CARTESIAN_POINT('Ctrl Pts',(-7.03871583934401,4.94861077170684,
-1.73752546803029));
#158799=CARTESIAN_POINT('Ctrl Pts',(-7.03965488600001,4.94797317400001,
-1.733712515));
#158800=CARTESIAN_POINT('Ctrl Pts',(-7.134100011,4.88384644,-1.350222703));
#158801=CARTESIAN_POINT('Ctrl Pts',(-7.186328152,4.818610636,-0.958742768));
#158802=CARTESIAN_POINT('',(-7.071211081057,4.94797317334255,-1.71462801588899));
#158803=CARTESIAN_POINT('Ctrl Pts',(-7.03889836730892,4.94745154526473,
-1.73678432215825));
#158804=CARTESIAN_POINT('Ctrl Pts',(-7.03927662665446,4.94771235963237,
-1.73524841857913));
#158805=CARTESIAN_POINT('Ctrl Pts',(-7.039654886,4.947973174,-1.733712515));
#158806=CARTESIAN_POINT('Ctrl Pts',(-7.077529493,4.974088171,-1.579924525));
#158807=CARTESIAN_POINT('Ctrl Pts',(-7.108651881,5.00031307,-1.424629229));
#158808=CARTESIAN_POINT('Ctrl Pts',(-7.1020274146377,4.94745154526474,-1.69864285574175));
#158809=CARTESIAN_POINT('Ctrl Pts',(-7.10239734631886,4.94771235963237,
-1.69709318237087));
#158810=CARTESIAN_POINT('Ctrl Pts',(-7.102767278,4.947973174,-1.695543509));
#158811=CARTESIAN_POINT('Ctrl Pts',(-7.139808047,4.974088171,-1.540376768));
#158812=CARTESIAN_POINT('Ctrl Pts',(-7.17003718,5.00031307,-1.383740452));
#158813=CARTESIAN_POINT('Origin',(0.195603365251878,5.0892570054678,0.0241714225221729));
#158814=CARTESIAN_POINT('Ctrl Pts',(-7.07205047200001,4.94766207,-1.789888972));
#158815=CARTESIAN_POINT('Ctrl Pts',(-7.11138533,4.973931887,-1.634472573));
#158816=CARTESIAN_POINT('Ctrl Pts',(-7.143854603,5.00031307,-1.477478196));
#158817=CARTESIAN_POINT('Ctrl Pts',(-7.039203447,4.94766207,-1.735544534));
#158818=CARTESIAN_POINT('Ctrl Pts',(-7.077344024,4.973931887,-1.580849986));
#158819=CARTESIAN_POINT('Ctrl Pts',(-7.108651881,5.00031307,-1.424629229));
#158820=CARTESIAN_POINT('Ctrl Pts',(-7.03965545684652,4.94797287211985,
-1.73371063429946));
#158821=CARTESIAN_POINT('Ctrl Pts',(-7.04471647548854,4.94882769743596,
-1.73500045180656));
#158822=CARTESIAN_POINT('Ctrl Pts',(-7.04977824253012,4.94967947055132,
-1.73628935882992));
#158823=CARTESIAN_POINT('Ctrl Pts',(-7.05484021799868,4.95052852741816,
-1.73757923153099));
#158824=CARTESIAN_POINT('Ctrl Pts',(-7.05953955902984,4.9513167587711,-1.73877669914946));
#158825=CARTESIAN_POINT('Ctrl Pts',(-7.06423908115425,4.95210264915737,
-1.73997499952157));
#158826=CARTESIAN_POINT('Ctrl Pts',(-7.06893877932178,4.95288622028444,
-1.74117412288784));
#158827=CARTESIAN_POINT('Ctrl Pts',(-7.07363848223743,4.95366979220316,
-1.74237324746559));
#158828=CARTESIAN_POINT('Ctrl Pts',(-7.07833836238181,4.95445104505539,
-1.74357319534238));
#158829=CARTESIAN_POINT('Ctrl Pts',(-7.08303841496067,4.95523000028386,
-1.74477395697837));
#158830=CARTESIAN_POINT('Ctrl Pts',(-7.011352625,5.000313899,-2.014580548));
#158831=CARTESIAN_POINT('Ctrl Pts',(-7.042175974,4.98224132,-1.907305922));
#158832=CARTESIAN_POINT('Ctrl Pts',(-7.069703033,4.964285714,-1.799138528));
#158833=CARTESIAN_POINT('Ctrl Pts',(-7.082426605,4.955986264,-1.749141335));
#158834=CARTESIAN_POINT('Ctrl Pts',(-7.094441776,4.947660853,-1.698969189));
#158835=CARTESIAN_POINT('Ctrl Pts',(-6.955609405,5.000313899,-2.04499335));
#158836=CARTESIAN_POINT('Ctrl Pts',(-6.986898075,4.98224132,-1.938571603));
#158837=CARTESIAN_POINT('Ctrl Pts',(-7.014916327,4.964285714,-1.831242452));
#158838=CARTESIAN_POINT('Ctrl Pts',(-7.02786694,4.955986264,-1.781632713));
#158839=CARTESIAN_POINT('Ctrl Pts',(-7.040114608,4.947660853,-1.73184477));
#158840=CARTESIAN_POINT('Ctrl Pts',(-7.03965488655287,4.94797317390935,
-1.73371251515132));
#158841=CARTESIAN_POINT('Ctrl Pts',(-7.02688358239494,4.9566446859759,-1.78556977598731));
#158842=CARTESIAN_POINT('Ctrl Pts',(-7.01355081990285,4.96527388717983,
-1.83724103979854));
#158843=CARTESIAN_POINT('Ctrl Pts',(-6.98571435793737,4.98260138847449,
-1.9404003540024));
#158844=CARTESIAN_POINT('Ctrl Pts',(-6.97121825042533,4.99129055630127,
-1.99185191186361));
#158845=CARTESIAN_POINT('Ctrl Pts',(-6.95615261950568,5.0000000003956,-2.04314481393163));
#158846=CARTESIAN_POINT('Ctrl Pts',(-6.955609405,5.000313899,-2.04499335));
#158847=CARTESIAN_POINT('Ctrl Pts',(-6.986898075,4.98224132,-1.938571603));
#158848=CARTESIAN_POINT('Ctrl Pts',(-7.014916327,4.964285714,-1.831242452));
#158849=CARTESIAN_POINT('Ctrl Pts',(-7.02762400500001,4.95614194999999,
-1.782563319));
#158850=CARTESIAN_POINT('Ctrl Pts',(-7.039654886,4.947973174,-1.733712515));
#158851=CARTESIAN_POINT('Ctrl Pts',(-6.990934579,5.000313899,-2.10974039));
#158852=CARTESIAN_POINT('Ctrl Pts',(-7.023213887,4.98224132,-2.002778163));
#158853=CARTESIAN_POINT('Ctrl Pts',(-7.052205779,4.964285714,-1.894878478));
#158854=CARTESIAN_POINT('Ctrl Pts',(-7.065355051,4.95614194999999,-1.845940579));
#158855=CARTESIAN_POINT('Ctrl Pts',(-7.077823892,4.947973174,-1.796824907));
#158856=CARTESIAN_POINT('',(-7.09645366749441,4.94797317334227,-1.82762921640457));
#158857=CARTESIAN_POINT('Ctrl Pts',(-6.901451545,4.818630405,-2.689112472));
#158858=CARTESIAN_POINT('Ctrl Pts',(-6.90465656,4.820029867,-2.680886986));
#158859=CARTESIAN_POINT('Ctrl Pts',(-6.907841959,4.821428571,-2.672653884));
#158860=CARTESIAN_POINT('Ctrl Pts',(-7.050608345,4.884117105,-2.3036545));
#158861=CARTESIAN_POINT('Ctrl Pts',(-7.153252451,4.947973174,-1.92154591));
#158862=CARTESIAN_POINT('Ctrl Pts',(-6.808984789,4.818630405,-2.49002533));
#158863=CARTESIAN_POINT('Ctrl Pts',(-6.811952522,4.820029867,-2.48191005));
#158864=CARTESIAN_POINT('Ctrl Pts',(-6.814900903,4.821428571,-2.47378772));
#158865=CARTESIAN_POINT('Ctrl Pts',(-6.94704436400001,4.884117105,-2.109753011));
#158866=CARTESIAN_POINT('Ctrl Pts',(-7.039654886,4.947973174,-1.733712515));
#158867=CARTESIAN_POINT('Ctrl Pts',(-6.81059626604813,4.81939091775241,
-2.48561436902601));
#158868=CARTESIAN_POINT('Ctrl Pts',(-6.82763962922413,4.82234724736873,
-2.49164451250913));
#158869=CARTESIAN_POINT('Ctrl Pts',(-6.84468815497496,4.82527010319989,
-2.49767662485868));
#158870=CARTESIAN_POINT('Ctrl Pts',(-6.86173573966136,4.82816321756086,
-2.50372552673113));
#158871=CARTESIAN_POINT('Ctrl Pts',(-6.87769488401649,4.83087161470757,
-2.5093882232332));
#158872=CARTESIAN_POINT('Ctrl Pts',(-6.89365472341908,4.83355328558158,
-2.51506181260813));
#158873=CARTESIAN_POINT('Ctrl Pts',(-6.90961513751605,4.83620904392258,
-2.52074582218012));
#158874=CARTESIAN_POINT('Ctrl Pts',(-6.925575722973,4.8388648307773,-2.52642989277884));
#158875=CARTESIAN_POINT('Ctrl Pts',(-6.94153692555988,4.84149471145331,
-2.5321243990602));
#158876=CARTESIAN_POINT('Ctrl Pts',(-6.9574986329725,4.84409946433526,-2.5378288981618));
#158877=CARTESIAN_POINT('Ctrl Pts',(-6.7068397085662,4.94924836941368,-3.14320295556554));
#158878=CARTESIAN_POINT('Ctrl Pts',(-6.7085382532831,4.94861077170684,-3.13956842828277));
#158879=CARTESIAN_POINT('Ctrl Pts',(-6.71023679800001,4.94797317400001,
-3.135933901));
#158880=CARTESIAN_POINT('Ctrl Pts',(-6.881068851,4.88384644,-2.770389355));
#158881=CARTESIAN_POINT('Ctrl Pts',(-7.011181266,4.818610636,-2.388450661));
#158882=CARTESIAN_POINT('Ctrl Pts',(-6.49890119506649,4.94924836941368,
-3.21354087208441));
#158883=CARTESIAN_POINT('Ctrl Pts',(-6.50063795953325,4.94861077170684,
-3.21001893104221));
#158884=CARTESIAN_POINT('Ctrl Pts',(-6.502374724,4.94797317400001,-3.20649699));
#158885=CARTESIAN_POINT('Ctrl Pts',(-6.67705074900001,4.88384644,-2.852275866));
#158886=CARTESIAN_POINT('Ctrl Pts',(-6.812214438,4.818610636,-2.481176021));
#158887=CARTESIAN_POINT('',(-6.53729575574303,4.94797317334255,-3.19464232459535));
#158888=CARTESIAN_POINT('Ctrl Pts',(-6.50097554455138,4.94745154526473,
-3.20933435087155));
#158889=CARTESIAN_POINT('Ctrl Pts',(-6.50167513427568,4.94771235963237,
-3.20791567043577));
#158890=CARTESIAN_POINT('Ctrl Pts',(-6.502374724,4.947973174,-3.20649699));
#158891=CARTESIAN_POINT('Ctrl Pts',(-6.572423716,4.974088171,-3.064446398));
#158892=CARTESIAN_POINT('Ctrl Pts',(-6.636202377,5.00031307,-2.919472213));
#158893=CARTESIAN_POINT('Ctrl Pts',(-6.570827957299,4.94745154526473,-3.18565548897648));
#158894=CARTESIAN_POINT('Ctrl Pts',(-6.5715223741495,4.94771235963237,-3.18422157048824));
#158895=CARTESIAN_POINT('Ctrl Pts',(-6.572216791,4.947973174,-3.182787652));
#158896=CARTESIAN_POINT('Ctrl Pts',(-6.64174783,4.974088171,-3.039211294));
#158897=CARTESIAN_POINT('Ctrl Pts',(-6.704942401,5.00031307,-2.892735418));
#158898=CARTESIAN_POINT('Origin',(0.185833529860157,5.08925709679066,0.0656549302348208));
#158899=CARTESIAN_POINT('Ctrl Pts',(-6.52193664200001,4.94766207,-3.268324166));
#158900=CARTESIAN_POINT('Ctrl Pts',(-6.593761804,4.97393188700001,-3.124997148));
#158901=CARTESIAN_POINT('Ctrl Pts',(-6.659221114,5.00031307,-2.978653146));
#158902=CARTESIAN_POINT('Ctrl Pts',(-6.50154001,4.94766207,-3.208189131));
#158903=CARTESIAN_POINT('Ctrl Pts',(-6.572043636,4.97393188700001,-3.065310352));
#158904=CARTESIAN_POINT('Ctrl Pts',(-6.63620237700001,5.00031307,-2.919472213));
#158905=CARTESIAN_POINT('Ctrl Pts',(-6.50237568605531,4.94797287219492,
-3.20649527578045));
#158906=CARTESIAN_POINT('Ctrl Pts',(-6.50704110849926,4.94882769745278,
-3.20884290710233));
#158907=CARTESIAN_POINT('Ctrl Pts',(-6.51170745733011,4.94967947057386,
-3.21118981052001));
#158908=CARTESIAN_POINT('Ctrl Pts',(-6.5163738021151,4.95052852744416,-3.21353770185232));
#158909=CARTESIAN_POINT('Ctrl Pts',(-6.52070585498803,4.9513167587952,-3.2157173927796));
#158910=CARTESIAN_POINT('Ctrl Pts',(-6.5250379056958,4.95210264917763,-3.2178979359278));
#158911=CARTESIAN_POINT('Ctrl Pts',(-6.52936995141139,4.95288622030084,
-3.22007932067324));
#158912=CARTESIAN_POINT('Ctrl Pts',(-6.53370200150367,4.95366979221571,
-3.22226070762255));
#158913=CARTESIAN_POINT('Ctrl Pts',(-6.53803404769612,4.95445104506405,
-3.22444293672171));
#158914=CARTESIAN_POINT('Ctrl Pts',(-6.54236608731522,4.9552300002817,-3.2266259975922));
#158915=CARTESIAN_POINT('Ctrl Pts',(-6.414355829,5.000313899,-3.474714335));
#158916=CARTESIAN_POINT('Ctrl Pts',(-6.46751942,4.98224132,-3.376573839));
#158917=CARTESIAN_POINT('Ctrl Pts',(-6.517655703,4.964285714,-3.276852842));
#158918=CARTESIAN_POINT('Ctrl Pts',(-6.540829724,4.955986264,-3.230759748));
#158919=CARTESIAN_POINT('Ctrl Pts',(-6.563349515,4.947660853,-3.184343505));
#158920=CARTESIAN_POINT('Ctrl Pts',(-6.353378002,5.000313899,-3.492432958));
#158921=CARTESIAN_POINT('Ctrl Pts',(-6.40681269,4.98224132,-3.395225431));
#158922=CARTESIAN_POINT('Ctrl Pts',(-6.457248486,4.964285714,-3.296428672));
#158923=CARTESIAN_POINT('Ctrl Pts',(-6.480560947,4.955986264,-3.25076278));
#158924=CARTESIAN_POINT('Ctrl Pts',(-6.503225208,4.947660853,-3.204771738));
#158925=CARTESIAN_POINT('Ctrl Pts',(-6.50237524706428,4.94797303335539,
-3.2064961659945));
#158926=CARTESIAN_POINT('Ctrl Pts',(-6.48752980748,4.95342302544615,-3.23660069140457));
#158927=CARTESIAN_POINT('Ctrl Pts',(-6.47248652405784,4.95886083281266,
-3.26657946034516));
#158928=CARTESIAN_POINT('Ctrl Pts',(-6.45724848618829,4.96428571404603,
-3.29642867215033));
#158929=CARTESIAN_POINT('Ctrl Pts',(-6.42397356473944,4.97613189118364,
-3.36160964736261));
#158930=CARTESIAN_POINT('Ctrl Pts',(-6.38965469195533,4.98803923904675,
-3.42639795188724));
#158931=CARTESIAN_POINT('Ctrl Pts',(-6.35430589758882,5.0000000002178,-3.49074441377445));
#158932=CARTESIAN_POINT('Ctrl Pts',(-6.353378002,5.000313899,-3.492432958));
#158933=CARTESIAN_POINT('Ctrl Pts',(-6.40681269,4.98224132,-3.395225431));
#158934=CARTESIAN_POINT('Ctrl Pts',(-6.457248486,4.964285714,-3.296428672));
#158935=CARTESIAN_POINT('Ctrl Pts',(-6.48012364,4.95614195,-3.251619405));
#158936=CARTESIAN_POINT('Ctrl Pts',(-6.502374724,4.947973174,-3.20649699));
#158937=CARTESIAN_POINT('Ctrl Pts',(-6.373958593,5.000313899,-3.563260116));
#158938=CARTESIAN_POINT('Ctrl Pts',(-6.42847694499999,4.98224132,-3.465737703));
#158939=CARTESIAN_POINT('Ctrl Pts',(-6.479986266,4.964285714,-3.366593053));
#158940=CARTESIAN_POINT('Ctrl Pts',(-6.503348317,4.95614195,-3.321626));
#158941=CARTESIAN_POINT('Ctrl Pts',(-6.526084062,4.947973174,-3.276339057));
#158942=CARTESIAN_POINT('',(-6.5376562666786,4.94797317334228,-3.31042803009703));
#158943=CARTESIAN_POINT('Ctrl Pts',(-6.162019751,4.818630405,-4.109850593));
#158944=CARTESIAN_POINT('Ctrl Pts',(-6.166918071,4.820029867,-4.102506398));
#158945=CARTESIAN_POINT('Ctrl Pts',(-6.171798871,4.821428571,-4.095150548));
#158946=CARTESIAN_POINT('Ctrl Pts',(-6.390551418,4.884117105,-3.765468718));
#158947=CARTESIAN_POINT('Ctrl Pts',(-6.572937813,4.947973174,-3.414359063));
#158948=CARTESIAN_POINT('Ctrl Pts',(-6.114512667,4.818630405,-3.895540379));
#158949=CARTESIAN_POINT('Ctrl Pts',(-6.119155562,4.820029867,-3.888252805));
#158950=CARTESIAN_POINT('Ctrl Pts',(-6.123781072,4.821428571,-3.880954185));
#158951=CARTESIAN_POINT('Ctrl Pts',(-6.331091794,4.884117105,-3.553837343));
#158952=CARTESIAN_POINT('Ctrl Pts',(-6.502374724,4.947973174,-3.20649699));
#158953=CARTESIAN_POINT('Ctrl Pts',(-6.11703469529526,4.81939091801858,
-3.8915789639107));
#158954=CARTESIAN_POINT('Ctrl Pts',(-6.13238329170512,4.82234724732519,
-3.90113194489536));
#158955=CARTESIAN_POINT('Ctrl Pts',(-6.14773650636247,4.82527010323118,
-3.91068795923837));
#158956=CARTESIAN_POINT('Ctrl Pts',(-6.16308519293364,4.82816321759971,
-3.92026016792834));
#158957=CARTESIAN_POINT('Ctrl Pts',(-6.17745390895555,4.83087161473765,
-3.92922121796549));
#158958=CARTESIAN_POINT('Ctrl Pts',(-6.19182096212693,4.83355328560386,
-3.93819305562455));
#158959=CARTESIAN_POINT('Ctrl Pts',(-6.20618633652024,4.83620904393796,
-3.94717519340763));
#158960=CARTESIAN_POINT('Ctrl Pts',(-6.22055186514831,4.83886483078577,
-3.956157427628));
#158961=CARTESIAN_POINT('Ctrl Pts',(-6.23491575311279,4.84149471145579,
-3.9651499862183));
#158962=CARTESIAN_POINT('Ctrl Pts',(-6.24927798597133,4.84409946433865,
-3.97415241254827));
#158963=CARTESIAN_POINT('Ctrl Pts',(-5.87434179975964,4.94924836941368,
-4.51148890129795));
#158964=CARTESIAN_POINT('Ctrl Pts',(-5.87678194937982,4.94861077170684,
-4.50830448414898));
#158965=CARTESIAN_POINT('Ctrl Pts',(-5.879222099,4.94797317400001,-4.505120067));
#158966=CARTESIAN_POINT('Ctrl Pts',(-6.124641466,4.88384644,-4.184845591));
#158967=CARTESIAN_POINT('Ctrl Pts',(-6.333817454,4.818610636,-3.839806735));
#158968=CARTESIAN_POINT('Ctrl Pts',(-5.6561442008214,4.94924836941368,-4.53548172299218));
#158969=CARTESIAN_POINT('Ctrl Pts',(-5.6585974739107,4.94861077170684,-4.53241547599609));
#158970=CARTESIAN_POINT('Ctrl Pts',(-5.661050747,4.94797317400001,-4.529349229));
#158971=CARTESIAN_POINT('Ctrl Pts',(-5.90779001400001,4.88384644,-4.22095978));
#158972=CARTESIAN_POINT('Ctrl Pts',(-6.119569149,4.818610636,-3.887592241));
#158973=CARTESIAN_POINT('',(-5.69770374701121,4.94797317334255,-4.5252787091336));
#158974=CARTESIAN_POINT('Ctrl Pts',(-5.65907433086952,4.94745154526473,
-4.5318194717201));
#158975=CARTESIAN_POINT('Ctrl Pts',(-5.66006253893476,4.94771235963237,
-4.53058435036005));
#158976=CARTESIAN_POINT('Ctrl Pts',(-5.661050747,4.947973174,-4.529349229));
#158977=CARTESIAN_POINT('Ctrl Pts',(-5.759998711,4.974088171,-4.405678164));
#158978=CARTESIAN_POINT('Ctrl Pts',(-5.853451427,5.00031307,-4.277803922));
#158979=CARTESIAN_POINT('Ctrl Pts',(-5.73238388827846,4.94745154526473,
-4.52371041336006));
#158980=CARTESIAN_POINT('Ctrl Pts',(-5.73337032013924,4.94771235963237,
-4.52245929818003));
#158981=CARTESIAN_POINT('Ctrl Pts',(-5.734356752,4.947973174,-4.521208183));
#158982=CARTESIAN_POINT('Ctrl Pts',(-5.833126867,4.974088171,-4.395935678));
#158983=CARTESIAN_POINT('Ctrl Pts',(-5.926331967,5.00031307,-4.266469291));
#158984=CARTESIAN_POINT('Origin',(0.167375319649697,5.08925700133457,0.104068977210618));
#158985=CARTESIAN_POINT('Ctrl Pts',(-5.666864302,4.94766207,-4.593936154));
#158986=CARTESIAN_POINT('Ctrl Pts',(-5.767821305,4.97393188700001,-4.469400329));
#158987=CARTESIAN_POINT('Ctrl Pts',(-5.863209847,5.00031307,-4.340549585));
#158988=CARTESIAN_POINT('Ctrl Pts',(-5.659871788,4.94766207,-4.53082237));
#158989=CARTESIAN_POINT('Ctrl Pts',(-5.75944179200001,4.97393188700001,
-4.406440213));
#158990=CARTESIAN_POINT('Ctrl Pts',(-5.853451427,5.00031307,-4.277803922));
#158991=CARTESIAN_POINT('Ctrl Pts',(-5.66105205514287,4.94797287208707,
-4.52934776177233));
#158992=CARTESIAN_POINT('Ctrl Pts',(-5.66510373101984,4.94882769740976,
-4.53264343487047));
#158993=CARTESIAN_POINT('Ctrl Pts',(-5.66915646832016,4.94967947055303,
-4.5359385960291));
#158994=CARTESIAN_POINT('Ctrl Pts',(-5.67320898930314,4.95052852744299,
-4.53923472113756));
#158995=CARTESIAN_POINT('Ctrl Pts',(-5.67697119202556,4.9513167588072,-4.54229471537536));
#158996=CARTESIAN_POINT('Ctrl Pts',(-5.68073320943725,4.95210264920075,
-4.54535554144628));
#158997=CARTESIAN_POINT('Ctrl Pts',(-5.68449504105515,4.95288622033218,
-4.54841718836571));
#158998=CARTESIAN_POINT('Ctrl Pts',(-5.68825687647365,4.95366979225525,
-4.55147883837835));
#158999=CARTESIAN_POINT('Ctrl Pts',(-5.69201852704637,4.95445104510896,
-4.55454131001399));
#159000=CARTESIAN_POINT('Ctrl Pts',(-5.69577999258466,4.95523000036888,
-4.55760459272089));
#159001=CARTESIAN_POINT('Ctrl Pts',(-5.517430884,5.000313899,-4.772374341));
#159002=CARTESIAN_POINT('Ctrl Pts',(-5.590448845,4.98224132,-4.68795691599999));
#159003=CARTESIAN_POINT('Ctrl Pts',(-5.660850037,4.964285714,-4.601345159));
#159004=CARTESIAN_POINT('Ctrl Pts',(-5.693390914,4.955986264,-4.561311425));
#159005=CARTESIAN_POINT('Ctrl Pts',(-5.725362325,4.947660853,-4.520821458));
#159006=CARTESIAN_POINT('Ctrl Pts',(-5.454069705,5.000313899,-4.776570282));
#159007=CARTESIAN_POINT('Ctrl Pts',(-5.527151864,4.98224132,-4.69312229100001));
#159008=CARTESIAN_POINT('Ctrl Pts',(-5.597646882,4.964285714,-4.607477551));
#159009=CARTESIAN_POINT('Ctrl Pts',(-5.630231128,4.955986264,-4.567890792));
#159010=CARTESIAN_POINT('Ctrl Pts',(-5.662252225,4.947660853,-4.527847142));
#159011=CARTESIAN_POINT('Ctrl Pts',(-5.661050747,4.947973174,-4.529349229));
#159012=CARTESIAN_POINT('Ctrl Pts',(-5.64008185355594,4.95342292106738,
-4.55555740236727));
#159013=CARTESIAN_POINT('Ctrl Pts',(-5.6189455709875,4.95886077964645,-4.58160167016205));
#159014=CARTESIAN_POINT('Ctrl Pts',(-5.59764688175189,4.9642857140632,-4.60747755130143));
#159015=CARTESIAN_POINT('Ctrl Pts',(-5.55113792653855,4.97613189126735,
-4.6639815070346));
#159016=CARTESIAN_POINT('Ctrl Pts',(-5.50369384036136,4.98803923897126,
-4.71987755304588));
#159017=CARTESIAN_POINT('Ctrl Pts',(-5.45533889445123,5.00000000010406,
-4.77512068459171));
#159018=CARTESIAN_POINT('Ctrl Pts',(-5.454069705,5.000313899,-4.776570282));
#159019=CARTESIAN_POINT('Ctrl Pts',(-5.527151864,4.98224132,-4.69312229100001));
#159020=CARTESIAN_POINT('Ctrl Pts',(-5.597646882,4.964285714,-4.607477551));
#159021=CARTESIAN_POINT('Ctrl Pts',(-5.629619895,4.95614195,-4.568633382));
#159022=CARTESIAN_POINT('Ctrl Pts',(-5.661050747,4.947973174,-4.529349229));
#159023=CARTESIAN_POINT('Ctrl Pts',(-5.458943387,5.000313899,-4.85016575900001));
#159024=CARTESIAN_POINT('Ctrl Pts',(-5.533151567,4.98224132,-4.766643201));
#159025=CARTESIAN_POINT('Ctrl Pts',(-5.604769797,4.964285714,-4.680889479));
#159026=CARTESIAN_POINT('Ctrl Pts',(-5.637252244,4.95614195,-4.641995881));
#159027=CARTESIAN_POINT('Ctrl Pts',(-5.669191793,4.947973174,-4.60265523400001));
#159028=CARTESIAN_POINT('',(-5.67316532544793,4.94797317334228,-4.63843490812138));
#159029=CARTESIAN_POINT('Ctrl Pts',(-5.134458762,4.81863040500001,-5.338416669));
#159030=CARTESIAN_POINT('Ctrl Pts',(-5.140821347,4.820029867,-5.33229717100001));
#159031=CARTESIAN_POINT('Ctrl Pts',(-5.147169327,4.821428571,-5.326162524));
#159032=CARTESIAN_POINT('Ctrl Pts',(-5.43167941,4.884117105,-5.051213803));
#159033=CARTESIAN_POINT('Ctrl Pts',(-5.685279909,4.947973174,-4.747520581));
#159034=CARTESIAN_POINT('Ctrl Pts',(-5.134132729,4.81863040500001,-5.118904289));
#159035=CARTESIAN_POINT('Ctrl Pts',(-5.140233688,4.820029867,-5.11278518));
#159036=CARTESIAN_POINT('Ctrl Pts',(-5.146320044,4.821428571,-5.106651545));
#159037=CARTESIAN_POINT('Ctrl Pts',(-5.41910440800001,4.884117105,-4.831748191));
#159038=CARTESIAN_POINT('Ctrl Pts',(-5.661050747,4.947973174,-4.529349229));
#159039=CARTESIAN_POINT('Ctrl Pts',(-5.13744737984433,4.8193909179173,-5.11557765142939));
#159040=CARTESIAN_POINT('Ctrl Pts',(-5.1503835258232,4.82234724732518,-5.1282067840203));
#159041=CARTESIAN_POINT('Ctrl Pts',(-5.16332353063032,4.8252701031319,-5.14083987093192));
#159042=CARTESIAN_POINT('Ctrl Pts',(-5.17625563150039,4.82816321749342,
-5.15348780056849));
#159043=CARTESIAN_POINT('Ctrl Pts',(-5.18836205414139,4.83087161464878,
-5.16532819550913));
#159044=CARTESIAN_POINT('Ctrl Pts',(-5.20046453379271,4.83355328553066,
-5.17717876839553));
#159045=CARTESIAN_POINT('Ctrl Pts',(-5.21256315969593,4.83620904387903,
-5.1890390397041));
#159046=CARTESIAN_POINT('Ctrl Pts',(-5.22466191549681,4.83886483074111,
-5.20089943835123));
#159047=CARTESIAN_POINT('Ctrl Pts',(-5.23675684956082,4.84149471142401,
-5.21276956729307));
#159048=CARTESIAN_POINT('Ctrl Pts',(-5.24884804582745,4.84409946429349,
-5.22464897735641));
#159049=CARTESIAN_POINT('Ctrl Pts',(-4.76716619730484,4.94924836941368,
-5.66882264040786));
#159050=CARTESIAN_POINT('Ctrl Pts',(-4.77023385315243,4.94861077170684,
-5.66623723320393));
#159051=CARTESIAN_POINT('Ctrl Pts',(-4.773301509,4.94797317400001,-5.663651826));
#159052=CARTESIAN_POINT('Ctrl Pts',(-5.08183265400001,4.88384644,-5.403623099));
#159053=CARTESIAN_POINT('Ctrl Pts',(-5.360291378,4.818610636,-5.11161771400001));
#159054=CARTESIAN_POINT('Ctrl Pts',(-4.54891219022449,4.94924836941368,
-5.64534848929436));
#159055=CARTESIAN_POINT('Ctrl Pts',(-4.55196725961225,4.94861077170684,
-5.64288131064718));
#159056=CARTESIAN_POINT('Ctrl Pts',(-4.555022329,4.94797317400001,-5.640414132));
#159057=CARTESIAN_POINT('Ctrl Pts',(-4.862287584,4.88384644,-5.392276306));
#159058=CARTESIAN_POINT('Ctrl Pts',(-5.14077960699999,4.818610636,-5.112228969));
#159059=CARTESIAN_POINT('',(-4.59169344389577,4.94797317334255,-5.64431809002532));
#159060=CARTESIAN_POINT('Ctrl Pts',(-4.55256109121282,4.94745154526473,
-5.6424017507755));
#159061=CARTESIAN_POINT('Ctrl Pts',(-4.55379171010641,4.94771235963237,
-5.64140794138775));
#159062=CARTESIAN_POINT('Ctrl Pts',(-4.55502232900001,4.947973174,-5.640414132));
#159063=CARTESIAN_POINT('Ctrl Pts',(-4.678242568,4.974088171,-5.540905315));
#159064=CARTESIAN_POINT('Ctrl Pts',(-4.796999593,5.00031307,-5.436110273));
#159065=CARTESIAN_POINT('Ctrl Pts',(-4.62589992017682,4.94745154526473,
-5.65024166521513));
#159066=CARTESIAN_POINT('Ctrl Pts',(-4.62713224258841,4.94771235963237,
-5.64923185410757));
#159067=CARTESIAN_POINT('Ctrl Pts',(-4.628364565,4.947973174,-5.648222043));
#159068=CARTESIAN_POINT('Ctrl Pts',(-4.751755375,4.974088171,-5.547110995));
#159069=CARTESIAN_POINT('Ctrl Pts',(-4.870612837,5.00031307,-5.440707802));
#159070=CARTESIAN_POINT('Origin',(0.141090112662756,5.08925706339396,0.137616244610315));
#159071=CARTESIAN_POINT('Ctrl Pts',(-4.546815687,4.94766207,-5.704740794));
#159072=CARTESIAN_POINT('Ctrl Pts',(-4.672183892,4.97393188700001,-5.604819318));
#159073=CARTESIAN_POINT('Ctrl Pts',(-4.793041404,5.00031307,-5.49948675));
#159074=CARTESIAN_POINT('Ctrl Pts',(-4.553554251,4.94766207,-5.641599391));
#159075=CARTESIAN_POINT('Ctrl Pts',(-4.677534851,4.97393188700001,-5.541529827));
#159076=CARTESIAN_POINT('Ctrl Pts',(-4.796999593,5.00031307,-5.436110273));
#159077=CARTESIAN_POINT('Ctrl Pts',(-4.55502392165559,4.94797287218644,
-5.64041298053945));
#159078=CARTESIAN_POINT('Ctrl Pts',(-4.55827239943767,4.9488276974756,-5.64450259314184));
#159079=CARTESIAN_POINT('Ctrl Pts',(-4.56152202378497,4.94967947059951,
-5.64859193398487));
#159080=CARTESIAN_POINT('Ctrl Pts',(-4.56477122964979,4.95052852747181,
-5.65268216973473));
#159081=CARTESIAN_POINT('Ctrl Pts',(-4.56778766590997,4.95131675882528,
-5.65647938540585));
#159082=CARTESIAN_POINT('Ctrl Pts',(-4.57080374237042,4.95210264920943,
-5.66027737362154));
#159083=CARTESIAN_POINT('Ctrl Pts',(-4.57381946092239,4.95288622033308,
-5.66407612355446));
#159084=CARTESIAN_POINT('Ctrl Pts',(-4.57683518252117,4.95366979224837,
-5.66787487732529));
#159085=CARTESIAN_POINT('Ctrl Pts',(-4.57985054697082,4.95445104509583,
-5.67167439377354));
#159086=CARTESIAN_POINT('Ctrl Pts',(-4.58286555616587,4.95523000030221,
-5.67547466231674));
#159087=CARTESIAN_POINT('Ctrl Pts',(-4.362517003,5.000313899,-5.846883427));
#159088=CARTESIAN_POINT('Ctrl Pts',(-4.451975096,4.98224132,-5.780136338));
#159089=CARTESIAN_POINT('Ctrl Pts',(-4.539349314,4.964285714,-5.710683691));
#159090=CARTESIAN_POINT('Ctrl Pts',(-4.579735474,4.955986264,-5.67858125));
#159091=CARTESIAN_POINT('Ctrl Pts',(-4.619663557,4.947660853,-5.645910824));
#159092=CARTESIAN_POINT('Ctrl Pts',(-4.29973517,5.000313899,-5.837360488));
#159093=CARTESIAN_POINT('Ctrl Pts',(-4.38904756,4.98224132,-5.77157397));
#159094=CARTESIAN_POINT('Ctrl Pts',(-4.476305531,4.964285714,-5.703085901));
#159095=CARTESIAN_POINT('Ctrl Pts',(-4.516637959,4.955986264,-5.671429308));
#159096=CARTESIAN_POINT('Ctrl Pts',(-4.556518621,4.947660853,-5.639205445));
#159097=CARTESIAN_POINT('Ctrl Pts',(-4.55502314960303,4.94797303331433,
-5.64041360402221));
#159098=CARTESIAN_POINT('Ctrl Pts',(-4.52890923100112,4.95342302539129,
-5.66150229278074));
#159099=CARTESIAN_POINT('Ctrl Pts',(-4.50266855884138,4.95886083277496,
-5.68239377597682));
#159100=CARTESIAN_POINT('Ctrl Pts',(-4.47630553123975,4.96428571399719,
-5.70308590101651));
#159101=CARTESIAN_POINT('Ctrl Pts',(-4.41873725026119,4.97613189112419,
-5.74827077517629));
#159102=CARTESIAN_POINT('Ctrl Pts',(-4.36038638074774,4.98803923912244,
-5.79266092730607));
#159103=CARTESIAN_POINT('Ctrl Pts',(-4.30128630597296,5.00000000033185,
-5.83621762044319));
#159104=CARTESIAN_POINT('Ctrl Pts',(-4.29973517,5.000313899,-5.837360488));
#159105=CARTESIAN_POINT('Ctrl Pts',(-4.38904756,4.98224132,-5.77157397));
#159106=CARTESIAN_POINT('Ctrl Pts',(-4.476305531,4.964285714,-5.703085901));
#159107=CARTESIAN_POINT('Ctrl Pts',(-4.515881381,4.95614195,-5.672023139));
#159108=CARTESIAN_POINT('Ctrl Pts',(-4.555022329,4.947973174,-5.640414132));
#159109=CARTESIAN_POINT('Ctrl Pts',(-4.288674056,5.000313899,-5.910283042));
#159110=CARTESIAN_POINT('Ctrl Pts',(-4.379102171,4.98224132,-5.844665759));
#159111=CARTESIAN_POINT('Ctrl Pts',(-4.467480522,4.964285714,-5.776312715));
#159112=CARTESIAN_POINT('Ctrl Pts',(-4.507564521,4.95614195,-5.745311193));
#159113=CARTESIAN_POINT('Ctrl Pts',(-4.54721441799999,4.947973174,-5.713756368));
#159114=CARTESIAN_POINT('',(-4.54340347883659,4.94797317334228,-5.74955372499979));
#159115=CARTESIAN_POINT('Ctrl Pts',(-3.866816188,4.818630405,-6.317364314));
#159116=CARTESIAN_POINT('Ctrl Pts',(-3.874345531,4.820029867,-6.312755654));
#159117=CARTESIAN_POINT('Ctrl Pts',(-3.881863866,4.821428571,-6.30812906));
#159118=CARTESIAN_POINT('Ctrl Pts',(-4.218828109,4.884117105,-6.10076974500001));
#159119=CARTESIAN_POINT('Ctrl Pts',(-4.531784635,4.947973174,-5.858693313));
#159120=CARTESIAN_POINT('Ctrl Pts',(-3.91368645,4.818630405,-6.102913924));
#159121=CARTESIAN_POINT('Ctrl Pts',(-3.9209602,4.820029867,-6.098249402));
#159122=CARTESIAN_POINT('Ctrl Pts',(-3.928222811,4.821428571,-6.093567555));
#159123=CARTESIAN_POINT('Ctrl Pts',(-4.253725723,4.884117105,-5.883731863));
#159124=CARTESIAN_POINT('Ctrl Pts',(-4.555022329,4.947973174,-5.640414132));
#159125=CARTESIAN_POINT('Ctrl Pts',(-3.91763873527576,4.81939091791743,
-6.10037761323303));
#159126=CARTESIAN_POINT('Ctrl Pts',(-3.92755755152312,4.8223472472166,-6.11549237277444));
#159127=CARTESIAN_POINT('Ctrl Pts',(-3.93747928571279,4.82527010307455,
-6.13061182384926));
#159128=CARTESIAN_POINT('Ctrl Pts',(-3.94739011022992,4.82816321744659,
-6.14574407138381));
#159129=CARTESIAN_POINT('Ctrl Pts',(-3.95666815648934,4.8308716146068,-6.15991016749337));
#159130=CARTESIAN_POINT('Ctrl Pts',(-3.96594016399411,4.83355328549382,
-6.17408535596271));
#159131=CARTESIAN_POINT('Ctrl Pts',(-3.97520632298064,4.83620904384735,
-6.18826918766501));
#159132=CARTESIAN_POINT('Ctrl Pts',(-3.98447258145384,4.83886483071459,
-6.20245317165289));
#159133=CARTESIAN_POINT('Ctrl Pts',(-3.99373301581997,4.84149471140265,
-6.21664583688259));
#159134=CARTESIAN_POINT('Ctrl Pts',(-4.00298780463037,4.84409946428194,
-6.23084676275461));
#159135=CARTESIAN_POINT('Ctrl Pts',(-3.43708320223719,4.94924836941368,
-6.56108853400832));
#159136=CARTESIAN_POINT('Ctrl Pts',(-3.4406349241186,4.94861077170685,-6.55922302750416));
#159137=CARTESIAN_POINT('Ctrl Pts',(-3.444186646,4.947973174,-6.557357521));
#159138=CARTESIAN_POINT('Ctrl Pts',(-3.801402994,4.88384644,-6.369733196));
#159139=CARTESIAN_POINT('Ctrl Pts',(-4.136124034,4.818610636,-6.14441513));
#159140=CARTESIAN_POINT('Ctrl Pts',(-3.22897810090943,4.94924836941368,
-6.49124503453278));
#159141=CARTESIAN_POINT('Ctrl Pts',(-3.23249211495472,4.94861077170685,
-6.48949228676639));
#159142=CARTESIAN_POINT('Ctrl Pts',(-3.236006129,4.947973174,-6.487739539));
#159143=CARTESIAN_POINT('Ctrl Pts',(-3.589429991,4.88384644,-6.311455985));
#159144=CARTESIAN_POINT('Ctrl Pts',(-3.921612925,4.818610636,-6.097823552));
#159145=CARTESIAN_POINT('',(-3.27098065792544,4.94797317334254,-6.49943543079898));
#159146=CARTESIAN_POINT('Ctrl Pts',(-3.23317515431105,4.94745154526474,
-6.48915159497978));
#159147=CARTESIAN_POINT('Ctrl Pts',(-3.23459064165553,4.94771235963237,
-6.48844556698989));
#159148=CARTESIAN_POINT('Ctrl Pts',(-3.236006129,4.947973174,-6.487739539));
#159149=CARTESIAN_POINT('Ctrl Pts',(-3.377737001,4.974088171,-6.417045892));
#159150=CARTESIAN_POINT('Ctrl Pts',(-3.51624539,5.00031307,-6.34023015));
#159151=CARTESIAN_POINT('Ctrl Pts',(-3.30311401212512,4.94745154526474,
-6.51257389780459));
#159152=CARTESIAN_POINT('Ctrl Pts',(-3.30453460306256,4.94771235963237,
-6.5118526084023));
#159153=CARTESIAN_POINT('Ctrl Pts',(-3.305955194,4.947973174,-6.511131319));
#159154=CARTESIAN_POINT('Ctrl Pts',(-3.448197082,4.974088171,-6.438909567));
#159155=CARTESIAN_POINT('Ctrl Pts',(-3.587149265,5.00031307,-6.360544862));
#159156=CARTESIAN_POINT('Origin',(0.10820841979828,5.0892568791216,0.164729784140485));
#159157=CARTESIAN_POINT('Ctrl Pts',(-3.214163023,4.94766207,-6.54879809400001));
#159158=CARTESIAN_POINT('Ctrl Pts',(-3.358080353,4.973931887,-6.478163184));
#159159=CARTESIAN_POINT('Ctrl Pts',(-3.498755672,5.00031307,-6.401274026));
#159160=CARTESIAN_POINT('Ctrl Pts',(-3.234317579,4.94766207,-6.488581494));
#159161=CARTESIAN_POINT('Ctrl Pts',(-3.376911579,4.973931887,-6.417503665));
#159162=CARTESIAN_POINT('Ctrl Pts',(-3.51624539,5.00031307,-6.34023015));
#159163=CARTESIAN_POINT('Ctrl Pts',(-3.23600793233001,4.94797287199268,
-6.4877387569128));
#159164=CARTESIAN_POINT('Ctrl Pts',(-3.238301316439,4.94882769736909,-6.49243108356366));
#159165=CARTESIAN_POINT('Ctrl Pts',(-3.2405958789538,4.94967947050675,-6.49712339103697));
#159166=CARTESIAN_POINT('Ctrl Pts',(-3.24288984038026,4.95052852738732,
-6.50181648251531));
#159167=CARTESIAN_POINT('Ctrl Pts',(-3.24501946491259,4.95131675875919,
-6.50617336603982));
#159168=CARTESIAN_POINT('Ctrl Pts',(-3.24714857197188,4.95210264915641,
-6.51053092668283));
#159169=CARTESIAN_POINT('Ctrl Pts',(-3.24927716574165,4.95288622029139,
-6.51488915429613));
#159170=CARTESIAN_POINT('Ctrl Pts',(-3.25140576166195,4.95366979221801,
-6.51924738631258));
#159171=CARTESIAN_POINT('Ctrl Pts',(-3.25353384482793,4.9544510450751,-6.52360628640031));
#159172=CARTESIAN_POINT('Ctrl Pts',(-3.25566141942808,4.95523000031271,
-6.52796584476247));
#159173=CARTESIAN_POINT('Ctrl Pts',(-3.003616676,5.000313899,-6.64799874200001));
#159174=CARTESIAN_POINT('Ctrl Pts',(-3.105331939,4.98224132,-6.602043008));
#159175=CARTESIAN_POINT('Ctrl Pts',(-3.205593663,4.964285714,-6.552997));
#159176=CARTESIAN_POINT('Ctrl Pts',(-3.251936692,4.955986264,-6.530326927));
#159177=CARTESIAN_POINT('Ctrl Pts',(-3.297954455,4.947660853,-6.507003675));
#159178=CARTESIAN_POINT('Ctrl Pts',(-2.944349797,5.000313899,-6.625202206));
#159179=CARTESIAN_POINT('Ctrl Pts',(-3.04571627,4.98224132,-6.580153264));
#159180=CARTESIAN_POINT('Ctrl Pts',(-3.145657109,4.964285714,-6.532024292));
#159181=CARTESIAN_POINT('Ctrl Pts',(-3.191851818,4.955986264,-6.50977809300001));
#159182=CARTESIAN_POINT('Ctrl Pts',(-3.237727271,4.947660853,-6.48688077));
#159183=CARTESIAN_POINT('Ctrl Pts',(-3.23600612947942,4.94797317382086,
-6.48773954002634));
#159184=CARTESIAN_POINT('Ctrl Pts',(-3.18821456999116,4.9566446780338,-6.51157739400629));
#159185=CARTESIAN_POINT('Ctrl Pts',(-3.14020122808787,4.96527388257548,
-6.53486694554253));
#159186=CARTESIAN_POINT('Ctrl Pts',(-3.04355614826285,4.9826013876045,-6.58043498550645));
#159187=CARTESIAN_POINT('Ctrl Pts',(-2.99495714815925,4.99129055431876,
-6.60269563274663));
#159188=CARTESIAN_POINT('Ctrl Pts',(-2.94611035073432,5.00000000038334,
-6.62441950656244));
#159189=CARTESIAN_POINT('Ctrl Pts',(-2.944349797,5.000313899,-6.625202206));
#159190=CARTESIAN_POINT('Ctrl Pts',(-3.04571627,4.98224132,-6.580153264));
#159191=CARTESIAN_POINT('Ctrl Pts',(-3.145657109,4.964285714,-6.532024292));
#159192=CARTESIAN_POINT('Ctrl Pts',(-3.190985273,4.95614195,-6.510195399));
#159193=CARTESIAN_POINT('Ctrl Pts',(-3.236006129,4.947973174,-6.487739539));
#159194=CARTESIAN_POINT('Ctrl Pts',(-2.917871093,5.000313899,-6.694042058));
#159195=CARTESIAN_POINT('Ctrl Pts',(-3.020290825,4.98224132,-6.649398243));
#159196=CARTESIAN_POINT('Ctrl Pts',(-3.121296823,4.964285714,-6.601641988));
#159197=CARTESIAN_POINT('Ctrl Pts',(-3.167108091,4.95614195,-6.579982139));
#159198=CARTESIAN_POINT('Ctrl Pts',(-3.21261435,4.947973174,-6.557688604));
#159199=CARTESIAN_POINT('',(-3.20119713487288,4.94797317334223,-6.59182979976144));
#159200=CARTESIAN_POINT('Ctrl Pts',(-2.418365587,4.818630405,-7.000919025));
#159201=CARTESIAN_POINT('Ctrl Pts',(-2.426709623,4.820029867,-6.998036699));
#159202=CARTESIAN_POINT('Ctrl Pts',(-2.435046765,4.821428571,-6.995134492));
#159203=CARTESIAN_POINT('Ctrl Pts',(-2.808709094,4.884117105,-6.865060475));
#159204=CARTESIAN_POINT('Ctrl Pts',(-3.166388148,4.947973174,-6.695920057));
#159205=CARTESIAN_POINT('Ctrl Pts',(-2.510240543,4.818630405,-6.801558087));
#159206=CARTESIAN_POINT('Ctrl Pts',(-2.518346971,4.820029867,-6.79856626));
#159207=CARTESIAN_POINT('Ctrl Pts',(-2.526446244,4.821428571,-6.795555119));
#159208=CARTESIAN_POINT('Ctrl Pts',(-2.88944755,4.884117105,-6.660598773));
#159209=CARTESIAN_POINT('Ctrl Pts',(-3.236006129,4.947973174,-6.487739539));
#159210=CARTESIAN_POINT('Ctrl Pts',(-2.51464565778541,4.81939091791719,
-6.79993069839959));
#159211=CARTESIAN_POINT('Ctrl Pts',(-2.5210833505913,4.82234724728871,-6.81682433556511));
#159212=CARTESIAN_POINT('Ctrl Pts',(-2.52752288517145,4.82527010314086,
-6.83372318185064));
#159213=CARTESIAN_POINT('Ctrl Pts',(-2.53394901425799,4.82816321751078,
-6.85063218017267));
#159214=CARTESIAN_POINT('Ctrl Pts',(-2.53996485306458,4.83087161466,-6.86646158647879));
#159215=CARTESIAN_POINT('Ctrl Pts',(-2.54597283970855,4.83355328553621,
-6.88229857441741));
#159216=CARTESIAN_POINT('Ctrl Pts',(-2.55197325652855,4.83620904387925,
-6.89814274625689));
#159217=CARTESIAN_POINT('Ctrl Pts',(-2.55797373777239,4.838864830736,-6.9139870882083));
#159218=CARTESIAN_POINT('Ctrl Pts',(-2.56396666486193,4.84149471141391,
-6.92983865642847));
#159219=CARTESIAN_POINT('Ctrl Pts',(-2.56995230260316,4.84409946428864,
-6.94569707856559));
#159220=CARTESIAN_POINT('Ctrl Pts',(-1.9462860173166,4.94924836941368,-7.14656521854563));
#159221=CARTESIAN_POINT('Ctrl Pts',(-1.9501557306583,4.94861077170684,-7.14550684177282));
#159222=CARTESIAN_POINT('Ctrl Pts',(-1.954025444,4.947973174,-7.144448465));
#159223=CARTESIAN_POINT('Ctrl Pts',(-2.343223955,4.88384644,-7.038001649));
#159224=CARTESIAN_POINT('Ctrl Pts',(-2.718556127,4.818610636,-6.889906523));
#159225=CARTESIAN_POINT('Ctrl Pts',(-1.75806058539699,4.94924836941368,
-7.03361817669735));
#159226=CARTESIAN_POINT('Ctrl Pts',(-1.76186923269849,4.94861077170684,
-7.03266181634868));
#159227=CARTESIAN_POINT('Ctrl Pts',(-1.76567788,4.947973174,-7.031705456));
#159228=CARTESIAN_POINT('Ctrl Pts',(-2.148734641,4.88384644,-6.935518997));
#159229=CARTESIAN_POINT('Ctrl Pts',(-2.519075981,4.818610636,-6.798290683));
#159230=CARTESIAN_POINT('',(-1.79732045262188,4.94797317334248,-7.05064639398859));
#159231=CARTESIAN_POINT('Ctrl Pts',(-1.76260954163828,4.94745154526473,
-7.0324759230231));
#159232=CARTESIAN_POINT('Ctrl Pts',(-1.76414371081914,4.94771235963237,
-7.03209068951155));
#159233=CARTESIAN_POINT('Ctrl Pts',(-1.76567788,4.947973174,-7.031705456));
#159234=CARTESIAN_POINT('Ctrl Pts',(-1.919292207,4.97408817100001,-6.993132535));
#159235=CARTESIAN_POINT('Ctrl Pts',(-2.07107546,5.00031307,-6.947887912));
#159236=CARTESIAN_POINT('Ctrl Pts',(-1.82587816458829,4.94745154526473,
-7.07038541198959));
#159237=CARTESIAN_POINT('Ctrl Pts',(-1.82742059879415,4.94771235963237,
-7.06998637099479));
#159238=CARTESIAN_POINT('Ctrl Pts',(-1.828963033,4.947973174,-7.06958733));
#159239=CARTESIAN_POINT('Ctrl Pts',(-1.983404926,4.97408817100001,-7.029631884));
#159240=CARTESIAN_POINT('Ctrl Pts',(-2.135954579,5.00031307,-6.982969915));
#159241=CARTESIAN_POINT('Origin',(0.0702666180962777,5.08925695913635,0.184140373501591));
#159242=CARTESIAN_POINT('Ctrl Pts',(-1.731219669,4.94766207,-7.086640874));
#159243=CARTESIAN_POINT('Ctrl Pts',(-1.886956709,4.97393188700001,-7.048595341));
#159244=CARTESIAN_POINT('Ctrl Pts',(-2.040872013,5.00031307,-7.003744844));
#159245=CARTESIAN_POINT('Ctrl Pts',(-1.763847811,4.94766207,-7.032164738));
#159246=CARTESIAN_POINT('Ctrl Pts',(-1.918387675,4.97393188700001,-6.993402164));
#159247=CARTESIAN_POINT('Ctrl Pts',(-2.07107546,5.00031307,-6.947887912));
#159248=CARTESIAN_POINT('Ctrl Pts',(-1.76567980883721,4.94797287199132,
-7.03170507974775));
#159249=CARTESIAN_POINT('Ctrl Pts',(-1.76691086312142,4.94882769741292,
-7.03678071229921));
#159250=CARTESIAN_POINT('Ctrl Pts',(-1.76814307271491,4.94967947055106,
-7.04185657940211));
#159251=CARTESIAN_POINT('Ctrl Pts',(-1.76937452674259,4.9505285274352,-7.04693308296692));
#159252=CARTESIAN_POINT('Ctrl Pts',(-1.77051776072215,4.95131675879317,
-7.05164591125135));
#159253=CARTESIAN_POINT('Ctrl Pts',(-1.77166034377292,4.95210264917935,
-7.05635928958518));
#159254=CARTESIAN_POINT('Ctrl Pts',(-1.772802282163,4.95288622030561,-7.06107320895169));
#159255=CARTESIAN_POINT('Ctrl Pts',(-1.77394422170679,4.95366979222352,
-7.06578713308069));
#159256=CARTESIAN_POINT('Ctrl Pts',(-1.77508551687588,4.95445104507422,
-7.07050159943266));
#159257=CARTESIAN_POINT('Ctrl Pts',(-1.77622617387012,4.95523000030894,
-7.07521659934531));
#159258=CARTESIAN_POINT('Ctrl Pts',(-1.504270571,5.000313899,-7.138261025));
#159259=CARTESIAN_POINT('Ctrl Pts',(-1.613486912,4.98224132,-7.11524548600001));
#159260=CARTESIAN_POINT('Ctrl Pts',(-1.721948015,4.964285714,-7.088899452));
#159261=CARTESIAN_POINT('Ctrl Pts',(-1.772080965,4.955986264,-7.07672177400001));
#159262=CARTESIAN_POINT('Ctrl Pts',(-1.822036668,4.947660853,-7.063836266));
#159263=CARTESIAN_POINT('Ctrl Pts',(-1.4512899,5.000313899,-7.103256832));
#159264=CARTESIAN_POINT('Ctrl Pts',(-1.559970672,4.98224132,-7.081051904));
#159265=CARTESIAN_POINT('Ctrl Pts',(-1.667921256,4.964285714,-7.055532488));
#159266=CARTESIAN_POINT('Ctrl Pts',(-1.717818234,4.955986264,-7.043736889));
#159267=CARTESIAN_POINT('Ctrl Pts',(-1.767543392,4.947660853,-7.031236759));
#159268=CARTESIAN_POINT('Ctrl Pts',(-1.7656778802699,4.9479731738047,-7.03170545720505));
#159269=CARTESIAN_POINT('Ctrl Pts',(-1.71387924127078,4.95664467553049,
-7.04471221882473));
#159270=CARTESIAN_POINT('Ctrl Pts',(-1.66198186828356,4.96527387858945,
-7.05713582273003));
#159271=CARTESIAN_POINT('Ctrl Pts',(-1.55780371363979,4.98260085164332,
-7.08086194272409));
#159272=CARTESIAN_POINT('Ctrl Pts',(-1.50554913342956,4.99129108543522,
-7.09215618765466));
#159273=CARTESIAN_POINT('Ctrl Pts',(-1.45317754970485,5.00000000046694,
-7.10287089874499));
#159274=CARTESIAN_POINT('Ctrl Pts',(-1.4512899,5.000313899,-7.103256832));
#159275=CARTESIAN_POINT('Ctrl Pts',(-1.559970672,4.98224132,-7.081051904));
#159276=CARTESIAN_POINT('Ctrl Pts',(-1.667921256,4.964285714,-7.055532488));
#159277=CARTESIAN_POINT('Ctrl Pts',(-1.71688224,4.95614195,-7.04395815700001));
#159278=CARTESIAN_POINT('Ctrl Pts',(-1.76567788,4.947973174,-7.031705456));
#159279=CARTESIAN_POINT('Ctrl Pts',(-1.41063172,5.000313899,-7.16479510800001));
#159280=CARTESIAN_POINT('Ctrl Pts',(-1.520254036,4.98224132,-7.143212256));
#159281=CARTESIAN_POINT('Ctrl Pts',(-1.629164754,4.964285714,-7.118285819));
#159282=CARTESIAN_POINT('Ctrl Pts',(-1.678561207,4.95614195,-7.106980434));
#159283=CARTESIAN_POINT('Ctrl Pts',(-1.727796006,4.947973174,-7.09499061));
#159284=CARTESIAN_POINT('',(-1.70930637157898,4.94797317334222,-7.12587923944055));
#159285=CARTESIAN_POINT('Ctrl Pts',(-0.856834899,4.818630405,-7.357118544));
#159286=CARTESIAN_POINT('Ctrl Pts',(-0.865603471,4.820029867,-7.35609732600001));
#159287=CARTESIAN_POINT('Ctrl Pts',(-0.874369584,4.821428571,-7.35505521));
#159288=CARTESIAN_POINT('Ctrl Pts',(-1.267257964,4.884117105,-7.308348606));
#159289=CARTESIAN_POINT('Ctrl Pts',(-1.652934871,4.947973174,-7.220053021));
#159290=CARTESIAN_POINT('Ctrl Pts',(-0.989418577999999,4.818630405,-7.182168954));
#159291=CARTESIAN_POINT('Ctrl Pts',(-0.997978637,4.820029867,-7.180989716));
#159292=CARTESIAN_POINT('Ctrl Pts',(-1.00653586,4.821428571,-7.179790078));
#159293=CARTESIAN_POINT('Ctrl Pts',(-1.390062022,4.884117105,-7.126023487));
#159294=CARTESIAN_POINT('Ctrl Pts',(-1.76567788,4.947973174,-7.031705456));
#159295=CARTESIAN_POINT('Ctrl Pts',(-0.994070543748172,4.81939091801866,
-7.18152658130227));
#159296=CARTESIAN_POINT('Ctrl Pts',(-0.996726094868206,4.82234724727202,
-7.19940916869544));
#159297=CARTESIAN_POINT('Ctrl Pts',(-0.999382324343524,4.82527010312014,
-7.2172972388855));
#159298=CARTESIAN_POINT('Ctrl Pts',(-1.00202327928225,4.82816321749345,
-7.2351923419871));
#159299=CARTESIAN_POINT('Ctrl Pts',(-1.00449561666861,4.830871614643,-7.25194489303674));
#159300=CARTESIAN_POINT('Ctrl Pts',(-1.0069586556332,4.83355328551821,-7.26870316048359));
#159301=CARTESIAN_POINT('Ctrl Pts',(-1.00941275741717,4.83620904385919,
-7.2854668165887));
#159302=CARTESIAN_POINT('Ctrl Pts',(-1.01186688554976,4.83886483071389,
-7.3022306526779));
#159303=CARTESIAN_POINT('Ctrl Pts',(-1.01431208269721,4.84149471138868,
-7.31899992217128));
#159304=CARTESIAN_POINT('Ctrl Pts',(-1.01674868753842,4.84409946427727,
-7.33577431846203));
#159305=CARTESIAN_POINT('Ctrl Pts',(-0.364482660369833,4.94924836941368,
-7.39787645705584));
#159306=CARTESIAN_POINT('Ctrl Pts',(-0.368489421684916,4.94861077170684,
-7.39767469852792));
#159307=CARTESIAN_POINT('Ctrl Pts',(-0.372496183,4.947973174,-7.39747294));
#159308=CARTESIAN_POINT('Ctrl Pts',(-0.775478368,4.88384644,-7.377180967));
#159309=CARTESIAN_POINT('Ctrl Pts',(-1.173871557,4.818610636,-7.313233544));
#159310=CARTESIAN_POINT('Ctrl Pts',(-0.204938109066286,4.94924836941368,
-7.24710715016634));
#159311=CARTESIAN_POINT('Ctrl Pts',(-0.208863301533143,4.94861077170684,
-7.24699189558318));
#159312=CARTESIAN_POINT('Ctrl Pts',(-0.212788494,4.947973174,-7.246876641));
#159313=CARTESIAN_POINT('Ctrl Pts',(-0.607566848,4.88384644,-7.235284849));
#159314=CARTESIAN_POINT('Ctrl Pts',(-0.998749843,4.818610636,-7.180877297));
#159315=CARTESIAN_POINT('',(-0.239619539500027,4.94797317334248,-7.2721769681318));
#159316=CARTESIAN_POINT('Ctrl Pts',(-0.209626264033116,4.94745154526473,
-7.24696949288303));
#159317=CARTESIAN_POINT('Ctrl Pts',(-0.211207379016558,4.94771235963237,
-7.24692306694152));
#159318=CARTESIAN_POINT('Ctrl Pts',(-0.212788494,4.947973174,-7.246876641));
#159319=CARTESIAN_POINT('Ctrl Pts',(-0.371103442,4.97408817100001,-7.242228073));
#159320=CARTESIAN_POINT('Ctrl Pts',(-0.529064344,5.00031307,-7.230670157));
#159321=CARTESIAN_POINT('Ctrl Pts',(-0.263266283044498,4.94745154526473,
-7.2975935627527));
#159322=CARTESIAN_POINT('Ctrl Pts',(-0.264858438022249,4.94771235963237,
-7.29753542887635));
#159323=CARTESIAN_POINT('Ctrl Pts',(-0.266450593,4.947973174,-7.297477295));
#159324=CARTESIAN_POINT('Ctrl Pts',(-0.425870961,4.97408817100001,-7.291656427));
#159325=CARTESIAN_POINT('Ctrl Pts',(-0.584885032,5.00031307,-7.278879055));
#159326=CARTESIAN_POINT('Origin',(0.0290390952789225,5.08925700087071,0.194940675385882));
#159327=CARTESIAN_POINT('Ctrl Pts',(-0.167326407,4.94766207,-7.293120202));
#159328=CARTESIAN_POINT('Ctrl Pts',(-0.327601066,4.973931887,-7.289443013));
#159329=CARTESIAN_POINT('Ctrl Pts',(-0.487559448,5.00031307,-7.278728336));
#159330=CARTESIAN_POINT('Ctrl Pts',(-0.21090248,4.94766207,-7.246931774));
#159331=CARTESIAN_POINT('Ctrl Pts',(-0.370162096,4.973931887,-7.242296951));
#159332=CARTESIAN_POINT('Ctrl Pts',(-0.529064344,5.00031307,-7.230670157));
#159333=CARTESIAN_POINT('Ctrl Pts',(-0.212790459169118,4.94797287208577,
-7.24687668792547));
#159334=CARTESIAN_POINT('Ctrl Pts',(-0.21290162157793,4.94882769743312,
-7.25209829529905));
#159335=CARTESIAN_POINT('Ctrl Pts',(-0.213013861400536,4.94967947056244,
-7.25732038006634));
#159336=CARTESIAN_POINT('Ctrl Pts',(-0.213125226487645,4.95052852743733,
-7.26254292398658));
#159337=CARTESIAN_POINT('Ctrl Pts',(-0.213228613500719,4.95131675879874,
-7.26739133052561));
#159338=CARTESIAN_POINT('Ctrl Pts',(-0.213331246546994,4.95210264918784,
-7.27224013431917));
#159339=CARTESIAN_POINT('Ctrl Pts',(-0.213433133688945,4.95288622031736,
-7.2770893279135));
#159340=CARTESIAN_POINT('Ctrl Pts',(-0.213535020933834,4.95366979223853,
-7.28193852640701));
#159341=CARTESIAN_POINT('Ctrl Pts',(-0.213636162297835,4.95445104509289,
-7.28678811592523));
#159342=CARTESIAN_POINT('Ctrl Pts',(-0.213736565703542,4.95523000035635,
-7.29163808949555));
#159343=CARTESIAN_POINT('Ctrl Pts',(0.0654135539999999,5.000313899,-7.29474615600001));
#159344=CARTESIAN_POINT('Ctrl Pts',(-0.0461970310000001,4.98224132,-7.29574699200001));
#159345=CARTESIAN_POINT('Ctrl Pts',(-0.157785991,4.964285714,-7.293332845));
#159346=CARTESIAN_POINT('Ctrl Pts',(-0.209364702,4.955986264,-7.292216977));
#159347=CARTESIAN_POINT('Ctrl Pts',(-0.260922472,4.947660853,-7.290371724));
#159348=CARTESIAN_POINT('Ctrl Pts',(0.1096307,5.000313899,-7.249171064));
#159349=CARTESIAN_POINT('Ctrl Pts',(-0.00128258,4.98224132,-7.250848428));
#159350=CARTESIAN_POINT('Ctrl Pts',(-0.112195259,4.964285714,-7.249131826));
#159351=CARTESIAN_POINT('Ctrl Pts',(-0.163461379,4.955986264,-7.248338377));
#159352=CARTESIAN_POINT('Ctrl Pts',(-0.214711149,4.947660853,-7.24681993199999));
#159353=CARTESIAN_POINT('Ctrl Pts',(-0.212789467012575,4.94797303324862,
-7.24687671705583));
#159354=CARTESIAN_POINT('Ctrl Pts',(-0.179238027472989,4.9534230253913,
-7.24786180670163));
#159355=CARTESIAN_POINT('Ctrl Pts',(-0.145705023109152,4.95886083279325,
-7.24861319334356));
#159356=CARTESIAN_POINT('Ctrl Pts',(-0.112195259296336,4.96428571396278,
-7.24913182606086));
#159357=CARTESIAN_POINT('Ctrl Pts',(-0.0390208298553256,4.97613189092785,
-7.25026435090952));
#159358=CARTESIAN_POINT('Ctrl Pts',(0.0342956684092139,4.98803923897761,
-7.25029060206938));
#159359=CARTESIAN_POINT('Ctrl Pts',(0.107704216070518,5.00000000011363,
-7.24919994256545));
#159360=CARTESIAN_POINT('Ctrl Pts',(0.1096307,5.000313899,-7.249171064));
#159361=CARTESIAN_POINT('Ctrl Pts',(-0.00128258,4.98224132,-7.250848428));
#159362=CARTESIAN_POINT('Ctrl Pts',(-0.112195259,4.964285714,-7.249131826));
#159363=CARTESIAN_POINT('Ctrl Pts',(-0.162499702,4.95614195,-7.248353261));
#159364=CARTESIAN_POINT('Ctrl Pts',(-0.212788494,4.947973174,-7.246876641));
#159365=CARTESIAN_POINT('Ctrl Pts',(0.162567224,5.000313899,-7.300530302));
#159366=CARTESIAN_POINT('Ctrl Pts',(0.050868142,4.98224132,-7.30301760200001));
#159367=CARTESIAN_POINT('Ctrl Pts',(-0.060854751,4.964285714,-7.302086516));
#159368=CARTESIAN_POINT('Ctrl Pts',(-0.111526666,4.95614195,-7.301664223));
#159369=CARTESIAN_POINT('Ctrl Pts',(-0.162187841,4.947973174,-7.30053874));
#159370=CARTESIAN_POINT('',(-0.137490340968732,4.94797317334227,-7.32673048557565));
#159371=CARTESIAN_POINT('Ctrl Pts',(0.744760437,4.818630405,-7.369307376));
#159372=CARTESIAN_POINT('Ctrl Pts',(0.735977338000001,4.820029867,-7.370195018));
#159373=CARTESIAN_POINT('Ctrl Pts',(0.727192148,4.821428571,-7.371061721));
#159374=CARTESIAN_POINT('Ctrl Pts',(0.33344874,4.884117105,-7.409906479));
#159375=CARTESIAN_POINT('Ctrl Pts',(-0.062192196,4.947973174,-7.40658433));
#159376=CARTESIAN_POINT('Ctrl Pts',(0.5776675,4.818630405,-7.226949582));
#159377=CARTESIAN_POINT('Ctrl Pts',(0.56905407,4.820029867,-7.227638074));
#159378=CARTESIAN_POINT('Ctrl Pts',(0.560439023,4.821428571,-7.228306033));
#159379=CARTESIAN_POINT('Ctrl Pts',(0.174321262,4.884117105,-7.258243263));
#159380=CARTESIAN_POINT('Ctrl Pts',(-0.212788494,4.947973174,-7.246876641));
#159381=CARTESIAN_POINT('Ctrl Pts',(0.572986203940172,4.8193909179172,-7.22732226363947));
#159382=CARTESIAN_POINT('Ctrl Pts',(0.57423696565771,4.82234724734176,-7.24535763046555));
#159383=CARTESIAN_POINT('Ctrl Pts',(0.575488243539231,4.8252701031345,-7.26339849828819));
#159384=CARTESIAN_POINT('Ctrl Pts',(0.576755950933578,4.82816321749379,
-7.28144295100099));
#159385=CARTESIAN_POINT('Ctrl Pts',(0.577942718779974,4.83087161464669,
-7.29833531621148));
#159386=CARTESIAN_POINT('Ctrl Pts',(0.579139796495352,4.83355328552718,
-7.31523126528801));
#159387=CARTESIAN_POINT('Ctrl Pts',(0.580346760832532,4.83620904387485,
-7.33213055581014));
#159388=CARTESIAN_POINT('Ctrl Pts',(0.581553738128358,4.83886483073622,
-7.34903002777252));
#159389=CARTESIAN_POINT('Ctrl Pts',(0.582770605614413,4.84149471141908,
-7.36593288621209));
#159390=CARTESIAN_POINT('Ctrl Pts',(0.583996966610964,4.84409946429569,
-7.38283890436021));
#159391=CARTESIAN_POINT('Ctrl Pts',(1.23436350016688,4.94924836941368,-7.30327121457896));
#159392=CARTESIAN_POINT('Ctrl Pts',(1.23040704258344,4.94861077170685,-7.30393550828948));
#159393=CARTESIAN_POINT('Ctrl Pts',(1.226450585,4.947973174,-7.304599802));
#159394=CARTESIAN_POINT('Ctrl Pts',(0.828527725,4.88384644,-7.371411501));
#159395=CARTESIAN_POINT('Ctrl Pts',(0.425701942,4.818610636,-7.394601894));
#159396=CARTESIAN_POINT('Ctrl Pts',(1.35776704393169,4.94924836941368,-7.12172944830898));
#159397=CARTESIAN_POINT('Ctrl Pts',(1.35390884396585,4.94861077170685,-7.12246068865449));
#159398=CARTESIAN_POINT('Ctrl Pts',(1.350050644,4.947973174,-7.123191929));
#159399=CARTESIAN_POINT('Ctrl Pts',(0.962010097,4.88384644,-7.196736822));
#159400=CARTESIAN_POINT('Ctrl Pts',(0.568276727,4.818610636,-7.227694069));
#159401=CARTESIAN_POINT('',(1.32928571593438,4.94797317334254,-7.15366863026892));
#159402=CARTESIAN_POINT('Ctrl Pts',(1.35315890319367,4.94745154526474,-7.12260282408957));
#159403=CARTESIAN_POINT('Ctrl Pts',(1.35160477359683,4.94771235963237,-7.12289737654479));
#159404=CARTESIAN_POINT('Ctrl Pts',(1.350050644,4.947973174,-7.123191929));
#159405=CARTESIAN_POINT('Ctrl Pts',(1.194437707,4.974088171,-7.152685076));
#159406=CARTESIAN_POINT('Ctrl Pts',(1.037685233,5.00031307,-7.175354302));
#159407=CARTESIAN_POINT('Ctrl Pts',(1.31165563666942,4.94745154526474,-7.18357434997128));
#159408=CARTESIAN_POINT('Ctrl Pts',(1.31008820833471,4.94771235963237,-7.18385984148564));
#159409=CARTESIAN_POINT('Ctrl Pts',(1.30852078,4.947973174,-7.184145333));
#159410=CARTESIAN_POINT('Ctrl Pts',(1.151576258,4.974088171,-7.21273122));
#159411=CARTESIAN_POINT('Ctrl Pts',(0.99353309,5.00031307,-7.2344359));
#159412=CARTESIAN_POINT('Origin',(-0.0135462464901456,5.08925699491388,
0.196625289502568));
#159413=CARTESIAN_POINT('Ctrl Pts',(1.404390852,4.94766207,-7.158581336));
#159414=CARTESIAN_POINT('Ctrl Pts',(1.247072838,4.97393188700001,-7.189444432));
#159415=CARTESIAN_POINT('Ctrl Pts',(1.088550856,5.00031307,-7.213366582));
#159416=CARTESIAN_POINT('Ctrl Pts',(1.351904417,4.94766207,-7.122840336));
#159417=CARTESIAN_POINT('Ctrl Pts',(1.195371852,4.97393188700001,-7.152549982));
#159418=CARTESIAN_POINT('Ctrl Pts',(1.037685233,5.00031307,-7.175354302));
#159419=CARTESIAN_POINT('Ctrl Pts',(1.35004873535491,4.94797287208564,-7.12319239739961));
#159420=CARTESIAN_POINT('Ctrl Pts',(1.35106266313749,4.94882769744714,-7.12831582295565));
#159421=CARTESIAN_POINT('Ctrl Pts',(1.35207564124165,4.94967947059234,-7.13343994654348));
#159422=CARTESIAN_POINT('Ctrl Pts',(1.35308957235425,4.95052852748342,-7.13856433053091));
#159423=CARTESIAN_POINT('Ctrl Pts',(1.35403086651912,4.95131675884083,-7.14332160909344));
#159424=CARTESIAN_POINT('Ctrl Pts',(1.35497298243889,4.95210264922691,-7.14807911356628));
#159425=CARTESIAN_POINT('Ctrl Pts',(1.35591591063016,4.95288622035062,-7.1528368383776));
#159426=CARTESIAN_POINT('Ctrl Pts',(1.35685883977408,4.95366979226598,-7.15759456799571));
#159427=CARTESIAN_POINT('Ctrl Pts',(1.35780258142974,4.95445104511169,-7.16235251915265));
#159428=CARTESIAN_POINT('Ctrl Pts',(1.35874712633804,4.95523000034704,-7.16711068663691));
#159429=CARTESIAN_POINT('Ctrl Pts',(1.632039014,5.000313899,-7.110137064));
#159430=CARTESIAN_POINT('Ctrl Pts',(1.523252973,4.98224132,-7.13510747800001));
#159431=CARTESIAN_POINT('Ctrl Pts',(1.41375393,4.964285714,-7.1567381));
#159432=CARTESIAN_POINT('Ctrl Pts',(1.363141222,4.955986264,-7.16673621900001));
#159433=CARTESIAN_POINT('Ctrl Pts',(1.312392169,4.947660853,-7.176017503));
#159434=CARTESIAN_POINT('Ctrl Pts',(1.665425089,5.000313899,-7.056122113));
#159435=CARTESIAN_POINT('Ctrl Pts',(1.557465485,4.98224132,-7.081603338));
#159436=CARTESIAN_POINT('Ctrl Pts',(1.448776863,4.964285714,-7.103769816));
#159437=CARTESIAN_POINT('Ctrl Pts',(1.398538749,4.955986264,-7.114015618));
#159438=CARTESIAN_POINT('Ctrl Pts',(1.34816075,4.947660853,-7.123549859));
#159439=CARTESIAN_POINT('Ctrl Pts',(1.35004971036774,4.94797303321381,-7.12319221260434));
#159440=CARTESIAN_POINT('Ctrl Pts',(1.38302850103403,4.95342302536017,-7.11694170312311));
#159441=CARTESIAN_POINT('Ctrl Pts',(1.41593904815349,4.95886083277475,-7.1104669176639));
#159442=CARTESIAN_POINT('Ctrl Pts',(1.44877686326084,4.96428571408279,-7.10376981626125));
#159443=CARTESIAN_POINT('Ctrl Pts',(1.52048397699665,4.97613189137991,-7.08914552447998));
#159444=CARTESIAN_POINT('Ctrl Pts',(1.59209201781199,4.9880392390861,-7.07341028179112));
#159445=CARTESIAN_POINT('Ctrl Pts',(1.66354985423409,5.0000000002771,-7.05656445327241));
#159446=CARTESIAN_POINT('Ctrl Pts',(1.665425089,5.000313899,-7.056122113));
#159447=CARTESIAN_POINT('Ctrl Pts',(1.557465485,4.98224132,-7.081603338));
#159448=CARTESIAN_POINT('Ctrl Pts',(1.448776863,4.964285714,-7.103769816));
#159449=CARTESIAN_POINT('Ctrl Pts',(1.399481142,4.95614195,-7.113823422));
#159450=CARTESIAN_POINT('Ctrl Pts',(1.350050644,4.947973174,-7.123191929));
#159451=CARTESIAN_POINT('Ctrl Pts',(1.728164706,5.000313899,-7.094900813));
#159452=CARTESIAN_POINT('Ctrl Pts',(1.619611782,4.98224132,-7.121341962));
#159453=CARTESIAN_POINT('Ctrl Pts',(1.510300752,4.964285714,-7.144449764));
#159454=CARTESIAN_POINT('Ctrl Pts',(1.460722737,4.95614195,-7.154930307));
#159455=CARTESIAN_POINT('Ctrl Pts',(1.411004048,4.947973174,-7.164721793));
#159456=CARTESIAN_POINT('',(1.44075458445333,4.94797317334226,-7.18499195770727));
#159457=CARTESIAN_POINT('Ctrl Pts',(2.311531602,4.818630405,-7.036915586));
#159458=CARTESIAN_POINT('Ctrl Pts',(2.303144664,4.820029867,-7.039670582));
#159459=CARTESIAN_POINT('Ctrl Pts',(2.294751182,4.821428571,-7.042405578));
#159460=CARTESIAN_POINT('Ctrl Pts',(1.918563751,4.884117105,-7.164985361));
#159461=CARTESIAN_POINT('Ctrl Pts',(1.531458517,4.947973174,-7.246791988));
#159462=CARTESIAN_POINT('Ctrl Pts',(2.117742488,4.818630405,-6.93380608));
#159463=CARTESIAN_POINT('Ctrl Pts',(2.10947844,4.820029867,-6.936330109));
#159464=CARTESIAN_POINT('Ctrl Pts',(2.1012084,4.821428571,-6.938834431));
#159465=CARTESIAN_POINT('Ctrl Pts',(1.730553477,4.884117105,-7.05107565));
#159466=CARTESIAN_POINT('Ctrl Pts',(1.350050644,4.947973174,-7.123191929));
#159467=CARTESIAN_POINT('Ctrl Pts',(2.11325075290604,4.81939091791738,-6.93517638941566));
#159468=CARTESIAN_POINT('Ctrl Pts',(2.11834934301391,4.8223472472358,-6.95252122234189));
#159469=CARTESIAN_POINT('Ctrl Pts',(2.1234496207869,4.82527010317062,-6.96987131670068));
#159470=CARTESIAN_POINT('Ctrl Pts',(2.12856671375808,4.82816321752733,-6.98722138055105));
#159471=CARTESIAN_POINT('Ctrl Pts',(2.13335709474407,4.83087161467446,-7.00346369165283));
#159472=CARTESIAN_POINT('Ctrl Pts',(2.13815831498521,4.83355328554903,-7.01970728651488));
#159473=CARTESIAN_POINT('Ctrl Pts',(2.14296990901817,4.83620904389083,-7.03595201936947));
#159474=CARTESIAN_POINT('Ctrl Pts',(2.14778155471109,4.83886483074633,-7.05219692663661));
#159475=CARTESIAN_POINT('Ctrl Pts',(2.15260358736129,4.84149471142336,-7.06844301510797));
#159476=CARTESIAN_POINT('Ctrl Pts',(2.15743557083302,4.84409946430342,-7.08469014864696));
#159477=CARTESIAN_POINT('Ctrl Pts',(2.77549219559838,4.94924836941368,-6.86717312735757));
#159478=CARTESIAN_POINT('Ctrl Pts',(2.77177104129919,4.94861077170685,-6.86867241167878));
#159479=CARTESIAN_POINT('Ctrl Pts',(2.768049887,4.947973174,-6.870171696));
#159480=CARTESIAN_POINT('Ctrl Pts',(2.393792782,4.88384644,-7.020963027));
#159481=CARTESIAN_POINT('Ctrl Pts',(2.005370091,4.818610636,-7.130206877));
#159482=CARTESIAN_POINT('Ctrl Pts',(2.85698451967887,4.94924836941368,-6.66334759239431));
#159483=CARTESIAN_POINT('Ctrl Pts',(2.85337371733943,4.94861077170685,-6.66489113569716));
#159484=CARTESIAN_POINT('Ctrl Pts',(2.849762915,4.947973174,-6.666434679));
#159485=CARTESIAN_POINT('Ctrl Pts',(2.486604518,4.88384644,-6.821677381));
#159486=CARTESIAN_POINT('Ctrl Pts',(2.108731308,4.818610636,-6.93655190100001));
#159487=CARTESIAN_POINT('',(2.83603504918524,4.94797317334254,-6.70066269744023));
#159488=CARTESIAN_POINT('Ctrl Pts',(2.85267186467479,4.94745154526474,-6.66519116319149));
#159489=CARTESIAN_POINT('Ctrl Pts',(2.8512173898374,4.94771235963237,-6.66581292109574));
#159490=CARTESIAN_POINT('Ctrl Pts',(2.849762915,4.947973174,-6.66643467899999));
#159491=CARTESIAN_POINT('Ctrl Pts',(2.704128277,4.974088171,-6.728690474));
#159492=CARTESIAN_POINT('Ctrl Pts',(2.555913802,5.00031307,-6.784526854));
#159493=CARTESIAN_POINT('Ctrl Pts',(2.82524599699793,4.94745154526474,-6.73365918371558));
#159494=CARTESIAN_POINT('Ctrl Pts',(2.82377658649896,4.94771235963237,-6.73427495135779));
#159495=CARTESIAN_POINT('Ctrl Pts',(2.822307176,4.947973174,-6.734890719));
#159496=CARTESIAN_POINT('Ctrl Pts',(2.67517705,4.974088171,-6.796546717));
#159497=CARTESIAN_POINT('Ctrl Pts',(2.525494709,5.00031307,-6.851718563));
#159498=CARTESIAN_POINT('Origin',(-0.0554978882862017,5.08925696267246,
0.189115584010757));
#159499=CARTESIAN_POINT('Ctrl Pts',(2.910440355,4.94766207,-6.68931516300001));
#159500=CARTESIAN_POINT('Ctrl Pts',(2.763435003,4.973931887,-6.75327541900001));
#159501=CARTESIAN_POINT('Ctrl Pts',(2.613761731,5.00031307,-6.810715823));
#159502=CARTESIAN_POINT('Ctrl Pts',(2.851497765,4.94766207,-6.665692799));
#159503=CARTESIAN_POINT('Ctrl Pts',(2.705011541,4.973931887,-6.728357725));
#159504=CARTESIAN_POINT('Ctrl Pts',(2.555913802,5.00031307,-6.784526854));
#159505=CARTESIAN_POINT('Ctrl Pts',(2.84976115133646,4.94797287201019,-6.66643554643429));
#159506=CARTESIAN_POINT('Ctrl Pts',(2.85185275935425,4.94882769742881,-6.67122122457105));
#159507=CARTESIAN_POINT('Ctrl Pts',(2.85394358965563,4.94967947057215,-6.67600778869325));
#159508=CARTESIAN_POINT('Ctrl Pts',(2.85603540668187,4.95052852746016,-6.68079440224708));
#159509=CARTESIAN_POINT('Ctrl Pts',(2.85797736816239,4.95131675881625,-6.68523810789968));
#159510=CARTESIAN_POINT('Ctrl Pts',(2.85992018076595,4.95210264919987,-6.68968185751783));
#159511=CARTESIAN_POINT('Ctrl Pts',(2.8618638340298,4.95288622032081,-6.69412564770306));
#159512=CARTESIAN_POINT('Ctrl Pts',(2.86380748925736,4.9536697922334,-6.69856944237792));
#159513=CARTESIAN_POINT('Ctrl Pts',(2.86575198563786,4.95445104507607,-6.70301327874052));
#159514=CARTESIAN_POINT('Ctrl Pts',(2.86769731302196,4.9552300003156,-6.70745715373435));
#159515=CARTESIAN_POINT('Ctrl Pts',(3.122352143,5.000313899,-6.593065866));
#159516=CARTESIAN_POINT('Ctrl Pts',(3.02147736,4.98224132,-6.640838268));
#159517=CARTESIAN_POINT('Ctrl Pts',(2.919188289,4.964285714,-6.685502236));
#159518=CARTESIAN_POINT('Ctrl Pts',(2.871908178,4.955986264,-6.70614684));
#159519=CARTESIAN_POINT('Ctrl Pts',(2.824340811,4.947660853,-6.72612067900001));
#159520=CARTESIAN_POINT('Ctrl Pts',(3.143346053,5.000313899,-6.533136734));
#159521=CARTESIAN_POINT('Ctrl Pts',(3.043388194,4.98224132,-6.581230346));
#159522=CARTESIAN_POINT('Ctrl Pts',(2.94200579,4.964285714,-6.626243425));
#159523=CARTESIAN_POINT('Ctrl Pts',(2.895144759,4.955986264,-6.647049396));
#159524=CARTESIAN_POINT('Ctrl Pts',(2.84799415,4.947660853,-6.667190512));
#159525=CARTESIAN_POINT('Ctrl Pts',(2.84976291533748,4.94797317387187,-6.66643467973655));
#159526=CARTESIAN_POINT('Ctrl Pts',(2.89887082684445,4.95664467876409,-6.64544206388029));
#159527=CARTESIAN_POINT('Ctrl Pts',(2.94770441222799,4.96527388208562,-6.62392545570605));
#159528=CARTESIAN_POINT('Ctrl Pts',(3.04499834694427,4.98260085372362,-6.57976772645109));
#159529=CARTESIAN_POINT('Ctrl Pts',(3.0934328535996,4.99129108975406,-6.55713586568035));
#159530=CARTESIAN_POINT('Ctrl Pts',(3.14160975151107,5.00000000050473,-6.53397185204522));
#159531=CARTESIAN_POINT('Ctrl Pts',(3.143346053,5.000313899,-6.533136734));
#159532=CARTESIAN_POINT('Ctrl Pts',(3.043388194,4.98224132,-6.581230346));
#159533=CARTESIAN_POINT('Ctrl Pts',(2.94200579,4.964285714,-6.626243425));
#159534=CARTESIAN_POINT('Ctrl Pts',(2.896023804,4.95614195,-6.646659106));
#159535=CARTESIAN_POINT('Ctrl Pts',(2.849762915,4.947973174,-6.66643467900001));
#159536=CARTESIAN_POINT('Ctrl Pts',(3.212955126,5.000313899,-6.557521647));
#159537=CARTESIAN_POINT('Ctrl Pts',(3.112624175,4.98224132,-6.606680287));
#159538=CARTESIAN_POINT('Ctrl Pts',(3.01083627,4.964285714,-6.652746481));
#159539=CARTESIAN_POINT('Ctrl Pts',(2.964670369,4.95614195,-6.673639803));
#159540=CARTESIAN_POINT('Ctrl Pts',(2.918218955,4.947973174,-6.693890418));
#159541=CARTESIAN_POINT('',(2.95163142719041,4.94797317334227,-6.70729119137599));
#159542=CARTESIAN_POINT('Ctrl Pts',(3.770218119,4.818630405,-6.375485444));
#159543=CARTESIAN_POINT('Ctrl Pts',(3.762619505,4.820029867,-6.379978973));
#159544=CARTESIAN_POINT('Ctrl Pts',(3.755010202,4.821428571,-6.384454377));
#159545=CARTESIAN_POINT('Ctrl Pts',(3.413968854,4.884117105,-6.585037491));
#159546=CARTESIAN_POINT('Ctrl Pts',(3.053499932,4.947973174,-6.748147707));
#159547=CARTESIAN_POINT('Ctrl Pts',(3.558794191,4.818630405,-6.316445512));
#159548=CARTESIAN_POINT('Ctrl Pts',(3.551265944,4.820029867,-6.320687056));
#159549=CARTESIAN_POINT('Ctrl Pts',(3.543727607,4.821428571,-6.324910643));
#159550=CARTESIAN_POINT('Ctrl Pts',(3.205866935,4.884117105,-6.514207577));
#159551=CARTESIAN_POINT('Ctrl Pts',(2.849762915,4.947973174,-6.666434679));
#159552=CARTESIAN_POINT('Ctrl Pts',(3.55470204599044,4.8193909179173,-6.31874937381797));
#159553=CARTESIAN_POINT('Ctrl Pts',(3.5634100609705,4.82234724728643,-6.3345926481873));
#159554=CARTESIAN_POINT('Ctrl Pts',(3.57212085391211,4.82527010311282,-6.35044069837409));
#159555=CARTESIAN_POINT('Ctrl Pts',(3.58084806296071,4.82816321747262,-6.3662851036461));
#159556=CARTESIAN_POINT('Ctrl Pts',(3.58901806429448,4.8308716146299,-6.38111788827223));
#159557=CARTESIAN_POINT('Ctrl Pts',(3.59719892743765,4.83355328551375,-6.39594959652601));
#159558=CARTESIAN_POINT('Ctrl Pts',(3.60539016647409,4.83620904386399,-6.41078018610813));
#159559=CARTESIAN_POINT('Ctrl Pts',(3.61358149345627,4.83886483072794,-6.42561093491979));
#159560=CARTESIAN_POINT('Ctrl Pts',(3.62178321847861,4.84149471141258,-6.44044060443103));
#159561=CARTESIAN_POINT('Ctrl Pts',(3.62999488635505,4.84409946430512,-6.45526915547616));
#159562=CARTESIAN_POINT('Ctrl Pts',(4.18684196093688,4.94924836941368,-6.10997365687233));
#159563=CARTESIAN_POINT('Ctrl Pts',(4.18353010696844,4.94861077170685,-6.11223782693617));
#159564=CARTESIAN_POINT('Ctrl Pts',(4.180218253,4.947973174,-6.114501997));
#159565=CARTESIAN_POINT('Ctrl Pts',(3.84712675,4.88384644,-6.342222125));
#159566=CARTESIAN_POINT('Ctrl Pts',(3.491269364,4.818610636,-6.532411311));
#159567=CARTESIAN_POINT('Ctrl Pts',(4.22261257419805,4.94924836941368,-5.89339500821419));
#159568=CARTESIAN_POINT('Ctrl Pts',(4.21941800659902,4.94861077170685,-5.8956786801071));
#159569=CARTESIAN_POINT('Ctrl Pts',(4.216223439,4.947973174,-5.897962352));
#159570=CARTESIAN_POINT('Ctrl Pts',(3.894928076,4.88384644,-6.127643887));
#159571=CARTESIAN_POINT('Ctrl Pts',(3.550583958,4.818610636,-6.321064274));
#159572=CARTESIAN_POINT('',(4.21017453526411,4.94797317334248,-5.93434122418425));
#159573=CARTESIAN_POINT('Ctrl Pts',(4.21879705989843,4.94745154526473,-5.89612257069493));
#159574=CARTESIAN_POINT('Ctrl Pts',(4.21751024944921,4.94771235963237,-5.89704246134746));
#159575=CARTESIAN_POINT('Ctrl Pts',(4.216223439,4.947973174,-5.897962352));
#159576=CARTESIAN_POINT('Ctrl Pts',(4.087376814,4.97408817100001,-5.990069784));
#159577=CARTESIAN_POINT('Ctrl Pts',(3.954630682,5.00031307,-6.076462471));
#159578=CARTESIAN_POINT('Ctrl Pts',(4.20673099430623,4.94745154526473,-5.96888559868221));
#159579=CARTESIAN_POINT('Ctrl Pts',(4.20542830965312,4.94771235963237,-5.9698028498411));
#159580=CARTESIAN_POINT('Ctrl Pts',(4.204125625,4.947973174,-5.970720101));
#159581=CARTESIAN_POINT('Ctrl Pts',(4.073689537,4.97408817100001,-6.062563244));
#159582=CARTESIAN_POINT('Ctrl Pts',(3.939367001,5.00031307,-6.148622482));
#159583=CARTESIAN_POINT('Origin',(-0.0948540586112023,5.08925688855765,
0.172762876232048));
#159584=CARTESIAN_POINT('Ctrl Pts',(4.280400903,4.94766207,-5.907264047));
#159585=CARTESIAN_POINT('Ctrl Pts',(4.150582018,4.973931887,-6.001330754));
#159586=CARTESIAN_POINT('Ctrl Pts',(4.016756013,5.00031307,-6.089603562));
#159587=CARTESIAN_POINT('Ctrl Pts',(4.217758247,4.94766207,-5.89686487600001));
#159588=CARTESIAN_POINT('Ctrl Pts',(4.088167896,4.973931887,-5.989554938));
#159589=CARTESIAN_POINT('Ctrl Pts',(3.954630682,5.00031307,-6.076462471));
#159590=CARTESIAN_POINT('Ctrl Pts',(4.21622190306857,4.94797287210893,-5.89796357864352));
#159591=CARTESIAN_POINT('Ctrl Pts',(4.21929338956627,4.94882769744785,-5.90218773665338));
#159592=CARTESIAN_POINT('Ctrl Pts',(4.22236430733007,4.94967947058069,-5.9064129267227));
#159593=CARTESIAN_POINT('Ctrl Pts',(4.22543619933326,4.95052852745714,-5.91063795296052));
#159594=CARTESIAN_POINT('Ctrl Pts',(4.22828802432798,4.95131675882064,-5.91456030290507));
#159595=CARTESIAN_POINT('Ctrl Pts',(4.23114068995999,4.95210264921027,-5.91848251282697));
#159596=CARTESIAN_POINT('Ctrl Pts',(4.23399418529024,4.95288622033926,-5.92240458167081));
#159597=CARTESIAN_POINT('Ctrl Pts',(4.2368476835034,4.9536697922599,-5.92632665447713));
#159598=CARTESIAN_POINT('Ctrl Pts',(4.23970201213683,4.95445104511264,-5.93024858719394));
#159599=CARTESIAN_POINT('Ctrl Pts',(4.24255716059392,4.95523000035748,-5.9341703789812));
#159600=CARTESIAN_POINT('Ctrl Pts',(4.466667556,5.000313899,-5.767710235));
#159601=CARTESIAN_POINT('Ctrl Pts',(4.378420824,4.98224132,-5.836050841));
#159602=CARTESIAN_POINT('Ctrl Pts',(4.288124647,4.964285714,-5.901659717));
#159603=CARTESIAN_POINT('Ctrl Pts',(4.246387899,4.955986264,-5.931985488));
#159604=CARTESIAN_POINT('Ctrl Pts',(4.204226416,4.947660853,-5.961717928));
#159605=CARTESIAN_POINT('Ctrl Pts',(4.474287649,5.000313899,-5.704669143));
#159606=CARTESIAN_POINT('Ctrl Pts',(4.387005454,4.98224132,-5.773126338));
#159607=CARTESIAN_POINT('Ctrl Pts',(4.297669796,4.964285714,-5.838881257));
#159608=CARTESIAN_POINT('Ctrl Pts',(4.256377018,4.955986264,-5.869274531));
#159609=CARTESIAN_POINT('Ctrl Pts',(4.214658508,4.947660853,-5.899080747));
#159610=CARTESIAN_POINT('Ctrl Pts',(4.21622343934038,4.94797317391062,-5.89796235245119));
#159611=CARTESIAN_POINT('Ctrl Pts',(4.25967046514281,4.95664468310041,-5.86690376849364));
#159612=CARTESIAN_POINT('Ctrl Pts',(4.30273688556295,4.96527388072572,-5.83539245009048));
#159613=CARTESIAN_POINT('Ctrl Pts',(4.38826353175028,4.98260085161193,-5.77135178628772));
#159614=CARTESIAN_POINT('Ctrl Pts',(4.43070047526962,4.99129108540162,-5.73883706723313));
#159615=CARTESIAN_POINT('Ctrl Pts',(4.47277146646463,5.00000000040085,-5.70585799033773));
#159616=CARTESIAN_POINT('Ctrl Pts',(4.474287649,5.000313899,-5.704669143));
#159617=CARTESIAN_POINT('Ctrl Pts',(4.387005454,4.98224132,-5.773126338));
#159618=CARTESIAN_POINT('Ctrl Pts',(4.297669796,4.964285714,-5.838881257));
#159619=CARTESIAN_POINT('Ctrl Pts',(4.25715161,4.95614195,-5.868704398));
#159620=CARTESIAN_POINT('Ctrl Pts',(4.216223439,4.947973174,-5.897962352));
#159621=CARTESIAN_POINT('Ctrl Pts',(4.547511336,5.000313899,-5.713520057));
#159622=CARTESIAN_POINT('Ctrl Pts',(4.460093721,4.98224132,-5.783097584));
#159623=CARTESIAN_POINT('Ctrl Pts',(4.370588431,4.964285714,-5.849968167));
#159624=CARTESIAN_POINT('Ctrl Pts',(4.32999331,4.95614195,-5.880297318));
#159625=CARTESIAN_POINT('Ctrl Pts',(4.288981187,4.947973174,-5.910060166));
#159626=CARTESIAN_POINT('',(4.32449326475501,4.94797317334227,-5.91596494312064));
#159627=CARTESIAN_POINT('Ctrl Pts',(5.052613427,4.818630405,-5.415944688));
#159628=CARTESIAN_POINT('Ctrl Pts',(5.046158441,4.820029867,-5.421966639));
#159629=CARTESIAN_POINT('Ctrl Pts',(5.039689118,4.821428571,-5.427973185));
#159630=CARTESIAN_POINT('Ctrl Pts',(4.749740568,4.884117105,-5.697180586));
#159631=CARTESIAN_POINT('Ctrl Pts',(4.432763084,4.947973174,-5.933967539));
#159632=CARTESIAN_POINT('Ctrl Pts',(4.833440632,4.818630405,-5.403734972));
#159633=CARTESIAN_POINT('Ctrl Pts',(4.827000198,4.820029867,-5.409495702));
#159634=CARTESIAN_POINT('Ctrl Pts',(4.82054605,4.821428571,-5.415241063));
#159635=CARTESIAN_POINT('Ctrl Pts',(4.531277618,4.884117105,-5.672742398));
#159636=CARTESIAN_POINT('Ctrl Pts',(4.216223439,4.947973174,-5.897962352));
#159637=CARTESIAN_POINT('Ctrl Pts',(4.82993942163252,4.81939091791738,-5.4068646610732));
#159638=CARTESIAN_POINT('Ctrl Pts',(4.84184968410277,4.82234724721574,-5.42046556271523));
#159639=CARTESIAN_POINT('Ctrl Pts',(4.8537636861635,4.82527010310443,-5.43407053107029));
#159640=CARTESIAN_POINT('Ctrl Pts',(4.86569293671696,4.82816321746756,-5.44766841099453));
#159641=CARTESIAN_POINT('Ctrl Pts',(4.87686053821621,4.83087161462581,-5.46039810457822));
#159642=CARTESIAN_POINT('Ctrl Pts',(4.8880385161992,4.83355328551165,-5.47312441198141));
#159643=CARTESIAN_POINT('Ctrl Pts',(4.89922638701532,4.8362090438646,-5.48584739635302));
#159644=CARTESIAN_POINT('Ctrl Pts',(4.9104143779507,4.83886483073126,-5.49857051732573));
#159645=CARTESIAN_POINT('Ctrl Pts',(4.92161229181196,4.84149471141935,-5.51129034895669));
#159646=CARTESIAN_POINT('Ctrl Pts',(4.93281967559905,4.84409946430769,-5.52400695080939));
#159647=CARTESIAN_POINT('Ctrl Pts',(5.40241964904355,4.94924836941368,-5.06707860853674));
#159648=CARTESIAN_POINT('Ctrl Pts',(5.39967195402178,4.94861077170685,-5.07000179426837));
#159649=CARTESIAN_POINT('Ctrl Pts',(5.396924259,4.947973174,-5.07292498));
#159650=CARTESIAN_POINT('Ctrl Pts',(5.120573347,4.88384644,-5.36692596499999));
#159651=CARTESIAN_POINT('Ctrl Pts',(4.81392076200001,4.818610636,-5.629167453));
#159652=CARTESIAN_POINT('Ctrl Pts',(5.39079595785796,4.94924836941368,-4.84787382396709));
#159653=CARTESIAN_POINT('Ctrl Pts',(5.38816699942898,4.94861077170685,-4.85079084248354));
#159654=CARTESIAN_POINT('Ctrl Pts',(5.385538041,4.947973174,-4.853707861));
#159655=CARTESIAN_POINT('Ctrl Pts',(5.121129126,4.88384644,-5.147088575));
#159656=CARTESIAN_POINT('Ctrl Pts',(4.826415248,4.818610636,-5.410010708));
#159657=CARTESIAN_POINT('',(5.3874509396897,4.94797317334254,-4.89053655053701));
#159658=CARTESIAN_POINT('Ctrl Pts',(5.38765599348884,4.94745154526474,-4.8513578403444));
#159659=CARTESIAN_POINT('Ctrl Pts',(5.38659701724442,4.94771235963237,-4.8525328506722));
#159660=CARTESIAN_POINT('Ctrl Pts',(5.385538041,4.947973174,-4.853707861));
#159661=CARTESIAN_POINT('Ctrl Pts',(5.279504153,4.974088171,-4.971360088));
#159662=CARTESIAN_POINT('Ctrl Pts',(5.168433427,5.00031307,-5.084269457));
#159663=CARTESIAN_POINT('Ctrl Pts',(5.39151392645153,4.94745154526474,-4.92501355593251));
#159664=CARTESIAN_POINT('Ctrl Pts',(5.39043887972577,4.94771235963237,-4.92618940096626));
#159665=CARTESIAN_POINT('Ctrl Pts',(5.389363833,4.947973174,-4.927365246));
#159666=CARTESIAN_POINT('Ctrl Pts',(5.281720829,4.974088171,-5.045101051));
#159667=CARTESIAN_POINT('Ctrl Pts',(5.169038872,5.00031307,-5.15802364600001));
#159668=CARTESIAN_POINT('Origin',(-0.129776799267178,5.08925709704122,0.148334366254367));
#159669=CARTESIAN_POINT('Ctrl Pts',(5.450214661,4.94766207,-4.84899583));
#159670=CARTESIAN_POINT('Ctrl Pts',(5.343652431,4.97393188700001,-4.968770532));
#159671=CARTESIAN_POINT('Ctrl Pts',(5.231931248,5.00031307,-5.083748206));
#159672=CARTESIAN_POINT('Ctrl Pts',(5.386801042,4.94766207,-4.852306105));
#159673=CARTESIAN_POINT('Ctrl Pts',(5.28016606400001,4.97393188700001,-4.97068722));
#159674=CARTESIAN_POINT('Ctrl Pts',(5.168433427,5.00031307,-5.084269457));
#159675=CARTESIAN_POINT('Ctrl Pts',(5.38553680511737,4.94797287199671,-4.85370938913422));
#159676=CARTESIAN_POINT('Ctrl Pts',(5.38944455129704,4.94882769741461,-4.85717450974945));
#159677=CARTESIAN_POINT('Ctrl Pts',(5.39335196362416,4.94967947056355,-4.86064076076593));
#159678=CARTESIAN_POINT('Ctrl Pts',(5.39726029218899,4.95052852745504,-4.86410664233588));
#159679=CARTESIAN_POINT('Ctrl Pts',(5.40088863229767,4.95131675882372,-4.86732423187668));
#159680=CARTESIAN_POINT('Ctrl Pts',(5.40451776328343,4.95210264921743,-4.87054150394423));
#159681=CARTESIAN_POINT('Ctrl Pts',(5.40814767425038,4.95288622034999,-4.87375845986201));
#159682=CARTESIAN_POINT('Ctrl Pts',(5.41177758888466,4.95366979227421,-4.87697541902991));
#159683=CARTESIAN_POINT('Ctrl Pts',(5.41540828441786,4.95445104513005,-4.88019206285825));
#159684=CARTESIAN_POINT('Ctrl Pts',(5.4190397503672,4.95523000038511,-4.88340839283606));
#159685=CARTESIAN_POINT('Ctrl Pts',(5.602126559,5.000313899,-4.672662884));
#159686=CARTESIAN_POINT('Ctrl Pts',(5.530634197,4.98224132,-4.758376164));
#159687=CARTESIAN_POINT('Ctrl Pts',(5.456553063,4.964285714,-4.84186215));
#159688=CARTESIAN_POINT('Ctrl Pts',(5.422311241,4.955986264,-4.880451088));
#159689=CARTESIAN_POINT('Ctrl Pts',(5.387527066,4.947660853,-4.918551872));
#159690=CARTESIAN_POINT('Ctrl Pts',(5.596016527,5.000313899,-4.609457563));
#159691=CARTESIAN_POINT('Ctrl Pts',(5.52549121500001,4.98224132,-4.695077359));
#159692=CARTESIAN_POINT('Ctrl Pts',(5.452379538,4.964285714,-4.77849949));
#159693=CARTESIAN_POINT('Ctrl Pts',(5.418585819,4.955986264,-4.817058913));
#159694=CARTESIAN_POINT('Ctrl Pts',(5.38425012,4.947660853,-4.855136522));
#159695=CARTESIAN_POINT('Ctrl Pts',(5.38553746950781,4.94797303313041,-4.85370865194204));
#159696=CARTESIAN_POINT('Ctrl Pts',(5.4080090089543,4.9534230252675,-4.82877475100876));
#159697=CARTESIAN_POINT('Ctrl Pts',(5.43029049427791,4.95886083271017,-4.80370360501776));
#159698=CARTESIAN_POINT('Ctrl Pts',(5.45237953810033,4.96428571402229,-4.77849949004151));
#159699=CARTESIAN_POINT('Ctrl Pts',(5.5006148297591,4.97613189137016,-4.72346189605064));
#159700=CARTESIAN_POINT('Ctrl Pts',(5.54809893169663,4.98803923916643,-4.66759983832208));
#159701=CARTESIAN_POINT('Ctrl Pts',(5.59479135902996,5.00000000040303,-4.61094455025893));
#159702=CARTESIAN_POINT('Ctrl Pts',(5.596016527,5.000313899,-4.609457563));
#159703=CARTESIAN_POINT('Ctrl Pts',(5.52549121500001,4.98224132,-4.695077359));
#159704=CARTESIAN_POINT('Ctrl Pts',(5.452379538,4.964285714,-4.77849949));
#159705=CARTESIAN_POINT('Ctrl Pts',(5.419219739,4.95614195,-4.816335595));
#159706=CARTESIAN_POINT('Ctrl Pts',(5.385538041,4.947973174,-4.853707861));
#159707=CARTESIAN_POINT('Ctrl Pts',(5.66943097000001,5.000313899,-4.60236062));
#159708=CARTESIAN_POINT('Ctrl Pts',(5.599014242,4.98224132,-4.68910366600001));
#159709=CARTESIAN_POINT('Ctrl Pts',(5.525976735,4.964285714,-4.773651843));
#159710=CARTESIAN_POINT('Ctrl Pts',(5.492850576,4.95614195,-4.811998667));
#159711=CARTESIAN_POINT('Ctrl Pts',(5.459195426,4.947973174,-4.84988207));
#159712=CARTESIAN_POINT('',(5.49514660316742,4.94797317334227,-4.84801474947653));
#159713=CARTESIAN_POINT('Ctrl Pts',(6.098754147,4.81863040500001,-4.203160378));
#159714=CARTESIAN_POINT('Ctrl Pts',(6.09374461600001,4.820029867,-4.21042917));
#159715=CARTESIAN_POINT('Ctrl Pts',(6.088717772,4.821428571,-4.217686));
#159716=CARTESIAN_POINT('Ctrl Pts',(5.863419691,4.884117105,-4.542929849));
#159717=CARTESIAN_POINT('Ctrl Pts',(5.60475516,4.947973174,-4.842321644));
#159718=CARTESIAN_POINT('Ctrl Pts',(5.882080762,4.81863040500001,-4.238351791));
#159719=CARTESIAN_POINT('Ctrl Pts',(5.877029288,4.820029867,-4.245362341));
#159720=CARTESIAN_POINT('Ctrl Pts',(5.871961118,4.821428571,-4.25236083));
#159721=CARTESIAN_POINT('Ctrl Pts',(5.64481079600001,4.884117105,-4.566026089));
#159722=CARTESIAN_POINT('Ctrl Pts',(5.385538041,4.947973174,-4.853707861));
#159723=CARTESIAN_POINT('Ctrl Pts',(5.87933419858875,4.8193909179172,-4.24216096606972));
#159724=CARTESIAN_POINT('Ctrl Pts',(5.89388979747093,4.82234724725715,-4.2528835319381));
#159725=CARTESIAN_POINT('Ctrl Pts',(5.90844992258693,4.82527010309212,-4.26360926566706));
#159726=CARTESIAN_POINT('Ctrl Pts',(5.92302341609072,4.82816321745518,-4.27432479842803));
#159727=CARTESIAN_POINT('Ctrl Pts',(5.93666643311167,4.8308716146208,-4.2843561746254));
#159728=CARTESIAN_POINT('Ctrl Pts',(5.95031885609539,4.83355328551246,-4.2943820131668));
#159729=CARTESIAN_POINT('Ctrl Pts',(5.96398022627268,4.83620904386994,-4.30440247969684));
#159730=CARTESIAN_POINT('Ctrl Pts',(5.97764174312615,4.83886483074115,-4.31442305381226));
#159731=CARTESIAN_POINT('Ctrl Pts',(5.99131224380473,4.84149471143251,-4.32443828234945));
#159732=CARTESIAN_POINT('Ctrl Pts',(6.00499129873184,4.84409946432866,-4.33444832088375));
#159733=CARTESIAN_POINT('Ctrl Pts',(6.36538619882948,4.94924836941368,-3.78725259602702));
#159734=CARTESIAN_POINT('Ctrl Pts',(6.36333114191474,4.94861077170685,-3.79069811251351));
#159735=CARTESIAN_POINT('Ctrl Pts',(6.361276085,4.947973174,-3.794143629));
#159736=CARTESIAN_POINT('Ctrl Pts',(6.154587625,4.88384644,-4.140678312));
#159737=CARTESIAN_POINT('Ctrl Pts',(5.911478575,4.818610636,-4.462709981));
#159738=CARTESIAN_POINT('Ctrl Pts',(6.30691171418917,4.94924836941368,-3.57567144780525));
#159739=CARTESIAN_POINT('Ctrl Pts',(6.30497129209459,4.94861077170685,-3.57908541640263));
#159740=CARTESIAN_POINT('Ctrl Pts',(6.30303087000001,4.947973174,-3.582499385));
#159741=CARTESIAN_POINT('Ctrl Pts',(6.107871869,4.88384644,-3.925861122));
#159742=CARTESIAN_POINT('Ctrl Pts',(5.876568725,4.818610636,-4.245991053));
#159743=CARTESIAN_POINT('',(6.31281612599007,4.94797317334248,-3.61805582352771));
#159744=CARTESIAN_POINT('Ctrl Pts',(6.30459412094996,4.94745154526473,-3.57974900934041));
#159745=CARTESIAN_POINT('Ctrl Pts',(6.30381249547498,4.94771235963237,-3.5811241971702));
#159746=CARTESIAN_POINT('Ctrl Pts',(6.30303087,4.947973174,-3.582499385));
#159747=CARTESIAN_POINT('Ctrl Pts',(6.224767747,4.97408817100001,-3.72019512));
#159748=CARTESIAN_POINT('Ctrl Pts',(6.140565969,5.00031307,-3.854341653));
#159749=CARTESIAN_POINT('Ctrl Pts',(6.32419565962129,4.94745154526473,-3.65085335360889));
#159750=CARTESIAN_POINT('Ctrl Pts',(6.32339851881065,4.94771235963237,-3.65223281130444));
#159751=CARTESIAN_POINT('Ctrl Pts',(6.322601378,4.947973174,-3.653612269));
#159752=CARTESIAN_POINT('Ctrl Pts',(6.242784725,4.97408817100001,-3.79173554));
#159753=CARTESIAN_POINT('Ctrl Pts',(6.157012229,5.00031307,-3.926241358));
#159754=CARTESIAN_POINT('Origin',(-0.158628913824926,5.08925704202097,0.116967444023323));
#159755=CARTESIAN_POINT('Ctrl Pts',(6.365182439,4.94766207,-3.563993958));
#159756=CARTESIAN_POINT('Ctrl Pts',(6.286859595,4.973931887,-3.703876123));
#159757=CARTESIAN_POINT('Ctrl Pts',(6.202467193,5.00031307,-3.840182435));
#159758=CARTESIAN_POINT('Ctrl Pts',(6.303963006,4.94766207,-3.580858894));
#159759=CARTESIAN_POINT('Ctrl Pts',(6.225269536,4.973931887,-3.719395692));
#159760=CARTESIAN_POINT('Ctrl Pts',(6.140565969,5.00031307,-3.854341653));
#159761=CARTESIAN_POINT('Ctrl Pts',(6.30302999118404,4.94797287209564,-3.58250114338846));
#159762=CARTESIAN_POINT('Ctrl Pts',(6.3075912746304,4.94882769739619,-3.58504520174211));
#159763=CARTESIAN_POINT('Ctrl Pts',(6.31215247530727,4.94967947051464,-3.58759043548581));
#159764=CARTESIAN_POINT('Ctrl Pts',(6.31671449138878,4.95052852737955,-3.59013511146802));
#159765=CARTESIAN_POINT('Ctrl Pts',(6.32094968965551,4.95131675874445,-3.59249748966149));
#159766=CARTESIAN_POINT('Ctrl Pts',(6.3251855920701,4.95210264913791,-3.59485938779982));
#159767=CARTESIAN_POINT('Ctrl Pts',(6.32942218826612,4.95288622027104,-3.59722080950912));
#159768=CARTESIAN_POINT('Ctrl Pts',(6.3336587887424,4.95366979219581,-3.59958223360419));
#159769=CARTESIAN_POINT('Ctrl Pts',(6.33789608407051,4.95445104505298,-3.60194318186425));
#159770=CARTESIAN_POINT('Ctrl Pts',(6.34213406430118,4.9552300003035,-3.6043036579765));
#159771=CARTESIAN_POINT('Ctrl Pts',(6.475636351,5.000313899,-3.35912701));
#159772=CARTESIAN_POINT('Ctrl Pts',(6.424241261,4.98224132,-3.458205105));
#159773=CARTESIAN_POINT('Ctrl Pts',(6.369839123,4.964285714,-3.555664489));
#159774=CARTESIAN_POINT('Ctrl Pts',(6.344693336,4.955986264,-3.600712219));
#159775=CARTESIAN_POINT('Ctrl Pts',(6.318912939,4.947660853,-3.645399798));
#159776=CARTESIAN_POINT('Ctrl Pts',(6.45608189200001,5.000313899,-3.298712871));
#159777=CARTESIAN_POINT('Ctrl Pts',(6.405611147,4.98224132,-3.397491781));
#159778=CARTESIAN_POINT('Ctrl Pts',(6.352142073,4.964285714,-3.494680397));
#159779=CARTESIAN_POINT('Ctrl Pts',(6.327427568,4.955986264,-3.539602974));
#159780=CARTESIAN_POINT('Ctrl Pts',(6.30208017899999,4.947660853,-3.58417151));
#159781=CARTESIAN_POINT('Ctrl Pts',(6.3030308705642,4.94797317389881,-3.58249938530178));
#159782=CARTESIAN_POINT('Ctrl Pts',(6.32942116704821,4.95664468470342,-3.536068436542));
#159783=CARTESIAN_POINT('Ctrl Pts',(6.35527594017604,4.96527388511,-3.48938640217459));
#159784=CARTESIAN_POINT('Ctrl Pts',(6.40600783802618,4.98260085337293,-3.39535297841428));
#159785=CARTESIAN_POINT('Ctrl Pts',(6.43086999418703,4.99129108928458,-3.3480245972018));
#159786=CARTESIAN_POINT('Ctrl Pts',(6.45520502561423,5.00000000025075,-3.30042846896562));
#159787=CARTESIAN_POINT('Ctrl Pts',(6.45608189200001,5.000313899,-3.298712871));
#159788=CARTESIAN_POINT('Ctrl Pts',(6.405611147,4.98224132,-3.397491781));
#159789=CARTESIAN_POINT('Ctrl Pts',(6.352142073,4.964285714,-3.494680397));
#159790=CARTESIAN_POINT('Ctrl Pts',(6.327891176,4.95614195,-3.538760292));
#159791=CARTESIAN_POINT('Ctrl Pts',(6.30303087,4.947973174,-3.582499385));
#159792=CARTESIAN_POINT('Ctrl Pts',(6.526254313,5.000313899,-3.275999914));
#159793=CARTESIAN_POINT('Ctrl Pts',(6.476131079,4.98224132,-3.375852472));
#159794=CARTESIAN_POINT('Ctrl Pts',(6.422976508,4.964285714,-3.474124865));
#159795=CARTESIAN_POINT('Ctrl Pts',(6.39886825300001,4.95614195,-3.518696306));
#159796=CARTESIAN_POINT('Ctrl Pts',(6.374143754,4.947973174,-3.562928878));
#159797=CARTESIAN_POINT('',(6.40885299445509,4.94797317334227,-3.5533767744738));
#159798=CARTESIAN_POINT('Ctrl Pts',(6.859723901,4.818630405,-2.793840961));
#159799=CARTESIAN_POINT('Ctrl Pts',(6.856394065,4.820029867,-2.802016714));
#159800=CARTESIAN_POINT('Ctrl Pts',(6.853044751,4.821428571,-2.810184506));
#159801=CARTESIAN_POINT('Ctrl Pts',(6.702931827,4.884117105,-3.176256762));
#159802=CARTESIAN_POINT('Ctrl Pts',(6.514675115,4.947973174,-3.524254171));
#159803=CARTESIAN_POINT('Ctrl Pts',(6.655681333,4.818630405,-2.874787991));
#159804=CARTESIAN_POINT('Ctrl Pts',(6.652255021,4.820029867,-2.882720556));
#159805=CARTESIAN_POINT('Ctrl Pts',(6.64880981,4.821428571,-2.890644931));
#159806=CARTESIAN_POINT('Ctrl Pts',(6.494398894,4.884117105,-3.245807475));
#159807=CARTESIAN_POINT('Ctrl Pts',(6.30303087,4.947973174,-3.582499385));
#159808=CARTESIAN_POINT('Ctrl Pts',(6.6538178429181,4.81939091791731,-2.87909853968817));
#159809=CARTESIAN_POINT('Ctrl Pts',(6.67033817410486,4.8223472472397,-2.88644139503092));
#159810=CARTESIAN_POINT('Ctrl Pts',(6.68686360748816,4.82527010311368,-2.89378637035384));
#159811=CARTESIAN_POINT('Ctrl Pts',(6.7033999037213,4.8281632174832,-2.90111850959978));
#159812=CARTESIAN_POINT('Ctrl Pts',(6.71888040393875,4.83087161463545,-2.90798251237229));
#159813=CARTESIAN_POINT('Ctrl Pts',(6.73436889977429,4.83355328551508,-2.91483908496541));
#159814=CARTESIAN_POINT('Ctrl Pts',(6.74986497879421,4.8362090438618,-2.92168848777077));
#159815=CARTESIAN_POINT('Ctrl Pts',(6.7653612241887,4.83886483072222,-2.92853796411515));
#159816=CARTESIAN_POINT('Ctrl Pts',(6.78086509422502,4.84149471140405,-2.93538028861221));
#159817=CARTESIAN_POINT('Ctrl Pts',(6.79637620263612,4.84409946426182,-2.9422157054656));
#159818=CARTESIAN_POINT('Ctrl Pts',(7.03071436425429,4.94924836941368,-2.33033886258751));
#159819=CARTESIAN_POINT('Ctrl Pts',(7.02944803762714,4.94861077170685,-2.33414560129375));
#159820=CARTESIAN_POINT('Ctrl Pts',(7.028181711,4.947973174,-2.33795234));
#159821=CARTESIAN_POINT('Ctrl Pts',(6.900820226,4.88384644,-2.720817143));
#159822=CARTESIAN_POINT('Ctrl Pts',(6.73262222,4.818610636,-3.08758115));
#159823=CARTESIAN_POINT('Ctrl Pts',(6.92812328853911,4.94924836941368,-2.13627464941378));
#159824=CARTESIAN_POINT('Ctrl Pts',(6.92696213476956,4.94861077170685,-2.14002593470689));
#159825=CARTESIAN_POINT('Ctrl Pts',(6.92580098100001,4.947973174,-2.14377722));
#159826=CARTESIAN_POINT('Ctrl Pts',(6.809017313,4.88384644,-2.521064766));
#159827=CARTESIAN_POINT('Ctrl Pts',(6.651940379,4.818610636,-2.883433576));
#159828=CARTESIAN_POINT('',(6.9430010461971,4.94797317334248,-2.17639882768109));
#159829=CARTESIAN_POINT('Ctrl Pts',(6.92673643454702,4.94745154526473,-2.1407550938548));
#159830=CARTESIAN_POINT('Ctrl Pts',(6.92626870777351,4.94771235963237,-2.1422661569274));
#159831=CARTESIAN_POINT('Ctrl Pts',(6.925800981,4.947973174,-2.14377722));
#159832=CARTESIAN_POINT('Ctrl Pts',(6.878968119,4.97408817100001,-2.295077963));
#159833=CARTESIAN_POINT('Ctrl Pts',(6.825572471,5.00031307,-2.444189118));
#159834=CARTESIAN_POINT('Ctrl Pts',(6.96116503193408,4.94745154526473,-2.20598330608988));
#159835=CARTESIAN_POINT('Ctrl Pts',(6.96068307046704,4.94771235963237,-2.20750187454494));
#159836=CARTESIAN_POINT('Ctrl Pts',(6.960201109,4.947973174,-2.209020443));
#159837=CARTESIAN_POINT('Ctrl Pts',(6.911942946,4.97408817100001,-2.36107269));
#159838=CARTESIAN_POINT('Ctrl Pts',(6.857090538,5.00031307,-2.510872388));
#159839=CARTESIAN_POINT('Origin',(-0.180064974145001,5.08925699270593,0.080132333575427));
#159840=CARTESIAN_POINT('Ctrl Pts',(6.982521361,4.94766207,-2.112343688));
#159841=CARTESIAN_POINT('Ctrl Pts',(6.936100192,4.973931887,-2.265792583));
#159842=CARTESIAN_POINT('Ctrl Pts',(6.882982665,5.00031307,-2.417054001));
#159843=CARTESIAN_POINT('Ctrl Pts',(6.926358667,4.94766207,-2.1419747));
#159844=CARTESIAN_POINT('Ctrl Pts',(6.879286323,4.973931887,-2.294189355));
#159845=CARTESIAN_POINT('Ctrl Pts',(6.825572471,5.00031307,-2.444189118));
#159846=CARTESIAN_POINT('Ctrl Pts',(6.92580050069003,4.94797287203559,-2.1437791256559));
#159847=CARTESIAN_POINT('Ctrl Pts',(6.93080204135417,4.94882769742158,-2.14528316368062));
#159848=CARTESIAN_POINT('Ctrl Pts',(6.93580375378228,4.94967947055423,-2.14678836796916));
#159849=CARTESIAN_POINT('Ctrl Pts',(6.94080614265597,4.95052852743683,-2.14829285226673));
#159850=CARTESIAN_POINT('Ctrl Pts',(6.94545016576042,4.95131675879576,-2.14968955692418));
#159851=CARTESIAN_POINT('Ctrl Pts',(6.95009477335998,4.95210264918661,-2.1510856413952));
#159852=CARTESIAN_POINT('Ctrl Pts',(6.95473995609888,4.95288622031847,-2.15248111144501));
#159853=CARTESIAN_POINT('Ctrl Pts',(6.95938514353082,4.95366979224198,-2.15387658290467));
#159854=CARTESIAN_POINT('Ctrl Pts',(6.96403090727515,4.95445104509922,-2.15527144029312));
#159855=CARTESIAN_POINT('Ctrl Pts',(6.96867723835465,4.95523000034217,-2.1566656893329));
#159856=CARTESIAN_POINT('Ctrl Pts',(7.04635258300001,5.000313899,-1.88852209));
#159857=CARTESIAN_POINT('Ctrl Pts',(7.017457945,4.98224132,-1.99633222));
#159858=CARTESIAN_POINT('Ctrl Pts',(6.985278584,4.964285714,-2.103207909));
#159859=CARTESIAN_POINT('Ctrl Pts',(6.970404623,4.955986264,-2.152608049));
#159860=CARTESIAN_POINT('Ctrl Pts',(6.954833465,4.947660853,-2.20179288));
#159861=CARTESIAN_POINT('Ctrl Pts',(7.014268043,5.000313899,-1.833724031));
#159862=CARTESIAN_POINT('Ctrl Pts',(6.986211822,4.98224132,-1.941043263));
#159863=CARTESIAN_POINT('Ctrl Pts',(6.954885505,4.964285714,-2.047453934));
#159864=CARTESIAN_POINT('Ctrl Pts',(6.940405838,4.955986264,-2.096639133));
#159865=CARTESIAN_POINT('Ctrl Pts',(6.925231974,4.947660853,-2.145614621));
#159866=CARTESIAN_POINT('Ctrl Pts',(6.92580079412434,4.94797303316317,-2.14377817766412));
#159867=CARTESIAN_POINT('Ctrl Pts',(6.93572593790158,4.95342302531133,-2.11171322693376));
#159868=CARTESIAN_POINT('Ctrl Pts',(6.94542096528859,4.9588608327439,-2.07960351790515));
#159869=CARTESIAN_POINT('Ctrl Pts',(6.95488550519347,4.96428571402583,-2.04745393411916));
#159870=CARTESIAN_POINT('Ctrl Pts',(6.97555298415225,4.97613189126264,-1.97724969495794));
#159871=CARTESIAN_POINT('Ctrl Pts',(6.99519251853477,4.98803923908107,-1.9066126073206));
#159872=CARTESIAN_POINT('Ctrl Pts',(7.01378048014667,5.00000000026952,-1.83558801947581));
#159873=CARTESIAN_POINT('Ctrl Pts',(7.014268043,5.000313899,-1.833724031));
#159874=CARTESIAN_POINT('Ctrl Pts',(6.986211822,4.98224132,-1.941043263));
#159875=CARTESIAN_POINT('Ctrl Pts',(6.954885505,4.964285714,-2.047453934));
#159876=CARTESIAN_POINT('Ctrl Pts',(6.940677455,4.95614195,-2.095716491));
#159877=CARTESIAN_POINT('Ctrl Pts',(6.925800981,4.947973174,-2.14377722));
#159878=CARTESIAN_POINT('Ctrl Pts',(7.077917257,5.000313899,-1.796457094));
#159879=CARTESIAN_POINT('Ctrl Pts',(7.050431225,4.98224132,-1.904750168));
#159880=CARTESIAN_POINT('Ctrl Pts',(7.019645038,4.964285714,-2.012151669));
#159881=CARTESIAN_POINT('Ctrl Pts',(7.005681963,4.95614195,-2.060863616));
#159882=CARTESIAN_POINT('Ctrl Pts',(6.991044205,4.947973174,-2.109377092));
#159883=CARTESIAN_POINT('',(7.02288854215139,4.94797317334226,-2.09258685113586));
#159884=CARTESIAN_POINT('Ctrl Pts',(7.299940589,4.81863040500001,-1.253884645));
#159885=CARTESIAN_POINT('Ctrl Pts',(7.298446148,4.820029867,-1.262585069));
#159886=CARTESIAN_POINT('Ctrl Pts',(7.296930973,4.821428571,-1.271281907));
#159887=CARTESIAN_POINT('Ctrl Pts',(7.22902232,4.884117105,-1.661065438));
#159888=CARTESIAN_POINT('Ctrl Pts',(7.11997610100001,4.947973174,-2.04139649));
#159889=CARTESIAN_POINT('Ctrl Pts',(7.118069642,4.81863040500001,-1.376802299));
#159890=CARTESIAN_POINT('Ctrl Pts',(7.116428702,4.820029867,-1.385285961));
#159891=CARTESIAN_POINT('Ctrl Pts',(7.114767544,4.821428571,-1.393765687));
#159892=CARTESIAN_POINT('Ctrl Pts',(7.040316119,4.884117105,-1.77381851));
#159893=CARTESIAN_POINT('Ctrl Pts',(6.925800981,4.947973174,-2.14377722));
#159894=CARTESIAN_POINT('Ctrl Pts',(7.11717635922453,4.81939091801856,-1.381412664868));
#159895=CARTESIAN_POINT('Ctrl Pts',(7.13488895149142,4.82234724724486,-1.38503246517534));
#159896=CARTESIAN_POINT('Ctrl Pts',(7.15260698192933,4.82527010311933,-1.38865323946183));
#159897=CARTESIAN_POINT('Ctrl Pts',(7.17033286187557,4.82816321748676,-1.39225914256787));
#159898=CARTESIAN_POINT('Ctrl Pts',(7.18692699429999,4.8308716146483,-1.39563481891414));
#159899=CARTESIAN_POINT('Ctrl Pts',(7.20352733814408,4.83355328553553,-1.39900151995689));
#159900=CARTESIAN_POINT('Ctrl Pts',(7.22013354659239,4.8362090438886,-1.40235958866371));
#159901=CARTESIAN_POINT('Ctrl Pts',(7.23673993333435,4.83886483075539,-1.40571769342466));
#159902=CARTESIAN_POINT('Ctrl Pts',(7.25335222902539,4.84149471144234,-1.40906717445856));
#159903=CARTESIAN_POINT('Ctrl Pts',(7.26997010912512,4.84409946433572,-1.41240835333832));
#159904=CARTESIAN_POINT('Ctrl Pts',(7.36729414063743,4.94924836941368,-0.764461072856926));
#159905=CARTESIAN_POINT('Ctrl Pts',(7.36687575631872,4.94861077170684,-0.768451034928463));
#159906=CARTESIAN_POINT('Ctrl Pts',(7.366457372,4.947973174,-0.772440997000001));
#159907=CARTESIAN_POINT('Ctrl Pts',(7.324378143,4.88384644,-1.173733589));
#159908=CARTESIAN_POINT('Ctrl Pts',(7.238955932,4.818610636,-1.568080456));
#159909=CARTESIAN_POINT('Ctrl Pts',(7.22538351839981,4.94924836941368,-0.596988021858047));
#159910=CARTESIAN_POINT('Ctrl Pts',(7.2250559271999,4.94861077170684,-0.600901217929023));
#159911=CARTESIAN_POINT('Ctrl Pts',(7.224728336,4.947973174,-0.604814414));
#159912=CARTESIAN_POINT('Ctrl Pts',(7.191780674,4.88384644,-0.998386224));
#159913=CARTESIAN_POINT('Ctrl Pts',(7.116274695,4.818610636,-1.38604995));
#159914=CARTESIAN_POINT('',(7.24853895434816,4.94797317334248,-0.632975841513029));
#159915=CARTESIAN_POINT('Ctrl Pts',(7.2249922513874,4.94745154526473,-0.601661848617231));
#159916=CARTESIAN_POINT('Ctrl Pts',(7.2248602936937,4.94771235963237,-0.603238131308616));
#159917=CARTESIAN_POINT('Ctrl Pts',(7.224728336,4.947973174,-0.604814414));
#159918=CARTESIAN_POINT('Ctrl Pts',(7.211515587,4.97408817100001,-0.762645510999999));
#159919=CARTESIAN_POINT('Ctrl Pts',(7.19142279,5.00031307,-0.919749016));
#159920=CARTESIAN_POINT('Ctrl Pts',(7.27263806430311,4.94745154526473,-0.657963931735703));
#159921=CARTESIAN_POINT('Ctrl Pts',(7.27249381815156,4.94771235963237,-0.659550604367851));
#159922=CARTESIAN_POINT('Ctrl Pts',(7.272349572,4.947973174,-0.661137277));
#159923=CARTESIAN_POINT('Ctrl Pts',(7.257906396,4.97408817100001,-0.820008705));
#159924=CARTESIAN_POINT('Ctrl Pts',(7.236538914,5.00031307,-0.978097815));
#159925=CARTESIAN_POINT('Origin',(-0.19308164471352,5.08925706922526,0.0395503117135843));
#159926=CARTESIAN_POINT('Ctrl Pts',(7.273365344,4.94766207,-0.561922576));
#159927=CARTESIAN_POINT('Ctrl Pts',(7.261016453,4.973931887,-0.7217631));
#159928=CARTESIAN_POINT('Ctrl Pts',(7.241657518,5.00031307,-0.880906808));
#159929=CARTESIAN_POINT('Ctrl Pts',(7.224885495,4.94766207,-0.602934150000001));
#159930=CARTESIAN_POINT('Ctrl Pts',(7.211635327,4.973931887,-0.761709274));
#159931=CARTESIAN_POINT('Ctrl Pts',(7.19142279,5.00031307,-0.919749016));
#159932=CARTESIAN_POINT('Ctrl Pts',(7.22472827651318,4.94797287212304,-0.604816378418453));
#159933=CARTESIAN_POINT('Ctrl Pts',(7.22993620750882,4.94882769746256,-0.605210069807342));
#159934=CARTESIAN_POINT('Ctrl Pts',(7.23514455707306,4.94967947060204,-0.605604862983575));
#159935=CARTESIAN_POINT('Ctrl Pts',(7.24035341250809,4.95052852749047,-0.605998807567377));
#159936=CARTESIAN_POINT('Ctrl Pts',(7.24518911107269,4.95131675884529,-0.606364530379651));
#159937=CARTESIAN_POINT('Ctrl Pts',(7.25002524716207,4.95210264923163,-0.606729521840045));
#159938=CARTESIAN_POINT('Ctrl Pts',(7.25486181286332,4.95288622035671,-0.607093789592621));
#159939=CARTESIAN_POINT('Ctrl Pts',(7.25969838345099,4.95366979227343,-0.607458057713219));
#159940=CARTESIAN_POINT('Ctrl Pts',(7.26453538487142,4.95445104512166,-0.60782160221566));
#159941=CARTESIAN_POINT('Ctrl Pts',(7.26937280966497,4.9552300003664,-0.60818443062782));
#159942=CARTESIAN_POINT('Ctrl Pts',(7.287589201,5.000313899,-0.329611976));
#159943=CARTESIAN_POINT('Ctrl Pts',(7.282546094,4.98224132,-0.441113058));
#159944=CARTESIAN_POINT('Ctrl Pts',(7.274094183,4.964285714,-0.552407665));
#159945=CARTESIAN_POINT('Ctrl Pts',(7.27018753600001,4.955986264,-0.603850319));
#159946=CARTESIAN_POINT('Ctrl Pts',(7.265553708,4.947660853,-0.655232575));
#159947=CARTESIAN_POINT('Ctrl Pts',(7.244474816,5.000313899,-0.282992293));
#159948=CARTESIAN_POINT('Ctrl Pts',(7.240144997,4.98224132,-0.393833719));
#159949=CARTESIAN_POINT('Ctrl Pts',(7.23242622,4.964285714,-0.5044908));
#159950=CARTESIAN_POINT('Ctrl Pts',(7.228858443,4.955986264,-0.555638777));
#159951=CARTESIAN_POINT('Ctrl Pts',(7.22456761900001,4.947660853,-0.606731178));
#159952=CARTESIAN_POINT('Ctrl Pts',(7.22472835929903,4.94797303325467,-0.604815389485618));
#159953=CARTESIAN_POINT('Ctrl Pts',(7.22752844201957,4.95342302547636,-0.571366486962385));
#159954=CARTESIAN_POINT('Ctrl Pts',(7.23009416642667,4.95886083287659,-0.537923340666376));
#159955=CARTESIAN_POINT('Ctrl Pts',(7.23242622053074,4.96428571409676,-0.504490799966201));
#159956=CARTESIAN_POINT('Ctrl Pts',(7.2375186690733,4.97613189123871,-0.431484999790809));
#159957=CARTESIAN_POINT('Ctrl Pts',(7.24151415645778,4.98803923915467,-0.358277448234716));
#159958=CARTESIAN_POINT('Ctrl Pts',(7.24439935455547,5.00000000038041,-0.28491751337921));
#159959=CARTESIAN_POINT('Ctrl Pts',(7.244474816,5.000313899,-0.282992293));
#159960=CARTESIAN_POINT('Ctrl Pts',(7.240144997,4.98224132,-0.393833719));
#159961=CARTESIAN_POINT('Ctrl Pts',(7.23242622,4.964285714,-0.5044908));
#159962=CARTESIAN_POINT('Ctrl Pts',(7.22892537,4.95614195,-0.554679316000001));
#159963=CARTESIAN_POINT('Ctrl Pts',(7.224728336,4.947973174,-0.604814414));
#159964=CARTESIAN_POINT('Ctrl Pts',(7.298624658,5.000313899,-0.232913937));
#159965=CARTESIAN_POINT('Ctrl Pts',(7.295061043,4.98224132,-0.344583863));
#159966=CARTESIAN_POINT('Ctrl Pts',(7.288082768,4.964285714,-0.456092497));
#159967=CARTESIAN_POINT('Ctrl Pts',(7.28491777100001,4.95614195,-0.506667235));
#159968=CARTESIAN_POINT('Ctrl Pts',(7.281051199,4.947973174,-0.557193178));
#159969=CARTESIAN_POINT('',(7.3085416277938,4.94797317334222,-0.533949891478464));
#159970=CARTESIAN_POINT('Ctrl Pts',(7.398820169,4.818630405,0.344701923));
#159971=CARTESIAN_POINT('Ctrl Pts',(7.399231002,4.820029867,0.335883649));
#159972=CARTESIAN_POINT('Ctrl Pts',(7.399620813,4.821428571,0.327064421));
#159973=CARTESIAN_POINT('Ctrl Pts',(7.417091764,4.884117105,-0.068204541));
#159974=CARTESIAN_POINT('Ctrl Pts',(7.392354919,4.947973174,-0.463085377));
#159975=CARTESIAN_POINT('Ctrl Pts',(7.247624926,4.818630405,0.185561138));
#159976=CARTESIAN_POINT('Ctrl Pts',(7.247846087,4.820029867,0.176923066));
#159977=CARTESIAN_POINT('Ctrl Pts',(7.248046656,4.821428571,0.168284491));
#159978=CARTESIAN_POINT('Ctrl Pts',(7.257035987,4.884117105,-0.218887764));
#159979=CARTESIAN_POINT('Ctrl Pts',(7.224728336,4.947973174,-0.604814414));
#159980=CARTESIAN_POINT('Ctrl Pts',(7.2477436202233,4.81939091791719,0.180866530341205));
#159981=CARTESIAN_POINT('Ctrl Pts',(7.26582025148185,4.82234724725628,0.181139042606722));
#159982=CARTESIAN_POINT('Ctrl Pts',(7.28390240363902,4.82527010311953,0.181411772860868));
#159983=CARTESIAN_POINT('Ctrl Pts',(7.30198902492249,4.82816321747991,0.181700714026033));
#159984=CARTESIAN_POINT('Ctrl Pts',(7.31892086638338,4.83087161463771,0.181971207111691));
#159985=CARTESIAN_POINT('Ctrl Pts',(7.33585684461923,4.83355328552332,0.182251800924294));
#159986=CARTESIAN_POINT('Ctrl Pts',(7.35279669465095,4.83620904387642,0.182542085962254));
#159987=CARTESIAN_POINT('Ctrl Pts',(7.3697367265584,4.83886483074323,0.182832374116876));
#159988=CARTESIAN_POINT('Ctrl Pts',(7.38668067542047,4.84149471143185,0.183132354622081));
#159989=CARTESIAN_POINT('Ctrl Pts',(7.40362829344876,4.84409946433362,0.183441643659611));
#159990=CARTESIAN_POINT('Ctrl Pts',(7.3593874306487,4.94924836941369,0.837162067481764));
#159991=CARTESIAN_POINT('Ctrl Pts',(7.35983655182435,4.94861077170684,0.833175448240883));
#159992=CARTESIAN_POINT('Ctrl Pts',(7.360285673,4.947973174,0.829188829));
#159993=CARTESIAN_POINT('Ctrl Pts',(7.405456278,4.88384644,0.428232444));
#159994=CARTESIAN_POINT('Ctrl Pts',(7.406804111,4.818610636,0.024741937));
#159995=CARTESIAN_POINT('Ctrl Pts',(7.18479284462102,4.94924836941369,0.970213102287845));
#159996=CARTESIAN_POINT('Ctrl Pts',(7.18531413381051,4.94861077170684,0.966320972143923));
#159997=CARTESIAN_POINT('Ctrl Pts',(7.185835423,4.947973174,0.962428842));
#159998=CARTESIAN_POINT('Ctrl Pts',(7.238264365,4.88384644,0.570975749));
#159999=CARTESIAN_POINT('Ctrl Pts',(7.24785991500001,4.818610636,0.176143831));
#160000=CARTESIAN_POINT('',(7.21514323698324,4.94797317334286,0.940044391966286));
#160001=CARTESIAN_POINT('Ctrl Pts',(7.18541545982678,4.94745154526474,0.965564436160455));
#160002=CARTESIAN_POINT('Ctrl Pts',(7.18562544141339,4.94771235963236,0.963996639080227));
#160003=CARTESIAN_POINT('Ctrl Pts',(7.185835423,4.947973174,0.962428842));
#160004=CARTESIAN_POINT('Ctrl Pts',(7.206860601,4.97408817100001,0.805447398));
#160005=CARTESIAN_POINT('Ctrl Pts',(7.221010173,5.00031307,0.647697528));
#160006=CARTESIAN_POINT('Ctrl Pts',(7.24405062408982,4.94745154526474,0.920821105528827));
#160007=CARTESIAN_POINT('Ctrl Pts',(7.2442508380449,4.94771235963236,0.919240519764414));
#160008=CARTESIAN_POINT('Ctrl Pts',(7.244451052,4.947973174,0.917659934));
#160009=CARTESIAN_POINT('Ctrl Pts',(7.26449821,4.97408817100001,0.759397976));
#160010=CARTESIAN_POINT('Ctrl Pts',(7.277614774,5.00031307,0.600411524));
#160011=CARTESIAN_POINT('Origin',(-0.197070757240472,5.08925702468576,-0.00288134842447038));
#160012=CARTESIAN_POINT('Ctrl Pts',(7.224114848,4.94766207,1.014773411));
#160013=CARTESIAN_POINT('Ctrl Pts',(7.246415654,4.973931887,0.856015224000001));
#160014=CARTESIAN_POINT('Ctrl Pts',(7.26172051400001,5.00031307,0.696430608));
#160015=CARTESIAN_POINT('Ctrl Pts',(7.185584706,4.94766207,0.96429893));
#160016=CARTESIAN_POINT('Ctrl Pts',(7.206776278,4.973931887,0.806387487000001));
#160017=CARTESIAN_POINT('Ctrl Pts',(7.221010173,5.00031307,0.647697528));
#160018=CARTESIAN_POINT('Ctrl Pts',(7.18583578693528,4.94797287209165,0.962426910232247));
#160019=CARTESIAN_POINT('Ctrl Pts',(7.19100659134204,4.94882769740662,0.963161974412689));
#160020=CARTESIAN_POINT('Ctrl Pts',(7.19617804139228,4.94967947052024,0.963896052513582));
#160021=CARTESIAN_POINT('Ctrl Pts',(7.20134980306533,4.95052852738558,0.964631068107125));
#160022=CARTESIAN_POINT('Ctrl Pts',(7.20615106539685,4.95131675874708,0.965313427988624));
#160023=CARTESIAN_POINT('Ctrl Pts',(7.21095259780624,4.95210264914231,0.965996596171963));
#160024=CARTESIAN_POINT('Ctrl Pts',(7.21575439420849,4.95288622027866,0.96668056348834));
#160025=CARTESIAN_POINT('Ctrl Pts',(7.22055619546201,4.95366979220666,0.967364531495733));
#160026=CARTESIAN_POINT('Ctrl Pts',(7.22535826191999,4.9544510450685,0.968049298811043));
#160027=CARTESIAN_POINT('Ctrl Pts',(7.23016058785084,4.95523000031898,0.968734856467267));
#160028=CARTESIAN_POINT('Ctrl Pts',(7.188066246,5.000313899,1.244710427));
#160029=CARTESIAN_POINT('Ctrl Pts',(7.20711048100001,4.98224132,1.13473206));
#160030=CARTESIAN_POINT('Ctrl Pts',(7.222781222,4.964285714,1.024222548));
#160031=CARTESIAN_POINT('Ctrl Pts',(7.230024561,4.955986264,0.973142781));
#160032=CARTESIAN_POINT('Ctrl Pts',(7.236544735,4.947660853,0.921965678));
#160033=CARTESIAN_POINT('Ctrl Pts',(7.135937999,5.000313899,1.28097185));
#160034=CARTESIAN_POINT('Ctrl Pts',(7.155537038,4.98224132,1.171791051));
#160035=CARTESIAN_POINT('Ctrl Pts',(7.171786724,4.964285714,1.062061763));
#160036=CARTESIAN_POINT('Ctrl Pts',(7.179297663,4.955986264,1.01134263));
#160037=CARTESIAN_POINT('Ctrl Pts',(7.186090511,4.947660853,0.960522341));
#160038=CARTESIAN_POINT('Ctrl Pts',(7.18583565516621,4.94797303325765,0.962427894050688));
#160039=CARTESIAN_POINT('Ctrl Pts',(7.1813797480107,4.95342302539181,0.995696714765073));
#160040=CARTESIAN_POINT('Ctrl Pts',(7.17669620014671,4.95886083279384,1.02890953346614));
#160041=CARTESIAN_POINT('Ctrl Pts',(7.17178672409145,4.96428571393831,1.06206176259658));
#160042=CARTESIAN_POINT('Ctrl Pts',(7.16106602474189,4.97613189084492,1.13445545159152));
#160043=CARTESIAN_POINT('Ctrl Pts',(7.14923064057945,4.98803923896588,1.20681036385963));
#160044=CARTESIAN_POINT('Ctrl Pts',(7.13627816756702,5.00000000009595,1.27907541649019));
#160045=CARTESIAN_POINT('Ctrl Pts',(7.135937999,5.000313899,1.28097185));
#160046=CARTESIAN_POINT('Ctrl Pts',(7.155537038,4.98224132,1.171791051));
#160047=CARTESIAN_POINT('Ctrl Pts',(7.171786724,4.964285714,1.062061763));
#160048=CARTESIAN_POINT('Ctrl Pts',(7.179156768,4.95614195,1.012294047));
#160049=CARTESIAN_POINT('Ctrl Pts',(7.185835423,4.947973174,0.962428842));
#160050=CARTESIAN_POINT('Ctrl Pts',(7.178056481,5.000313899,1.341520017));
#160051=CARTESIAN_POINT('Ctrl Pts',(7.198581915,4.98224132,1.2316948));
#160052=CARTESIAN_POINT('Ctrl Pts',(7.215737847,4.964285714,1.121293053));
#160053=CARTESIAN_POINT('Ctrl Pts',(7.22351892000001,4.95614195,1.071220344));
#160054=CARTESIAN_POINT('Ctrl Pts',(7.23060433,4.947973174,1.021044471));
#160055=CARTESIAN_POINT('',(7.25245542892245,4.94797317334225,1.04965397099054));
#160056=CARTESIAN_POINT('Ctrl Pts',(7.15173914100001,4.818630405,1.927170612));
#160057=CARTESIAN_POINT('Ctrl Pts',(7.154036037,4.820029867,1.918646822));
#160058=CARTESIAN_POINT('Ctrl Pts',(7.156312608,4.821428571,1.91011758));
#160059=CARTESIAN_POINT('Ctrl Pts',(7.258346241,4.884117105,1.527845525));
#160060=CARTESIAN_POINT('Ctrl Pts',(7.319075436,4.947973174,1.136879092));
#160061=CARTESIAN_POINT('Ctrl Pts',(7.038289323,4.818630405,1.739247943));
#160062=CARTESIAN_POINT('Ctrl Pts',(7.040362243,4.820029867,1.730859367));
#160063=CARTESIAN_POINT('Ctrl Pts',(7.042415162,4.821428571,1.722465874));
#160064=CARTESIAN_POINT('Ctrl Pts',(7.134424917,4.884117105,1.346277931));
#160065=CARTESIAN_POINT('Ctrl Pts',(7.185835423,4.947973174,0.962428842));
#160066=CARTESIAN_POINT('Ctrl Pts',(7.03941444436566,4.81939091775252,1.73468860817442));
#160067=CARTESIAN_POINT('Ctrl Pts',(7.05700987218026,4.82234724734587,1.73884069106666));
#160068=CARTESIAN_POINT('Ctrl Pts',(7.0746106448554,4.82527010316785,1.74299417296875));
#160069=CARTESIAN_POINT('Ctrl Pts',(7.09221229723318,4.82816321752951,1.74716444778148));
#160070=CARTESIAN_POINT('Ctrl Pts',(7.10869013359083,4.83087161467271,1.75106846227147));
#160071=CARTESIAN_POINT('Ctrl Pts',(7.12516983864926,4.83355328554229,1.75498323062839));
#160072=CARTESIAN_POINT('Ctrl Pts',(7.1416512416553,4.8362090438783,1.7589082959611));
#160073=CARTESIAN_POINT('Ctrl Pts',(7.15813282161496,4.83886483072803,1.76283340343552));
#160074=CARTESIAN_POINT('Ctrl Pts',(7.17461614338329,4.84149471139851,1.76676881869245));
#160075=CARTESIAN_POINT('Ctrl Pts',(7.19110104734923,4.84409946426157,1.77071411358907));
#160076=CARTESIAN_POINT('Ctrl Pts',(7.0073639444683,4.94924836941368,2.39964043902942));
#160077=CARTESIAN_POINT('Ctrl Pts',(7.00865957073415,4.94861077170684,2.39584357251471));
#160078=CARTESIAN_POINT('Ctrl Pts',(7.009955197,4.947973174,2.392046706));
#160079=CARTESIAN_POINT('Ctrl Pts',(7.140263509,4.88384644,2.010174804));
#160080=CARTESIAN_POINT('Ctrl Pts',(7.228318362,4.818610636,1.616407425));
#160081=CARTESIAN_POINT('Ctrl Pts',(6.80824924266725,4.94924836941368,2.49204813906551));
#160082=CARTESIAN_POINT('Ctrl Pts',(6.80959503733362,4.94861077170684,2.48835906653275));
#160083=CARTESIAN_POINT('Ctrl Pts',(6.810940832,4.947973174,2.484669994));
#160084=CARTESIAN_POINT('Ctrl Pts',(6.94629485800001,4.88384644,2.11363953));
#160085=CARTESIAN_POINT('Ctrl Pts',(7.040543261,4.818610636,1.730101323));
#160086=CARTESIAN_POINT('',(6.84437544064191,4.94797317334249,2.46910919426462));
#160087=CARTESIAN_POINT('Ctrl Pts',(6.80985662727826,4.94745154526473,2.48764200003715));
#160088=CARTESIAN_POINT('Ctrl Pts',(6.81039872963913,4.94771235963237,2.48615599701857));
#160089=CARTESIAN_POINT('Ctrl Pts',(6.810940832,4.947973174,2.484669994));
#160090=CARTESIAN_POINT('Ctrl Pts',(6.865220823,4.97408817100001,2.335878481));
#160091=CARTESIAN_POINT('Ctrl Pts',(6.912951145,5.00031307,2.184858455));
#160092=CARTESIAN_POINT('Ctrl Pts',(6.87673942742404,4.94745154526473,2.45654957195124));
#160093=CARTESIAN_POINT('Ctrl Pts',(6.87727473971202,4.94771235963237,2.45504897947562));
#160094=CARTESIAN_POINT('Ctrl Pts',(6.877810052,4.947973174,2.453548387));
#160095=CARTESIAN_POINT('Ctrl Pts',(6.931410162,4.97408817100001,2.303296051));
#160096=CARTESIAN_POINT('Ctrl Pts',(6.978397455,5.00031307,2.150846288));
#160097=CARTESIAN_POINT('Origin',(-0.191843328106668,5.08925706687508,-0.0451781557118802));
#160098=CARTESIAN_POINT('Ctrl Pts',(6.83707277,4.94766207,2.544019722));
#160099=CARTESIAN_POINT('Ctrl Pts',(6.892980514,4.973931887,2.393767227));
#160100=CARTESIAN_POINT('Ctrl Pts',(6.942233529,5.00031307,2.241203703));
#160101=CARTESIAN_POINT('Ctrl Pts',(6.810293963,4.94766207,2.486442465));
#160102=CARTESIAN_POINT('Ctrl Pts',(6.86493638100001,4.973931887,2.336778465));
#160103=CARTESIAN_POINT('Ctrl Pts',(6.912951145,5.00031307,2.184858455));
#160104=CARTESIAN_POINT('Ctrl Pts',(6.81094160271618,4.94797287204861,2.48466818632));
#160105=CARTESIAN_POINT('Ctrl Pts',(6.81583349962326,4.94882769745355,2.48649763558292));
#160106=CARTESIAN_POINT('Ctrl Pts',(6.82072623906249,4.94967947058637,2.48832626024999));
#160107=CARTESIAN_POINT('Ctrl Pts',(6.82561908128822,4.95052852746818,2.49015586746808));
#160108=CARTESIAN_POINT('Ctrl Pts',(6.83016140554712,4.95131675882604,2.49185440358831));
#160109=CARTESIAN_POINT('Ctrl Pts',(6.8347038197908,4.95210264921486,2.49355378715903));
#160110=CARTESIAN_POINT('Ctrl Pts',(6.83924632006457,4.95288622034428,2.49525400793252));
#160111=CARTESIAN_POINT('Ctrl Pts',(6.84378882492764,4.95366979226534,2.49695423042375));
#160112=CARTESIAN_POINT('Ctrl Pts',(6.84833141696647,4.95445104511974,2.49865529054903));
#160113=CARTESIAN_POINT('Ctrl Pts',(6.85287409254451,4.95523000036724,2.50035717833961));
#160114=CARTESIAN_POINT('Ctrl Pts',(6.752437304,5.000313899,2.760831554));
#160115=CARTESIAN_POINT('Ctrl Pts',(6.794678393,4.98224132,2.657518367));
#160116=CARTESIAN_POINT('Ctrl Pts',(6.833739039,4.964285714,2.552961253));
#160117=CARTESIAN_POINT('Ctrl Pts',(6.851793672,4.955986264,2.504632806));
#160118=CARTESIAN_POINT('Ctrl Pts',(6.86916297300001,4.947660853,2.45605384));
#160119=CARTESIAN_POINT('Ctrl Pts',(6.693732651,5.000313899,2.785039173));
#160120=CARTESIAN_POINT('Ctrl Pts',(6.73634412,4.98224132,2.682624175));
#160121=CARTESIAN_POINT('Ctrl Pts',(6.775802451,4.964285714,2.578953498));
#160122=CARTESIAN_POINT('Ctrl Pts',(6.794040902,4.955986264,2.531034781));
#160123=CARTESIAN_POINT('Ctrl Pts',(6.811599798,4.947660853,2.482862903));
#160124=CARTESIAN_POINT('Ctrl Pts',(6.81094126263909,4.94797303316575,2.4846691185281));
#160125=CARTESIAN_POINT('Ctrl Pts',(6.79943771959581,4.95342302528782,2.51620224415172));
#160126=CARTESIAN_POINT('Ctrl Pts',(6.78772389566368,4.95886083271677,2.54763174148845));
#160127=CARTESIAN_POINT('Ctrl Pts',(6.77580245123129,4.96428571398709,2.57895349783444));
#160128=CARTESIAN_POINT('Ctrl Pts',(6.74976989148222,4.97613189122178,2.64735003178943));
#160129=CARTESIAN_POINT('Ctrl Pts',(6.72265704507204,4.98803923914334,2.71546906758587));
#160130=CARTESIAN_POINT('Ctrl Pts',(6.69447254313508,5.00000000036334,2.78326020476335));
#160131=CARTESIAN_POINT('Ctrl Pts',(6.693732651,5.000313899,2.785039173));
#160132=CARTESIAN_POINT('Ctrl Pts',(6.73634412,4.98224132,2.682624175));
#160133=CARTESIAN_POINT('Ctrl Pts',(6.775802451,4.964285714,2.578953498));
#160134=CARTESIAN_POINT('Ctrl Pts',(6.793698776,4.95614194999999,2.531933665));
#160135=CARTESIAN_POINT('Ctrl Pts',(6.81094083200001,4.947973174,2.484669994));
#160136=CARTESIAN_POINT('Ctrl Pts',(6.72185036,5.000313899,2.853225986));
#160137=CARTESIAN_POINT('Ctrl Pts',(6.76550509700001,4.98224132,2.750380783));
#160138=CARTESIAN_POINT('Ctrl Pts',(6.805993045,4.964285714,2.646248186));
#160139=CARTESIAN_POINT('Ctrl Pts',(6.824356353,4.95614194999999,2.59901885));
#160140=CARTESIAN_POINT('Ctrl Pts',(6.84206244,4.947973174,2.551539214));
#160141=CARTESIAN_POINT('',(6.85725247507841,4.94797317334239,2.58417718027227));
#160142=CARTESIAN_POINT('Ctrl Pts',(6.570250739,4.818630405,3.419526946));
#160143=CARTESIAN_POINT('Ctrl Pts',(6.574326298,4.820029867,3.411696201));
#160144=CARTESIAN_POINT('Ctrl Pts',(6.578383179,4.821428571,3.403855764));
#160145=CARTESIAN_POINT('Ctrl Pts',(6.760208514,4.884117105,3.052455232));
#160146=CARTESIAN_POINT('Ctrl Pts',(6.903564121,4.947973174,2.683684359));
#160147=CARTESIAN_POINT('Ctrl Pts',(6.499851134,4.818630405,3.211609446));
#160148=CARTESIAN_POINT('Ctrl Pts',(6.503678886,4.820029867,3.203862607));
#160149=CARTESIAN_POINT('Ctrl Pts',(6.507488162,4.821428571,3.196106666));
#160150=CARTESIAN_POINT('Ctrl Pts',(6.678216068,4.884117105,2.848493166));
#160151=CARTESIAN_POINT('Ctrl Pts',(6.810940832,4.947973174,2.484669994));
#160152=CARTESIAN_POINT('Ctrl Pts',(6.5019300724108,4.81939091791719,3.2073985743076));
#160153=CARTESIAN_POINT('Ctrl Pts',(6.51822155404743,4.82234724730935,3.21523608098732));
#160154=CARTESIAN_POINT('Ctrl Pts',(6.53451795468387,4.82527010309894,3.22307610241689));
#160155=CARTESIAN_POINT('Ctrl Pts',(6.55081160437425,4.8281632174668,3.23093271345656));
#160156=CARTESIAN_POINT('Ctrl Pts',(6.56606495036695,4.83087161462078,3.2382877019825));
#160157=CARTESIAN_POINT('Ctrl Pts',(6.58131780960935,4.83355328550247,3.24565359466761));
#160158=CARTESIAN_POINT('Ctrl Pts',(6.59657011355836,4.8362090438514,3.25302990859615));
#160159=CARTESIAN_POINT('Ctrl Pts',(6.61182258126467,4.83886483071405,3.26040630172093));
#160160=CARTESIAN_POINT('Ctrl Pts',(6.62707453419009,4.84149471139827,3.26779313607204));
#160161=CARTESIAN_POINT('Ctrl Pts',(6.64232590857355,4.8440994642892,3.2751899592442));
#160162=CARTESIAN_POINT('Ctrl Pts',(6.32768390839934,4.94924836941368,3.8499142910946));
#160163=CARTESIAN_POINT('Ctrl Pts',(6.32976545769967,4.94861077170685,3.8464847145473));
#160164=CARTESIAN_POINT('Ctrl Pts',(6.331847007,4.947973174,3.843055138));
#160165=CARTESIAN_POINT('Ctrl Pts',(6.541199953,4.88384644,3.498123623));
#160166=CARTESIAN_POINT('Ctrl Pts',(6.71184448,4.818610636,3.132491498));
#160167=CARTESIAN_POINT('Ctrl Pts',(6.11335947344275,4.94924836941368,3.89735777600251));
#160168=CARTESIAN_POINT('Ctrl Pts',(6.11546684572137,4.94861077170685,3.89404425800126));
#160169=CARTESIAN_POINT('Ctrl Pts',(6.117574218,4.947973174,3.89073074));
#160170=CARTESIAN_POINT('Ctrl Pts',(6.329524324,4.88384644,3.557471876));
#160171=CARTESIAN_POINT('Ctrl Pts',(6.50401862899999,4.818610636,3.2031612));
#160172=CARTESIAN_POINT('',(6.15357225586438,4.94797317334249,3.88272119488466));
#160173=CARTESIAN_POINT('Ctrl Pts',(6.11587646793651,4.94745154526473,3.89340019023023));
#160174=CARTESIAN_POINT('Ctrl Pts',(6.11672534296826,4.94771235963237,3.89206546511511));
#160175=CARTESIAN_POINT('Ctrl Pts',(6.117574218,4.947973174,3.89073074));
#160176=CARTESIAN_POINT('Ctrl Pts',(6.20257095,4.97408817100001,3.757086483));
#160177=CARTESIAN_POINT('Ctrl Pts',(6.281650205,5.00031307,3.619857829));
#160178=CARTESIAN_POINT('Ctrl Pts',(6.18787953798209,4.94745154526473,3.87741250926571));
#160179=CARTESIAN_POINT('Ctrl Pts',(6.18872491799105,4.94771235963237,3.87606207613285));
#160180=CARTESIAN_POINT('Ctrl Pts',(6.189570298,4.947973174,3.874711643));
#160181=CARTESIAN_POINT('Ctrl Pts',(6.274217078,4.97408817100001,3.739494563));
#160182=CARTESIAN_POINT('Ctrl Pts',(6.352878027,5.00031307,3.60070987));
#160183=CARTESIAN_POINT('Origin',(-0.177646785006003,5.08925693465323,-0.0853629412040702));
#160184=CARTESIAN_POINT('Ctrl Pts',(6.130336769,4.94766207,3.954310498));
#160185=CARTESIAN_POINT('Ctrl Pts',(6.217237265,4.973931887,3.819589334));
#160186=CARTESIAN_POINT('Ctrl Pts',(6.29813542,5.00031307,3.681180604));
#160187=CARTESIAN_POINT('Ctrl Pts',(6.116561444,4.94766207,3.892322713));
#160188=CARTESIAN_POINT('Ctrl Pts',(6.202099688,4.973931887,3.757904278));
#160189=CARTESIAN_POINT('Ctrl Pts',(6.281650205,5.00031307,3.619857829));
#160190=CARTESIAN_POINT('Ctrl Pts',(6.11757535950015,4.94797287221035,3.89072913977308));
#160191=CARTESIAN_POINT('Ctrl Pts',(6.12195960931022,4.94882769747571,3.89356743017046));
#160192=CARTESIAN_POINT('Ctrl Pts',(6.12634485893963,4.94967947060649,3.8964050970286));
#160193=CARTESIAN_POINT('Ctrl Pts',(6.13072999775624,4.95052852749173,3.89924374556819));
#160194=CARTESIAN_POINT('Ctrl Pts',(6.13480098985002,4.95131675883662,3.90187903631836));
#160195=CARTESIAN_POINT('Ctrl Pts',(6.1388718876706,4.95210264921789,3.90451517405683));
#160196=CARTESIAN_POINT('Ctrl Pts',(6.14294268953924,4.9528862203413,3.90715214791331));
#160197=CARTESIAN_POINT('Ctrl Pts',(6.14701349552063,4.95366979225636,3.90978912443392));
#160198=CARTESIAN_POINT('Ctrl Pts',(6.15108420657628,4.95445104510628,3.91242693774001));
#160199=CARTESIAN_POINT('Ctrl Pts',(6.15515482124631,4.95523000034099,3.91506557728136));
#160200=CARTESIAN_POINT('Ctrl Pts',(6.001071897,5.000313899,4.147859266));
#160201=CARTESIAN_POINT('Ctrl Pts',(6.064534695,4.98224132,4.05604207));
#160202=CARTESIAN_POINT('Ctrl Pts',(6.125158813,4.964285714,3.962326327));
#160203=CARTESIAN_POINT('Ctrl Pts',(6.153180527,4.955986264,3.919008985));
#160204=CARTESIAN_POINT('Ctrl Pts',(6.180586785,4.947660853,3.875299654));
#160205=CARTESIAN_POINT('Ctrl Pts',(5.93853580499999,5.000313899,4.158881159));
#160206=CARTESIAN_POINT('Ctrl Pts',(6.002167238,4.98224132,4.068020773));
#160207=CARTESIAN_POINT('Ctrl Pts',(6.062989186,4.964285714,3.975256234));
#160208=CARTESIAN_POINT('Ctrl Pts',(6.091102341,4.955986264,3.932378558));
#160209=CARTESIAN_POINT('Ctrl Pts',(6.118606248,4.947660853,3.889107555));
#160210=CARTESIAN_POINT('Ctrl Pts',(6.11757421810585,4.94797317397983,3.8907307400712));
#160211=CARTESIAN_POINT('Ctrl Pts',(6.08891330775294,4.95664469842826,3.93579560534761));
#160212=CARTESIAN_POINT('Ctrl Pts',(6.05977978348553,4.96527389211456,3.98050483093599));
#160213=CARTESIAN_POINT('Ctrl Pts',(6.00046157189516,4.98260138557519,4.06937581674763));
#160214=CARTESIAN_POINT('Ctrl Pts',(5.97029573984605,4.99129055034349,4.1135054048051));
#160215=CARTESIAN_POINT('Ctrl Pts',(5.93964082487683,5.00000000023931,4.15730283636664));
#160216=CARTESIAN_POINT('Ctrl Pts',(5.93853580499999,5.000313899,4.158881159));
#160217=CARTESIAN_POINT('Ctrl Pts',(6.002167238,4.98224132,4.068020773));
#160218=CARTESIAN_POINT('Ctrl Pts',(6.062989186,4.964285714,3.975256234));
#160219=CARTESIAN_POINT('Ctrl Pts',(6.090574979,4.95614194999999,3.93318288));
#160220=CARTESIAN_POINT('Ctrl Pts',(6.117574218,4.947973174,3.89073074));
#160221=CARTESIAN_POINT('Ctrl Pts',(5.951337988,5.000313899,4.231518279));
#160222=CARTESIAN_POINT('Ctrl Pts',(6.01608078,4.98224132,4.140462018));
#160223=CARTESIAN_POINT('Ctrl Pts',(6.078007573,4.964285714,4.047467695));
#160224=CARTESIAN_POINT('Ctrl Pts',(6.106094468,4.95614194999999,4.005290123));
#160225=CARTESIAN_POINT('Ctrl Pts',(6.133593314,4.947973174,3.96272682));
#160226=CARTESIAN_POINT('',(6.14141201680087,4.94797317334243,3.99786713737824));
#160227=CARTESIAN_POINT('Ctrl Pts',(5.681544715,4.818630405,4.75199));
#160228=CARTESIAN_POINT('Ctrl Pts',(5.687208368,4.820029867,4.745218458));
#160229=CARTESIAN_POINT('Ctrl Pts',(5.692855864,4.821428571,4.738433436));
#160230=CARTESIAN_POINT('Ctrl Pts',(5.945970951,4.884117105,4.434335525));
#160231=CARTESIAN_POINT('Ctrl Pts',(6.16524982,4.947973174,4.105003528));
#160232=CARTESIAN_POINT('Ctrl Pts',(5.65748713,4.818630405,4.533799662));
#160233=CARTESIAN_POINT('Ctrl Pts',(5.662890733,4.820029867,4.52705679300001));
#160234=CARTESIAN_POINT('Ctrl Pts',(5.668278248,4.821428571,4.520301063));
#160235=CARTESIAN_POINT('Ctrl Pts',(5.90974125700001,4.884117105,4.217516027));
#160236=CARTESIAN_POINT('Ctrl Pts',(6.11757421800001,4.947973174,3.89073074));
#160237=CARTESIAN_POINT('Ctrl Pts',(5.6604226771306,4.81939091801856,4.53013414802792));
#160238=CARTESIAN_POINT('Ctrl Pts',(5.67464844079712,4.82234724726659,4.54129060488698));
#160239=CARTESIAN_POINT('Ctrl Pts',(5.68887846756111,4.82527010310083,4.55245057562458));
#160240=CARTESIAN_POINT('Ctrl Pts',(5.70310224161804,4.8281632174612,4.56362615650414));
#160241=CARTESIAN_POINT('Ctrl Pts',(5.71641786775918,4.8308716146174,4.57408820801779));
#160242=CARTESIAN_POINT('Ctrl Pts',(5.72973067446047,4.83355328549926,4.58456080411798));
#160243=CARTESIAN_POINT('Ctrl Pts',(5.7430406985932,4.83620904384686,4.59504345844529));
#160244=CARTESIAN_POINT('Ctrl Pts',(5.75635086562983,4.83886483070819,4.60552622532028));
#160245=CARTESIAN_POINT('Ctrl Pts',(5.7696582853675,4.84149471138958,4.61601907864709));
#160246=CARTESIAN_POINT('Ctrl Pts',(5.78296299265857,4.84409946425117,4.62652156278843));
#160247=CARTESIAN_POINT('Ctrl Pts',(5.35212840517261,4.94924836941368,5.12017042975023));
#160248=CARTESIAN_POINT('Ctrl Pts',(5.35489854658631,4.94861077170684,5.11726850637511));
#160249=CARTESIAN_POINT('Ctrl Pts',(5.357668688,4.94797317400001,5.114366583));
#160250=CARTESIAN_POINT('Ctrl Pts',(5.636277158,4.88384644,4.82250407099999));
#160251=CARTESIAN_POINT('Ctrl Pts',(5.88153221,4.818610636,4.50210375));
#160252=CARTESIAN_POINT('Ctrl Pts',(5.13261580896174,4.94924836941368,5.12043129408338));
#160253=CARTESIAN_POINT('Ctrl Pts',(5.13538622048087,4.94861077170684,5.11764826704169));
#160254=CARTESIAN_POINT('Ctrl Pts',(5.138156632,4.94797317400001,5.11486524));
#160255=CARTESIAN_POINT('Ctrl Pts',(5.416792268,4.88384644,4.834960791));
#160256=CARTESIAN_POINT('Ctrl Pts',(5.663373315,4.818610636,4.526444819));
#160257=CARTESIAN_POINT('',(5.175034871687,4.94797317334255,5.11478146784614));
#160258=CARTESIAN_POINT('Ctrl Pts',(5.13592472148641,4.94745154526473,5.11710731389588));
#160259=CARTESIAN_POINT('Ctrl Pts',(5.13704067674321,4.94771235963237,5.11598627694794));
#160260=CARTESIAN_POINT('Ctrl Pts',(5.138156632,4.947973174,5.11486524));
#160261=CARTESIAN_POINT('Ctrl Pts',(5.249895753,4.974088171,5.002617296));
#160262=CARTESIAN_POINT('Ctrl Pts',(5.356626283,5.00031307,4.885596675));
#160263=CARTESIAN_POINT('Ctrl Pts',(5.20968127961232,4.94745154526473,5.11697194808294));
#160264=CARTESIAN_POINT('Ctrl Pts',(5.21079719830616,4.94771235963237,5.11583481904147));
#160265=CARTESIAN_POINT('Ctrl Pts',(5.211913117,4.947973174,5.11469769));
#160266=CARTESIAN_POINT('Ctrl Pts',(5.323648577,4.974088171,5.000838466));
#160267=CARTESIAN_POINT('Ctrl Pts',(5.430305083,5.00031307,4.88220826));
#160268=CARTESIAN_POINT('Origin',(-0.155143030563726,5.08925727759442,-0.121555994973399));
#160269=CARTESIAN_POINT('Ctrl Pts',(5.136953033,4.94766207,5.17970211));
#160270=CARTESIAN_POINT('Ctrl Pts',(5.250782913,4.97393188700001,5.06681169));
#160271=CARTESIAN_POINT('Ctrl Pts',(5.359543499,5.00031307,4.949029591));
#160272=CARTESIAN_POINT('Ctrl Pts',(5.136825309,4.94766207,5.116202277));
#160273=CARTESIAN_POINT('Ctrl Pts',(5.249259707,4.97393188700001,5.003314665));
#160274=CARTESIAN_POINT('Ctrl Pts',(5.356626283,5.00031307,4.885596675));
#160275=CARTESIAN_POINT('Ctrl Pts',(5.13815809084062,4.94797287201475,5.11486392257979));
#160276=CARTESIAN_POINT('Ctrl Pts',(5.14182969055117,4.94882769741438,5.11857833976555));
#160277=CARTESIAN_POINT('Ctrl Pts',(5.1455024010555,4.94967947055841,5.12229236245135));
#160278=CARTESIAN_POINT('Ctrl Pts',(5.14917479227229,4.95052852744747,5.12600732004938));
#160279=CARTESIAN_POINT('Ctrl Pts',(5.15258409735191,4.95131675881877,5.12945614210069));
#160280=CARTESIAN_POINT('Ctrl Pts',(5.15599312825447,4.95210264921763,5.13290577107319));
#160281=CARTESIAN_POINT('Ctrl Pts',(5.15940188569591,4.95288622035444,5.13635619600154));
#160282=CARTESIAN_POINT('Ctrl Pts',(5.16281064658125,4.9536697922829,5.13980662441589));
#160283=CARTESIAN_POINT('Ctrl Pts',(5.1662191348642,4.95445104514204,5.14325784965854));
#160284=CARTESIAN_POINT('Ctrl Pts',(5.1696273514169,4.95523000038884,5.14670986113548));
#160285=CARTESIAN_POINT('Ctrl Pts',(4.969103039,5.000313899,5.340937689));
#160286=CARTESIAN_POINT('Ctrl Pts',(5.050820094,4.98224132,5.264909753));
#160287=CARTESIAN_POINT('Ctrl Pts',(5.130172969,4.964285714,5.186417426));
#160288=CARTESIAN_POINT('Ctrl Pts',(5.16685149900001,4.955986264,5.150136659));
#160289=CARTESIAN_POINT('Ctrl Pts',(5.203013228,4.947660853,5.113340763));
#160290=CARTESIAN_POINT('Ctrl Pts',(4.905659624,5.000313899,5.338258485));
#160291=CARTESIAN_POINT('Ctrl Pts',(4.987335687,4.98224132,5.263201242));
#160292=CARTESIAN_POINT('Ctrl Pts',(5.066677286,4.964285714,5.185680407));
#160293=CARTESIAN_POINT('Ctrl Pts',(5.103350603,4.955986264,5.149848684));
#160294=CARTESIAN_POINT('Ctrl Pts',(5.139513471,4.947660853,5.113501861));
#160295=CARTESIAN_POINT('Ctrl Pts',(5.1381573905858,4.9479730331745,5.11486462602031));
#160296=CARTESIAN_POINT('Ctrl Pts',(5.11447664210774,4.95342302529756,5.13865310318677));
#160297=CARTESIAN_POINT('Ctrl Pts',(5.09064856021101,4.95886083272451,5.16225923533607));
#160298=CARTESIAN_POINT('Ctrl Pts',(5.06667728621878,4.96428571397019,5.1856804068723));
#160299=CARTESIAN_POINT('Ctrl Pts',(5.01433181580533,4.97613189117016,5.23682463158556));
#160300=CARTESIAN_POINT('Ctrl Pts',(4.96112242201154,4.98803923912007,5.28726340536358));
#160301=CARTESIAN_POINT('Ctrl Pts',(4.90707810144186,5.00000000032828,5.3369546096604));
#160302=CARTESIAN_POINT('Ctrl Pts',(4.905659624,5.000313899,5.338258485));
#160303=CARTESIAN_POINT('Ctrl Pts',(4.987335687,4.98224132,5.263201242));
#160304=CARTESIAN_POINT('Ctrl Pts',(5.066677286,4.964285714,5.185680407));
#160305=CARTESIAN_POINT('Ctrl Pts',(5.102662666,4.95614194999999,5.150520834));
#160306=CARTESIAN_POINT('Ctrl Pts',(5.138156632,4.947973174,5.11486524));
#160307=CARTESIAN_POINT('Ctrl Pts',(4.902547666,5.000313899,5.41194948));
#160308=CARTESIAN_POINT('Ctrl Pts',(4.985351212,4.98224132,5.33693985));
#160309=CARTESIAN_POINT('Ctrl Pts',(5.065821221,4.964285714,5.259432113));
#160310=CARTESIAN_POINT('Ctrl Pts',(5.102318391,4.95614194999999,5.224278481));
#160311=CARTESIAN_POINT('Ctrl Pts',(5.138324182,4.947973174,5.188621724));
#160312=CARTESIAN_POINT('',(5.13840595762541,4.94797317334228,5.22462127032716));
#160313=CARTESIAN_POINT('Ctrl Pts',(4.527175975,4.818630405,5.862255283));
#160314=CARTESIAN_POINT('Ctrl Pts',(4.534162896,4.820029867,5.856859574));
#160315=CARTESIAN_POINT('Ctrl Pts',(4.541136935,4.821428571,5.851447226));
#160316=CARTESIAN_POINT('Ctrl Pts',(4.853706394,4.884117105,5.608871218));
#160317=CARTESIAN_POINT('Ctrl Pts',(5.138655289,4.947973174,5.334377295));
#160318=CARTESIAN_POINT('Ctrl Pts',(4.550585316,4.818630405,5.643994444));
#160319=CARTESIAN_POINT('Ctrl Pts',(4.557312103,4.820029867,5.638570835));
#160320=CARTESIAN_POINT('Ctrl Pts',(4.564025943,4.821428571,5.633131207));
#160321=CARTESIAN_POINT('Ctrl Pts',(4.864933514,4.884117105,5.389332525));
#160322=CARTESIAN_POINT('Ctrl Pts',(5.138156632,4.947973174,5.11486524));
#160323=CARTESIAN_POINT('Ctrl Pts',(4.55424020907722,4.81939091801857,5.64104568384217));
#160324=CARTESIAN_POINT('Ctrl Pts',(4.56573507336455,4.82234724734205,5.65499942765427));
#160325=CARTESIAN_POINT('Ctrl Pts',(4.57723334628362,4.82527010319568,5.66895751963913));
#160326=CARTESIAN_POINT('Ctrl Pts',(4.5887221569022,4.82816321758488,5.68292951270901));
#160327=CARTESIAN_POINT('Ctrl Pts',(4.59947743918297,4.83087161473403,5.69600943320562));
#160328=CARTESIAN_POINT('Ctrl Pts',(4.61022770116185,4.83355328560802,5.7090990456699));
#160329=CARTESIAN_POINT('Ctrl Pts',(4.62097308340232,4.83620904394719,5.72219788303831));
#160330=CARTESIAN_POINT('Ctrl Pts',(4.63171858101127,4.83886483080008,5.73529686104324));
#160331=CARTESIAN_POINT('Ctrl Pts',(4.64245922725937,4.84149471147249,5.74840509909905));
#160332=CARTESIAN_POINT('Ctrl Pts',(4.65319515431945,4.84409946436975,5.76152215993885));
#160333=CARTESIAN_POINT('Ctrl Pts',(4.12631332540522,4.94924836941368,6.15101308899583));
#160334=CARTESIAN_POINT('Ctrl Pts',(4.12964253020261,4.94861077170684,6.14877450949792));
#160335=CARTESIAN_POINT('Ctrl Pts',(4.132971735,4.94797317400001,6.14653593));
#160336=CARTESIAN_POINT('Ctrl Pts',(4.467808307,4.88384644,5.921389587));
#160337=CARTESIAN_POINT('Ctrl Pts',(4.77620603,4.818610636,5.661202634));
#160338=CARTESIAN_POINT('Ctrl Pts',(3.91187673525438,4.94924836941368,6.10407913568029));
#160339=CARTESIAN_POINT('Ctrl Pts',(3.91518064462719,4.94861077170684,6.10195673084015));
#160340=CARTESIAN_POINT('Ctrl Pts',(3.918484554,4.94797317400001,6.099834326));
#160341=CARTESIAN_POINT('Ctrl Pts',(4.250777025,4.88384644,5.886372312));
#160342=CARTESIAN_POINT('Ctrl Pts',(4.557914959,4.818610636,5.638076909));
#160343=CARTESIAN_POINT('',(3.95451860864093,4.94797317334255,6.10768024367488));
#160344=CARTESIAN_POINT('Ctrl Pts',(3.91582284472911,4.94745154526473,6.1015441866602));
#160345=CARTESIAN_POINT('Ctrl Pts',(3.91715369936455,4.94771235963237,6.1006892563301));
#160346=CARTESIAN_POINT('Ctrl Pts',(3.918484554,4.947973174,6.099834326));
#160347=CARTESIAN_POINT('Ctrl Pts',(4.051741265,4.974088171,6.014231285));
#160348=CARTESIAN_POINT('Ctrl Pts',(4.181132469,5.00031307,5.922890449));
#160349=CARTESIAN_POINT('Ctrl Pts',(3.98788411345982,4.94745154526474,6.11726746511525));
#160350=CARTESIAN_POINT('Ctrl Pts',(3.98921839172991,4.94771235963237,6.11639681105762));
#160351=CARTESIAN_POINT('Ctrl Pts',(3.99055267,4.947973174,6.115526157));
#160352=CARTESIAN_POINT('Ctrl Pts',(4.124152185,4.974088171,6.02834872));
#160353=CARTESIAN_POINT('Ctrl Pts',(4.253817109,5.00031307,5.935420018));
#160354=CARTESIAN_POINT('Origin',(-0.125384865003265,5.08925684212034,-0.152065231848668));
#160355=CARTESIAN_POINT('Ctrl Pts',(3.903371084,4.94766207,6.162896608));
#160356=CARTESIAN_POINT('Ctrl Pts',(4.038807786,4.973931887,6.077115563));
#160357=CARTESIAN_POINT('Ctrl Pts',(4.170345281,5.00031307,5.985467455));
#160358=CARTESIAN_POINT('Ctrl Pts',(3.916896932,4.94766207,6.100853909));
#160359=CARTESIAN_POINT('Ctrl Pts',(4.050970176,4.973931887,6.014775618));
#160360=CARTESIAN_POINT('Ctrl Pts',(4.181132469,5.00031307,5.922890449));
#160361=CARTESIAN_POINT('Ctrl Pts',(3.91848626136233,4.94797287209023,6.0998333531052));
#160362=CARTESIAN_POINT('Ctrl Pts',(3.92127353100262,4.94882769745733,6.10425021460731));
#160363=CARTESIAN_POINT('Ctrl Pts',(3.92406197047932,4.94967947057366,6.10866692966534));
#160364=CARTESIAN_POINT('Ctrl Pts',(3.92684989716656,4.95052852744272,6.11308448915988));
#160365=CARTESIAN_POINT('Ctrl Pts',(3.92943809980516,4.95131675879719,6.11718557947632));
#160366=CARTESIAN_POINT('Ctrl Pts',(3.93202586122446,4.95210264918639,6.12128739892803));
#160367=CARTESIAN_POINT('Ctrl Pts',(3.93461318446858,4.95288622031634,6.12538993694027));
#160368=CARTESIAN_POINT('Ctrl Pts',(3.93720051032669,4.95366979223794,6.12949247909733));
#160369=CARTESIAN_POINT('Ctrl Pts',(3.9397873986607,4.95445104509302,6.1335957408516));
#160370=CARTESIAN_POINT('Ctrl Pts',(3.94237385257086,4.95523000032935,6.13769971199802));
#160371=CARTESIAN_POINT('Ctrl Pts',(3.704784445,5.000313899,6.284279802));
#160372=CARTESIAN_POINT('Ctrl Pts',(3.80093476,4.98224132,6.227596108));
#160373=CARTESIAN_POINT('Ctrl Pts',(3.895305939,4.964285714,6.16799741));
#160374=CARTESIAN_POINT('Ctrl Pts',(3.938926237,4.955986264,6.140449667));
#160375=CARTESIAN_POINT('Ctrl Pts',(3.982152555,4.947660853,6.112287742));
#160376=CARTESIAN_POINT('Ctrl Pts',(3.643400252,5.000313899,6.268024777));
#160377=CARTESIAN_POINT('Ctrl Pts',(3.739301863,4.98224132,6.21228027));
#160378=CARTESIAN_POINT('Ctrl Pts',(3.833453187,4.964285714,6.153627927));
#160379=CARTESIAN_POINT('Ctrl Pts',(3.876971864,4.955986264,6.126517609));
#160380=CARTESIAN_POINT('Ctrl Pts',(3.920102756,4.947660853,6.098794502));
#160381=CARTESIAN_POINT('Ctrl Pts',(3.9184854264898,4.94797303320567,6.09983388941806));
#160382=CARTESIAN_POINT('Ctrl Pts',(3.890244500683,4.95342302541711,6.1179755445405));
#160383=CARTESIAN_POINT('Ctrl Pts',(3.86189888534793,4.95886083283601,6.13590744510505));
#160384=CARTESIAN_POINT('Ctrl Pts',(3.83345318681619,4.96428571407458,6.15362792729177));
#160385=CARTESIAN_POINT('Ctrl Pts',(3.77133702917533,4.9761318912024,6.19232369985351));
#160386=CARTESIAN_POINT('Ctrl Pts',(3.70852879586539,4.98803923906917,6.23014479602785));
#160387=CARTESIAN_POINT('Ctrl Pts',(3.64506586129705,5.00000000025158,6.26705631602723));
#160388=CARTESIAN_POINT('Ctrl Pts',(3.643400252,5.000313899,6.268024777));
#160389=CARTESIAN_POINT('Ctrl Pts',(3.739301863,4.98224132,6.21228027));
#160390=CARTESIAN_POINT('Ctrl Pts',(3.833453187,4.964285714,6.153627927));
#160391=CARTESIAN_POINT('Ctrl Pts',(3.876155517,4.95614194999999,6.127026159));
#160392=CARTESIAN_POINT('Ctrl Pts',(3.918484554,4.947973174,6.099834326));
#160393=CARTESIAN_POINT('Ctrl Pts',(3.624519664,5.000313899,6.339323939));
#160394=CARTESIAN_POINT('Ctrl Pts',(3.721512162,4.98224132,6.283868307));
#160395=CARTESIAN_POINT('Ctrl Pts',(3.816762699,4.964285714,6.225471331));
#160396=CARTESIAN_POINT('Ctrl Pts',(3.859963578,4.95614194999999,6.198985384));
#160397=CARTESIAN_POINT('Ctrl Pts',(3.902792722,4.947973174,6.171902443));
#160398=CARTESIAN_POINT('',(3.89513374808462,4.94797317334224,6.20707791914326));
#160399=CARTESIAN_POINT('Ctrl Pts',(3.161121518,4.818630405,6.698408024));
#160400=CARTESIAN_POINT('Ctrl Pts',(3.169105006,4.820029867,6.694640446));
#160401=CARTESIAN_POINT('Ctrl Pts',(3.177079491,4.821428571,6.690853848));
#160402=CARTESIAN_POINT('Ctrl Pts',(3.534487921,4.884117105,6.521142326));
#160403=CARTESIAN_POINT('Ctrl Pts',(3.871782949,4.947973174,6.314321508));
#160404=CARTESIAN_POINT('Ctrl Pts',(3.23090319,4.818630405,6.490282319));
#160405=CARTESIAN_POINT('Ctrl Pts',(3.238638624,4.820029867,6.486431571));
#160406=CARTESIAN_POINT('Ctrl Pts',(3.246364857,4.821428571,6.482562396));
#160407=CARTESIAN_POINT('Ctrl Pts',(3.592646886,4.884117105,6.309149825));
#160408=CARTESIAN_POINT('Ctrl Pts',(3.918484554,4.947973174,6.099834326));
#160409=CARTESIAN_POINT('Ctrl Pts',(3.2351065298675,4.8193909179172,6.4881881934962));
#160410=CARTESIAN_POINT('Ctrl Pts',(3.24333300793021,4.82234724737653,6.50428676221164));
#160411=CARTESIAN_POINT('Ctrl Pts',(3.25156188047758,4.8252701031888,6.52039031048622));
#160412=CARTESIAN_POINT('Ctrl Pts',(3.25977852354582,4.82816321755467,6.53650540076862));
#160413=CARTESIAN_POINT('Ctrl Pts',(3.26747055705677,4.83087161470281,6.55159158784706));
#160414=CARTESIAN_POINT('Ctrl Pts',(3.27515560415933,4.83355328557703,6.56668616107939));
#160415=CARTESIAN_POINT('Ctrl Pts',(3.28283390253395,4.83620904391764,6.58178869453964));
#160416=CARTESIAN_POINT('Ctrl Pts',(3.2905122833471,4.83886483077196,6.59689139014914));
#160417=CARTESIAN_POINT('Ctrl Pts',(3.2981839355909,4.84149471144699,6.61200208641192));
#160418=CARTESIAN_POINT('Ctrl Pts',(3.30584908222536,4.84409946430701,6.62712038446017));
#160419=CARTESIAN_POINT('Ctrl Pts',(2.70755642147094,4.94924836941368,6.89424121325815));
#160420=CARTESIAN_POINT('Ctrl Pts',(2.71128901973547,4.94861077170684,6.89277065112908));
#160421=CARTESIAN_POINT('Ctrl Pts',(2.715021618,4.94797317400001,6.891300089));
#160422=CARTESIAN_POINT('Ctrl Pts',(3.090429706,4.88384644,6.743397508));
#160423=CARTESIAN_POINT('Ctrl Pts',(3.447549765,4.818610636,6.555589976));
#160424=CARTESIAN_POINT('Ctrl Pts',(2.50822265177515,4.94924836941368,6.80230702168493));
#160425=CARTESIAN_POINT('Ctrl Pts',(2.51190557188757,4.94861077170684,6.80094448034247));
#160426=CARTESIAN_POINT('Ctrl Pts',(2.515588492,4.94797317400001,6.799581939));
#160427=CARTESIAN_POINT('Ctrl Pts',(2.886000173,4.88384644,6.662543607));
#160428=CARTESIAN_POINT('Ctrl Pts',(3.239333565,4.818610636,6.486078789));
#160429=CARTESIAN_POINT('',(2.54909345025193,4.94797317334255,6.81499067990194));
#160430=CARTESIAN_POINT('Ctrl Pts',(2.51262144250503,4.94745154526473,6.80067963526152));
#160431=CARTESIAN_POINT('Ctrl Pts',(2.51410496725252,4.94771235963237,6.80013078713076));
#160432=CARTESIAN_POINT('Ctrl Pts',(2.515588492,4.947973174,6.799581939));
#160433=CARTESIAN_POINT('Ctrl Pts',(2.664131859,4.974088171,6.744626503));
#160434=CARTESIAN_POINT('Ctrl Pts',(2.810133548,5.00031307,6.68323645));
#160435=CARTESIAN_POINT('Ctrl Pts',(2.57961791904852,4.94745154526473,6.83152635453666));
#160436=CARTESIAN_POINT('Ctrl Pts',(2.58110816752426,4.94771235963237,6.83096288626833));
#160437=CARTESIAN_POINT('Ctrl Pts',(2.582598416,4.947973174,6.830399418));
#160438=CARTESIAN_POINT('Ctrl Pts',(2.731815021,4.974088171,6.773980087));
#160439=CARTESIAN_POINT('Ctrl Pts',(2.878425375,5.00031307,6.711098133));
#160440=CARTESIAN_POINT('Origin',(-0.089764152265116,5.08925712536846,-0.175464601845655));
#160441=CARTESIAN_POINT('Ctrl Pts',(2.48727184,4.94766207,6.85792091));
#160442=CARTESIAN_POINT('Ctrl Pts',(2.637982497,4.97393188700001,6.803260266));
#160443=CARTESIAN_POINT('Ctrl Pts',(2.786146352,5.00031307,6.742031513));
#160444=CARTESIAN_POINT('Ctrl Pts',(2.513818808,4.94766207,6.800236393));
#160445=CARTESIAN_POINT('Ctrl Pts',(2.663261782,4.97393188700001,6.744992349));
#160446=CARTESIAN_POINT('Ctrl Pts',(2.810133548,5.00031307,6.68323645));
#160447=CARTESIAN_POINT('Ctrl Pts',(2.51559036884464,4.94797287220619,6.79958135590101));
#160448=CARTESIAN_POINT('Ctrl Pts',(2.51736297941983,4.94882769749915,6.80449413410756));
#160449=CARTESIAN_POINT('Ctrl Pts',(2.51913676346908,4.94967947062019,6.80940702092935));
#160450=CARTESIAN_POINT('Ctrl Pts',(2.52090986519437,4.95052852749235,6.81432062220744));
#160451=CARTESIAN_POINT('Ctrl Pts',(2.52255594381641,4.9513167588421,6.81888221836729));
#160452=CARTESIAN_POINT('Ctrl Pts',(2.5242014347969,4.95210264922525,6.82344443176355));
#160453=CARTESIAN_POINT('Ctrl Pts',(2.52584634338302,4.95288622034841,6.82800725272412));
#160454=CARTESIAN_POINT('Ctrl Pts',(2.527491253631,4.95366979226322,6.83257007829454));
#160455=CARTESIAN_POINT('Ctrl Pts',(2.52913558189762,4.95445104511072,6.83713351258166));
#160456=CARTESIAN_POINT('Ctrl Pts',(2.53077933337913,4.95523000032694,6.84169754621404));
#160457=CARTESIAN_POINT('Ctrl Pts',(2.267234248,5.000313899,6.933775975));
#160458=CARTESIAN_POINT('Ctrl Pts',(2.373321941,4.98224132,6.89908699));
#160459=CARTESIAN_POINT('Ctrl Pts',(2.478298732,4.964285714,6.861168691));
#160460=CARTESIAN_POINT('Ctrl Pts',(2.526821163,4.955986264,6.843642074));
#160461=CARTESIAN_POINT('Ctrl Pts',(2.575090855,4.947660853,6.825430939));
#160462=CARTESIAN_POINT('Ctrl Pts',(2.210779533,5.000313899,6.904705197));
#160463=CARTESIAN_POINT('Ctrl Pts',(2.316422439,4.98224132,6.870879977));
#160464=CARTESIAN_POINT('Ctrl Pts',(2.420981077,4.964285714,6.833838645));
#160465=CARTESIAN_POINT('Ctrl Pts',(2.469310228,4.955986264,6.81671738));
#160466=CARTESIAN_POINT('Ctrl Pts',(2.517392394,4.947660853,6.798914291));
#160467=CARTESIAN_POINT('Ctrl Pts',(2.51558943810921,4.94797303333726,6.79958170023568));
#160468=CARTESIAN_POINT('Ctrl Pts',(2.48410885035045,4.95342302538865,6.81122824905784));
#160469=CARTESIAN_POINT('Ctrl Pts',(2.4525711111243,4.95886083276052,6.82264744228887));
#160470=CARTESIAN_POINT('Ctrl Pts',(2.42098107736794,4.96428571399539,6.83383864515312));
#160471=CARTESIAN_POINT('Ctrl Pts',(2.35199871314928,4.97613189113004,6.85827659379836));
#160472=CARTESIAN_POINT('Ctrl Pts',(2.28252848394537,4.9880392390776,6.88171154060857));
#160473=CARTESIAN_POINT('Ctrl Pts',(2.21261439168749,5.00000000026428,6.90411743489196));
#160474=CARTESIAN_POINT('Ctrl Pts',(2.210779533,5.000313899,6.904705197));
#160475=CARTESIAN_POINT('Ctrl Pts',(2.316422439,4.98224132,6.870879977));
#160476=CARTESIAN_POINT('Ctrl Pts',(2.420981077,4.964285714,6.833838645));
#160477=CARTESIAN_POINT('Ctrl Pts',(2.468403645,4.95614194999999,6.81703855));
#160478=CARTESIAN_POINT('Ctrl Pts',(2.515588492,4.947973174,6.799581939));
#160479=CARTESIAN_POINT('Ctrl Pts',(2.177013151,5.000313899,6.970278656));
#160480=CARTESIAN_POINT('Ctrl Pts',(2.283659339,4.98224132,6.936970065));
#160481=CARTESIAN_POINT('Ctrl Pts',(2.389236596,4.964285714,6.900414428));
#160482=CARTESIAN_POINT('Ctrl Pts',(2.437121158,4.95614194999999,6.88383462));
#160483=CARTESIAN_POINT('Ctrl Pts',(2.484771012,4.947973174,6.866591863));
#160484=CARTESIAN_POINT('',(2.4697294127037,4.94797317334223,6.89929850335895));
#160485=CARTESIAN_POINT('Ctrl Pts',(1.647256531,4.818630405,7.221350651));
#160486=CARTESIAN_POINT('Ctrl Pts',(1.655863289,4.820029867,7.219387371));
#160487=CARTESIAN_POINT('Ctrl Pts',(1.664465341,4.821428571,7.21740358));
#160488=CARTESIAN_POINT('Ctrl Pts',(2.050000721,4.884117105,7.128492066));
#160489=CARTESIAN_POINT('Ctrl Pts',(2.423870341,4.947973174,6.999015065));
#160490=CARTESIAN_POINT('Ctrl Pts',(1.760147622,4.818630405,7.033091806));
#160491=CARTESIAN_POINT('Ctrl Pts',(1.768530003,4.820029867,7.030993976));
#160492=CARTESIAN_POINT('Ctrl Pts',(1.776907359,4.821428571,7.028876172));
#160493=CARTESIAN_POINT('Ctrl Pts',(2.152372083,4.884117105,6.933958291));
#160494=CARTESIAN_POINT('Ctrl Pts',(2.515588492,4.947973174,6.799581939));
#160495=CARTESIAN_POINT('Ctrl Pts',(1.76470286479964,4.81939091791719,7.03195023316287));
#160496=CARTESIAN_POINT('Ctrl Pts',(1.76927629608275,4.82234724726155,7.04944087630683));
#160497=CARTESIAN_POINT('Ctrl Pts',(1.77385099516533,4.82527010308462,7.06693689689648));
#160498=CARTESIAN_POINT('Ctrl Pts',(1.77841126959503,4.82816321744559,7.08444156064864));
#160499=CARTESIAN_POINT('Ctrl Pts',(1.78268038335581,4.83087161460903,7.10082860095823));
#160500=CARTESIAN_POINT('Ctrl Pts',(1.78694087127104,4.8335532854988,7.11722232948686));
#160501=CARTESIAN_POINT('Ctrl Pts',(1.79119305702643,4.83620904385498,7.13362238136058));
#160502=CARTESIAN_POINT('Ctrl Pts',(1.79544528843569,4.83886483072488,7.15002260931446));
#160503=CARTESIAN_POINT('Ctrl Pts',(1.79968922868213,4.84149471141551,7.16642920442718));
#160504=CARTESIAN_POINT('Ctrl Pts',(1.80392518127354,4.84409946430028,7.18284182514446));
#160505=CARTESIAN_POINT('Ctrl Pts',(1.16219718885009,4.94924836941368,7.31510228082506));
#160506=CARTESIAN_POINT('Ctrl Pts',(1.16615864842505,4.94861077170684,7.31446849791253));
#160507=CARTESIAN_POINT('Ctrl Pts',(1.170120108,4.94797317400001,7.31383471500001));
#160508=CARTESIAN_POINT('Ctrl Pts',(1.568546046,4.88384644,7.250091656));
#160509=CARTESIAN_POINT('Ctrl Pts',(1.957689904,4.818610636,7.143445216));
#160510=CARTESIAN_POINT('Ctrl Pts',(0.987286864787931,4.94924836941368,
7.18246659083401));
#160511=CARTESIAN_POINT('Ctrl Pts',(0.991176586393966,4.94861077170684,
7.18192762391701));
#160512=CARTESIAN_POINT('Ctrl Pts',(0.995066308,4.94797317400001,7.181388657));
#160513=CARTESIAN_POINT('Ctrl Pts',(1.386277161,4.88384644,7.127181768));
#160514=CARTESIAN_POINT('Ctrl Pts',(1.769284534,4.818610636,7.030798834));
#160515=CARTESIAN_POINT('',(1.02447551553818,4.94797317334255,7.20363972606343));
#160516=CARTESIAN_POINT('Ctrl Pts',(0.991932654222761,4.94745154526474,
7.18182286178785));
#160517=CARTESIAN_POINT('Ctrl Pts',(0.99349948111138,4.94771235963237,7.18160575939393));
#160518=CARTESIAN_POINT('Ctrl Pts',(0.995066308,4.947973174,7.181388657));
#160519=CARTESIAN_POINT('Ctrl Pts',(1.151950608,4.974088171,7.159650482));
#160520=CARTESIAN_POINT('Ctrl Pts',(1.307735906,5.00031307,7.131081741));
#160521=CARTESIAN_POINT('Ctrl Pts',(1.05073165838991,4.94745154526473,7.22635066464237));
#160522=CARTESIAN_POINT('Ctrl Pts',(1.05230819469495,4.94771235963237,7.22612072932119));
#160523=CARTESIAN_POINT('Ctrl Pts',(1.053884731,4.947973174,7.225890794));
#160524=CARTESIAN_POINT('Ctrl Pts',(1.211741222,4.974088171,7.202867675));
#160525=CARTESIAN_POINT('Ctrl Pts',(1.368441669,5.00031307,7.172972758));
#160526=CARTESIAN_POINT('Origin',(-0.0499455387825083,5.08925704570198,
-0.190657335926088));
#160527=CARTESIAN_POINT('Ctrl Pts',(0.95487053,4.94766207,7.23227645200001));
#160528=CARTESIAN_POINT('Ctrl Pts',(1.113808078,4.97393188700001,7.21129208));
#160529=CARTESIAN_POINT('Ctrl Pts',(1.271670316,5.00031307,7.18334567));
#160530=CARTESIAN_POINT('Ctrl Pts',(0.993197311,4.94766207,7.18164738100001));
#160531=CARTESIAN_POINT('Ctrl Pts',(1.151022227,4.97393188700001,7.159820734));
#160532=CARTESIAN_POINT('Ctrl Pts',(1.307735906,5.00031307,7.131081741));
#160533=CARTESIAN_POINT('Ctrl Pts',(0.995068266814636,4.94797287211291,
7.18138849127666));
#160534=CARTESIAN_POINT('Ctrl Pts',(0.995743332761482,4.94882769742648,
7.18656747044334));
#160535=CARTESIAN_POINT('Ctrl Pts',(0.99641952126286,4.94967947057192,7.19174680788969));
#160536=CARTESIAN_POINT('Ctrl Pts',(0.997094889799226,4.95052852746446,
7.19692669639858));
#160537=CARTESIAN_POINT('Ctrl Pts',(0.997721875648572,4.95131675882001,
7.20173550317798));
#160538=CARTESIAN_POINT('Ctrl Pts',(0.998348154901802,4.9521026492053,7.20654478642679));
#160539=CARTESIAN_POINT('Ctrl Pts',(0.998973734766601,4.95288622032942,
7.21135453783823));
#160540=CARTESIAN_POINT('Ctrl Pts',(0.999599315263429,4.95366979224519,
7.21616429410901));
#160541=CARTESIAN_POINT('Ctrl Pts',(1.00022419652744,4.95445104509255,7.22097451975665));
#160542=CARTESIAN_POINT('Ctrl Pts',(1.00084838567572,4.95523000033943,7.22578520694037));
#160543=CARTESIAN_POINT('Ctrl Pts',(0.723670697,5.000313899,7.259056491));
#160544=CARTESIAN_POINT('Ctrl Pts',(0.834735225,4.98224132,7.247984233));
#160545=CARTESIAN_POINT('Ctrl Pts',(0.945409031,4.964285714,7.233519349));
#160546=CARTESIAN_POINT('Ctrl Pts',(0.996564739,4.955986264,7.226833383));
#160547=CARTESIAN_POINT('Ctrl Pts',(1.047620768,4.947660853,7.219424571));
#160548=CARTESIAN_POINT('Ctrl Pts',(0.67478522,5.000313899,7.218529276));
#160549=CARTESIAN_POINT('Ctrl Pts',(0.785229676,4.98224132,7.208204972));
#160550=CARTESIAN_POINT('Ctrl Pts',(0.895306583,4.964285714,7.194506663));
#160551=CARTESIAN_POINT('Ctrl Pts',(0.946186392000001,4.955986264,7.188175023));
#160552=CARTESIAN_POINT('Ctrl Pts',(0.99697156,4.947660853,7.181124404));
#160553=CARTESIAN_POINT('Ctrl Pts',(0.99506728359157,4.94797303328102,7.18138862751167));
#160554=CARTESIAN_POINT('Ctrl Pts',(0.961819030399578,4.95342302542127,
7.18599549061261));
#160555=CARTESIAN_POINT('Ctrl Pts',(0.928563837219034,4.95886083281524,
7.19036802794514));
#160556=CARTESIAN_POINT('Ctrl Pts',(0.895306583038016,4.96428571399449,
7.19450666299911));
#160557=CARTESIAN_POINT('Ctrl Pts',(0.822683552230544,4.97613189103025,
7.20354409641358));
#160558=CARTESIAN_POINT('Ctrl Pts',(0.749799676836577,4.98803923906901,
7.21149710151008));
#160559=CARTESIAN_POINT('Ctrl Pts',(0.676703532269287,5.00000000025134,
7.21834969580106));
#160560=CARTESIAN_POINT('Ctrl Pts',(0.67478522,5.000313899,7.218529276));
#160561=CARTESIAN_POINT('Ctrl Pts',(0.785229676,4.98224132,7.208204972));
#160562=CARTESIAN_POINT('Ctrl Pts',(0.895306583,4.964285714,7.194506663));
#160563=CARTESIAN_POINT('Ctrl Pts',(0.945231961,4.95614194999999,7.188293795));
#160564=CARTESIAN_POINT('Ctrl Pts',(0.995066308,4.947973174,7.181388657));
#160565=CARTESIAN_POINT('Ctrl Pts',(0.627711922,5.000313899,7.275310889));
#160566=CARTESIAN_POINT('Ctrl Pts',(0.739025144,4.98224132,7.265706814));
#160567=CARTESIAN_POINT('Ctrl Pts',(0.849992445,4.964285714,7.252701816));
#160568=CARTESIAN_POINT('Ctrl Pts',(0.900321661,4.95614194999999,7.2468034));
#160569=CARTESIAN_POINT('Ctrl Pts',(0.950564171,4.947973174,7.240207079));
#160570=CARTESIAN_POINT('',(0.928843275000543,4.94797317334227,7.26891555701107));
#160571=CARTESIAN_POINT('Ctrl Pts',(0.056367661,4.818630405,7.406630948));
#160572=CARTESIAN_POINT('Ctrl Pts',(0.065195244,4.820029867,7.406563766));
#160573=CARTESIAN_POINT('Ctrl Pts',(0.074022642,4.821428571,7.406475542));
#160574=CARTESIAN_POINT('Ctrl Pts',(0.469657766,4.884117105,7.402521441));
#160575=CARTESIAN_POINT('Ctrl Pts',(0.86262025,4.947973174,7.35644245600001));
#160576=CARTESIAN_POINT('Ctrl Pts',(0.207089507,4.818630405,7.24704173700001));
#160577=CARTESIAN_POINT('Ctrl Pts',(0.215726884,4.820029867,7.246794918));
#160578=CARTESIAN_POINT('Ctrl Pts',(0.224363648,4.821428571,7.24652751));
#160579=CARTESIAN_POINT('Ctrl Pts',(0.611454754,4.884117105,7.234542573));
#160580=CARTESIAN_POINT('Ctrl Pts',(0.995066308,4.947973174,7.181388657));
#160581=CARTESIAN_POINT('Ctrl Pts',(0.211783655067681,4.81939091801857,
7.24690609670381));
#160582=CARTESIAN_POINT('Ctrl Pts',(0.212490191699886,4.8223472472686,7.26497097077347));
#160583=CARTESIAN_POINT('Ctrl Pts',(0.21319680923074,4.82527010317956,7.2830413693019));
#160584=CARTESIAN_POINT('Ctrl Pts',(0.213887481742358,4.82816321755752,
7.30111710804181));
#160585=CARTESIAN_POINT('Ctrl Pts',(0.214534056753162,4.83087161470481,
7.31803876161052));
#160586=CARTESIAN_POINT('Ctrl Pts',(0.215170769813655,4.8335532855769,7.33496509272996));
#160587=CARTESIAN_POINT('Ctrl Pts',(0.215798015478006,4.8362090439141,7.35189581463962));
#160588=CARTESIAN_POINT('Ctrl Pts',(0.216425267876818,4.83886483076503,
7.36882671832704));
#160589=CARTESIAN_POINT('Ctrl Pts',(0.217043054200761,4.84149471143539,
7.38576205795811));
#160590=CARTESIAN_POINT('Ctrl Pts',(0.21765174428364,4.84409946429302,7.40270156517168));
#160591=CARTESIAN_POINT('Ctrl Pts',(-0.437505093897724,4.94924836941368,
7.39391729643459));
#160592=CARTESIAN_POINT('Ctrl Pts',(-0.433500006448862,4.94861077170685,
7.39414992771729));
#160593=CARTESIAN_POINT('Ctrl Pts',(-0.429494919,4.947973174,7.39438255900001));
#160594=CARTESIAN_POINT('Ctrl Pts',(-0.026681084,4.88384644,7.417779576));
#160595=CARTESIAN_POINT('Ctrl Pts',(0.37629064,4.818610636,7.397280897));
#160596=CARTESIAN_POINT('Ctrl Pts',(-0.5798133580548,4.94924836941368,7.22678200501259));
#160597=CARTESIAN_POINT('Ctrl Pts',(-0.5758987140274,4.94861077170685,7.2270918140063));
#160598=CARTESIAN_POINT('Ctrl Pts',(-0.57198407,4.947973174,7.227401623));
#160599=CARTESIAN_POINT('Ctrl Pts',(-0.178266631,4.88384644,7.25856083000001));
#160600=CARTESIAN_POINT('Ctrl Pts',(0.216505724,4.818610636,7.246766539));
#160601=CARTESIAN_POINT('Ctrl Pts',(0.459542598,0.940053947,7.48590813500001));
#160602=CARTESIAN_POINT('Ctrl Pts',(0.867851637,0.874398499000001,7.460842987));
#160603=CARTESIAN_POINT('Ctrl Pts',(1.271012251,0.809170361000001,7.391517291));
#160604=CARTESIAN_POINT('Ctrl Pts',(0.206665513,0.940053947,7.24705384));
#160605=CARTESIAN_POINT('Ctrl Pts',(0.601946558,0.874398499000001,7.235781541));
#160606=CARTESIAN_POINT('Ctrl Pts',(0.993656627,0.809170361000001,7.18158384400001));
#160607=CARTESIAN_POINT('',(0.988998381141225,0.809946052584885,7.18222682884825));
#160608=CARTESIAN_POINT('Origin',(-0.00457861362387568,0.946423635872504,
-0.198602844994274));
#160609=CARTESIAN_POINT('Ctrl Pts',(1.02255389472722,0.849330499449965,
7.42996524443304));
#160610=CARTESIAN_POINT('Ctrl Pts',(1.01691672373786,0.843074444461056,
7.38864113427304));
#160611=CARTESIAN_POINT('Ctrl Pts',(1.01129781035107,0.836669224966113,
7.34731392216213));
#160612=CARTESIAN_POINT('Ctrl Pts',(1.00011311603077,0.82355155051849,7.2647479618169));
#160613=CARTESIAN_POINT('Ctrl Pts',(0.994541071872439,0.816831759747733,
7.22346300196618));
#160614=CARTESIAN_POINT('Ctrl Pts',(0.988998378925275,0.809946053603692,
7.18222682897598));
#160615=CARTESIAN_POINT('Ctrl Pts',(0.773595447487787,0.809162772000001,
7.46052528797153));
#160616=CARTESIAN_POINT('Ctrl Pts',(1.18052789164326,0.874819703,7.41832972190814));
#160617=CARTESIAN_POINT('Ctrl Pts',(1.58045672673546,0.940053947,7.33212411374811));
#160618=CARTESIAN_POINT('Ctrl Pts',(1.59428862386671,0.942310131784066,
7.3291426155425));
#160619=CARTESIAN_POINT('Ctrl Pts',(1.60812052099803,0.944566316568131,
7.32616111733674));
#160620=CARTESIAN_POINT('Ctrl Pts',(0.984324587,0.809162772000001,7.182868863));
#160621=CARTESIAN_POINT('Ctrl Pts',(1.376112332,0.874819703,7.12917913000001));
#160622=CARTESIAN_POINT('Ctrl Pts',(1.759736143,0.940053947,7.03319477300001));
#160623=CARTESIAN_POINT('Ctrl Pts',(1.77300411626237,0.942310131784066,
7.02987506800317));
#160624=CARTESIAN_POINT('Ctrl Pts',(1.7862720895248,0.944566316568132,7.02655536300634));
#160625=CARTESIAN_POINT('Origin',(-0.0260253471876515,0.803577338089193,
-0.196947453086254));
#160626=CARTESIAN_POINT('Ctrl Pts',(2.058047714,0.940053947,7.212103688));
#160627=CARTESIAN_POINT('Ctrl Pts',(2.451422449,0.874398499000001,7.099850175));
#160628=CARTESIAN_POINT('Ctrl Pts',(2.830254416,0.809170361000001,6.945477661));
#160629=CARTESIAN_POINT('Ctrl Pts',(1.759736143,0.940053947,7.033194773));
#160630=CARTESIAN_POINT('Ctrl Pts',(2.143352525,0.874398499000001,6.937212273));
#160631=CARTESIAN_POINT('Ctrl Pts',(2.514253728,0.809170361000001,6.800075602));
#160632=CARTESIAN_POINT('',(2.50984261151385,0.809946052722277,6.80170493911415));
#160633=CARTESIAN_POINT('Origin',(-0.0471666674626342,0.94642390327405,
-0.192979181616322));
#160634=CARTESIAN_POINT('Ctrl Pts',(2.59587005248641,0.849330499397736,
7.03643792480018));
#160635=CARTESIAN_POINT('Ctrl Pts',(2.58148121593858,0.843074445580346,
6.99729178184802));
#160636=CARTESIAN_POINT('Ctrl Pts',(2.56710953902123,0.836669225428602,
6.95813867299499));
#160637=CARTESIAN_POINT('Ctrl Pts',(2.538437094516,0.823551550486689,6.87990743449499));
#160638=CARTESIAN_POINT('Ctrl Pts',(2.52412027548073,0.816831759701209,
6.84078551863939));
#160639=CARTESIAN_POINT('Ctrl Pts',(2.50984260926868,0.809946053624328,
6.80170493977546));
#160640=CARTESIAN_POINT('Ctrl Pts',(2.35930162164549,0.809162772,7.119802199134));
#160641=CARTESIAN_POINT('Ctrl Pts',(2.74764941145811,0.874819703,6.99111469553932));
#160642=CARTESIAN_POINT('Ctrl Pts',(3.1196964750598,0.940053947,6.82095164824368));
#160643=CARTESIAN_POINT('Ctrl Pts',(3.13256405620265,0.942310131795108,
6.81506640674388));
#160644=CARTESIAN_POINT('Ctrl Pts',(3.14543163734554,0.944566316590221,
6.80918116524396));
#160645=CARTESIAN_POINT('Ctrl Pts',(2.505416106,0.809162772000001,6.803336691));
#160646=CARTESIAN_POINT('Ctrl Pts',(2.876502367,0.874819703,6.66667941000001));
#160647=CARTESIAN_POINT('Ctrl Pts',(3.230523466,0.940053947,6.49047133400001));
#160648=CARTESIAN_POINT('Ctrl Pts',(3.24276760300128,0.942310131795108,
6.48437701976457));
#160649=CARTESIAN_POINT('Ctrl Pts',(3.2550117400026,0.944566316590218,6.47828270552914));
#160650=CARTESIAN_POINT('Origin',(-0.0677547966818837,0.803577340718484,
-0.186748302152657));
#160651=CARTESIAN_POINT('Ctrl Pts',(3.560320807,0.940053947,6.601069288));
#160652=CARTESIAN_POINT('Ctrl Pts',(3.920367472,0.874398499000001,6.406876261));
#160653=CARTESIAN_POINT('Ctrl Pts',(4.257157031,0.809170361000001,6.174675215));
#160654=CARTESIAN_POINT('Ctrl Pts',(3.230523466,0.940053947,6.490471334));
#160655=CARTESIAN_POINT('Ctrl Pts',(3.58453771,0.874398499000001,6.314266669));
#160656=CARTESIAN_POINT('Ctrl Pts',(3.917287119,0.809170361000001,6.100603383));
#160657=CARTESIAN_POINT('',(3.91332939130414,0.809946052687199,6.10314288710069));
#160658=CARTESIAN_POINT('Origin',(-0.0875486649536983,0.94642384785471,
-0.178327848723953));
#160659=CARTESIAN_POINT('Ctrl Pts',(4.04780621107471,0.84933049940968,6.31389458846495));
#160660=CARTESIAN_POINT('Ctrl Pts',(4.02533850999492,0.843074444501961,
6.27875682894537));
#160661=CARTESIAN_POINT('Ctrl Pts',(4.00288607621306,0.836669224983247,
6.24360858740351));
#160662=CARTESIAN_POINT('Ctrl Pts',(3.95806657572774,0.8235515505967,6.17337008284586));
#160663=CARTESIAN_POINT('Ctrl Pts',(3.93567442065259,0.816831759834135,
6.13824050874194));
#160664=CARTESIAN_POINT('Ctrl Pts',(3.91332938911934,0.809946053720409,
6.10314288828895));
#160665=CARTESIAN_POINT('Ctrl Pts',(3.83468947317847,0.809162772000001,
6.44616507150864));
#160666=CARTESIAN_POINT('Ctrl Pts',(4.18629389863323,0.874819703,6.23700291524641));
#160667=CARTESIAN_POINT('Ctrl Pts',(4.51306268385258,0.940053947,5.99083906467152));
#160668=CARTESIAN_POINT('Ctrl Pts',(4.52436427523322,0.942310131810363,
5.9823252672168));
#160669=CARTESIAN_POINT('Ctrl Pts',(4.5356658666138,0.944566316620727,5.97381146976219));
#160670=CARTESIAN_POINT('Ctrl Pts',(3.909357153,0.809162772000001,6.105688057));
#160671=CARTESIAN_POINT('Ctrl Pts',(4.242390347,0.874819703,5.89245317));
#160672=CARTESIAN_POINT('Ctrl Pts',(4.550255102,0.940053947,5.644260669));
#160673=CARTESIAN_POINT('Ctrl Pts',(4.56090288054828,0.942310131810363,
5.6356767088517));
#160674=CARTESIAN_POINT('Ctrl Pts',(4.57155065909668,0.944566316620727,
5.62709274870327));
#160675=CARTESIAN_POINT('Origin',(-0.106316028050865,0.803577351965726,
-0.167816835776771));
#160676=CARTESIAN_POINT('Ctrl Pts',(4.896117256,0.940053947,5.681376225));
#160677=CARTESIAN_POINT('Ctrl Pts',(5.206000469,0.874398499000001,5.414323933));
#160678=CARTESIAN_POINT('Ctrl Pts',(5.484999715,0.809170361000001,5.115151819));
#160679=CARTESIAN_POINT('Ctrl Pts',(4.550255102,0.940053947,5.644260669));
#160680=CARTESIAN_POINT('Ctrl Pts',(4.858113896,0.874398499000001,5.396072974));
#160681=CARTESIAN_POINT('Ctrl Pts',(5.13715251700001,0.809170361000001,
5.115873729));
#160682=CARTESIAN_POINT('',(5.13383323727461,0.809946052692845,5.11920465507359));
#160683=CARTESIAN_POINT('Origin',(-0.123836949338836,0.946423886243637,
-0.155338165371992));
#160684=CARTESIAN_POINT('Ctrl Pts',(5.31047145097424,0.849330499403383,
5.29612055860465));
#160685=CARTESIAN_POINT('Ctrl Pts',(5.28097545619076,0.843074445266492,
5.26663419557828));
#160686=CARTESIAN_POINT('Ctrl Pts',(5.25149211254345,0.836669225282618,
5.23713430764829));
#160687=CARTESIAN_POINT('Ctrl Pts',(5.19262126283321,0.823551550467761,
5.17817280592604));
#160688=CARTESIAN_POINT('Ctrl Pts',(5.16320080379069,0.81683175968613,5.14867819294392));
#160689=CARTESIAN_POINT('Ctrl Pts',(5.13383323576534,0.809946053571207,
5.11920465637222));
#160690=CARTESIAN_POINT('Ctrl Pts',(5.13077150802369,0.809162772000001,
5.47111243079908));
#160691=CARTESIAN_POINT('Ctrl Pts',(5.42919193653831,0.874819703,5.19125581030733));
#160692=CARTESIAN_POINT('Ctrl Pts',(5.69540309763417,0.940053947,4.88060150441881));
#160693=CARTESIAN_POINT('Ctrl Pts',(5.70461024979998,0.942310131934013,
4.8698572461634));
#160694=CARTESIAN_POINT('Ctrl Pts',(5.71381740196581,0.944566316868028,
4.8591129879081));
#160695=CARTESIAN_POINT('Ctrl Pts',(5.130501005,0.809162772000001,5.122544235));
#160696=CARTESIAN_POINT('Ctrl Pts',(5.40990887,0.874819703,4.842702369));
#160697=CARTESIAN_POINT('Ctrl Pts',(5.657221867,0.940053947,4.534130649));
#160698=CARTESIAN_POINT('Ctrl Pts',(5.66577540918279,0.942310131934013,
4.52345841884851));
#160699=CARTESIAN_POINT('Ctrl Pts',(5.67432895136558,0.944566316868028,
4.51278618869704));
#160700=CARTESIAN_POINT('Origin',(-0.139906057813666,0.803577330930769,
-0.141038569020607));
#160701=CARTESIAN_POINT('Ctrl Pts',(6.002976704,0.940053947,4.496028325));
#160702=CARTESIAN_POINT('Ctrl Pts',(6.24820667,0.874398499000001,4.168603835));
#160703=CARTESIAN_POINT('Ctrl Pts',(6.456369908,0.809170361,3.816449609));
#160704=CARTESIAN_POINT('Ctrl Pts',(5.657221867,0.940053947,4.534130649));
#160705=CARTESIAN_POINT('Ctrl Pts',(5.904530075,0.874398499000001,4.225564904));
#160706=CARTESIAN_POINT('Ctrl Pts',(6.116810374,0.809170361,3.891931506));
#160707=CARTESIAN_POINT('',(6.11428474814677,0.809946052705531,3.89589810483794));
#160708=CARTESIAN_POINT('Origin',(-0.154334695472245,0.946423870006678,
-0.125085081308661));
#160709=CARTESIAN_POINT('Ctrl Pts',(6.32482494729746,0.849330499396653,
4.03070581739706));
#160710=CARTESIAN_POINT('Ctrl Pts',(6.28967985561757,0.843074445169154,
4.00824959584534));
#160711=CARTESIAN_POINT('Ctrl Pts',(6.25454421281167,0.836669225267164,
3.98577744660042));
#160712=CARTESIAN_POINT('Ctrl Pts',(6.18437475129884,0.823551550514595,
3.9408499247295));
#160713=CARTESIAN_POINT('Ctrl Pts',(6.14930165691336,0.816831759845914,
3.91836940879918));
#160714=CARTESIAN_POINT('Ctrl Pts',(6.1142847471491,0.809946053730446,3.89589810607854));
#160715=CARTESIAN_POINT('Ctrl Pts',(6.18694436872949,0.809162772000001,
4.24023665216759));
#160716=CARTESIAN_POINT('Ctrl Pts',(6.41822699307587,0.874819703,3.90277135387516));
#160717=CARTESIAN_POINT('Ctrl Pts',(6.6114327918787,0.940053947,3.54215244291957));
#160718=CARTESIAN_POINT('Ctrl Pts',(6.61811498814797,0.942310131982987,
3.5296801136399));
#160719=CARTESIAN_POINT('Ctrl Pts',(6.62479718441722,0.944566316965973,
3.51720778436022));
#160720=CARTESIAN_POINT('Ctrl Pts',(6.111748332,0.809162772000001,3.899875938));
#160721=CARTESIAN_POINT('Ctrl Pts',(6.324466068,0.874819703,3.566512188));
#160722=CARTESIAN_POINT('Ctrl Pts',(6.499663225,0.940053947,3.211989719));
#160723=CARTESIAN_POINT('Ctrl Pts',(6.50572257620033,0.942310131982987,
3.19972824064686));
#160724=CARTESIAN_POINT('Ctrl Pts',(6.5117819274008,0.944566316965973,3.18746676229378));
#160725=CARTESIAN_POINT('Origin',(-0.166954220895447,0.803577360084644,
-0.107665456760575));
#160726=CARTESIAN_POINT('Ctrl Pts',(6.829143632,0.940053947,3.100451136));
#160727=CARTESIAN_POINT('Ctrl Pts',(6.998253672,0.874398499000001,2.727964456));
#160728=CARTESIAN_POINT('Ctrl Pts',(7.125847419,0.809170361,2.339294456));
#160729=CARTESIAN_POINT('Ctrl Pts',(6.499663225,0.940053947,3.211989719));
#160730=CARTESIAN_POINT('Ctrl Pts',(6.674856991,0.874398499000001,2.857474115));
#160731=CARTESIAN_POINT('Ctrl Pts',(6.810452976,0.809170361,2.486006892));
#160732=CARTESIAN_POINT('',(6.80883909887103,0.809946052703242,2.49042368839839));
#160733=CARTESIAN_POINT('Origin',(-0.177616241857739,0.946423877604977,
-0.0889833580990079));
#160734=CARTESIAN_POINT('Ctrl Pts',(7.04343665837362,0.849330499394402,
2.57681975190768));
#160735=CARTESIAN_POINT('Ctrl Pts',(7.00428581770227,0.843074445515644,
2.56244370102973));
#160736=CARTESIAN_POINT('Ctrl Pts',(6.96514077770283,0.83666922543599,2.54805006240474));
#160737=CARTESIAN_POINT('Ctrl Pts',(6.88695374929916,0.823551550542199,
2.51925728103009));
#160738=CARTESIAN_POINT('Ctrl Pts',(6.84786799755061,0.816831759784013,
2.50484202561442));
#160739=CARTESIAN_POINT('Ctrl Pts',(6.80883909801412,0.809946053662277,
2.49042369025996));
#160740=CARTESIAN_POINT('Ctrl Pts',(6.95382258706006,0.809162772,2.81109212166397));
#160741=CARTESIAN_POINT('Ctrl Pts',(7.10715288826951,0.874819703,2.4317976459104));
#160742=CARTESIAN_POINT('Ctrl Pts',(7.21831923755852,0.940053947,2.03807626899816));
#160743=CARTESIAN_POINT('Ctrl Pts',(7.22216402529775,0.942310131745766,
2.02445906260161));
#160744=CARTESIAN_POINT('Ctrl Pts',(7.22600881303697,0.944566316491536,
2.01084185620499));
#160745=CARTESIAN_POINT('Ctrl Pts',(6.807217099,0.809162772000001,2.494853776));
#160746=CARTESIAN_POINT('Ctrl Pts',(6.94329826,0.874819703,2.12355586));
#160747=CARTESIAN_POINT('Ctrl Pts',(7.038187555,0.940053947,1.73965972));
#160748=CARTESIAN_POINT('Ctrl Pts',(7.04146938624059,0.942310131745766,
1.72638232822052));
#160749=CARTESIAN_POINT('Ctrl Pts',(7.04475121748121,0.944566316491536,
1.71310493644103));
#160750=CARTESIAN_POINT('Origin',(-0.186195806700906,0.803577371035635,
-0.0692580764843428));
#160751=CARTESIAN_POINT('Ctrl Pts',(7.335987395,0.940053947,1.559900299));
#160752=CARTESIAN_POINT('Ctrl Pts',(7.42107011,0.874398499000001,1.15976849));
#160753=CARTESIAN_POINT('Ctrl Pts',(7.462128226,0.809170361,0.752756495));
#160754=CARTESIAN_POINT('Ctrl Pts',(7.038187555,0.940053947,1.73965972));
#160755=CARTESIAN_POINT('Ctrl Pts',(7.133075012,0.874398499000001,1.355771012));
#160756=CARTESIAN_POINT('Ctrl Pts',(7.185646366,0.809170361,0.963839358));
#160757=CARTESIAN_POINT('',(7.18501970015274,0.809946052684096,0.968499827292238));
#160758=CARTESIAN_POINT('Origin',(-0.192592153795034,0.946423760555048,
-0.0487206444150247));
#160759=CARTESIAN_POINT('Ctrl Pts',(7.43270510014592,0.849330499432997,
1.00244445911311));
#160760=CARTESIAN_POINT('Ctrl Pts',(7.39137915765184,0.843074445435521,
0.996820785600723));
#160761=CARTESIAN_POINT('Ctrl Pts',(7.35005510021506,0.836669225363939,
0.991178688685446));
#160762=CARTESIAN_POINT('Ctrl Pts',(7.26750644432747,0.823551550483965,
0.979866966386957));
#160763=CARTESIAN_POINT('Ctrl Pts',(7.2262356410549,0.816831759582578,0.974191012744954));
#160764=CARTESIAN_POINT('Ctrl Pts',(7.18501969968291,0.809946053480066,
0.968499829781929));
#160765=CARTESIAN_POINT('Ctrl Pts',(7.39554779057258,0.809162772,1.25050404734931));
#160766=CARTESIAN_POINT('Ctrl Pts',(7.46375621382019,0.874819703,0.84711578386319));
#160767=CARTESIAN_POINT('Ctrl Pts',(7.48768509771001,0.940053947,0.438701914431586));
#160768=CARTESIAN_POINT('Ctrl Pts',(7.48851269958806,0.942310131747133,
0.424576555015612));
#160769=CARTESIAN_POINT('Ctrl Pts',(7.48934030146606,0.94456631649427,0.410451195599633));
#160770=CARTESIAN_POINT('Ctrl Pts',(7.184387961,0.809162772000001,0.973175025));
#160771=CARTESIAN_POINT('Ctrl Pts',(7.237469544,0.874819703,0.581304421));
#160772=CARTESIAN_POINT('Ctrl Pts',(7.24761405700001,0.940053947,0.185985165));
#160773=CARTESIAN_POINT('Ctrl Pts',(7.24796491406668,0.942310131747134,
0.17231269451601));
#160774=CARTESIAN_POINT('Ctrl Pts',(7.24831577113348,0.944566316494269,
0.158640224032027));
#160775=CARTESIAN_POINT('Origin',(-0.196731118555223,0.803577356082231,
-0.0276122899099263));
#160776=CARTESIAN_POINT('Ctrl Pts',(7.49980854,0.940053947,-0.053589743));
#160777=CARTESIAN_POINT('Ctrl Pts',(7.496885558,0.874398499000001,-0.462656961));
#160778=CARTESIAN_POINT('Ctrl Pts',(7.44948821,0.809170361,-0.868979523));
#160779=CARTESIAN_POINT('Ctrl Pts',(7.247614057,0.940053947,0.185985165));
#160780=CARTESIAN_POINT('Ctrl Pts',(7.257758374,0.874398499000001,-0.209326436));
#160781=CARTESIAN_POINT('Ctrl Pts',(7.224846918,0.809170361,-0.603396233));
#160782=CARTESIAN_POINT('',(7.22523676689643,0.809946052675541,-0.598710008135555));
#160783=CARTESIAN_POINT('Origin',(-0.198563384833296,0.946423902094758,
-0.00617996603265752));
#160784=CARTESIAN_POINT('Ctrl Pts',(7.47442851183213,0.849330499401343,
-0.61880402232886));
#160785=CARTESIAN_POINT('Ctrl Pts',(7.43285981681545,0.843074444412867,
-0.615412360954006));
#160786=CARTESIAN_POINT('Ctrl Pts',(7.39128901257921,0.836669224881622,
-0.612039098317023));
#160787=CARTESIAN_POINT('Ctrl Pts',(7.30823861543218,0.823551550480405,
-0.60534083824266));
#160788=CARTESIAN_POINT('Ctrl Pts',(7.26671253872467,0.816831759653862,
-0.602012088542576));
#160789=CARTESIAN_POINT('Ctrl Pts',(7.22523676694034,0.809946053561054,
-0.59871000573749));
#160790=CARTESIAN_POINT('Ctrl Pts',(7.49146539823555,0.809162772000001,
-0.368556206897238));
#160791=CARTESIAN_POINT('Ctrl Pts',(7.47136259378149,0.874819703,-0.777176271136419));
#160792=CARTESIAN_POINT('Ctrl Pts',(7.40693512425472,0.940053947,-1.18118565372789));
#160793=CARTESIAN_POINT('Ctrl Pts',(7.4047068423435,0.942310131931147,-1.19515868116184));
#160794=CARTESIAN_POINT('Ctrl Pts',(7.40247856043215,0.944566316862295,
-1.20913170859578));
#160795=CARTESIAN_POINT('Ctrl Pts',(7.225624826,0.809162772000001,-0.594008309));
#160796=CARTESIAN_POINT('Ctrl Pts',(7.193224795,0.874819703,-0.988128168));
#160797=CARTESIAN_POINT('Ctrl Pts',(7.118150181,0.940053947,-1.376385849));
#160798=CARTESIAN_POINT('Ctrl Pts',(7.11555365803243,0.942310131931147,
-1.38981408968405));
#160799=CARTESIAN_POINT('Ctrl Pts',(7.11295713506485,0.944566316862295,
-1.40324233036812));
#160800=CARTESIAN_POINT('Origin',(-0.198067613676669,0.803577356916781,
0.0153246665703818));
#160801=CARTESIAN_POINT('Ctrl Pts',(7.312946974,0.940053947,-1.664573988));
#160802=CARTESIAN_POINT('Ctrl Pts',(7.222154969,0.874398499000001,-2.063449087));
#160803=CARTESIAN_POINT('Ctrl Pts',(7.088518405,0.809170361,-2.450083024));
#160804=CARTESIAN_POINT('Ctrl Pts',(7.118150181,0.940053947,-1.376385849));
#160805=CARTESIAN_POINT('Ctrl Pts',(7.04307702,0.874398499000001,-1.764636013));
#160806=CARTESIAN_POINT('Ctrl Pts',(6.926221658,0.809170361,-2.142417687));
#160807=CARTESIAN_POINT('',(6.92760979279974,0.809946052722275,-2.13792482936519));
#160808=CARTESIAN_POINT('Origin',(-0.19524961185327,0.946423874648229,0.036649780107621));
#160809=CARTESIAN_POINT('Ctrl Pts',(7.16665595397255,0.849330499387892,
-2.2111179158326));
#160810=CARTESIAN_POINT('Ctrl Pts',(7.12678822298043,0.843074445056534,
-2.19886951017339));
#160811=CARTESIAN_POINT('Ctrl Pts',(7.08691447053379,0.836669225196569,
-2.18663861775412));
#160812=CARTESIAN_POINT('Ctrl Pts',(7.00724567148069,0.823551550493151,
-2.16224357833837));
#160813=CARTESIAN_POINT('Ctrl Pts',(6.96740603447509,0.816831759727534,
-2.15006577416038));
#160814=CARTESIAN_POINT('Ctrl Pts',(6.92760979323707,0.809946053613321,
-2.13792482742635));
#160815=CARTESIAN_POINT('Ctrl Pts',(7.23709041010625,0.809162772000001,
-1.97038318210479));
#160816=CARTESIAN_POINT('Ctrl Pts',(7.1296163636436,0.874819703,-2.36512842791326));
#160817=CARTESIAN_POINT('Ctrl Pts',(6.97984509784344,0.940053947,-2.74584229453887));
#160818=CARTESIAN_POINT('Ctrl Pts',(6.97466512443654,0.942310131771728,
-2.75900962469549));
#160819=CARTESIAN_POINT('Ctrl Pts',(6.96948515102947,0.944566316543458,
-2.77217695485211));
#160820=CARTESIAN_POINT('Ctrl Pts',(6.928999505,0.809162772000001,-2.133416475));
#160821=CARTESIAN_POINT('Ctrl Pts',(6.81263284900001,0.874819703,-2.511356981));
#160822=CARTESIAN_POINT('Ctrl Pts',(6.655849513,0.940053947,-2.874398591));
#160823=CARTESIAN_POINT('Ctrl Pts',(6.65042702086314,0.942310131771728,
-2.88695471032876));
#160824=CARTESIAN_POINT('Ctrl Pts',(6.64500452872626,0.944566316543458,
-2.89951082965752));
#160825=CARTESIAN_POINT('Origin',(-0.190142576295623,0.803577351896187,
0.0575450801711413));
#160826=CARTESIAN_POINT('Ctrl Pts',(6.784140134,0.940053947,-3.197724603));
#160827=CARTESIAN_POINT('Ctrl Pts',(6.609724441,0.874398499000001,-3.567756627));
#160828=CARTESIAN_POINT('Ctrl Pts',(6.396097357,0.809170361,-3.916623367));
#160829=CARTESIAN_POINT('Ctrl Pts',(6.655849513,0.940053947,-2.874398591));
#160830=CARTESIAN_POINT('Ctrl Pts',(6.499069213,0.874398499000001,-3.237433171));
#160831=CARTESIAN_POINT('Ctrl Pts',(6.303733971,0.809170361,-3.581262071));
#160832=CARTESIAN_POINT('',(6.30605548324046,0.809946052678392,-3.5771726618393));
#160833=CARTESIAN_POINT('Origin',(-0.1828060003259,0.946423907519971,0.0777657385988639));
#160834=CARTESIAN_POINT('Ctrl Pts',(6.52377852850538,0.849330499411468,
-3.70004239318147));
#160835=CARTESIAN_POINT('Ctrl Pts',(6.48747592982481,0.843074445384863,
-3.67950996577842));
#160836=CARTESIAN_POINT('Ctrl Pts',(6.45116368279414,0.836669225346678,
-3.65899334610276));
#160837=CARTESIAN_POINT('Ctrl Pts',(6.37860170748226,0.823551550490179,
-3.61804221184952));
#160838=CARTESIAN_POINT('Ctrl Pts',(6.34231136673367,0.816831759681685,
-3.59758477350974));
#160839=CARTESIAN_POINT('Ctrl Pts',(6.30605548418455,0.809946053571847,
-3.57717265986101));
#160840=CARTESIAN_POINT('Ctrl Pts',(6.64431711846076,0.809162772000001,
-3.48007722958917));
#160841=CARTESIAN_POINT('Ctrl Pts',(6.45449719567497,0.874819703,-3.8424898080853));
#160842=CARTESIAN_POINT('Ctrl Pts',(6.22638527100719,0.940053947,-4.18210640003388));
#160843=CARTESIAN_POINT('Ctrl Pts',(6.21849581559411,0.942310131810126,
-4.1938523443269));
#160844=CARTESIAN_POINT('Ctrl Pts',(6.21060636018102,0.944566316620252,
-4.20559828861992));
#160845=CARTESIAN_POINT('Ctrl Pts',(6.308381869,0.809162772000001,-3.573068457));
#160846=CARTESIAN_POINT('Ctrl Pts',(6.113489763,0.874819703,-3.917157533));
#160847=CARTESIAN_POINT('Ctrl Pts',(5.88232872,0.940053947,-4.238007649));
#160848=CARTESIAN_POINT('Ctrl Pts',(5.87433380809593,0.942310131810126,
-4.24910453789851));
#160849=CARTESIAN_POINT('Ctrl Pts',(5.86633889619174,0.944566316620252,
-4.26020142679696));
#160850=CARTESIAN_POINT('Origin',(-0.173326571395247,0.80357735796664,0.0970746776577225));
#160851=CARTESIAN_POINT('Ctrl Pts',(5.938114442,0.940053947,-4.58135317));
#160852=CARTESIAN_POINT('Ctrl Pts',(5.688230544,0.874398499000001,-4.905239832));
#160853=CARTESIAN_POINT('Ctrl Pts',(5.404601906,0.809170361,-5.200026753));
#160854=CARTESIAN_POINT('Ctrl Pts',(5.88232872,0.940053947,-4.238007649));
#160855=CARTESIAN_POINT('Ctrl Pts',(5.651172152,0.874398499000001,-4.55885155200001));
#160856=CARTESIAN_POINT('Ctrl Pts',(5.38649069,0.809170361,-4.85265062));
#160857=CARTESIAN_POINT('',(5.38963702945792,0.809946052688611,-4.84915587636754));
#160858=CARTESIAN_POINT('Origin',(-0.161814908904617,0.946423888559224,
0.115245624273202));
#160859=CARTESIAN_POINT('Ctrl Pts',(5.57585646967174,0.849330499367115,
-5.01595700001293));
#160860=CARTESIAN_POINT('Ctrl Pts',(5.54481647208769,0.84307444565754,-4.98810062512837));
#160861=CARTESIAN_POINT('Ctrl Pts',(5.51376365132296,0.836669225498839,
-4.96025761229804));
#160862=CARTESIAN_POINT('Ctrl Pts',(5.45170141738891,0.823551550511566,
-4.90466521235823));
#160863=CARTESIAN_POINT('Ctrl Pts',(5.42065726996587,0.816831759876436,
-4.87688470765218));
#160864=CARTESIAN_POINT('Ctrl Pts',(5.38963703080557,0.809946053748422,
-4.84915587459674));
#160865=CARTESIAN_POINT('Ctrl Pts',(5.74086294257922,0.809162772000001,
-4.82704673403754));
#160866=CARTESIAN_POINT('Ctrl Pts',(5.47757291233011,0.874819703,-5.14018063457471));
#160867=CARTESIAN_POINT('Ctrl Pts',(5.18178659015694,0.940053947,-5.42281985940062));
#160868=CARTESIAN_POINT('Ctrl Pts',(5.1715565548202,0.942310131857983,-5.43259519057982));
#160869=CARTESIAN_POINT('Ctrl Pts',(5.16132651948343,0.944566316715966,
-5.44237052175898));
#160870=CARTESIAN_POINT('Ctrl Pts',(5.392791307,0.809162772000001,-4.845647729));
#160871=CARTESIAN_POINT('Ctrl Pts',(5.128486691,0.874819703,-5.139796152));
#160872=CARTESIAN_POINT('Ctrl Pts',(4.833756773,0.940053947,-5.403452179));
#160873=CARTESIAN_POINT('Ctrl Pts',(4.8235632743494,0.942310131857983,-5.41257095925034));
#160874=CARTESIAN_POINT('Ctrl Pts',(4.81336977569886,0.944566316715967,
-5.4216897395007));
#160875=CARTESIAN_POINT('Origin',(-0.148406033224281,0.803577342228433,
0.132065168002498));
#160876=CARTESIAN_POINT('Ctrl Pts',(4.814429119,0.940053947,-5.750762755));
#160877=CARTESIAN_POINT('Ctrl Pts',(4.500761309,0.874398499000001,-6.013359475));
#160878=CARTESIAN_POINT('Ctrl Pts',(4.160393277,0.809170361,-6.240282668));
#160879=CARTESIAN_POINT('Ctrl Pts',(4.833756773,0.940053947,-5.403452179));
#160880=CARTESIAN_POINT('Ctrl Pts',(4.539032563,0.874398499000001,-5.667103101));
#160881=CARTESIAN_POINT('Ctrl Pts',(4.217381091,0.809170361,-5.89713462));
#160882=CARTESIAN_POINT('',(4.22120513711784,0.809946052707974,-5.89439795128935));
#160883=CARTESIAN_POINT('Origin',(-0.133257209627604,0.946423898125065,
0.147336455417874));
#160884=CARTESIAN_POINT('Ctrl Pts',(4.3672135600113,0.849330499383033,-6.09733103232013));
#160885=CARTESIAN_POINT('Ctrl Pts',(4.34288755318523,0.843074444573075,
-6.06345323611053));
#160886=CARTESIAN_POINT('Ctrl Pts',(4.3185461571543,0.836669224993378,-6.0295857421921));
#160887=CARTESIAN_POINT('Ctrl Pts',(4.26988562827292,0.8235515505247,-5.96195151866442));
#160888=CARTESIAN_POINT('Ctrl Pts',(4.24553926283837,0.816831759838917,
-5.92814693247654));
#160889=CARTESIAN_POINT('Ctrl Pts',(4.22120513897645,0.809946053714662,
-5.89439794974384));
#160890=CARTESIAN_POINT('Ctrl Pts',(4.56897239579151,0.809162772,-5.94830889693425));
#160891=CARTESIAN_POINT('Ctrl Pts',(4.2445234080415,0.874819703,-6.19752232790785));
#160892=CARTESIAN_POINT('Ctrl Pts',(3.89489332643903,0.940053947,-6.40996828922183));
#160893=CARTESIAN_POINT('Ctrl Pts',(3.88280105600422,0.942310131926778,
-6.41731592362796));
#160894=CARTESIAN_POINT('Ctrl Pts',(3.87070878556934,0.944566316853557,
-6.42466355803407));
#160895=CARTESIAN_POINT('Ctrl Pts',(4.225039818,0.809162772000001,-5.891649899));
#160896=CARTESIAN_POINT('Ctrl Pts',(3.903681281,0.874819703,-6.122103616));
#160897=CARTESIAN_POINT('Ctrl Pts',(3.559163733,0.940053947,-6.316237292));
#160898=CARTESIAN_POINT('Ctrl Pts',(3.54724828413225,0.942310131926778,
-6.32295157956916));
#160899=CARTESIAN_POINT('Ctrl Pts',(3.53533283526452,0.944566316853556,
-6.32966586713822));
#160900=CARTESIAN_POINT('Origin',(-0.116546242053256,0.803577346880212,
0.160880395793309));
#160901=CARTESIAN_POINT('Ctrl Pts',(3.465626441,0.940053947,-6.651273064));
#160902=CARTESIAN_POINT('Ctrl Pts',(3.102841477,0.874398499000001,-6.840301112));
#160903=CARTESIAN_POINT('Ctrl Pts',(2.721649282,0.809170361,-6.988749902));
#160904=CARTESIAN_POINT('Ctrl Pts',(3.559163733,0.940053947,-6.31623729200001));
#160905=CARTESIAN_POINT('Ctrl Pts',(3.214652856,0.874398499000001,-6.51036720800001));
#160906=CARTESIAN_POINT('Ctrl Pts',(2.85107144,0.809170361,-6.66587516));
#160907=CARTESIAN_POINT('',(2.85539438458225,0.809946052650979,-6.66402452877942));
#160908=CARTESIAN_POINT('Origin',(-0.0984686780031424,0.946423832486099,
0.172538085307491));
#160909=CARTESIAN_POINT('Ctrl Pts',(2.9543645978865,0.84933049941643,-6.89360064286475));
#160910=CARTESIAN_POINT('Ctrl Pts',(2.93789004392451,0.843074444415432,
-6.85528551721847));
#160911=CARTESIAN_POINT('Ctrl Pts',(2.92139824653569,0.836669224896916,
-6.81697714634658));
#160912=CARTESIAN_POINT('Ctrl Pts',(2.88841473288365,0.823551550476378,
-6.74046359851006));
#160913=CARTESIAN_POINT('Ctrl Pts',(2.8719045584201,0.816831759630593,-6.70221559503671));
#160914=CARTESIAN_POINT('Ctrl Pts',(2.85539438671172,0.809946053538579,
-6.66402452769881));
#160915=CARTESIAN_POINT('Ctrl Pts',(3.18344177798828,0.809162772,-6.79143474774354));
#160916=CARTESIAN_POINT('Ctrl Pts',(2.81300470637386,0.874819703,-6.9650747653572));
#160917=CARTESIAN_POINT('Ctrl Pts',(2.42587918038149,0.940053947,-7.09739372560097));
#160918=CARTESIAN_POINT('Ctrl Pts',(2.41249009638585,0.94231013191591,-7.10197009567725));
#160919=CARTESIAN_POINT('Ctrl Pts',(2.39910101239022,0.944566316831819,
-7.10654646575353));
#160920=CARTESIAN_POINT('Ctrl Pts',(2.859730162,0.809162772000001,-6.662165068));
#160921=CARTESIAN_POINT('Ctrl Pts',(2.496344072,0.874819703,-6.818148319));
#160922=CARTESIAN_POINT('Ctrl Pts',(2.118148151,0.940053947,-6.933682168));
#160923=CARTESIAN_POINT('Ctrl Pts',(2.10506790541275,0.94231013191591,-6.93767800992912));
#160924=CARTESIAN_POINT('Ctrl Pts',(2.09198765982549,0.94456631683182,-6.94167385185837));
#160925=CARTESIAN_POINT('Origin',(-0.0792369432847576,0.803577312784041,
0.182173122882493));
#160926=CARTESIAN_POINT('Ctrl Pts',(1.954774922,0.940053947,-7.240777238));
#160927=CARTESIAN_POINT('Ctrl Pts',(1.559836226,0.874398499000001,-7.347397871));
#160928=CARTESIAN_POINT('Ctrl Pts',(1.155643991,0.809170361,-7.410430957));
#160929=CARTESIAN_POINT('Ctrl Pts',(2.118148151,0.940053947,-6.933682168));
#160930=CARTESIAN_POINT('Ctrl Pts',(1.739959553,0.874398499000001,-7.04921378));
#160931=CARTESIAN_POINT('Ctrl Pts',(1.351448856,0.809170361,-7.122926785));
#160932=CARTESIAN_POINT('',(1.35606856387977,0.809946052736701,-7.12204872627898));
#160933=CARTESIAN_POINT('Origin',(-0.0590759568677302,0.946423831175772,
0.189672134415341));
#160934=CARTESIAN_POINT('Ctrl Pts',(1.40337283024097,0.849330499423155,
-7.36753314860582));
#160935=CARTESIAN_POINT('Ctrl Pts',(1.39552006198321,0.843074444748845,
-7.32657226924519));
#160936=CARTESIAN_POINT('Ctrl Pts',(1.38764900074009,0.836669225060746,
-7.28561427662802));
#160937=CARTESIAN_POINT('Ctrl Pts',(1.37188477410703,0.823551550508327,
-7.20379909165716));
#160938=CARTESIAN_POINT('Ctrl Pts',(1.36398278850603,0.81683175972654,-7.16289610614498));
#160939=CARTESIAN_POINT('Ctrl Pts',(1.35606856587717,0.809946053612075,
-7.12204872574442));
#160940=CARTESIAN_POINT('Ctrl Pts',(1.64905696119522,0.809162772000001,
-7.31700065792982));
#160941=CARTESIAN_POINT('Ctrl Pts',(1.24995303106729,0.874819703,-7.40694804797127));
#160942=CARTESIAN_POINT('Ctrl Pts',(0.843433619571964,0.940053947,-7.45295291915762));
#160943=CARTESIAN_POINT('Ctrl Pts',(0.829373781529389,0.94231013177134,
-7.45454403884281));
#160944=CARTESIAN_POINT('Ctrl Pts',(0.815313943486812,0.944566316542682,
-7.45613515852813));
#160945=CARTESIAN_POINT('Ctrl Pts',(1.360702703,0.809162772000001,-7.12116480300001));
#160946=CARTESIAN_POINT('Ctrl Pts',(0.97228059,0.874819703,-7.19538398400001));
#160947=CARTESIAN_POINT('Ctrl Pts',(0.578090317,0.940053947,-7.226915773));
#160948=CARTESIAN_POINT('Ctrl Pts',(0.564456893257817,0.94231013177134,
-7.22800632817153));
#160949=CARTESIAN_POINT('Ctrl Pts',(0.550823469515642,0.944566316542682,
-7.22909688334309));
#160950=CARTESIAN_POINT('Origin',(-0.0382226035147889,0.803577363718229,
0.194947726870536));
#160951=CARTESIAN_POINT('Ctrl Pts',(0.3525203,0.940053947,-7.491710715));
#160952=CARTESIAN_POINT('Ctrl Pts',(-0.056105233,0.874398499000001,-7.510938472));
#160953=CARTESIAN_POINT('Ctrl Pts',(-0.464397928,0.809170361,-7.485608497));
#160954=CARTESIAN_POINT('Ctrl Pts',(0.578090316999999,0.940053947,-7.226915773));
#160955=CARTESIAN_POINT('Ctrl Pts',(0.183907677,0.874398499000001,-7.258446951));
#160956=CARTESIAN_POINT('Ctrl Pts',(-0.211365974,0.809170361,-7.246918271));
#160957=CARTESIAN_POINT('',(-0.206665515349642,0.809946052703829,-7.24705384080755));
#160958=CARTESIAN_POINT('Origin',(-0.0169208965170819,0.946423889145898,
0.197937327803924));
#160959=CARTESIAN_POINT('Ctrl Pts',(-0.213239090823349,0.84933049680011,
-7.49696797599282));
#160960=CARTESIAN_POINT('Ctrl Pts',(-0.212102887475241,0.843074442824839,
-7.45527663117971));
#160961=CARTESIAN_POINT('Ctrl Pts',(-0.210985170255643,0.83666922533313,
-7.41358418244774));
#160962=CARTESIAN_POINT('Ctrl Pts',(-0.208792991489413,0.823551550440252,
-7.33029294605962));
#160963=CARTESIAN_POINT('Ctrl Pts',(-0.207717300195503,0.81683175959965,
-7.28864755583171));
#160964=CARTESIAN_POINT('Ctrl Pts',(-0.206665513343767,0.809946053541909,
-7.24705384071953));
#160965=CARTESIAN_POINT('Ctrl Pts',(0.0375640730725487,0.809162772000001,
-7.50043175005473));
#160966=CARTESIAN_POINT('Ctrl Pts',(-0.371545059360011,0.874819703,-7.50248067266858));
#160967=CARTESIAN_POINT('Ctrl Pts',(-0.778449959964432,0.940053947,-7.46002031823397));
#160968=CARTESIAN_POINT('Ctrl Pts',(-0.792523130628518,0.942310131793034,
-7.45855178882197));
#160969=CARTESIAN_POINT('Ctrl Pts',(-0.806596301292605,0.944566316586069,
-7.45708325941005));
#160970=CARTESIAN_POINT('Ctrl Pts',(-0.201949703,0.809162772000001,-7.247186786));
#160971=CARTESIAN_POINT('Ctrl Pts',(-0.597245653,0.874819703,-7.236171492));
#160972=CARTESIAN_POINT('Ctrl Pts',(-0.988998379000001,0.940053947,-7.182226828));
#160973=CARTESIAN_POINT('Ctrl Pts',(-1.0025474981257,0.942310131793034,
-7.18036110344923));
#160974=CARTESIAN_POINT('Ctrl Pts',(-1.0160966172514,0.944566316586069,
-7.17849537889843));
#160975=CARTESIAN_POINT('Origin',(0.00457900919291515,0.803577353390686,
0.198606638624294));
#160976=CARTESIAN_POINT('Ctrl Pts',(-1.266217779,0.940053947,-7.392340126));
#160977=CARTESIAN_POINT('Ctrl Pts',(-1.669423273,0.874398499000001,-7.323275938));
#160978=CARTESIAN_POINT('Ctrl Pts',(-2.062725117,0.809170361,-7.210767303));
#160979=CARTESIAN_POINT('Ctrl Pts',(-0.988998379000001,0.940053947,-7.182226828));
#160980=CARTESIAN_POINT('Ctrl Pts',(-1.380743519,0.874398499000001,-7.128283209));
#160981=CARTESIAN_POINT('Ctrl Pts',(-1.764297565,0.809170361,-7.032051913));
#160982=CARTESIAN_POINT('',(-1.75973614513862,0.809946052657848,-7.03319477389625));
#160983=CARTESIAN_POINT('Origin',(0.0260254480477046,0.946423936792007,
0.196947624644461));
#160984=CARTESIAN_POINT('Ctrl Pts',(-1.81988018914672,0.849330499393605,
-7.27585294610869));
#160985=CARTESIAN_POINT('Ctrl Pts',(-1.80980814109725,0.843074444356029,
-7.23538056476307));
#160986=CARTESIAN_POINT('Ctrl Pts',(-1.79975390841227,0.836669224901153,
-7.19490312626225));
#160987=CARTESIAN_POINT('Ctrl Pts',(-1.77970782869062,0.823551550531388,
-7.11403044988765));
#160988=CARTESIAN_POINT('Ctrl Pts',(-1.76970475880954,0.816831759807746,
-7.07358994854385));
#160989=CARTESIAN_POINT('Ctrl Pts',(-1.75973614281132,0.809946053652001,
-7.03319477430111));
#160990=CARTESIAN_POINT('Ctrl Pts',(-1.57568526882621,0.809162772000001,
-7.33315098852158));
#160991=CARTESIAN_POINT('Ctrl Pts',(-1.97567011476372,0.874819703,-7.24720563828579));
#160992=CARTESIAN_POINT('Ctrl Pts',(-2.36393408428844,0.940053947,-7.11826545847411));
#160993=CARTESIAN_POINT('Ctrl Pts',(-2.37736254142904,0.942310131756794,
-7.11380594686806));
#160994=CARTESIAN_POINT('Ctrl Pts',(-2.39079099856963,0.944566316513591,
-7.10934643526207));
#160995=CARTESIAN_POINT('Ctrl Pts',(-1.755159165,0.809162772000001,-7.03433837));
#160996=CARTESIAN_POINT('Ctrl Pts',(-2.138845352,0.874819703,-6.938603662));
#160997=CARTESIAN_POINT('Ctrl Pts',(-2.509842609,0.940053947,-6.801704939));
#160998=CARTESIAN_POINT('Ctrl Pts',(-2.52267388142274,0.942310131756794,
-6.79697017404961));
#160999=CARTESIAN_POINT('Ctrl Pts',(-2.53550515384552,0.944566316513591,
-6.79223540909921));
#161000=CARTESIAN_POINT('Origin',(0.047166591713389,0.803577351524094,0.192979168030507));
#161001=CARTESIAN_POINT('Ctrl Pts',(-2.825748922,0.940053947,-6.947311928));
#161002=CARTESIAN_POINT('Ctrl Pts',(-3.204680937,0.874398499000001,-6.79318516));
#161003=CARTESIAN_POINT('Ctrl Pts',(-3.564601571,0.809170361,-6.598758644));
#161004=CARTESIAN_POINT('Ctrl Pts',(-2.509842609,0.940053947,-6.801704939));
#161005=CARTESIAN_POINT('Ctrl Pts',(-2.880832682,0.874398499000001,-6.66480886600001));
#161006=CARTESIAN_POINT('Ctrl Pts',(-3.234732564,0.809170361,-6.488374622));
#161007=CARTESIAN_POINT('',(-3.23052346880049,0.809946052708776,-6.49047133375201));
#161008=CARTESIAN_POINT('Origin',(0.0677547936442369,0.946423863393157,
0.18674810450875));
#161009=CARTESIAN_POINT('Ctrl Pts',(-3.34142571289718,0.849330499364931,
-6.71452710196662));
#161010=CARTESIAN_POINT('Ctrl Pts',(-3.32288878222837,0.843074445722822,
-6.6771661432789));
#161011=CARTESIAN_POINT('Ctrl Pts',(-3.30436815677359,0.836669225509062,
-6.63979640280475));
#161012=CARTESIAN_POINT('Ctrl Pts',(-3.2674055064749,0.823551550480611,
-6.56512379521472));
#161013=CARTESIAN_POINT('Ctrl Pts',(-3.24894279036105,0.816831759752248,
-6.52777913445038));
#161014=CARTESIAN_POINT('Ctrl Pts',(-3.23052346667513,0.809946053623409,
-6.49047133463251));
#161015=CARTESIAN_POINT('Ctrl Pts',(-3.11525731968697,0.809162772000001,
-6.82298023806838));
#161016=CARTESIAN_POINT('Ctrl Pts',(-3.48741503215244,0.874819703,-6.65305932401257));
#161017=CARTESIAN_POINT('Ctrl Pts',(-3.83888327807438,0.940053947,-6.4436684167713));
#161018=CARTESIAN_POINT('Ctrl Pts',(-3.85103912327679,0.942310131964536,
-6.43642644403335));
#161019=CARTESIAN_POINT('Ctrl Pts',(-3.86319496847921,0.94456631692907,
-6.4291844712954));
#161020=CARTESIAN_POINT('Ctrl Pts',(-3.226299335,0.809162772000001,-6.49257211000001));
#161021=CARTESIAN_POINT('Ctrl Pts',(-3.58043502,0.874819703,-6.316594438));
#161022=CARTESIAN_POINT('Ctrl Pts',(-3.913329389,0.940053947,-6.103142887));
#161023=CARTESIAN_POINT('Ctrl Pts',(-3.92484283997394,0.942310131964536,
-6.09576047324775));
#161024=CARTESIAN_POINT('Ctrl Pts',(-3.93635629094792,0.944566316929071,
-6.08837805949553));
#161025=CARTESIAN_POINT('Origin',(0.0875487564160587,0.803577348034149,
0.178328165777322));
#161026=CARTESIAN_POINT('Ctrl Pts',(-4.253151186,0.940053947,-6.177435146));
#161027=CARTESIAN_POINT('Ctrl Pts',(-4.590091282,0.874398499000001,-5.945452595));
#161028=CARTESIAN_POINT('Ctrl Pts',(-4.899801218,0.809170361,-5.678199365));
#161029=CARTESIAN_POINT('Ctrl Pts',(-3.913329389,0.940053947,-6.10314288700001));
#161030=CARTESIAN_POINT('Ctrl Pts',(-4.246217311,0.874398499000001,-5.889695469));
#161031=CARTESIAN_POINT('Ctrl Pts',(-4.553915063,0.809170361,-5.641308146));
#161032=CARTESIAN_POINT('',(-4.55025510443955,0.809946052699697,-5.64426066870771));
#161033=CARTESIAN_POINT('Origin',(0.106316175334812,0.946423914870134,0.16781693033121));
#161034=CARTESIAN_POINT('Ctrl Pts',(-4.70672988353109,0.849330499400675,
-5.83923743366635));
#161035=CARTESIAN_POINT('Ctrl Pts',(-4.68059483219139,0.843074445265959,
-5.80673484298954));
#161036=CARTESIAN_POINT('Ctrl Pts',(-4.65447382012871,0.836669225283608,
-5.77422017452406));
#161037=CARTESIAN_POINT('Ctrl Pts',(-4.60232293361958,0.82355155046795,
-5.70923924925526));
#161038=CARTESIAN_POINT('Ctrl Pts',(-4.576263867122,0.81683175966244,-5.67673662375688));
#161039=CARTESIAN_POINT('Ctrl Pts',(-4.55025510290105,0.809946053539602,
-5.64426066976175));
#161040=CARTESIAN_POINT('Ctrl Pts',(-4.50916339980242,0.809162772,-5.99377451447543));
#161041=CARTESIAN_POINT('Ctrl Pts',(-4.83609229828455,0.874819703,-5.74782334932259));
#161042=CARTESIAN_POINT('Ctrl Pts',(-5.13433055676909,0.940053947,-5.46777260226367));
#161043=CARTESIAN_POINT('Ctrl Pts',(-5.14464539279509,0.942310131480023,
-5.45808679753304));
#161044=CARTESIAN_POINT('Ctrl Pts',(-5.15496022882122,0.94456631596005,
-5.44840099280254));
#161045=CARTESIAN_POINT('Ctrl Pts',(-4.546581334,0.809162772000001,-5.647220394));
#161046=CARTESIAN_POINT('Ctrl Pts',(-4.85460752600001,0.874819703,-5.399228277));
#161047=CARTESIAN_POINT('Ctrl Pts',(-5.133833235,0.940053947,-5.119204656));
#161048=CARTESIAN_POINT('Ctrl Pts',(-5.14349050505391,0.942310131480023,
-5.10951978944833));
#161049=CARTESIAN_POINT('Ctrl Pts',(-5.15314777510765,0.944566315960048,
-5.09983492289654));
#161050=CARTESIAN_POINT('Origin',(0.123836934952264,0.803577357315555,0.15533825453458));
#161051=CARTESIAN_POINT('Ctrl Pts',(-5.481680828,0.940053947,-5.118708363));
#161052=CARTESIAN_POINT('Ctrl Pts',(-5.76087406,0.874398499,-4.819717273));
#161053=CARTESIAN_POINT('Ctrl Pts',(-6.00589160500001,0.809170361000001,
-4.492133795));
#161054=CARTESIAN_POINT('Ctrl Pts',(-5.133833235,0.940053947,-5.119204656));
#161055=CARTESIAN_POINT('Ctrl Pts',(-5.413053537,0.874398499,-4.83918645700001));
#161056=CARTESIAN_POINT('Ctrl Pts',(-5.660161555,0.809170361000001,-4.530460371));
#161057=CARTESIAN_POINT('',(-5.65722186906473,0.809946052729482,-4.53413064781464));
#161058=CARTESIAN_POINT('Origin',(0.139906077312995,0.946423851366999,0.141038475290444));
#161059=CARTESIAN_POINT('Ctrl Pts',(-5.85195259570582,0.849330499374381,
-4.69091151222383));
#161060=CARTESIAN_POINT('Ctrl Pts',(-5.81944146920473,0.843074444858608,
-4.66478707599213));
#161061=CARTESIAN_POINT('Ctrl Pts',(-5.78694146035946,0.836669225061311,
-4.63864782873581));
#161062=CARTESIAN_POINT('Ctrl Pts',(-5.72204085546356,0.8235515504247,-4.5863970212619));
#161063=CARTESIAN_POINT('Ctrl Pts',(-5.68960393149267,0.8168317595591,-4.56025621791836));
#161064=CARTESIAN_POINT('Ctrl Pts',(-5.6572218677119,0.809946053455765,
-4.53413064930002));
#161065=CARTESIAN_POINT('Ctrl Pts',(-5.6922260106926,0.809162772,-4.88430655563095));
#161066=CARTESIAN_POINT('Ctrl Pts',(-5.95863926358306,0.874819703,-4.57382554315626));
#161067=CARTESIAN_POINT('Ctrl Pts',(-6.18970224440444,0.940053947,-4.23620981689925));
#161068=CARTESIAN_POINT('Ctrl Pts',(-6.19769376537438,0.94231013198918,
-4.22453307341324));
#161069=CARTESIAN_POINT('Ctrl Pts',(-6.20568528634422,0.944566316978359,
-4.21285632992723));
#161070=CARTESIAN_POINT('Ctrl Pts',(-5.654270243,0.809162772000001,-4.537810928));
#161071=CARTESIAN_POINT('Ctrl Pts',(-5.90178398,0.874819703,-4.229400204));
#161072=CARTESIAN_POINT('Ctrl Pts',(-6.114284746,0.940053947,-3.895898106));
#161073=CARTESIAN_POINT('Ctrl Pts',(-6.12163427607869,0.942310131989179,
-3.88436363604635));
#161074=CARTESIAN_POINT('Ctrl Pts',(-6.12898380615742,0.944566316978361,
-3.87282916609264));
#161075=CARTESIAN_POINT('Origin',(0.154334891428051,0.80357731127327,0.125085317688508));
#161076=CARTESIAN_POINT('Ctrl Pts',(-6.453893166,0.940053947,-3.820636465));
#161077=CARTESIAN_POINT('Ctrl Pts',(-6.66228477,0.874398499000001,-3.468617329));
#161078=CARTESIAN_POINT('Ctrl Pts',(-6.831153176,0.809170361000001,-3.096021041));
#161079=CARTESIAN_POINT('Ctrl Pts',(-6.114284746,0.940053947,-3.895898106));
#161080=CARTESIAN_POINT('Ctrl Pts',(-6.326781397,0.874398499000001,-3.562402465));
#161081=CARTESIAN_POINT('Ctrl Pts',(-6.501745184,0.809170361000001,-3.207773304));
#161082=CARTESIAN_POINT('',(-6.49966322680666,0.80994605270483,-3.21198971733521));
#161083=CARTESIAN_POINT('Origin',(0.16695401651229,0.946423774500962,0.107665247463179));
#161084=CARTESIAN_POINT('Ctrl Pts',(-6.72354450891877,0.849330499373838,
-3.32324378223985));
#161085=CARTESIAN_POINT('Ctrl Pts',(-6.68617749493505,0.843074445191609,
-3.30471905299559));
#161086=CARTESIAN_POINT('Ctrl Pts',(-6.64881815156924,0.83666922520071,
-3.28617746743303));
#161087=CARTESIAN_POINT('Ctrl Pts',(-6.57420250684033,0.823551550405508,
-3.24909996596334));
#161088=CARTESIAN_POINT('Ctrl Pts',(-6.53690444003405,0.816831759514636,
-3.23054329983008));
#161089=CARTESIAN_POINT('Ctrl Pts',(-6.49966322605802,0.809946053424266,
-3.21198971904584));
#161090=CARTESIAN_POINT('Ctrl Pts',(-6.60912646082584,0.809162772000001,
-3.54645385105304));
#161091=CARTESIAN_POINT('Ctrl Pts',(-6.8025668788176,0.874819703,-3.18596073831698));
#161092=CARTESIAN_POINT('Ctrl Pts',(-6.95565033526458,0.940053947,-2.80656656937156));
#161093=CARTESIAN_POINT('Ctrl Pts',(-6.96094486404493,0.942310131896384,
-2.79344488141654));
#161094=CARTESIAN_POINT('Ctrl Pts',(-6.96623939282528,0.944566316792772,
-2.78032319346146));
#161095=CARTESIAN_POINT('Ctrl Pts',(-6.49757176,0.809162772000001,-3.216218467));
#161096=CARTESIAN_POINT('Ctrl Pts',(-6.672999573,0.874819703,-2.861810077));
#161097=CARTESIAN_POINT('Ctrl Pts',(-6.808839097,0.940053947,-2.49042369));
#161098=CARTESIAN_POINT('Ctrl Pts',(-6.81353722889499,0.942310131896384,
-2.47757895837298));
#161099=CARTESIAN_POINT('Ctrl Pts',(-6.81823536078983,0.94456631679277,
-2.46473422674598));
#161100=CARTESIAN_POINT('Origin',(0.177616129434592,0.803577343094904,0.0889833830637288));
#161101=CARTESIAN_POINT('Ctrl Pts',(-7.124328633,0.940053947,-2.343915853));
#161102=CARTESIAN_POINT('Ctrl Pts',(-7.252174449,0.874398499000001,-1.955328694));
#161103=CARTESIAN_POINT('Ctrl Pts',(-7.336997617,0.809170361000001,-1.555141784));
#161104=CARTESIAN_POINT('Ctrl Pts',(-6.808839097,0.940053947,-2.49042369));
#161105=CARTESIAN_POINT('Ctrl Pts',(-6.94467599,0.874398499000001,-2.119044493));
#161106=CARTESIAN_POINT('Ctrl Pts',(-7.039314433,0.809170361000001,-1.735094322));
#161107=CARTESIAN_POINT('',(-7.03818755630073,0.809946052706088,-1.73965971724958));
#161108=CARTESIAN_POINT('Origin',(0.186195892311229,0.946423873731715,0.0692580378799948));
#161109=CARTESIAN_POINT('Ctrl Pts',(-7.28075095342902,0.849330499377566,
-1.80018486679473));
#161110=CARTESIAN_POINT('Ctrl Pts',(-7.24027528502148,0.843074444394666,
-1.79012603746491));
#161111=CARTESIAN_POINT('Ctrl Pts',(-7.19980349267496,0.836669224887264,
-1.78004909903632));
#161112=CARTESIAN_POINT('Ctrl Pts',(-7.11896175544258,0.823551550465569,
-1.75987860727529));
#161113=CARTESIAN_POINT('Ctrl Pts',(-7.07854656259585,0.81683175970302,
-1.74977376760367));
#161114=CARTESIAN_POINT('Ctrl Pts',(-7.03818755564693,0.809946053586523,
-1.73965971925911));
#161115=CARTESIAN_POINT('Ctrl Pts',(-7.21699150217467,0.809162772,-2.04277290610175));
#161116=CARTESIAN_POINT('Ctrl Pts',(-7.32841402766746,0.874819703,-1.64912395008306));
#161117=CARTESIAN_POINT('Ctrl Pts',(-7.39635994642254,0.940053947,-1.24569138826099));
#161118=CARTESIAN_POINT('Ctrl Pts',(-7.3987099168532,0.942310131731566,
-1.23173831192582));
#161119=CARTESIAN_POINT('Ctrl Pts',(-7.40105988728378,0.944566316463135,
-1.21778523559063));
#161120=CARTESIAN_POINT('Ctrl Pts',(-7.037054042,0.809162772000001,-1.744239205));
#161121=CARTESIAN_POINT('Ctrl Pts',(-7.132193124,0.874819703,-1.360404892));
#161122=CARTESIAN_POINT('Ctrl Pts',(-7.185019699,0.940053947,-0.96849983));
#161123=CARTESIAN_POINT('Ctrl Pts',(-7.18684675339088,0.942310131731566,
-0.954945442566497));
#161124=CARTESIAN_POINT('Ctrl Pts',(-7.18867380778176,0.944566316463134,
-0.941391055132988));
#161125=CARTESIAN_POINT('Origin',(0.192592437819522,0.80357736821388,0.0487207840258531));
#161126=CARTESIAN_POINT('Ctrl Pts',(-7.461638412,0.940053947,-0.75759634));
#161127=CARTESIAN_POINT('Ctrl Pts',(-7.50296051,0.874398499000001,-0.350611062));
#161128=CARTESIAN_POINT('Ctrl Pts',(-7.499772204,0.809170361000001,0.058454175));
#161129=CARTESIAN_POINT('Ctrl Pts',(-7.18501969900001,0.940053947,-0.96849983));
#161130=CARTESIAN_POINT('Ctrl Pts',(-7.237845252,0.874398499000001,-0.576602356));
#161131=CARTESIAN_POINT('Ctrl Pts',(-7.247733164,0.809170361000001,-0.181284259));
#161132=CARTESIAN_POINT('',(-7.247614058022,0.809946052668477,-0.185985163060946));
#161133=CARTESIAN_POINT('Origin',(0.196730823848642,0.946423822056388,0.0276121826915415));
#161134=CARTESIAN_POINT('Ctrl Pts',(-7.49751757546059,0.84933049942428,
-0.192951307212126));
#161135=CARTESIAN_POINT('Ctrl Pts',(-7.45582586103834,0.84307444538524,
-0.191828720249307));
#161136=CARTESIAN_POINT('Ctrl Pts',(-7.41413402924456,0.836669225354686,
-0.190687614096639));
#161137=CARTESIAN_POINT('Ctrl Pts',(-7.33084626478269,0.823551550492759,
-0.188367281286457));
#161138=CARTESIAN_POINT('Ctrl Pts',(-7.28920371489587,0.816831759718861,
-0.187186759113356));
#161139=CARTESIAN_POINT('Ctrl Pts',(-7.24761405780495,0.809946053597453,
-0.185985165250054));
#161140=CARTESIAN_POINT('Ctrl Pts',(-7.48739804276063,0.809162772000001,
-0.443574171164248));
#161141=CARTESIAN_POINT('Ctrl Pts',(-7.51159268225307,0.874819703,-0.0351759592752993));
#161142=CARTESIAN_POINT('Ctrl Pts',(-7.49122398729508,0.940053947,0.373430937495418));
#161143=CARTESIAN_POINT('Ctrl Pts',(-7.49051951773755,0.942310131753154,
0.387562972972483));
#161144=CARTESIAN_POINT('Ctrl Pts',(-7.48981504818013,0.944566316506309,
0.401695008449552));
#161145=CARTESIAN_POINT('Ctrl Pts',(-7.24749149900001,0.809162772000001,
-0.190701257));
#161146=CARTESIAN_POINT('Ctrl Pts',(-7.25789325,0.874819703,0.204611314));
#161147=CARTESIAN_POINT('Ctrl Pts',(-7.225236766,0.940053947,0.598710006));
#161148=CARTESIAN_POINT('Ctrl Pts',(-7.22410731225338,0.942310131753154,
0.612340262221383));
#161149=CARTESIAN_POINT('Ctrl Pts',(-7.22297785850692,0.944566316506312,
0.625970518442767));
#161150=CARTESIAN_POINT('Origin',(0.198563202851664,0.80357734792354,0.00618004660839541));
#161151=CARTESIAN_POINT('Ctrl Pts',(-7.450050271,0.940053947,0.864147535));
#161152=CARTESIAN_POINT('Ctrl Pts',(-7.402916477,0.874398499000001,1.270500754));
#161153=CARTESIAN_POINT('Ctrl Pts',(-7.311865778,0.809170361000001,1.669316881));
#161154=CARTESIAN_POINT('Ctrl Pts',(-7.225236766,0.940053947,0.598710006));
#161155=CARTESIAN_POINT('Ctrl Pts',(-7.192580914,0.874398499000001,0.992801067));
#161156=CARTESIAN_POINT('Ctrl Pts',(-7.11725594700001,0.809170361000001,
1.381002455));
#161157=CARTESIAN_POINT('',(-7.11815018152856,0.809946052682178,1.3763858514358));
#161158=CARTESIAN_POINT('Origin',(0.19806736417516,0.946423835782391,-0.0153247141242421));
#161159=CARTESIAN_POINT('Ctrl Pts',(-7.36370860838713,0.849330499437629,
1.42330444072714));
#161160=CARTESIAN_POINT('Ctrl Pts',(-7.32275029711717,0.843074444948691,
1.41543829550887));
#161161=CARTESIAN_POINT('Ctrl Pts',(-7.28178789480018,0.836669225164592,
1.40759021220572));
#161162=CARTESIAN_POINT('Ctrl Pts',(-7.19994855029583,0.823551550483622,
1.39195189002707));
#161163=CARTESIAN_POINT('Ctrl Pts',(-7.15902580303483,0.81683175974397,
1.38415289520237));
#161164=CARTESIAN_POINT('Ctrl Pts',(-7.11815018169161,0.809946053567181,
1.37638584979312));
#161165=CARTESIAN_POINT('Ctrl Pts',(-7.40770217163706,0.809162772000001,
1.17636559945578));
#161166=CARTESIAN_POINT('Ctrl Pts',(-7.34353761129164,0.874819703,1.58041682072337));
#161167=CARTESIAN_POINT('Ctrl Pts',(-7.23580672022556,0.940053947,1.97509204848353));
#161168=CARTESIAN_POINT('Ctrl Pts',(-7.23208075077751,0.942310131811108,
1.98874224506117));
#161169=CARTESIAN_POINT('Ctrl Pts',(-7.22835478132945,0.944566316622219,
2.00239244163875));
#161170=CARTESIAN_POINT('Ctrl Pts',(-7.11904430900001,0.809162772000001,
1.371753671));
#161171=CARTESIAN_POINT('Ctrl Pts',(-7.044222355,0.874819703,1.760060122));
#161172=CARTESIAN_POINT('Ctrl Pts',(-6.927609792,0.940053947,2.137924827));
#161173=CARTESIAN_POINT('Ctrl Pts',(-6.92357664196574,0.942310131811108,
2.15099361657736));
#161174=CARTESIAN_POINT('Ctrl Pts',(-6.91954349193137,0.944566316622219,
2.1640624061548));
#161175=CARTESIAN_POINT('Origin',(0.195249511379292,0.803577352408136,-0.0366496854475287));
#161176=CARTESIAN_POINT('Ctrl Pts',(-7.090106059,0.940053947,2.445484832));
#161177=CARTESIAN_POINT('Ctrl Pts',(-6.95672029700001,0.874398499000001,
2.832205366));
#161178=CARTESIAN_POINT('Ctrl Pts',(-6.782064634,0.809170361000001,3.202124185));
#161179=CARTESIAN_POINT('Ctrl Pts',(-6.927609792,0.940053947,2.137924827));
#161180=CARTESIAN_POINT('Ctrl Pts',(-6.810999487,0.874398499000001,2.515782215));
#161181=CARTESIAN_POINT('Ctrl Pts',(-6.653983753,0.809170361000001,2.87871503));
#161182=CARTESIAN_POINT('',(-6.655849513603,0.809946052668528,2.8743985932961));
#161183=CARTESIAN_POINT('Origin',(0.190142419849683,0.946423866384608,-0.0575450923149956));
#161184=CARTESIAN_POINT('Ctrl Pts',(-6.885580810478,0.849330499379893,2.97300805530621));
#161185=CARTESIAN_POINT('Ctrl Pts',(-6.84727107633071,0.843074445841034,
2.9565209924128));
#161186=CARTESIAN_POINT('Ctrl Pts',(-6.80895345511024,0.83666922557787,
2.940050685833));
#161187=CARTESIAN_POINT('Ctrl Pts',(-6.73238924394341,0.823551550535741,
2.90718493774205));
#161188=CARTESIAN_POINT('Ctrl Pts',(-6.694099800825,0.816831759741263,2.89077109770459));
#161189=CARTESIAN_POINT('Ctrl Pts',(-6.65584951439853,0.809946053640974,
2.87439859102855));
#161190=CARTESIAN_POINT('Ctrl Pts',(-6.9816303808209,0.809162772000001,
2.74129982289529));
#161191=CARTESIAN_POINT('Ctrl Pts',(-6.83210688278208,0.874819703,3.12211106708376));
#161192=CARTESIAN_POINT('Ctrl Pts',(-6.64205117335252,0.940053947,3.48440004939027));
#161193=CARTESIAN_POINT('Ctrl Pts',(-6.63547792639119,0.942310131765159,
3.4969301383795));
#161194=CARTESIAN_POINT('Ctrl Pts',(-6.62890467942987,0.944566316530321,
3.50946022736874));
#161195=CARTESIAN_POINT('Ctrl Pts',(-6.657718518,0.809162772000001,2.870066921));
#161196=CARTESIAN_POINT('Ctrl Pts',(-6.501171452,0.874819703,3.233210475));
#161197=CARTESIAN_POINT('Ctrl Pts',(-6.306055484,0.940053947,3.577172659));
#161198=CARTESIAN_POINT('Ctrl Pts',(-6.29930722346308,0.942310131765159,
3.58906889925277));
#161199=CARTESIAN_POINT('Ctrl Pts',(-6.2925589629262,0.944566316530321,
3.60096513950554));
#161200=CARTESIAN_POINT('Origin',(0.182806037430469,0.803577345213135,-0.077765686486444));
#161201=CARTESIAN_POINT('Ctrl Pts',(-6.398636369,0.940053947,3.912473977));
#161202=CARTESIAN_POINT('Ctrl Pts',(-6.185235608,0.874398499000001,4.261479203));
#161203=CARTESIAN_POINT('Ctrl Pts',(-5.935141687,0.809170361000001,4.585203721));
#161204=CARTESIAN_POINT('Ctrl Pts',(-6.306055484,0.940053947,3.577172659));
#161205=CARTESIAN_POINT('Ctrl Pts',(-6.110943294,0.874398499000001,3.921128183));
#161206=CARTESIAN_POINT('Ctrl Pts',(-5.879578673,0.809170361000001,4.241822088));
#161207=CARTESIAN_POINT('',(-5.88232871960182,0.809946052669728,4.23800765141649));
#161208=CARTESIAN_POINT('Origin',(0.173326479965217,0.946423872780383,-0.0970747065690575));
#161209=CARTESIAN_POINT('Ctrl Pts',(-6.0854909077331,0.8493304994229,4.38369711687508));
#161210=CARTESIAN_POINT('Ctrl Pts',(-6.05162106171033,0.843074445266074,
4.35936004959652));
#161211=CARTESIAN_POINT('Ctrl Pts',(-6.01773991588643,0.836669225298237,
4.33503765500536));
#161212=CARTESIAN_POINT('Ctrl Pts',(-5.95003089877634,0.82355155048126,
4.28648124866588));
#161213=CARTESIAN_POINT('Ctrl Pts',(-5.91616513215529,0.816831759747061,
4.26222005696166));
#161214=CARTESIAN_POINT('Ctrl Pts',(-5.8823287207792,0.809946053616843,
4.23800764950177));
#161215=CARTESIAN_POINT('Ctrl Pts',(-6.2291053126731,0.809162772000001,
4.17805391238259));
#161216=CARTESIAN_POINT('Ctrl Pts',(-6.00121443024314,0.874819703,4.51781886922408));
#161217=CARTESIAN_POINT('Ctrl Pts',(-5.73772069546419,0.940053947,4.83078137711899));
#161218=CARTESIAN_POINT('Ctrl Pts',(-5.72860752855345,0.942310131779373,
4.84160546587255));
#161219=CARTESIAN_POINT('Ctrl Pts',(-5.71949436164269,0.944566316558748,
4.85242955462612));
#161220=CARTESIAN_POINT('Ctrl Pts',(-5.88508521,0.809162772000001,4.234179032));
#161221=CARTESIAN_POINT('Ctrl Pts',(-5.65413299700001,0.874819703,4.5551795));
#161222=CARTESIAN_POINT('Ctrl Pts',(-5.38963702999999,0.940053947,4.849155874));
#161223=CARTESIAN_POINT('Ctrl Pts',(-5.38048919998988,0.942310131779373,
4.85932331030102));
#161224=CARTESIAN_POINT('Ctrl Pts',(-5.37134136997988,0.944566316558748,
4.86949074660191));
#161225=CARTESIAN_POINT('Origin',(0.161815073416527,0.803577351637582,-0.115245659545124));
#161226=CARTESIAN_POINT('Ctrl Pts',(-5.407973553,0.940053947,5.196520186));
#161227=CARTESIAN_POINT('Ctrl Pts',(-5.124536177,0.874398499000001,5.491491009));
#161228=CARTESIAN_POINT('Ctrl Pts',(-4.81069811,0.809170361000001,5.753884227));
#161229=CARTESIAN_POINT('Ctrl Pts',(-5.38963703,0.940053947,4.849155874));
#161230=CARTESIAN_POINT('Ctrl Pts',(-5.125146184,0.874398499000001,5.143126555));
#161231=CARTESIAN_POINT('Ctrl Pts',(-4.830251029,0.809170361000001,5.406586261));
#161232=CARTESIAN_POINT('',(-4.83375677212873,0.809946052702061,5.40345218124008));
#161233=CARTESIAN_POINT('Origin',(0.148405984167564,0.946423872553155,-0.132065222751626));
#161234=CARTESIAN_POINT('Ctrl Pts',(-5.00085021302196,0.849330499383347,
5.58940937375437));
#161235=CARTESIAN_POINT('Ctrl Pts',(-4.9730039753034,0.84307444525625,5.55836027797521));
#161236=CARTESIAN_POINT('Ctrl Pts',(-4.94514354752411,0.836669225265375,
5.52732308242854));
#161237=CARTESIAN_POINT('Ctrl Pts',(-4.88945572164077,0.823551550481411,
5.46534646060306));
#161238=CARTESIAN_POINT('Ctrl Pts',(-4.86159715640179,0.816831759647414,
5.43437234271068));
#161239=CARTESIAN_POINT('Ctrl Pts',(-4.83375677361857,0.809946053577941,
5.40345217970358));
#161240=CARTESIAN_POINT('Ctrl Pts',(-5.1853142030829,0.809162772,5.4194468453736));
#161241=CARTESIAN_POINT('Ctrl Pts',(-4.88971186043539,0.874819703,5.7022784826116));
#161242=CARTESIAN_POINT('Ctrl Pts',(-4.56510077445979,0.940053947,5.95128073642129));
#161243=CARTESIAN_POINT('Ctrl Pts',(-4.55387380829232,0.942310131960985,
5.95989270317139));
#161244=CARTESIAN_POINT('Ctrl Pts',(-4.54264684212497,0.944566316921971,
5.96850466992152));
#161245=CARTESIAN_POINT('Ctrl Pts',(-4.837271857,0.809162772000001,5.400305637));
#161246=CARTESIAN_POINT('Ctrl Pts',(-4.54271356700001,0.874819703,5.664153394));
#161247=CARTESIAN_POINT('Ctrl Pts',(-4.221205138,0.940053947,5.894397949));
#161248=CARTESIAN_POINT('Ctrl Pts',(-4.21008548001271,0.942310131960985,
5.90236116387744));
#161249=CARTESIAN_POINT('Ctrl Pts',(-4.19896582202542,0.944566316921971,
5.91032437875497));
#161250=CARTESIAN_POINT('Origin',(0.133257403895742,0.803577328187921,-0.147336580872585));
#161251=CARTESIAN_POINT('Ctrl Pts',(-4.164439905,0.940053947,6.237582888));
#161252=CARTESIAN_POINT('Ctrl Pts',(-3.824219129,0.874398499000001,6.464726799));
#161253=CARTESIAN_POINT('Ctrl Pts',(-3.461311636,0.809170361000001,6.653519501));
#161254=CARTESIAN_POINT('Ctrl Pts',(-4.221205138,0.940053947,5.894397949));
#161255=CARTESIAN_POINT('Ctrl Pts',(-3.899702935,0.874398499000001,6.124638046));
#161256=CARTESIAN_POINT('Ctrl Pts',(-3.555066216,0.809170361000001,6.318544469));
#161257=CARTESIAN_POINT('',(-3.55916373151898,0.809946052669262,6.31623729403005));
#161258=CARTESIAN_POINT('Origin',(0.116546246060481,0.946423908382474,-0.160880525506759));
#161259=CARTESIAN_POINT('Ctrl Pts',(-3.68237532007637,0.849330499360679,
6.53376706035624));
#161260=CARTESIAN_POINT('Ctrl Pts',(-3.66185475181377,0.84307444585648,
6.49745776082882));
#161261=CARTESIAN_POINT('Ctrl Pts',(-3.64131776402704,0.836669225572331,
6.46115702750206));
#161262=CARTESIAN_POINT('Ctrl Pts',(-3.60025502958651,0.82355155050574,
6.38865814675778));
#161263=CARTESIAN_POINT('Ctrl Pts',(-3.57970630226656,0.816831759753065,
6.35241941900083));
#161264=CARTESIAN_POINT('Ctrl Pts',(-3.55916373330938,0.809946053662904,
6.31623729282445));
#161265=CARTESIAN_POINT('Ctrl Pts',(-3.89906356435541,0.809162772,6.40743246670616));
#161266=CARTESIAN_POINT('Ctrl Pts',(-3.54957179938179,0.874819703,6.62010589188594));
#161267=CARTESIAN_POINT('Ctrl Pts',(-3.17902181502426,0.940053947,6.79350482401382));
#161268=CARTESIAN_POINT('Ctrl Pts',(-3.16620601068798,0.942310131974825,
6.79950198196843));
#161269=CARTESIAN_POINT('Ctrl Pts',(-3.15339020635174,0.94456631694965,
6.80549913992302));
#161270=CARTESIAN_POINT('Ctrl Pts',(-3.563273049,0.809162772000001,6.313919953));
#161271=CARTESIAN_POINT('Ctrl Pts',(-3.2188819,0.874819703,6.508277771));
#161272=CARTESIAN_POINT('Ctrl Pts',(-2.855394386,0.940053947,6.664024527));
#161273=CARTESIAN_POINT('Ctrl Pts',(-2.84282284355026,0.942310131974825,
6.66941116857376));
#161274=CARTESIAN_POINT('Ctrl Pts',(-2.83025130110046,0.944566316949653,
6.67479781014762));
#161275=CARTESIAN_POINT('Origin',(0.0984688995454319,0.803577314516454,
-0.172538347558309));
#161276=CARTESIAN_POINT('Ctrl Pts',(-2.726181675,0.940053947,6.986983146));
#161277=CARTESIAN_POINT('Ctrl Pts',(-2.345085845,0.874398499000001,7.135679149));
#161278=CARTESIAN_POINT('Ctrl Pts',(-1.950078078,0.809170361000001,7.24204359900001));
#161279=CARTESIAN_POINT('Ctrl Pts',(-2.855394386,0.940053947,6.664024527));
#161280=CARTESIAN_POINT('Ctrl Pts',(-2.491913911,0.874398499000001,6.819768268));
#161281=CARTESIAN_POINT('Ctrl Pts',(-2.113650457,0.809170361000001,6.93505456));
#161282=CARTESIAN_POINT('',(-2.11814814972717,0.809946052719587,6.93368216984298));
#161283=CARTESIAN_POINT('Origin',(0.0792368644578836,0.946423905641289,
-0.182173114611933));
#161284=CARTESIAN_POINT('Ctrl Pts',(-2.19171665082089,0.849330499388496,
7.17261306095222));
#161285=CARTESIAN_POINT('Ctrl Pts',(-2.17948126560287,0.843074444602531,
7.13274132886931));
#161286=CARTESIAN_POINT('Ctrl Pts',(-2.16722800712273,0.836669224998938,
7.09287444566833));
#161287=CARTESIAN_POINT('Ctrl Pts',(-2.14271041383307,0.82355155055306,
7.0132432779999));
#161288=CARTESIAN_POINT('Ctrl Pts',(-2.13043235937359,0.816831759769418,
6.97343442234686));
#161289=CARTESIAN_POINT('Ctrl Pts',(-2.11814815162338,0.809946053689787,
6.93368216908896));
#161290=CARTESIAN_POINT('Ctrl Pts',(-2.43049704742019,0.809162772000001,
7.0958136667112));
#161291=CARTESIAN_POINT('Ctrl Pts',(-2.04345770500201,0.874819703,7.22838450695476));
#161292=CARTESIAN_POINT('Ctrl Pts',(-1.64429532972973,0.940053947,7.3180721746251));
#161293=CARTESIAN_POINT('Ctrl Pts',(-1.63048994008922,0.94231013198164,
7.32117410325077));
#161294=CARTESIAN_POINT('Ctrl Pts',(-1.61668455044872,0.944566316963281,
7.32427603187633));
#161295=CARTESIAN_POINT('Ctrl Pts',(-2.122659554,0.809162772000001,6.932302389));
#161296=CARTESIAN_POINT('Ctrl Pts',(-1.744538893,0.874819703,7.04808231200001));
#161297=CARTESIAN_POINT('Ctrl Pts',(-1.356068566,0.940053947,7.122048725));
#161298=CARTESIAN_POINT('Ctrl Pts',(-1.34263297046233,0.942310131981639,
7.1246069198977));
#161299=CARTESIAN_POINT('Ctrl Pts',(-1.32919737492467,0.94456631696328,
7.12716511479539));
#161300=CARTESIAN_POINT('Origin',(0.0590761169157883,0.803577364487472,
-0.189672464537588));
#161301=CARTESIAN_POINT('Ctrl Pts',(-1.16045022,0.940053947,7.409679837));
#161302=CARTESIAN_POINT('Ctrl Pts',(-0.756298953000001,0.874398499000001,
7.47297507200001));
#161303=CARTESIAN_POINT('Ctrl Pts',(-0.347661035,0.809170361000001,7.491937787));
#161304=CARTESIAN_POINT('Ctrl Pts',(-1.356068566,0.940053947,7.122048725));
#161305=CARTESIAN_POINT('Ctrl Pts',(-0.967605761,0.874398499000001,7.196013706));
#161306=CARTESIAN_POINT('Ctrl Pts',(-0.573402753,0.809170361000001,7.227289207));
#161307=CARTESIAN_POINT('',(-0.578090314703847,0.809946052713699,7.22691577389676));
#161308=CARTESIAN_POINT('Origin',(0.0382225075640378,0.946423838787555,
-0.194947625922174));
#161309=CARTESIAN_POINT('Ctrl Pts',(-0.598575746204804,0.849330499425487,
7.47607564640176));
#161310=CARTESIAN_POINT('Ctrl Pts',(-0.595197661092526,0.843074444324486,
7.43450584510454));
#161311=CARTESIAN_POINT('Ctrl Pts',(-0.591801078470085,0.83666922486761,
7.39293694026594));
#161312=CARTESIAN_POINT('Ctrl Pts',(-0.584975040072362,0.823551550502395,
7.30989694812043));
#161313=CARTESIAN_POINT('Ctrl Pts',(-0.581541766932348,0.816831759718931,
7.26837938286832));
#161314=CARTESIAN_POINT('Ctrl Pts',(-0.578090316529954,0.809946053577953,
7.22691577360123));
#161315=CARTESIAN_POINT('Ctrl Pts',(-0.848283189425136,0.809162772000001,
7.45240250623194));
#161316=CARTESIAN_POINT('Ctrl Pts',(-0.441793800398221,0.874819703,7.49867189599368));
#161317=CARTESIAN_POINT('Ctrl Pts',(-0.032683421404803,0.940053947,7.50045460502934));
#161318=CARTESIAN_POINT('Ctrl Pts',(-0.0185339724271852,0.942310131771804,
7.50051626161846));
#161319=CARTESIAN_POINT('Ctrl Pts',(-0.00438452344956661,0.944566316543609,
7.50057791820755));
#161320=CARTESIAN_POINT('Ctrl Pts',(-0.582792857,0.809162772000001,7.226538071));
#161321=CARTESIAN_POINT('Ctrl Pts',(-0.188623186,0.874819703,7.25832635800001));
#161322=CARTESIAN_POINT('Ctrl Pts',(0.206665513,0.940053947,7.24705384000001));
#161323=CARTESIAN_POINT('Ctrl Pts',(0.220336926792266,0.942310131771804,
7.24666396986597));
#161324=CARTESIAN_POINT('Ctrl Pts',(0.234008340584527,0.944566316543609,
7.24627409973195));
#161325=CARTESIAN_POINT('Origin',(0.0169207711628139,0.803576816201109,
-0.197933668297665));
#161326=CARTESIAN_POINT('Ctrl Pts',(0.201949703,0.940837228,7.247186786));
#161327=CARTESIAN_POINT('Ctrl Pts',(0.597245653,0.875180297,7.236171492));
#161328=CARTESIAN_POINT('Ctrl Pts',(0.988998379000001,0.809946053,7.182226828));
#161329=CARTESIAN_POINT('Ctrl Pts',(1.0025474970505,0.807689868386007,7.18036110359729));
#161330=CARTESIAN_POINT('Ctrl Pts',(1.016096615101,0.805433683772012,7.17849537919455));
#161331=CARTESIAN_POINT('Ctrl Pts',(-0.0375640730680385,0.940837228,7.50043175004996));
#161332=CARTESIAN_POINT('Ctrl Pts',(0.371545059364261,0.875180297,7.50248067266357));
#161333=CARTESIAN_POINT('Ctrl Pts',(0.778449959968396,0.809946053,7.46002031822874));
#161334=CARTESIAN_POINT('Ctrl Pts',(0.792523129515691,0.807689868386006,
7.45855178893327));
#161335=CARTESIAN_POINT('Ctrl Pts',(0.806596299062982,0.805433683772012,
7.45708325963789));
#161336=CARTESIAN_POINT('',(0.213239091069717,0.900669500237862,7.49696799323959));
#161337=CARTESIAN_POINT('',(0.778885076486235,0.809946052263419,7.4594462526428));
#161338=CARTESIAN_POINT('Origin',(0.0019124482713892,0.946416032070669,
-0.191459090284092));
#161339=CARTESIAN_POINT('',(0.883941732031841,0.809946053334084,7.32083652775467));
#161340=CARTESIAN_POINT('Ctrl Pts',(0.213239091291757,0.900669500620797,
7.49696799318031));
#161341=CARTESIAN_POINT('Ctrl Pts',(0.212102887926396,0.90692555462208,
7.45527664792096));
#161342=CARTESIAN_POINT('Ctrl Pts',(0.210985170232026,0.913330774802257,
7.41358418156647));
#161343=CARTESIAN_POINT('Ctrl Pts',(0.208792991462068,0.926448449729418,
7.3302929450039));
#161344=CARTESIAN_POINT('Ctrl Pts',(0.207717300174009,0.933168240538447,
7.28864755498878));
#161345=CARTESIAN_POINT('Ctrl Pts',(0.206665513330684,0.940053946543812,
7.24705384020173));
#161346=CARTESIAN_POINT('Ctrl Pts',(0.988998379000001,0.809946053,7.182226828));
#161347=CARTESIAN_POINT('Ctrl Pts',(1.380743519,0.875601501,7.128283209));
#161348=CARTESIAN_POINT('Ctrl Pts',(1.764297565,0.940829639,7.032051913));
#161349=CARTESIAN_POINT('Ctrl Pts',(1.266217779,0.809946053,7.392340126));
#161350=CARTESIAN_POINT('Ctrl Pts',(1.669423273,0.875601501,7.323275938));
#161351=CARTESIAN_POINT('Ctrl Pts',(2.062725117,0.940829639,7.210767303));
#161352=CARTESIAN_POINT('',(1.26621779070058,0.809946052007887,7.39234012253307));
#161353=CARTESIAN_POINT('',(1.81988019092492,0.90066950060491,7.27585294567191));
#161354=CARTESIAN_POINT('Origin',(-0.0314977611305134,0.803573282467146,
-0.190000801682366));
#161355=CARTESIAN_POINT('Ctrl Pts',(1.75973614606893,0.940053944097848,
7.03319478750167));
#161356=CARTESIAN_POINT('Ctrl Pts',(1.76970476259936,0.933168237615819,
7.07358996388049));
#161357=CARTESIAN_POINT('Ctrl Pts',(1.77970782974647,0.926448448759319,
7.11403045415623));
#161358=CARTESIAN_POINT('Ctrl Pts',(1.79975390956644,0.913330774361959,
7.19490313090962));
#161359=CARTESIAN_POINT('Ctrl Pts',(1.80980814175334,0.906925555236439,
7.23538056739943));
#161360=CARTESIAN_POINT('Ctrl Pts',(1.81988018914809,0.900669500605544,
7.27585294611419));
#161361=CARTESIAN_POINT('',(1.12760809690174,0.809946050061996,7.28728347422995));
#161362=CARTESIAN_POINT('Origin',(3.62231945827407E-13,0.714028547999755,
1.57773100140091E-12));
#161363=CARTESIAN_POINT('',(2.00688844721255,0.749999999457025,7.22650665628683));
#161364=CARTESIAN_POINT('',(1.81501009314308,0.714243089266212,7.24021154783803));
#161365=CARTESIAN_POINT('Origin',(1.418460290385,0.473618757495434,-0.336301876236789));
#161366=CARTESIAN_POINT('',(1.6362104624896,0.750000000179527,7.31934527981378));
#161367=CARTESIAN_POINT('Origin',(0.,0.750000000000029,0.));
#161368=CARTESIAN_POINT('Origin',(-1.44669394436553,0.692075205405702,0.130173868264863));
#161369=CARTESIAN_POINT('Ctrl Pts',(1.755159165,0.940837228,7.03433837));
#161370=CARTESIAN_POINT('Ctrl Pts',(2.138845352,0.875180297,6.938603662));
#161371=CARTESIAN_POINT('Ctrl Pts',(2.509842609,0.809946053,6.801704939));
#161372=CARTESIAN_POINT('Ctrl Pts',(2.52267388045516,0.807689868413341,
6.79697017440664));
#161373=CARTESIAN_POINT('Ctrl Pts',(2.53550515191036,0.80543368382668,6.79223540981329));
#161374=CARTESIAN_POINT('Ctrl Pts',(1.57568526882813,0.940837228000001,
7.33315098851839));
#161375=CARTESIAN_POINT('Ctrl Pts',(1.97567011476546,0.875180297,7.2472056382825));
#161376=CARTESIAN_POINT('Ctrl Pts',(2.36393408428999,0.809946053,7.11826545847073));
#161377=CARTESIAN_POINT('Ctrl Pts',(2.37736254041797,0.807689868413341,
7.11380594720096));
#161378=CARTESIAN_POINT('Ctrl Pts',(2.39079099654594,0.80543368382668,7.10934643593125));
#161379=CARTESIAN_POINT('',(2.36423562280412,0.809946052264267,7.11761127582573));
#161380=CARTESIAN_POINT('Origin',(-0.0392902992667366,0.94641605726145,
-0.187394038683174));
#161381=CARTESIAN_POINT('',(2.43703911643165,0.809946053334091,6.9596580948236));
#161382=CARTESIAN_POINT('Origin',(1.50704101975485E-14,0.901573517999972,
-2.42861286636753E-14));
#161383=CARTESIAN_POINT('Origin',(-0.0598766578396351,0.803569475455572,
-0.183507600577532));
#161384=CARTESIAN_POINT('Origin',(-0.0100119907423271,0.946349155189795,
-0.187382485778542));
#161385=CARTESIAN_POINT('Ctrl Pts',(2.509842609,0.809946053,6.801704939));
#161386=CARTESIAN_POINT('Ctrl Pts',(2.880832682,0.875601501,6.66480886600001));
#161387=CARTESIAN_POINT('Ctrl Pts',(3.234732564,0.940829639,6.488374622));
#161388=CARTESIAN_POINT('Ctrl Pts',(2.825748922,0.809946053,6.947311928));
#161389=CARTESIAN_POINT('Ctrl Pts',(3.204680937,0.875601501,6.79318516));
#161390=CARTESIAN_POINT('Ctrl Pts',(3.564601571,0.940829639,6.598758644));
#161391=CARTESIAN_POINT('',(2.82574893270958,0.809946052007888,6.94731192209775));
#161392=CARTESIAN_POINT('',(3.34142571447524,0.900669500630793,6.7145271012109));
#161393=CARTESIAN_POINT('Origin',(-0.0716058869392666,0.803573306649502,
-0.178787532532706));
#161394=CARTESIAN_POINT('Ctrl Pts',(3.23052347273381,0.940053944111675,
6.49047134690417));
#161395=CARTESIAN_POINT('Ctrl Pts',(3.24894279738607,0.933168237661529,
6.52777914866813));
#161396=CARTESIAN_POINT('Ctrl Pts',(3.26740550839828,0.926448448819339,
6.56512379910516));
#161397=CARTESIAN_POINT('Ctrl Pts',(3.30436815694365,0.913330774448048,
6.63979640314351));
#161398=CARTESIAN_POINT('Ctrl Pts',(3.32288877927613,0.906925555273596,
6.67716613732868));
#161399=CARTESIAN_POINT('Ctrl Pts',(3.34142571288598,0.90066950063885,6.71452710194404));
#161400=CARTESIAN_POINT('',(2.66779578238773,0.809946050061996,6.87450842694637));
#161401=CARTESIAN_POINT('Origin',(-3.44385978068296E-12,0.714028548,-7.08114122893733E-12));
#161402=CARTESIAN_POINT('',(3.51345383299265,0.750000000485261,6.62613325171387));
#161403=CARTESIAN_POINT('',(3.32900763030012,0.714243089209672,6.68076590610822));
#161404=CARTESIAN_POINT('Origin',(1.31300551899894,0.473612695239739,-0.633360103017074));
#161405=CARTESIAN_POINT('',(3.17139964474746,0.750000001078249,6.79648617292802));
#161406=CARTESIAN_POINT('Origin',(0.,0.750000001663587,0.));
#161407=CARTESIAN_POINT('Origin',(-1.38488278791584,0.692074389599663,0.438133504989625));
#161408=CARTESIAN_POINT('Ctrl Pts',(3.226299335,0.940837228,6.49257211000001));
#161409=CARTESIAN_POINT('Ctrl Pts',(3.58043502,0.875180297,6.316594438));
#161410=CARTESIAN_POINT('Ctrl Pts',(3.913329389,0.809946053,6.103142887));
#161411=CARTESIAN_POINT('Ctrl Pts',(3.92484283829835,0.807689868363815,
6.09576047432214));
#161412=CARTESIAN_POINT('Ctrl Pts',(3.93635628759674,0.805433683727629,
6.0883780616443));
#161413=CARTESIAN_POINT('Ctrl Pts',(3.11525731968877,0.940837228,6.82298023806302));
#161414=CARTESIAN_POINT('Ctrl Pts',(3.48741503215394,0.875180297,6.65305932400711));
#161415=CARTESIAN_POINT('Ctrl Pts',(3.83888327807559,0.809946053,6.44366841676578));
#161416=CARTESIAN_POINT('Ctrl Pts',(3.8510391215089,0.807689868363815,6.43642644508177));
#161417=CARTESIAN_POINT('Ctrl Pts',(3.86319496494222,0.805433683727626,
6.42918447339777));
#161418=CARTESIAN_POINT('',(3.83903713685176,0.809946052264257,6.44296470667385));
#161419=CARTESIAN_POINT('Origin',(-0.0786558313566327,0.946416059587553,
-0.17456648136527));
#161420=CARTESIAN_POINT('',(3.87618326074108,0.809946053334091,6.27305378442417));
#161421=CARTESIAN_POINT('Origin',(-3.5301622736128E-13,0.901573518000111,
-7.81926606796546E-13));
#161422=CARTESIAN_POINT('Origin',(-0.0979259484658586,0.803569487859856,
-0.166346363162171));
#161423=CARTESIAN_POINT('Origin',(-0.0500596334563524,0.946349154708691,
-0.180849358721544));
#161424=CARTESIAN_POINT('Ctrl Pts',(3.913329389,0.809946053,6.10314288700001));
#161425=CARTESIAN_POINT('Ctrl Pts',(4.246217311,0.875601501,5.889695469));
#161426=CARTESIAN_POINT('Ctrl Pts',(4.553915063,0.940829639,5.641308146));
#161427=CARTESIAN_POINT('Ctrl Pts',(4.253151186,0.809946053,6.177435146));
#161428=CARTESIAN_POINT('Ctrl Pts',(4.590091282,0.875601501,5.945452595));
#161429=CARTESIAN_POINT('Ctrl Pts',(4.899801218,0.940829639,5.678199365));
#161430=CARTESIAN_POINT('',(4.25315119522186,0.809946052117954,6.17743513791709));
#161431=CARTESIAN_POINT('',(4.706729884842,0.900669500619148,5.83923743243706));
#161432=CARTESIAN_POINT('Origin',(-0.108365671154418,0.803573282975787,
-0.159214253083495));
#161433=CARTESIAN_POINT('Ctrl Pts',(4.55025511129989,0.940053944236844,
5.64426068024899));
#161434=CARTESIAN_POINT('Ctrl Pts',(4.57626387687572,0.933168237793891,
5.67673663592812));
#161435=CARTESIAN_POINT('Ctrl Pts',(4.60232293632015,0.926448448835655,
5.7092392526236));
#161436=CARTESIAN_POINT('Ctrl Pts',(4.65447382124695,0.913330774452229,
5.77422017591404));
#161437=CARTESIAN_POINT('Ctrl Pts',(4.6805948299349,0.90692555527452,5.80673484018321));
#161438=CARTESIAN_POINT('Ctrl Pts',(4.70672988344559,0.900669500619791,
5.83923743356002));
#161439=CARTESIAN_POINT('',(4.08324030258406,0.809946050061996,6.14028900646922));
#161440=CARTESIAN_POINT('Origin',(-6.76672259891653E-12,0.714028548000489,
-8.63588714428154E-12));
#161441=CARTESIAN_POINT('',(4.85573401221774,0.749999999448248,5.7159292241174));
#161442=CARTESIAN_POINT('',(4.6873444694292,0.714243089225114,5.80893507623871));
#161443=CARTESIAN_POINT('Origin',(1.14615087329816,0.473617861364629,-0.900814468059661));
#161444=CARTESIAN_POINT('',(4.55829771058855,0.750000000258868,5.95583092318158));
#161445=CARTESIAN_POINT('Origin',(0.,0.750000000000029,0.));
#161446=CARTESIAN_POINT('Origin',(-1.25832425134463,0.692075148191809,0.725594522822336));
#161447=CARTESIAN_POINT('Ctrl Pts',(4.546581334,0.940837228,5.647220394));
#161448=CARTESIAN_POINT('Ctrl Pts',(4.85460752600001,0.875180297,5.399228277));
#161449=CARTESIAN_POINT('Ctrl Pts',(5.133833235,0.809946053,5.119204656));
#161450=CARTESIAN_POINT('Ctrl Pts',(5.14349050550429,0.807689868414757,
5.10951978899666));
#161451=CARTESIAN_POINT('Ctrl Pts',(5.15314777600842,0.805433683829514,
5.0998349219932));
#161452=CARTESIAN_POINT('Ctrl Pts',(4.50916339980159,0.940837228,5.99377451448312));
#161453=CARTESIAN_POINT('Ctrl Pts',(4.83609229828414,0.875180297,5.74782334933033));
#161454=CARTESIAN_POINT('Ctrl Pts',(5.1343305567691,0.809946053,5.4677726022714));
#161455=CARTESIAN_POINT('Ctrl Pts',(5.14464539327617,0.807689868414757,
5.45808679708906));
#161456=CARTESIAN_POINT('Ctrl Pts',(5.15496022978334,0.805433683829514,
5.44840099190685));
#161457=CARTESIAN_POINT('',(5.13432954268828,0.809946052265052,5.46705226768057));
#161458=CARTESIAN_POINT('Origin',(-0.11434362939921,0.946416045952697,-0.153576652678157));
#161459=CARTESIAN_POINT('',(5.1340813834691,0.809946053334091,5.29312845107504));
#161460=CARTESIAN_POINT('Origin',(6.66133814775094E-13,0.901573517999972,
8.30065183254902E-13));
#161461=CARTESIAN_POINT('Origin',(-0.131395602648939,0.803569504711666,
-0.141405634131786));
#161462=CARTESIAN_POINT('Origin',(-0.0877662100594562,0.946349440318976,
-0.165859511884162));
#161463=CARTESIAN_POINT('Ctrl Pts',(5.133833235,0.809946053,5.119204656));
#161464=CARTESIAN_POINT('Ctrl Pts',(5.413053537,0.875601501,4.839186457));
#161465=CARTESIAN_POINT('Ctrl Pts',(5.660161555,0.940829639,4.530460371));
#161466=CARTESIAN_POINT('Ctrl Pts',(5.481680828,0.809946053,5.118708363));
#161467=CARTESIAN_POINT('Ctrl Pts',(5.76087406,0.875601501,4.819717273));
#161468=CARTESIAN_POINT('Ctrl Pts',(6.00589160500001,0.940829639,4.492133795));
#161469=CARTESIAN_POINT('',(5.48168083522909,0.809946052117951,5.11870835314386));
#161470=CARTESIAN_POINT('',(5.85195259677292,0.900669500639929,4.69091151073651));
#161471=CARTESIAN_POINT('Origin',(-0.140058776189231,0.803573323345158,
-0.132196708794412));
#161472=CARTESIAN_POINT('Ctrl Pts',(5.65722187832807,0.940053944286819,
4.53413065786505));
#161473=CARTESIAN_POINT('Ctrl Pts',(5.68960394382895,0.933168237856532,
4.56025622786481));
#161474=CARTESIAN_POINT('Ctrl Pts',(5.72204085889477,0.926448448864469,
4.5863970240271));
#161475=CARTESIAN_POINT('Ctrl Pts',(5.78694146272018,0.913330774478859,
4.63864783063363));
#161476=CARTESIAN_POINT('Ctrl Pts',(5.81944146835668,0.906925555304823,
4.66478707531063));
#161477=CARTESIAN_POINT('Ctrl Pts',(5.85195259562809,0.900669500640576,
4.69091151216137));
#161478=CARTESIAN_POINT('',(5.30775704407508,0.809946050061996,5.11895649646111));
#161479=CARTESIAN_POINT('Origin',(3.37230243729891E-12,0.714028547998777,
2.2963402013243E-12));
#161480=CARTESIAN_POINT('',(5.97096547083895,0.749999999471665,4.53845469731977));
#161481=CARTESIAN_POINT('',(5.82650629090568,0.714243089334641,4.66548489856268));
#161482=CARTESIAN_POINT('Origin',(0.925704659898806,0.473619308971619,-1.12614361973372));
#161483=CARTESIAN_POINT('',(5.73205483888752,0.750000000168396,4.83668763995693));
#161484=CARTESIAN_POINT('Origin',(0.,0.750000000000029,0.));
#161485=CARTESIAN_POINT('Origin',(-1.07292362222049,0.692075011843041,0.979133253777728));
#161486=CARTESIAN_POINT('Ctrl Pts',(5.654270243,0.940837228,4.537810928));
#161487=CARTESIAN_POINT('Ctrl Pts',(5.90178398,0.875180297,4.229400204));
#161488=CARTESIAN_POINT('Ctrl Pts',(6.114284746,0.809946053,3.895898106));
#161489=CARTESIAN_POINT('Ctrl Pts',(6.12163427499651,0.807689868343035,
3.88436363774475));
#161490=CARTESIAN_POINT('Ctrl Pts',(6.12898380399303,0.805433683686068,
3.87282916948945));
#161491=CARTESIAN_POINT('Ctrl Pts',(5.69222601069185,0.940837228000001,
4.88430655562403));
#161492=CARTESIAN_POINT('Ctrl Pts',(5.95863926358193,0.875180297000001,
4.57382554314938));
#161493=CARTESIAN_POINT('Ctrl Pts',(6.18970224440294,0.809946053,4.23620981689245));
#161494=CARTESIAN_POINT('Ctrl Pts',(6.19769376419614,0.807689868343035,
4.2245330751258));
#161495=CARTESIAN_POINT('Ctrl Pts',(6.20568528398925,0.805433683686067,
4.21285633335913));
#161496=CARTESIAN_POINT('',(6.18954640337577,0.80994605226505,4.23550654132665));
#161497=CARTESIAN_POINT('Origin',(-0.144684598915065,0.946416036811265,
-0.125405476138852));
#161498=CARTESIAN_POINT('',(6.15191556712846,0.809946053334099,4.0657023142925));
#161499=CARTESIAN_POINT('Origin',(2.28983498828939E-13,0.901573518000056,
2.2291196666302E-13));
#161500=CARTESIAN_POINT('Origin',(-0.158721396605581,0.803569456127978,
-0.109853265678252));
#161501=CARTESIAN_POINT('Origin',(-0.121369578731334,0.946349488399566,
-0.143115011248638));
#161502=CARTESIAN_POINT('Ctrl Pts',(6.114284746,0.809946053,3.895898106));
#161503=CARTESIAN_POINT('Ctrl Pts',(6.326781397,0.875601501000001,3.562402465));
#161504=CARTESIAN_POINT('Ctrl Pts',(6.501745184,0.940829639,3.207773304));
#161505=CARTESIAN_POINT('Ctrl Pts',(6.453893166,0.809946053,3.820636465));
#161506=CARTESIAN_POINT('Ctrl Pts',(6.66228477,0.875601501000001,3.468617329));
#161507=CARTESIAN_POINT('Ctrl Pts',(6.831153176,0.940829639,3.096021041));
#161508=CARTESIAN_POINT('',(6.45389317097018,0.809946052117965,3.82063645379648));
#161509=CARTESIAN_POINT('',(6.7235445095841,0.900669500649203,3.32324378054198));
#161510=CARTESIAN_POINT('Origin',(-0.165202437510702,0.803573330537153,
-0.0989974117660164));
#161511=CARTESIAN_POINT('Ctrl Pts',(6.49966323789617,0.940053944386922,
3.21198972494361));
#161512=CARTESIAN_POINT('Ctrl Pts',(6.53690445380191,0.933168237977147,
3.23054330668388));
#161513=CARTESIAN_POINT('Ctrl Pts',(6.57420251069174,0.9264484489006,3.24909996787951));
#161514=CARTESIAN_POINT('Ctrl Pts',(6.64881815322706,0.913330774524643,
3.28617746825447));
#161515=CARTESIAN_POINT('Ctrl Pts',(6.68617749184471,0.906925555326163,
3.3047190514635));
#161516=CARTESIAN_POINT('Ctrl Pts',(6.72354450877726,0.900669500649855,
3.3232437821697));
#161517=CARTESIAN_POINT('',(6.28408896547809,0.809946050062004,3.85826727006272));
#161518=CARTESIAN_POINT('Origin',(-5.95443833129039E-12,0.714028548,-2.89200087488783E-12));
#161519=CARTESIAN_POINT('',(6.80700121913307,0.749999998604196,3.14876707365042));
#161520=CARTESIAN_POINT('',(6.69322715423015,0.714243089177093,3.30388183145284));
#161521=CARTESIAN_POINT('Origin',(0.661978250407972,0.47361279085057,-1.29881298243699));
#161522=CARTESIAN_POINT('',(6.63778745394538,0.749999999337654,3.49138621564948));
#161523=CARTESIAN_POINT('Origin',(0.,0.749999998746365,0.));
#161524=CARTESIAN_POINT('Origin',(-0.837356842110112,0.692075333990243,
1.18688780490404));
#161525=CARTESIAN_POINT('Ctrl Pts',(6.49757176,0.940837228,3.216218467));
#161526=CARTESIAN_POINT('Ctrl Pts',(6.672999573,0.875180297,2.861810077));
#161527=CARTESIAN_POINT('Ctrl Pts',(6.808839097,0.809946053,2.49042369));
#161528=CARTESIAN_POINT('Ctrl Pts',(6.81353722819479,0.807689868439873,
2.47757896028733));
#161529=CARTESIAN_POINT('Ctrl Pts',(6.81823535938943,0.805433683879746,
2.46473423057468));
#161530=CARTESIAN_POINT('Ctrl Pts',(6.60912646082343,0.940837228000001,
3.5464538510459));
#161531=CARTESIAN_POINT('Ctrl Pts',(6.80256687881479,0.875180297,3.18596073830997));
#161532=CARTESIAN_POINT('Ctrl Pts',(6.9556503352614,0.809946053,2.80656656936472));
#161533=CARTESIAN_POINT('Ctrl Pts',(6.96094486325265,0.807689868439873,
2.79344488336533));
#161534=CARTESIAN_POINT('Ctrl Pts',(6.96623939124391,0.805433683879747,
2.78032319736588));
#161535=CARTESIAN_POINT('',(6.95534695426759,0.809946052265058,2.80591323721172));
#161536=CARTESIAN_POINT('Origin',(-0.168260697371486,0.946416079492337,
-0.0913707898677996));
#161537=CARTESIAN_POINT('',(6.88209301623501,0.809946053334099,2.64816845608985));
#161538=CARTESIAN_POINT('Origin',(4.74880551548651E-13,0.901573518000028,
1.86049092798513E-13));
#161539=CARTESIAN_POINT('Origin',(-0.178625726215517,0.803569088508976,
-0.0731646177719986));
#161540=CARTESIAN_POINT('Origin',(-0.149297058360928,0.946349510647673,
-0.113677938552454));
#161541=CARTESIAN_POINT('Ctrl Pts',(6.808839097,0.809946053,2.49042369));
#161542=CARTESIAN_POINT('Ctrl Pts',(6.94467599,0.875601501000001,2.119044493));
#161543=CARTESIAN_POINT('Ctrl Pts',(7.039314433,0.940829639,1.735094322));
#161544=CARTESIAN_POINT('Ctrl Pts',(7.124328633,0.809946053,2.343915853));
#161545=CARTESIAN_POINT('Ctrl Pts',(7.252174449,0.875601501000001,1.955328694));
#161546=CARTESIAN_POINT('Ctrl Pts',(7.336997617,0.940829639,1.555141784));
#161547=CARTESIAN_POINT('',(7.12432863543045,0.809946052007898,2.34391584102206));
#161548=CARTESIAN_POINT('',(7.28075095350219,0.900669500656451,1.80018486554858));
#161549=CARTESIAN_POINT('Origin',(-0.182621433654452,0.803573323859441,
-0.0611692180826484));
#161550=CARTESIAN_POINT('Ctrl Pts',(7.03818756905568,0.940053944125792,
1.73965972261936));
#161551=CARTESIAN_POINT('Ctrl Pts',(7.07854657807296,0.93316823769528,1.7497737714771));
#161552=CARTESIAN_POINT('Ctrl Pts',(7.11896175957167,0.926448448847887,
1.75987860830767));
#161553=CARTESIAN_POINT('Ctrl Pts',(7.19980349681002,0.913330774458309,
1.78004910006589));
#161554=CARTESIAN_POINT('Ctrl Pts',(7.24027528686602,0.906925555320786,
1.79012603792324));
#161555=CARTESIAN_POINT('Ctrl Pts',(7.28075095320631,0.900669500656858,
1.80018486673939));
#161556=CARTESIAN_POINT('',(6.96658387093794,0.809946050062004,2.41716975438613));
#161557=CARTESIAN_POINT('Origin',(1.87913920535188E-12,0.714028547999755,
3.01625044385467E-13));
#161558=CARTESIAN_POINT('',(7.32474915823918,0.749999999442343,1.61184659974827));
#161559=CARTESIAN_POINT('',(7.24698015457827,0.714243089244742,1.78779292270851));
#161560=CARTESIAN_POINT('Origin',(0.367293486184526,0.473617512480871,-1.41075299706784));
#161561=CARTESIAN_POINT('',(7.23314450366846,0.750000000163903,1.98283145817019));
#161562=CARTESIAN_POINT('Origin',(0.,0.750000000000029,0.));
#161563=CARTESIAN_POINT('Origin',(-0.56263078148524,0.692074923964662,1.33914628784326));
#161564=CARTESIAN_POINT('Ctrl Pts',(7.037054042,0.940837228,1.744239205));
#161565=CARTESIAN_POINT('Ctrl Pts',(7.132193124,0.875180297,1.360404892));
#161566=CARTESIAN_POINT('Ctrl Pts',(7.185019699,0.809946053,0.96849983));
#161567=CARTESIAN_POINT('Ctrl Pts',(7.18684675325495,0.807689868436296,
0.95494544357495));
#161568=CARTESIAN_POINT('Ctrl Pts',(7.1886738075099,0.805433683872588,0.941391057149892));
#161569=CARTESIAN_POINT('Ctrl Pts',(7.21699150217313,0.940837228,2.04277290609919));
#161570=CARTESIAN_POINT('Ctrl Pts',(7.32841402766577,0.875180297,1.64912395008058));
#161571=CARTESIAN_POINT('Ctrl Pts',(7.39635994642072,0.809946053,1.24569138825861));
#161572=CARTESIAN_POINT('Ctrl Pts',(7.39870991667655,0.807689868436296,
1.23173831296156));
#161573=CARTESIAN_POINT('Ctrl Pts',(7.40105988693226,0.805433683872588,
1.21778523766448));
#161574=CARTESIAN_POINT('',(7.39592321120424,0.809946052265051,1.2451185486005));
#161575=CARTESIAN_POINT('Origin',(-0.183968858291761,0.946416066937409,
-0.0530635107189836));
#161576=CARTESIAN_POINT('',(7.2904714443072,0.809946053334099,1.10680918397649));
#161577=CARTESIAN_POINT('Origin',(-5.77229236631283E-13,0.901573518000083,
-6.7762635780344E-14));
#161578=CARTESIAN_POINT('Origin',(-0.190178238047356,0.80356947493056,-0.0330548264754186));
#161579=CARTESIAN_POINT('Origin',(-0.170244477781741,0.946349173716153,
-0.0789258546339719));
#161580=CARTESIAN_POINT('Ctrl Pts',(7.18501969900001,0.809946053,0.96849983));
#161581=CARTESIAN_POINT('Ctrl Pts',(7.237845252,0.875601501000001,0.576602356));
#161582=CARTESIAN_POINT('Ctrl Pts',(7.247733164,0.940829639,0.181284259));
#161583=CARTESIAN_POINT('Ctrl Pts',(7.461638412,0.809946053,0.75759634));
#161584=CARTESIAN_POINT('Ctrl Pts',(7.50296051,0.875601501000001,0.350611062));
#161585=CARTESIAN_POINT('Ctrl Pts',(7.499772204,0.940829639,-0.058454175));
#161586=CARTESIAN_POINT('Ctrl Pts',(7.24761407171315,0.940053944099865,
0.185985165651885));
#161587=CARTESIAN_POINT('Ctrl Pts',(7.28920373107082,0.933168237642109,
0.187186759575636));
#161588=CARTESIAN_POINT('Ctrl Pts',(7.33084626931037,0.926448448776613,
0.188367281414812));
#161589=CARTESIAN_POINT('Ctrl Pts',(7.41413403095609,0.913330774393281,
0.1906876141421));
#161590=CARTESIAN_POINT('Ctrl Pts',(7.45582585695214,0.906925555228153,
0.191828720139254));
#161591=CARTESIAN_POINT('Ctrl Pts',(7.4975175753614,0.900669500590605,0.192951307209456));
#161592=CARTESIAN_POINT('',(7.32332905762014,0.809946050062004,0.863048067009758));
#161593=CARTESIAN_POINT('Origin',(4.06966127464159E-12,0.714028547998533,
5.3952271795131E-13));
#161594=CARTESIAN_POINT('',(7.46187241744399,0.7142430893127,0.188108803996591));
#161595=CARTESIAN_POINT('Origin',(0.0554340383527208,0.473613023976932,
-1.4567289021525));
#161596=CARTESIAN_POINT('Origin',(-0.261598757446677,0.692074811532284,
1.42878662012929));
#161597=CARTESIAN_POINT('Ctrl Pts',(7.24749149900001,0.940837228,0.190701257));
#161598=CARTESIAN_POINT('Ctrl Pts',(7.25789325,0.875180297,-0.204611314));
#161599=CARTESIAN_POINT('Ctrl Pts',(7.225236766,0.809946053,-0.598710006));
#161600=CARTESIAN_POINT('Ctrl Pts',(7.22474524731287,0.808964200515023,
-0.604641657174902));
#161601=CARTESIAN_POINT('Ctrl Pts',(7.22425372862578,0.807982348030045,
-0.610573308349804));
#161602=CARTESIAN_POINT('Ctrl Pts',(7.48711801034727,0.940837228000001,
0.443279003673952));
#161603=CARTESIAN_POINT('Ctrl Pts',(7.51129655000436,0.875180297,0.0348960660811571));
#161604=CARTESIAN_POINT('Ctrl Pts',(7.49091351204778,0.809946053,-0.37369389589682));
#161605=CARTESIAN_POINT('Ctrl Pts',(7.49060672323194,0.808964200515023,
-0.379843657814883));
#161606=CARTESIAN_POINT('Ctrl Pts',(7.49029993441611,0.807982348030045,
-0.385993419732945));
#161607=CARTESIAN_POINT('',(7.35795553086503,0.809946053334099,-0.486303255542236));
#161608=CARTESIAN_POINT('Ctrl Pts',(7.225236766,0.809946053,-0.598710006));
#161609=CARTESIAN_POINT('Ctrl Pts',(7.192580914,0.875601501000001,-0.992801067));
#161610=CARTESIAN_POINT('Ctrl Pts',(7.11725594700001,0.940829639,-1.381002455));
#161611=CARTESIAN_POINT('Ctrl Pts',(7.450050271,0.809946053,-0.864147535));
#161612=CARTESIAN_POINT('Ctrl Pts',(7.402916477,0.875601501000001,-1.270500754));
#161613=CARTESIAN_POINT('Ctrl Pts',(7.311865778,0.940829639,-1.669316881));
#161614=CARTESIAN_POINT('',(7.45005026817131,0.809946052007895,-0.864147546869791));
#161615=CARTESIAN_POINT('',(7.36370860794726,0.900669500577546,-1.42330444245839));
#161616=CARTESIAN_POINT('Origin',(-0.191427337976096,0.803573322522903,
0.0211651271455665));
#161617=CARTESIAN_POINT('Ctrl Pts',(7.11815019508415,0.940053944176777,
-1.37638585233793));
#161618=CARTESIAN_POINT('Ctrl Pts',(7.15902581858686,0.933168237674186,
-1.38415289816254));
#161619=CARTESIAN_POINT('Ctrl Pts',(7.19994855461074,0.926448448807835,
-1.3919518908494));
#161620=CARTESIAN_POINT('Ctrl Pts',(7.28178789774418,0.913330774380453,
-1.40759021277047));
#161621=CARTESIAN_POINT('Ctrl Pts',(7.32275029601023,0.906925555220636,
-1.41543829529631));
#161622=CARTESIAN_POINT('Ctrl Pts',(7.36370860828366,0.900669500578175,
-1.42330444070726));
#161623=CARTESIAN_POINT('',(7.3376435167032,0.809946050062004,-0.731428788525407));
#161624=CARTESIAN_POINT('Origin',(1.30971622436249E-13,0.714028547998533,
8.56519716263548E-15));
#161625=CARTESIAN_POINT('',(7.32455911184973,0.749999999450591,-1.61270998931781));
#161626=CARTESIAN_POINT('',(7.32785581902563,0.714243089095246,-1.42037107428952));
#161627=CARTESIAN_POINT('Origin',(-0.259012497022776,0.473616870185757,
-1.43458741474906));
#161628=CARTESIAN_POINT('',(7.3971934782476,0.750000000283857,-1.23754945340732));
#161629=CARTESIAN_POINT('Origin',(0.,0.750000000000029,0.));
#161630=CARTESIAN_POINT('Origin',(0.0516617329994917,0.69207504842183,1.45161927898567));
#161631=CARTESIAN_POINT('Ctrl Pts',(7.11904430900001,0.940837228,-1.371753671));
#161632=CARTESIAN_POINT('Ctrl Pts',(7.044222355,0.875180297,-1.760060122));
#161633=CARTESIAN_POINT('Ctrl Pts',(6.927609792,0.809946053,-2.137924827));
#161634=CARTESIAN_POINT('Ctrl Pts',(6.92357664226118,0.807689868354167,
-2.15099361562003));
#161635=CARTESIAN_POINT('Ctrl Pts',(6.91954349252227,0.805433683708332,
-2.16406240424011));
#161636=CARTESIAN_POINT('Ctrl Pts',(7.40770217163526,0.940837228000001,
-1.17636559945699));
#161637=CARTESIAN_POINT('Ctrl Pts',(7.34353761128978,0.875180297,-1.58041682072448));
#161638=CARTESIAN_POINT('Ctrl Pts',(7.23580672022365,0.809946053,-1.97509204848454));
#161639=CARTESIAN_POINT('Ctrl Pts',(7.23208075104854,0.807689868354167,
-1.98874224406225));
#161640=CARTESIAN_POINT('Ctrl Pts',(7.2283547818734,0.80543368370833,-2.00239243963988));
#161641=CARTESIAN_POINT('',(7.23516982194198,0.809946052264276,-1.97542856151036));
#161642=CARTESIAN_POINT('Origin',(-0.18924613883507,0.946416062892984,0.0290873232071368));
#161643=CARTESIAN_POINT('',(7.08138979442916,0.809946053334099,-2.05667669546547));
#161644=CARTESIAN_POINT('Origin',(1.14708589848966E-12,0.901573517999861,
-2.58528008029169E-13));
#161645=CARTESIAN_POINT('Origin',(-0.186480273030153,0.803569488776888,
0.0498539794532992));
#161646=CARTESIAN_POINT('Origin',(-0.187649829682202,0.946349141882412,
-0.000147355372646651));
#161647=CARTESIAN_POINT('Ctrl Pts',(6.927609792,0.809946053,-2.137924827));
#161648=CARTESIAN_POINT('Ctrl Pts',(6.810999487,0.875601501,-2.515782215));
#161649=CARTESIAN_POINT('Ctrl Pts',(6.653983753,0.940829639,-2.87871503));
#161650=CARTESIAN_POINT('Ctrl Pts',(7.090106059,0.809946053,-2.445484832));
#161651=CARTESIAN_POINT('Ctrl Pts',(6.956720297,0.875601501,-2.832205366));
#161652=CARTESIAN_POINT('Ctrl Pts',(6.782064634,0.940829639,-3.202124185));
#161653=CARTESIAN_POINT('',(7.09010605367899,0.809946052117973,-2.44548484305816));
#161654=CARTESIAN_POINT('',(6.88558080984488,0.900669500611653,-2.97300805691043));
#161655=CARTESIAN_POINT('Origin',(-0.182401896597097,0.803573307003854,
0.0618214724472022));
#161656=CARTESIAN_POINT('Ctrl Pts',(6.65584952666731,0.940053944150437,
-2.87439859628003));
#161657=CARTESIAN_POINT('Ctrl Pts',(6.6940998150624,0.933168237732746,-2.89077110380397));
#161658=CARTESIAN_POINT('Ctrl Pts',(6.73238924787852,0.926448448773642,
-2.90718493942895));
#161659=CARTESIAN_POINT('Ctrl Pts',(6.80895345513282,0.913330774434679,
-2.94005068584498));
#161660=CARTESIAN_POINT('Ctrl Pts',(6.84727106960049,0.906925555258089,
-2.95652098951638));
#161661=CARTESIAN_POINT('Ctrl Pts',(6.88558081045313,0.900669500624169,
-2.97300805529551));
#161662=CARTESIAN_POINT('',(7.00885791987027,0.809946050062004,-2.29170484671772));
#161663=CARTESIAN_POINT('Origin',(1.46397650946373E-11,0.714028547998777,
-6.56484415439973E-12));
#161664=CARTESIAN_POINT('',(6.80663001399836,0.749999999460468,-3.14956942225839));
#161665=CARTESIAN_POINT('',(6.85119682732554,0.7142430892164,-2.96243597874438));
#161666=CARTESIAN_POINT('Origin',(-0.561351999888413,0.473617915787033,
-1.34536704192595));
#161667=CARTESIAN_POINT('',(6.95821465439766,0.750000000203561,-2.79879417363605));
#161668=CARTESIAN_POINT('Origin',(0.,0.750000000000029,0.));
#161669=CARTESIAN_POINT('Origin',(0.362509541410632,0.692075069548214,1.40657521275727));
#161670=CARTESIAN_POINT('Ctrl Pts',(6.657718518,0.940837228,-2.870066921));
#161671=CARTESIAN_POINT('Ctrl Pts',(6.501171452,0.875180297,-3.233210475));
#161672=CARTESIAN_POINT('Ctrl Pts',(6.306055484,0.809946053,-3.577172659));
#161673=CARTESIAN_POINT('Ctrl Pts',(6.2993072239509,0.807689868397938,-3.5890688983928));
#161674=CARTESIAN_POINT('Ctrl Pts',(6.29255896390185,0.805433683795875,
-3.60096513778561));
#161675=CARTESIAN_POINT('Ctrl Pts',(6.98163038081954,0.940837228000001,
-2.74129982289584));
#161676=CARTESIAN_POINT('Ctrl Pts',(6.83210688278068,0.875180297,-3.12211106708423));
#161677=CARTESIAN_POINT('Ctrl Pts',(6.6420511733511,0.809946053,-3.48440004939066));
#161678=CARTESIAN_POINT('Ctrl Pts',(6.63547792686494,0.807689868397938,
-3.4969301374741));
#161679=CARTESIAN_POINT('Ctrl Pts',(6.62890468037882,0.805433683795875,
-3.50946022555754));
#161680=CARTESIAN_POINT('',(6.6413568236661,0.80994605226505,-3.48459178218603));
#161681=CARTESIAN_POINT('Origin',(-0.178568867614937,0.946416037059252,
0.0690896628819765));
#161682=CARTESIAN_POINT('',(6.47370614201999,0.809946053334099,-3.53088221829681));
#161683=CARTESIAN_POINT('Origin',(-1.32836450172924E-12,0.901573518000083,
6.05635333550403E-13));
#161684=CARTESIAN_POINT('Origin',(-0.171403251577942,0.803569519200059,
0.0887761307562095));
#161685=CARTESIAN_POINT('Origin',(-0.183294010153269,0.946349438276496,
0.0401950578583943));
#161686=CARTESIAN_POINT('Ctrl Pts',(6.306055484,0.809946053,-3.577172659));
#161687=CARTESIAN_POINT('Ctrl Pts',(6.110943294,0.875601501000001,-3.921128183));
#161688=CARTESIAN_POINT('Ctrl Pts',(5.879578673,0.940829639,-4.241822088));
#161689=CARTESIAN_POINT('Ctrl Pts',(6.398636369,0.809946053,-3.912473977));
#161690=CARTESIAN_POINT('Ctrl Pts',(6.185235608,0.875601501,-4.261479203));
#161691=CARTESIAN_POINT('Ctrl Pts',(5.935141687,0.940829639,-4.585203721));
#161692=CARTESIAN_POINT('',(6.39863636144931,0.809946052007894,-3.91247398658227));
#161693=CARTESIAN_POINT('',(6.0854909065751,0.900669500598591,-4.38369711823371));
#161694=CARTESIAN_POINT('Origin',(-0.164847907856605,0.80357330245582,0.0995873118686996));
#161695=CARTESIAN_POINT('Ctrl Pts',(5.8823287320493,0.940053944089694,-4.23800765756635));
#161696=CARTESIAN_POINT('Ctrl Pts',(5.9161651452579,0.933168237624726,-4.26222006634371));
#161697=CARTESIAN_POINT('Ctrl Pts',(5.95003090244124,0.926448448791528,
-4.2864812512914));
#161698=CARTESIAN_POINT('Ctrl Pts',(6.01773991754674,0.913330774397287,
-4.33503765619876));
#161699=CARTESIAN_POINT('Ctrl Pts',(6.05162105897944,0.906925555238692,
-4.35936004763431));
#161700=CARTESIAN_POINT('Ctrl Pts',(6.08549090761331,0.900669500599227,
-4.383697116789));
#161701=CARTESIAN_POINT('',(6.35234591730059,0.809946050062004,-3.74482333360496));
#161702=CARTESIAN_POINT('Origin',(8.25164589435268E-12,0.714028547998533,
-6.10449191196238E-12));
#161703=CARTESIAN_POINT('',(5.97043046128455,0.749999999462928,-4.53915849030982));
#161704=CARTESIAN_POINT('',(6.05418348661255,0.714243089235877,-4.36598066940676));
#161705=CARTESIAN_POINT('Origin',(-0.837442198376062,0.473618072624967,
-1.19323890730608));
#161706=CARTESIAN_POINT('',(6.19387744755386,0.750000000332207,-4.22917038787356));
#161707=CARTESIAN_POINT('Origin',(0.,0.750000000000029,0.));
#161708=CARTESIAN_POINT('Origin',(0.656406169991699,0.692075080705617,1.29576162756753));
#161709=CARTESIAN_POINT('Ctrl Pts',(5.88508521,0.940837228,-4.234179032));
#161710=CARTESIAN_POINT('Ctrl Pts',(5.65413299700001,0.875180297,-4.5551795));
#161711=CARTESIAN_POINT('Ctrl Pts',(5.38963702999999,0.809946053,-4.849155874));
#161712=CARTESIAN_POINT('Ctrl Pts',(5.38048920064803,0.807689868382952,
-4.85932330956951));
#161713=CARTESIAN_POINT('Ctrl Pts',(5.37134137129619,0.805433683765901,
-4.86949074513889));
#161714=CARTESIAN_POINT('Ctrl Pts',(6.2291053126719,0.940837228,-4.17805391238279));
#161715=CARTESIAN_POINT('Ctrl Pts',(6.00121443024192,0.875180297,-4.51781886922421));
#161716=CARTESIAN_POINT('Ctrl Pts',(5.73772069546297,0.809946053,-4.83078137711905));
#161717=CARTESIAN_POINT('Ctrl Pts',(5.7286075292079,0.807689868382952,-4.84160546509385));
#161718=CARTESIAN_POINT('Ctrl Pts',(5.7194943629528,0.805433683765901,-4.85242955306867));
#161719=CARTESIAN_POINT('',(5.73700136409408,0.809946052264276,-4.83081936142431));
#161720=CARTESIAN_POINT('Origin',(-0.159541768734545,0.946416043065824,
0.105861393742597));
#161721=CARTESIAN_POINT('',(5.56331918515664,0.809946053334099,-4.83998761354413));
#161722=CARTESIAN_POINT('Origin',(1.38777878078145E-14,0.901573518000056,
-3.03576608295941E-15));
#161723=CARTESIAN_POINT('Origin',(-0.14831164317236,0.803569412242196,0.1235471652116));
#161724=CARTESIAN_POINT('Origin',(-0.170368230555993,0.94634918625941,0.0786583648630335));
#161725=CARTESIAN_POINT('Ctrl Pts',(5.38963703,0.809946053,-4.849155874));
#161726=CARTESIAN_POINT('Ctrl Pts',(5.125146184,0.875601501000001,-5.143126555));
#161727=CARTESIAN_POINT('Ctrl Pts',(4.830251029,0.940829639,-5.406586261));
#161728=CARTESIAN_POINT('Ctrl Pts',(5.407973553,0.809946053,-5.196520186));
#161729=CARTESIAN_POINT('Ctrl Pts',(5.124536177,0.875601501000001,-5.491491009));
#161730=CARTESIAN_POINT('Ctrl Pts',(4.81069811,0.940829639,-5.753884227));
#161731=CARTESIAN_POINT('',(5.40797354355034,0.8099460520079,-5.19652019377016));
#161732=CARTESIAN_POINT('',(5.00085021158662,0.900669500636843,-5.58940937485491));
#161733=CARTESIAN_POINT('Origin',(-0.13958530168794,0.803573298460263,0.132696195845124));
#161734=CARTESIAN_POINT('Ctrl Pts',(4.83375678258189,0.940053944205177,
-5.40345218965847));
#161735=CARTESIAN_POINT('Ctrl Pts',(4.8615971667985,0.933168237817763,-5.43437235426476));
#161736=CARTESIAN_POINT('Ctrl Pts',(4.88945572450934,0.926448448826654,
-5.46534646379243));
#161737=CARTESIAN_POINT('Ctrl Pts',(4.94514354866678,0.913330774481685,
-5.5273230837034));
#161738=CARTESIAN_POINT('Ctrl Pts',(4.97300397282262,0.906925555301418,
-5.55836027520916));
#161739=CARTESIAN_POINT('Ctrl Pts',(5.00085021292921,0.900669500637492,
-5.58940937365095));
#161740=CARTESIAN_POINT('',(5.39880527916107,0.809946050062004,-5.02283804326252));
#161741=CARTESIAN_POINT('Origin',(1.91383367487141E-12,0.714028548001467,
-1.57773100140091E-12));
#161742=CARTESIAN_POINT('',(4.85506021197657,0.750000000749204,-5.71650155683177));
#161743=CARTESIAN_POINT('',(4.97408325374587,0.714243089138568,-5.5653769574538));
#161744=CARTESIAN_POINT('Origin',(-1.0743706025104,0.473612770293792,-0.985320519253279));
#161745=CARTESIAN_POINT('',(5.13992141815109,0.750000001354628,-5.46179529301488));
#161746=CARTESIAN_POINT('Origin',(0.,0.750000002055273,0.));
#161747=CARTESIAN_POINT('Origin',(0.91961459177966,0.692074279456245,1.12435267143665));
#161748=CARTESIAN_POINT('Ctrl Pts',(4.837271857,0.940837228,-5.400305637));
#161749=CARTESIAN_POINT('Ctrl Pts',(4.54271356700001,0.875180297,-5.664153394));
#161750=CARTESIAN_POINT('Ctrl Pts',(4.221205138,0.809946053,-5.894397949));
#161751=CARTESIAN_POINT('Ctrl Pts',(4.21008548164904,0.807689868371028,
-5.9023611627056));
#161752=CARTESIAN_POINT('Ctrl Pts',(4.19896582529809,0.805433683742054,
-5.9103243764113));
#161753=CARTESIAN_POINT('Ctrl Pts',(5.1853142030758,0.940837228000001,-5.41944684537321));
#161754=CARTESIAN_POINT('Ctrl Pts',(4.8897118604283,0.875180297,-5.70227848261083));
#161755=CARTESIAN_POINT('Ctrl Pts',(4.56510077445277,0.809946053,-5.95128073642013));
#161756=CARTESIAN_POINT('Ctrl Pts',(4.55387380993742,0.807689868371028,
-5.9598927019029));
#161757=CARTESIAN_POINT('Ctrl Pts',(4.54264684542219,0.805433683742056,
-5.96850466738573));
#161758=CARTESIAN_POINT('',(4.56439009325036,0.809946052265046,-5.95116319851744));
#161759=CARTESIAN_POINT('Origin',(-0.133054682399875,0.946416046548661,
0.137683166548233));
#161760=CARTESIAN_POINT('',(4.39279760585611,0.809946053334099,-5.92278056671925));
#161761=CARTESIAN_POINT('Origin',(-2.0643209364124E-13,0.901573518000139,
2.51534904016637E-13));
#161762=CARTESIAN_POINT('Origin',(-0.118285670479293,0.803569491232197,
0.152541959866282));
#161763=CARTESIAN_POINT('Origin',(-0.14947577587879,0.946349162772959,0.113443387801616));
#161764=CARTESIAN_POINT('Ctrl Pts',(4.221205138,0.809946053,-5.894397949));
#161765=CARTESIAN_POINT('Ctrl Pts',(3.899702935,0.875601501000001,-6.124638046));
#161766=CARTESIAN_POINT('Ctrl Pts',(3.555066216,0.940829639,-6.318544469));
#161767=CARTESIAN_POINT('Ctrl Pts',(4.164439905,0.809946053,-6.237582888));
#161768=CARTESIAN_POINT('Ctrl Pts',(3.824219129,0.875601501000001,-6.464726799));
#161769=CARTESIAN_POINT('Ctrl Pts',(3.461311636,0.940829639,-6.653519501));
#161770=CARTESIAN_POINT('',(4.16443989410765,0.809946052117949,-6.23758289353459));
#161771=CARTESIAN_POINT('',(3.68237531859818,0.900669500629599,-6.53376706126185));
#161772=CARTESIAN_POINT('Origin',(-0.107796101370615,0.803573316163276,
0.159600559105972));
#161773=CARTESIAN_POINT('Ctrl Pts',(3.55916373987558,0.940053944136155,
-6.31623730438967));
#161774=CARTESIAN_POINT('Ctrl Pts',(3.57970630987706,0.933168237731745,
-6.35241943241517));
#161775=CARTESIAN_POINT('Ctrl Pts',(3.60025503167879,0.926448448810044,
-6.38865815044762));
#161776=CARTESIAN_POINT('Ctrl Pts',(3.64131776395972,0.913330774465002,
-6.46115702738743));
#161777=CARTESIAN_POINT('Ctrl Pts',(3.66185474806907,0.906925555285222,
-6.49745775420293));
#161778=CARTESIAN_POINT('Ctrl Pts',(3.68237532006268,0.900669500643497,
-6.53376706033201));
#161779=CARTESIAN_POINT('',(4.1928225065985,0.809946050062004,-6.06599042879995));
#161780=CARTESIAN_POINT('Origin',(1.32012456521835E-12,0.714028548,-2.06258621293642E-12));
#161781=CARTESIAN_POINT('',(3.51267275150287,0.749999999475252,-6.62654735398287));
#161782=CARTESIAN_POINT('',(3.66140041731029,0.714243089203531,-6.50454240349333));
#161783=CARTESIAN_POINT('Origin',(-1.26107012722738,0.473618310017934,-0.731321202018131));
#161784=CARTESIAN_POINT('',(3.84562836831758,0.750000000182253,-6.43903272670087));
#161785=CARTESIAN_POINT('Origin',(0.,0.750000000000029,0.));
#161786=CARTESIAN_POINT('Origin',(1.13981441991433,0.692074972328244,0.900383294543275));
#161787=CARTESIAN_POINT('Ctrl Pts',(3.563273049,0.940837228,-6.313919953));
#161788=CARTESIAN_POINT('Ctrl Pts',(3.2188819,0.875180297,-6.508277771));
#161789=CARTESIAN_POINT('Ctrl Pts',(2.855394386,0.809946053,-6.664024527));
#161790=CARTESIAN_POINT('Ctrl Pts',(2.84282284542823,0.807689868362209,
-6.6694111677691));
#161791=CARTESIAN_POINT('Ctrl Pts',(2.83025130485638,0.805433683724415,
-6.67479780853829));
#161792=CARTESIAN_POINT('Ctrl Pts',(3.89906356434784,0.940837228,-6.40743246670405));
#161793=CARTESIAN_POINT('Ctrl Pts',(3.54957179937433,0.875180297,-6.62010589188342));
#161794=CARTESIAN_POINT('Ctrl Pts',(3.17902181501696,0.809946053,-6.7935048240109));
#161795=CARTESIAN_POINT('Ctrl Pts',(3.16620601259514,0.807689868362209,
-6.79950198106963));
#161796=CARTESIAN_POINT('Ctrl Pts',(3.15339021017337,0.805433683724414,
-6.80549913812837));
#161797=CARTESIAN_POINT('',(3.17835301629486,0.809946052265058,-6.79323725863071));
#161798=CARTESIAN_POINT('Origin',(-0.100346118795918,0.946416093894335,
0.163066990765337));
#161799=CARTESIAN_POINT('',(3.01687369313244,0.809946053334099,-6.72863088383735));
#161800=CARTESIAN_POINT('Origin',(5.75277672720809E-13,0.901573517999806,
-9.22872889219661E-13));
#161801=CARTESIAN_POINT('Origin',(-0.0827278906056161,0.803569457020606,
0.174402821713849));
#161802=CARTESIAN_POINT('Origin',(-0.121594340985359,0.946349478271723,
0.14292426058979));
#161803=CARTESIAN_POINT('Ctrl Pts',(2.855394386,0.809946053,-6.664024527));
#161804=CARTESIAN_POINT('Ctrl Pts',(2.491913911,0.875601501000001,-6.819768268));
#161805=CARTESIAN_POINT('Ctrl Pts',(2.113650457,0.940829639,-6.93505456));
#161806=CARTESIAN_POINT('Ctrl Pts',(2.726181675,0.809946053,-6.986983146));
#161807=CARTESIAN_POINT('Ctrl Pts',(2.345085845,0.875601501,-7.135679149));
#161808=CARTESIAN_POINT('Ctrl Pts',(1.950078078,0.940829639,-7.24204359900001));
#161809=CARTESIAN_POINT('',(2.7261816631742,0.80994605211795,-6.98698314906222));
#161810=CARTESIAN_POINT('',(2.19171664906142,0.900669500617564,-7.1726130614454));
#161811=CARTESIAN_POINT('Origin',(-0.0709664804698285,0.803573343433978,
0.179042142867073));
#161812=CARTESIAN_POINT('Ctrl Pts',(2.11814815554889,0.940053944109833,
-6.9336821817921));
#161813=CARTESIAN_POINT('Ctrl Pts',(2.13043236392346,0.933168237714838,
-6.97343443708677));
#161814=CARTESIAN_POINT('Ctrl Pts',(2.14271041508717,0.926448448760565,
-7.01324328206604));
#161815=CARTESIAN_POINT('Ctrl Pts',(2.16722800824216,0.913330774417522,
-7.09287444931125));
#161816=CARTESIAN_POINT('Ctrl Pts',(2.17948126585138,0.906925555270505,
-7.13274132967918));
#161817=CARTESIAN_POINT('Ctrl Pts',(2.19171665080781,0.900669500618194,
-7.17261306090959));
#161818=CARTESIAN_POINT('',(2.7907880137327,0.809946050062004,-6.82550384335576));
#161819=CARTESIAN_POINT('Origin',(4.21732961053412E-12,0.714028547999755,
-1.32797418894715E-11));
#161820=CARTESIAN_POINT('',(2.00603661220003,0.749999999425987,-7.2267431670167));
#161821=CARTESIAN_POINT('',(2.17751456677922,0.714243089251923,-7.13956267616647));
#161822=CARTESIAN_POINT('Origin',(-1.3887988617426,0.473616821962798,-0.443132249548737));
#161823=CARTESIAN_POINT('',(2.3715180151596,0.750000000306954,-7.11518814286577));
#161824=CARTESIAN_POINT('Origin',(0.,0.750000000000029,0.));
#161825=CARTESIAN_POINT('Origin',(1.30672170332859,0.692075255289197,0.634308337555363));
#161826=CARTESIAN_POINT('Ctrl Pts',(2.122659554,0.940837228,-6.932302389));
#161827=CARTESIAN_POINT('Ctrl Pts',(1.744538893,0.875180297,-7.04808231200001));
#161828=CARTESIAN_POINT('Ctrl Pts',(1.356068566,0.809946053,-7.122048725));
#161829=CARTESIAN_POINT('Ctrl Pts',(1.34263297247409,0.807689868356189,
-7.12460691951465));
#161830=CARTESIAN_POINT('Ctrl Pts',(1.32919737894819,0.805433683712374,
-7.12716511402929));
#161831=CARTESIAN_POINT('Ctrl Pts',(2.43049704741223,0.940837228,-7.09581366670697));
#161832=CARTESIAN_POINT('Ctrl Pts',(2.04345770499428,0.875180297,-7.2283845069501));
#161833=CARTESIAN_POINT('Ctrl Pts',(1.64429532972229,0.809946053,-7.31807217462003));
#161834=CARTESIAN_POINT('Ctrl Pts',(1.63048994214892,0.807689868356189,
-7.32117410278123));
#161835=CARTESIAN_POINT('Ctrl Pts',(1.61668455457555,0.805433683712374,
-7.32427603094229));
#161836=CARTESIAN_POINT('',(1.64369968581408,0.809946052265051,-7.31766709281447));
#161837=CARTESIAN_POINT('Origin',(-0.0629454776259189,0.946416037296776,
0.180825992163296));
#161838=CARTESIAN_POINT('',(1.49988411999609,0.809946053334099,-7.2198578984163));
#161839=CARTESIAN_POINT('Origin',(-4.83228908276789E-13,0.901573518000167,
1.90602741922952E-12));
#161840=CARTESIAN_POINT('Origin',(-0.0433024034837949,0.803569395438105,
0.188109806131513));
#161841=CARTESIAN_POINT('Origin',(-0.0880268758334116,0.94634945669678,
0.165721505977623));
#161842=CARTESIAN_POINT('Ctrl Pts',(1.356068566,0.809946053,-7.122048725));
#161843=CARTESIAN_POINT('Ctrl Pts',(0.967605761,0.875601501000001,-7.196013706));
#161844=CARTESIAN_POINT('Ctrl Pts',(0.573402753,0.940829639,-7.227289207));
#161845=CARTESIAN_POINT('Ctrl Pts',(1.16045022,0.809946053,-7.409679837));
#161846=CARTESIAN_POINT('Ctrl Pts',(0.756298953000001,0.875601501000001,
-7.47297507200001));
#161847=CARTESIAN_POINT('Ctrl Pts',(0.347661035,0.940829639,-7.491937787));
#161848=CARTESIAN_POINT('',(1.16045020779686,0.809946052007894,-7.40967983745501));
#161849=CARTESIAN_POINT('',(0.598575744401869,0.900669500572252,-7.47607564655911));
#161850=CARTESIAN_POINT('Origin',(-0.0308185621163465,0.803573345307439,
0.190111958624054));
#161851=CARTESIAN_POINT('Ctrl Pts',(0.578090317678941,0.940053944129792,
-7.22691578740449));
#161852=CARTESIAN_POINT('Ctrl Pts',(0.581541768262509,0.933168237656136,
-7.26837939890857));
#161853=CARTESIAN_POINT('Ctrl Pts',(0.584975040441821,0.926448448774479,
-7.30989695258816));
#161854=CARTESIAN_POINT('Ctrl Pts',(0.591801078877184,0.913330774363199,
-7.39293694524516));
#161855=CARTESIAN_POINT('Ctrl Pts',(0.595197661337425,0.906925555221954,
-7.43450584811815));
#161856=CARTESIAN_POINT('Ctrl Pts',(0.598575746205688,0.900669500572879,
-7.47607564641263));
#161857=CARTESIAN_POINT('',(1.25825937515092,0.809946050062004,-7.265864284091));
#161858=CARTESIAN_POINT('Origin',(5.75901088969988E-13,0.714028548000245,
-1.11187101192733E-11));
#161859=CARTESIAN_POINT('',(0.405600432040824,0.74999999933706,-7.48902450137263));
#161860=CARTESIAN_POINT('',(0.5918105554394,0.714243089348684,-7.44074493336252));
#161861=CARTESIAN_POINT('Origin',(-1.45159130690835,0.473612960585341,-0.134218633737058));
#161862=CARTESIAN_POINT('',(0.786518113978562,0.750000000212775,-7.45864526972393));
#161863=CARTESIAN_POINT('Origin',(0.,0.750000000000029,0.));
#161864=CARTESIAN_POINT('Origin',(1.41252863802681,0.69207492570701,0.338569540540863));
#161865=CARTESIAN_POINT('Ctrl Pts',(0.582792857,0.940837228,-7.226538071));
#161866=CARTESIAN_POINT('Ctrl Pts',(0.188623186,0.875180297,-7.25832635800001));
#161867=CARTESIAN_POINT('Ctrl Pts',(-0.206665513,0.809946053,-7.24705384000001));
#161868=CARTESIAN_POINT('Ctrl Pts',(-0.220336925761674,0.807689868398275,
-7.24666396989535));
#161869=CARTESIAN_POINT('Ctrl Pts',(-0.234008338523342,0.805433683796549,
-7.24627409979073));
#161870=CARTESIAN_POINT('Ctrl Pts',(0.848283189422318,0.940837228,-7.45240250622955));
#161871=CARTESIAN_POINT('Ctrl Pts',(0.441793800395535,0.875180297,-7.49867189599113));
#161872=CARTESIAN_POINT('Ctrl Pts',(0.0326834214022629,0.809946053,-7.50045460502665));
#161873=CARTESIAN_POINT('Ctrl Pts',(0.0185339734912782,0.807689868398275,
-7.50051626161112));
#161874=CARTESIAN_POINT('Ctrl Pts',(0.00438452558029279,0.805433683796549,
-7.50057791819554));
#161875=CARTESIAN_POINT('',(0.0321887839317885,0.809946052265054,-7.49993094798273));
#161876=CARTESIAN_POINT('Origin',(-0.0226016246518017,0.946416076947056,
0.190129940226492));
#161877=CARTESIAN_POINT('',(-0.0872383680465476,0.809946053334099,-7.37349238247579));
#161878=CARTESIAN_POINT('Origin',(-1.08545578124744E-13,0.901573518000028,
1.85615411929518E-13));
#161879=CARTESIAN_POINT('Origin',(-0.00185196880873136,0.803569459122582,
0.193020748408552));
#161880=CARTESIAN_POINT('Origin',(-0.0503436538305299,0.946349183241457,
0.180770695181811));
#161881=CARTESIAN_POINT('Ctrl Pts',(-0.206665513,0.809946053,-7.24705384));
#161882=CARTESIAN_POINT('Ctrl Pts',(-0.601946558,0.875601501000001,-7.235781541));
#161883=CARTESIAN_POINT('Ctrl Pts',(-0.993656627,0.940829639,-7.18158384400001));
#161884=CARTESIAN_POINT('Ctrl Pts',(-0.459542598,0.809946053,-7.48590813500001));
#161885=CARTESIAN_POINT('Ctrl Pts',(-0.867851637,0.875601501000001,-7.460842987));
#161886=CARTESIAN_POINT('Ctrl Pts',(-1.271012251,0.940829639,-7.391517291));
#161887=CARTESIAN_POINT('',(-0.459542610028098,0.809946052117958,-7.48590813281646));
#161888=CARTESIAN_POINT('',(-1.0225538965043,0.900669500589206,-7.42996524392277));
#161889=CARTESIAN_POINT('Origin',(0.0107703977697209,0.803573338426796,
0.192292192038651));
#161890=CARTESIAN_POINT('Ctrl Pts',(-0.988998380749854,0.940053944129632,
-7.18222684255033));
#161891=CARTESIAN_POINT('Ctrl Pts',(-0.994541073994604,0.933168237660314,
-7.22346301771727));
#161892=CARTESIAN_POINT('Ctrl Pts',(-1.00011311661772,0.926448448773653,
-7.26474796616579));
#161893=CARTESIAN_POINT('Ctrl Pts',(-1.01129781094299,0.913330774359142,
-7.34731392651569));
#161894=CARTESIAN_POINT('Ctrl Pts',(-1.01691672399893,0.906925555249925,
-7.38864113618631));
#161895=CARTESIAN_POINT('Ctrl Pts',(-1.02255389469136,0.900669500589833,
-7.42996524417017));
#161896=CARTESIAN_POINT('',(-0.333104073596248,0.809946050062004,-7.36648098668171));
#161897=CARTESIAN_POINT('Origin',(4.5102810375397E-14,0.714028548000489,
-7.69349861595714E-13));
#161898=CARTESIAN_POINT('',(-1.21380115554419,0.749999993612532,-7.40112736975039));
#161899=CARTESIAN_POINT('',(-1.02156586106537,0.71424308919482,-7.39400622708004));
#161900=CARTESIAN_POINT('Origin',(-1.44650614712913,0.47361195078468,0.180945298525509));
#161901=CARTESIAN_POINT('',(-0.83525852122216,0.749999995259856,-7.45334442616223));
#161902=CARTESIAN_POINT('Origin',(0.,0.749999992945671,0.));
#161903=CARTESIAN_POINT('Origin',(1.45228896547467,0.692075656665917,0.0270087042234279));
#161904=CARTESIAN_POINT('Ctrl Pts',(-0.984324587,0.940837228,-7.182868863));
#161905=CARTESIAN_POINT('Ctrl Pts',(-1.376112332,0.875180297,-7.12917913000001));
#161906=CARTESIAN_POINT('Ctrl Pts',(-1.759736143,0.809946053,-7.03319477300001));
#161907=CARTESIAN_POINT('Ctrl Pts',(-1.77300411522825,0.807689868391784,
-7.02987506826191));
#161908=CARTESIAN_POINT('Ctrl Pts',(-1.78627208745656,0.805433683783566,
-7.02655536352382));
#161909=CARTESIAN_POINT('Ctrl Pts',(-0.773595447491138,0.940837228,-7.46052528796711));
#161910=CARTESIAN_POINT('Ctrl Pts',(-1.18052789164637,0.875180297000001,
-7.41832972190354));
#161911=CARTESIAN_POINT('Ctrl Pts',(-1.58045672673831,0.809946053,-7.33212411374335));
#161912=CARTESIAN_POINT('Ctrl Pts',(-1.59428862279148,0.807689868391784,
-7.32914261577011));
#161913=CARTESIAN_POINT('Ctrl Pts',(-1.60812051884472,0.805433683783564,
-7.32616111779673));
#161914=CARTESIAN_POINT('',(-1.58082722719252,0.809946052264272,-7.33150636799885));
#161915=CARTESIAN_POINT('Origin',(0.0187991128872561,0.946416066667061,
0.190543491964065));
#161916=CARTESIAN_POINT('',(-1.6702816869935,0.809946053334099,-7.1823505580364));
#161917=CARTESIAN_POINT('Origin',(1.48020701598583E-13,0.901573518000111,
3.93348548177741E-13));
#161918=CARTESIAN_POINT('Origin',(0.039683511241196,0.803566823389688,0.18890083934363));
#161919=CARTESIAN_POINT('Origin',(-0.0103065067715735,0.946349447599535,
0.18736394721752));
#161920=CARTESIAN_POINT('Ctrl Pts',(-1.759736143,0.809946053,-7.033194773));
#161921=CARTESIAN_POINT('Ctrl Pts',(-2.143352525,0.875601501000001,-6.937212273));
#161922=CARTESIAN_POINT('Ctrl Pts',(-2.514253728,0.940829639,-6.800075602));
#161923=CARTESIAN_POINT('Ctrl Pts',(-2.058047714,0.809946053,-7.212103688));
#161924=CARTESIAN_POINT('Ctrl Pts',(-2.451422449,0.875601501000001,-7.099850175));
#161925=CARTESIAN_POINT('Ctrl Pts',(-2.830254416,0.940829639,-6.945477661));
#161926=CARTESIAN_POINT('',(-2.05804772526778,0.809946052007895,-7.21210368328908));
#161927=CARTESIAN_POINT('',(-2.59587005412185,0.900669500603544,-7.03643792418539));
#161928=CARTESIAN_POINT('Origin',(0.0518557822968624,0.803573351669035,
0.185481350724109));
#161929=CARTESIAN_POINT('Ctrl Pts',(-2.50984261394196,0.940053944121885,
-6.80170495256707));
#161930=CARTESIAN_POINT('Ctrl Pts',(-2.52412028091269,0.933168237719441,
-6.84078553349327));
#161931=CARTESIAN_POINT('Ctrl Pts',(-2.53843709602442,0.92644844880531,
-6.87990743861688));
#161932=CARTESIAN_POINT('Ctrl Pts',(-2.56710953932711,0.913330774449358,
-6.95813867382332));
#161933=CARTESIAN_POINT('Ctrl Pts',(-2.58148121400414,0.906925555260774,
-6.9972917765852));
#161934=CARTESIAN_POINT('Ctrl Pts',(-2.59587005247871,0.900669500605613,
-7.03643792477924));
#161935=CARTESIAN_POINT('',(-1.90889194599726,0.809946050062004,-7.12264922581068));
#161936=CARTESIAN_POINT('Origin',(7.51352105532455E-13,0.714028548000978,
1.77202003071031E-12));
#161937=CARTESIAN_POINT('',(-2.77644680466804,0.750000002949537,-6.96716175156718));
#161938=CARTESIAN_POINT('',(-2.58717499223844,0.714243089251773,-7.00153200770937));
#161939=CARTESIAN_POINT('Origin',(-1.37378926289037,0.473612105092906,0.487673478742248));
#161940=CARTESIAN_POINT('',(-2.41797933832242,0.750000003586779,-7.09953350177321));
#161941=CARTESIAN_POINT('Origin',(0.,0.750000005151019,0.));
#161942=CARTESIAN_POINT('Origin',(1.42412805266309,0.692072907189111,-0.28584551893436));
#161943=CARTESIAN_POINT('Ctrl Pts',(-2.505416106,0.940837228,-6.803336691));
#161944=CARTESIAN_POINT('Ctrl Pts',(-2.876502367,0.875180297,-6.66667941000001));
#161945=CARTESIAN_POINT('Ctrl Pts',(-3.230523466,0.809946053,-6.49047133400001));
#161946=CARTESIAN_POINT('Ctrl Pts',(-3.2427676021491,0.807689868361921,
-6.48437702018873));
#161947=CARTESIAN_POINT('Ctrl Pts',(-3.25501173829825,0.805433683723839,
-6.47828270637748));
#161948=CARTESIAN_POINT('Ctrl Pts',(-2.35930162164529,0.940837228000001,
-7.11980219913443));
#161949=CARTESIAN_POINT('Ctrl Pts',(-2.74764941145793,0.875180297,-6.99111469553976));
#161950=CARTESIAN_POINT('Ctrl Pts',(-3.11969647505965,0.809946053,-6.82095164824412));
#161951=CARTESIAN_POINT('Ctrl Pts',(-3.13256405530693,0.807689868361921,
-6.81506640715394));
#161952=CARTESIAN_POINT('Ctrl Pts',(-3.14543163555424,0.805433683723839,
-6.8091811660636));
#161953=CARTESIAN_POINT('',(-3.11992551634625,0.809946052264273,-6.82026869839655));
#161954=CARTESIAN_POINT('Origin',(0.0593207810513757,0.946416086011058,
0.182047336412849));
#161955=CARTESIAN_POINT('',(-3.17522449034723,0.809946053334099,-6.6553700036187));
#161956=CARTESIAN_POINT('Origin',(1.27068494615301E-13,0.901573517999972,
7.12103986888479E-13));
#161957=CARTESIAN_POINT('Origin',(0.0793673685408737,0.803569481651845,
0.175960361352385));
#161958=CARTESIAN_POINT('Origin',(0.030212969465585,0.94634916292647,0.185201735070449));
#161959=CARTESIAN_POINT('Ctrl Pts',(-3.230523466,0.809946053,-6.490471334));
#161960=CARTESIAN_POINT('Ctrl Pts',(-3.58453771,0.875601501000001,-6.314266669));
#161961=CARTESIAN_POINT('Ctrl Pts',(-3.917287119,0.940829639,-6.100603383));
#161962=CARTESIAN_POINT('Ctrl Pts',(-3.560320807,0.809946053,-6.601069288));
#161963=CARTESIAN_POINT('Ctrl Pts',(-3.920367472,0.875601501000001,-6.406876261));
#161964=CARTESIAN_POINT('Ctrl Pts',(-4.257157031,0.940829639,-6.174675215));
#161965=CARTESIAN_POINT('',(-3.56032081704273,0.809946052117963,-6.60106928096141));
#161966=CARTESIAN_POINT('',(-4.04780621259384,0.90066950059267,-6.3138945874699));
#161967=CARTESIAN_POINT('Origin',(0.0905162729336373,0.803573320004725,
0.169997196395875));
#161968=CARTESIAN_POINT('Ctrl Pts',(-3.91332939641532,0.940053944031305,
-6.10314289974884));
#161969=CARTESIAN_POINT('Ctrl Pts',(-3.93567442913333,0.93316823759177,
-6.13824052205359));
#161970=CARTESIAN_POINT('Ctrl Pts',(-3.958066578088,0.926448448694993,-6.17337008654871));
#161971=CARTESIAN_POINT('Ctrl Pts',(-4.00288607856968,0.913330774344538,
-6.24360859109266));
#161972=CARTESIAN_POINT('Ctrl Pts',(-4.02533851098805,0.906925555221556,
-6.27875683049853));
#161973=CARTESIAN_POINT('Ctrl Pts',(-4.04780621106401,0.900669500593302,
-6.31389458844821));
#161974=CARTESIAN_POINT('',(-3.39542215258008,0.809946050062012,-6.54577030265895));
#161975=CARTESIAN_POINT('Origin',(-4.97171748214953E-12,0.714028548000734,
-7.79931674799172E-12));
#161976=CARTESIAN_POINT('',(-4.2092688339877,0.749999999449173,-6.20741939744525));
#161977=CARTESIAN_POINT('',(-4.0318106961935,0.71424308931512,-6.28167393347094));
#161978=CARTESIAN_POINT('Origin',(-1.23682663949029,0.473618831716048,0.771614155931688));
#161979=CARTESIAN_POINT('',(-3.88763818141073,0.750000000078679,-6.41375626069604));
#161980=CARTESIAN_POINT('Origin',(0.,0.750000000000029,0.));
#161981=CARTESIAN_POINT('Origin',(1.32939781459024,0.692075009954695,-0.585293017614466));
#161982=CARTESIAN_POINT('Ctrl Pts',(-3.909357153,0.940837228,-6.105688057));
#161983=CARTESIAN_POINT('Ctrl Pts',(-4.242390347,0.875180297,-5.89245317));
#161984=CARTESIAN_POINT('Ctrl Pts',(-4.550255102,0.809946053,-5.644260669));
#161985=CARTESIAN_POINT('Ctrl Pts',(-4.56090287975081,0.807689868358617,
-5.63567670949461));
#161986=CARTESIAN_POINT('Ctrl Pts',(-4.57155065750173,0.805433683717232,
-5.62709274998908));
#161987=CARTESIAN_POINT('Ctrl Pts',(-3.83468947317919,0.940837228,-6.44616507150536));
#161988=CARTESIAN_POINT('Ctrl Pts',(-4.18629389863377,0.875180297,-6.2370029152431));
#161989=CARTESIAN_POINT('Ctrl Pts',(-4.51306268385293,0.809946053,-5.99083906466819));
#161990=CARTESIAN_POINT('Ctrl Pts',(-4.52436427438713,0.807689868358617,
-5.98232526785112));
#161991=CARTESIAN_POINT('Ctrl Pts',(-4.53566586492127,0.805433683717232,
-5.97381147103415));
#161992=CARTESIAN_POINT('',(-4.51313955625589,0.809946052264272,-5.99012284469398));
#161993=CARTESIAN_POINT('Origin',(0.0970686782388863,0.94641608406807,0.165038954722597));
#161994=CARTESIAN_POINT('',(-4.53169732561459,0.809946053334099,-5.8171917447422));
#161995=CARTESIAN_POINT('Origin',(-1.98625837999344E-13,0.901573518000194,
-1.70436581514721E-13));
#161996=CARTESIAN_POINT('Origin',(0.115336598673815,0.803569483310559,0.154782889231857));
#161997=CARTESIAN_POINT('Origin',(0.0693193576764495,0.946349490873314,
0.174376799761953));
#161998=CARTESIAN_POINT('Ctrl Pts',(-4.550255102,0.809946053,-5.644260669));
#161999=CARTESIAN_POINT('Ctrl Pts',(-4.858113896,0.875601501000001,-5.396072974));
#162000=CARTESIAN_POINT('Ctrl Pts',(-5.13715251700001,0.940829639,-5.115873729));
#162001=CARTESIAN_POINT('Ctrl Pts',(-4.896117256,0.809946053,-5.681376225));
#162002=CARTESIAN_POINT('Ctrl Pts',(-5.206000469,0.875601501000001,-5.414323933));
#162003=CARTESIAN_POINT('Ctrl Pts',(-5.484999715,0.940829639,-5.115151819));
#162004=CARTESIAN_POINT('',(-4.89611726426675,0.809946052007887,-5.68137621598616));
#162005=CARTESIAN_POINT('',(-4.72318619291123,0.809946050061974,-5.66281843539706));
#162006=CARTESIAN_POINT('',(-5.31047145213963,0.900669500617274,-5.29612055723789));
#162007=CARTESIAN_POINT('Origin',(0.124944554358871,0.80357329647491,0.146564579444741));
#162008=CARTESIAN_POINT('Ctrl Pts',(-5.13383324548517,0.940053944149821,
-5.11920466612712));
#162009=CARTESIAN_POINT('Ctrl Pts',(-5.16320081509185,0.933168237703474,
-5.14867820427879));
#162010=CARTESIAN_POINT('Ctrl Pts',(-5.19262126598659,0.926448448811985,
-5.17817280908736));
#162011=CARTESIAN_POINT('Ctrl Pts',(-5.2514921139098,0.913330774430546,
-5.23713430901364));
#162012=CARTESIAN_POINT('Ctrl Pts',(-5.28097545369162,0.906925555263916,
-5.2666341930799));
#162013=CARTESIAN_POINT('Ctrl Pts',(-5.31047145087381,0.900669500617917,
-5.29612055850425));
#162014=CARTESIAN_POINT('Origin',(6.80922332407796E-12,0.714028548,6.68866004249757E-12));
#162015=CARTESIAN_POINT('',(-5.44527015389778,0.75000000074245,-5.15742500300344));
#162016=CARTESIAN_POINT('',(-5.28792341382218,0.714243089165336,-5.26809176682636));
#162017=CARTESIAN_POINT('Origin',(-1.0420408579184,0.473612704232346,1.01945056925008));
#162018=CARTESIAN_POINT('',(-5.17551536390861,0.750000001358042,-5.42807891669345));
#162019=CARTESIAN_POINT('Origin',(0.,0.750000002043061,0.));
#162020=CARTESIAN_POINT('Origin',(1.17249077617713,0.692074247261673,-0.857394588708109));
#162021=CARTESIAN_POINT('Ctrl Pts',(-5.130501005,0.940837228,-5.122544235));
#162022=CARTESIAN_POINT('Ctrl Pts',(-5.40990887,0.875180297,-4.842702369));
#162023=CARTESIAN_POINT('Ctrl Pts',(-5.657221867,0.809946053,-4.534130649));
#162024=CARTESIAN_POINT('Ctrl Pts',(-5.66577540788212,0.807689868409067,
-4.52345842047135));
#162025=CARTESIAN_POINT('Ctrl Pts',(-5.67432894876434,0.805433683818132,
-4.51278619194269));
#162026=CARTESIAN_POINT('Ctrl Pts',(-5.13077150802368,0.940837228,-5.47111243078886));
#162027=CARTESIAN_POINT('Ctrl Pts',(-5.42919193653774,0.875180297000001,
-5.19125581029712));
#162028=CARTESIAN_POINT('Ctrl Pts',(-5.69540309763305,0.809946053,-4.88060150440865));
#162029=CARTESIAN_POINT('Ctrl Pts',(-5.70461024839882,0.807689868409067,
-4.86985724778707));
#162030=CARTESIAN_POINT('Ctrl Pts',(-5.71381739916451,0.805433683818133,
-4.85911299116537));
#162031=CARTESIAN_POINT('',(-5.6953242076193,0.809946052265042,-4.87988550210847));
#162032=CARTESIAN_POINT('Origin',(0.130277874055508,0.946416059068594,0.140313630459598));
#162033=CARTESIAN_POINT('',(-5.67627303080642,0.809946053334091,-4.70700806542456));
#162034=CARTESIAN_POINT('Origin',(-3.98552718605671E-13,0.901573518000056,
-3.54750950837257E-13));
#162035=CARTESIAN_POINT('Origin',(0.14591442777288,0.803569496728868,0.126370695433855));
#162036=CARTESIAN_POINT('Origin',(0.105184722484503,0.946349189289516,0.155398444855144));
#162037=CARTESIAN_POINT('Ctrl Pts',(-5.657221867,0.809946053,-4.534130649));
#162038=CARTESIAN_POINT('Ctrl Pts',(-5.904530075,0.875601501,-4.225564904));
#162039=CARTESIAN_POINT('Ctrl Pts',(-6.116810374,0.940829639,-3.891931506));
#162040=CARTESIAN_POINT('Ctrl Pts',(-6.002976704,0.809946053,-4.496028325));
#162041=CARTESIAN_POINT('Ctrl Pts',(-6.24820667,0.875601501,-4.168603835));
#162042=CARTESIAN_POINT('Ctrl Pts',(-6.456369908,0.940829639,-3.816449609));
#162043=CARTESIAN_POINT('',(-6.00297671011313,0.809946052117936,-4.49602831442525));
#162044=CARTESIAN_POINT('',(-6.3248249481419,0.900669500625308,-4.03070581579533));
#162045=CARTESIAN_POINT('Origin',(0.153530836917978,0.803573322659294,0.116278825060671));
#162046=CARTESIAN_POINT('Ctrl Pts',(-6.11428475835875,0.940053944065295,
-3.89589811327206));
#162047=CARTESIAN_POINT('Ctrl Pts',(-6.149301669923,0.933168237633643,-3.91836941714209));
#162048=CARTESIAN_POINT('Ctrl Pts',(-6.18437475489027,0.926448448797304,
-3.94084992703146));
#162049=CARTESIAN_POINT('Ctrl Pts',(-6.2545442145559,0.913330774423472,
-3.98577744771472));
#162050=CARTESIAN_POINT('Ctrl Pts',(-6.28967985315877,0.906925555268892,
-4.00824959427422));
#162051=CARTESIAN_POINT('Ctrl Pts',(-6.32482494717043,0.900669500625957,
-4.0307058173159));
#162052=CARTESIAN_POINT('',(-5.83009929659162,0.809946050061996,-4.51507947267794));
#162053=CARTESIAN_POINT('Origin',(-7.43242273282263E-12,0.714028547999266,
-4.59875193481452E-12));
#162054=CARTESIAN_POINT('',(-6.42665668287943,0.749999999391371,-3.8662751550363));
#162055=CARTESIAN_POINT('',(-6.29677870903883,0.714243089259356,-4.00817948512182));
#162056=CARTESIAN_POINT('Origin',(-0.798522356592828,0.473612937660149,
1.21962839912454));
#162057=CARTESIAN_POINT('',(-6.22139120767294,0.750000000236834,-4.18859062748345));
#162058=CARTESIAN_POINT('Origin',(0.,0.750000000000029,0.));
#162059=CARTESIAN_POINT('Origin',(0.960772761012999,0.692075178873913,-1.08939629753758));
#162060=CARTESIAN_POINT('Ctrl Pts',(-6.111748332,0.940837228,-3.899875938));
#162061=CARTESIAN_POINT('Ctrl Pts',(-6.324466068,0.875180297,-3.566512188));
#162062=CARTESIAN_POINT('Ctrl Pts',(-6.499663225,0.809946053,-3.211989719));
#162063=CARTESIAN_POINT('Ctrl Pts',(-6.50572257530016,0.807689868352189,
-3.1997282424684));
#162064=CARTESIAN_POINT('Ctrl Pts',(-6.51178192560047,0.805433683704377,
-3.18746676593687));
#162065=CARTESIAN_POINT('Ctrl Pts',(-6.18694436872785,0.940837228,-4.24023665216015));
#162066=CARTESIAN_POINT('Ctrl Pts',(-6.41822699307382,0.875180297000001,
-3.90277135386781));
#162067=CARTESIAN_POINT('Ctrl Pts',(-6.61143279187626,0.809946053,-3.54215244291236));
#162068=CARTESIAN_POINT('Ctrl Pts',(-6.61811498715281,0.807689868352189,
-3.52968011548556));
#162069=CARTESIAN_POINT('Ctrl Pts',(-6.62479718242936,0.805433683704377,
-3.51720778805875));
#162070=CARTESIAN_POINT('',(-6.6112018269334,0.809946052265044,-3.54147013934983));
#162071=CARTESIAN_POINT('Origin',(0.157395165769212,0.946416051811995,0.109027188938045));
#162072=CARTESIAN_POINT('',(-6.55543251743721,0.809946053334091,-3.37672992068055));
#162073=CARTESIAN_POINT('Origin',(1.56125112837913E-14,0.901573518000056,
-2.27682456221956E-14));
#162074=CARTESIAN_POINT('Origin',(0.169668356951714,0.803569306176809,0.0920486297458446));
#162075=CARTESIAN_POINT('Origin',(0.136131335377041,0.946349429981463,0.129153532124544));
#162076=CARTESIAN_POINT('Ctrl Pts',(-6.499663225,0.809946053,-3.211989719));
#162077=CARTESIAN_POINT('Ctrl Pts',(-6.674856991,0.875601501,-2.857474115));
#162078=CARTESIAN_POINT('Ctrl Pts',(-6.810452976,0.940829639,-2.486006892));
#162079=CARTESIAN_POINT('Ctrl Pts',(-6.829143632,0.809946053,-3.100451136));
#162080=CARTESIAN_POINT('Ctrl Pts',(-6.998253672,0.875601501,-2.727964456));
#162081=CARTESIAN_POINT('Ctrl Pts',(-7.125847419,0.940829639,-2.339294456));
#162082=CARTESIAN_POINT('',(-6.8291436357368,0.809946052117954,-3.10045112431753));
#162083=CARTESIAN_POINT('',(-7.04343665893579,0.900669500612243,-2.57681975023539));
#162084=CARTESIAN_POINT('Origin',(0.174937395336665,0.803573296031086,0.0805555129405777));
#162085=CARTESIAN_POINT('Ctrl Pts',(-6.8088391104413,0.940053944145248,
-2.49042369485089));
#162086=CARTESIAN_POINT('Ctrl Pts',(-6.8478680119646,0.933168237710336,
-2.50484203093422));
#162087=CARTESIAN_POINT('Ctrl Pts',(-6.88695375326514,0.92644844877595,
-2.51925728249278));
#162088=CARTESIAN_POINT('Ctrl Pts',(-6.96514077864709,0.913330774422057,
-2.54805006275026));
#162089=CARTESIAN_POINT('Ctrl Pts',(-7.00428581293043,0.906925555246983,
-2.56244369927751));
#162090=CARTESIAN_POINT('Ctrl Pts',(-7.04343665832799,0.90066950061289,
-2.57681975189093));
#162091=CARTESIAN_POINT('',(-6.66440343625349,0.809946050061996,-3.15622041112841));
#162092=CARTESIAN_POINT('Origin',(-5.22889023746309E-12,0.714028547999755,
-2.12872254545804E-12));
#162093=CARTESIAN_POINT('',(-7.10753989224886,0.749999998867154,-2.39434257513311));
#162094=CARTESIAN_POINT('',(-7.01120363025577,0.714243089287394,-2.56084918553649));
#162095=CARTESIAN_POINT('Origin',(-0.517668238337649,0.473612986217688,
1.36277345844869));
#162096=CARTESIAN_POINT('',(-6.97636171019226,0.749999999742988,-2.75324849672299));
#162097=CARTESIAN_POINT('Origin',(0.,0.749999999161366,0.));
#162098=CARTESIAN_POINT('Origin',(0.704122757021434,0.69207529282193,-1.27046448369264));
#162099=CARTESIAN_POINT('Ctrl Pts',(-6.807217099,0.940837228,-2.494853776));
#162100=CARTESIAN_POINT('Ctrl Pts',(-6.94329826,0.875180297,-2.12355586));
#162101=CARTESIAN_POINT('Ctrl Pts',(-7.038187555,0.809946053,-1.73965972));
#162102=CARTESIAN_POINT('Ctrl Pts',(-7.04146938600978,0.807689868412916,
-1.72638232915434));
#162103=CARTESIAN_POINT('Ctrl Pts',(-7.04475121701958,0.80543368382583,
-1.71310493830869));
#162104=CARTESIAN_POINT('Ctrl Pts',(-6.95382258706004,0.940837228000001,
-2.81109212166392));
#162105=CARTESIAN_POINT('Ctrl Pts',(-7.10715288826948,0.875180297,-2.43179764591034));
#162106=CARTESIAN_POINT('Ctrl Pts',(-7.21831923755849,0.809946053,-2.03807626899811));
#162107=CARTESIAN_POINT('Ctrl Pts',(-7.22216402502731,0.807689868412915,
-2.02445906355928));
#162108=CARTESIAN_POINT('Ctrl Pts',(-7.22600881249612,0.805433683825832,
-2.01084185812038));
#162109=CARTESIAN_POINT('',(-7.2179469973611,0.809946052265047,-2.03745956795825));
#162110=CARTESIAN_POINT('Origin',(0.177153184908597,0.946416038992782,0.0726429565010295));
#162111=CARTESIAN_POINT('',(-7.12806726602417,0.809946053334091,-1.88855963752162));
#162112=CARTESIAN_POINT('Origin',(-3.76001313417973E-13,0.901573517999806,
-6.46184494801361E-14));
#162113=CARTESIAN_POINT('Origin',(0.185488957796006,0.803569127013547,0.0534228253417359));
#162114=CARTESIAN_POINT('Origin',(0.160712844055243,0.946349502133253,0.0968698011685543));
#162115=CARTESIAN_POINT('Ctrl Pts',(-7.038187555,0.809946053,-1.73965972));
#162116=CARTESIAN_POINT('Ctrl Pts',(-7.133075012,0.875601501,-1.355771012));
#162117=CARTESIAN_POINT('Ctrl Pts',(-7.185646366,0.940829639,-0.963839358));
#162118=CARTESIAN_POINT('Ctrl Pts',(-7.335987395,0.809946053,-1.559900299));
#162119=CARTESIAN_POINT('Ctrl Pts',(-7.42107011,0.875601501,-1.15976849));
#162120=CARTESIAN_POINT('Ctrl Pts',(-7.462128226,0.940829639,-0.752756495));
#162121=CARTESIAN_POINT('',(-7.33598739610994,0.809946052007895,-1.5599002868475));
#162122=CARTESIAN_POINT('',(-7.43270510030618,0.900669500577752,-1.00244445737222));
#162123=CARTESIAN_POINT('Origin',(0.188164822724248,0.803573315666638,0.0410658480750598));
#162124=CARTESIAN_POINT('Ctrl Pts',(-7.18501971321784,0.940053944258733,
-0.968499831650855));
#162125=CARTESIAN_POINT('Ctrl Pts',(-7.22623565673749,0.933168237835753,
-0.974191014905439));
#162126=CARTESIAN_POINT('Ctrl Pts',(-7.26750644861614,0.926448448817741,
-0.979866966976774));
#162127=CARTESIAN_POINT('Ctrl Pts',(-7.35005510155544,0.913330774439853,
-0.991178688866976));
#162128=CARTESIAN_POINT('Ctrl Pts',(-7.39137915317629,0.906925555242182,
-0.996820784991662));
#162129=CARTESIAN_POINT('Ctrl Pts',(-7.43270510007076,0.900669500578381,
-1.00244445910288));
#162130=CARTESIAN_POINT('',(-7.18708747905281,0.809946050061996,-1.6497799918444));
#162131=CARTESIAN_POINT('Origin',(1.55084278752327E-12,0.714028547998288,
3.34855840972148E-13));
#162132=CARTESIAN_POINT('',(-7.45608243706208,0.749999999447828,-0.810453196812189));
#162133=CARTESIAN_POINT('',(-7.39779246228466,0.714243089163989,-0.99377642309357));
#162134=CARTESIAN_POINT('Origin',(-0.212611893476207,0.47361691107108,1.44219440505136));
#162135=CARTESIAN_POINT('',(-7.40512529159642,0.750000000292744,-1.18916753241498));
#162136=CARTESIAN_POINT('Origin',(0.,0.750000000000029,0.));
#162137=CARTESIAN_POINT('Origin',(0.414546568407169,0.692075061657456,-1.39212726711968));
#162138=CARTESIAN_POINT('Ctrl Pts',(-7.184387961,0.940837228,-0.973175025));
#162139=CARTESIAN_POINT('Ctrl Pts',(-7.237469544,0.875180297,-0.581304421));
#162140=CARTESIAN_POINT('Ctrl Pts',(-7.24761405700001,0.809946053,-0.185985165));
#162141=CARTESIAN_POINT('Ctrl Pts',(-7.24796491404188,0.807689868412287,
-0.172312695482098));
#162142=CARTESIAN_POINT('Ctrl Pts',(-7.2483157710839,0.805433683824573,
-0.158640225964204));
#162143=CARTESIAN_POINT('Ctrl Pts',(-7.3955477905724,0.940837228,-1.25050404734907));
#162144=CARTESIAN_POINT('Ctrl Pts',(-7.46375621382,0.875180297000001,-0.847115783862962));
#162145=CARTESIAN_POINT('Ctrl Pts',(-7.4876850977098,0.809946053,-0.438701914431369));
#162146=CARTESIAN_POINT('Ctrl Pts',(-7.48851269952937,0.807689868412287,
-0.424576556013486));
#162147=CARTESIAN_POINT('Ctrl Pts',(-7.48934030134893,0.805433683824576,
-0.410451197595596));
#162148=CARTESIAN_POINT('',(-7.48718898778801,0.809946052265052,-0.438179652160465));
#162149=CARTESIAN_POINT('Origin',(0.188627531184321,0.946416067397882,0.0328619060441109));
#162150=CARTESIAN_POINT('',(-7.36740151108662,0.809946053334091,-0.312082404455189));
#162151=CARTESIAN_POINT('Origin',(-4.90926743701436E-13,0.901573517999861,
-5.01443504774546E-14));
#162152=CARTESIAN_POINT('Origin',(0.192637052573005,0.803569461496135,0.0122991578322531));
#162153=CARTESIAN_POINT('Origin',(0.177779897331626,0.946349182381831,0.0600565242311453));
#162154=CARTESIAN_POINT('Ctrl Pts',(-7.247614057,0.809946053,-0.185985165));
#162155=CARTESIAN_POINT('Ctrl Pts',(-7.257758374,0.875601501,0.209326436));
#162156=CARTESIAN_POINT('Ctrl Pts',(-7.224846918,0.940829639,0.603396233));
#162157=CARTESIAN_POINT('Ctrl Pts',(-7.49980854,0.809946053,0.053589743));
#162158=CARTESIAN_POINT('Ctrl Pts',(-7.496885558,0.875601501,0.462656961));
#162159=CARTESIAN_POINT('Ctrl Pts',(-7.44948821,0.940829639,0.868979523));
#162160=CARTESIAN_POINT('',(-7.49980853848092,0.809946052117954,0.0535897551571855));
#162161=CARTESIAN_POINT('',(-7.47442851167214,0.90066950059978,0.618804024144828));
#162162=CARTESIAN_POINT('Origin',(0.19259339066803,0.803573308386867,-0.000344107343095319));
#162163=CARTESIAN_POINT('Ctrl Pts',(-7.22523678067821,0.940053944158219,
0.598710006831233));
#162164=CARTESIAN_POINT('Ctrl Pts',(-7.26671255469412,0.933168237733409,
0.602012089818992));
#162165=CARTESIAN_POINT('Ctrl Pts',(-7.30823861989039,0.926448448798157,
0.605340838600035));
#162166=CARTESIAN_POINT('Ctrl Pts',(-7.3912890171494,0.913330774413794,
0.612039098687823));
#162167=CARTESIAN_POINT('Ctrl Pts',(-7.43285981896345,0.906925555263889,
0.615412361129273));
#162168=CARTESIAN_POINT('Ctrl Pts',(-7.47442851182048,0.900669500600411,
0.618804022327912));
#162169=CARTESIAN_POINT('',(-7.37371129866262,0.809946050061996,-0.0661976928859446));
#162170=CARTESIAN_POINT('Origin',(8.59208537651313E-12,0.714028548000978,
-4.4278816724308E-13));
#162171=CARTESIAN_POINT('',(-7.45598684901459,0.749999993899794,0.811332053920997));
#162172=CARTESIAN_POINT('',(-7.43846874078927,0.714243089245729,0.619764219404089));
#162173=CARTESIAN_POINT('Origin',(0.102370559289628,0.473612122600343,1.45418114526299));
#162174=CARTESIAN_POINT('',(-7.48763343938384,0.749999995439564,0.4305176098096));
#162175=CARTESIAN_POINT('Origin',(0.,0.749999993327366,0.));
#162176=CARTESIAN_POINT('Origin',(0.105594438791012,0.69207569376148,-1.44869683082552));
#162177=CARTESIAN_POINT('Ctrl Pts',(-7.225624826,0.940837228,0.594008309));
#162178=CARTESIAN_POINT('Ctrl Pts',(-7.193224795,0.875180297,0.988128168));
#162179=CARTESIAN_POINT('Ctrl Pts',(-7.118150181,0.809946053,1.376385849));
#162180=CARTESIAN_POINT('Ctrl Pts',(-7.11555365842227,0.807689868407598,
1.38981408766792));
#162181=CARTESIAN_POINT('Ctrl Pts',(-7.11295713584455,0.805433683815197,
1.40324232633587));
#162182=CARTESIAN_POINT('Ctrl Pts',(-7.49146539822841,0.940837228000001,
0.368556206903295));
#162183=CARTESIAN_POINT('Ctrl Pts',(-7.47136259377401,0.875180297,0.777176271142086));
#162184=CARTESIAN_POINT('Ctrl Pts',(-7.40693512424696,0.809946053,1.18118565373313));
#162185=CARTESIAN_POINT('Ctrl Pts',(-7.40470684267029,0.807689868407598,
1.19515867906914));
#162186=CARTESIAN_POINT('Ctrl Pts',(-7.40247856109349,0.805433683815198,
1.20913170440515));
#162187=CARTESIAN_POINT('',(-7.40633834297572,0.809946052264265,1.18158905489033));
#162188=CARTESIAN_POINT('Origin',(0.191281854905171,0.946416077062279,-0.00845573081088166));
#162189=CARTESIAN_POINT('',(-7.26224424964502,0.809946053334091,1.27898745451562));
#162190=CARTESIAN_POINT('Origin',(1.35958952429682E-12,0.901573518000083,
-9.95975220699497E-14));
#162191=CARTESIAN_POINT('Origin',(0.190772156346956,0.803567066281397,-0.0293984664076719));
#162192=CARTESIAN_POINT('Origin',(0.186530734540632,0.946349387717187,0.0204350879223742));
#162193=CARTESIAN_POINT('Ctrl Pts',(-7.118150181,0.809946053,1.376385849));
#162194=CARTESIAN_POINT('Ctrl Pts',(-7.04307702,0.875601501,1.764636013));
#162195=CARTESIAN_POINT('Ctrl Pts',(-6.926221658,0.940829639,2.142417687));
#162196=CARTESIAN_POINT('Ctrl Pts',(-7.312946974,0.809946053,1.664573988));
#162197=CARTESIAN_POINT('Ctrl Pts',(-7.222154969,0.875601501,2.063449087));
#162198=CARTESIAN_POINT('Ctrl Pts',(-7.088518405,0.940829639,2.450083024));
#162199=CARTESIAN_POINT('',(-7.31294696989878,0.809946052117947,1.66457399951245));
#162200=CARTESIAN_POINT('',(-7.16665595331403,0.900669500631217,2.21111791752741));
#162201=CARTESIAN_POINT('Origin',(0.188016845196407,0.803573325729783,-0.0417380006118342));
#162202=CARTESIAN_POINT('Ctrl Pts',(-6.92760980580542,0.940053944212052,
2.13792483126068));
#162203=CARTESIAN_POINT('Ctrl Pts',(-6.96740604904775,0.933168237787557,
2.15006577861116));
#162204=CARTESIAN_POINT('Ctrl Pts',(-7.00724567548623,0.926448448831224,
2.16224357956276));
#162205=CARTESIAN_POINT('Ctrl Pts',(-7.08691447273129,0.913330774457708,
2.18663861842916));
#162206=CARTESIAN_POINT('Ctrl Pts',(-7.12678822078421,0.90692555528841,
2.1988695094987));
#162207=CARTESIAN_POINT('Ctrl Pts',(-7.1666559538467,0.900669500631857,
2.21111791579394));
#162208=CARTESIAN_POINT('',(-7.21554857376483,0.809946050061996,1.52047993622552));
#162209=CARTESIAN_POINT('Origin',(6.07066480418084E-12,0.714028547999755,
-1.82102596890665E-12));
#162210=CARTESIAN_POINT('',(-7.10725761130664,0.749999998991949,2.39518035554988));
#162211=CARTESIAN_POINT('',(-7.13133048835984,0.714243089300439,2.20432537570086));
#162212=CARTESIAN_POINT('Origin',(0.412603354274212,0.473613015875695,1.39817395588609));
#162213=CARTESIAN_POINT('',(-7.22002817973684,0.749999999822909,2.03007218619174));
#162214=CARTESIAN_POINT('Origin',(0.,0.749999999379636,0.));
#162215=CARTESIAN_POINT('Origin',(-0.208305057603325,0.692075220411731,
-1.43752493983075));
#162216=CARTESIAN_POINT('Ctrl Pts',(-6.928999505,0.940837228,2.133416475));
#162217=CARTESIAN_POINT('Ctrl Pts',(-6.81263284900001,0.875180297,2.511356981));
#162218=CARTESIAN_POINT('Ctrl Pts',(-6.655849513,0.809946053,2.874398591));
#162219=CARTESIAN_POINT('Ctrl Pts',(-6.65042702125904,0.807689868393002,
2.88695470941201));
#162220=CARTESIAN_POINT('Ctrl Pts',(-6.64500452951808,0.805433683786001,
2.89951082782398));
#162221=CARTESIAN_POINT('Ctrl Pts',(-7.23709041010449,0.940837228,1.97038318210572));
#162222=CARTESIAN_POINT('Ctrl Pts',(-7.12961636364179,0.875180297,2.3651284279141));
#162223=CARTESIAN_POINT('Ctrl Pts',(-6.97984509784159,0.809946053,2.74584229453961));
#162224=CARTESIAN_POINT('Ctrl Pts',(-6.97466512481288,0.807689868393001,
2.75900962373485));
#162225=CARTESIAN_POINT('Ctrl Pts',(-6.96948515178403,0.805433683786001,
2.77217695293011));
#162226=CARTESIAN_POINT('',(-6.97917554963226,0.809946052264273,2.7461079740992));
#162227=CARTESIAN_POINT('Origin',(0.184991985497199,0.946416080281647,-0.0493779501458091));
#162228=CARTESIAN_POINT('',(-6.81751251872002,0.809946053334091,2.81025328239219));
#162229=CARTESIAN_POINT('Origin',(-1.13407547241984E-12,0.901573518,4.45823933326039E-13));
#162230=CARTESIAN_POINT('Origin',(0.179996582079746,0.803569217500806,-0.0697236045505898));
#162231=CARTESIAN_POINT('Origin',(0.186565303897439,0.946349423399718,-0.0201418751128665));
#162232=CARTESIAN_POINT('Ctrl Pts',(-6.655849513,0.809946053,2.874398591));
#162233=CARTESIAN_POINT('Ctrl Pts',(-6.499069213,0.875601501,3.237433171));
#162234=CARTESIAN_POINT('Ctrl Pts',(-6.303733971,0.940829639,3.581262071));
#162235=CARTESIAN_POINT('Ctrl Pts',(-6.784140134,0.809946053,3.197724603));
#162236=CARTESIAN_POINT('Ctrl Pts',(-6.609724441,0.875601501,3.567756627));
#162237=CARTESIAN_POINT('Ctrl Pts',(-6.396097357,0.940829639,3.916623367));
#162238=CARTESIAN_POINT('',(-6.78414012751564,0.809946052117958,3.19772461340661));
#162239=CARTESIAN_POINT('',(-6.52377852755123,0.900669500602261,3.70004239467368));
#162240=CARTESIAN_POINT('Origin',(0.174648437993212,0.803573303207944,-0.0811801132144108));
#162241=CARTESIAN_POINT('Ctrl Pts',(-6.30605549606934,0.940053944170996,
3.57717266655217));
#162242=CARTESIAN_POINT('Ctrl Pts',(-6.3423113804959,0.933168237742285,
3.59758478126356));
#162243=CARTESIAN_POINT('Ctrl Pts',(-6.37860171123587,0.92644844881477,
3.61804221396549));
#162244=CARTESIAN_POINT('Ctrl Pts',(-6.45116368405659,0.913330774441575,
3.65899334681766));
#162245=CARTESIAN_POINT('Ctrl Pts',(-6.48747592609581,0.906925555257983,
3.67950996366937));
#162246=CARTESIAN_POINT('Ctrl Pts',(-6.523778528422,0.900669500602901,3.70004239313431));
#162247=CARTESIAN_POINT('',(-6.71999481604169,0.809946050061996,3.03606161350816));
#162248=CARTESIAN_POINT('Origin',(1.29674916637956E-11,0.714028548000978,
-7.12841244365769E-12));
#162249=CARTESIAN_POINT('',(-6.42620090260971,0.749999999423274,3.86703266739492));
#162250=CARTESIAN_POINT('',(-6.49073914757855,0.714243089136802,3.68581472836303));
#162251=CARTESIAN_POINT('Origin',(0.703519225223311,0.473616182160146,1.27678862258471));
#162252=CARTESIAN_POINT('',(-6.61482242335707,0.750000000270831,3.53470286042756));
#162253=CARTESIAN_POINT('Origin',(0.,0.750000000000029,0.));
#162254=CARTESIAN_POINT('Origin',(-0.512460977771081,0.692075222204829,
-1.35913646868323));
#162255=CARTESIAN_POINT('Ctrl Pts',(-6.308381869,0.940837228,3.573068457));
#162256=CARTESIAN_POINT('Ctrl Pts',(-6.113489763,0.875180297,3.917157533));
#162257=CARTESIAN_POINT('Ctrl Pts',(-5.88232872,0.809946053,4.238007649));
#162258=CARTESIAN_POINT('Ctrl Pts',(-5.87433380866454,0.807689868350337,
4.24910453710929));
#162259=CARTESIAN_POINT('Ctrl Pts',(-5.86633889732895,0.805433683700671,
4.26020142521853));
#162260=CARTESIAN_POINT('Ctrl Pts',(-6.64431711846015,0.940837228,3.48007722958934));
#162261=CARTESIAN_POINT('Ctrl Pts',(-6.45449719567435,0.875180297,3.84248980808543));
#162262=CARTESIAN_POINT('Ctrl Pts',(-6.22638527100657,0.809946053,4.18210640003399));
#162263=CARTESIAN_POINT('Ctrl Pts',(-6.21849581615458,0.807689868350337,
4.19385234349162));
#162264=CARTESIAN_POINT('Ctrl Pts',(-6.21060636130262,0.805433683700673,
4.20559828694927));
#162265=CARTESIAN_POINT('',(-6.22567426167375,0.809946052265036,4.18222193646299));
#162266=CARTESIAN_POINT('Origin',(0.170052079903854,0.946416046042726,-0.0879912919240844));
#162267=CARTESIAN_POINT('',(-6.05400147933149,0.809946053334091,4.21011478918027));
#162268=CARTESIAN_POINT('Origin',(1.12713657851593E-12,0.901573518000139,
-5.95226992694542E-13));
#162269=CARTESIAN_POINT('Origin',(0.160800309337056,0.803569514372434,-0.106787821028391));
#162270=CARTESIAN_POINT('Origin',(0.177873690556483,0.946349453047268,-0.0597770055129204));
#162271=CARTESIAN_POINT('Ctrl Pts',(-5.88232872,0.809946053,4.238007649));
#162272=CARTESIAN_POINT('Ctrl Pts',(-5.651172152,0.875601501,4.55885155200001));
#162273=CARTESIAN_POINT('Ctrl Pts',(-5.38649069,0.940829639,4.85265062));
#162274=CARTESIAN_POINT('Ctrl Pts',(-5.938114442,0.809946053,4.58135317));
#162275=CARTESIAN_POINT('Ctrl Pts',(-5.688230544,0.875601501,4.905239832));
#162276=CARTESIAN_POINT('Ctrl Pts',(-5.404601906,0.940829639,5.200026753));
#162277=CARTESIAN_POINT('',(-5.93811443344712,0.809946052007899,4.58135317874226));
#162278=CARTESIAN_POINT('',(-5.57585646849975,0.900669500631655,5.01595700132481));
#162279=CARTESIAN_POINT('Origin',(0.153113955462107,0.803573294511166,-0.116826443349924));
#162280=CARTESIAN_POINT('Ctrl Pts',(-5.3896370410399,0.940053943979818,
4.84915588374515));
#162281=CARTESIAN_POINT('Ctrl Pts',(-5.42065728185389,0.933168237522385,
4.8768847182855));
#162282=CARTESIAN_POINT('Ctrl Pts',(-5.45170142069717,0.926448448772325,
4.9046652153187));
#162283=CARTESIAN_POINT('Ctrl Pts',(-5.5137636518489,0.913330774406861,
4.96025761277208));
#162284=CARTESIAN_POINT('Ctrl Pts',(-5.54481646756075,0.906925555254912,
4.98810062106575));
#162285=CARTESIAN_POINT('Ctrl Pts',(-5.57585646965406,0.900669500636448,
5.01595699999707));
#162286=CARTESIAN_POINT('',(-5.9102215701673,0.809946050061996,4.40968042401888));
#162287=CARTESIAN_POINT('Origin',(3.37403716077489E-12,0.714028547998533,
-2.77989437025283E-12));
#162288=CARTESIAN_POINT('',(-5.44466217806886,0.750000000797388,5.15806683544274));
#162289=CARTESIAN_POINT('',(-5.54664805887057,0.714243089237145,4.99495947994093));
#162290=CARTESIAN_POINT('Origin',(0.961541774337511,0.473612790912695,1.09570374294362));
#162291=CARTESIAN_POINT('',(-5.70031492472452,0.750000001422546,4.87405475630863));
#162292=CARTESIAN_POINT('Origin',(0.,0.750000002126994,0.));
#162293=CARTESIAN_POINT('Origin',(-0.792659925892832,0.692074230931837,
-1.21718943245041));
#162294=CARTESIAN_POINT('Ctrl Pts',(-5.392791307,0.940837228,4.845647729));
#162295=CARTESIAN_POINT('Ctrl Pts',(-5.128486691,0.875180297,5.139796152));
#162296=CARTESIAN_POINT('Ctrl Pts',(-4.833756773,0.809946053,5.403452179));
#162297=CARTESIAN_POINT('Ctrl Pts',(-4.82356327583318,0.807689868470432,
5.412570957923));
#162298=CARTESIAN_POINT('Ctrl Pts',(-4.81336977866643,0.805433683940862,
5.421689736846));
#162299=CARTESIAN_POINT('Ctrl Pts',(-5.74086294257407,0.940837228000001,
4.82704673403782));
#162300=CARTESIAN_POINT('Ctrl Pts',(-5.47757291232495,0.875180297000001,
5.1401806345747));
#162301=CARTESIAN_POINT('Ctrl Pts',(-5.18178659015179,0.809946053,5.42281985940034));
#162302=CARTESIAN_POINT('Ctrl Pts',(-5.17155655630415,0.807689868470432,
5.43259518915661));
#162303=CARTESIAN_POINT('Ctrl Pts',(-5.16132652245651,0.805433683940861,
5.44237051891284));
#162304=CARTESIAN_POINT('',(-5.18106736691782,0.809946052265036,5.42277984867541));
#162305=CARTESIAN_POINT('Origin',(0.147161080574969,0.946416070009224,-0.122490500035624));
#162306=CARTESIAN_POINT('',(-5.0074120594976,0.809946053334091,5.4131160078898));
#162307=CARTESIAN_POINT('Origin',(3.17020715234761E-13,0.901573518000139,
-3.02275565688959E-13));
#162308=CARTESIAN_POINT('Origin',(0.134085142685041,0.803569523315697,-0.138858993640414));
#162309=CARTESIAN_POINT('Origin',(0.160865042239952,0.946349178674713,-0.0966172917225144));
#162310=CARTESIAN_POINT('Ctrl Pts',(-4.833756773,0.809946053,5.403452179));
#162311=CARTESIAN_POINT('Ctrl Pts',(-4.539032563,0.875601501,5.667103101));
#162312=CARTESIAN_POINT('Ctrl Pts',(-4.217381091,0.940829639,5.89713462));
#162313=CARTESIAN_POINT('Ctrl Pts',(-4.814429119,0.809946053,5.750762755));
#162314=CARTESIAN_POINT('Ctrl Pts',(-4.500761309,0.875601501,6.013359475));
#162315=CARTESIAN_POINT('Ctrl Pts',(-4.160393277,0.940829639,6.240282668));
#162316=CARTESIAN_POINT('',(-4.81442910876821,0.809946052117945,5.75076276168269));
#162317=CARTESIAN_POINT('',(-4.36721355850133,0.90066950062204,6.09733103335733));
#162318=CARTESIAN_POINT('Origin',(0.124420020444259,0.803573308344962,-0.147010115980704));
#162319=CARTESIAN_POINT('Ctrl Pts',(-4.22120514702725,0.94005394400724,
5.89439796090951));
#162320=CARTESIAN_POINT('Ctrl Pts',(-4.24553927219527,0.933168237550762,
5.92814694546217));
#162321=CARTESIAN_POINT('Ctrl Pts',(-4.26988563088799,0.926448448753514,
5.96195152229541));
#162322=CARTESIAN_POINT('Ctrl Pts',(-4.31854615956295,0.913330774374134,
6.02958574554369));
#162323=CARTESIAN_POINT('Ctrl Pts',(-4.34288755386442,0.906925555252343,
6.06345323705642));
#162324=CARTESIAN_POINT('Ctrl Pts',(-4.36721355998907,0.900669500622685,
6.09733103228917));
#162325=CARTESIAN_POINT('',(-4.82409293229943,0.809946050061996,5.57710747885074));
#162326=CARTESIAN_POINT('Origin',(-1.24032728532342E-13,0.714028548000245,
3.13984949151802E-13));
#162327=CARTESIAN_POINT('',(-4.20853710845448,0.749999998091708,6.20791551735464));
#162328=CARTESIAN_POINT('',(-4.34320187174526,0.714243089326984,6.0705454777832));
#162329=CARTESIAN_POINT('Origin',(1.17460218335671,0.47361248030911,0.863386897244571));
#162330=CARTESIAN_POINT('',(-4.51926702152341,0.749999998623412,5.98550127963007));
#162331=CARTESIAN_POINT('Origin',(0.,0.749999997908146,0.));
#162332=CARTESIAN_POINT('Origin',(-1.03578289774064,0.692075300936382,-1.018343469197));
#162333=CARTESIAN_POINT('Ctrl Pts',(-4.225039818,0.940837228,5.891649899));
#162334=CARTESIAN_POINT('Ctrl Pts',(-3.903681281,0.875180297,6.122103616));
#162335=CARTESIAN_POINT('Ctrl Pts',(-3.559163733,0.809946053,6.316237292));
#162336=CARTESIAN_POINT('Ctrl Pts',(-3.54724828593257,0.807689868414112,
6.32295157855468));
#162337=CARTESIAN_POINT('Ctrl Pts',(-3.53533283886516,0.805433683828222,
6.32966586510928));
#162338=CARTESIAN_POINT('Ctrl Pts',(-4.56897239578246,0.940837228,5.94830889693276));
#162339=CARTESIAN_POINT('Ctrl Pts',(-4.24452340803253,0.875180297,6.19752232790587));
#162340=CARTESIAN_POINT('Ctrl Pts',(-3.89489332643019,0.809946053,6.40996828921937));
#162341=CARTESIAN_POINT('Ctrl Pts',(-3.88280105782242,0.807689868414112,
6.41731592251532));
#162342=CARTESIAN_POINT('Ctrl Pts',(-3.87070878921457,0.805433683828225,
6.42466355581122));
#162343=CARTESIAN_POINT('',(-3.89419951934794,0.809946052265047,6.40977460218573));
#162344=CARTESIAN_POINT('Origin',(0.117388635218625,0.946416084216885,-0.151261912564934));
#162345=CARTESIAN_POINT('',(-3.72668161723396,0.809946053334091,6.36300593903434));
#162346=CARTESIAN_POINT('Origin',(-7.9580439460436E-14,0.901573517999945,
1.06251812903579E-13));
#162347=CARTESIAN_POINT('Origin',(0.101098668520509,0.803568548821323,-0.164434834408524));
#162348=CARTESIAN_POINT('Origin',(0.13633379929227,0.94634946544834,-0.128939078902941));
#162349=CARTESIAN_POINT('Ctrl Pts',(-3.559163733,0.809946053,6.316237292));
#162350=CARTESIAN_POINT('Ctrl Pts',(-3.214652856,0.875601501,6.51036720800001));
#162351=CARTESIAN_POINT('Ctrl Pts',(-2.85107144,0.940829639,6.66587516));
#162352=CARTESIAN_POINT('Ctrl Pts',(-3.465626441,0.809946053,6.651273064));
#162353=CARTESIAN_POINT('Ctrl Pts',(-3.102841477,0.875601501,6.840301112));
#162354=CARTESIAN_POINT('Ctrl Pts',(-2.721649282,0.940829639,6.988749902));
#162355=CARTESIAN_POINT('',(-3.46562642958225,0.809946052007886,6.65127306832622));
#162356=CARTESIAN_POINT('',(-2.95436459608682,0.90066950062014,6.89360064336847));
#162357=CARTESIAN_POINT('Origin',(0.0899083630963088,0.803573330762241,
-0.170319809647436));
#162358=CARTESIAN_POINT('Ctrl Pts',(-2.85539439212087,0.940053944205486,
6.66402454021118));
#162359=CARTESIAN_POINT('Ctrl Pts',(-2.87190456469636,0.933168237788074,
6.70221560956731));
#162360=CARTESIAN_POINT('Ctrl Pts',(-2.88841473462254,0.926448448815871,
6.74046360253844));
#162361=CARTESIAN_POINT('Ctrl Pts',(-2.92139824827267,0.913330774428465,
6.81697715038138));
#162362=CARTESIAN_POINT('Ctrl Pts',(-2.93789004469382,0.906925555292992,
6.85528551900787));
#162363=CARTESIAN_POINT('Ctrl Pts',(-2.95436459778852,0.900669500620776,
6.89360064263689));
#162364=CARTESIAN_POINT('',(-3.51239507107219,0.809946050061996,6.48375518662845));
#162365=CARTESIAN_POINT('Origin',(3.7398469737715E-12,0.714028548000245,
-8.67752050770498E-12));
#162366=CARTESIAN_POINT('',(-2.77562550215833,0.750000003027913,6.96748898868309));
#162367=CARTESIAN_POINT('',(-2.93667239101668,0.714243089168973,6.8622795164615));
#162368=CARTESIAN_POINT('Origin',(1.33273820257263,0.473612193361007,0.590704469769952));
#162369=CARTESIAN_POINT('',(-3.12690324859456,0.750000003690145,6.81707239937356));
#162370=CARTESIAN_POINT('Origin',(0.,0.750000005282026,0.));
#162371=CARTESIAN_POINT('Origin',(-1.23048643239192,0.692072905717779,-0.771849190163528));
#162372=CARTESIAN_POINT('Ctrl Pts',(-2.859730162,0.940837228,6.662165068));
#162373=CARTESIAN_POINT('Ctrl Pts',(-2.496344072,0.875180297,6.818148319));
#162374=CARTESIAN_POINT('Ctrl Pts',(-2.118148151,0.809946053,6.933682168));
#162375=CARTESIAN_POINT('Ctrl Pts',(-2.10506790742243,0.807689868430738,
6.93767800931519));
#162376=CARTESIAN_POINT('Ctrl Pts',(-2.09198766384487,0.805433683861471,
6.9416738506305));
#162377=CARTESIAN_POINT('Ctrl Pts',(-3.18344177797812,0.940837228,6.79143474773948));
#162378=CARTESIAN_POINT('Ctrl Pts',(-2.81300470636392,0.875180297,6.96507476535259));
#162379=CARTESIAN_POINT('Ctrl Pts',(-2.42587918037184,0.809946053,7.09739372559584));
#162380=CARTESIAN_POINT('Ctrl Pts',(-2.41249009843335,0.807689868430738,
7.10197009496898));
#162381=CARTESIAN_POINT('Ctrl Pts',(-2.39910101649486,0.805433683861474,
7.10654646434213));
#162382=CARTESIAN_POINT('',(-2.42524323109857,0.809946052265054,7.09705541884243));
#162383=CARTESIAN_POINT('Origin',(0.0821273247219212,0.946416076993006,
-0.172960606955359));
#162384=CARTESIAN_POINT('',(-2.2716956840529,0.809946053334091,7.0153687836305));
#162385=CARTESIAN_POINT('Origin',(2.4459601011273E-13,0.90157351800025,
-7.43762690325056E-13));
#162386=CARTESIAN_POINT('Origin',(0.0633873961025447,0.803569528795175,
-0.182327060850242));
#162387=CARTESIAN_POINT('Origin',(0.105428588023943,0.946349169809241,-0.155232932580697));
#162388=CARTESIAN_POINT('Ctrl Pts',(-2.118148151,0.809946053,6.933682168));
#162389=CARTESIAN_POINT('Ctrl Pts',(-1.739959553,0.875601501,7.04921378));
#162390=CARTESIAN_POINT('Ctrl Pts',(-1.351448856,0.940829639,7.122926785));
#162391=CARTESIAN_POINT('Ctrl Pts',(-1.954774922,0.809946053,7.24077723800001));
#162392=CARTESIAN_POINT('Ctrl Pts',(-1.559836226,0.875601501,7.347397871));
#162393=CARTESIAN_POINT('Ctrl Pts',(-1.155643991,0.940829639,7.410430957));
#162394=CARTESIAN_POINT('',(-1.95477490990743,0.80994605211794,7.24077723976916));
#162395=CARTESIAN_POINT('',(-1.40337282846125,0.900669500586772,7.36753314887519));
#162396=CARTESIAN_POINT('Origin',(0.0511926721787856,0.803573321280154,
-0.185665675624656));
#162397=CARTESIAN_POINT('Ctrl Pts',(-1.3560685684962,0.940053944109252,
7.12204873926195));
#162398=CARTESIAN_POINT('Ctrl Pts',(-1.36398279154419,0.933168237664389,
7.16289612185191));
#162399=CARTESIAN_POINT('Ctrl Pts',(-1.37188477495162,0.926448448773429,
7.20379909602903));
#162400=CARTESIAN_POINT('Ctrl Pts',(-1.38764900142186,0.913330774387375,
7.28561428017792));
#162401=CARTESIAN_POINT('Ctrl Pts',(-1.39552006200217,0.906925555236195,
7.32657226934425));
#162402=CARTESIAN_POINT('Ctrl Pts',(-1.4033728302277,0.900669500587413,
7.36753314853664));
#162403=CARTESIAN_POINT('',(-2.03646151908971,0.809946050061996,7.08722970800272));
#162404=CARTESIAN_POINT('Origin',(-1.49132008825381E-12,0.714028547998533,
8.0183255868338E-12));
#162405=CARTESIAN_POINT('',(-1.21292876289188,0.7499999994391,7.40127039826681));
#162406=CARTESIAN_POINT('',(-1.39282737462974,0.714243089195332,7.33314099135441));
#162407=CARTESIAN_POINT('Origin',(1.42856879364856,0.473617195858478,0.290378570482246));
#162408=CARTESIAN_POINT('',(-1.58832891769568,0.750000000357976,7.32988480500076));
#162409=CARTESIAN_POINT('Origin',(0.,0.750000000000029,0.));
#162410=CARTESIAN_POINT('Origin',(-1.36764246652044,0.692075156497888,-0.489307690687903));
#162411=CARTESIAN_POINT('Ctrl Pts',(-1.360702703,0.940837228,7.12116480300001));
#162412=CARTESIAN_POINT('Ctrl Pts',(-0.97228059,0.875180297,7.19538398400001));
#162413=CARTESIAN_POINT('Ctrl Pts',(-0.578090317,0.809946053,7.226915773));
#162414=CARTESIAN_POINT('Ctrl Pts',(-0.564456894327321,0.807689868405652,
7.22800632808598));
#162415=CARTESIAN_POINT('Ctrl Pts',(-0.550823471654651,0.8054336838113,
7.22909688317197));
#162416=CARTESIAN_POINT('Ctrl Pts',(-1.64905696119033,0.940837228,7.3170006579265));
#162417=CARTESIAN_POINT('Ctrl Pts',(-1.24995303106258,0.875180297,7.40694804796768));
#162418=CARTESIAN_POINT('Ctrl Pts',(-0.843433619567465,0.809946053,7.45295291915378));
#162419=CARTESIAN_POINT('Ctrl Pts',(-0.829373782627856,0.807689868405651,
7.45454403871418));
#162420=CARTESIAN_POINT('Ctrl Pts',(-0.815313945688232,0.805433683811302,
7.45613515827444));
#162421=CARTESIAN_POINT('',(-0.842885264404958,0.809946052265035,7.45248581153022));
#162422=CARTESIAN_POINT('Origin',(0.0430257963966185,0.946416066071054,
-0.186571768009569));
#162423=CARTESIAN_POINT('',(-0.710487785962877,0.809946053334091,7.3397007811972));
#162424=CARTESIAN_POINT('Origin',(2.90349341791618E-13,0.901573517999945,
-8.2572837456496E-13));
#162425=CARTESIAN_POINT('Origin',(0.0227102601950326,0.803569500238102,
-0.19168863190188));
#162426=CARTESIAN_POINT('Origin',(0.0695932217806294,0.946349460745737,
-0.174267442991308));
#162427=CARTESIAN_POINT('Origin',(6.5199683488542E-13,0.714028547998044,
9.41868111281607E-12));
#162428=CARTESIAN_POINT('',(0.406483194510219,0.749999999382397,7.48897663951845));
#162429=CARTESIAN_POINT('',(0.216144698514716,0.714243089127833,7.46111294407942));
#162430=CARTESIAN_POINT('Origin',(1.45759410732055,0.473613193749064,-0.0235166762380834));
#162431=CARTESIAN_POINT('',(0.0245138937354052,0.750000000265122,7.49995993809237));
#162432=CARTESIAN_POINT('Origin',(0.,0.750000000000029,0.));
#162433=CARTESIAN_POINT('Origin',(-1.4408544571891,0.692072055132696,-0.1838623608636));
#162434=CARTESIAN_POINT('Origin',(-1.29562159612018E-13,0.901573518000111,
-1.69222275081538E-12));
#162435=CARTESIAN_POINT('Origin',(-0.0190280583507755,0.803569332138143,
-0.192089151140023));
#162436=CARTESIAN_POINT('',(-0.352520287816385,0.809946052007895,7.49171071413411));
#162437=CARTESIAN_POINT('Origin',(0.0100831895880892,0.803573329523321,
-0.192329770834291));
#162438=CARTESIAN_POINT('Origin',(0.0305037823483433,0.946349178008734,
-0.185153758430255));
#162439=CARTESIAN_POINT('Ctrl Pts',(-0.578090316999999,0.809946053,7.226915773));
#162440=CARTESIAN_POINT('Ctrl Pts',(-0.183907677,0.875601501,7.258446951));
#162441=CARTESIAN_POINT('Ctrl Pts',(0.211365974,0.940829639,7.246918271));
#162442=CARTESIAN_POINT('Ctrl Pts',(-0.3525203,0.809946053,7.491710715));
#162443=CARTESIAN_POINT('Ctrl Pts',(0.056105233,0.875601501,7.510938472));
#162444=CARTESIAN_POINT('Ctrl Pts',(0.464397928,0.940829639,7.485608497));
#162445=CARTESIAN_POINT('',(-0.465305290421314,0.809946050061996,7.35931324514306));
#162446=CARTESIAN_POINT('Origin',(-6.831,5.5,-6.831));
#162447=CARTESIAN_POINT('Ctrl Pts',(-0.0319404048748598,0.679837254,7.50015957748802));
#162448=CARTESIAN_POINT('Ctrl Pts',(0.374474514429064,0.744719353,7.50189034821298));
#162449=CARTESIAN_POINT('Ctrl Pts',(0.778696744357235,0.809946053,7.4596947157045));
#162450=CARTESIAN_POINT('Ctrl Pts',(0.784807551964174,0.810932114094676,
7.45905682552177));
#162451=CARTESIAN_POINT('Ctrl Pts',(0.790918359571115,0.811918175189354,
7.45841893533904));
#162452=CARTESIAN_POINT('Ctrl Pts',(0.207112381,0.679837254,7.247041083));
#162453=CARTESIAN_POINT('Ctrl Pts',(0.599811441,0.744719353,7.23581818000001));
#162454=CARTESIAN_POINT('Ctrl Pts',(0.988998379,0.809946053,7.182226828));
#162455=CARTESIAN_POINT('Ctrl Pts',(0.994881891397807,0.810932114094676,
7.18141666364678));
#162456=CARTESIAN_POINT('Ctrl Pts',(1.00076540379561,0.811918175189354,
7.18060649929357));
#162457=CARTESIAN_POINT('',(0.211783654916351,0.680609079917163,7.24690609400179));
#162458=CARTESIAN_POINT('Origin',(0.680510006550487,-0.209901599065594,
14.713132500196));
#162459=CARTESIAN_POINT('Origin',(-0.0261189597533898,0.803568149720519,
-0.197293460469613));
#162460=CARTESIAN_POINT('Ctrl Pts',(1.266217779,0.809946053,7.392340126));
#162461=CARTESIAN_POINT('Ctrl Pts',(1.672049896,0.744288122,7.32282603));
#162462=CARTESIAN_POINT('Ctrl Pts',(2.067833513,0.679844992,7.209304028));
#162463=CARTESIAN_POINT('Ctrl Pts',(0.988998379000001,0.809946053,7.182226828));
#162464=CARTESIAN_POINT('Ctrl Pts',(1.383295485,0.744288122,7.127931801));
#162465=CARTESIAN_POINT('Ctrl Pts',(1.769279415,0.679844992,7.030800122));
#162466=CARTESIAN_POINT('',(1.76470286410966,0.680609079808175,7.03195023234919));
#162467=CARTESIAN_POINT('Origin',(-0.00355486455109438,0.946280588255798,
-0.191345552750808));
#162468=CARTESIAN_POINT('Origin',(5.41950269662529,-0.919059860839161,19.7580986531931));
#162469=CARTESIAN_POINT('Ctrl Pts',(1.5811189502161,0.679837254,7.33167625657691));
#162470=CARTESIAN_POINT('Ctrl Pts',(1.97840417914827,0.744719353,7.24599936953168));
#162471=CARTESIAN_POINT('Ctrl Pts',(2.36410510414471,0.809946053,7.11789441685984));
#162472=CARTESIAN_POINT('Ctrl Pts',(2.36993592080826,0.810932114750492,
7.1159577959074));
#162473=CARTESIAN_POINT('Ctrl Pts',(2.3757667374718,0.811918176500982,7.11402117495497));
#162474=CARTESIAN_POINT('Ctrl Pts',(1.76016982,0.679837254,7.03308625));
#162475=CARTESIAN_POINT('Ctrl Pts',(2.141275202,0.744719353,6.93770704300001));
#162476=CARTESIAN_POINT('Ctrl Pts',(2.509842609,0.809946053,6.801704939));
#162477=CARTESIAN_POINT('Ctrl Pts',(2.51541441046351,0.810932114750492,
6.79964893321188));
#162478=CARTESIAN_POINT('Ctrl Pts',(2.52098621192704,0.811918176500982,
6.79759292742373));
#162479=CARTESIAN_POINT('Origin',(-0.0679205186180731,0.803568141971726,
-0.187065872158867));
#162480=CARTESIAN_POINT('Ctrl Pts',(2.825748922,0.809946053,6.947311928));
#162481=CARTESIAN_POINT('Ctrl Pts',(3.207149434,0.744288122,6.792181124));
#162482=CARTESIAN_POINT('Ctrl Pts',(3.569275975,0.679844992,6.596231425));
#162483=CARTESIAN_POINT('Ctrl Pts',(2.509842609,0.809946053,6.801704939));
#162484=CARTESIAN_POINT('Ctrl Pts',(2.883249442,0.744288122,6.663917077));
#162485=CARTESIAN_POINT('Ctrl Pts',(3.239328843,0.679844992,6.486081147));
#162486=CARTESIAN_POINT('',(3.23510652851057,0.68060907995182,6.48818819109484));
#162487=CARTESIAN_POINT('Origin',(-0.0446053175177707,0.946280595435742,
-0.186107667924471));
#162488=CARTESIAN_POINT('Origin',(9.53942525657404,-0.918876384710192,18.1296796878941));
#162489=CARTESIAN_POINT('Ctrl Pts',(3.12024693994115,0.679837254,6.82037190337756));
#162490=CARTESIAN_POINT('Ctrl Pts',(3.4898258629797,0.744719353,6.65129351328347));
#162491=CARTESIAN_POINT('Ctrl Pts',(3.8389705365879,0.809946053,6.44326928575995));
#162492=CARTESIAN_POINT('Ctrl Pts',(3.84424871724141,0.810932115031176,
6.44012448781177));
#162493=CARTESIAN_POINT('Ctrl Pts',(3.84952689789492,0.811918177062351,
6.43697968986362));
#162494=CARTESIAN_POINT('Ctrl Pts',(3.230923675,0.679837254,6.490272121));
#162495=CARTESIAN_POINT('Ctrl Pts',(3.582615315,0.744719353,6.315196435));
#162496=CARTESIAN_POINT('Ctrl Pts',(3.913329389,0.809946053,6.10314288700001));
#162497=CARTESIAN_POINT('Ctrl Pts',(3.91832894580031,0.810932115031176,
6.09993717596052));
#162498=CARTESIAN_POINT('Ctrl Pts',(3.92332850260062,0.811918177062351,
6.09673146492104));
#162499=CARTESIAN_POINT('Origin',(-0.106546367331508,0.803568122919176,
-0.168091762861144));
#162500=CARTESIAN_POINT('Ctrl Pts',(4.253151186,0.809946053,6.177435146));
#162501=CARTESIAN_POINT('Ctrl Pts',(4.592286229,0.744288122,5.943941379));
#162502=CARTESIAN_POINT('Ctrl Pts',(4.903823059,0.679844992,5.674726372));
#162503=CARTESIAN_POINT('Ctrl Pts',(3.913329389,0.809946053,6.103142887));
#162504=CARTESIAN_POINT('Ctrl Pts',(4.24838586,0.744288122,5.888304997));
#162505=CARTESIAN_POINT('Ctrl Pts',(4.557910854,0.679844992,5.638080227));
#162506=CARTESIAN_POINT('',(4.55424020729894,0.680609079944476,5.64104568189662));
#162507=CARTESIAN_POINT('Origin',(-0.083570205332133,0.946280566572918,
-0.172167845103236));
#162508=CARTESIAN_POINT('Origin',(13.2145781900805,-0.919019804357942,15.6560946877858));
#162509=CARTESIAN_POINT('Ctrl Pts',(4.51347565132549,0.679837254,5.99015454003778));
#162510=CARTESIAN_POINT('Ctrl Pts',(4.83806716842846,0.744719353,5.74558056475493));
#162511=CARTESIAN_POINT('Ctrl Pts',(5.13432997385664,0.809946053,5.46736404465009));
#162512=CARTESIAN_POINT('Ctrl Pts',(5.13880871367383,0.810932114743429,
5.46315811875066));
#162513=CARTESIAN_POINT('Ctrl Pts',(5.14328745349099,0.811918176486856,
5.4589521928512));
#162514=CARTESIAN_POINT('Ctrl Pts',(4.55060313,0.679837254,5.643980081));
#162515=CARTESIAN_POINT('Ctrl Pts',(4.856436318,0.744719353,5.39739426));
#162516=CARTESIAN_POINT('Ctrl Pts',(5.133833235,0.809946053,5.119204656));
#162517=CARTESIAN_POINT('Ctrl Pts',(5.13802677058587,0.810932114743429,
5.11499913700358));
#162518=CARTESIAN_POINT('Ctrl Pts',(5.14222030617174,0.811918176486856,
5.11079361800716));
#162519=CARTESIAN_POINT('Origin',(-0.140189871307624,0.803568097858735,
-0.141257253492768));
#162520=CARTESIAN_POINT('Ctrl Pts',(5.481680828,0.809946053,5.11870836300001));
#162521=CARTESIAN_POINT('Ctrl Pts',(5.762692823,0.744288122,4.81776954));
#162522=CARTESIAN_POINT('Ctrl Pts',(6.00907282800001,0.679844992,4.487877421));
#162523=CARTESIAN_POINT('Ctrl Pts',(5.133833235,0.809946053,5.119204656));
#162524=CARTESIAN_POINT('Ctrl Pts',(5.414872477,0.744288122,4.83736232));
#162525=CARTESIAN_POINT('Ctrl Pts',(5.663370019,0.679844992,4.526448942));
#162526=CARTESIAN_POINT('',(5.66042267655931,0.680609079843256,4.53013414747271));
#162527=CARTESIAN_POINT('Origin',(-0.118627125200667,0.946280598598074,
-0.150177324068743));
#162528=CARTESIAN_POINT('Origin',(16.2709444742823,-0.918980550492197,12.4491087468896));
#162529=CARTESIAN_POINT('Ctrl Pts',(5.69565925739822,0.679837254,4.87984420868066));
#162530=CARTESIAN_POINT('Ctrl Pts',(5.96008583006358,0.744719353,4.57121065596384));
#162531=CARTESIAN_POINT('Ctrl Pts',(6.1896138473021,0.809946053,4.23581093640374));
#162532=CARTESIAN_POINT('Ctrl Pts',(6.19308372685913,0.810932114726258,
4.2307405461118));
#162533=CARTESIAN_POINT('Ctrl Pts',(6.19655360641617,0.811918176452514,
4.22567015581985));
#162534=CARTESIAN_POINT('Ctrl Pts',(5.65750144,0.679837254,4.533781805));
#162535=CARTESIAN_POINT('Ctrl Pts',(5.903175755,0.744719353,4.227215929));
#162536=CARTESIAN_POINT('Ctrl Pts',(6.114284746,0.809946053,3.895898106));
#162537=CARTESIAN_POINT('Ctrl Pts',(6.11747617674989,0.810932114726258,
3.89088942359714));
#162538=CARTESIAN_POINT('Ctrl Pts',(6.12066760749978,0.811918176452514,
3.88588074119426));
#162539=CARTESIAN_POINT('Origin',(-0.167278719693816,0.803568145827063,
-0.107818265580796));
#162540=CARTESIAN_POINT('Ctrl Pts',(6.453893166,0.809946053,3.820636465));
#162541=CARTESIAN_POINT('Ctrl Pts',(6.663642306,0.744288122,3.466324153));
#162542=CARTESIAN_POINT('Ctrl Pts',(6.833345029,0.679844992,3.09118031));
#162543=CARTESIAN_POINT('Ctrl Pts',(6.114284746,0.809946053,3.895898106));
#162544=CARTESIAN_POINT('Ctrl Pts',(6.328165675,0.744288122,3.560229957));
#162545=CARTESIAN_POINT('Ctrl Pts',(6.504016297,0.679844992,3.203165935));
#162546=CARTESIAN_POINT('',(6.50193007002564,0.680609079906773,3.20739857317831));
#162547=CARTESIAN_POINT('Origin',(-0.148137647194987,0.946280588273123,
-0.121165073592281));
#162548=CARTESIAN_POINT('Origin',(18.5668200740015,-0.919005909663884,8.6603200934186));
#162549=CARTESIAN_POINT('Ctrl Pts',(6.61152016658401,0.679837254,3.54135778485581));
#162550=CARTESIAN_POINT('Ctrl Pts',(6.803417501554,0.744719353,3.18309601629077));
#162551=CARTESIAN_POINT('Ctrl Pts',(6.9554782573042,0.809946053,2.8061960172087));
#162552=CARTESIAN_POINT('Ctrl Pts',(6.9577770284796,0.810932114506048,2.80049824956562));
#162553=CARTESIAN_POINT('Ctrl Pts',(6.96007579965497,0.811918176012098,
2.79480048192255));
#162554=CARTESIAN_POINT('Ctrl Pts',(6.499861271,0.679837254,3.211588931));
#162555=CARTESIAN_POINT('Ctrl Pts',(6.673889256,0.744719353,2.859377679));
#162556=CARTESIAN_POINT('Ctrl Pts',(6.808839097,0.809946053,2.49042369));
#162557=CARTESIAN_POINT('Ctrl Pts',(6.81087919474306,0.810932114506048,
2.48484604578289));
#162558=CARTESIAN_POINT('Ctrl Pts',(6.81291929248613,0.811918176012098,
2.47926840156579));
#162559=CARTESIAN_POINT('Origin',(-0.18654538333014,0.803568163185117,-0.0693374685299075));
#162560=CARTESIAN_POINT('Ctrl Pts',(7.124328633,0.809946053,2.343915853));
#162561=CARTESIAN_POINT('Ctrl Pts',(7.253007281,0.744288122,1.9527973));
#162562=CARTESIAN_POINT('Ctrl Pts',(7.33809761200001,0.679844992,1.549943043));
#162563=CARTESIAN_POINT('Ctrl Pts',(6.808839097,0.809946053,2.49042369));
#162564=CARTESIAN_POINT('Ctrl Pts',(6.945560879,0.744288122,2.116625199));
#162565=CARTESIAN_POINT('Ctrl Pts',(7.040542002,0.679844992,1.730106449));
#162566=CARTESIAN_POINT('',(7.03941444172257,0.680609079894364,1.73468860760923));
#162567=CARTESIAN_POINT('Origin',(-0.170721307163793,0.946280565852508,
-0.0864871263428832));
#162568=CARTESIAN_POINT('Origin',(19.9937280304115,-0.918922005754596,4.46638008064186));
#162569=CARTESIAN_POINT('Ctrl Pts',(7.21823374108708,0.679837254,2.03728140705634));
#162570=CARTESIAN_POINT('Ctrl Pts',(7.32862893308932,0.744719353,1.64614334500659));
#162571=CARTESIAN_POINT('Ctrl Pts',(7.39611223383465,0.809946053,1.2453664911386));
#162572=CARTESIAN_POINT('Ctrl Pts',(7.39713240963888,0.810932114742612,
1.23930776483597));
#162573=CARTESIAN_POINT('Ctrl Pts',(7.39815258544312,0.811918176485222,
1.23324903853334));
#162574=CARTESIAN_POINT('Ctrl Pts',(7.038294813,0.679837254,1.739225727));
#162575=CARTESIAN_POINT('Ctrl Pts',(7.13253911200001,0.744719353,1.357838106));
#162576=CARTESIAN_POINT('Ctrl Pts',(7.18501969900001,0.809946053,0.96849983));
#162577=CARTESIAN_POINT('Ctrl Pts',(7.18581307194498,0.810932114742612,
0.962614025890673));
#162578=CARTESIAN_POINT('Ctrl Pts',(7.18660644488997,0.811918176485222,
0.956728221781344));
#162579=CARTESIAN_POINT('Origin',(-0.197089526502294,0.803568141080806,
-0.0276146383221554));
#162580=CARTESIAN_POINT('Ctrl Pts',(7.461638412,0.809946053,0.75759634));
#162581=CARTESIAN_POINT('Ctrl Pts',(7.503229697,0.744288122,0.347959816));
#162582=CARTESIAN_POINT('Ctrl Pts',(7.499728906,0.679844992,-0.063767838));
#162583=CARTESIAN_POINT('Ctrl Pts',(7.185019699,0.809946053,0.96849983));
#162584=CARTESIAN_POINT('Ctrl Pts',(7.238189376,0.744288122,0.574049398));
#162585=CARTESIAN_POINT('Ctrl Pts',(7.247859787,0.679844992,0.176149108));
#162586=CARTESIAN_POINT('',(7.24774361921728,0.680609079812669,0.180866530829771));
#162587=CARTESIAN_POINT('Origin',(-0.185321732206588,0.946280559786437,
-0.0477650476507504));
#162588=CARTESIAN_POINT('Origin',(20.4864779452742,-0.918914818035844,0.063898929278453));
#162589=CARTESIAN_POINT('Ctrl Pts',(7.48743072874736,0.679837254,0.437944015219146));
#162590=CARTESIAN_POINT('Ctrl Pts',(7.51116182146427,0.744719353,0.0322188409795213));
#162591=CARTESIAN_POINT('Ctrl Pts',(7.49091222296789,0.809946053,-0.373694987688807));
#162592=CARTESIAN_POINT('Ctrl Pts',(7.49060610072142,0.810932114226693,
-0.37983136876938));
#162593=CARTESIAN_POINT('Ctrl Pts',(7.49029997847496,0.811918175453385,
-0.385967749849952));
#162594=CARTESIAN_POINT('Ctrl Pts',(7.24762551100001,0.679837254,0.185538262));
#162595=CARTESIAN_POINT('Ctrl Pts',(7.257679367,0.744719353,-0.207192467));
#162596=CARTESIAN_POINT('Ctrl Pts',(7.225236766,0.809946053,-0.598710006));
#162597=CARTESIAN_POINT('Ctrl Pts',(7.22474631667573,0.810932114226693,
-0.604628751924261));
#162598=CARTESIAN_POINT('Ctrl Pts',(7.22425586735147,0.811918175453385,
-0.610547497848522));
#162599=CARTESIAN_POINT('Origin',(-0.198417951097591,0.803568118635443,
0.0153993916838719));
#162600=CARTESIAN_POINT('Ctrl Pts',(7.450050271,0.809946053,-0.864147535));
#162601=CARTESIAN_POINT('Ctrl Pts',(7.402609431,0.744288122,-1.273147882));
#162602=CARTESIAN_POINT('Ctrl Pts',(7.310681212,0.679844992,-1.674497005));
#162603=CARTESIAN_POINT('Ctrl Pts',(7.225236766,0.809946053,-0.598710006));
#162604=CARTESIAN_POINT('Ctrl Pts',(7.192368183,0.744288122,-0.995368314));
#162605=CARTESIAN_POINT('Ctrl Pts',(7.116275704,0.679844992,-1.386044769));
#162606=CARTESIAN_POINT('',(7.11717635838003,0.680609079831188,-1.38141266477938));
#162607=CARTESIAN_POINT('Origin',(-0.191257343635393,0.946280592086966,
-0.00680959738268955));
#162608=CARTESIAN_POINT('Origin',(20.0210910547472,-0.918903429656103,-4.34154776765039));
#162609=CARTESIAN_POINT('Ctrl Pts',(7.40652377624533,0.679837254,-1.18187115244431));
#162610=CARTESIAN_POINT('Ctrl Pts',(7.34248112992593,0.744719353,-1.58321218171481));
#162611=CARTESIAN_POINT('Ctrl Pts',(7.23544548158936,0.809946053,-1.97528290532036));
#162612=CARTESIAN_POINT('Ctrl Pts',(7.23382737490774,0.810932114753538,
-1.98121001715079));
#162613=CARTESIAN_POINT('Ctrl Pts',(7.23220926822613,0.811918176507078,
-1.98713712898122));
#162614=CARTESIAN_POINT('Ctrl Pts',(7.118065296,0.679837254,-1.376824766));
#162615=CARTESIAN_POINT('Ctrl Pts',(7.0434586,0.744719353,-1.762534951));
#162616=CARTESIAN_POINT('Ctrl Pts',(6.927609792,0.809946053,-2.137924827));
#162617=CARTESIAN_POINT('Ctrl Pts',(6.9258584527668,0.810932114753538,-2.14359976685422));
#162618=CARTESIAN_POINT('Ctrl Pts',(6.92410711353362,0.811918176507078,
-2.14927470670844));
#162619=CARTESIAN_POINT('Origin',(-0.190468597948358,0.803568146623334,
0.0576933426523757));
#162620=CARTESIAN_POINT('Ctrl Pts',(7.090106059,0.809946053,-2.445484832));
#162621=CARTESIAN_POINT('Ctrl Pts',(6.955851376,0.744288122,-2.8347246));
#162622=CARTESIAN_POINT('Ctrl Pts',(6.779794189,0.679844992,-3.206928554));
#162623=CARTESIAN_POINT('Ctrl Pts',(6.927609792,0.809946053,-2.137924827));
#162624=CARTESIAN_POINT('Ctrl Pts',(6.81023984700001,0.744288122,-2.518243711));
#162625=CARTESIAN_POINT('Ctrl Pts',(6.65194247900001,0.679844992,-2.883428734));
#162626=CARTESIAN_POINT('',(6.6538178404657,0.680609079934148,-2.8790985384958));
#162627=CARTESIAN_POINT('Origin',(-0.188249734722257,0.946280573583837,
0.0344642921835409));
#162628=CARTESIAN_POINT('Origin',(18.6195617475465,-0.918877917958552,-8.54391955967953));
#162629=CARTESIAN_POINT('Ctrl Pts',(6.97929600465152,0.679837254,-2.74642333766407));
#162630=CARTESIAN_POINT('Ctrl Pts',(6.83047418193199,0.744719353,-3.12461396142994));
#162631=CARTESIAN_POINT('Ctrl Pts',(6.64165735171076,0.809946053,-3.48450878846813));
#162632=CARTESIAN_POINT('Ctrl Pts',(6.63880292162864,0.810932114753182,
-3.48994948260275));
#162633=CARTESIAN_POINT('Ctrl Pts',(6.63594849154651,0.811918176506363,
-3.49539017673736));
#162634=CARTESIAN_POINT('Ctrl Pts',(6.655672259,0.679837254,-2.874808998));
#162635=CARTESIAN_POINT('Ctrl Pts',(6.49989353800001,0.744719353,-3.235463259));
#162636=CARTESIAN_POINT('Ctrl Pts',(6.306055484,0.809946053,-3.577172659));
#162637=CARTESIAN_POINT('Ctrl Pts',(6.30312514578941,0.810932114753182,
-3.58233843574545));
#162638=CARTESIAN_POINT('Ctrl Pts',(6.30019480757882,0.811918176506363,
-3.58750421249091));
#162639=CARTESIAN_POINT('Origin',(-0.173613336813595,0.803568116995496,
0.0972897037180659));
#162640=CARTESIAN_POINT('Ctrl Pts',(6.398636369,0.809946053,-3.912473977));
#162641=CARTESIAN_POINT('Ctrl Pts',(6.183845441,0.744288122,-4.263752746));
#162642=CARTESIAN_POINT('Ctrl Pts',(5.93189152599999,0.679844992,-4.589407688));
#162643=CARTESIAN_POINT('Ctrl Pts',(6.306055484,0.809946053,-3.577172659));
#162644=CARTESIAN_POINT('Ctrl Pts',(6.109672265,0.744288122,-3.92336883));
#162645=CARTESIAN_POINT('Ctrl Pts',(5.876571816,0.679844992,-4.245986775));
#162646=CARTESIAN_POINT('',(5.87933419646206,0.680609079917205,-4.24216096441692));
#162647=CARTESIAN_POINT('Origin',(-0.176439515626958,0.946280541725487,
0.0741265169878685));
#162648=CARTESIAN_POINT('Origin',(16.348679514349,-0.919047985408652,-12.3476875756904));
#162649=CARTESIAN_POINT('Ctrl Pts',(6.22572410826749,0.679837254,-4.1825558210505));
#162650=CARTESIAN_POINT('Ctrl Pts',(5.9990818528282,0.744719353,-4.51991226497366));
#162651=CARTESIAN_POINT('Ctrl Pts',(5.73731270545755,0.809946053,-4.83080291392708));
#162652=CARTESIAN_POINT('Ctrl Pts',(5.73335542199936,0.810932114740028,
-4.83550278950358));
#162653=CARTESIAN_POINT('Ctrl Pts',(5.72939813854119,0.811918176480054,
-4.84020266508007));
#162654=CARTESIAN_POINT('Ctrl Pts',(5.88206738500001,0.679837254,-4.238370357));
#162655=CARTESIAN_POINT('Ctrl Pts',(5.65240067800001,0.744719353,-4.557104901));
#162656=CARTESIAN_POINT('Ctrl Pts',(5.38963703,0.809946053,-4.849155874));
#162657=CARTESIAN_POINT('Ctrl Pts',(5.38566471222273,0.810932114740028,
-4.85357094161209));
#162658=CARTESIAN_POINT('Ctrl Pts',(5.38169239444545,0.811918176480054,
-4.85798600922415));
#162659=CARTESIAN_POINT('Origin',(-0.148639930843035,0.803568108054348,
0.13233683330104));
#162660=CARTESIAN_POINT('Ctrl Pts',(5.407973553,0.809946053,-5.196520186));
#162661=CARTESIAN_POINT('Ctrl Pts',(5.122689766,0.744288122,-5.493412553));
#162662=CARTESIAN_POINT('Ctrl Pts',(4.806620207,0.679844992,-5.75729121900001));
#162663=CARTESIAN_POINT('Ctrl Pts',(5.38963702999999,0.809946053,-4.849155874));
#162664=CARTESIAN_POINT('Ctrl Pts',(5.123423198,0.744288122,-5.145041583));
#162665=CARTESIAN_POINT('Ctrl Pts',(4.826419186,0.679844992,-5.410007194));
#162666=CARTESIAN_POINT('',(4.8299394211557,0.680609079820267,-5.4068646602954));
#162667=CARTESIAN_POINT('Origin',(-0.156379663221219,0.946280575238907,
0.110322979496779));
#162668=CARTESIAN_POINT('Origin',(13.3109697368389,-0.918851572015798,-15.5721798564474));
#162669=CARTESIAN_POINT('Ctrl Pts',(5.18104427232235,0.679837254,-5.42311664268225));
#162670=CARTESIAN_POINT('Ctrl Pts',(4.88717912351137,0.744719353,-5.70386449497362));
#162671=CARTESIAN_POINT('Ctrl Pts',(4.56469769334661,0.809946053,-5.95121406393451));
#162672=CARTESIAN_POINT('Ctrl Pts',(4.55982259305757,0.810932115062118,
-5.95495336127798));
#162673=CARTESIAN_POINT('Ctrl Pts',(4.55494749276852,0.811918177124235,
-5.95869265862146));
#162674=CARTESIAN_POINT('Ctrl Pts',(4.833423576,0.679837254,-5.403750228));
#162675=CARTESIAN_POINT('Ctrl Pts',(4.540607845,0.744719353,-5.665661383));
#162676=CARTESIAN_POINT('Ctrl Pts',(4.221205138,0.809946053,-5.894397949));
#162677=CARTESIAN_POINT('Ctrl Pts',(4.21637658018686,0.810932115062118,
-5.89785586500604));
#162678=CARTESIAN_POINT('Ctrl Pts',(4.21154802237372,0.811918177124235,
-5.9013137810121));
#162679=CARTESIAN_POINT('Origin',(-0.116716233245275,0.803568103427335,
0.161195976465628));
#162680=CARTESIAN_POINT('Ctrl Pts',(4.164439905,0.809946053,-6.237582888));
#162681=CARTESIAN_POINT('Ctrl Pts',(3.822002811,0.744288122,-6.46620649400001));
#162682=CARTESIAN_POINT('Ctrl Pts',(3.45659667,0.679844992,-6.655970212));
#162683=CARTESIAN_POINT('Ctrl Pts',(4.221205138,0.809946053,-5.894397949));
#162684=CARTESIAN_POINT('Ctrl Pts',(3.897608556,0.744288122,-6.12613791));
#162685=CARTESIAN_POINT('Ctrl Pts',(3.55058856,0.679844992,-6.321061689));
#162686=CARTESIAN_POINT('',(3.55470204592073,0.680609079806426,-6.31874937276602));
#162687=CARTESIAN_POINT('Origin',(-0.129007325136785,0.946280573576781,
0.141360544234609));
#162688=CARTESIAN_POINT('Origin',(9.65240306669682,-0.91890051911108,-18.0699482044124));
#162689=CARTESIAN_POINT('Ctrl Pts',(3.89410456449864,0.679837254,-6.4100985573269));
#162690=CARTESIAN_POINT('Ctrl Pts',(3.54675733026341,0.744719353,-6.62111036018678));
#162691=CARTESIAN_POINT('Ctrl Pts',(3.17864249022696,0.809946053,-6.79335305972249));
#162692=CARTESIAN_POINT('Ctrl Pts',(3.17307753073869,0.810932114694818,
-6.79595693096271));
#162693=CARTESIAN_POINT('Ctrl Pts',(3.16751257125042,0.811918176389634,
-6.79856080220291));
#162694=CARTESIAN_POINT('Ctrl Pts',(3.558774254,0.679837254,-6.316456745));
#162695=CARTESIAN_POINT('Ctrl Pts',(3.216501235,0.744719353,-6.509297835));
#162696=CARTESIAN_POINT('Ctrl Pts',(2.855394386,0.809946053,-6.664024527));
#162697=CARTESIAN_POINT('Ctrl Pts',(2.84993536950008,0.810932114694818,
-6.66636360078645));
#162698=CARTESIAN_POINT('Ctrl Pts',(2.84447635300018,0.811918176389633,
-6.66870267457291));
#162699=CARTESIAN_POINT('Origin',(-0.0793350860434211,0.803568151356397,
0.18251784667311));
#162700=CARTESIAN_POINT('Ctrl Pts',(2.726181675,0.809946053,-6.986983146));
#162701=CARTESIAN_POINT('Ctrl Pts',(2.342603253,0.744288122,-7.136647807));
#162702=CARTESIAN_POINT('Ctrl Pts',(1.944946514,0.679844992,-7.243423435));
#162703=CARTESIAN_POINT('Ctrl Pts',(2.855394386,0.809946053,-6.664024527));
#162704=CARTESIAN_POINT('Ctrl Pts',(2.489546071,0.744288122,-6.82078283800001));
#162705=CARTESIAN_POINT('Ctrl Pts',(2.108736358,0.679844992,-6.936550365));
#162706=CARTESIAN_POINT('',(2.11325075223419,0.680609079948131,-6.9351763867474));
#162707=CARTESIAN_POINT('Origin',(-0.0956029385533522,0.946280548888431,
0.165788545440595));
#162708=CARTESIAN_POINT('Origin',(5.54219511633975,-0.918869543282762,-19.7223186336196));
#162709=CARTESIAN_POINT('Ctrl Pts',(2.42508085481774,0.679837254,-7.09735138772923));
#162710=CARTESIAN_POINT('Ctrl Pts',(2.04049310563864,0.744719353,-7.22876046326209));
#162711=CARTESIAN_POINT('Ctrl Pts',(1.64395749819145,0.809946053,-7.31784241489472));
#162712=CARTESIAN_POINT('Ctrl Pts',(1.6379628885056,0.810932114781724,-7.31918910739864));
#162713=CARTESIAN_POINT('Ctrl Pts',(1.63196827881974,0.811918176563451,
-7.32053579990259));
#162714=CARTESIAN_POINT('Ctrl Pts',(2.117720602,0.679837254,-6.933812764));
#162715=CARTESIAN_POINT('Ctrl Pts',(1.741994603,0.744719353,-7.048566756));
#162716=CARTESIAN_POINT('Ctrl Pts',(1.356068566,0.809946053,-7.122048725));
#162717=CARTESIAN_POINT('Ctrl Pts',(1.35023434603091,0.810932114781724,
-7.12315958544943));
#162718=CARTESIAN_POINT('Ctrl Pts',(1.34440012606181,0.811918176563451,
-7.12427044589887));
#162719=CARTESIAN_POINT('Origin',(-0.0382443479738842,0.803568118805305,
0.195305453929068));
#162720=CARTESIAN_POINT('Ctrl Pts',(1.16045022,0.809946053,-7.409679837));
#162721=CARTESIAN_POINT('Ctrl Pts',(0.75366617,0.744288122,-7.473387399));
#162722=CARTESIAN_POINT('Ctrl Pts',(0.342352821,0.679844992,-7.49218222900001));
#162723=CARTESIAN_POINT('Ctrl Pts',(1.356068566,0.809946053,-7.122048725));
#162724=CARTESIAN_POINT('Ctrl Pts',(0.965075178000001,0.744288122,-7.19649554));
#162725=CARTESIAN_POINT('Ctrl Pts',(0.568281989,0.679844992,-7.227693656));
#162726=CARTESIAN_POINT('',(0.572986203812444,0.680609079901549,-7.22732226094589));
#162727=CARTESIAN_POINT('Origin',(-0.0577281455887602,0.946280608526164,
0.182464146390054));
#162728=CARTESIAN_POINT('Origin',(1.17292302164358,-0.918918442993689,-20.4529436923275));
#162729=CARTESIAN_POINT('Ctrl Pts',(0.842663060359861,0.679837254,-7.45273995492195));
#162730=CARTESIAN_POINT('Ctrl Pts',(0.43881769232648,0.744719353,-7.49840176169412));
#162731=CARTESIAN_POINT('Ctrl Pts',(0.0324028797431824,0.809946053,-7.50015759317151));
#162732=CARTESIAN_POINT('Ctrl Pts',(0.0262589216279636,0.810932114778227,
-7.50018413687691));
#162733=CARTESIAN_POINT('Ctrl Pts',(0.020114963512745,0.811918176556457,
-7.50021068058231));
#162734=CARTESIAN_POINT('Ctrl Pts',(0.577644689,0.679837254,-7.226951405));
#162735=CARTESIAN_POINT('Ctrl Pts',(0.186034238,0.744719353,-7.25825252900001));
#162736=CARTESIAN_POINT('Ctrl Pts',(-0.206665513,0.809946053,-7.24705384));
#162737=CARTESIAN_POINT('Ctrl Pts',(-0.212602134272893,0.810932114778227,
-7.2468845443099));
#162738=CARTESIAN_POINT('Ctrl Pts',(-0.218538755545785,0.811918176556456,
-7.24671524861982));
#162739=CARTESIAN_POINT('Origin',(0.00463467896617421,0.803568114703985,
0.198960813235042));
#162740=CARTESIAN_POINT('Ctrl Pts',(-0.459542598,0.809946053,-7.485908135));
#162741=CARTESIAN_POINT('Ctrl Pts',(-0.870511505,0.744288122,-7.460679703));
#162742=CARTESIAN_POINT('Ctrl Pts',(-1.276248909,0.679844992,-7.390614908));
#162743=CARTESIAN_POINT('Ctrl Pts',(-0.206665513,0.809946053,-7.24705384000001));
#162744=CARTESIAN_POINT('Ctrl Pts',(-0.604521557,0.744288122,-7.235708109));
#162745=CARTESIAN_POINT('Ctrl Pts',(-0.998744615,0.679844992,-7.180878024));
#162746=CARTESIAN_POINT('',(-0.994070543634724,0.680609079119151,-7.18152658032342));
#162747=CARTESIAN_POINT('Origin',(-0.0171541070111382,0.946280593383585,
0.190607868645933));
#162748=CARTESIAN_POINT('Origin',(-3.25137816860814,-0.918993617172282,
-20.2274616516324));
#162749=CARTESIAN_POINT('Ctrl Pts',(-0.779156723184081,0.679837254,-7.45964668465108));
#162750=CARTESIAN_POINT('Ctrl Pts',(-1.18337634970542,0.744719353,-7.41742612728615));
#162751=CARTESIAN_POINT('Ctrl Pts',(-1.58066686107051,0.809946053,-7.33177373711505));
#162752=CARTESIAN_POINT('Ctrl Pts',(-1.58667286991739,0.810932112636579,
-7.33047889367327));
#162753=CARTESIAN_POINT('Ctrl Pts',(-1.59267887876426,0.811918172273156,
-7.32918405023149));
#162754=CARTESIAN_POINT('Ctrl Pts',(-0.989441248,0.679837254,-7.182165831));
#162755=CARTESIAN_POINT('Ctrl Pts',(-1.37862488,0.744719353,-7.12855048));
#162756=CARTESIAN_POINT('Ctrl Pts',(-1.759736143,0.809946053,-7.033194773));
#162757=CARTESIAN_POINT('Ctrl Pts',(-1.76549756330012,0.810932112636579,
-7.03175324040997));
#162758=CARTESIAN_POINT('Ctrl Pts',(-1.77125898360023,0.811918172273156,
-7.03031170781994));
#162759=CARTESIAN_POINT('Origin',(0.0472970133577211,0.803568096753134,
0.193313010487212));
#162760=CARTESIAN_POINT('Ctrl Pts',(-2.058047714,0.809946053,-7.212103688));
#162761=CARTESIAN_POINT('Ctrl Pts',(-2.45398503,0.744288122,-7.099118916));
#162762=CARTESIAN_POINT('Ctrl Pts',(-2.835174659,0.679844992,-6.943470649));
#162763=CARTESIAN_POINT('Ctrl Pts',(-1.759736143,0.809946053,-7.03319477300001));
#162764=CARTESIAN_POINT('Ctrl Pts',(-2.145851537,0.744288122,-6.936587009));
#162765=CARTESIAN_POINT('Ctrl Pts',(-2.519071031,0.679844992,-6.798292516));
#162766=CARTESIAN_POINT('',(-2.51464565671269,0.680609079944213,-6.799930695879));
#162767=CARTESIAN_POINT('Origin',(0.0242221099862061,0.94628052984048,0.189839453464968));
#162768=CARTESIAN_POINT('Origin',(-7.52367615252197,-0.918977858636926,
-19.0556263464347));
#162769=CARTESIAN_POINT('Ctrl Pts',(-2.3645440035047,0.679837254,-7.1177486281266));
#162770=CARTESIAN_POINT('Ctrl Pts',(-2.75023702794865,0.744719353,-6.9896198925137));
#162771=CARTESIAN_POINT('Ctrl Pts',(-3.11982637566339,0.809946053,-6.82056429141002));
#162772=CARTESIAN_POINT('Ctrl Pts',(-3.12541363059661,0.810932115513994,
-6.81800859886343));
#162773=CARTESIAN_POINT('Ctrl Pts',(-3.13100088552983,0.811918178027987,
-6.81545290631684));
#162774=CARTESIAN_POINT('Ctrl Pts',(-2.510262011,0.679837254,-6.801550164));
#162775=CARTESIAN_POINT('Ctrl Pts',(-2.878821031,0.744719353,-6.665525334));
#162776=CARTESIAN_POINT('Ctrl Pts',(-3.230523466,0.809946053,-6.490471334));
#162777=CARTESIAN_POINT('Ctrl Pts',(-3.23584031611251,0.810932115513994,
-6.48782496085335));
#162778=CARTESIAN_POINT('Ctrl Pts',(-3.24115716622503,0.811918178027986,
-6.48517858770671));
#162779=CARTESIAN_POINT('Origin',(0.0877477662178078,0.803568115035289,
0.178625850947978));
#162780=CARTESIAN_POINT('Ctrl Pts',(-3.560320807,0.809946053,-6.601069288));
#162781=CARTESIAN_POINT('Ctrl Pts',(-3.922712942,0.744288122,-6.405611219));
#162782=CARTESIAN_POINT('Ctrl Pts',(-4.261530793,0.679844992,-6.171657419));
#162783=CARTESIAN_POINT('Ctrl Pts',(-3.230523466,0.809946053,-6.49047133400001));
#162784=CARTESIAN_POINT('Ctrl Pts',(-3.586843883,0.744288122,-6.31311881));
#162785=CARTESIAN_POINT('Ctrl Pts',(-3.921608485,0.679844992,-6.09782640700001));
#162786=CARTESIAN_POINT('',(-3.91763873447842,0.680609079056139,-6.10037761276869));
#162787=CARTESIAN_POINT('Origin',(0.0644657035781965,0.94628054675428,0.180194127610646));
#162788=CARTESIAN_POINT('Origin',(-11.444372356347,-0.919014173525902,-16.9930411751167));
#162789=CARTESIAN_POINT('Ctrl Pts',(-3.83936783438881,0.679837254,-6.44303255478497));
#162790=CARTESIAN_POINT('Ctrl Pts',(-4.18849968021581,0.744719353,-6.23498679924312));
#162791=CARTESIAN_POINT('Ctrl Pts',(-4.51310627720805,0.809946053,-5.99043283899561));
#162792=CARTESIAN_POINT('Ctrl Pts',(-4.51801350316094,0.810932114768393,
-5.98673580525775));
#162793=CARTESIAN_POINT('Ctrl Pts',(-4.52292072911385,0.811918176536784,
-5.9830387715199));
#162794=CARTESIAN_POINT('Ctrl Pts',(-3.913705713,0.679837254,-6.10290157100001));
#162795=CARTESIAN_POINT('Ctrl Pts',(-4.24440671,0.744719353,-5.890827631));
#162796=CARTESIAN_POINT('Ctrl Pts',(-4.550255102,0.809946053,-5.644260669));
#162797=CARTESIAN_POINT('Ctrl Pts',(-4.55487875161397,0.810932114768393,
-5.64053320379669));
#162798=CARTESIAN_POINT('Ctrl Pts',(-4.55950240122794,0.811918176536784,
-5.63680573859337));
#162799=CARTESIAN_POINT('Origin',(0.124095595416366,0.80356814062132,0.155586552527208));
#162800=CARTESIAN_POINT('Ctrl Pts',(-4.896117256,0.809946053,-5.681376225));
#162801=CARTESIAN_POINT('Ctrl Pts',(-5.208019157,0.744288122,-5.41258426));
#162802=CARTESIAN_POINT('Ctrl Pts',(-5.488622484,0.679844992,-5.11126434800001));
#162803=CARTESIAN_POINT('Ctrl Pts',(-4.550255102,0.809946053,-5.644260669));
#162804=CARTESIAN_POINT('Ctrl Pts',(-4.86011939600001,0.744288122,-5.394456192));
#162805=CARTESIAN_POINT('Ctrl Pts',(-5.14077588500001,0.679844992,-5.112232712));
#162806=CARTESIAN_POINT('',(-5.13744737780991,0.68060907991806,-5.1155776495944));
#162807=CARTESIAN_POINT('Origin',(0.101694863213478,0.946280537045227,0.162122989659684));
#162808=CARTESIAN_POINT('Origin',(-14.8290719530443,-0.918907507355324,
-14.1348558842815));
#162809=CARTESIAN_POINT('Ctrl Pts',(-5.13466709208186,0.679837254,-5.46704744072571));
#162810=CARTESIAN_POINT('Ctrl Pts',(-5.4309127425148,0.744719353,-5.1888126525784));
#162811=CARTESIAN_POINT('Ctrl Pts',(-5.69535834529991,0.809946053,-4.88019540489622));
#162812=CARTESIAN_POINT('Ctrl Pts',(-5.69935609130509,0.810932115073296,
-4.87552989578561));
#162813=CARTESIAN_POINT('Ctrl Pts',(-5.7033538373103,0.811918177146594,
-4.87086438667502));
#162814=CARTESIAN_POINT('Ctrl Pts',(-5.134148886,0.679837254,-5.118888084));
#162815=CARTESIAN_POINT('Ctrl Pts',(-5.411528649,0.744719353,-4.840681376));
#162816=CARTESIAN_POINT('Ctrl Pts',(-5.657221867,0.809946053,-4.534130649));
#162817=CARTESIAN_POINT('Ctrl Pts',(-5.66093612456532,0.810932115073296,
-4.52949638043458));
#162818=CARTESIAN_POINT('Ctrl Pts',(-5.66465038213065,0.811918177146594,
-4.52486211186916));
#162819=CARTESIAN_POINT('Origin',(0.154640799378106,0.803568169766499,0.125272107590645));
#162820=CARTESIAN_POINT('Ctrl Pts',(-6.002976704,0.809946053,-4.496028325));
#162821=CARTESIAN_POINT('Ctrl Pts',(-6.24980418500001,0.744288122,-4.166470877));
#162822=CARTESIAN_POINT('Ctrl Pts',(-6.459072287,0.679844992,-3.811874236));
#162823=CARTESIAN_POINT('Ctrl Pts',(-5.657221867,0.809946053,-4.534130649));
#162824=CARTESIAN_POINT('Ctrl Pts',(-5.906141128,0.744288122,-4.223554798));
#162825=CARTESIAN_POINT('Ctrl Pts',(-6.119566318,0.679844992,-3.887596697));
#162826=CARTESIAN_POINT('',(-6.11703469298358,0.680609079912898,-3.89157896256683));
#162827=CARTESIAN_POINT('Origin',(0.134168955827877,0.946280612859217,0.136471289280882));
#162828=CARTESIAN_POINT('Origin',(-17.5208345759338,-0.918884980963102,
-10.6165118135106));
#162829=CARTESIAN_POINT('Ctrl Pts',(-6.18987502407395,0.679837254,-4.2354292642493));
#162830=CARTESIAN_POINT('Ctrl Pts',(-6.41938236008868,0.744719353,-3.90001539367355));
#162831=CARTESIAN_POINT('Ctrl Pts',(-6.61130178639777,0.809946053,-3.5417654580932));
#162832=CARTESIAN_POINT('Ctrl Pts',(-6.61420311981289,0.810932114744282,
-3.53634963058135));
#162833=CARTESIAN_POINT('Ctrl Pts',(-6.61710445322799,0.811918176488562,
-3.53093380306951));
#162834=CARTESIAN_POINT('Ctrl Pts',(-6.114524963,0.679837254,-3.895521079));
#162835=CARTESIAN_POINT('Ctrl Pts',(-6.32561352300001,0.744719353,-3.564190239));
#162836=CARTESIAN_POINT('Ctrl Pts',(-6.499663225,0.809946053,-3.211989719));
#162837=CARTESIAN_POINT('Ctrl Pts',(-6.50229441365044,0.810932114744282,
-3.20666534325988));
#162838=CARTESIAN_POINT('Ctrl Pts',(-6.50492560230089,0.811918176488562,
-3.20134096751977));
#162839=CARTESIAN_POINT('Origin',(0.177955159893456,0.803568129644429,0.0891001020318583));
#162840=CARTESIAN_POINT('Ctrl Pts',(-6.829143632,0.809946053,-3.100451136));
#162841=CARTESIAN_POINT('Ctrl Pts',(-6.999355314,0.744288122,-2.725537947));
#162842=CARTESIAN_POINT('Ctrl Pts',(-7.127503049,0.679844992,-2.334245122));
#162843=CARTESIAN_POINT('Ctrl Pts',(-6.499663225,0.809946053,-3.211989719));
#162844=CARTESIAN_POINT('Ctrl Pts',(-6.675998265,0.744288122,-2.855164676));
#162845=CARTESIAN_POINT('Ctrl Pts',(-6.812212632,0.679844992,-2.481180981));
#162846=CARTESIAN_POINT('',(-6.81059626498796,0.680609079812778,-2.4856143691262));
#162847=CARTESIAN_POINT('Origin',(0.160369492607678,0.946280612470604,0.104438320064307));
#162848=CARTESIAN_POINT('Origin',(-19.3937873098339,-0.9189196105624,-6.60195672059528));
#162849=CARTESIAN_POINT('Ctrl Pts',(-6.95565127974782,0.679837254,-2.80576712312369));
#162850=CARTESIAN_POINT('Ctrl Pts',(-7.1076887940586,0.744719353,-2.42885774909654));
#162851=CARTESIAN_POINT('Ctrl Pts',(-7.21810810459673,0.809946053,-2.03772649393948));
#162852=CARTESIAN_POINT('Ctrl Pts',(-7.21977736329806,0.81093211455031,
-2.03181358570044));
#162853=CARTESIAN_POINT('Ctrl Pts',(-7.22144662199938,0.811918176100622,
-2.0259006774614));
#162854=CARTESIAN_POINT('Ctrl Pts',(-6.80899264800001,0.679837254,-2.490003838));
#162855=CARTESIAN_POINT('Ctrl Pts',(-6.943919739,0.744719353,-2.121041529));
#162856=CARTESIAN_POINT('Ctrl Pts',(-7.038187555,0.809946053,-1.73965972));
#162857=CARTESIAN_POINT('Ctrl Pts',(-7.03961264424704,0.81093211455031,
-1.73389419855183));
#162858=CARTESIAN_POINT('Ctrl Pts',(-7.04103773349406,0.811918176100623,
-1.72812867710368));
#162859=CARTESIAN_POINT('Origin',(0.192948619704593,0.803568097880944,0.0487619255622365));
#162860=CARTESIAN_POINT('Ctrl Pts',(-7.335987395,0.809946053,-1.559900299));
#162861=CARTESIAN_POINT('Ctrl Pts',(-7.421624369,0.744288122,-1.157161891));
#162862=CARTESIAN_POINT('Ctrl Pts',(-7.46265969,0.679844992,-0.7474693));
#162863=CARTESIAN_POINT('Ctrl Pts',(-7.038187555,0.809946053,-1.73965972));
#162864=CARTESIAN_POINT('Ctrl Pts',(-7.133693143,0.744288122,-1.353270226));
#162865=CARTESIAN_POINT('Ctrl Pts',(-7.186327454,0.679844992,-0.958748));
#162866=CARTESIAN_POINT('',(-7.18570192399795,0.680609079819347,-0.963425209256815));
#162867=CARTESIAN_POINT('Origin',(0.179071211428947,0.946280567038781,0.0675218811833105));
#162868=CARTESIAN_POINT('Origin',(-20.3590065423551,-0.918863189645757,
-2.27845220396367));
#162869=CARTESIAN_POINT('Ctrl Pts',(-7.39618901112522,0.679837254,-1.24491042948448));
#162870=CARTESIAN_POINT('Ctrl Pts',(-7.46364759923879,0.744719353,-0.844129415789026));
#162871=CARTESIAN_POINT('Ctrl Pts',(-7.48740370966554,0.809946053,-0.438405704310963));
#162872=CARTESIAN_POINT('Ctrl Pts',(-7.48776284161505,0.810932114754673,
-0.432272194032922));
#162873=CARTESIAN_POINT('Ctrl Pts',(-7.48812197356457,0.811918176509348,
-0.42613868375488));
#162874=CARTESIAN_POINT('Ctrl Pts',(-7.185079405,0.679837254,-0.968056785));
#162875=CARTESIAN_POINT('Ctrl Pts',(-7.23753598500001,0.744719353,-0.578715273));
#162876=CARTESIAN_POINT('Ctrl Pts',(-7.247614057,0.809946053,-0.185985165));
#162877=CARTESIAN_POINT('Ctrl Pts',(-7.24776641180808,0.810932114754673,
-0.180048084948309));
#162878=CARTESIAN_POINT('Ctrl Pts',(-7.24791876661615,0.811918176509348,
-0.174111004896619));
#162879=CARTESIAN_POINT('Origin',(0.198919786025193,0.803568105559062,0.00614363756408852));
#162880=CARTESIAN_POINT('Ctrl Pts',(-7.49980854000001,0.809946053,0.053589743));
#162881=CARTESIAN_POINT('Ctrl Pts',(-7.496866517,0.744288122,0.465321769));
#162882=CARTESIAN_POINT('Ctrl Pts',(-7.448870658,0.679844992,0.874257356));
#162883=CARTESIAN_POINT('Ctrl Pts',(-7.24761405700001,0.809946053,-0.185985165));
#162884=CARTESIAN_POINT('Ctrl Pts',(-7.257824457,0.744288122,0.211901635));
#162885=CARTESIAN_POINT('Ctrl Pts',(-7.224417591,0.679844992,0.608514971));
#162886=CARTESIAN_POINT('',(-7.22481214561418,0.680609079902423,0.603812642589529));
#162887=CARTESIAN_POINT('Origin',(0.189399765800756,0.946280567050045,0.02744823793889));
#162888=CARTESIAN_POINT('Origin',(-20.3741608616577,-0.919019427051703,
2.15155633872438));
#162889=CARTESIAN_POINT('Ctrl Pts',(-7.49088916474174,0.679837254,0.374156892912213));
#162890=CARTESIAN_POINT('Ctrl Pts',(-7.47061453742044,0.744719353,0.780069471217557));
#162891=CARTESIAN_POINT('Ctrl Pts',(-7.40659663794375,0.809946053,1.18141444887646));
#162892=CARTESIAN_POINT('Ctrl Pts',(-7.40562885218112,0.810932112713297,
1.18748175127876));
#162893=CARTESIAN_POINT('Ctrl Pts',(-7.40466106641846,0.811918172426596,
1.19354905368104));
#162894=CARTESIAN_POINT('Ctrl Pts',(-7.225199835,0.679837254,0.599155527));
#162895=CARTESIAN_POINT('Ctrl Pts',(-7.192733093,0.744719353,0.990671065));
#162896=CARTESIAN_POINT('Ctrl Pts',(-7.118150181,0.809946053,1.376385849));
#162897=CARTESIAN_POINT('Ctrl Pts',(-7.11702267945809,0.810932112713297,
1.38221686312957));
#162898=CARTESIAN_POINT('Ctrl Pts',(-7.11589517791618,0.811918172426596,
1.38804787725915));
#162899=CARTESIAN_POINT('Origin',(0.195589888903499,0.803568151949699,-0.0367618791827232));
#162900=CARTESIAN_POINT('Ctrl Pts',(-7.312946974,0.809946053,1.664573988));
#162901=CARTESIAN_POINT('Ctrl Pts',(-7.221563518,0.744288122,2.0660475));
#162902=CARTESIAN_POINT('Ctrl Pts',(-7.086780713,0.679844992,2.455104709));
#162903=CARTESIAN_POINT('Ctrl Pts',(-7.118150181,0.809946053,1.376385849));
#162904=CARTESIAN_POINT('Ctrl Pts',(-7.042587967,0.744288122,1.767165211));
#162905=CARTESIAN_POINT('Ctrl Pts',(-6.924701991,0.679844992,2.147324459));
#162906=CARTESIAN_POINT('',(-6.92609818329531,0.680609079950017,2.1428168859889));
#162907=CARTESIAN_POINT('Origin',(0.190872315132972,0.946280526448961,-0.0139088557421879));
#162908=CARTESIAN_POINT('Origin',(-19.4345323938522,-0.918914486389337,
6.48082719568603));
#162909=CARTESIAN_POINT('Ctrl Pts',(-7.23532366753185,0.679837254,1.97572905333991));
#162910=CARTESIAN_POINT('Ctrl Pts',(-7.12826384427363,0.744719353,2.36779317643012));
#162911=CARTESIAN_POINT('Ctrl Pts',(-6.97946534152131,0.809946053,2.74599297580928));
#162912=CARTESIAN_POINT('Ctrl Pts',(-6.97721588704522,0.810932114617301,
2.75171039376601));
#162913=CARTESIAN_POINT('Ctrl Pts',(-6.97496643256913,0.811918176234604,
2.75742781172276));
#162914=CARTESIAN_POINT('Ctrl Pts',(-6.92747795,0.679837254,2.138351993));
#162915=CARTESIAN_POINT('Ctrl Pts',(-6.811605995,0.744719353,2.513734725));
#162916=CARTESIAN_POINT('Ctrl Pts',(-6.655849513,0.809946053,2.874398591));
#162917=CARTESIAN_POINT('Ctrl Pts',(-6.65349487159478,0.810932114617301,
2.87985091029578));
#162918=CARTESIAN_POINT('Ctrl Pts',(-6.65114023018955,0.811918176234604,
2.88530322959156));
#162919=CARTESIAN_POINT('Origin',(0.183114638037944,0.803568143872066,-0.0779485444577915));
#162920=CARTESIAN_POINT('Ctrl Pts',(-6.784140134,0.809946053,3.197724603));
#162921=CARTESIAN_POINT('Ctrl Pts',(-6.608588236,0.744288122,3.570167146));
#162922=CARTESIAN_POINT('Ctrl Pts',(-6.393320778,0.679844992,3.921154095));
#162923=CARTESIAN_POINT('Ctrl Pts',(-6.655849513,0.809946053,2.874398591));
#162924=CARTESIAN_POINT('Ctrl Pts',(-6.49804789100001,0.744288122,3.239798106));
#162925=CARTESIAN_POINT('Ctrl Pts',(-6.301195022,0.679844992,3.585727442));
#162926=CARTESIAN_POINT('',(-6.30352756759927,0.680609079949565,3.58162539327411));
#162927=CARTESIAN_POINT('Origin',(0.183420109496064,0.946280576848784,-0.0546157096338185));
#162928=CARTESIAN_POINT('Origin',(-17.5862892028171,-0.918828340772164,
10.5067409239504));
#162929=CARTESIAN_POINT('Ctrl Pts',(-6.64144247684645,0.679837254,3.48491831999589));
#162930=CARTESIAN_POINT('Ctrl Pts',(-6.45260345462069,0.744719353,3.84480150431211));
#162931=CARTESIAN_POINT('Ctrl Pts',(-6.22598200120882,0.809946053,4.18217192206895));
#162932=CARTESIAN_POINT('Ctrl Pts',(-6.22255606118742,0.810932114816432,
4.18727210476934));
#162933=CARTESIAN_POINT('Ctrl Pts',(-6.21913012116601,0.811918176632866,
4.19237228746973));
#162934=CARTESIAN_POINT('Ctrl Pts',(-6.305834896,0.679837254,3.577561496));
#162935=CARTESIAN_POINT('Ctrl Pts',(-6.111975772,0.744719353,3.919258944));
#162936=CARTESIAN_POINT('Ctrl Pts',(-5.88232872,0.809946053,4.238007649));
#162937=CARTESIAN_POINT('Ctrl Pts',(-5.87885704062279,0.810932114816432,
4.24282631876312));
#162938=CARTESIAN_POINT('Ctrl Pts',(-5.87538536124559,0.811918176632866,
4.24764498852623));
#162939=CARTESIAN_POINT('Origin',(0.16207692372856,0.803568121700288,-0.115490408361313));
#162940=CARTESIAN_POINT('Ctrl Pts',(-5.938114442,0.809946053,4.58135317));
#162941=CARTESIAN_POINT('Ctrl Pts',(-5.686602712,0.744288122,4.907349744));
#162942=CARTESIAN_POINT('Ctrl Pts',(-5.400916269,0.679844992,5.203854673));
#162943=CARTESIAN_POINT('Ctrl Pts',(-5.88232872,0.809946053,4.238007649));
#162944=CARTESIAN_POINT('Ctrl Pts',(-5.649666317,0.744288122,4.560941642));
#162945=CARTESIAN_POINT('Ctrl Pts',(-5.383051178,0.679844992,4.856465795));
#162946=CARTESIAN_POINT('',(-5.38621100825962,0.680609079924947,4.85296107797159));
#162947=CARTESIAN_POINT('Origin',(0.167390889420725,0.946280564445741,-0.0927685709128245));
#162948=CARTESIAN_POINT('Origin',(-14.9171667056585,-0.918935963699563,
14.0422811013448));
#162949=CARTESIAN_POINT('Ctrl Pts',(-5.73701481756621,0.679837254,4.83115667912201));
#162950=CARTESIAN_POINT('Ctrl Pts',(-5.47522650015516,0.744719353,5.1420311871362));
#162951=CARTESIAN_POINT('Ctrl Pts',(-5.18137866338577,0.809946053,5.42279715848552));
#162952=CARTESIAN_POINT('Ctrl Pts',(-5.17693643039999,0.810932115043126,
5.42704162689108));
#162953=CARTESIAN_POINT('Ctrl Pts',(-5.17249419741424,0.811918177086253,
5.43128609529664));
#162954=CARTESIAN_POINT('Ctrl Pts',(-5.389338011,0.679837254,4.8494882));
#162955=CARTESIAN_POINT('Ctrl Pts',(-5.12655635500001,0.744719353,5.14152297));
#162956=CARTESIAN_POINT('Ctrl Pts',(-4.833756773,0.809946053,5.403452179));
#162957=CARTESIAN_POINT('Ctrl Pts',(-4.82933038696402,0.810932115043127,
5.4074118833999));
#162958=CARTESIAN_POINT('Ctrl Pts',(-4.82490400092802,0.811918177086251,
5.4113715877998));
#162959=CARTESIAN_POINT('Origin',(0.133460466573784,0.803568152816683,-0.147631903631662));
#162960=CARTESIAN_POINT('Ctrl Pts',(-4.814429119,0.809946053,5.75076275500001));
#162961=CARTESIAN_POINT('Ctrl Pts',(-4.498717966,0.744288122,6.015070122));
#162962=CARTESIAN_POINT('Ctrl Pts',(-4.155970918,0.679844992,6.24322879000001));
#162963=CARTESIAN_POINT('Ctrl Pts',(-4.833756773,0.809946053,5.403452179));
#162964=CARTESIAN_POINT('Ctrl Pts',(-4.537112626,0.744288122,5.66882061600001));
#162965=CARTESIAN_POINT('Ctrl Pts',(-4.213201843,0.679844992,5.900121205));
#162966=CARTESIAN_POINT('',(-4.21704120849093,0.680609079904585,5.89737769623315));
#162967=CARTESIAN_POINT('Origin',(0.143534843142958,0.946280593422227,-0.126583721164557));
#162968=CARTESIAN_POINT('Origin',(-11.5499800133793,-0.918992406372022,
16.9210941645051));
#162969=CARTESIAN_POINT('Ctrl Pts',(-4.56433072088425,0.679837254,5.95149552184957));
#162970=CARTESIAN_POINT('Ctrl Pts',(-4.24183403969426,0.744719353,6.19882520562349));
#162971=CARTESIAN_POINT('Ctrl Pts',(-3.89449981646425,0.809946053,6.40985842675195));
#162972=CARTESIAN_POINT('Ctrl Pts',(-3.88924901058972,0.810932114023159,
6.41304870977939));
#162973=CARTESIAN_POINT('Ctrl Pts',(-3.88399820471517,0.811918175046322,
6.41623899280684));
#162974=CARTESIAN_POINT('Ctrl Pts',(-4.22084167,0.679837254,5.894658226));
#162975=CARTESIAN_POINT('Ctrl Pts',(-3.90142486,0.744719353,6.123375096));
#162976=CARTESIAN_POINT('Ctrl Pts',(-3.559163733,0.809946053,6.316237292));
#162977=CARTESIAN_POINT('Ctrl Pts',(-3.55398961937663,0.810932114023161,
6.31915287556189));
#162978=CARTESIAN_POINT('Ctrl Pts',(-3.54881550575326,0.811918175046319,
6.3220684591238));
#162979=CARTESIAN_POINT('Origin',(0.0986037502081683,0.803568105149723,
-0.172870385270595));
#162980=CARTESIAN_POINT('Ctrl Pts',(-3.465626441,0.809946053,6.651273064));
#162981=CARTESIAN_POINT('Ctrl Pts',(-3.100478168,0.744288122,6.841532507));
#162982=CARTESIAN_POINT('Ctrl Pts',(-2.716696986,0.679844992,6.99067646800001));
#162983=CARTESIAN_POINT('Ctrl Pts',(-3.559163733,0.809946053,6.316237292));
#162984=CARTESIAN_POINT('Ctrl Pts',(-3.212408591,0.744288122,6.511631839));
#162985=CARTESIAN_POINT('Ctrl Pts',(-2.846347872,0.679844992,6.667893505));
#162986=CARTESIAN_POINT('',(-2.85068724914484,0.680609079940132,6.66603948790399));
#162987=CARTESIAN_POINT('Origin',(0.112967313262388,0.946280564787144,-0.154480030424337));
#162988=CARTESIAN_POINT('Origin',(-7.64227220663124,-0.918948768628997,
19.0080412821093));
#162989=CARTESIAN_POINT('Ctrl Pts',(-3.17822359332481,0.679837254,6.7935490476677));
#162990=CARTESIAN_POINT('Ctrl Pts',(-2.81009813331689,0.744719353,6.9657690488301));
#162991=CARTESIAN_POINT('Ctrl Pts',(-2.42551848805247,0.809946053,7.0972018388643));
#162992=CARTESIAN_POINT('Ctrl Pts',(-2.4197046177963,0.810932115511907,
7.09918876978505));
#162993=CARTESIAN_POINT('Ctrl Pts',(-2.41389074754013,0.811918178023817,
7.1011757007058));
#162994=CARTESIAN_POINT('Ctrl Pts',(-2.854983464,0.679837254,6.664200584));
#162995=CARTESIAN_POINT('Ctrl Pts',(-2.493867074,0.744719353,6.818905009));
#162996=CARTESIAN_POINT('Ctrl Pts',(-2.118148151,0.809946053,6.933682168));
#162997=CARTESIAN_POINT('Ctrl Pts',(-2.11246823242395,0.810932115511907,
6.93541730796129));
#162998=CARTESIAN_POINT('Ctrl Pts',(-2.10678831384789,0.811918178023817,
6.93715244792259));
#162999=CARTESIAN_POINT('Origin',(0.0591363929493419,0.803568159525722,
-0.190025607610674));
#163000=CARTESIAN_POINT('Ctrl Pts',(-1.954774922,0.809946053,7.240777238));
#163001=CARTESIAN_POINT('Ctrl Pts',(-1.557263457,0.744288122,7.348092436));
#163002=CARTESIAN_POINT('Ctrl Pts',(-1.150393323,0.679844992,7.411247884));
#163003=CARTESIAN_POINT('Ctrl Pts',(-2.118148151,0.809946053,6.933682168));
#163004=CARTESIAN_POINT('Ctrl Pts',(-1.7374959,0.744288122,7.049966394));
#163005=CARTESIAN_POINT('Ctrl Pts',(-1.346401839,0.679844992,7.123882515));
#163006=CARTESIAN_POINT('',(-1.35103832225975,0.680609079911867,7.12300468231609));
#163007=CARTESIAN_POINT('Origin',(0.0771176410036584,0.946280540915505,
-0.175153319735645));
#163008=CARTESIAN_POINT('Origin',(-3.37736490900802,-0.918896036187134,
20.2060467750998));
#163009=CARTESIAN_POINT('Ctrl Pts',(-1.64350626238501,0.679837254,7.31794377079529));
#163010=CARTESIAN_POINT('Ctrl Pts',(-1.24696516207443,0.744719353,7.40700127184289));
#163011=CARTESIAN_POINT('Ctrl Pts',(-0.843122609833158,0.809946053,7.45268798029123));
#163012=CARTESIAN_POINT('Ctrl Pts',(-0.837017537601804,0.810932114802311,
7.45337864712052));
#163013=CARTESIAN_POINT('Ctrl Pts',(-0.830912465370449,0.811918176604621,
7.45406931394981));
#163014=CARTESIAN_POINT('Ctrl Pts',(-1.355629403,0.679837254,7.12213233));
#163015=CARTESIAN_POINT('Ctrl Pts',(-0.969698837,0.744719353,7.195590502));
#163016=CARTESIAN_POINT('Ctrl Pts',(-0.578090316999999,0.809946053,7.226915773));
#163017=CARTESIAN_POINT('Ctrl Pts',(-0.572170192219328,0.810932114802312,
7.22738933142286));
#163018=CARTESIAN_POINT('Ctrl Pts',(-0.566250067438653,0.811918176604621,
7.22786288984572));
#163019=CARTESIAN_POINT('Origin',(0.0169039340594927,0.803568164770754,
-0.198295592186956));
#163020=CARTESIAN_POINT('Ctrl Pts',(-0.3525203,0.809946053,7.49171071500001));
#163021=CARTESIAN_POINT('Ctrl Pts',(0.058767163,0.744288122,7.51106372900001));
#163022=CARTESIAN_POINT('Ctrl Pts',(0.469701454,0.679844992,7.485277586));
#163023=CARTESIAN_POINT('Ctrl Pts',(-0.578090317,0.809946053,7.226915773));
#163024=CARTESIAN_POINT('Ctrl Pts',(-0.181339832,0.744288122,7.258652356));
#163025=CARTESIAN_POINT('Ctrl Pts',(0.216500448,0.679844992,7.246766697));
#163026=CARTESIAN_POINT('Origin',(0.0376618935714465,0.946280616501933,
-0.18763604326458));
#163027=CARTESIAN_POINT('Ctrl Pts',(0.211783654,0.680609079,7.246906077));
#163028=CARTESIAN_POINT('Ctrl Pts',(0.604481562,0.745496505000001,7.23542986900001));
#163029=CARTESIAN_POINT('Ctrl Pts',(0.993639891,0.810723991,7.18158616));
#163030=CARTESIAN_POINT('Ctrl Pts',(0.464829365,0.680609079,7.485581718));
#163031=CARTESIAN_POINT('Ctrl Pts',(0.870460713,0.745496505,7.46039338));
#163032=CARTESIAN_POINT('Ctrl Pts',(1.270995025,0.810723991,7.391520253));
#163033=CARTESIAN_POINT('Ctrl Pts',(0.4838423694909,0.680609079,7.50351500371454));
#163034=CARTESIAN_POINT('Ctrl Pts',(0.890445492716139,0.745496505,7.4772963823391));
#163035=CARTESIAN_POINT('Ctrl Pts',(1.29183455785545,0.810723991,7.40729399536943));
#163036=CARTESIAN_POINT('',(0.395386353409136,0.680609080400561,7.42008227489806));
#163037=CARTESIAN_POINT('',(0.304135795241984,0.680609082082805,7.33401370379862));
#163038=CARTESIAN_POINT('',(1.02663072523825,0.76798017562717,7.44739982155537));
#163039=CARTESIAN_POINT('Ctrl Pts',(0.395386359566659,0.680609079136169,
7.42008227135047));
#163040=CARTESIAN_POINT('Ctrl Pts',(0.500009482076225,0.695136944977305,
7.42905580208087));
#163041=CARTESIAN_POINT('Ctrl Pts',(0.604810648040692,0.709660812710993,
7.43582945914476));
#163042=CARTESIAN_POINT('Ctrl Pts',(0.815284577790083,0.738780776738529,
7.44500505794044));
#163043=CARTESIAN_POINT('Ctrl Pts',(0.920936382652429,0.753373671667379,
7.44737846514938));
#163044=CARTESIAN_POINT('Ctrl Pts',(1.02660466604954,0.767949007798904,
7.44752577326926));
#163045=CARTESIAN_POINT('Ctrl Pts',(0.988998379602801,0.809946052545264,
7.18222682905853));
#163046=CARTESIAN_POINT('Ctrl Pts',(0.994923072744043,0.802922931274876,
7.22424856499997));
#163047=CARTESIAN_POINT('Ctrl Pts',(1.00087662461022,0.796078752403875,
7.26632383852537));
#163048=CARTESIAN_POINT('Ctrl Pts',(1.01341493206971,0.782074139994843,
7.35464723293283));
#163049=CARTESIAN_POINT('Ctrl Pts',(1.0200128069643,0.774939590237252,7.40095924419224));
#163050=CARTESIAN_POINT('Ctrl Pts',(1.02663085166062,0.767997185229757,
7.44726315247994));
#163051=CARTESIAN_POINT('Origin',(-5.43456338958359E-14,0.560925699999933,
-6.93889390390723E-14));
#163052=CARTESIAN_POINT('',(1.63504458648,0.680609080181315,7.24848815475887));
#163053=CARTESIAN_POINT('',(1.00401106526424,0.562053379613689,7.24279548290209));
#163054=CARTESIAN_POINT('Ctrl Pts',(1.63504458645295,0.680609079948412,
7.24848815266485));
#163055=CARTESIAN_POINT('Ctrl Pts',(1.58723214217251,0.671661524751094,
7.25010086045261));
#163056=CARTESIAN_POINT('Ctrl Pts',(1.53425686505398,0.661738573429343,
7.25142167916517));
#163057=CARTESIAN_POINT('Ctrl Pts',(1.42431339294704,0.641119488187471,
7.25276715487363));
#163058=CARTESIAN_POINT('Ctrl Pts',(1.37187915142337,0.631275792584381,
7.25284991854614));
#163059=CARTESIAN_POINT('Ctrl Pts',(1.21423924388054,0.601654471621312,
7.25142233155372));
#163060=CARTESIAN_POINT('Ctrl Pts',(1.1090790626735,0.581858135018139,7.24822487778146));
#163061=CARTESIAN_POINT('Ctrl Pts',(1.0040110651189,0.562053380213309,7.24279548352759));
#163062=CARTESIAN_POINT('Ctrl Pts',(1.02663059881587,0.767963166024584,
7.4475364906308));
#163063=CARTESIAN_POINT('Ctrl Pts',(1.12966842526234,0.753333602537456,
7.41856499043498));
#163064=CARTESIAN_POINT('Ctrl Pts',(1.23208600136148,0.738713518212131,
7.38742430932713));
#163065=CARTESIAN_POINT('Ctrl Pts',(1.43495011980214,0.709588701416252,
7.3210310126199));
#163066=CARTESIAN_POINT('Ctrl Pts',(1.53538301094752,0.695086898841886,
7.28581043640534));
#163067=CARTESIAN_POINT('Ctrl Pts',(1.63504458150421,0.680609078982399,
7.24848815279085));
#163068=CARTESIAN_POINT('Ctrl Pts',(1.00401106512942,0.562053379355767,
7.24279548266039));
#163069=CARTESIAN_POINT('Ctrl Pts',(0.904086842224673,0.582224590119512,
7.27701127625761));
#163070=CARTESIAN_POINT('Ctrl Pts',(0.803350409959279,0.602198953310061,
7.30891500817337));
#163071=CARTESIAN_POINT('Ctrl Pts',(0.651321854294389,0.631811121642218,
7.3532027391429));
#163072=CARTESIAN_POINT('Ctrl Pts',(0.600593664771072,0.641604433043982,
7.3673457081378));
#163073=CARTESIAN_POINT('Ctrl Pts',(0.494453675786446,0.66191430093601,
7.39561665600437));
#163074=CARTESIAN_POINT('Ctrl Pts',(0.443161379792506,0.671620850615904,
7.40853555255282));
#163075=CARTESIAN_POINT('Ctrl Pts',(0.395386352780817,0.680609080018574,
7.42008227259572));
#163076=CARTESIAN_POINT('Ctrl Pts',(0.984280001000001,0.810731746,7.182874973));
#163077=CARTESIAN_POINT('Ctrl Pts',(1.378634468,0.745065281,7.128835996));
#163078=CARTESIAN_POINT('Ctrl Pts',(1.764702859,0.680609079,7.03195021400001));
#163079=CARTESIAN_POINT('Ctrl Pts',(0.773984637,0.810731746,7.45995628600001));
#163080=CARTESIAN_POINT('Ctrl Pts',(1.183551433,0.745065281,7.417462952));
#163081=CARTESIAN_POINT('Ctrl Pts',(1.586004669,0.680609079,7.330388065));
#163082=CARTESIAN_POINT('Ctrl Pts',(0.758157006316509,0.810731746,7.48081048177514));
#163083=CARTESIAN_POINT('Ctrl Pts',(1.16886874018232,0.745065281,7.43918611687617));
#163084=CARTESIAN_POINT('Ctrl Pts',(1.5725551620716,0.680609079,7.35284963523035));
#163085=CARTESIAN_POINT('',(1.69948476214558,0.680609081791274,7.14086879303845));
#163086=CARTESIAN_POINT('Ctrl Pts',(1.764702859,0.680609079,7.03195021400001));
#163087=CARTESIAN_POINT('Ctrl Pts',(2.145752663,0.745496505000001,6.936323872));
#163088=CARTESIAN_POINT('Ctrl Pts',(2.51423788,0.810723991,6.800081461));
#163089=CARTESIAN_POINT('Ctrl Pts',(2.06314071,0.680609079,7.210648404));
#163090=CARTESIAN_POINT('Ctrl Pts',(2.453873874,0.745496505000001,7.098850206));
#163091=CARTESIAN_POINT('Ctrl Pts',(2.83023823,0.810723991,6.94548425700001));
#163092=CARTESIAN_POINT('Ctrl Pts',(2.085564327413,0.680609079,7.22407518559466));
#163093=CARTESIAN_POINT('Ctrl Pts',(2.47702506654861,0.745496505000001,
7.11106188867009));
#163094=CARTESIAN_POINT('Ctrl Pts',(2.85398143458022,0.810723991,6.95640933455756));
#163095=CARTESIAN_POINT('',(1.98124079348741,0.680609080419527,7.1616084961454));
#163096=CARTESIAN_POINT('',(1.87253223753562,0.680609082082805,7.09651615128199));
#163097=CARTESIAN_POINT('',(2.60359948730395,0.767980175627753,7.05258849344245));
#163098=CARTESIAN_POINT('Ctrl Pts',(1.9812407986416,0.680609079126786,7.16160849143538));
#163099=CARTESIAN_POINT('Ctrl Pts',(2.08534693316848,0.695136944794904,
7.14788134749876));
#163100=CARTESIAN_POINT('Ctrl Pts',(2.18915404078839,0.709660812349475,
7.13196748774765));
#163101=CARTESIAN_POINT('Ctrl Pts',(2.39667969198913,0.738780776740227,
7.09568289240512));
#163102=CARTESIAN_POINT('Ctrl Pts',(2.50037162874458,0.753373671672762,
7.07528879568255));
#163103=CARTESIAN_POINT('Ctrl Pts',(2.60360111327753,0.767949007806505,
7.05271710243074));
#163104=CARTESIAN_POINT('Ctrl Pts',(2.50984261070199,0.809946052649527,
6.80170493940386));
#163105=CARTESIAN_POINT('Ctrl Pts',(2.52466221878819,0.802922931334229,
6.84147059690226));
#163106=CARTESIAN_POINT('Ctrl Pts',(2.53952151974974,0.796078752498655,
6.88128233605344));
#163107=CARTESIAN_POINT('Ctrl Pts',(2.57075360736643,0.782074140027835,
6.96484541348759));
#163108=CARTESIAN_POINT('Ctrl Pts',(2.58715294097028,0.774939590254329,
7.0086563276866));
#163109=CARTESIAN_POINT('Ctrl Pts',(2.603570230945,0.767997185232552,7.05245499244542));
#163110=CARTESIAN_POINT('Origin',(8.00141203294302E-14,0.560925700000022,
-2.07733136248223E-13));
#163111=CARTESIAN_POINT('',(3.15502884266931,0.680609080190964,6.72753627498307));
#163112=CARTESIAN_POINT('',(2.53752478129952,0.562053379772718,6.85763024758604));
#163113=CARTESIAN_POINT('Ctrl Pts',(3.15502884219952,0.68060907997646,6.7275362729842));
#163114=CARTESIAN_POINT('Ctrl Pts',(3.1086809112377,0.671661524850685,6.73938953863211));
#163115=CARTESIAN_POINT('Ctrl Pts',(3.05722810394215,0.661738573577959,
6.75206759590499));
#163116=CARTESIAN_POINT('Ctrl Pts',(2.95014428708656,0.641119488421689,
6.77701621164918));
#163117=CARTESIAN_POINT('Ctrl Pts',(2.89895372092233,0.631275792858778,
6.78836885231258));
#163118=CARTESIAN_POINT('Ctrl Pts',(2.74469245849335,0.601654472053282,
6.8208625617643));
#163119=CARTESIAN_POINT('Ctrl Pts',(2.64130350622483,0.581858135561308,
6.84034619314135));
#163120=CARTESIAN_POINT('Ctrl Pts',(2.53752478128929,0.562053380894578,
6.85763024881006));
#163121=CARTESIAN_POINT('Ctrl Pts',(2.6036287436629,0.767963166022953,7.05272199443948));
#163122=CARTESIAN_POINT('Ctrl Pts',(2.69802958696195,0.753333602540172,
7.00227774486911));
#163123=CARTESIAN_POINT('Ctrl Pts',(2.79135837124678,0.738713518219378,
6.94984836411526));
#163124=CARTESIAN_POINT('Ctrl Pts',(2.97520704219334,0.709588701614233,
6.84139751752858));
#163125=CARTESIAN_POINT('Ctrl Pts',(3.06572048612681,0.695086898944589,
6.78541027559763));
#163126=CARTESIAN_POINT('Ctrl Pts',(3.15502883751132,0.680609078987249,
6.72753627409024));
#163127=CARTESIAN_POINT('Ctrl Pts',(2.53752478053378,0.562053378680438,
6.85763024672876));
#163128=CARTESIAN_POINT('Ctrl Pts',(2.44729211420189,0.58222458955668,6.9125268486052));
#163129=CARTESIAN_POINT('Ctrl Pts',(2.35576920258763,0.602198952866584,
6.96534004450702));
#163130=CARTESIAN_POINT('Ctrl Pts',(2.2168143959035,0.631811365719166,7.04127462546337));
#163131=CARTESIAN_POINT('Ctrl Pts',(2.17031136200528,0.641604918880096,
7.06599260123164));
#163132=CARTESIAN_POINT('Ctrl Pts',(2.07273008286579,0.66191481702943,7.11641958370329));
#163133=CARTESIAN_POINT('Ctrl Pts',(2.02541538654176,0.671621107824337,
7.14006213116803));
#163134=CARTESIAN_POINT('Ctrl Pts',(1.98124079243869,0.680609080077605,
7.16160849413794));
#163135=CARTESIAN_POINT('Ctrl Pts',(2.505373877,0.810731746,6.803352243));
#163136=CARTESIAN_POINT('Ctrl Pts',(2.878891773,0.745065281,6.665802114));
#163137=CARTESIAN_POINT('Ctrl Pts',(3.23510652,0.680609079,6.488188176));
#163138=CARTESIAN_POINT('Ctrl Pts',(2.359559393,0.810731746,7.119162835));
#163139=CARTESIAN_POINT('Ctrl Pts',(2.750415934,0.745065281,6.98961821800001));
#163140=CARTESIAN_POINT('Ctrl Pts',(3.124741511,0.680609079,6.818063544));
#163141=CARTESIAN_POINT('Ctrl Pts',(2.34858483909455,0.810731746,7.14293194401264));
#163142=CARTESIAN_POINT('Ctrl Pts',(2.74074635261154,0.745065281,7.01398985236249));
#163143=CARTESIAN_POINT('Ctrl Pts',(3.11643501971519,0.680609079,6.84289122166883));
#163144=CARTESIAN_POINT('',(3.1948274609048,0.680609081791274,6.60858026205276));
#163145=CARTESIAN_POINT('Ctrl Pts',(3.23510652,0.680609079,6.488188176));
#163146=CARTESIAN_POINT('Ctrl Pts',(3.586690754,0.745496505000001,6.31288308));
#163147=CARTESIAN_POINT('Ctrl Pts',(3.917272901,0.810723991,6.100612512));
#163148=CARTESIAN_POINT('Ctrl Pts',(3.564981888,0.680609079,6.59855318500001));
#163149=CARTESIAN_POINT('Ctrl Pts',(3.922546621,0.745496505000001,6.405372686));
#163150=CARTESIAN_POINT('Ctrl Pts',(4.257142641,0.810723991,6.174685136));
#163151=CARTESIAN_POINT('Ctrl Pts',(3.58976761490954,0.680609079,6.60684564099643));
#163152=CARTESIAN_POINT('Ctrl Pts',(3.94778170251245,0.745496505000001,
6.41232204426881));
#163153=CARTESIAN_POINT('Ctrl Pts',(4.28267931144474,0.810723991,6.18025070411462));
#163154=CARTESIAN_POINT('',(3.47445461509448,0.680609080408186,6.56826586412171));
#163155=CARTESIAN_POINT('',(3.35549859635723,0.680609082082805,6.52846725931103));
#163156=CARTESIAN_POINT('',(4.05882683126017,0.767980175582968,6.32800596564452));
#163157=CARTESIAN_POINT('Ctrl Pts',(3.47445461920584,0.680609079123292,
6.56826585833953));
#163158=CARTESIAN_POINT('Ctrl Pts',(3.57317587970167,0.695136944718301,
6.5324799059097));
#163159=CARTESIAN_POINT('Ctrl Pts',(3.67113502507767,0.70966081219651,6.49462264385934));
#163160=CARTESIAN_POINT('Ctrl Pts',(3.86600872735986,0.738780776674586,
6.41457448117895));
#163161=CARTESIAN_POINT('Ctrl Pts',(3.96289227645095,0.753373671607418,
6.37236648572888));
#163162=CARTESIAN_POINT('Ctrl Pts',(4.05885606630356,0.767949007742122,
6.32813121830147));
#163163=CARTESIAN_POINT('Ctrl Pts',(3.91332939002799,0.809946052501965,
6.10314288788829));
#163164=CARTESIAN_POINT('Ctrl Pts',(3.93635096497877,0.802922931194473,
6.13879306854643));
#163165=CARTESIAN_POINT('Ctrl Pts',(3.95942121084569,0.796078752396678,
6.17447972056928));
#163166=CARTESIAN_POINT('Ctrl Pts',(4.00788670128113,0.782074139948338,
6.24937516371998));
#163167=CARTESIAN_POINT('Ctrl Pts',(4.0333206790917,0.774939590190608,6.28863643094237));
#163168=CARTESIAN_POINT('Ctrl Pts',(4.05876956016351,0.767997185182016,
6.32788187504603));
#163169=CARTESIAN_POINT('Origin',(-5.14345510627123E-13,0.560925699999955,
-8.15320033709099E-13));
#163170=CARTESIAN_POINT('',(4.52748745641034,0.680609080270237,5.89201227580179));
#163171=CARTESIAN_POINT('',(3.95238665241763,0.562053379603276,6.15180984556242));
#163172=CARTESIAN_POINT('Ctrl Pts',(4.52748745566869,0.680609080100659,
5.89201227426056));
#163173=CARTESIAN_POINT('Ctrl Pts',(4.48477121484114,0.671661524881241,
5.91355185251235));
#163174=CARTESIAN_POINT('Ctrl Pts',(4.43724675273578,0.661738573524651,
5.9369943366818));
#163175=CARTESIAN_POINT('Ctrl Pts',(4.33802971034782,0.641119488246075,
5.98437952315467));
#163176=CARTESIAN_POINT('Ctrl Pts',(4.2904764331093,0.631275792632267,6.00647120401911));
#163177=CARTESIAN_POINT('Ctrl Pts',(4.14680689960514,0.601654471665006,
6.07136684033878));
#163178=CARTESIAN_POINT('Ctrl Pts',(4.05002352800819,0.581858135071578,
6.11262052392551));
#163179=CARTESIAN_POINT('Ctrl Pts',(3.95238665256539,0.562053380281048,
6.15180984627309));
#163180=CARTESIAN_POINT('Ctrl Pts',(4.05888410235683,0.767963165983919,
6.328130056243));
#163181=CARTESIAN_POINT('Ctrl Pts',(4.14023388382345,0.753333602501295,
6.25857177437937));
#163182=CARTESIAN_POINT('Ctrl Pts',(4.22010992589841,0.738713518183888,
6.18730523359868));
#163183=CARTESIAN_POINT('Ctrl Pts',(4.37634659231398,0.709588701304981,
6.04186787645319));
#163184=CARTESIAN_POINT('Ctrl Pts',(4.45270827935236,0.695086898787018,
5.96773187095885));
#163185=CARTESIAN_POINT('Ctrl Pts',(4.52748745077445,0.680609078979747,
5.89201227660773));
#163186=CARTESIAN_POINT('Ctrl Pts',(3.95238665216459,0.562053379311736,
6.15180984537846));
#163187=CARTESIAN_POINT('Ctrl Pts',(3.87606472234309,0.582224590119441,
6.2248203509263));
#163188=CARTESIAN_POINT('Ctrl Pts',(3.79803484175112,0.602198953352741,
6.29607352398231));
#163189=CARTESIAN_POINT('Ctrl Pts',(3.67865339709232,0.631811121720754,
6.40010311370272));
#163190=CARTESIAN_POINT('Ctrl Pts',(3.63855221784974,0.641604433110253,
6.43423913857157));
#163191=CARTESIAN_POINT('Ctrl Pts',(3.55409282914178,0.661914302620708,
6.50446418606829));
#163192=CARTESIAN_POINT('Ctrl Pts',(3.51296570938833,0.67162085133905,6.53772613200226));
#163193=CARTESIAN_POINT('Ctrl Pts',(3.47445461360268,0.680609080045858,
6.56826586234716));
#163194=CARTESIAN_POINT('Ctrl Pts',(3.909319254,0.810731746,6.105712323));
#163195=CARTESIAN_POINT('Ctrl Pts',(4.244535298,0.745065281,5.891082733));
#163196=CARTESIAN_POINT('Ctrl Pts',(4.554240196,0.680609079,5.64104566900001));
#163197=CARTESIAN_POINT('Ctrl Pts',(3.834803774,0.810731746,6.44548524300001));
#163198=CARTESIAN_POINT('Ctrl Pts',(4.188674043,0.745065281,6.234946704));
#163199=CARTESIAN_POINT('Ctrl Pts',(4.517368912,0.680609079,5.98693394900001));
#163200=CARTESIAN_POINT('Ctrl Pts',(3.82919545491968,0.810731746,6.47105784818504));
#163201=CARTESIAN_POINT('Ctrl Pts',(4.18446971200371,0.745065281,6.26082721727852));
#163202=CARTESIAN_POINT('Ctrl Pts',(4.51459383861158,0.680609079,6.0129668194906));
#163203=CARTESIAN_POINT('',(4.5407835784437,0.680609081791273,5.7672818619153));
#163204=CARTESIAN_POINT('Ctrl Pts',(4.554240196,0.680609079,5.641045669));
#163205=CARTESIAN_POINT('Ctrl Pts',(4.859919172,0.745496505000001,5.394258892));
#163206=CARTESIAN_POINT('Ctrl Pts',(5.13714059500001,0.810723991,5.11588570100001));
#163207=CARTESIAN_POINT('Ctrl Pts',(4.900128476,0.680609079,5.677916952));
#163208=CARTESIAN_POINT('Ctrl Pts',(5.207805447,0.745496505,5.412387059));
#163209=CARTESIAN_POINT('Ctrl Pts',(5.484987794,0.810723991,5.115164602));
#163210=CARTESIAN_POINT('Ctrl Pts',(4.92611735858291,0.680609079,5.68068733625404));
#163211=CARTESIAN_POINT('Ctrl Pts',(5.23394445221053,0.745496505,5.41374914852672));
#163212=CARTESIAN_POINT('Ctrl Pts',(5.51112386317125,0.810723991,5.11511042104527));
#163213=CARTESIAN_POINT('',(4.80520680196463,0.680609080418716,5.66779841952658));
#163214=CARTESIAN_POINT('',(4.68047638465213,0.680609082082805,5.65450231179023));
#163215=CARTESIAN_POINT('',(5.32426794337827,0.767980175627075,5.30753291231732));
#163216=CARTESIAN_POINT('Ctrl Pts',(4.80520680463989,0.680609079133469,
5.66779841310038));
#163217=CARTESIAN_POINT('Ctrl Pts',(4.89392709595556,0.695136944934551,
5.61162696295109));
#163218=CARTESIAN_POINT('Ctrl Pts',(4.98145781965976,0.709660812623477,
5.55359646132803));
#163219=CARTESIAN_POINT('Ctrl Pts',(5.15456749200145,0.738780776780364,
5.4335276963075));
#163220=CARTESIAN_POINT('Ctrl Pts',(5.24011248597806,0.753373671704646,
5.37147940132803));
#163221=CARTESIAN_POINT('Ctrl Pts',(5.32432342063299,0.767949007828576,
5.30764895191927));
#163222=CARTESIAN_POINT('Ctrl Pts',(5.13383323629986,0.809946052590815,
5.11920465603347));
#163223=CARTESIAN_POINT('Ctrl Pts',(5.16398031444869,0.802922931346625,
5.14907239727279));
#163224=CARTESIAN_POINT('Ctrl Pts',(5.19418276650767,0.796078752460896,
5.17896529494774));
#163225=CARTESIAN_POINT('Ctrl Pts',(5.2576154669957,0.782074140043799,5.24169107672195));
#163226=CARTESIAN_POINT('Ctrl Pts',(5.29089482450484,0.774939590271432,
5.27456688412485));
#163227=CARTESIAN_POINT('Ctrl Pts',(5.32418533538452,0.767997185238257,
5.30742403456664));
#163228=CARTESIAN_POINT('Origin',(4.23272528138341E-13,0.560925700000045,
4.69242700251726E-13));
#163229=CARTESIAN_POINT('',(5.68824578855907,0.680609080239763,4.78098433135749));
#163230=CARTESIAN_POINT('',(5.18243931891629,0.562053379594032,5.15833765197501));
#163231=CARTESIAN_POINT('Ctrl Pts',(5.68824578738182,0.680609080006679,
4.78098432984365));
#163232=CARTESIAN_POINT('Ctrl Pts',(5.65115860086945,0.671661524746398,
4.8112030540888));
#163233=CARTESIAN_POINT('Ctrl Pts',(5.60978467527665,0.661738573380851,
4.84431382069644));
#163234=CARTESIAN_POINT('Ctrl Pts',(5.52307368641531,0.641119488099716,
4.91191989931352));
#163235=CARTESIAN_POINT('Ctrl Pts',(5.48138123678228,0.631275792512947,
4.94371763787759));
#163236=CARTESIAN_POINT('Ctrl Pts',(5.35502126062242,0.601654471582552,
5.03798075320548));
#163237=CARTESIAN_POINT('Ctrl Pts',(5.26936895293617,0.581858134996619,
5.0990755126484));
#163238=CARTESIAN_POINT('Ctrl Pts',(5.18243931919477,0.562053380229362,
5.15833765259582));
#163239=CARTESIAN_POINT('Ctrl Pts',(5.32435055137201,0.767963166015893,
5.307641790068));
#163240=CARTESIAN_POINT('Ctrl Pts',(5.38884544570401,0.753333602523817,
5.22222194381651));
#163241=CARTESIAN_POINT('Ctrl Pts',(5.45153383068676,0.738713518204724,
5.1354505872009));
#163242=CARTESIAN_POINT('Ctrl Pts',(5.57285303448452,0.709588702185143,
4.95982721477735));
#163243=CARTESIAN_POINT('Ctrl Pts',(5.63149237997482,0.695086899228591,
4.87100895977395));
#163244=CARTESIAN_POINT('Ctrl Pts',(5.68824578310611,0.680609079003327,
4.78098433337133));
#163245=CARTESIAN_POINT('Ctrl Pts',(5.18243931864758,0.562053379320748,
5.15833765185759));
#163246=CARTESIAN_POINT('Ctrl Pts',(5.12359685382635,0.582224590076786,
5.24604817094438));
#163247=CARTESIAN_POINT('Ctrl Pts',(5.06270859463274,0.602198953250477,
5.33240960193516));
#163248=CARTESIAN_POINT('Ctrl Pts',(4.96848150840265,0.631811121639871,
5.45967051949857));
#163249=CARTESIAN_POINT('Ctrl Pts',(4.93665610844004,0.641604433114055,
5.50162903160987));
#163250=CARTESIAN_POINT('Ctrl Pts',(4.8692674654864,0.661914356005798,5.5883687565125));
#163251=CARTESIAN_POINT('Ctrl Pts',(4.8362522563773,0.671620886396292,5.629694100555));
#163252=CARTESIAN_POINT('Ctrl Pts',(4.80520680015511,0.680609080072647,
5.6677984181339));
#163253=CARTESIAN_POINT('Ctrl Pts',(5.130469208,0.810731746,5.12257608100001));
#163254=CARTESIAN_POINT('Ctrl Pts',(5.41170907,0.745065281,4.840902871));
#163255=CARTESIAN_POINT('Ctrl Pts',(5.660422662,0.680609079,4.530134136));
#163256=CARTESIAN_POINT('Ctrl Pts',(5.130736993,0.810731746,5.47042392400001));
#163257=CARTESIAN_POINT('Ctrl Pts',(5.431074409,0.745065281,5.188736012));
#163258=CARTESIAN_POINT('Ctrl Pts',(5.698769164,0.680609079,4.875861977));
#163259=CARTESIAN_POINT('Ctrl Pts',(5.13075714752001,0.810731746,5.49660427881381));
#163260=CARTESIAN_POINT('Ctrl Pts',(5.43253191824237,0.745065281,5.21491526028523));
#163261=CARTESIAN_POINT('Ctrl Pts',(5.70165526793432,0.680609079,4.9018827723809));
#163262=CARTESIAN_POINT('',(5.674417702854,0.680609081791274,4.65631177227276));
#163263=CARTESIAN_POINT('Ctrl Pts',(5.660422662,0.680609079,4.530134136));
#163264=CARTESIAN_POINT('Ctrl Pts',(5.905903171,0.745496505000001,4.223405152));
#163265=CARTESIAN_POINT('Ctrl Pts',(6.116801304,0.810723991,3.891945762));
#163266=CARTESIAN_POINT('Ctrl Pts',(6.006150502,0.680609079,4.491787634));
#163267=CARTESIAN_POINT('Ctrl Pts',(6.249553078,0.745496505000001,4.166324228));
#163268=CARTESIAN_POINT('Ctrl Pts',(6.456361013,0.810723991,3.816464655));
#163269=CARTESIAN_POINT('Ctrl Pts',(6.03212733019216,0.680609079,4.48890640669061));
#163270=CARTESIAN_POINT('Ctrl Pts',(6.27537377728876,0.745496505000001,
4.16203535917243));
#163271=CARTESIAN_POINT('Ctrl Pts',(6.48187438855481,0.810723991,3.81079325824962));
#163272=CARTESIAN_POINT('',(5.91127285818404,0.680609080424646,4.502311021008));
#163273=CARTESIAN_POINT('',(5.7866002991413,0.680609082082805,4.51613912119474));
#163274=CARTESIAN_POINT('',(6.34075220412026,0.767980175591255,4.0388855187467));
#163275=CARTESIAN_POINT('Ctrl Pts',(5.91127285940175,0.68060907913183,4.50231101419889));
#163276=CARTESIAN_POINT('Ctrl Pts',(5.98584371810131,0.695136944892643,
4.42838058139215));
#163277=CARTESIAN_POINT('Ctrl Pts',(6.05885317952404,0.709660812546431,
4.35289028258863));
#163278=CARTESIAN_POINT('Ctrl Pts',(6.20210440905884,0.738780776759475,
4.19841519563974));
#163279=CARTESIAN_POINT('Ctrl Pts',(6.27231085937759,0.753373671676262,
4.11942791022291));
#163280=CARTESIAN_POINT('Ctrl Pts',(6.34083132940497,0.767949007777661,
4.03898691946156));
#163281=CARTESIAN_POINT('Ctrl Pts',(6.11428474712324,0.809946052491448,
3.89589810638952));
#163282=CARTESIAN_POINT('Ctrl Pts',(6.15014768492995,0.802922931193169,
3.9185868255266));
#163283=CARTESIAN_POINT('Ctrl Pts',(6.18607010946796,0.796078752357421,
3.94128820902625));
#163284=CARTESIAN_POINT('Ctrl Pts',(6.26150397751342,0.782074139939529,
3.98891134102536));
#163285=CARTESIAN_POINT('Ctrl Pts',(6.30107260881191,0.774939590191973,
4.01386445207685));
#163286=CARTESIAN_POINT('Ctrl Pts',(6.34064812196814,0.767997185198326,
4.03879694473977));
#163287=CARTESIAN_POINT('Origin',(1.99493199737333E-14,0.560925700000045,
3.53449908230274E-14));
#163288=CARTESIAN_POINT('',(6.5830280693915,0.680609080232035,3.4464028733435));
#163289=CARTESIAN_POINT('',(6.17016688332989,0.562053379630163,3.92366732259758));
#163290=CARTESIAN_POINT('Ctrl Pts',(6.58302806789696,0.680609079983393,
3.44640287209903));
#163291=CARTESIAN_POINT('Ctrl Pts',(6.55330409170877,0.671661524738439,
3.48388774809406));
#163292=CARTESIAN_POINT('Ctrl Pts',(6.52001530162182,0.661738573384056,
3.52511857431923));
#163293=CARTESIAN_POINT('Ctrl Pts',(6.44986487602543,0.641119488114012,
3.6097843597748));
#163294=CARTESIAN_POINT('Ctrl Pts',(6.41598274652342,0.631275792517561,
3.64980132916812));
#163295=CARTESIAN_POINT('Ctrl Pts',(6.31284077969711,0.601654471558908,
3.76902428504385));
#163296=CARTESIAN_POINT('Ctrl Pts',(6.24232454263553,0.581858134953565,
3.84710339731782));
#163297=CARTESIAN_POINT('Ctrl Pts',(6.17016688366903,0.562053380161616,
3.92366732305467));
#163298=CARTESIAN_POINT('Ctrl Pts',(6.34085628627237,0.767963165984184,
4.03897409275364));
#163299=CARTESIAN_POINT('Ctrl Pts',(6.38548058389055,0.753333602495987,
3.94168681918178));
#163300=CARTESIAN_POINT('Ctrl Pts',(6.42805007255938,0.738713518174777,
3.84346797891347));
#163301=CARTESIAN_POINT('Ctrl Pts',(6.50877906791305,0.709588701869491,
3.6458705387371));
#163302=CARTESIAN_POINT('Ctrl Pts',(6.54695415822974,0.695086899074947,
3.54652308034844));
#163303=CARTESIAN_POINT('Ctrl Pts',(6.58302806441533,0.680609078994068,
3.44640287661631));
#163304=CARTESIAN_POINT('Ctrl Pts',(6.17016688308926,0.562053379401562,
3.92366732254997));
#163305=CARTESIAN_POINT('Ctrl Pts',(6.13155529124598,0.582224590154151,
4.02197660907586));
#163306=CARTESIAN_POINT('Ctrl Pts',(6.09065572053444,0.602198953333873,
4.11940813371797));
#163307=CARTESIAN_POINT('Ctrl Pts',(6.02598894669228,0.631811121710703,
4.26394979991525));
#163308=CARTESIAN_POINT('Ctrl Pts',(6.00392744676189,0.641604433160521,
4.31176886545943));
#163309=CARTESIAN_POINT('Ctrl Pts',(5.95676085305035,0.661914328754221,
4.41096709673942));
#163310=CARTESIAN_POINT('Ctrl Pts',(5.93340123289289,0.671620868693789,
4.45842361264364));
#163311=CARTESIAN_POINT('Ctrl Pts',(5.91127285614981,0.680609080090536,
4.50231102005075));
#163312=CARTESIAN_POINT('Ctrl Pts',(6.111724124,0.810731746,3.899913875));
#163313=CARTESIAN_POINT('Ctrl Pts',(6.32583734,0.745065281,3.564367771));
#163314=CARTESIAN_POINT('Ctrl Pts',(6.501930055,0.680609079,3.207398566));
#163315=CARTESIAN_POINT('Ctrl Pts',(6.186762652,0.810731746,4.239571663));
#163316=CARTESIAN_POINT('Ctrl Pts',(6.419523772,0.745065281,3.899905791));
#163317=CARTESIAN_POINT('Ctrl Pts',(6.61370130300001,0.680609079,3.536800117));
#163318=CARTESIAN_POINT('Ctrl Pts',(6.19241033773507,0.810731746,4.26513560322141));
#163319=CARTESIAN_POINT('Ctrl Pts',(6.42657497009355,0.745065281,3.92515966177328));
#163320=CARTESIAN_POINT('Ctrl Pts',(6.62211363330213,0.680609079,3.56159213371832));
#163321=CARTESIAN_POINT('',(6.5427223617568,0.680609081791281,3.32761771924868));
#163322=CARTESIAN_POINT('Ctrl Pts',(6.501930055,0.680609079,3.207398566));
#163323=CARTESIAN_POINT('Ctrl Pts',(6.675733702,0.745496505000001,2.855069682));
#163324=CARTESIAN_POINT('Ctrl Pts',(6.81044718200001,0.810723991,2.486022764));
#163325=CARTESIAN_POINT('Ctrl Pts',(6.831331606,0.680609079,3.095627318));
#163326=CARTESIAN_POINT('Ctrl Pts',(6.999078553,0.745496505000001,2.725448706));
#163327=CARTESIAN_POINT('Ctrl Pts',(7.12584196800001,0.810723991,2.339311063));
#163328=CARTESIAN_POINT('Ctrl Pts',(6.85608173160809,0.680609079,3.08722920202582));
#163329=CARTESIAN_POINT('Ctrl Pts',(7.02337359852327,0.745496505000001,
2.71570942144684));
#163330=CARTESIAN_POINT('Ctrl Pts',(7.14953967235489,0.810723991,2.32828763880268));
#163331=CARTESIAN_POINT('',(6.74093436582087,0.680609080455689,3.12630056270069));
#163332=CARTESIAN_POINT('',(6.62214921468494,0.680609082082812,3.16660628438882));
#163333=CARTESIAN_POINT('',(7.06074993928123,0.767980175616009,2.58138432684563));
#163334=CARTESIAN_POINT('Ctrl Pts',(6.74093436550991,0.680609079128079,
3.12630055604194));
#163335=CARTESIAN_POINT('Ctrl Pts',(6.79786894095172,0.695136944786355,
3.03806804583507));
#163336=CARTESIAN_POINT('Ctrl Pts',(6.85294329871174,0.709660812346982,
2.94864779267141));
#163337=CARTESIAN_POINT('Ctrl Pts',(6.95963781737309,0.738780776736229,
2.76698946628084));
#163338=CARTESIAN_POINT('Ctrl Pts',(7.01122294842257,0.753373671662706,
2.6747565480841));
#163339=CARTESIAN_POINT('Ctrl Pts',(7.0608490127954,0.767949007789042,2.58146634729615));
#163340=CARTESIAN_POINT('Ctrl Pts',(6.80883909838719,0.809946052553749,
2.49042368966192));
#163341=CARTESIAN_POINT('Ctrl Pts',(6.84874098462263,0.80292293123736,2.50487248776642));
#163342=CARTESIAN_POINT('Ctrl Pts',(6.88870368917698,0.796078752408176,
2.51932086611966));
#163343=CARTESIAN_POINT('Ctrl Pts',(6.97261152107854,0.782074139968656,
2.54961454392142));
#163344=CARTESIAN_POINT('Ctrl Pts',(7.01661924109567,0.774939590214728,
2.56547817894248));
#163345=CARTESIAN_POINT('Ctrl Pts',(7.06062924972398,0.767997185218944,
2.58132019820442));
#163346=CARTESIAN_POINT('Origin',(1.26504709485609E-12,0.560925699999955,
4.67941657644744E-13));
#163347=CARTESIAN_POINT('',(7.16999527408755,0.680609080192563,1.95067144819131));
#163348=CARTESIAN_POINT('',(6.86938430225266,0.562053379538648,2.5055306689776));
#163349=CARTESIAN_POINT('Ctrl Pts',(7.1699952722679,0.68060907998119,1.95067144725986));
#163350=CARTESIAN_POINT('Ctrl Pts',(7.14902436655433,0.671661524774049,
1.99366972355771));
#163351=CARTESIAN_POINT('Ctrl Pts',(7.125377258842,0.661738573439555,2.04109270155846));
#163352=CARTESIAN_POINT('Ctrl Pts',(7.07506755250471,0.641119488180572,
2.13885931550801));
#163353=CARTESIAN_POINT('Ctrl Pts',(7.05058003388874,0.631275792568541,
2.1852243666409));
#163354=CARTESIAN_POINT('Ctrl Pts',(6.97547888030251,0.60165447159557,2.32383242984726));
#163355=CARTESIAN_POINT('Ctrl Pts',(6.92339597490006,0.581858135006135,
2.4152450022131));
#163356=CARTESIAN_POINT('Ctrl Pts',(6.86938430282194,0.562053380243108,
2.50553066947269));
#163357=CARTESIAN_POINT('Ctrl Pts',(7.06087062883848,0.767963166013075,
2.58144845548684));
#163358=CARTESIAN_POINT('Ctrl Pts',(7.08353774714955,0.75333360255102,2.47684279946778));
#163359=CARTESIAN_POINT('Ctrl Pts',(7.10399783748468,0.738713518238969,
2.37176907944768));
#163360=CARTESIAN_POINT('Ctrl Pts',(7.14036182541816,0.709588701622422,
2.16143700787481));
#163361=CARTESIAN_POINT('Ctrl Pts',(7.1562876362193,0.695086898948571,2.05620572292349));
#163362=CARTESIAN_POINT('Ctrl Pts',(7.16999527007506,0.680609078987201,
1.95067145153359));
#163363=CARTESIAN_POINT('Ctrl Pts',(6.86938430192758,0.562053379235629,
2.50553066898454));
#163364=CARTESIAN_POINT('Ctrl Pts',(6.85280901821899,0.582224589991481,
2.60984189004187));
#163365=CARTESIAN_POINT('Ctrl Pts',(6.83381055446812,0.602198953194961,
2.71378771864018));
#163366=CARTESIAN_POINT('Ctrl Pts',(6.8017278394544,0.631811121640532,2.86885152610303));
#163367=CARTESIAN_POINT('Ctrl Pts',(6.79046181068709,0.641604433126681,
2.920295178957));
#163368=CARTESIAN_POINT('Ctrl Pts',(6.76572262811083,0.661914332930743,
3.02731365616675));
#163369=CARTESIAN_POINT('Ctrl Pts',(6.75311089226061,0.671620871200531,
3.07868228515498));
#163370=CARTESIAN_POINT('Ctrl Pts',(6.74093436379984,0.680609080182541,
3.12630056223545));
#163371=CARTESIAN_POINT('Ctrl Pts',(6.807201613,0.810731746,2.49489603));
#163372=CARTESIAN_POINT('Ctrl Pts',(6.94417648700001,0.745065281,2.121166795));
#163373=CARTESIAN_POINT('Ctrl Pts',(7.039414425,0.680609079,1.734688604));
#163374=CARTESIAN_POINT('Ctrl Pts',(6.953502166,0.810731746,2.810481743));
#163375=CARTESIAN_POINT('Ctrl Pts',(7.107803339,0.745065281,2.428720309));
#163376=CARTESIAN_POINT('Ctrl Pts',(7.21938412,0.680609079,2.032361415));
#163377=CARTESIAN_POINT('Ctrl Pts',(6.96451330330129,0.810731746,2.83423392674035));
#163378=CARTESIAN_POINT('Ctrl Pts',(7.12011851961009,0.745065281,2.4518679588257));
#163379=CARTESIAN_POINT('Ctrl Pts',(7.23292932527149,0.680609079,2.0547654054537));
#163380=CARTESIAN_POINT('',(7.10509659429687,0.680609081791282,1.84332795993776));
#163381=CARTESIAN_POINT('Ctrl Pts',(7.039414425,0.680609079,1.734688604));
#163382=CARTESIAN_POINT('Ctrl Pts',(7.133414344,0.745496505000001,1.353234327));
#163383=CARTESIAN_POINT('Ctrl Pts',(7.185644119,0.810723991,0.963856104));
#163384=CARTESIAN_POINT('Ctrl Pts',(7.337087236,0.680609079,1.554718909));
#163385=CARTESIAN_POINT('Ctrl Pts',(7.421334894,0.745496505000001,1.157134232));
#163386=CARTESIAN_POINT('Ctrl Pts',(7.462126472,0.810723991,0.752773886));
#163387=CARTESIAN_POINT('Ctrl Pts',(7.35945337054856,0.680609079,1.54119659099081));
#163388=CARTESIAN_POINT('Ctrl Pts',(7.44296827643409,0.745496505000001,
1.14239992994863));
#163389=CARTESIAN_POINT('Ctrl Pts',(7.48290042675498,0.810723991,0.736913877580905));
#163390=CARTESIAN_POINT('',(7.2553972746655,0.680609080401357,1.60410776492566));
#163391=CARTESIAN_POINT('',(7.14805379311743,0.680609082082812,1.66900645776976));
#163392=CARTESIAN_POINT('',(7.45059485449452,0.767980175618517,1.00318047335778));
#163393=CARTESIAN_POINT('Ctrl Pts',(7.25539727289291,0.68060907913724,1.60410775805583));
#163394=CARTESIAN_POINT('Ctrl Pts',(7.29203336852415,0.695136944988277,
1.50569882284163));
#163395=CARTESIAN_POINT('Ctrl Pts',(7.3265974075645,0.709660812732467,1.40652980529827));
#163396=CARTESIAN_POINT('Ctrl Pts',(7.39174629634048,0.738780776713929,
1.20618238492266));
#163397=CARTESIAN_POINT('Ctrl Pts',(7.42229804465085,0.753373671641964,
1.10501654288154));
#163398=CARTESIAN_POINT('Ctrl Pts',(7.45070924368572,0.767949007780856,
1.00323927836238));
#163399=CARTESIAN_POINT('Ctrl Pts',(7.18501969994167,0.809946052636564,
0.968499828836897));
#163400=CARTESIAN_POINT('Ctrl Pts',(7.22709476677672,0.802922931348075,
0.974033096202646));
#163401=CARTESIAN_POINT('Ctrl Pts',(7.26922914024265,0.796078752458098,
0.979552879520431));
#163402=CARTESIAN_POINT('Ctrl Pts',(7.35768749908181,0.782074140010044,
0.991100604673837));
#163403=CARTESIAN_POINT('Ctrl Pts',(7.40407655575484,0.774939590240218,
0.997132997879333));
#163404=CARTESIAN_POINT('Ctrl Pts',(7.45046320082775,0.767997185218328,
1.00314378867028));
#163405=CARTESIAN_POINT('Origin',(-1.05861500121485E-12,0.560925700000134,
-1.37422625362538E-14));
#163406=CARTESIAN_POINT('',(7.42170146886965,0.680609080233179,0.363728792693982));
#163407=CARTESIAN_POINT('',(7.24739694553545,0.562053379620976,0.970238187390015));
#163408=CARTESIAN_POINT('Ctrl Pts',(7.42170146700829,0.680609079992507,
0.363728792197865));
#163409=CARTESIAN_POINT('Ctrl Pts',(7.41046420776432,0.671661524759858,
0.410229917826462));
#163410=CARTESIAN_POINT('Ctrl Pts',(7.39756449471215,0.661738573404569,
0.461627602379835));
#163411=CARTESIAN_POINT('Ctrl Pts',(7.36944793333281,0.641119488121199,
0.567923587341595));
#163412=CARTESIAN_POINT('Ctrl Pts',(7.35550003476589,0.631275792530468,
0.618468741997286));
#163413=CARTESIAN_POINT('Ctrl Pts',(7.31195134080634,0.601654471595934,
0.769980753821589));
#163414=CARTESIAN_POINT('Ctrl Pts',(7.28073710570731,0.581858135014435,
0.870452436201094));
#163415=CARTESIAN_POINT('Ctrl Pts',(7.24739694613023,0.562053380253525,
0.970238187714283));
#163416=CARTESIAN_POINT('Ctrl Pts',(7.45072650816129,0.767963166018706,
1.00321715804528));
#163417=CARTESIAN_POINT('Ctrl Pts',(7.45037655791925,0.753333602551921,
0.896184363727295));
#163418=CARTESIAN_POINT('Ctrl Pts',(7.4477705588714,0.73871351824202,0.78916889425916));
#163419=CARTESIAN_POINT('Ctrl Pts',(7.43806919902117,0.709588701781099,
0.575937088238746));
#163420=CARTESIAN_POINT('Ctrl Pts',(7.43100105757009,0.695086899033531,
0.469742473131814));
#163421=CARTESIAN_POINT('Ctrl Pts',(7.42170146573539,0.680609078990994,
0.363728797710933));
#163422=CARTESIAN_POINT('Ctrl Pts',(7.24739694525172,0.562053379348888,
0.970238187458852));
#163423=CARTESIAN_POINT('Ctrl Pts',(7.25363301157249,0.58222459010264,1.07567386611614));
#163424=CARTESIAN_POINT('Ctrl Pts',(7.25742400185949,0.602198953284748,
1.18127360706405));
#163425=CARTESIAN_POINT('Ctrl Pts',(7.25942549781448,0.631811121645755,
1.33960894389367));
#163426=CARTESIAN_POINT('Ctrl Pts',(7.25948172723322,0.641604433069193,
1.39227173559095));
#163427=CARTESIAN_POINT('Ctrl Pts',(7.25832674329939,0.661914312715681,
1.50210626427859));
#163428=CARTESIAN_POINT('Ctrl Pts',(7.25705260194503,0.671620857839493,
1.5549851053256));
#163429=CARTESIAN_POINT('Ctrl Pts',(7.25539727228099,0.680609080020491,
1.60410776491499));
#163430=CARTESIAN_POINT('Ctrl Pts',(7.18438192,0.810731746,0.97321962));
#163431=CARTESIAN_POINT('Ctrl Pts',(7.23781366,0.745065281,0.578782418));
#163432=CARTESIAN_POINT('Ctrl Pts',(7.2477436,0.680609079,0.180866531));
#163433=CARTESIAN_POINT('Ctrl Pts',(7.39510364700001,0.810731746,1.24997682));
#163434=CARTESIAN_POINT('Ctrl Pts',(7.463729921,0.745065281,0.843970566000001));
#163435=CARTESIAN_POINT('Ctrl Pts',(7.48749656,0.680609079,0.432891753));
#163436=CARTESIAN_POINT('Ctrl Pts',(7.41096336723259,0.810731746,1.27080662159114));
#163437=CARTESIAN_POINT('Ctrl Pts',(7.48073323976765,0.745065281,0.863929636648076));
#163438=CARTESIAN_POINT('Ctrl Pts',(7.50554128146593,0.680609079,0.451860131673525));
#163439=CARTESIAN_POINT('',(7.33524440713602,0.680609081791281,0.272846233901281));
#163440=CARTESIAN_POINT('Ctrl Pts',(7.2477436,0.680609079,0.180866531));
#163441=CARTESIAN_POINT('Ctrl Pts',(7.25754446000001,0.745496505000001,
-0.211876761));
#163442=CARTESIAN_POINT('Ctrl Pts',(7.22484832400001,0.810723991,-0.603379396));
#163443=CARTESIAN_POINT('Ctrl Pts',(7.499768822,0.680609079,-0.058886428));
#163444=CARTESIAN_POINT('Ctrl Pts',(7.496577864,0.745496505000001,-0.465286552));
#163445=CARTESIAN_POINT('Ctrl Pts',(7.449490235,0.810723991,-0.868962162));
#163446=CARTESIAN_POINT('Ctrl Pts',(7.51870515021548,0.680609079,-0.076900659616291));
#163447=CARTESIAN_POINT('Ctrl Pts',(7.51453803067176,0.745496505000001,
-0.4843269120771));
#163448=CARTESIAN_POINT('Ctrl Pts',(7.46636907325234,0.810723991,-0.888917158509634));
#163449=CARTESIAN_POINT('',(7.43060587058891,0.680609080425494,0.00690867068859535));
#163450=CARTESIAN_POINT('',(7.33880352304754,0.680609082082812,0.0942407518356454));
#163451=CARTESIAN_POINT('',(7.49205823513684,0.767980175622892,-0.621930984430037));
#163452=CARTESIAN_POINT('Ctrl Pts',(7.43060586743964,0.680609079131675,
0.00690866453753127));
#163453=CARTESIAN_POINT('Ctrl Pts',(7.44523041930225,0.695136944893849,
-0.0970752012570951));
#163454=CARTESIAN_POINT('Ctrl Pts',(7.45766796293523,0.709660812543815,
-0.201355948185125));
#163455=CARTESIAN_POINT('Ctrl Pts',(7.47822493391373,0.738780776767852,
-0.411024444247337));
#163456=CARTESIAN_POINT('Ctrl Pts',(7.48631473371831,0.753373671689276,
-0.516392807950393));
#163457=CARTESIAN_POINT('Ctrl Pts',(7.49218259132217,0.767949007805525,
-0.621898144596978));
#163458=CARTESIAN_POINT('Ctrl Pts',(7.22523676700086,0.80994605257742,-0.598710006733521));
#163459=CARTESIAN_POINT('Ctrl Pts',(7.26751763093187,0.802922931299024,
-0.602350999705705));
#163460=CARTESIAN_POINT('Ctrl Pts',(7.3098535164192,0.79607875240577,-0.606017910679099));
#163461=CARTESIAN_POINT('Ctrl Pts',(7.39872618738651,0.782074139992209,
-0.613756097291337));
#163462=CARTESIAN_POINT('Ctrl Pts',(7.44532747993427,0.774939590232648,
-0.617837014054864));
#163463=CARTESIAN_POINT('Ctrl Pts',(7.49192177335025,0.767997185228654,
-0.621938509756826));
#163464=CARTESIAN_POINT('Origin',(9.68409380464053E-13,0.560925700000022,
-7.01377161644451E-14));
#163465=CARTESIAN_POINT('',(7.32637715136353,0.680609080273142,-1.24022141673702));
#163466=CARTESIAN_POINT('',(7.28652936266848,0.562053379784689,-0.610421555804528));
#163467=CARTESIAN_POINT('Ctrl Pts',(7.32637714962487,0.680609080098861,
-1.24022141680518));
#163468=CARTESIAN_POINT('Ctrl Pts',(7.32539897868996,0.671661524913783,
-1.19239178347266));
#163469=CARTESIAN_POINT('Ctrl Pts',(7.32384983662865,0.661738573559669,
-1.13942269132726));
#163470=CARTESIAN_POINT('Ctrl Pts',(7.31924111951911,0.641119488285343,
-1.02956761794737));
#163471=CARTESIAN_POINT('Ctrl Pts',(7.31648502923072,0.631275792705557,
-0.977205795057172));
#163472=CARTESIAN_POINT('Ctrl Pts',(7.30652508348097,0.601654471841923,
-0.819874368190679));
#163473=CARTESIAN_POINT('Ctrl Pts',(7.29763906171505,0.581858135332135,
-0.715041520235852));
#163474=CARTESIAN_POINT('Ctrl Pts',(7.2865293635274,0.562053380619792,-0.610421555555234));
#163475=CARTESIAN_POINT('Ctrl Pts',(7.49219469692343,0.76796316601713,-0.621923459103248));
#163476=CARTESIAN_POINT('Ctrl Pts',(7.46884404140746,0.753333602554716,
-0.726378657295504));
#163477=CARTESIAN_POINT('Ctrl Pts',(7.44329380657706,0.73871351824609,-0.830331951877381));
#163478=CARTESIAN_POINT('Ctrl Pts',(7.38798072444135,0.709588702079347,
-1.03649300931035));
#163479=CARTESIAN_POINT('Ctrl Pts',(7.35824912877455,0.695086899177824,
-1.13868541307905));
#163480=CARTESIAN_POINT('Ctrl Pts',(7.32637714941249,0.680609078999391,
-1.24022141147247));
#163481=CARTESIAN_POINT('Ctrl Pts',(7.28652936194102,0.562053379030082,
-0.610421555448924));
#163482=CARTESIAN_POINT('Ctrl Pts',(7.31528607861313,0.582225215395378,
-0.508788322522507));
#163483=CARTESIAN_POINT('Ctrl Pts',(7.34168762411948,0.60219834043125,-0.406478737699217));
#163484=CARTESIAN_POINT('Ctrl Pts',(7.37768078505445,0.63181136590102,-0.252270992317658));
#163485=CARTESIAN_POINT('Ctrl Pts',(7.38905691094103,0.641604918991269,
-0.200850235723201));
#163486=CARTESIAN_POINT('Ctrl Pts',(7.41154005366641,0.661914800536601,
-0.0933352359651138));
#163487=CARTESIAN_POINT('Ctrl Pts',(7.42166281552644,0.671621097024362,
-0.0414200839496619));
#163488=CARTESIAN_POINT('Ctrl Pts',(7.4306058683949,0.68060908009308,0.00690867115641031));
#163489=CARTESIAN_POINT('Ctrl Pts',(7.22562851299999,0.810731746,-0.593963458000001));
#163490=CARTESIAN_POINT('Ctrl Pts',(7.193018709,0.745065281,-0.990665182));
#163491=CARTESIAN_POINT('Ctrl Pts',(7.11717634,0.680609079,-1.381412661));
#163492=CARTESIAN_POINT('Ctrl Pts',(7.4909183,0.810731746,-0.36897563));
#163493=CARTESIAN_POINT('Ctrl Pts',(7.470660787,0.745065281,-0.780242304));
#163494=CARTESIAN_POINT('Ctrl Pts',(7.405501982,0.680609079,-1.186819448));
#163495=CARTESIAN_POINT('Ctrl Pts',(7.51088502066177,0.810731746,-0.352042188404765));
#163496=CARTESIAN_POINT('Ctrl Pts',(7.49155718816973,0.745065281,-0.764405076063766));
#163497=CARTESIAN_POINT('Ctrl Pts',(7.4272024689224,0.680609079,-1.1721736209948));
#163498=CARTESIAN_POINT('',(7.22240434444543,0.680609081791281,-1.31039347883568));
#163499=CARTESIAN_POINT('Ctrl Pts',(7.11717634000001,0.680609079,-1.381412661));
#163500=CARTESIAN_POINT('Ctrl Pts',(7.04231986300001,0.745496505000001,
-1.767080728));
#163501=CARTESIAN_POINT('Ctrl Pts',(6.926226651,0.810723991,-2.142401545));
#163502=CARTESIAN_POINT('Ctrl Pts',(7.311769554,0.680609079,-1.669738302));
#163503=CARTESIAN_POINT('Ctrl Pts',(7.221289184,0.745496505000001,-2.065951054));
#163504=CARTESIAN_POINT('Ctrl Pts',(7.088524115,0.810723991,-2.450066505));
#163505=CARTESIAN_POINT('Ctrl Pts',(7.32639063412096,0.680609079,-1.69140212167456));
#163506=CARTESIAN_POINT('Ctrl Pts',(7.23473633730893,0.745496505000001,
-2.08840716586741));
#163507=CARTESIAN_POINT('Ctrl Pts',(7.10071860100388,0.810723991,-2.47318341610961));
#163508=CARTESIAN_POINT('',(7.25836759458169,0.680609080422382,-1.59061346520233));
#163509=CARTESIAN_POINT('',(7.18819554290371,0.680609082082812,-1.48664064912483));
#163510=CARTESIAN_POINT('',(7.18320129951193,0.76798017563633,-2.21796164054473));
#163511=CARTESIAN_POINT('Ctrl Pts',(7.25836759016924,0.68060907912728,-1.5906134705797));
#163512=CARTESIAN_POINT('Ctrl Pts',(7.25029677077617,0.695136944811777,
-1.69531009716092));
#163513=CARTESIAN_POINT('Ctrl Pts',(7.2400262535728,0.709660812377614,-1.79982652179942));
#163514=CARTESIAN_POINT('Ctrl Pts',(7.21503008497306,0.73878077675353,-2.00901222711682));
#163515=CARTESIAN_POINT('Ctrl Pts',(7.20027966622202,0.753373671680877,
-2.11365620488811));
#163516=CARTESIAN_POINT('Ctrl Pts',(7.18332980791151,0.767949007807122,
-2.21795630136356));
#163517=CARTESIAN_POINT('Ctrl Pts',(6.92760979322194,0.809946052627665,
-2.13792482796008));
#163518=CARTESIAN_POINT('Ctrl Pts',(6.96811944822111,0.802922931326775,
-2.1505698326309));
#163519=CARTESIAN_POINT('Ctrl Pts',(7.00867726647099,0.796078752464882,
-2.16325197719105));
#163520=CARTESIAN_POINT('Ctrl Pts',(7.09380866237873,0.782074140016891,
-2.1899142465429));
#163521=CARTESIAN_POINT('Ctrl Pts',(7.1384431660475,0.774939590251537,-2.20391765404315));
#163522=CARTESIAN_POINT('Ctrl Pts',(7.18306641038926,0.767997185238686,
-2.21793965470795));
#163523=CARTESIAN_POINT('Origin',(7.68482499857726E-13,0.560925699999978,
-3.48679418671338E-13));
#163524=CARTESIAN_POINT('',(6.88847958174721,0.680609080136121,-2.78618024951889));
#163525=CARTESIAN_POINT('',(6.98495176503208,0.562053379593368,-2.16253866235914));
#163526=CARTESIAN_POINT('Ctrl Pts',(6.88847957946011,0.680609079829239,
-2.7861802491228));
#163527=CARTESIAN_POINT('Ctrl Pts',(6.89780623497149,0.671661524659695,
-2.73925856817232));
#163528=CARTESIAN_POINT('Ctrl Pts',(6.90768010001637,0.661738573367639,
-2.6871948444348));
#163529=CARTESIAN_POINT('Ctrl Pts',(6.92679472560154,0.641119488158189,
-2.57891738392072));
#163530=CARTESIAN_POINT('Ctrl Pts',(6.93535931529209,0.631275792572596,
-2.5271872733699));
#163531=CARTESIAN_POINT('Ctrl Pts',(6.95945383363896,0.601654471656685,
-2.3713930736837));
#163532=CARTESIAN_POINT('Ctrl Pts',(6.97331152558087,0.581858135084815,
-2.26710092725075));
#163533=CARTESIAN_POINT('Ctrl Pts',(6.98495176580074,0.562053380312653,
-2.16253866230847));
#163534=CARTESIAN_POINT('Ctrl Pts',(7.18333618863459,0.767963166033974,
-2.21798362638151));
#163535=CARTESIAN_POINT('Ctrl Pts',(7.13807667852258,0.753333602535863,
-2.31497701929691));
#163536=CARTESIAN_POINT('Ctrl Pts',(7.09077690848965,0.738713518201341,
-2.41100739830454));
#163537=CARTESIAN_POINT('Ctrl Pts',(6.9924384802054,0.709588701397635,-2.60045785090637));
#163538=CARTESIAN_POINT('Ctrl Pts',(6.94143364784321,0.695086898839987,
-2.69386963643605));
#163539=CARTESIAN_POINT('Ctrl Pts',(6.88847958060598,0.680609078980756,
-2.78618024402691));
#163540=CARTESIAN_POINT('Ctrl Pts',(6.98495176477214,0.562053379283973,
-2.16253866215263));
#163541=CARTESIAN_POINT('Ctrl Pts',(7.0348827576773,0.582224590025707,-2.06946628806565));
#163542=CARTESIAN_POINT('Ctrl Pts',(7.08266354766498,0.602198953223101,
-1.97521835430801));
#163543=CARTESIAN_POINT('Ctrl Pts',(7.15096333852608,0.631811121595153,
-1.83235750092));
#163544=CARTESIAN_POINT('Ctrl Pts',(7.17312690322427,0.641604433008838,
-1.78458565585862));
#163545=CARTESIAN_POINT('Ctrl Pts',(7.21819699626072,0.661914315589568,
-1.68441755785409));
#163546=CARTESIAN_POINT('Ctrl Pts',(7.23924386442132,0.67162086007449,-1.63589102589247));
#163547=CARTESIAN_POINT('Ctrl Pts',(7.25836759253305,0.680609080085683,
-1.59061346427022));
#163548=CARTESIAN_POINT('Ctrl Pts',(6.929012748,0.810731746,-2.133373465));
#163549=CARTESIAN_POINT('Ctrl Pts',(6.811886199,0.745065281,-2.513790379));
#163550=CARTESIAN_POINT('Ctrl Pts',(6.653817825,0.680609079,-2.879098531));
#163551=CARTESIAN_POINT('Ctrl Pts',(7.23646594,0.810731746,-1.97067519));
#163552=CARTESIAN_POINT('Ctrl Pts',(7.128271858,0.745065281,-2.36797191));
#163553=CARTESIAN_POINT('Ctrl Pts',(6.977234361,0.680609079,-2.751036289));
#163554=CARTESIAN_POINT('Ctrl Pts',(7.2596060389333,0.810731746,-1.95842989778076));
#163555=CARTESIAN_POINT('Ctrl Pts',(7.15208424844132,0.745065281,-2.35699705630923));
#163556=CARTESIAN_POINT('Ctrl Pts',(7.00157592203899,0.680609079,-2.74139783662219));
#163557=CARTESIAN_POINT('',(6.77185268139767,0.680609081791281,-2.83236064878544));
#163558=CARTESIAN_POINT('Ctrl Pts',(6.653817825,0.680609079,-2.879098531));
#163559=CARTESIAN_POINT('Ctrl Pts',(6.497804216,0.745496505000001,-3.239657963));
#163560=CARTESIAN_POINT('Ctrl Pts',(6.303742317,0.810723991,-3.58124738));
#163561=CARTESIAN_POINT('Ctrl Pts',(6.781880067,0.680609079,-3.202515068));
#163562=CARTESIAN_POINT('Ctrl Pts',(6.60834104800001,0.745496505000001,
-3.570013982));
#163563=CARTESIAN_POINT('Ctrl Pts',(6.39610648500001,0.810723991,-3.916608461));
#163564=CARTESIAN_POINT('Ctrl Pts',(6.79150223349964,0.680609079,-3.22681549972093));
#163565=CARTESIAN_POINT('Ctrl Pts',(6.6166464140879,0.745496505000001,-3.59483582307768));
#163566=CARTESIAN_POINT('Ctrl Pts',(6.40304641818575,0.810723991,-3.94180636561641));
#163567=CARTESIAN_POINT('',(6.74673611715292,0.680609080387324,-3.11376028311889));
#163568=CARTESIAN_POINT('',(6.70055573137004,0.680609082082812,-2.9971333764053));
#163569=CARTESIAN_POINT('',(6.53846585449635,0.767980175610573,-3.71028287566516));
#163570=CARTESIAN_POINT('Ctrl Pts',(6.74673611150703,0.680609079138449,
-3.11376028760432));
#163571=CARTESIAN_POINT('Ctrl Pts',(6.71634730295497,0.695136945031465,
-3.21427417927895));
#163572=CARTESIAN_POINT('Ctrl Pts',(6.68384896227507,0.709660812809216,
-3.31413921196611));
#163573=CARTESIAN_POINT('Ctrl Pts',(6.61446844803407,0.738780776729096,
-3.51306083143574));
#163574=CARTESIAN_POINT('Ctrl Pts',(6.57756752389879,0.753373671653006,
-3.61208738714968));
#163575=CARTESIAN_POINT('Ctrl Pts',(6.53859250620473,0.767949007785863,
-3.71030528682909));
#163576=CARTESIAN_POINT('Ctrl Pts',(6.30605548416853,0.809946052542317,
-3.57717266017008));
#163577=CARTESIAN_POINT('Ctrl Pts',(6.3428997437586,0.802922931278537,-3.59823041009158));
#163578=CARTESIAN_POINT('Ctrl Pts',(6.37978305667582,0.796078752422255,
-3.61933478530699));
#163579=CARTESIAN_POINT('Ctrl Pts',(6.4571925281524,0.78207413999555,-3.66367443941286));
#163580=CARTESIAN_POINT('Ctrl Pts',(6.49777318326057,0.774939590234295,
-3.68694555399608));
#163581=CARTESIAN_POINT('Ctrl Pts',(6.53833884531886,0.767997185214201,
-3.71023240666292));
#163582=CARTESIAN_POINT('Origin',(1.00700697780454E-12,0.560925699999933,
-5.77012396196785E-13));
#163583=CARTESIAN_POINT('',(6.12848436165721,0.680609080255617,-4.2018603922199));
#163584=CARTESIAN_POINT('',(6.3567655862665,0.562053379588068,-3.61353786574919));
#163585=CARTESIAN_POINT('Ctrl Pts',(6.12848435999572,0.680609080058053,
-4.20186039153242));
#163586=CARTESIAN_POINT('Ctrl Pts',(6.14767973809234,0.671661524805192,
-4.15804066821971));
#163587=CARTESIAN_POINT('Ctrl Pts',(6.16851491939803,0.661738573445309,
-4.10931675421297));
#163588=CARTESIAN_POINT('Ctrl Pts',(6.21045910905953,0.641119488185435,
-4.00767983985874));
#163589=CARTESIAN_POINT('Ctrl Pts',(6.22994390802001,0.631275792590329,
-3.95900028417221));
#163590=CARTESIAN_POINT('Ctrl Pts',(6.2869662575588,0.601654471628634,-3.81202807549649));
#163591=CARTESIAN_POINT('Ctrl Pts',(6.32291969295443,0.581858135013998,
-3.71315321560427));
#163592=CARTESIAN_POINT('Ctrl Pts',(6.35676558692114,0.562053380206358,
-3.6135378658487));
#163593=CARTESIAN_POINT('Ctrl Pts',(6.53859286367383,0.767963166006944,
-3.71033334466741));
#163594=CARTESIAN_POINT('Ctrl Pts',(6.47354078340064,0.753333602518642,
-3.79532962912656));
#163595=CARTESIAN_POINT('Ctrl Pts',(6.40670316287955,0.738713518200544,
-3.87894681883908));
#163596=CARTESIAN_POINT('Ctrl Pts',(6.26993758578123,0.709588701540351,
-4.04282816925933));
#163597=CARTESIAN_POINT('Ctrl Pts',(6.20004444501731,0.695086898908745,
-4.12309150837784));
#163598=CARTESIAN_POINT('Ctrl Pts',(6.12848436216369,0.680609078985776,
-4.20186038647418));
#163599=CARTESIAN_POINT('Ctrl Pts',(6.35676558608643,0.562053379322113,
-3.6135378655278));
#163600=CARTESIAN_POINT('Ctrl Pts',(6.42553702937026,0.582224590083683,
-3.53337515935516));
#163601=CARTESIAN_POINT('Ctrl Pts',(6.49246125085151,0.602198953290983,
-3.45160214738175));
#163602=CARTESIAN_POINT('Ctrl Pts',(6.58987509110844,0.631811121652785,
-3.32676373741278));
#163603=CARTESIAN_POINT('Ctrl Pts',(6.62179001855158,0.641604433060423,
-3.28487328276653));
#163604=CARTESIAN_POINT('Ctrl Pts',(6.68733942155397,0.661914267144304,
-3.19673600722322));
#163605=CARTESIAN_POINT('Ctrl Pts',(6.7183260480719,0.671620828781777,-3.15386839323973));
#163606=CARTESIAN_POINT('Ctrl Pts',(6.74673611518767,0.680609079979072,
-3.11376028163534));
#163607=CARTESIAN_POINT('Ctrl Pts',(6.308404047,0.810731746,-3.573029299));
#163608=CARTESIAN_POINT('Ctrl Pts',(6.112237461,0.745065281,-3.919373532));
#163609=CARTESIAN_POINT('Ctrl Pts',(5.879334183,0.680609079,-4.242160954));
#163610=CARTESIAN_POINT('Ctrl Pts',(6.643644474,0.810731746,-3.480228168));
#163611=CARTESIAN_POINT('Ctrl Pts',(6.452572859,0.745065281,-3.844977782));
#163612=CARTESIAN_POINT('Ctrl Pts',(6.222719017,0.680609079,-4.186617732));
#163613=CARTESIAN_POINT('Ctrl Pts',(6.66887594644061,0.810731746,-3.47324360113186));
#163614=CARTESIAN_POINT('Ctrl Pts',(6.47818779837961,0.745065281,-3.83937847426548));
#163615=CARTESIAN_POINT('Ctrl Pts',(6.24856346855714,0.680609079,-4.18243733738681));
#163616=CARTESIAN_POINT('',(6.00465671315862,0.680609081791282,-4.22188978249707));
#163617=CARTESIAN_POINT('Ctrl Pts',(5.879334183,0.680609079,-4.242160954));
#163618=CARTESIAN_POINT('Ctrl Pts',(5.649458466,0.745496505000001,-4.560752393));
#163619=CARTESIAN_POINT('Ctrl Pts',(5.386501999,0.810723991,-4.852638067));
#163620=CARTESIAN_POINT('Ctrl Pts',(5.934877406,0.680609079,-4.585545789));
#163621=CARTESIAN_POINT('Ctrl Pts',(5.68639423,0.745496505000001,-4.907147023));
#163622=CARTESIAN_POINT('Ctrl Pts',(5.404614025,0.810723991,-5.200014158));
#163623=CARTESIAN_POINT('Ctrl Pts',(5.93905073708842,0.680609079,-4.61134657134199));
#163624=CARTESIAN_POINT('Ctrl Pts',(5.68916945916119,0.745496505000001,
-4.93317395122199));
#163625=CARTESIAN_POINT('Ctrl Pts',(5.40597490175684,0.810723991,-5.22611482990271));
#163626=CARTESIAN_POINT('',(5.91963475714295,0.680609080402124,-4.49131113113577));
#163627=CARTESIAN_POINT('',(5.89960538046839,0.680609082082812,-4.36748347900849));
#163628=CARTESIAN_POINT('',(5.58799901358701,0.767980175609575,-5.02911540651578));
#163629=CARTESIAN_POINT('Ctrl Pts',(5.91963475075909,0.680609079135094,
-4.49131113423801));
#163630=CARTESIAN_POINT('Ctrl Pts',(5.86834890042719,0.695136944971322,
-4.58294237093696));
#163631=CARTESIAN_POINT('Ctrl Pts',(5.81514232318593,0.709660812691301,
-4.6734864315971));
#163632=CARTESIAN_POINT('Ctrl Pts',(5.70462161828251,0.738780776758252,
-4.85284261521551));
#163633=CARTESIAN_POINT('Ctrl Pts',(5.64729563502227,0.753373671679497,
-4.94162137712873));
#163634=CARTESIAN_POINT('Ctrl Pts',(5.5881178864952,0.767949007801361,-5.02916452012994));
#163635=CARTESIAN_POINT('Ctrl Pts',(5.38963703028742,0.809946052468512,
-4.84915587539728));
#163636=CARTESIAN_POINT('Ctrl Pts',(5.42109309803381,0.802922931155035,
-4.87764173345527));
#163637=CARTESIAN_POINT('Ctrl Pts',(5.45257728230892,0.796078752405789,
-4.9061815214961));
#163638=CARTESIAN_POINT('Ctrl Pts',(5.51864524857705,0.782074139963076,
-4.96612528710073));
#163639=CARTESIAN_POINT('Ctrl Pts',(5.55327454877581,0.774939590215754,
-4.99757597712486));
#163640=CARTESIAN_POINT('Ctrl Pts',(5.58788582318887,0.76799718521808,-5.029038814209));
#163641=CARTESIAN_POINT('Origin',(-3.43475248243408E-13,0.560925700000089,
3.95950633391706E-13));
#163642=CARTESIAN_POINT('',(5.08192802476734,0.680609080255333,-5.42106621224534));
#163643=CARTESIAN_POINT('',(5.43134411396266,0.562053379559575,-4.89557205454599));
#163644=CARTESIAN_POINT('Ctrl Pts',(5.08192802331054,0.680609080058393,
-5.42106621122977));
#163645=CARTESIAN_POINT('Ctrl Pts',(5.1100945693517,0.671661524800105,-5.38239740756182));
#163646=CARTESIAN_POINT('Ctrl Pts',(5.14091683688863,0.661738573453892,
-5.33929157974953));
#163647=CARTESIAN_POINT('Ctrl Pts',(5.20372932683127,0.641119488223043,
-5.24904764102523));
#163648=CARTESIAN_POINT('Ctrl Pts',(5.23322324759152,0.631275792608505,
-5.20569484202607));
#163649=CARTESIAN_POINT('Ctrl Pts',(5.32050712680759,0.601654471599338,
-5.07441688130195));
#163650=CARTESIAN_POINT('Ctrl Pts',(5.37687516309367,0.58185813495123,-4.98558258638997));
#163651=CARTESIAN_POINT('Ctrl Pts',(5.43134411450069,0.562053380097903,
-4.89557205475313));
#163652=CARTESIAN_POINT('Ctrl Pts',(5.58811220398515,0.767963166001071,
-5.02919199882256));
#163653=CARTESIAN_POINT('Ctrl Pts',(5.50630931642712,0.753333602510161,
-5.09821684315267));
#163654=CARTESIAN_POINT('Ctrl Pts',(5.42305909815561,0.738713518179266,
-5.16551099681846));
#163655=CARTESIAN_POINT('Ctrl Pts',(5.25426137545546,0.709588701049038,
-5.29616033816167));
#163656=CARTESIAN_POINT('Ctrl Pts',(5.16874805351855,0.695086898663409,
-5.35952220462778));
#163657=CARTESIAN_POINT('Ctrl Pts',(5.08192802658712,0.680609078972075,
-5.42106620666916));
#163658=CARTESIAN_POINT('Ctrl Pts',(5.43134411385099,0.562053379328016,
-4.89557205432403));
#163659=CARTESIAN_POINT('Ctrl Pts',(5.51574033120653,0.582224590136018,
-4.83206733521017));
#163660=CARTESIAN_POINT('Ctrl Pts',(5.59867868192533,0.602198953374283,
-4.7665928602493));
#163661=CARTESIAN_POINT('Ctrl Pts',(5.72065160839433,0.631811121718146,
-4.66561419936138));
#163662=CARTESIAN_POINT('Ctrl Pts',(5.76082559180801,0.641604433083129,
-4.63156388649604));
#163663=CARTESIAN_POINT('Ctrl Pts',(5.84378956186459,0.661914308017457,
-4.55957825087984));
#163664=CARTESIAN_POINT('Ctrl Pts',(5.88326695168444,0.67162085454678,-4.52437410847237));
#163665=CARTESIAN_POINT('Ctrl Pts',(5.9196347555966,0.680609080023521,-4.49131112933193));
#163666=CARTESIAN_POINT('Ctrl Pts',(5.392821385,0.810731746,-4.845614255));
#163667=CARTESIAN_POINT('Ctrl Pts',(5.126787292,0.745065281,-5.141691134));
#163668=CARTESIAN_POINT('Ctrl Pts',(4.829939409,0.680609079,-5.406864646));
#163669=CARTESIAN_POINT('Ctrl Pts',(5.74017357700001,0.810731746,-4.827049544));
#163670=CARTESIAN_POINT('Ctrl Pts',(5.475158725,0.745065281,-5.142196766));
#163671=CARTESIAN_POINT('Ctrl Pts',(5.177236248,0.680609079,-5.426437582));
#163672=CARTESIAN_POINT('Ctrl Pts',(5.76631662721193,0.810731746,-4.82565229307423));
#163673=CARTESIAN_POINT('Ctrl Pts',(5.50137848717533,0.745065281,-5.14223482179199));
#163674=CARTESIAN_POINT('Ctrl Pts',(5.20337513213411,0.680609079,-5.42791071578303));
#163675=CARTESIAN_POINT('',(4.95668967087975,0.680609081791281,-5.41400804255423));
#163676=CARTESIAN_POINT('Ctrl Pts',(4.829939409,0.680609079,-5.40686464600001));
#163677=CARTESIAN_POINT('Ctrl Pts',(4.536950317,0.745496505000001,-5.66859111));
#163678=CARTESIAN_POINT('Ctrl Pts',(4.217394834,0.810723991,-5.89712479200001));
#163679=CARTESIAN_POINT('Ctrl Pts',(4.810366473,0.680609079,-5.754161485));
#163680=CARTESIAN_POINT('Ctrl Pts',(4.498557937,0.745496505000001,-6.014827323));
#163681=CARTESIAN_POINT('Ctrl Pts',(4.16040782,0.810723991,-6.240272973));
#163682=CARTESIAN_POINT('Ctrl Pts',(4.80889582836633,0.680609079,-5.78025620234674));
#163683=CARTESIAN_POINT('Ctrl Pts',(4.49567326258934,0.745496505000001,
-6.04084234847347));
#163684=CARTESIAN_POINT('Ctrl Pts',(4.15612600728023,0.810723991,-6.26605597412672));
#163685=CARTESIAN_POINT('',(4.81573785460079,0.680609080426409,-5.65885326274786));
#163686=CARTESIAN_POINT('',(4.82279603853048,0.680609082082812,-5.53361490783603));
#163687=CARTESIAN_POINT('',(4.37624354905032,0.76798017563068,-6.11279209097898));
#163688=CARTESIAN_POINT('Ctrl Pts',(4.81573784785622,0.680609079124368,
-5.65885326435406));
#163689=CARTESIAN_POINT('Ctrl Pts',(4.7459530260031,0.69513694474491,-5.73731727061858));
#163690=CARTESIAN_POINT('Ctrl Pts',(4.67452609357664,0.709660812247418,
-5.81430661899299));
#163691=CARTESIAN_POINT('Ctrl Pts',(4.52803302162047,0.738780776727708,
-5.96571087218322));
#163692=CARTESIAN_POINT('Ctrl Pts',(4.45296247846833,0.753373671660118,
-6.04009064412939));
#163693=CARTESIAN_POINT('Ctrl Pts',(4.37634908483691,0.767949007797225,
-6.11286561045525));
#163694=CARTESIAN_POINT('Ctrl Pts',(4.22120513800344,0.80994605254875,-5.89439795062712));
#163695=CARTESIAN_POINT('Ctrl Pts',(4.24580216291263,0.802922931255788,
-5.92897994973941));
#163696=CARTESIAN_POINT('Ctrl Pts',(4.27041505395194,0.796078752431283,
-5.96362066270131));
#163697=CARTESIAN_POINT('Ctrl Pts',(4.3220522501715,0.782074139997033,-6.03636563608711));
#163698=CARTESIAN_POINT('Ctrl Pts',(4.34911096790233,0.774939590239716,
-6.07452530240738));
#163699=CARTESIAN_POINT('Ctrl Pts',(4.37614947000743,0.767997185231775,
-6.11269295679182));
#163700=CARTESIAN_POINT('Origin',(5.86119694445664E-13,0.5609257,-8.27463098040937E-13));
#163701=CARTESIAN_POINT('',(3.7977463825975,0.68060908017408,-6.38678900099291));
#163702=CARTESIAN_POINT('',(4.25195902659592,0.562053379571023,-5.94869473597743));
#163703=CARTESIAN_POINT('Ctrl Pts',(3.79774638114675,0.680609079925947,
-6.3867889994241));
#163704=CARTESIAN_POINT('Ctrl Pts',(3.8335670582867,0.671661524756492,-6.35507922606506));
#163705=CARTESIAN_POINT('Ctrl Pts',(3.87293519691386,0.66173857344991,-6.3196070651455));
#163706=CARTESIAN_POINT('Ctrl Pts',(3.95367894493431,0.641119488224729,
-6.24497580820599));
#163707=CARTESIAN_POINT('Ctrl Pts',(3.99180288446093,0.631275792626585,
-6.2089768947307));
#163708=CARTESIAN_POINT('Ctrl Pts',(4.10526699590558,0.601654471696003,
-6.0995315939306));
#163709=CARTESIAN_POINT('Ctrl Pts',(4.17941392619882,0.581858135115378,
-6.02489165720565));
#163710=CARTESIAN_POINT('Ctrl Pts',(4.25195902726286,0.562053380317572,
-5.94869473641836));
#163711=CARTESIAN_POINT('Ctrl Pts',(4.3763376280932,0.767963166029586,-6.11289122516614));
#163712=CARTESIAN_POINT('Ctrl Pts',(4.28160894554066,0.753333602562223,
-6.16271710418354));
#163713=CARTESIAN_POINT('Ctrl Pts',(4.18583881739736,0.738713518245378,
-6.21054162179682));
#163714=CARTESIAN_POINT('Ctrl Pts',(3.99290174802687,0.709588701510303,
-6.30184993204269));
#163715=CARTESIAN_POINT('Ctrl Pts',(3.89576675037785,0.695086898897569,
-6.34534759749871));
#163716=CARTESIAN_POINT('Ctrl Pts',(3.79774638490242,0.680609078983362,
-6.38678899609424));
#163717=CARTESIAN_POINT('Ctrl Pts',(4.2519590265095,0.562053379244821,-5.94869473563823));
#163718=CARTESIAN_POINT('Ctrl Pts',(4.34803374463893,0.582224590082613,
-5.90481741360385));
#163719=CARTESIAN_POINT('Ctrl Pts',(4.44310811953507,0.602198953317149,
-5.85870298923816));
#163720=CARTESIAN_POINT('Ctrl Pts',(4.58393681431553,0.631811121707079,
-5.78630572681304));
#163721=CARTESIAN_POINT('Ctrl Pts',(4.63049136343402,0.641604433135485,
-5.76168771002945));
#163722=CARTESIAN_POINT('Ctrl Pts',(4.72699058372725,0.661914332869367,
-5.70921979554073));
#163723=CARTESIAN_POINT('Ctrl Pts',(4.77311282974381,0.671620871273028,
-5.68332519320183));
#163724=CARTESIAN_POINT('Ctrl Pts',(4.8157378535464,0.680609080098608,-5.65885326079093));
#163725=CARTESIAN_POINT('Ctrl Pts',(4.225076389,0.810731746,-5.891623674));
#163726=CARTESIAN_POINT('Ctrl Pts',(3.901614248,0.745065281,-6.123588974));
#163727=CARTESIAN_POINT('Ctrl Pts',(3.554702037,0.680609079,-6.318749356));
#163728=CARTESIAN_POINT('Ctrl Pts',(4.568298544,0.810731746,-5.948163449));
#163729=CARTESIAN_POINT('Ctrl Pts',(4.241732254,0.745065281,-6.198972345));
#163730=CARTESIAN_POINT('Ctrl Pts',(3.889671666,0.680609079,-6.412523242));
#163731=CARTESIAN_POINT('Ctrl Pts',(4.59413075144553,0.810731746,-5.95241884794627));
#163732=CARTESIAN_POINT('Ctrl Pts',(4.26733083136151,0.745065281,-6.20464598479641));
#163733=CARTESIAN_POINT('Ctrl Pts',(3.91488275688742,0.680609079,-6.41958102204373));
#163734=CARTESIAN_POINT('',(3.67695332919104,0.680609081791273,-6.35297330357109));
#163735=CARTESIAN_POINT('Ctrl Pts',(3.554702037,0.680609079,-6.318749356));
#163736=CARTESIAN_POINT('Ctrl Pts',(3.212299413,0.745496505000001,-6.511372807));
#163737=CARTESIAN_POINT('Ctrl Pts',(2.851086974,0.810723991,-6.665868515));
#163738=CARTESIAN_POINT('Ctrl Pts',(3.460928151,0.680609079,-6.653718985));
#163739=CARTESIAN_POINT('Ctrl Pts',(3.100374075,0.745496505000001,-6.841260983));
#163740=CARTESIAN_POINT('Ctrl Pts',(2.721665569,0.810723991,-6.988743559));
#163741=CARTESIAN_POINT('Ctrl Pts',(3.45388229633626,0.680609079,-6.67888747724637));
#163742=CARTESIAN_POINT('Ctrl Pts',(3.09196438123154,0.745496505000001,
-6.86604767194434));
#163743=CARTESIAN_POINT('Ctrl Pts',(2.71194127955328,0.810723991,-7.01300330477373));
#163744=CARTESIAN_POINT('',(3.48666240302753,0.680609080421826,-6.5617937045755));
#163745=CARTESIAN_POINT('',(3.52082035429993,0.680609082082812,-6.43977814068483));
#163746=CARTESIAN_POINT('',(2.95985979999369,0.767980175639301,-6.91064141109326));
#163747=CARTESIAN_POINT('Ctrl Pts',(3.48666239612088,0.680609079139956,
-6.56179370465681));
#163748=CARTESIAN_POINT('Ctrl Pts',(3.40164166089227,0.695136945044024,
-6.62342159344771));
#163749=CARTESIAN_POINT('Ctrl Pts',(3.3153342144121,0.709660812849234,-6.68325629570886));
#163750=CARTESIAN_POINT('Ctrl Pts',(3.13971863331975,0.73878077678132,-6.79962911927942));
#163751=CARTESIAN_POINT('Ctrl Pts',(3.05041374545117,0.753373671704107,
-6.85613198576015));
#163752=CARTESIAN_POINT('Ctrl Pts',(2.959947063858,0.767949007827794,-6.91073589883575));
#163753=CARTESIAN_POINT('Ctrl Pts',(2.85539438562627,0.809946052527927,
-6.66402452831394));
#163754=CARTESIAN_POINT('Ctrl Pts',(2.87198223802458,0.802922931249818,
-6.70308565289529));
#163755=CARTESIAN_POINT('Ctrl Pts',(2.88857296395146,0.796078752434789,
-6.74220752935955));
#163756=CARTESIAN_POINT('Ctrl Pts',(2.92336489219696,0.782074140012189,
-6.82435223668418));
#163757=CARTESIAN_POINT('Ctrl Pts',(2.94158779189988,0.774939590256684,
-6.86743657576036));
#163758=CARTESIAN_POINT('Ctrl Pts',(2.95978923143777,0.767997185246865,
-6.91052437038489));
#163759=CARTESIAN_POINT('Origin',(-1.68051336735253E-13,0.560925699999978,
5.18682319317065E-13));
#163760=CARTESIAN_POINT('',(2.3359863380162,0.680609080244164,-7.05387263538529));
#163761=CARTESIAN_POINT('',(2.87375705924332,0.562053379750906,-6.72366306359679));
#163762=CARTESIAN_POINT('Ctrl Pts',(2.33598633705615,0.680609080018014,
-7.05387263374758));
#163763=CARTESIAN_POINT('Ctrl Pts',(2.37778621086744,0.671661524820673,
-7.03060460389659));
#163764=CARTESIAN_POINT('Ctrl Pts',(2.42385941050709,0.661738573500913,
-7.0044247484152));
#163765=CARTESIAN_POINT('Ctrl Pts',(2.51875892880942,0.641119488297372,
-6.94889584785191));
#163766=CARTESIAN_POINT('Ctrl Pts',(2.56373025394769,0.631275792746461,
-6.92193408914264));
#163767=CARTESIAN_POINT('Ctrl Pts',(2.69806914162172,0.601654471945102,
-6.83943898895643));
#163768=CARTESIAN_POINT('Ctrl Pts',(2.78652793768544,0.581858135446601,
-6.78248349093925));
#163769=CARTESIAN_POINT('Ctrl Pts',(2.87375705997847,0.562053380737001,
-6.72366306435497));
#163770=CARTESIAN_POINT('Ctrl Pts',(2.9599303685496,0.767963166031737,-6.91075845180163));
#163771=CARTESIAN_POINT('Ctrl Pts',(2.85670529872925,0.753333602552418,
-6.93905556288548));
#163772=CARTESIAN_POINT('Ctrl Pts',(2.75289336527756,0.738713518238556,
-6.96517422327883));
#163773=CARTESIAN_POINT('Ctrl Pts',(2.54483847479892,0.709588702262668,
-7.01287202811285));
#163774=CARTESIAN_POINT('Ctrl Pts',(2.44062372419453,0.695086899270088,
-7.03447158992617));
#163775=CARTESIAN_POINT('Ctrl Pts',(2.33598634187701,0.680609079004666,
-7.05387263108362));
#163776=CARTESIAN_POINT('Ctrl Pts',(2.87375705921098,0.562053378832269,
-6.72366306261159));
#163777=CARTESIAN_POINT('Ctrl Pts',(2.9770211335591,0.582225215204339,-6.70146410395925));
#163778=CARTESIAN_POINT('Ctrl Pts',(3.0797795908864,0.602198340253702,-6.67686751428585));
#163779=CARTESIAN_POINT('Ctrl Pts',(3.23288349207581,0.631811365792358,
-6.63643569582469));
#163780=CARTESIAN_POINT('Ctrl Pts',(3.28364302353049,0.641604918933792,
-6.62240072356809));
#163781=CARTESIAN_POINT('Ctrl Pts',(3.38916501123893,0.66191478057786,-6.59190394743353));
#163782=CARTESIAN_POINT('Ctrl Pts',(3.43977429202624,0.671621084023588,
-6.57653002766987));
#163783=CARTESIAN_POINT('Ctrl Pts',(3.4866624024038,0.680609080079151,-6.56179370238188));
#163784=CARTESIAN_POINT('Ctrl Pts',(2.859771516,0.810731746,-6.662147317));
#163785=CARTESIAN_POINT('Ctrl Pts',(2.494006057,0.745065281,-6.819154599));
#163786=CARTESIAN_POINT('Ctrl Pts',(2.113250748,0.680609079,-6.93517637));
#163787=CARTESIAN_POINT('Ctrl Pts',(3.182814947,0.810731746,-6.79114784200001));
#163788=CARTESIAN_POINT('Ctrl Pts',(2.809967097,0.745065281,-6.965890866));
#163789=CARTESIAN_POINT('Ctrl Pts',(2.420230359,0.680609079,-7.098766443));
#163790=CARTESIAN_POINT('Ctrl Pts',(3.20712842706674,0.810731746,-6.80085691326475));
#163791=CARTESIAN_POINT('Ctrl Pts',(2.83374752932183,0.745065281,-6.97693479681675));
#163792=CARTESIAN_POINT('Ctrl Pts',(2.44333481473786,0.680609079,-7.11107885550346));
#163793=CARTESIAN_POINT('',(2.22528673569468,0.680609081791282,-6.99488059468723));
#163794=CARTESIAN_POINT('Ctrl Pts',(2.113250748,0.680609079,-6.93517637));
#163795=CARTESIAN_POINT('Ctrl Pts',(1.73744496,0.745496505000001,-7.04968994800001));
#163796=CARTESIAN_POINT('Ctrl Pts',(1.351465456,0.810723991,-7.122923636));
#163797=CARTESIAN_POINT('Ctrl Pts',(1.949660675,0.680609079,-7.24215598100001));
#163798=CARTESIAN_POINT('Ctrl Pts',(1.557220167,0.745496505000001,-7.34780488300001));
#163799=CARTESIAN_POINT('Ctrl Pts',(1.155661261,0.810723991,-7.410428264));
#163800=CARTESIAN_POINT('Ctrl Pts',(1.93736906680233,0.680609079,-7.26522139709702));
#163801=CARTESIAN_POINT('Ctrl Pts',(1.54367868185706,0.745496505000001,
-7.37020423713987));
#163802=CARTESIAN_POINT('Ctrl Pts',(1.14094919195899,0.810723991,-7.43203039533711));
#163803=CARTESIAN_POINT('',(1.99455449275703,0.68060908041698,-7.15791196576213));
#163804=CARTESIAN_POINT('',(2.05354654700497,0.680609082082812,-7.04721236860769));
#163805=CARTESIAN_POINT('',(1.40507629648974,0.767980175645073,-7.38535681937711));
#163806=CARTESIAN_POINT('Ctrl Pts',(1.99455448593649,0.680609079136802,
-7.15791196436369));
#163807=CARTESIAN_POINT('Ctrl Pts',(1.89827331417205,0.695136945000173,
-7.19982208236072));
#163808=CARTESIAN_POINT('Ctrl Pts',(1.80112099588355,0.709660812754888,
-7.23970433265933));
#163809=CARTESIAN_POINT('Ctrl Pts',(1.60459449158103,0.738780776796205,
-7.31560426581368));
#163810=CARTESIAN_POINT('Ctrl Pts',(1.50523105622012,0.753373671720888,
-7.3515882156345));
#163811=CARTESIAN_POINT('Ctrl Pts',(1.40514120807807,0.76794900784462,-7.38546785721208));
#163812=CARTESIAN_POINT('Ctrl Pts',(1.35606856510727,0.809946052688147,
-7.12204872604119));
#163813=CARTESIAN_POINT('Ctrl Pts',(1.36387161560445,0.802922931425193,
-7.16376252090609));
#163814=CARTESIAN_POINT('Ctrl Pts',(1.37166441273046,0.79607875249018,-7.20553626587412));
#163815=CARTESIAN_POINT('Ctrl Pts',(1.38798424115962,0.782074140061212,
-7.29323971148109));
#163816=CARTESIAN_POINT('Ctrl Pts',(1.39651924027891,0.774939590284013,
-7.3392341474405));
#163817=CARTESIAN_POINT('Ctrl Pts',(1.40503253810627,0.767997185255711,
-7.38522734486377));
#163818=CARTESIAN_POINT('Origin',(6.91720986045752E-14,0.560925700000067,
-4.49727061146987E-13));
#163819=CARTESIAN_POINT('',(0.764998169984091,0.680609080258875,-7.39112502442283));
#163820=CARTESIAN_POINT('',(1.36118141054067,0.562053379621627,-7.18424037696642));
#163821=CARTESIAN_POINT('Ctrl Pts',(0.764998169435021,0.68060908006245,
-7.39112502271931));
#163822=CARTESIAN_POINT('Ctrl Pts',(0.810822724249504,0.671661524822522,
-7.3773867236855));
#163823=CARTESIAN_POINT('Ctrl Pts',(0.861446653293738,0.66173857347019,
-7.36172331463118));
#163824=CARTESIAN_POINT('Ctrl Pts',(0.966064546025971,0.641119488217196,
-7.32789324004562));
#163825=CARTESIAN_POINT('Ctrl Pts',(1.01578044798146,0.631275792611451,
-7.31122933773633));
#163826=CARTESIAN_POINT('Ctrl Pts',(1.16471257591828,0.601654471644855,
-7.25954181665948));
#163827=CARTESIAN_POINT('Ctrl Pts',(1.26334700347819,0.581858135037895,
-7.22293393264052));
#163828=CARTESIAN_POINT('Ctrl Pts',(1.36118141087409,0.562053380214067,
-7.18424037750623));
#163829=CARTESIAN_POINT('Ctrl Pts',(1.40512005487322,0.767963166034435,
-7.38548629389044));
#163830=CARTESIAN_POINT('Ctrl Pts',(1.29822528732601,0.753333602530371,
-7.39093149553088));
#163831=CARTESIAN_POINT('Ctrl Pts',(1.19122567919874,0.738713518197604,
-7.39412301911702));
#163832=CARTESIAN_POINT('Ctrl Pts',(0.977781373906088,0.709588701609241,
-7.39598002441255));
#163833=CARTESIAN_POINT('Ctrl Pts',(0.871359841310341,0.695086898941891,
-7.39467150955204));
#163834=CARTESIAN_POINT('Ctrl Pts',(0.764998174704899,0.680609078987347,
-7.39112502109302));
#163835=CARTESIAN_POINT('Ctrl Pts',(1.36118141059066,0.562053379366792,
-7.18424037669758));
#163836=CARTESIAN_POINT('Ctrl Pts',(1.46680007254095,0.582224590158785,
-7.18475912476055));
#163837=CARTESIAN_POINT('Ctrl Pts',(1.57245018243156,0.602198953355514,
-7.18282750052659));
#163838=CARTESIAN_POINT('Ctrl Pts',(1.73066166566679,0.631811121704626,
-7.17625395876863));
#163839=CARTESIAN_POINT('Ctrl Pts',(1.78325026707083,0.641604433121933,
-7.17345899964121));
#163840=CARTESIAN_POINT('Ctrl Pts',(1.89286125451794,0.661914325723975,
-7.1663593834956));
#163841=CARTESIAN_POINT('Ctrl Pts',(1.94559354184426,0.671620866139669,
-7.16222430769084));
#163842=CARTESIAN_POINT('Ctrl Pts',(1.99455449261922,0.680609080066209,
-7.15791196346636));
#163843=CARTESIAN_POINT('Ctrl Pts',(1.360746905,0.810731746,-7.121156357));
#163844=CARTESIAN_POINT('Ctrl Pts',(0.969780916,0.745065281,-7.195864134));
#163845=CARTESIAN_POINT('Ctrl Pts',(0.572986203,0.680609079,-7.227322244));
#163846=CARTESIAN_POINT('Ctrl Pts',(1.648506461,0.810731746,-7.31658571));
#163847=CARTESIAN_POINT('Ctrl Pts',(1.246811002,0.745065281,-7.407092072));
#163848=CARTESIAN_POINT('Ctrl Pts',(0.837621771,0.680609079,-7.453079214));
#163849=CARTESIAN_POINT('Ctrl Pts',(1.67016434216083,0.810731746,-7.3312944681085));
#163850=CARTESIAN_POINT('Ctrl Pts',(1.26766134234651,0.745065281,-7.42298989184181));
#163851=CARTESIAN_POINT('Ctrl Pts',(0.857539252672341,0.680609079,-7.47007054417667));
#163852=CARTESIAN_POINT('',(0.669568207960791,0.680609081791281,-7.30971504256078));
#163853=CARTESIAN_POINT('Ctrl Pts',(0.572986203,0.680609079,-7.227322244));
#163854=CARTESIAN_POINT('Ctrl Pts',(0.181349511,0.745496505000001,-7.25837142200001));
#163855=CARTESIAN_POINT('Ctrl Pts',(-0.211349085,0.810723991,-7.24691876300001));
#163856=CARTESIAN_POINT('Ctrl Pts',(0.347229232,0.680609079,-7.491957812));
#163857=CARTESIAN_POINT('Ctrl Pts',(-0.0587476260000001,0.745496505000001,
-7.510773593));
#163858=CARTESIAN_POINT('Ctrl Pts',(-0.464380483,0.810723991,-7.485609579));
#163859=CARTESIAN_POINT('Ctrl Pts',(0.330266612023814,0.680609079,-7.51184163907424));
#163860=CARTESIAN_POINT('Ctrl Pts',(-0.0767877178485978,0.745496505000001,
-7.52973824374311));
#163861=CARTESIAN_POINT('Ctrl Pts',(-0.483392411744903,0.810723991,-7.50354400461565));
#163862=CARTESIAN_POINT('',(0.409183430363367,0.68060908042706,-7.41933421904734));
#163863=CARTESIAN_POINT('',(0.490593424731522,0.680609082082812,-7.32390426471177));
#163864=CARTESIAN_POINT('',(-0.215407013297438,0.767980175633115,-7.51474115102437));
#163865=CARTESIAN_POINT('Ctrl Pts',(0.409183424044645,0.68060907912779,
-7.41933421624228));
#163866=CARTESIAN_POINT('Ctrl Pts',(0.306143817310809,0.695136944806357,
-7.43956689283184));
#163867=CARTESIAN_POINT('Ctrl Pts',(0.202689362634763,0.70966081237921,
-7.4576318414953));
#163868=CARTESIAN_POINT('Ctrl Pts',(-0.0055587055481005,0.738780776750879,
-7.48950988760412));
#163869=CARTESIAN_POINT('Ctrl Pts',(-0.11033456455517,0.753373671687691,
-7.50329235124383));
#163870=CARTESIAN_POINT('Ctrl Pts',(-0.215367489144336,0.767949007826713,
-7.51486354692501));
#163871=CARTESIAN_POINT('Ctrl Pts',(-0.206665514471121,0.809946052642357,
-7.24705384082526));
#163872=CARTESIAN_POINT('Ctrl Pts',(-0.208012127760169,0.802922931364602,
-7.28946981573807));
#163873=CARTESIAN_POINT('Ctrl Pts',(-0.209381642207943,0.796078752490285,
-7.33194213449867));
#163874=CARTESIAN_POINT('Ctrl Pts',(-0.212297010597966,0.782074140047893,
-7.42110340320246));
#163875=CARTESIAN_POINT('Ctrl Pts',(-0.213848999176155,0.774939590272211,
-7.46785728735778));
#163876=CARTESIAN_POINT('Ctrl Pts',(-0.215421915454735,0.76799718524202,
-7.51460529679075));
#163877=CARTESIAN_POINT('Origin',(-5.12014475956279E-14,0.560925700000022,
9.36750677027476E-14));
#163878=CARTESIAN_POINT('',(-0.84176046229091,0.680609080286941,-7.38277662196963));
#163879=CARTESIAN_POINT('',(-0.215041571561947,0.562053379558999,-7.3088905962547));
#163880=CARTESIAN_POINT('Ctrl Pts',(-0.841760462439525,0.680609080144953,
-7.38277662033779));
#163881=CARTESIAN_POINT('Ctrl Pts',(-0.794053931958486,0.671661524879478,
-7.37921043980768));
#163882=CARTESIAN_POINT('Ctrl Pts',(-0.741246392298931,0.661738573515153,
-7.37479588085074));
#163883=CARTESIAN_POINT('Ctrl Pts',(-0.631801941938972,0.641119488276378,
-7.36424648905931));
#163884=CARTESIAN_POINT('Ctrl Pts',(-0.579666123820091,0.63127579267547,
-7.35865962885286));
#163885=CARTESIAN_POINT('Ctrl Pts',(-0.423104657345012,0.60165447171773,
-7.34019653839765));
#163886=CARTESIAN_POINT('Ctrl Pts',(-0.318906635060471,0.581858135111766,
-7.32564801267825));
#163887=CARTESIAN_POINT('Ctrl Pts',(-0.215041571295957,0.562053380310879,
-7.30889059701473));
#163888=CARTESIAN_POINT('Ctrl Pts',(-0.215392111140141,0.767963166024209,
-7.514877005258));
#163889=CARTESIAN_POINT('Ctrl Pts',(-0.320958295798627,0.75333360254386,
-7.49721568589562));
#163890=CARTESIAN_POINT('Ctrl Pts',(-0.426142395756981,0.738713518225547,
-7.47733084058546));
#163891=CARTESIAN_POINT('Ctrl Pts',(-0.634995693504388,0.709588701579514,
-7.433260213766));
#163892=CARTESIAN_POINT('Ctrl Pts',(-0.73864785765739,0.695086898924898,
-7.40910480755326));
#163893=CARTESIAN_POINT('Ctrl Pts',(-0.841760457205502,0.680609078986858,
-7.38277661976896));
#163894=CARTESIAN_POINT('Ctrl Pts',(-0.215041571424503,0.562053379230467,
-7.30889059593007));
#163895=CARTESIAN_POINT('Ctrl Pts',(-0.112003730550206,0.582224590007247,
-7.33210210620165));
#163896=CARTESIAN_POINT('Ctrl Pts',(-0.00840841935307247,0.602198953227445,
-7.35292729293288));
#163897=CARTESIAN_POINT('Ctrl Pts',(0.147517284441341,0.631811121614305,
-7.3805182291761));
#163898=CARTESIAN_POINT('Ctrl Pts',(0.199477227084608,0.641604433037009,
-7.38909360944579));
#163899=CARTESIAN_POINT('Ctrl Pts',(0.308051845719433,0.661914338321119,
-7.40572311100768));
#163900=CARTESIAN_POINT('Ctrl Pts',(0.360440179027586,0.671620874009537,
-7.41302058903849));
#163901=CARTESIAN_POINT('Ctrl Pts',(0.409183430708766,0.680609080099152,
-7.41933421684758));
#163902=CARTESIAN_POINT('Ctrl Pts',(-0.201904718,0.810731746,-7.24718804));
#163903=CARTESIAN_POINT('Ctrl Pts',(-0.599790104,0.745065281,-7.23610306));
#163904=CARTESIAN_POINT('Ctrl Pts',(-0.994070541000001,0.680609079,-7.18152656200001));
#163905=CARTESIAN_POINT('Ctrl Pts',(0.037115645,0.810731746,-7.499908161));
#163906=CARTESIAN_POINT('Ctrl Pts',(-0.37464459,0.745065281,-7.501945886));
#163907=CARTESIAN_POINT('Ctrl Pts',(-0.78415308,0.680609079,-7.458894285));
#163908=CARTESIAN_POINT('Ctrl Pts',(0.0551052287059663,0.810731746,-7.51892884071888));
#163909=CARTESIAN_POINT('Ctrl Pts',(-0.357699280323076,0.745065281,-7.52195423052317));
#163910=CARTESIAN_POINT('Ctrl Pts',(-0.768353891643804,0.680609079,-7.47977003720628));
#163911=CARTESIAN_POINT('',(-0.917458585476369,0.680609081791282,-7.28275533886137));
#163912=CARTESIAN_POINT('Ctrl Pts',(-0.994070541,0.680609079,-7.181526562));
#163913=CARTESIAN_POINT('Ctrl Pts',(-1.38322564,0.745496505000001,-7.127659516));
#163914=CARTESIAN_POINT('Ctrl Pts',(-1.764281177,0.810723991,-7.03205602400001));
#163915=CARTESIAN_POINT('Ctrl Pts',(-1.271438263,0.680609079,-7.391444023));
#163916=CARTESIAN_POINT('Ctrl Pts',(-1.671968444,0.745496505000001,-7.32254687700001));
#163917=CARTESIAN_POINT('Ctrl Pts',(-2.062708312,0.810723991,-7.21077211));
#163918=CARTESIAN_POINT('Ctrl Pts',(-1.29227874146047,0.680609079,-7.40721651553411));
#163919=CARTESIAN_POINT('Ctrl Pts',(-1.69366360789286,0.745496505000001,
-7.33719005833291));
#163920=CARTESIAN_POINT('Ctrl Pts',(-2.08513112397734,0.810723991,-7.22420023607741));
#163921=CARTESIAN_POINT('',(-1.19532059374951,0.680609080406583,-7.33383665026911));
#163922=CARTESIAN_POINT('',(-1.09428701315318,0.680609082082812,-7.25737241764844));
#163923=CARTESIAN_POINT('',(-1.82581813019941,0.76798017564556,-7.29274453850138));
#163924=CARTESIAN_POINT('Ctrl Pts',(-1.19532059940679,0.680609079142472,
-7.33383664609925));
#163925=CARTESIAN_POINT('Ctrl Pts',(-1.30030062681116,0.695136945115343,
-7.33144582430566));
#163926=CARTESIAN_POINT('Ctrl Pts',(-1.40521980584584,0.709660812978692,
-7.32684877463772));
#163927=CARTESIAN_POINT('Ctrl Pts',(-1.61545198357233,0.738780776798224,
-7.31321435110408));
#163928=CARTESIAN_POINT('Ctrl Pts',(-1.7207410634257,0.753373671714424,
-7.30415087586492));
#163929=CARTESIAN_POINT('Ctrl Pts',(-1.82580584156822,0.767949007826193,
-7.29287256937691));
#163930=CARTESIAN_POINT('Ctrl Pts',(-1.75973614394106,0.809946052460278,
-7.03319477416626));
#163931=CARTESIAN_POINT('Ctrl Pts',(-1.77016945517068,0.802922931140822,
-7.07432960524266));
#163932=CARTESIAN_POINT('Ctrl Pts',(-1.78063724403593,0.796078752428626,
-7.11551453861799));
#163933=CARTESIAN_POINT('Ctrl Pts',(-1.80265149000155,0.78207413998448,
-7.20196454829124));
#163934=CARTESIAN_POINT('Ctrl Pts',(-1.81421789693137,0.774939590244176,
-7.24729172070654));
#163935=CARTESIAN_POINT('Ctrl Pts',(-1.82580347933559,0.76799718525082,
-7.29260865692637));
#163936=CARTESIAN_POINT('Origin',(-1.14166488762724E-13,0.560925699999978,
-5.13911829758129E-13));
#163937=CARTESIAN_POINT('',(-2.40915931034892,0.680609080213132,-7.02921779044765));
#163938=CARTESIAN_POINT('',(-1.78120945046844,0.562053379756257,-7.09178521403228));
#163939=CARTESIAN_POINT('Ctrl Pts',(-2.40915931011412,0.680609079936094,
-7.02921778843984));
#163940=CARTESIAN_POINT('Ctrl Pts',(-2.36180150889329,0.671661524763371,
-7.03599047701499));
#163941=CARTESIAN_POINT('Ctrl Pts',(-2.30927958083451,0.661738573470731,
-7.04303118800338));
#163942=CARTESIAN_POINT('Ctrl Pts',(-2.20012607373983,0.641119488286034,
-7.05625575679003));
#163943=CARTESIAN_POINT('Ctrl Pts',(-2.1480081524798,0.631275792729284,
-7.06200717403117));
#163944=CARTESIAN_POINT('Ctrl Pts',(-1.99113798809114,0.601654471923386,
-7.07763182771462));
#163945=CARTESIAN_POINT('Ctrl Pts',(-1.88624855517428,0.581858135430499,
-7.08582293316892));
#163946=CARTESIAN_POINT('Ctrl Pts',(-1.78120945034197,0.562053380742793,
-7.09178521508122));
#163947=CARTESIAN_POINT('Ctrl Pts',(-1.82583278106323,0.7679631660403,-7.29288042007639));
#163948=CARTESIAN_POINT('Ctrl Pts',(-1.9251342252849,0.753333602553888,
-7.25293840338144));
#163949=CARTESIAN_POINT('Ctrl Pts',(-2.02358452538462,0.738713518227169,
-7.21090698245767));
#163950=CARTESIAN_POINT('Ctrl Pts',(-2.2180810666693,0.70958870158529,-7.12296941717666));
#163951=CARTESIAN_POINT('Ctrl Pts',(-2.3141172022883,0.695086898937427,
-7.07709659967735));
#163952=CARTESIAN_POINT('Ctrl Pts',(-2.40915930432956,0.68060907898539,
-7.02921778941742));
#163953=CARTESIAN_POINT('Ctrl Pts',(-1.78120944989328,0.562053378830073,
-7.09178521322179));
#163954=CARTESIAN_POINT('Ctrl Pts',(-1.68556739894358,0.582225215193757,
-7.13660553132821));
#163955=CARTESIAN_POINT('Ctrl Pts',(-1.58887688169021,0.602198340238744,
-7.17921112563103));
#163956=CARTESIAN_POINT('Ctrl Pts',(-1.44252363383872,0.631811365737381,
-7.23967816847744));
#163957=CARTESIAN_POINT('Ctrl Pts',(-1.39362071976889,0.641604918834856,
-7.25922338390512));
#163958=CARTESIAN_POINT('Ctrl Pts',(-1.29115944627396,0.661914798004255,
-7.29880433212849));
#163959=CARTESIAN_POINT('Ctrl Pts',(-1.24156587658882,0.671621094886457,
-7.31719267986154));
#163960=CARTESIAN_POINT('Ctrl Pts',(-1.19532059288389,0.680609080033675,
-7.33383664806536));
#163961=CARTESIAN_POINT('Ctrl Pts',(-1.755115501,0.810731746,-7.034349265));
#163962=CARTESIAN_POINT('Ctrl Pts',(-2.141315605,0.745065281,-6.937989849));
#163963=CARTESIAN_POINT('Ctrl Pts',(-2.51464565,0.680609079,-6.79993068000001));
#163964=CARTESIAN_POINT('Ctrl Pts',(-1.576010657,0.810731746,-7.332543243));
#163965=CARTESIAN_POINT('Ctrl Pts',(-1.978582217,0.745065281,-7.246017048));
#163966=CARTESIAN_POINT('Ctrl Pts',(-2.369261804,0.680609079,-7.115939748));
#163967=CARTESIAN_POINT('Ctrl Pts',(-1.5625305438092,0.810731746,-7.35498645830609));
#163968=CARTESIAN_POINT('Ctrl Pts',(-1.96633428198512,0.745065281,-7.26920034899641));
#163969=CARTESIAN_POINT('Ctrl Pts',(-2.35831966164122,0.680609079,-7.13972379487905));
#163970=CARTESIAN_POINT('',(-2.46158603461972,0.680609081791281,-6.91526209026196));
#163971=CARTESIAN_POINT('Ctrl Pts',(-2.51464565,0.680609079,-6.79993068));
#163972=CARTESIAN_POINT('Ctrl Pts',(-2.883122697,0.745496505000001,-6.663666173));
#163973=CARTESIAN_POINT('Ctrl Pts',(-3.234717443,0.810723991,-6.488382161));
#163974=CARTESIAN_POINT('Ctrl Pts',(-2.830654719,0.680609079,-6.945314526));
#163975=CARTESIAN_POINT('Ctrl Pts',(-3.207009877,0.745496505000001,-6.791926008));
#163976=CARTESIAN_POINT('Ctrl Pts',(-3.564586193,0.810723991,-6.598766951));
#163977=CARTESIAN_POINT('Ctrl Pts',(-2.85439857823173,0.680609079,-6.95623817950437));
#163978=CARTESIAN_POINT('Ctrl Pts',(-3.23134567101129,0.745496505000001,
-6.80156302087739));
#163979=CARTESIAN_POINT('Ctrl Pts',(-3.58937142207502,0.810723991,-6.60706089308014));
#163980=CARTESIAN_POINT('',(-2.74393275571236,0.680609080390424,-6.90541703064292));
#163981=CARTESIAN_POINT('',(-2.62997704800503,0.680609082082812,-6.85299031890594));
#163982=CARTESIAN_POINT('',(-3.35085602073211,0.767980175593935,-6.72974729659381));
#163983=CARTESIAN_POINT('Ctrl Pts',(-2.74393276050547,0.680609079132267,
-6.90541702525689));
#163984=CARTESIAN_POINT('Ctrl Pts',(-2.84594445597044,0.695136944937039,
-6.88051449714559));
#163985=CARTESIAN_POINT('Ctrl Pts',(-2.94742245181023,0.70966081261579,
-6.85347040226978));
#163986=CARTESIAN_POINT('Ctrl Pts',(-3.14980852231464,0.738780776766089,
-6.79496103952786));
#163987=CARTESIAN_POINT('Ctrl Pts',(-3.25068762275745,0.753373671682622,
-6.76347542344459));
#163988=CARTESIAN_POINT('Ctrl Pts',(-3.35087154228855,0.767949007788142,
-6.72987497586571));
#163989=CARTESIAN_POINT('Ctrl Pts',(-3.23052346694552,0.809946052592434,
-6.49047133466123));
#163990=CARTESIAN_POINT('Ctrl Pts',(-3.24955562579035,0.802922931297973,
-6.52840160248477));
#163991=CARTESIAN_POINT('Ctrl Pts',(-3.26863222728892,0.796078752413679,
-6.56637339069007));
#163992=CARTESIAN_POINT('Ctrl Pts',(-3.30871598903657,0.782074139977129,
-6.64606983483956));
#163993=CARTESIAN_POINT('Ctrl Pts',(-3.32975598209915,0.774939590214679,
-6.68785084763502));
#163994=CARTESIAN_POINT('Ctrl Pts',(-3.35081250185054,0.767997185203043,
-6.72961774137811));
#163995=CARTESIAN_POINT('Origin',(5.85469173142172E-13,0.560925700000111,
1.36782946080771E-12));
#163996=CARTESIAN_POINT('',(-3.86390854712789,0.680609080271912,-6.34698054711008));
#163997=CARTESIAN_POINT('',(-3.26408995016512,0.562053379612811,-6.54307583813135));
#163998=CARTESIAN_POINT('Ctrl Pts',(-3.86390854656277,0.680609080104214,
-6.34698054551348));
#163999=CARTESIAN_POINT('Ctrl Pts',(-3.81911387217345,0.671661524886997,
-6.36377541977018));
#164000=CARTESIAN_POINT('Ctrl Pts',(-3.76933342214294,0.66173857352756,
-6.38194218488432));
#164001=CARTESIAN_POINT('Ctrl Pts',(-3.66557475447777,0.641119488245391,
-6.41832234811752));
#164002=CARTESIAN_POINT('Ctrl Pts',(-3.61591170567734,0.631275792618738,
-6.4351431129641));
#164003=CARTESIAN_POINT('Ctrl Pts',(-3.46606791648177,0.601654471617293,
-6.48412491938828));
#164004=CARTESIAN_POINT('Ctrl Pts',(-3.36539158528181,0.581858135000715,
-6.51467264899996));
#164005=CARTESIAN_POINT('Ctrl Pts',(-3.26408995022167,0.56205338015989,
-6.54307583871452));
#164006=CARTESIAN_POINT('Ctrl Pts',(-3.35089953961369,0.767963165984828,
-6.7298768518095));
#164007=CARTESIAN_POINT('Ctrl Pts',(-3.43929301839793,0.753333602505536,
-6.66952178206919));
#164008=CARTESIAN_POINT('Ctrl Pts',(-3.52640609218595,0.738713518184776,
-6.60730912803424));
#164009=CARTESIAN_POINT('Ctrl Pts',(-3.69745143796608,0.709588701116743,
-6.47961648509564));
#164010=CARTESIAN_POINT('Ctrl Pts',(-3.78138100101789,0.695086898699007,
-6.41417121913299));
#164011=CARTESIAN_POINT('Ctrl Pts',(-3.86390854139516,0.680609078973892,
-6.34698054733611));
#164012=CARTESIAN_POINT('Ctrl Pts',(-3.26408994997813,0.562053379377489,
-6.54307583796165));
#164013=CARTESIAN_POINT('Ctrl Pts',(-3.18032159845886,0.582224590134105,
-6.60740650056184));
#164014=CARTESIAN_POINT('Ctrl Pts',(-3.09504530934754,0.602198953333155,
-6.66980547027568));
#164015=CARTESIAN_POINT('Ctrl Pts',(-2.96511610677917,0.631811121670721,
-6.76031782940335));
#164016=CARTESIAN_POINT('Ctrl Pts',(-2.92155924884402,0.641604433060527,
-6.78991804730418));
#164017=CARTESIAN_POINT('Ctrl Pts',(-2.83000234288128,0.661914293374162,
-6.85059973890839));
#164018=CARTESIAN_POINT('Ctrl Pts',(-2.78552004907774,0.671620845873208,
-6.87922008882333));
#164019=CARTESIAN_POINT('Ctrl Pts',(-2.74393275435454,0.680609079990549,
-6.90541702862458));
#164020=CARTESIAN_POINT('Ctrl Pts',(-3.226259034,0.810731746,-6.492592136));
#164021=CARTESIAN_POINT('Ctrl Pts',(-3.582715568,0.745065281,-6.315463943));
#164022=CARTESIAN_POINT('Ctrl Pts',(-3.917638724,0.680609079,-6.100377597));
#164023=CARTESIAN_POINT('Ctrl Pts',(-3.115444452,0.810731746,-6.822316752));
#164024=CARTESIAN_POINT('Ctrl Pts',(-3.490003539,0.745065281,-6.651272505));
#164025=CARTESIAN_POINT('Ctrl Pts',(-3.84358648,0.680609079,-6.440251778));
#164026=CARTESIAN_POINT('Ctrl Pts',(-3.10710412403857,0.810731746,-6.84713308379284));
#164027=CARTESIAN_POINT('Ctrl Pts',(-3.48302567819979,0.745065281,-6.67654673776603));
#164028=CARTESIAN_POINT('Ctrl Pts',(-3.83801302576597,0.680609079,-6.46583200475358));
#164029=CARTESIAN_POINT('',(-3.89061245650934,0.680609081791279,-6.22441887193084));
#164030=CARTESIAN_POINT('Ctrl Pts',(-3.917638724,0.680609079,-6.100377597));
#164031=CARTESIAN_POINT('Ctrl Pts',(-4.248208141,0.745496505000001,-5.888087205));
#164032=CARTESIAN_POINT('Ctrl Pts',(-4.553901916,0.810723991,-5.64131875900001));
#164033=CARTESIAN_POINT('Ctrl Pts',(-4.257512905,0.680609079,-6.174429841));
#164034=CARTESIAN_POINT('Ctrl Pts',(-4.592095092,0.745496505000001,-5.94372222700001));
#164035=CARTESIAN_POINT('Ctrl Pts',(-4.899787985,0.810723991,-5.67821078400001));
#164036=CARTESIAN_POINT('Ctrl Pts',(-4.28304990857418,0.680609079,-6.17999387770952));
#164037=CARTESIAN_POINT('Ctrl Pts',(-4.61793360162425,0.745496505000001,
-5.94790245555247));
#164038=CARTESIAN_POINT('Ctrl Pts',(-4.92577670163132,0.810723991,-5.68098272675691));
#164039=CARTESIAN_POINT('',(-4.16424167156072,0.68060908040942,-6.15410778545866));
#164040=CARTESIAN_POINT('',(-4.04043957907103,0.680609082082812,-6.12713362678962));
#164041=CARTESIAN_POINT('',(-4.71921160804611,0.767980175629172,-5.85207455067974));
#164042=CARTESIAN_POINT('Ctrl Pts',(-4.16424167499564,0.680609079127669,
-6.15410777928402));
#164043=CARTESIAN_POINT('Ctrl Pts',(-4.25851508568839,0.695136944827101,
-6.10785795963635));
#164044=CARTESIAN_POINT('Ctrl Pts',(-4.35180690085521,0.709660812410746,
-6.05963137155408));
#164045=CARTESIAN_POINT('Ctrl Pts',(-4.53688351532785,0.738780776763756,
-5.95898290182754));
#164046=CARTESIAN_POINT('Ctrl Pts',(-4.62863564177466,0.753373671697259,
-5.90654737729357));
#164047=CARTESIAN_POINT('Ctrl Pts',(-4.7192542139961,0.767949007827546,
-5.85219590820191));
#164048=CARTESIAN_POINT('Ctrl Pts',(-4.55025510319298,0.809946052614754,
-5.64426066970121));
#164049=CARTESIAN_POINT('Ctrl Pts',(-4.57699618717919,0.802922931345544,
-5.67721279729065));
#164050=CARTESIAN_POINT('Ctrl Pts',(-4.6037896005029,0.796078752452168,
-5.71019592084041));
#164051=CARTESIAN_POINT('Ctrl Pts',(-4.66006860596506,0.782074140026348,
-5.77941228251503));
#164052=CARTESIAN_POINT('Ctrl Pts',(-4.68959837845096,0.774939590259562,
-5.81569350193402));
#164053=CARTESIAN_POINT('Ctrl Pts',(-4.71914125606377,0.767997185239498,
-5.85195737967383));
#164054=CARTESIAN_POINT('Origin',(-2.12503625807159E-14,0.560925699999978,
6.54858112181245E-14));
#164055=CARTESIAN_POINT('',(-4.594345237046,0.562053379770818,-5.68841950555253));
#164056=CARTESIAN_POINT('Ctrl Pts',(-4.5943452360446,0.562053378678052,
-5.68841950498304));
#164057=CARTESIAN_POINT('Ctrl Pts',(-4.52636453261428,0.582224589590113,
-5.76925387232301));
#164058=CARTESIAN_POINT('Ctrl Pts',(-4.45649588941519,0.602198952910481,
-5.84852587065802));
#164059=CARTESIAN_POINT('Ctrl Pts',(-4.34906095411072,0.631811365757422,
-5.96485399947606));
#164060=CARTESIAN_POINT('Ctrl Pts',(-4.31288469410678,0.641604918902546,
-6.0031265574176));
#164061=CARTESIAN_POINT('Ctrl Pts',(-4.23651301061102,0.661914787148201,
-6.0820715827627));
#164062=CARTESIAN_POINT('Ctrl Pts',(-4.19922415999308,0.67162108824664,
-6.11958420968522));
#164063=CARTESIAN_POINT('Ctrl Pts',(-4.16424166988398,0.680609080047746,
-6.1541077838538));
#164064=CARTESIAN_POINT('',(-5.13798571439363,0.680609080190355,-5.36796554832296));
#164065=CARTESIAN_POINT('Ctrl Pts',(-5.13798571330918,0.680609079974861,
-5.36796554657682));
#164066=CARTESIAN_POINT('Ctrl Pts',(-5.09784871543656,0.671661524847478,
-5.39399729660559));
#164067=CARTESIAN_POINT('Ctrl Pts',(-5.053137422544,0.661738573571544,-5.42244065785812));
#164068=CARTESIAN_POINT('Ctrl Pts',(-4.95962523510226,0.641119488400852,
-5.48027531923473));
#164069=CARTESIAN_POINT('Ctrl Pts',(-4.91473924827774,0.631275792831726,
-5.50737891125491));
#164070=CARTESIAN_POINT('Ctrl Pts',(-4.77892836490913,0.601654472016654,
-5.58742753516421));
#164071=CARTESIAN_POINT('Ctrl Pts',(-4.6871726497635,0.581858135529807,
-5.63890351086657));
#164072=CARTESIAN_POINT('Ctrl Pts',(-4.59434523742545,0.562053380890475,
-5.68841950671169));
#164073=CARTESIAN_POINT('Ctrl Pts',(-4.71928196002846,0.767963166018845,
-5.85219172168565));
#164074=CARTESIAN_POINT('Ctrl Pts',(-4.79263429243288,0.753333602530235,
-5.7742457349207));
#164075=CARTESIAN_POINT('Ctrl Pts',(-4.8643368292945,0.738713518208989,
-5.69476084238225));
#164076=CARTESIAN_POINT('Ctrl Pts',(-5.00393308407793,0.709588701590787,
-5.53328389173144));
#164077=CARTESIAN_POINT('Ctrl Pts',(-5.07183162414147,0.695086898935622,
-5.45132632333071));
#164078=CARTESIAN_POINT('Ctrl Pts',(-5.13798570921413,0.680609078986734,
-5.36796554912861));
#164079=CARTESIAN_POINT('Ctrl Pts',(-4.54654628,0.810731746,-5.647248615));
#164080=CARTESIAN_POINT('Ctrl Pts',(-4.85659173300001,0.745065281,-5.397633963));
#164081=CARTESIAN_POINT('Ctrl Pts',(-5.137447365,0.680609079,-5.11557763800001));
#164082=CARTESIAN_POINT('Ctrl Pts',(-4.509203528,0.810731746,-5.993086312));
#164083=CARTESIAN_POINT('Ctrl Pts',(-4.838236174,0.745065281,-5.745521853));
#164084=CARTESIAN_POINT('Ctrl Pts',(-5.138189324,0.680609079,-5.46342479300001));
#164085=CARTESIAN_POINT('Ctrl Pts',(-4.50639297011688,0.810731746,-6.01911537556728));
#164086=CARTESIAN_POINT('Ctrl Pts',(-4.8368546646499,0.745065281,-5.77170522190873));
#164087=CARTESIAN_POINT('Ctrl Pts',(-5.13824516666302,0.680609079,-5.48960509603734));
#164088=CARTESIAN_POINT('',(-5.13771816422049,0.680609081791273,-5.24252874552383));
#164089=CARTESIAN_POINT('Ctrl Pts',(-5.137447365,0.680609079,-5.115577638));
#164090=CARTESIAN_POINT('Ctrl Pts',(-5.41465209400001,0.745496505000001,
-4.837187824));
#164091=CARTESIAN_POINT('Ctrl Pts',(-5.66015099700001,0.810723991,-4.530473562));
#164092=CARTESIAN_POINT('Ctrl Pts',(-5.48529452,0.680609079,-5.114835679));
#164093=CARTESIAN_POINT('Ctrl Pts',(-5.762459044,0.745496505000001,-4.81759660100001));
#164094=CARTESIAN_POINT('Ctrl Pts',(-6.005881136,0.810723991,-4.492147791));
#164095=CARTESIAN_POINT('Ctrl Pts',(-5.51143058654251,0.680609079,-5.11477993069355));
#164096=CARTESIAN_POINT('Ctrl Pts',(-5.78859208967389,0.745496505000001,
-4.81612458232567));
#164097=CARTESIAN_POINT('Ctrl Pts',(-6.03185813707295,0.810723991,-4.48926812133259));
#164098=CARTESIAN_POINT('',(-5.38983527524761,0.680609080402338,-5.11503929999281));
#164099=CARTESIAN_POINT('',(-5.26439847106798,0.680609082082805,-5.11530686482352));
#164100=CARTESIAN_POINT('',(-5.86690210549644,0.767980175626098,-4.70076530286576));
#164101=CARTESIAN_POINT('Ctrl Pts',(-5.38983527725203,0.680609079140822,
-5.11503929321169));
#164102=CARTESIAN_POINT('Ctrl Pts',(-5.47196228524896,0.695136945077434,
-5.04960477097213));
#164103=CARTESIAN_POINT('Ctrl Pts',(-5.55270570005654,0.709660812908944,
-4.98245070991648));
#164104=CARTESIAN_POINT('Ctrl Pts',(-5.71181887766143,0.73878077677887,
-4.84436934646061));
#164105=CARTESIAN_POINT('Ctrl Pts',(-5.79015380252541,0.753373671697209,
-4.77343574038703));
#164106=CARTESIAN_POINT('Ctrl Pts',(-5.86696980358536,0.767949007805755,
-4.7008746641221));
#164107=CARTESIAN_POINT('Ctrl Pts',(-5.65722186833464,0.809946052775441,
-4.53413064874382));
#164108=CARTESIAN_POINT('Ctrl Pts',(-5.69042149382425,0.802922931489543,
-4.5605638312732));
#164109=CARTESIAN_POINT('Ctrl Pts',(-5.72367888890452,0.796078752502292,
-4.58701603616805));
#164110=CARTESIAN_POINT('Ctrl Pts',(-5.79352159409118,0.782074140054355,
-4.64251583519036));
#164111=CARTESIAN_POINT('Ctrl Pts',(-5.83016036667187,0.77493959026445,
-4.67160079174287));
#164112=CARTESIAN_POINT('Ctrl Pts',(-5.86680821002045,0.76799718523115,
-4.7006659948091));
#164113=CARTESIAN_POINT('Origin',(1.16920362280837E-12,0.560925700000067,
9.99200722162641E-13));
#164114=CARTESIAN_POINT('',(-6.171816381008,0.680609080257676,-4.13795044509658));
#164115=CARTESIAN_POINT('',(-5.7097740415247,0.56205337966577,-4.56777900317126));
#164116=CARTESIAN_POINT('Ctrl Pts',(-6.17181637974723,0.680609080059578,
-4.13795044380038));
#164117=CARTESIAN_POINT('Ctrl Pts',(-6.13821381882902,0.671661524822212,
-4.17200185466163));
#164118=CARTESIAN_POINT('Ctrl Pts',(-6.10066233257506,0.66173857345913,
-4.20939183272496));
#164119=CARTESIAN_POINT('Ctrl Pts',(-6.02176915015887,0.641119488189323,
-4.28597670856538));
#164120=CARTESIAN_POINT('Ctrl Pts',(-5.98375904373633,0.631275792604873,
-4.32209579415727));
#164121=CARTESIAN_POINT('Ctrl Pts',(-5.86833143070661,0.601654471690628,
-4.42946825164726));
#164122=CARTESIAN_POINT('Ctrl Pts',(-5.78978672597655,0.581858135122761,
-4.49946551441468));
#164123=CARTESIAN_POINT('Ctrl Pts',(-5.70977404189956,0.562053380358149,
-4.56777900381104));
#164124=CARTESIAN_POINT('Ctrl Pts',(-5.86699600097242,0.767963166021046,
-4.70086461092242));
#164125=CARTESIAN_POINT('Ctrl Pts',(-5.92187731353065,0.753333602539643,
-4.60897237482362));
#164126=CARTESIAN_POINT('Ctrl Pts',(-5.97481658259202,0.738713518220881,
-4.51593186898607));
#164127=CARTESIAN_POINT('Ctrl Pts',(-6.07643638237694,0.709588701895203,
-4.32822109318138));
#164128=CARTESIAN_POINT('Ctrl Pts',(-6.12512903837064,0.69508689908163,
-4.23358346708829));
#164129=CARTESIAN_POINT('Ctrl Pts',(-6.17181637588744,0.680609078995239,
-4.13795044764606));
#164130=CARTESIAN_POINT('Ctrl Pts',(-5.70977404121975,0.562053379367947,
-4.56777900307571));
#164131=CARTESIAN_POINT('Ctrl Pts',(-5.66075968858094,0.582224590114487,
-4.66133734899429));
#164132=CARTESIAN_POINT('Ctrl Pts',(-5.6095656720655,0.602198953299526,
-4.75377570448088));
#164133=CARTESIAN_POINT('Ctrl Pts',(-5.52965027461911,0.631811121650233,
-4.89047835301904));
#164134=CARTESIAN_POINT('Ctrl Pts',(-5.50254794981892,0.641604433065763,
-4.93563183327623));
#164135=CARTESIAN_POINT('Ctrl Pts',(-5.44493274063811,0.661914290831286,
-5.02914878027505));
#164136=CARTESIAN_POINT('Ctrl Pts',(-5.4165790761668,0.671620843889875,
-5.07380153903629));
#164137=CARTESIAN_POINT('Ctrl Pts',(-5.38983527320803,0.680609080021972,
-5.11503929875299));
#164138=CARTESIAN_POINT('Ctrl Pts',(-5.654242076,0.810731746,-4.537846025));
#164139=CARTESIAN_POINT('Ctrl Pts',(-5.903379066,0.745065281,-4.227416618));
#164140=CARTESIAN_POINT('Ctrl Pts',(-6.117034678,0.680609079,-3.891578954));
#164141=CARTESIAN_POINT('Ctrl Pts',(-5.69211725800001,0.810731746,-4.883625817));
#164142=CARTESIAN_POINT('Ctrl Pts',(-5.960238263,0.745065281,-4.571116985));
#164143=CARTESIAN_POINT('Ctrl Pts',(-6.19253614600001,0.680609079,-4.231134137));
#164144=CARTESIAN_POINT('Ctrl Pts',(-5.69496788857757,0.810731746,-4.90965052225889));
#164145=CARTESIAN_POINT('Ctrl Pts',(-5.96451770291355,0.745065281,-4.59698518480662));
#164146=CARTESIAN_POINT('Ctrl Pts',(-6.19821867429337,0.680609079,-4.25669035445733));
#164147=CARTESIAN_POINT('',(-6.14458988136026,0.680609081791273,-4.01550380117678));
#164148=CARTESIAN_POINT('Ctrl Pts',(-6.117034678,0.680609079,-3.891578954));
#164149=CARTESIAN_POINT('Ctrl Pts',(-6.327912933,0.745496505000001,-3.560106917));
#164150=CARTESIAN_POINT('Ctrl Pts',(-6.501737708,0.810723991,-3.207788456));
#164151=CARTESIAN_POINT('Ctrl Pts',(-6.45658986,0.680609079,-3.816077485));
#164152=CARTESIAN_POINT('Ctrl Pts',(-6.66337681600001,0.745496505000001,
-3.466205512));
#164153=CARTESIAN_POINT('Ctrl Pts',(-6.831145961,0.810723991,-3.096036961));
#164154=CARTESIAN_POINT('Ctrl Pts',(-6.48210289523078,0.680609079,-3.81040455835748));
#164155=CARTESIAN_POINT('Ctrl Pts',(-6.68858244477358,0.745496505000001,
-3.4591500760032));
#164156=CARTESIAN_POINT('Ctrl Pts',(-6.85589659008656,0.810723991,-3.08764032922948));
#164157=CARTESIAN_POINT('',(-6.36340617191394,0.680609080415348,-3.83679726143964));
#164158=CARTESIAN_POINT('',(-6.24095952935366,0.680609082082805,-3.86402377588782));
#164159=CARTESIAN_POINT('',(-6.74026278091922,0.767980175615045,-3.32965349430743));
#164160=CARTESIAN_POINT('Ctrl Pts',(-6.36340617240637,0.680609079133212,
-3.83679725446595));
#164161=CARTESIAN_POINT('Ctrl Pts',(-6.42954660781029,0.695136944914254,
-3.75523767683706));
#164162=CARTESIAN_POINT('Ctrl Pts',(-6.49396614771468,0.709660812589365,
-3.67229619395753));
#164163=CARTESIAN_POINT('Ctrl Pts',(-6.61967593729421,0.738780776744085,
-3.50323846473616));
#164164=CARTESIAN_POINT('Ctrl Pts',(-6.68093080659687,0.753373671673061,
-3.4171235537493));
#164165=CARTESIAN_POINT('Ctrl Pts',(-6.74035240571884,0.767949007805381,
-3.3297457456512));
#164166=CARTESIAN_POINT('Ctrl Pts',(-6.4996632263326,0.809946052740608,
-3.2119897183158));
#164167=CARTESIAN_POINT('Ctrl Pts',(-6.53776901585845,0.802922931466638,
-3.23066796985503));
#164168=CARTESIAN_POINT('Ctrl Pts',(-6.57593531355083,0.796078752499066,
-3.24935238013516));
#164169=CARTESIAN_POINT('Ctrl Pts',(-6.65607595132773,0.782074140053557,
-3.28854050775976));
#164170=CARTESIAN_POINT('Ctrl Pts',(-6.69811053569426,0.774939590261598,
-3.30906922110622));
#164171=CARTESIAN_POINT('Ctrl Pts',(-6.74014973236584,0.767997185222975,
-3.32957669279489));
#164172=CARTESIAN_POINT('Origin',(-9.28077059647592E-14,0.560925699999911,
-3.27429056090622E-14));
#164173=CARTESIAN_POINT('',(-6.91705977240974,0.68060908019651,-2.71444937956975));
#164174=CARTESIAN_POINT('',(-6.5582201603214,0.562053379605623,-3.23355422947506));
#164175=CARTESIAN_POINT('Ctrl Pts',(-6.91705977069972,0.68060907998662,
-2.71444937844625));
#164176=CARTESIAN_POINT('Ctrl Pts',(-6.89156286604869,0.671661524826028,
-2.75492824303347));
#164177=CARTESIAN_POINT('Ctrl Pts',(-6.86292705281543,0.661738573476922,
-2.79951652352871));
#164178=CARTESIAN_POINT('Ctrl Pts',(-6.80234183353219,0.641119488147585,
-2.89127058978293));
#164179=CARTESIAN_POINT('Ctrl Pts',(-6.77298491792337,0.631275792530207,
-2.93471628064139));
#164180=CARTESIAN_POINT('Ctrl Pts',(-6.68333784270071,0.601654471575429,
-3.06439195463014));
#164181=CARTESIAN_POINT('Ctrl Pts',(-6.62167681188939,0.581858135004092,
-3.1496375100711));
#164182=CARTESIAN_POINT('Ctrl Pts',(-6.55822016075729,0.562053380204891,
-3.23355422994611));
#164183=CARTESIAN_POINT('Ctrl Pts',(-6.7403758294726,0.767963166007114,
-3.32973029581996));
#164184=CARTESIAN_POINT('Ctrl Pts',(-6.77421993302505,0.75333360253631,
-3.2281885891875));
#164185=CARTESIAN_POINT('Ctrl Pts',(-6.80592055292293,0.738713518224552,
-3.12594294066681));
#164186=CARTESIAN_POINT('Ctrl Pts',(-6.86481227006701,0.709588701971743,
-2.92077548577845));
#164187=CARTESIAN_POINT('Ctrl Pts',(-6.89202222679128,0.695086899117976,
-2.81788295276974));
#164188=CARTESIAN_POINT('Ctrl Pts',(-6.91705976808422,0.680609078997742,
-2.71444938240418));
#164189=CARTESIAN_POINT('Ctrl Pts',(-6.55822016004584,0.562053379347851,
-3.23355422945103));
#164190=CARTESIAN_POINT('Ctrl Pts',(-6.53046401461873,0.582224590123798,
-3.33546187009727));
#164191=CARTESIAN_POINT('Ctrl Pts',(-6.50033839978795,0.602198953325635,
-3.43674426839289));
#164192=CARTESIAN_POINT('Ctrl Pts',(-6.45167840855641,0.631811121666125,
-3.58743033294494));
#164193=CARTESIAN_POINT('Ctrl Pts',(-6.43491638461924,0.641604433068652,
-3.63735434851988));
#164194=CARTESIAN_POINT('Ctrl Pts',(-6.39875152628777,0.661914313305449,
-3.74107060286569));
#164195=CARTESIAN_POINT('Ctrl Pts',(-6.38065978734003,0.671620858343132,
-3.79077456868463));
#164196=CARTESIAN_POINT('Ctrl Pts',(-6.36340616973765,0.680609080062905,
-3.83679726069259));
#164197=CARTESIAN_POINT('Ctrl Pts',(-6.49755179600001,0.810731746,-3.216258799));
#164198=CARTESIAN_POINT('Ctrl Pts',(-6.674130955,0.745065281,-2.85952997));
#164199=CARTESIAN_POINT('Ctrl Pts',(-6.810596247,0.680609079,-2.485614363));
#164200=CARTESIAN_POINT('Ctrl Pts',(-6.608873911,0.810731746,-3.545812407));
#164201=CARTESIAN_POINT('Ctrl Pts',(-6.803546235,0.745065281,-3.182971767));
#164202=CARTESIAN_POINT('Ctrl Pts',(-6.95732686000001,0.680609079,-2.80100035));
#164203=CARTESIAN_POINT('Ctrl Pts',(-6.61725243779714,0.810731746,-3.57061586798096));
#164204=CARTESIAN_POINT('Ctrl Pts',(-6.81328652237631,0.745065281,-3.20731522978346));
#164205=CARTESIAN_POINT('Ctrl Pts',(-6.96837036535365,0.680609079,-2.8247375018096));
#164206=CARTESIAN_POINT('',(-6.86414740406235,0.680609081791274,-2.60071836199947));
#164207=CARTESIAN_POINT('Ctrl Pts',(-6.810596247,0.680609079,-2.485614363));
#164208=CARTESIAN_POINT('Ctrl Pts',(-6.945287596,0.745496505000001,-2.116559367));
#164209=CARTESIAN_POINT('Ctrl Pts',(-7.03931039,0.810723991,-1.735110727));
#164210=CARTESIAN_POINT('Ctrl Pts',(-7.125982234,0.680609079,-2.33888375));
#164211=CARTESIAN_POINT('Ctrl Pts',(-7.25272249400001,0.745496505000001,
-1.952738506));
#164212=CARTESIAN_POINT('Ctrl Pts',(-7.33699399300001,0.810723991,-1.555158883));
#164213=CARTESIAN_POINT('Ctrl Pts',(-7.14967927697468,0.680609079,-2.32785890493623));
#164214=CARTESIAN_POINT('Ctrl Pts',(-7.27582211887275,0.745496505000001,
-1.94042955714596));
#164215=CARTESIAN_POINT('Ctrl Pts',(-7.35936093834291,0.810723991,-1.54163790630347));
#164216=CARTESIAN_POINT('',(-7.03943126796915,0.680609080398537,-2.37915084812029));
#164217=CARTESIAN_POINT('',(-6.92454921546236,0.680609082082805,-2.43259874169282));
#164218=CARTESIAN_POINT('',(-7.29845626022657,0.767980175663714,-1.80285078869209));
#164219=CARTESIAN_POINT('Ctrl Pts',(-7.03943126697314,0.680609079127621,
-2.37915084103021));
#164220=CARTESIAN_POINT('Ctrl Pts',(-7.08649247720474,0.695136944835417,
-2.28527984298937));
#164221=CARTESIAN_POINT('Ctrl Pts',(-7.13157595674395,0.709660812421988,
-2.19042918962929));
#164222=CARTESIAN_POINT('Ctrl Pts',(-7.21800430741299,0.73878077676706,
-1.99830004607331));
#164223=CARTESIAN_POINT('Ctrl Pts',(-7.25931491163413,0.7533736717087,-1.9010304675125));
#164224=CARTESIAN_POINT('Ctrl Pts',(-7.29856362095871,0.767949007853029,
-1.80292161657032));
#164225=CARTESIAN_POINT('Ctrl Pts',(-7.03818755585394,0.80994605260326,
-1.73965971901071));
#164226=CARTESIAN_POINT('Ctrl Pts',(-7.0794177252991,0.802922931357737,
-1.74970966491208));
#164227=CARTESIAN_POINT('Ctrl Pts',(-7.1207083119314,0.796078752449335,
-1.7597526181006));
#164228=CARTESIAN_POINT('Ctrl Pts',(-7.20739959525797,0.782074140048543,
-1.78079668077467));
#164229=CARTESIAN_POINT('Ctrl Pts',(-7.2528645008597,0.774939590288263,
-1.791809251067));
#164230=CARTESIAN_POINT('Ctrl Pts',(-7.29832934463069,0.767997185271285,
-1.80280008485094));
#164231=CARTESIAN_POINT('Origin',(-1.32272665043232E-13,0.560925699999955,
-3.29597460435593E-14));
#164232=CARTESIAN_POINT('',(-7.33886913689214,0.680609080243553,-1.16402367627227));
#164233=CARTESIAN_POINT('',(-7.10001119469846,0.562053379812254,-1.74813204992909));
#164234=CARTESIAN_POINT('Ctrl Pts',(-7.33886913513934,0.680609080018306,
-1.16402367559671));
#164235=CARTESIAN_POINT('Ctrl Pts',(-7.32267009318878,0.671661524821512,
-1.20903724808586));
#164236=CARTESIAN_POINT('Ctrl Pts',(-7.30428893170297,0.661738573525927,
-1.25873893268598));
#164237=CARTESIAN_POINT('Ctrl Pts',(-7.26484457355725,0.641119488408449,
-1.36137187037028));
#164238=CARTESIAN_POINT('Ctrl Pts',(-7.24551354579363,0.631275792887089,
-1.41011269380347));
#164239=CARTESIAN_POINT('Ctrl Pts',(-7.1858388065163,0.601654472133851,
-1.55602809298206));
#164240=CARTESIAN_POINT('Ctrl Pts',(-7.14394465112516,0.581858135634878,
-1.65253595324458));
#164241=CARTESIAN_POINT('Ctrl Pts',(-7.10001119570797,0.562053380932133,
-1.74813205062504));
#164242=CARTESIAN_POINT('Ctrl Pts',(-7.29858317582244,0.767963166056144,
-1.80290149253324));
#164243=CARTESIAN_POINT('Ctrl Pts',(-7.30980755765121,0.753333602557733,
-1.6964582926769));
#164244=CARTESIAN_POINT('Ctrl Pts',(-7.3187872425921,0.738713518228104,
-1.58978839432786));
#164245=CARTESIAN_POINT('Ctrl Pts',(-7.33219716607111,0.709588701809224,
-1.37675766104373));
#164246=CARTESIAN_POINT('Ctrl Pts',(-7.33665211594474,0.695086899044866,
-1.270421362579));
#164247=CARTESIAN_POINT('Ctrl Pts',(-7.33886913326281,0.680609078992077,
-1.16402368087677));
#164248=CARTESIAN_POINT('Ctrl Pts',(-7.10001119357155,0.562053378727583,
-1.74813205008095));
#164249=CARTESIAN_POINT('Ctrl Pts',(-7.09481110174453,0.582224589605302,
-1.85362389826389));
#164250=CARTESIAN_POINT('Ctrl Pts',(-7.08716252876118,0.602198952927782,
-1.95901448777532));
#164251=CARTESIAN_POINT('Ctrl Pts',(-7.07203310580689,0.631811365744268,
-2.11663935704751));
#164252=CARTESIAN_POINT('Ctrl Pts',(-7.06639500129622,0.64160491886239,
-2.16900081468051));
#164253=CARTESIAN_POINT('Ctrl Pts',(-7.05337152457618,0.661914791451309,
-2.27806659903441));
#164254=CARTESIAN_POINT('Ctrl Pts',(-7.04638780387179,0.671621091156144,
-2.33049638581521));
#164255=CARTESIAN_POINT('Ctrl Pts',(-7.03943126560501,0.680609080016027,
-2.37915084785294));
#164256=CARTESIAN_POINT('Ctrl Pts',(-7.037043215,0.810731746,-1.744282886));
#164257=CARTESIAN_POINT('Ctrl Pts',(-7.13280789900001,0.745065281,-1.357934879));
#164258=CARTESIAN_POINT('Ctrl Pts',(-7.18570190500001,0.680609079,-0.963425207));
#164259=CARTESIAN_POINT('Ctrl Pts',(-7.21660696600001,0.810731746,-2.042200749));
#164260=CARTESIAN_POINT('Ctrl Pts',(-7.328727947,0.745065281,-1.645994327));
#164261=CARTESIAN_POINT('Ctrl Pts',(-7.396800703,0.680609079,-1.239894901));
#164262=CARTESIAN_POINT('Ctrl Pts',(-7.2301216182923,0.810731746,-2.06462318285809));
#164263=CARTESIAN_POINT('Ctrl Pts',(-7.34347363654515,0.745065281,-1.66767477897067));
#164264=CARTESIAN_POINT('Ctrl Pts',(-7.41268880312268,0.680609079,-1.26070306391127));
#164265=CARTESIAN_POINT('',(-7.26274502348097,0.680609081791273,-1.06432622257033));
#164266=CARTESIAN_POINT('Ctrl Pts',(-7.185701905,0.680609079,-0.963425207));
#164267=CARTESIAN_POINT('Ctrl Pts',(-7.237908331,0.745496505000001,-0.574043853));
#164268=CARTESIAN_POINT('Ctrl Pts',(-7.247732742,0.810723991,-0.181301149));
#164269=CARTESIAN_POINT('Ctrl Pts',(-7.462171599,0.680609079,-0.75232641));
#164270=CARTESIAN_POINT('Ctrl Pts',(-7.502938928,0.745496505,-0.347963618));
#164271=CARTESIAN_POINT('Ctrl Pts',(-7.49977234,0.810723991,0.058436696));
#164272=CARTESIAN_POINT('Ctrl Pts',(-7.48294460305386,0.680609079,-0.736465155544213));
#164273=CARTESIAN_POINT('Ctrl Pts',(-7.522852436733,0.745496505,-0.330976708620506));
#164274=CARTESIAN_POINT('Ctrl Pts',(-7.51870974870921,0.810723991,0.0764497923144575));
#164275=CARTESIAN_POINT('',(-7.28559392484547,0.680609082082805,-0.887152541785874));
#164276=CARTESIAN_POINT('Ctrl Pts',(-7.24761405796479,0.809946052533277,
-0.185985164613406));
#164277=CARTESIAN_POINT('Ctrl Pts',(-7.29004073015667,0.802922931301267,
-0.186936880615135));
#164278=CARTESIAN_POINT('Ctrl Pts',(-7.33252490372907,0.796078752413943,
-0.187868779482898));
#164279=CARTESIAN_POINT('Ctrl Pts',(-7.42171324432903,0.782074140020066,
-0.189784780224056));
#164280=CARTESIAN_POINT('Ctrl Pts',(-7.46848258277582,0.774939590255079,
-0.190766271942571));
#164281=CARTESIAN_POINT('Ctrl Pts',(-7.51524718812475,0.767997185234041,
-0.191726548669481));
#164282=CARTESIAN_POINT('Ctrl Pts',(-7.247490315,0.810731746,-0.190746244));
#164283=CARTESIAN_POINT('Ctrl Pts',(-7.257962673,0.745065281,0.207155738));
#164284=CARTESIAN_POINT('Ctrl Pts',(-7.224812129,0.680609079,0.603812641));
#164285=CARTESIAN_POINT('Ctrl Pts',(-7.48689949900001,0.810731746,-0.443098054));
#164286=CARTESIAN_POINT('Ctrl Pts',(-7.511226485,0.745065281,-0.032052021));
#164287=CARTESIAN_POINT('Ctrl Pts',(-7.49040836500001,0.680609079,0.379186656));
#164288=CARTESIAN_POINT('Ctrl Pts',(-7.50491834708005,0.810731746,-0.462091013464394));
#164289=CARTESIAN_POINT('Ctrl Pts',(-7.53028808521247,0.745065281,-0.0500557090664949));
#164290=CARTESIAN_POINT('Ctrl Pts',(-7.51039815046754,0.680609079,0.362280447846572));
#164291=CARTESIAN_POINT('',(-7.32174475728359,0.680609081791271,0.521832628067191));
#164292=CARTESIAN_POINT('Ctrl Pts',(-7.224812129,0.680609079,0.603812641));
#164293=CARTESIAN_POINT('Ctrl Pts',(-7.192092516,0.745496505000001,0.995313314));
#164294=CARTESIAN_POINT('Ctrl Pts',(-7.117259166,0.810723991,1.380985869));
#164295=CARTESIAN_POINT('Ctrl Pts',(-7.449438113,0.680609079,0.869408877));
#164296=CARTESIAN_POINT('Ctrl Pts',(-7.402326278,0.745496505000001,1.273081663));
#164297=CARTESIAN_POINT('Ctrl Pts',(-7.311869668,0.810723991,1.66929984));
#164298=CARTESIAN_POINT('Ctrl Pts',(-7.46631575460598,0.680609079,0.889364885665074));
#164299=CARTESIAN_POINT('Ctrl Pts',(-7.41812253640843,0.745496505000001,
1.2939522433328));
#164300=CARTESIAN_POINT('Ctrl Pts',(-7.32649204715234,0.810723991,1.69096278293244));
#164301=CARTESIAN_POINT('',(-7.38779429941529,0.680609080381726,0.79652164116979));
#164302=CARTESIAN_POINT('',(-7.30679216084005,0.680609082082804,0.700745251313463));
#164303=CARTESIAN_POINT('',(-7.3808969011864,0.767980175586769,1.42831918057935));
#164304=CARTESIAN_POINT('Ctrl Pts',(-7.38779429547985,0.680609079134893,
0.796521647287301));
#164305=CARTESIAN_POINT('Ctrl Pts',(-7.39109048409698,0.695136944972495,
0.901477148014278));
#164306=CARTESIAN_POINT('Ctrl Pts',(-7.39218038627761,0.709660812691676,
1.00649133226492));
#164307=CARTESIAN_POINT('Ctrl Pts',(-7.38994769944287,0.738780776730923,
1.21715334075509));
#164308=CARTESIAN_POINT('Ctrl Pts',(-7.38659775244984,0.753373671654153,
1.32277869175213));
#164309=CARTESIAN_POINT('Ctrl Pts',(-7.38102407900311,0.767949007775986,
1.42829997853959));
#164310=CARTESIAN_POINT('Ctrl Pts',(-7.11815018181283,0.809946052543578,
1.37638584987182));
#164311=CARTESIAN_POINT('Ctrl Pts',(-7.15978953283649,0.80292293127717,
1.38457686486786));
#164312=CARTESIAN_POINT('Ctrl Pts',(-7.20148078055054,0.79607875240361,
1.39279959469045));
#164313=CARTESIAN_POINT('Ctrl Pts',(-7.2889958308382,0.78207413997985,1.41010124571203));
#164314=CARTESIAN_POINT('Ctrl Pts',(-7.33488271979528,0.774939590214053,
1.4191967259174));
#164315=CARTESIAN_POINT('Ctrl Pts',(-7.38076042572,0.767997185194551,1.42831190766354));
#164316=CARTESIAN_POINT('Origin',(-3.9118014383277E-13,0.560925700000022,
4.52112305926455E-14));
#164317=CARTESIAN_POINT('',(-7.1493380926488,0.680609080220652,2.02507189136407));
#164318=CARTESIAN_POINT('',(-7.17781723606865,0.562053379630161,1.39465563927328));
#164319=CARTESIAN_POINT('Ctrl Pts',(-7.14933809065069,0.680609079955072,
2.02507189123788));
#164320=CARTESIAN_POINT('Ctrl Pts',(-7.15353694685268,0.671661524738824,
1.97741687808363));
#164321=CARTESIAN_POINT('Ctrl Pts',(-7.15772385219997,0.661738573386025,
1.92459080120668));
#164322=CARTESIAN_POINT('Ctrl Pts',(-7.1650195743026,0.641119488092974,
1.81488141282109));
#164323=CARTESIAN_POINT('Ctrl Pts',(-7.1679409492184,0.631275792509169,
1.76252855139152));
#164324=CARTESIAN_POINT('Ctrl Pts',(-7.17504990849782,0.601654471589547,
1.60504254835791));
#164325=CARTESIAN_POINT('Ctrl Pts',(-7.17755040153564,0.581858135011411,
1.49986348694586));
#164326=CARTESIAN_POINT('Ctrl Pts',(-7.1778172367069,0.562053380235276,
1.39465563916099));
#164327=CARTESIAN_POINT('Ctrl Pts',(-7.3810333766528,0.767963165978988,
1.42832645349517));
#164328=CARTESIAN_POINT('Ctrl Pts',(-7.34652601019056,0.753333602506669,
1.52964468079876));
#164329=CARTESIAN_POINT('Ctrl Pts',(-7.30988622378075,0.738713518198376,
1.630226130322));
#164330=CARTESIAN_POINT('Ctrl Pts',(-7.23260745793012,0.7095887019381,1.82919826716056));
#164331=CARTESIAN_POINT('Ctrl Pts',(-7.19200120797997,0.695086899113309,
1.92757706315618));
#164332=CARTESIAN_POINT('Ctrl Pts',(-7.14933809126938,0.680609078995803,
2.02507188553382));
#164333=CARTESIAN_POINT('Ctrl Pts',(-7.17781723583245,0.562053379369874,
1.39465563912421));
#164334=CARTESIAN_POINT('Ctrl Pts',(-7.21739263744442,0.582224590179618,
1.29673036939688));
#164335=CARTESIAN_POINT('Ctrl Pts',(-7.25470334031654,0.602198953386825,
1.1978689089469));
#164336=CARTESIAN_POINT('Ctrl Pts',(-7.30715677953051,0.631811121695678,
1.04846100592241));
#164337=CARTESIAN_POINT('Ctrl Pts',(-7.32402537537675,0.641604433053326,
0.998572898853101));
#164338=CARTESIAN_POINT('Ctrl Pts',(-7.35800117062359,0.661914304541736,
0.894119113304538));
#164339=CARTESIAN_POINT('Ctrl Pts',(-7.37367802588683,0.671620852112805,
0.843601466303717));
#164340=CARTESIAN_POINT('Ctrl Pts',(-7.38779429705825,0.680609079964133,
0.796521640383342));
#164341=CARTESIAN_POINT('Ctrl Pts',(-7.119052823,0.810731746,1.371709481));
#164342=CARTESIAN_POINT('Ctrl Pts',(-7.043743179,0.745065281,1.762559983));
#164343=CARTESIAN_POINT('Ctrl Pts',(-6.926098167,0.680609079,2.14281688));
#164344=CARTESIAN_POINT('Ctrl Pts',(-7.407112933,0.810731746,1.176723413));
#164345=CARTESIAN_POINT('Ctrl Pts',(-7.342508421,0.745065281,1.583389001));
#164346=CARTESIAN_POINT('Ctrl Pts',(-7.233772858,0.680609079,1.980537866));
#164347=CARTESIAN_POINT('Ctrl Pts',(-7.42879343523788,0.810731746,1.16204801804986));
#164348=CARTESIAN_POINT('Ctrl Pts',(-7.36499463229034,0.745065281,1.56990390972439));
#164349=CARTESIAN_POINT('Ctrl Pts',(-7.25692962839339,0.680609079,1.96832412864432));
#164350=CARTESIAN_POINT('',(-7.03838784414309,0.680609081791273,2.08359116440669));
#164351=CARTESIAN_POINT('Ctrl Pts',(-6.926098167,0.680609079,2.14281688));
#164352=CARTESIAN_POINT('Ctrl Pts',(-6.809982448,0.745496505000001,2.518130736));
#164353=CARTESIAN_POINT('Ctrl Pts',(-6.653990461,0.810723991,2.878699522));
#164354=CARTESIAN_POINT('Ctrl Pts',(-7.08837718100001,0.680609079,2.450491571));
#164355=CARTESIAN_POINT('Ctrl Pts',(-6.955589078,0.745496505000001,2.834599059));
#164356=CARTESIAN_POINT('Ctrl Pts',(-6.78207209700001,0.810723991,3.202108379));
#164357=CARTESIAN_POINT('Ctrl Pts',(-7.10057028074634,0.680609079,2.47360921328975));
#164358=CARTESIAN_POINT('Ctrl Pts',(-6.9665294708429,0.745496505000001,
2.85837742524577));
#164359=CARTESIAN_POINT('Ctrl Pts',(-6.79169572068939,0.810723991,3.22640823364571));
#164360=CARTESIAN_POINT('',(-7.04384316618178,0.680609080443654,2.36605680054315));
#164361=CARTESIAN_POINT('',(-6.98532390492157,0.680609082082805,2.25510654365759));
#164362=CARTESIAN_POINT('',(-6.90128923026718,0.76798017566292,2.98160052805709));
#164363=CARTESIAN_POINT('Ctrl Pts',(-7.04384316132244,0.680609079132359,
2.36605680523004));
#164364=CARTESIAN_POINT('Ctrl Pts',(-7.02449995680018,0.695136944893178,
2.4692670872381));
#164365=CARTESIAN_POINT('Ctrl Pts',(-7.00298943239152,0.709660812558863,
2.57206039456985));
#164366=CARTESIAN_POINT('Ctrl Pts',(-6.95552283949714,0.73878077680655,
2.77731728216213));
#164367=CARTESIAN_POINT('Ctrl Pts',(-6.9295448841773,0.753373671737292,
2.87975303164855));
#164368=CARTESIAN_POINT('Ctrl Pts',(-6.90141756260734,0.767949007858333,
2.98160911443684));
#164369=CARTESIAN_POINT('Ctrl Pts',(-6.65584951416331,0.809946052493932,
2.87439859193774));
#164370=CARTESIAN_POINT('Ctrl Pts',(-6.69475453452101,0.802922931174187,
2.89134933527514));
#164371=CARTESIAN_POINT('Ctrl Pts',(-6.73370341957374,0.796078752424214,
2.90834220783244));
#164372=CARTESIAN_POINT('Ctrl Pts',(-6.81545307337181,0.782074139996443,
2.9440525048495));
#164373=CARTESIAN_POINT('Ctrl Pts',(-6.85831189299476,0.774939590258443,
2.96279966249814));
#164374=CARTESIAN_POINT('Ctrl Pts',(-6.90115750899145,0.767997185272505,
2.98156408697476));
#164375=CARTESIAN_POINT('Origin',(1.39471767468535E-12,0.5609257,-6.60929644347164E-13));
#164376=CARTESIAN_POINT('',(-6.54685994543919,0.680609080168776,3.51462319239164));
#164377=CARTESIAN_POINT('',(-6.71019412140591,0.562053379647482,2.90506789591289));
#164378=CARTESIAN_POINT('Ctrl Pts',(-6.54685994337891,0.680609079914941,
3.51462319179381));
#164379=CARTESIAN_POINT('Ctrl Pts',(-6.56120505181549,0.671661524687892,
3.46898495629405));
#164380=CARTESIAN_POINT('Ctrl Pts',(-6.5766501145436,0.661738573380289,
3.41829398489273));
#164381=CARTESIAN_POINT('Ctrl Pts',(-6.60735954205801,0.641119488174177,
3.31271790618056));
#164382=CARTESIAN_POINT('Ctrl Pts',(-6.62146693454012,0.631275792558321,
3.26221703469908));
#164383=CARTESIAN_POINT('Ctrl Pts',(-6.66226452575419,0.601654471559685,
3.10994118271523));
#164384=CARTESIAN_POINT('Ctrl Pts',(-6.68731694782609,0.581858134941924,
3.0077586812105));
#164385=CARTESIAN_POINT('Ctrl Pts',(-6.71019412196659,0.562053380171493,
2.90506789593674));
#164386=CARTESIAN_POINT('Ctrl Pts',(-6.90142095154291,0.767963166053335,
2.98163696913943));
#164387=CARTESIAN_POINT('Ctrl Pts',(-6.84593992415734,0.753333602551252,
3.07316836886803));
#164388=CARTESIAN_POINT('Ctrl Pts',(-6.78853471705588,0.738713518208592,
3.16352180901211));
#164389=CARTESIAN_POINT('Ctrl Pts',(-6.67028955484223,0.709588701147707,
3.34122944213753));
#164390=CARTESIAN_POINT('Ctrl Pts',(-6.60948412490161,0.695086898711526,
3.42857905058261));
#164391=CARTESIAN_POINT('Ctrl Pts',(-6.54685994492008,0.680609078974318,
3.51462318693433));
#164392=CARTESIAN_POINT('Ctrl Pts',(-6.7101941212339,0.562053379422081,
2.90506789574284));
#164393=CARTESIAN_POINT('Ctrl Pts',(-6.76989531021481,0.582224590210383,
2.81793960600833));
#164394=CARTESIAN_POINT('Ctrl Pts',(-6.82758600118962,0.602198953412185,
2.72941016993194));
#164395=CARTESIAN_POINT('Ctrl Pts',(-6.91093139096509,0.631811121780453,
2.59477127936949));
#164396=CARTESIAN_POINT('Ctrl Pts',(-6.93813007693746,0.641604433206543,
2.54967577767941));
#164397=CARTESIAN_POINT('Ctrl Pts',(-6.99376615698564,0.661914357167096,
2.45496761047726));
#164398=CARTESIAN_POINT('Ctrl Pts',(-7.01993624758915,0.671620886225413,
2.4090011686433));
#164399=CARTESIAN_POINT('Ctrl Pts',(-7.04384316433259,0.680609080145789,
2.36605679945138));
#164400=CARTESIAN_POINT('Ctrl Pts',(-6.657736333,0.810731746,2.870025595));
#164401=CARTESIAN_POINT('Ctrl Pts',(-6.500166082,0.745065281,3.235548881));
#164402=CARTESIAN_POINT('Ctrl Pts',(-6.303527553,0.680609079,3.581625384));
#164403=CARTESIAN_POINT('Ctrl Pts',(-6.980977999,0.810731746,2.741522602));
#164404=CARTESIAN_POINT('Ctrl Pts',(-6.830462824,0.745065281,3.124792514));
#164405=CARTESIAN_POINT('Ctrl Pts',(-6.638894171,0.680609079,3.489281327));
#164406=CARTESIAN_POINT('Ctrl Pts',(-7.00530639894729,0.810731746,2.73185097690657));
#164407=CARTESIAN_POINT('Ctrl Pts',(-6.85532221586027,0.745065281,3.11645656762765));
#164408=CARTESIAN_POINT('Ctrl Pts',(-6.66413514105389,0.680609079,3.4823311612641));
#164409=CARTESIAN_POINT('',(-6.42592373772969,0.680609081791273,3.54792329397902));
#164410=CARTESIAN_POINT('Ctrl Pts',(-6.303527553,0.680609079,3.581625384));
#164411=CARTESIAN_POINT('Ctrl Pts',(-6.10944517000001,0.745496505000001,
3.923203163));
#164412=CARTESIAN_POINT('Ctrl Pts',(-5.87958855800001,0.810723991,4.241808386));
#164413=CARTESIAN_POINT('Ctrl Pts',(-6.39587161000001,0.680609079,3.916992003));
#164414=CARTESIAN_POINT('Ctrl Pts',(-6.18361626300001,0.745496505000001,
4.263573754));
#164415=CARTESIAN_POINT('Ctrl Pts',(-5.935152372,0.810723991,4.585189889));
#164416=CARTESIAN_POINT('Ctrl Pts',(-6.40281003213691,0.680609079,3.94219032381072));
#164417=CARTESIAN_POINT('Ctrl Pts',(-6.18918922968903,0.745496505000001,
4.28914805645182));
#164418=CARTESIAN_POINT('Ctrl Pts',(-5.93932725027147,0.810723991,4.61099042126185));
#164419=CARTESIAN_POINT('',(-6.37052975546877,0.680609080438259,3.8249577733505));
#164420=CARTESIAN_POINT('',(-6.33722966772581,0.68060908208268,3.70402156086006));
#164421=CARTESIAN_POINT('',(-6.09898494522745,0.767980175587502,4.39546554820092));
#164422=CARTESIAN_POINT('Ctrl Pts',(-6.37052974967258,0.680609079127803,
3.82495777693731));
#164423=CARTESIAN_POINT('Ctrl Pts',(-6.3294516189924,0.695136944801263,
3.92159684217388));
#164424=CARTESIAN_POINT('Ctrl Pts',(-6.28634647644809,0.709660812370041,
4.01736277163909));
#164425=CARTESIAN_POINT('Ctrl Pts',(-6.19586546215903,0.73878077674373,
4.20761695386509));
#164426=CARTESIAN_POINT('Ctrl Pts',(-6.14847419881717,0.753373671664429,
4.30207331998296));
#164427=CARTESIAN_POINT('Ctrl Pts',(-6.09910843141784,0.76794900777477,
4.39550152147733));
#164428=CARTESIAN_POINT('Ctrl Pts',(-5.8823287202579,0.80994605250801,4.23800765046644));
#164429=CARTESIAN_POINT('Ctrl Pts',(-5.91668025409125,0.802922931192687,
4.26292552407541));
#164430=CARTESIAN_POINT('Ctrl Pts',(-5.95106557075331,0.796078752403965,
4.2878939716896));
#164431=CARTESIAN_POINT('Ctrl Pts',(-6.02322730488898,0.782074139955645,
4.34034314065554));
#164432=CARTESIAN_POINT('Ctrl Pts',(-6.06105402446624,0.774939590200093,
4.36786537940377));
#164433=CARTESIAN_POINT('Ctrl Pts',(-6.09886413726223,0.767997185194965,
4.39540164292246));
#164434=CARTESIAN_POINT('Origin',(-1.0542781925249E-12,0.560925699999866,
7.22295487309843E-13));
#164435=CARTESIAN_POINT('',(-5.63825790320071,0.680609080157228,4.83983461982158));
#164436=CARTESIAN_POINT('',(-5.92880978678887,0.562053379604336,4.27964240775555));
#164437=CARTESIAN_POINT('Ctrl Pts',(-5.6382579012457,0.680609079874176,
4.83983461876012));
#164438=CARTESIAN_POINT('Ctrl Pts',(-5.66207850044105,0.671661524698012,
4.7983471543782));
#164439=CARTESIAN_POINT('Ctrl Pts',(-5.68805952660668,0.661738573402297,
4.75216154169928));
#164440=CARTESIAN_POINT('Ctrl Pts',(-5.74074672097875,0.641119488182738,
4.65565539206355));
#164441=CARTESIAN_POINT('Ctrl Pts',(-5.76538048503894,0.631275792582272,
4.60936787529185));
#164442=CARTESIAN_POINT('Ctrl Pts',(-5.83795905812051,0.601654471648306,
4.46942242443583));
#164443=CARTESIAN_POINT('Ctrl Pts',(-5.8843919857667,0.581858135073001,
4.37501442338295));
#164444=CARTESIAN_POINT('Ctrl Pts',(-5.9288097875027,0.562053380293896,
4.27964240794481));
#164445=CARTESIAN_POINT('Ctrl Pts',(-6.09910575319267,0.767963165980039,
4.39552945347938));
#164446=CARTESIAN_POINT('Ctrl Pts',(-6.02524529610966,0.753333602494622,
4.47299411909348));
#164447=CARTESIAN_POINT('Ctrl Pts',(-5.94975887205415,0.738713518171871,
4.54889472340646));
#164448=CARTESIAN_POINT('Ctrl Pts',(-5.79607632924243,0.709588701400169,
4.69702843502404));
#164449=CARTESIAN_POINT('Ctrl Pts',(-5.71791491197682,0.695086898841296,
4.7692644888865));
#164450=CARTESIAN_POINT('Ctrl Pts',(-5.63825790391852,0.68060907898151,
4.83983461427586));
#164451=CARTESIAN_POINT('Ctrl Pts',(-5.92880978661593,0.562053379307726,
4.27964240748837));
#164452=CARTESIAN_POINT('Ctrl Pts',(-6.00584520189072,0.582224590082771,
4.20738511946269));
#164453=CARTESIAN_POINT('Ctrl Pts',(-6.08121832855712,0.602198953299093,
4.13332724547259));
#164454=CARTESIAN_POINT('Ctrl Pts',(-6.19155853115221,0.631811121691396,
4.01975293231709));
#164455=CARTESIAN_POINT('Ctrl Pts',(-6.22781552682973,0.641604433120965,
3.98155865187309));
#164456=CARTESIAN_POINT('Ctrl Pts',(-6.30251013258213,0.661914305404527,
3.90102502652879));
#164457=CARTESIAN_POINT('Ctrl Pts',(-6.33794987209892,0.671620853463615,
3.86175899060336));
#164458=CARTESIAN_POINT('Ctrl Pts',(-6.37052975388443,0.680609080131929,
3.82495777187308));
#164459=CARTESIAN_POINT('Ctrl Pts',(-5.885111492,0.810731746,4.234142502));
#164460=CARTESIAN_POINT('Ctrl Pts',(-5.652648444,0.745065281,4.557247111));
#164461=CARTESIAN_POINT('Ctrl Pts',(-5.38621099600001,0.680609079,4.852961066));
#164462=CARTESIAN_POINT('Ctrl Pts',(-6.22842029200001,0.810731746,4.17813124));
#164463=CARTESIAN_POINT('Ctrl Pts',(-5.999032377,0.745065281,4.520084201));
#164464=CARTESIAN_POINT('Ctrl Pts',(-5.733588172,0.680609079,4.83486987100001));
#164465=CARTESIAN_POINT('Ctrl Pts',(-6.25425902122499,0.810731746,4.17391561886717));
#164466=CARTESIAN_POINT('Ctrl Pts',(-6.02510255245916,0.745065281,4.51728717870199));
#164467=CARTESIAN_POINT('Ctrl Pts',(-5.75973310271428,0.680609079,4.83350825868783));
#164468=CARTESIAN_POINT('',(-5.512990579203,0.680609081791274,4.84635847385095));
#164469=CARTESIAN_POINT('Ctrl Pts',(-5.386210996,0.680609079,4.852961066));
#164470=CARTESIAN_POINT('Ctrl Pts',(-5.123237026,0.745496505000001,5.144830971));
#164471=CARTESIAN_POINT('Ctrl Pts',(-4.830263629,0.810723991,5.406575004));
#164472=CARTESIAN_POINT('Ctrl Pts',(-5.40430219,0.680609079,5.200338242));
#164473=CARTESIAN_POINT('Ctrl Pts',(-5.122504424,0.745496505000001,5.493188479));
#164474=CARTESIAN_POINT('Ctrl Pts',(-4.810711519,0.810723991,5.75387301500001));
#164475=CARTESIAN_POINT('Ctrl Pts',(-5.40566150155319,0.680609079,5.22643899624792));
#164476=CARTESIAN_POINT('Ctrl Pts',(-5.12244937874635,0.745496505000001,
5.51936289210171));
#164477=CARTESIAN_POINT('Ctrl Pts',(-4.80924243912545,0.810723991,5.77996782105572));
#164478=CARTESIAN_POINT('',(-5.3993374531762,0.680609080406291,5.10500797269187));
#164479=CARTESIAN_POINT('',(-5.39281361407524,0.680609082082614,4.97974064684016));
#164480=CARTESIAN_POINT('',(-5.01149890225682,0.767980175651308,5.60380348523056));
#164481=CARTESIAN_POINT('Ctrl Pts',(-5.39933744653031,0.680609079136191,
5.10500797506104));
#164482=CARTESIAN_POINT('Ctrl Pts',(-5.33844515663971,0.695136944985681,
5.19055708977868));
#164483=CARTESIAN_POINT('Ctrl Pts',(-5.27576094361556,0.709660812727179,
5.27481773443682));
#164484=CARTESIAN_POINT('Ctrl Pts',(-5.14649630147005,0.738780776769514,
5.44117313407239));
#164485=CARTESIAN_POINT('Ctrl Pts',(-5.07990769298335,0.753373671694956,
5.5232334420372));
#164486=CARTESIAN_POINT('Ctrl Pts',(-5.01161176825204,0.767949007809954,
5.60386516329118));
#164487=CARTESIAN_POINT('Ctrl Pts',(-4.833756773168,0.80994605261842,5.40345218029789));
#164488=CARTESIAN_POINT('Ctrl Pts',(-4.86194858070813,0.802922931354232,
5.43517205213695));
#164489=CARTESIAN_POINT('Ctrl Pts',(-4.89016251007618,0.796078752434557,
5.46694857875674));
#164490=CARTESIAN_POINT('Ctrl Pts',(-4.94936212170107,0.782074140029164,
5.53368415521112));
#164491=CARTESIAN_POINT('Ctrl Pts',(-4.98038800577312,0.774939590264265,
5.56869456611257));
#164492=CARTESIAN_POINT('Ctrl Pts',(-5.01139465640152,0.767997185250274,
5.60371510391402));
#164493=CARTESIAN_POINT('Origin',(-1.02652261690928E-12,0.5609257,1.19218870886506E-12));
#164494=CARTESIAN_POINT('',(-4.46601718720579,0.680609080243162,5.93874075972541));
#164495=CARTESIAN_POINT('',(-4.87020089678171,0.562053379627107,5.45410559592523));
#164496=CARTESIAN_POINT('Ctrl Pts',(-4.46601718577088,0.68060908001573,
5.9387407584783));
#164497=CARTESIAN_POINT('Ctrl Pts',(-4.498199451366,0.671661524767342,5.9033439723503));
#164498=CARTESIAN_POINT('Ctrl Pts',(-4.53350159734835,0.661738573394949,
5.863823305951));
#164499=CARTESIAN_POINT('Ctrl Pts',(-4.60570296414624,0.641119488096921,
5.78089960549891));
#164500=CARTESIAN_POINT('Ctrl Pts',(-4.63971125229766,0.63127579251093,
5.74098979630539));
#164501=CARTESIAN_POINT('Ctrl Pts',(-4.74067711382384,0.601654471587487,
5.61991844014854));
#164502=CARTESIAN_POINT('Ctrl Pts',(-4.80631939498106,0.581858135014818,
5.53769935257863));
#164503=CARTESIAN_POINT('Ctrl Pts',(-4.8702008973831,0.562053380258828,
5.45410559623515));
#164504=CARTESIAN_POINT('Ctrl Pts',(-5.01160314811211,0.767963166052343,
5.60389186654709));
#164505=CARTESIAN_POINT('Ctrl Pts',(-4.92281689431306,0.753333602579392,
5.66366763626224));
#164506=CARTESIAN_POINT('Ctrl Pts',(-4.83277891469519,0.738713518264693,
5.72156637672409));
#164507=CARTESIAN_POINT('Ctrl Pts',(-4.65084501993623,0.709588702238808,
5.83319959762432));
#164508=CARTESIAN_POINT('Ctrl Pts',(-4.55898235436246,0.695086899255936,
5.88694442006499));
#164509=CARTESIAN_POINT('Ctrl Pts',(-4.4660171894992,0.680609079003592,
5.93874075440816));
#164510=CARTESIAN_POINT('Ctrl Pts',(-4.87020089667959,0.562053379355376,
5.45410559565212));
#164511=CARTESIAN_POINT('Ctrl Pts',(-4.96096844761636,0.582224590156947,
5.40009798016166));
#164512=CARTESIAN_POINT('Ctrl Pts',(-5.05049964606646,0.602198953364876,
5.34397453247609));
#164513=CARTESIAN_POINT('Ctrl Pts',(-5.18267527581382,0.631811121689457,
5.25677540579544));
#164514=CARTESIAN_POINT('Ctrl Pts',(-5.22629524420352,0.641604433078536,
5.22726826882805));
#164515=CARTESIAN_POINT('Ctrl Pts',(-5.31655605975392,0.661914345679666,
5.16467448282507));
#164516=CARTESIAN_POINT('Ctrl Pts',(-5.3596082152923,0.671620878862863,
5.13394499620549));
#164517=CARTESIAN_POINT('Ctrl Pts',(-5.39933745184495,0.680609080035479,
5.10500797074894));
#164518=CARTESIAN_POINT('Ctrl Pts',(-4.837305378,0.810731746,5.400275611));
#164519=CARTESIAN_POINT('Ctrl Pts',(-4.540819247,0.745065281,5.66585353));
#164520=CARTESIAN_POINT('Ctrl Pts',(-4.217041199,0.680609079,5.897377682));
#164521=CARTESIAN_POINT('Ctrl Pts',(-5.184628575,0.810731746,5.419375106));
#164522=CARTESIAN_POINT('Ctrl Pts',(-4.88709384300001,0.745065281,5.704021776));
#164523=CARTESIAN_POINT('Ctrl Pts',(-4.56018596200001,0.680609079,5.954385274));
#164524=CARTESIAN_POINT('Ctrl Pts',(-5.21076944247076,0.810731746,5.42081260678274));
#164525=CARTESIAN_POINT('Ctrl Pts',(-4.91315578876324,0.745065281,5.70689446365488));
#164526=CARTESIAN_POINT('Ctrl Pts',(-4.58601234460372,0.680609079,5.95867588263245));
#164527=CARTESIAN_POINT('',(-4.34227610870454,0.680609081791272,5.91818331762197));
#164528=CARTESIAN_POINT('Ctrl Pts',(-4.217041199,0.680609079,5.897377682));
#164529=CARTESIAN_POINT('Ctrl Pts',(-3.897472013,0.745496505000001,6.125892201));
#164530=CARTESIAN_POINT('Ctrl Pts',(-3.555080941,0.810723991,6.318536183));
#164531=CARTESIAN_POINT('Ctrl Pts',(-4.160033607,0.680609079,6.240522445));
#164532=CARTESIAN_POINT('Ctrl Pts',(-3.821869971,0.745496505000001,6.465947816));
#164533=CARTESIAN_POINT('Ctrl Pts',(-3.461327142,0.810723991,6.653511435));
#164534=CARTESIAN_POINT('Ctrl Pts',(-4.15575024804733,0.680609079,6.2663051897379));
#164535=CARTESIAN_POINT('Ctrl Pts',(-3.81618948754017,0.745496505000001,
6.4914984525348));
#164536=CARTESIAN_POINT('Ctrl Pts',(-3.45428279649785,0.810723991,6.67868035012586));
#164537=CARTESIAN_POINT('',(-4.17567813270082,0.680609080429674,6.14635367235228));
#164538=CARTESIAN_POINT('',(-4.19623558931298,0.680609082082512,6.02261259398236));
#164539=CARTESIAN_POINT('',(-3.68968074061468,0.767980175621886,6.55011379903614));
#164540=CARTESIAN_POINT('Ctrl Pts',(-4.17567812587055,0.680609079129443,
6.14635367319251));
#164541=CARTESIAN_POINT('Ctrl Pts',(-4.09781893374167,0.695136944833282,
6.21681265412599));
#164542=CARTESIAN_POINT('Ctrl Pts',(-4.01848669565778,0.709660812426448,
6.28562807827921));
#164543=CARTESIAN_POINT('Ctrl Pts',(-3.85648269393038,0.73878077672691,
6.42030610538059));
#164544=CARTESIAN_POINT('Ctrl Pts',(-3.77381034952353,0.753373671653238,
6.48613330649975));
#164545=CARTESIAN_POINT('Ctrl Pts',(-3.68977770889971,0.767949007783995,
6.55019829795612));
#164546=CARTESIAN_POINT('Ctrl Pts',(-3.55916373241255,0.809946052468782,
6.31623729349231));
#164547=CARTESIAN_POINT('Ctrl Pts',(-3.57987759654876,0.80292293116247,
6.35327597790358));
#164548=CARTESIAN_POINT('Ctrl Pts',(-3.60060088545173,0.796078752430467,
6.39037474676793));
#164549=CARTESIAN_POINT('Ctrl Pts',(-3.64407026689995,0.782074139979874,
6.46827624924014));
#164550=CARTESIAN_POINT('Ctrl Pts',(-3.66684457949304,0.774939590228884,
6.50913778396703));
#164551=CARTESIAN_POINT('Ctrl Pts',(-3.6895979313482,0.767997185221761,
6.55000507424667));
#164552=CARTESIAN_POINT('Origin',(-3.39355279987963E-13,0.560925700000022,
7.31619625993218E-13));
#164553=CARTESIAN_POINT('',(-3.08495047167216,0.680609080268415,6.75995798165497));
#164554=CARTESIAN_POINT('',(-3.58386682551787,0.562053379558525,6.37354086850205));
#164555=CARTESIAN_POINT('Ctrl Pts',(-3.08495047063983,0.680609080090048,
6.75995798025519));
#164556=CARTESIAN_POINT('Ctrl Pts',(-3.12398959543952,0.671661524832574,
6.73230698711131));
#164557=CARTESIAN_POINT('Ctrl Pts',(-3.16696217186839,0.661738573458893,
6.70129920981335));
#164558=CARTESIAN_POINT('Ctrl Pts',(-3.25530165505472,0.641119488173938,
6.63583537910247));
#164559=CARTESIAN_POINT('Ctrl Pts',(-3.29709427764183,0.63127579255954,
6.60416941568338));
#164560=CARTESIAN_POINT('Ctrl Pts',(-3.42172637630531,0.601654471555052,
6.50763331609108));
#164561=CARTESIAN_POINT('Ctrl Pts',(-3.50350865092829,0.581858134924881,
6.44144761507033));
#164562=CARTESIAN_POINT('Ctrl Pts',(-3.58386682596175,0.562053380097039,
6.37354086887026));
#164563=CARTESIAN_POINT('Ctrl Pts',(-3.68976354988115,0.767963166022011,
6.5502225238256));
#164564=CARTESIAN_POINT('Ctrl Pts',(-3.5902030457854,0.753333602537464,
6.58951434920594));
#164565=CARTESIAN_POINT('Ctrl Pts',(-3.48982358633362,0.738713518218971,
6.62670394518843));
#164566=CARTESIAN_POINT('Ctrl Pts',(-3.28814535830902,0.70958870162373,
6.69661683535173));
#164567=CARTESIAN_POINT('Ctrl Pts',(-3.18687684475388,0.695086898950739,
6.72935737524069));
#164568=CARTESIAN_POINT('Ctrl Pts',(-3.08495047502156,0.680609078987373,
6.75995797704349));
#164569=CARTESIAN_POINT('Ctrl Pts',(-3.5838668254829,0.562053379326887,
6.37354086825596));
#164570=CARTESIAN_POINT('Ctrl Pts',(-3.68412232234193,0.582224590112365,
6.34030826119271));
#164571=CARTESIAN_POINT('Ctrl Pts',(-3.78362521335049,0.602198953309315,
6.30474350967115));
#164572=CARTESIAN_POINT('Ctrl Pts',(-3.93145588525735,0.63181112170061,
6.247996903327));
#164573=CARTESIAN_POINT('Ctrl Pts',(-3.98039920558153,0.641604433162138,
6.22855663050104));
#164574=CARTESIAN_POINT('Ctrl Pts',(-4.08200559680042,0.661914347710843,
6.18682965572533));
#164575=CARTESIAN_POINT('Ctrl Pts',(-4.13065714833452,0.671620880942573,
6.16607354790408));
#164576=CARTESIAN_POINT('Ctrl Pts',(-4.17567813186649,0.680609080106447,
6.14635367030016));
#164577=CARTESIAN_POINT('Ctrl Pts',(-3.563312241,0.810731746,6.313897835));
#164578=CARTESIAN_POINT('Ctrl Pts',(-3.216666389,0.745065281,6.509530936));
#164579=CARTESIAN_POINT('Ctrl Pts',(-2.850687243,0.680609079,6.666039472));
#164580=CARTESIAN_POINT('Ctrl Pts',(-3.898409388,0.810731746,6.407215015));
#164581=CARTESIAN_POINT('Ctrl Pts',(-3.546640232,0.745065281,6.621245631));
#164582=CARTESIAN_POINT('Ctrl Pts',(-3.173554525,0.680609079,6.79548023900001));
#164583=CARTESIAN_POINT('Ctrl Pts',(-3.92363007654055,0.810731746,6.41423842165485));
#164584=CARTESIAN_POINT('Ctrl Pts',(-3.57147532115351,0.745065281,6.62965370475778));
#164585=CARTESIAN_POINT('Ctrl Pts',(-3.19785474728526,0.680609079,6.80522244450126));
#164586=CARTESIAN_POINT('',(-2.96852163335115,0.680609081791273,6.71328048691971));
#164587=CARTESIAN_POINT('Ctrl Pts',(-2.850687243,0.680609079,6.666039472));
#164588=CARTESIAN_POINT('Ctrl Pts',(-2.48946554,0.745496505000001,6.82051352));
#164589=CARTESIAN_POINT('Ctrl Pts',(-2.11366662,0.810723991,6.93504963400001));
#164590=CARTESIAN_POINT('Ctrl Pts',(-2.721246476,0.680609079,6.988906754));
#164591=CARTESIAN_POINT('Ctrl Pts',(-2.342529127,0.745496505000001,7.13636662));
#164592=CARTESIAN_POINT('Ctrl Pts',(-1.950094955,0.810723991,7.242039054));
#164593=CARTESIAN_POINT('Ctrl Pts',(-2.71152073168206,0.680609079,7.01316591675172));
#164594=CARTESIAN_POINT('Ctrl Pts',(-2.33148881862611,0.745496505000001,
7.16009876068353));
#164595=CARTESIAN_POINT('Ctrl Pts',(-1.93780472968444,0.810723991,7.26510520754985));
#164596=CARTESIAN_POINT('',(-2.75676874420522,0.68060908040802,6.90030270532544));
#164597=CARTESIAN_POINT('',(-2.80344625281094,0.680609082082373,6.7838738706396));
#164598=CARTESIAN_POINT('',(-2.19533720895636,0.767980175607453,7.19014807126775));
#164599=CARTESIAN_POINT('Ctrl Pts',(-2.75676873714112,0.680609079124013,
6.90030270471387));
#164600=CARTESIAN_POINT('Ctrl Pts',(-2.66558325206307,0.69513694475478,
6.95237696872478));
#164601=CARTESIAN_POINT('Ctrl Pts',(-2.57331247625661,0.709660812263954,
7.00252944006454));
#164602=CARTESIAN_POINT('Ctrl Pts',(-2.38614424234407,0.738780776730211,
7.09923269868999));
#164603=CARTESIAN_POINT('Ctrl Pts',(-2.29125382900687,0.753373671657563,
7.14574878616535));
#164604=CARTESIAN_POINT('Ctrl Pts',(-2.19541374540066,0.767949007772609,
7.19025143996891));
#164605=CARTESIAN_POINT('Ctrl Pts',(-2.11814815146974,0.80994605258979,
6.93368216929435));
#164606=CARTESIAN_POINT('Ctrl Pts',(-2.13041551445766,0.8029229313052,6.9743077780005));
#164607=CARTESIAN_POINT('Ctrl Pts',(-2.14267916591134,0.796078752395621,
7.01499409375212));
#164608=CARTESIAN_POINT('Ctrl Pts',(-2.16838573688887,0.782074139977238,
7.10041893415635));
#164609=CARTESIAN_POINT('Ctrl Pts',(-2.18184357659784,0.774939590214724,
7.14522095300597));
#164610=CARTESIAN_POINT('Ctrl Pts',(-2.19527970834756,0.767997185208149,
7.19002408685864));
#164611=CARTESIAN_POINT('Origin',(-2.64545330086463E-14,0.5609257,1.60895602396849E-13));
#164612=CARTESIAN_POINT('',(-1.55963490112623,0.680609080260179,7.2650870814962));
#164613=CARTESIAN_POINT('',(-2.12995512369142,0.562053379543022,6.9949564542138));
#164614=CARTESIAN_POINT('Ctrl Pts',(-1.55963490040577,0.68060908007041,
7.2650870798815));
#164615=CARTESIAN_POINT('Ctrl Pts',(-1.60370545790053,0.671661524877215,
7.24647480959136));
#164616=CARTESIAN_POINT('Ctrl Pts',(-1.65233911476708,0.66173857351751,
7.22542981061857));
#164617=CARTESIAN_POINT('Ctrl Pts',(-1.75268605847454,0.64111948821144,
7.18048686545229));
#164618=CARTESIAN_POINT('Ctrl Pts',(-1.8003088388687,0.631275792597886,
7.1585454131383));
#164619=CARTESIAN_POINT('Ctrl Pts',(-1.94277951599448,0.60165447163943,
7.09105849111672));
#164620=CARTESIAN_POINT('Ctrl Pts',(-2.03687773564085,0.581858135058827,
7.0440009466781));
#164621=CARTESIAN_POINT('Ctrl Pts',(-2.12995512416222,0.56205338025852,
6.99495645481837));
#164622=CARTESIAN_POINT('Ctrl Pts',(-2.19539470956517,0.767963166006757,
7.19027205567687));
#164623=CARTESIAN_POINT('Ctrl Pts',(-2.08971529368618,0.753333602535716,
7.20724269465628));
#164624=CARTESIAN_POINT('Ctrl Pts',(-1.98368798634468,0.738713518218528,
7.2219842019864));
#164625=CARTESIAN_POINT('Ctrl Pts',(-1.77169567685954,0.709588701411639,
7.2469077103715));
#164626=CARTESIAN_POINT('Ctrl Pts',(-1.66575651738361,0.695086898844228,
7.25711305757202));
#164627=CARTESIAN_POINT('Ctrl Pts',(-1.5596349054588,0.680609078981565,
7.26508707768309));
#164628=CARTESIAN_POINT('Ctrl Pts',(-2.12995512371633,0.562053379235256,
6.99495645388449));
#164629=CARTESIAN_POINT('Ctrl Pts',(-2.23501073117867,0.582224590034869,
6.984052774955));
#164630=CARTESIAN_POINT('Ctrl Pts',(-2.33983267040083,0.602198953270739,
6.97070968781844));
#164631=CARTESIAN_POINT('Ctrl Pts',(-2.49640598601594,0.631811121639731,
6.94706901029063));
#164632=CARTESIAN_POINT('Ctrl Pts',(-2.54838412220583,0.641604433021573,
6.93860460746325));
#164633=CARTESIAN_POINT('Ctrl Pts',(-2.65658491108027,0.661914316173451,
6.91969558617028));
#164634=CARTESIAN_POINT('Ctrl Pts',(-2.70856101523815,0.671620860105384,
6.90988338572812));
#164635=CARTESIAN_POINT('Ctrl Pts',(-2.75676874381832,0.680609080045511,
6.90030270303855));
#164636=CARTESIAN_POINT('Ctrl Pts',(-2.122702584,0.810731746,6.932289213));
#164637=CARTESIAN_POINT('Ctrl Pts',(-1.742105785,0.745065281,7.04882990900001));
#164638=CARTESIAN_POINT('Ctrl Pts',(-1.35103832,0.680609079,7.123004665));
#164639=CARTESIAN_POINT('Ctrl Pts',(-2.429904911,0.810731746,7.09546067));
#164640=CARTESIAN_POINT('Ctrl Pts',(-2.040349667,0.745065281,7.2288674));
#164641=CARTESIAN_POINT('Ctrl Pts',(-1.638531205,0.680609079,7.3188261));
#164642=CARTESIAN_POINT('Ctrl Pts',(-2.45302612909604,0.810731746,7.10774157581601));
#164643=CARTESIAN_POINT('Ctrl Pts',(-2.06279663837835,0.745065281,7.24241770782328));
#164644=CARTESIAN_POINT('Ctrl Pts',(-1.66016901536446,0.680609079,7.33356436761252));
#164645=CARTESIAN_POINT('',(-1.45596238572947,0.680609081791274,7.19447212189389));
#164646=CARTESIAN_POINT('Ctrl Pts',(-1.35103832,0.680609079,7.123004665));
#164647=CARTESIAN_POINT('Ctrl Pts',(-0.965054425,0.745496505000001,7.196215207));
#164648=CARTESIAN_POINT('Ctrl Pts',(-0.573419596,0.810723991,7.227287871));
#164649=CARTESIAN_POINT('Ctrl Pts',(-1.155216884,0.680609079,7.410497551));
#164650=CARTESIAN_POINT('Ctrl Pts',(-0.753654224,0.745496505000001,7.47309685200001));
#164651=CARTESIAN_POINT('Ctrl Pts',(-0.347678495,0.810723991,7.491936977));
#164652=CARTESIAN_POINT('Ctrl Pts',(-1.14050351955617,0.680609079,7.43209880004164));
#164653=CARTESIAN_POINT('Ctrl Pts',(-0.737770323522364,0.745496505000001,
7.49390080806278));
#164654=CARTESIAN_POINT('Ctrl Pts',(-0.330717067503553,0.810723991,7.51182182120221));
#164655=CARTESIAN_POINT('',(-1.27957088547559,0.680609082082176,7.22792874414072));
#164656=CARTESIAN_POINT('Ctrl Pts',(-0.578090315820934,0.809946052643239,
7.22691577379934));
#164657=CARTESIAN_POINT('Ctrl Pts',(-0.581337569923514,0.802922931341175,
7.26922869880324));
#164658=CARTESIAN_POINT('Ctrl Pts',(-0.584568148992888,0.796078752436324,
7.31160011357802));
#164659=CARTESIAN_POINT('Ctrl Pts',(-0.5913098993982,0.782074139999187,
7.40055392161798));
#164660=CARTESIAN_POINT('Ctrl Pts',(-0.59482199270295,0.774939590230869,
7.44720153191403));
#164661=CARTESIAN_POINT('Ctrl Pts',(-0.598312645844489,0.76799718521972,
7.49384556457247));
#164662=CARTESIAN_POINT('Ctrl Pts',(-0.582837713,0.810731746,7.226534453));
#164663=CARTESIAN_POINT('Ctrl Pts',(-0.186086252,0.745065281,7.258533431));
#164664=CARTESIAN_POINT('Ctrl Pts',(0.211783654,0.680609079,7.246906077));
#164665=CARTESIAN_POINT('Ctrl Pts',(-0.847780781,0.810731746,7.451930471));
#164666=CARTESIAN_POINT('Ctrl Pts',(-0.438654618,0.745065281,7.498475363));
#164667=CARTESIAN_POINT('Ctrl Pts',(-0.026891988,0.680609079,7.499951788));
#164668=CARTESIAN_POINT('Ctrl Pts',(-0.867721406319764,0.810731746,7.46889463457459));
#164669=CARTESIAN_POINT('Ctrl Pts',(-0.457663876072119,0.745065281,7.51653430751449));
#164670=CARTESIAN_POINT('Ctrl Pts',(-0.0448556267017154,0.680609079,7.51899697287656));
#164671=CARTESIAN_POINT('',(0.124676045108029,0.680609081791274,7.33925823720938));
#164672=CARTESIAN_POINT('Ctrl Pts',(0.38842861563543,0.681884070047851,
7.42155191714904));
#164673=CARTESIAN_POINT('Ctrl Pts',(0.392458295317715,0.681246574523926,
7.42133662307453));
#164674=CARTESIAN_POINT('Ctrl Pts',(0.396487975,0.680609079,7.421121329));
#164675=CARTESIAN_POINT('Ctrl Pts',(0.402929351,0.679590053,7.420777185));
#164676=CARTESIAN_POINT('Ctrl Pts',(0.40937012,0.678571429,7.420421861));
#164677=CARTESIAN_POINT('Ctrl Pts',(0.808182013,0.615498301,7.398420191));
#164678=CARTESIAN_POINT('Ctrl Pts',(1.202338414,0.551245526,7.333800299));
#164679=CARTESIAN_POINT('Ctrl Pts',(0.203913492723899,0.681884070047851,
7.2471360750122));
#164680=CARTESIAN_POINT('Ctrl Pts',(0.207848573361949,0.681246574523926,
7.2470210760061));
#164681=CARTESIAN_POINT('Ctrl Pts',(0.211783654,0.680609079,7.246906077));
#164682=CARTESIAN_POINT('Ctrl Pts',(0.218073815,0.679590053,7.246722253));
#164683=CARTESIAN_POINT('Ctrl Pts',(0.224363648,0.678571429,7.24652751));
#164684=CARTESIAN_POINT('Ctrl Pts',(0.613829558,0.615498301,7.234469046));
#164685=CARTESIAN_POINT('Ctrl Pts',(0.999759533999999,0.551245526,7.180736792));
#164686=CARTESIAN_POINT('',(0.995066308632371,0.55202682598065,7.18138865692373));
#164687=CARTESIAN_POINT('Origin',(-0.0491214261700275,0.411147083219614,
-0.184599448970936));
#164688=CARTESIAN_POINT('Origin',(1.09128087012227,0.300047239099359,9.32655164468723));
#164689=CARTESIAN_POINT('Ctrl Pts',(0.837099778000001,0.551266351,7.384409824));
#164690=CARTESIAN_POINT('Ctrl Pts',(1.239349841,0.615380951,7.338810589));
#164691=CARTESIAN_POINT('Ctrl Pts',(1.634266632,0.680609079,7.24978738));
#164692=CARTESIAN_POINT('Ctrl Pts',(1.63822684695898,0.681263184913293,
7.2488946576544));
#164693=CARTESIAN_POINT('Ctrl Pts',(1.64218706191796,0.681917290826586,
7.2480019353088));
#164694=CARTESIAN_POINT('Ctrl Pts',(0.990426433,0.551266351,7.182030039));
#164695=CARTESIAN_POINT('Ctrl Pts',(1.381652286,0.615380951,7.12807866));
#164696=CARTESIAN_POINT('Ctrl Pts',(1.764702859,0.680609079,7.03195021400001));
#164697=CARTESIAN_POINT('Ctrl Pts',(1.76854407984401,0.681263184913293,
7.03098624052886));
#164698=CARTESIAN_POINT('Ctrl Pts',(1.77238530068803,0.681917290826586,
7.03002226705771));
#164699=CARTESIAN_POINT('Origin',(-0.0663475152002066,0.803452713883071,
-0.180685821127333));
#164700=CARTESIAN_POINT('Ctrl Pts',(1.97476165197866,0.681884070047877,
7.16453948434253));
#164701=CARTESIAN_POINT('Ctrl Pts',(1.97865083848933,0.681246574523938,
7.16346296267127));
#164702=CARTESIAN_POINT('Ctrl Pts',(1.982540025,0.680609079,7.16238644100001));
#164703=CARTESIAN_POINT('Ctrl Pts',(1.988756825,0.679590053,7.160665639));
#164704=CARTESIAN_POINT('Ctrl Pts',(1.994970628,0.678571429,7.158934046));
#164705=CARTESIAN_POINT('Ctrl Pts',(2.379728812,0.615498301,7.051713995));
#164706=CARTESIAN_POINT('Ctrl Pts',(2.750778689,0.551245526,6.903872905));
#164707=CARTESIAN_POINT('Ctrl Pts',(1.75706614025095,0.681884070047877,
7.03386668559918));
#164708=CARTESIAN_POINT('Ctrl Pts',(1.76088449962548,0.681246574523938,
7.03290844979959));
#164709=CARTESIAN_POINT('Ctrl Pts',(1.764702859,0.680609079,7.031950214));
#164710=CARTESIAN_POINT('Ctrl Pts',(1.770806443,0.679590053,7.03041849));
#164711=CARTESIAN_POINT('Ctrl Pts',(1.776907359,0.678571429,7.028876172));
#164712=CARTESIAN_POINT('Ctrl Pts',(2.154675559,0.615498301,6.93337597));
#164713=CARTESIAN_POINT('Ctrl Pts',(2.52003186,0.551245526,6.79793640900001));
#164714=CARTESIAN_POINT('Ctrl Pts',(1.75488918513368,0.681884070047877,
7.03255995761175));
#164715=CARTESIAN_POINT('Ctrl Pts',(1.75870683623684,0.681246574523938,
7.03160290467088));
#164716=CARTESIAN_POINT('Ctrl Pts',(1.76252448734,0.680609079,7.03064585173001));
#164717=CARTESIAN_POINT('Ctrl Pts',(1.76862693918,0.679590053,7.02911601851));
#164718=CARTESIAN_POINT('Ctrl Pts',(1.77472672631,0.678571429,7.02757559326));
#164719=CARTESIAN_POINT('Ctrl Pts',(2.15242502647,0.615498301,6.93219258975));
#164720=CARTESIAN_POINT('Ctrl Pts',(2.51772439171,0.551245526,6.79687704404));
#164721=CARTESIAN_POINT('',(2.51558848957853,0.552026826152232,6.79958193857544));
#164722=CARTESIAN_POINT('Origin',(-0.0876565386706685,0.411145059523696,
-0.169723290623195));
#164723=CARTESIAN_POINT('Ctrl Pts',(2.53752478119287,0.562053380749443,
6.85763024745969));
#164724=CARTESIAN_POINT('Ctrl Pts',(2.53022429687456,0.558751695416953,
6.83826947494369));
#164725=CARTESIAN_POINT('Ctrl Pts',(2.52291237727739,0.555410033627866,
6.81891978007072));
#164726=CARTESIAN_POINT('Ctrl Pts',(2.51558848261983,0.552026824786843,
6.79958194233847));
#164727=CARTESIAN_POINT('Ctrl Pts',(2.404958681,0.551266351,7.031814718));
#164728=CARTESIAN_POINT('Ctrl Pts',(2.788001874,0.615380951000001,6.900809695));
#164729=CARTESIAN_POINT('Ctrl Pts',(3.154548371,0.680609079,6.728972363));
#164730=CARTESIAN_POINT('Ctrl Pts',(3.15822408941376,0.681263184913293,
6.72724918285622));
#164731=CARTESIAN_POINT('Ctrl Pts',(3.16189980782752,0.681917290826586,
6.72552600271243));
#164732=CARTESIAN_POINT('Ctrl Pts',(2.51119550620449,0.551266351,6.80120460239308));
#164733=CARTESIAN_POINT('Ctrl Pts',(2.88167670203736,0.615380951000001,
6.66441255329342));
#164734=CARTESIAN_POINT('Ctrl Pts',(3.23510692508309,0.680609079,6.48818696522738));
#164735=CARTESIAN_POINT('Ctrl Pts',(3.23865111385439,0.681263184913293,
6.48641977976979));
#164736=CARTESIAN_POINT('Ctrl Pts',(3.24219530262569,0.681917290826586,
6.48465259431219));
#164737=CARTESIAN_POINT('Origin',(-0.103639972525845,0.803453476587346,
-0.162201929279258));
#164738=CARTESIAN_POINT('Ctrl Pts',(3.46875702882675,0.681884070047877,
6.57252115311179));
#164739=CARTESIAN_POINT('Ctrl Pts',(3.47232386791338,0.681246574523938,
6.5706337390559));
#164740=CARTESIAN_POINT('Ctrl Pts',(3.475890707,0.680609079,6.568746325));
#164741=CARTESIAN_POINT('Ctrl Pts',(3.48159224,0.679590053,6.565729325));
#164742=CARTESIAN_POINT('Ctrl Pts',(3.487288527,0.678571429,6.562702432));
#164743=CARTESIAN_POINT('Ctrl Pts',(3.840002137,0.615498301,6.37527749));
#164744=CARTESIAN_POINT('Ctrl Pts',(4.17059561,0.551245526,6.151128087));
#164745=CARTESIAN_POINT('Ctrl Pts',(3.22806032850427,0.681884070047877,
6.49170151124601));
#164746=CARTESIAN_POINT('Ctrl Pts',(3.23158342425213,0.681246574523938,
6.48994484362301));
#164747=CARTESIAN_POINT('Ctrl Pts',(3.23510652,0.680609079,6.488188176));
#164748=CARTESIAN_POINT('Ctrl Pts',(3.24073813,0.679590053,6.485380172));
#164749=CARTESIAN_POINT('Ctrl Pts',(3.246364857,0.678571429,6.482562396));
#164750=CARTESIAN_POINT('Ctrl Pts',(3.594771326,0.615498301,6.308085939));
#164751=CARTESIAN_POINT('Ctrl Pts',(3.922470298,0.551245526,6.09727207499999));
#164752=CARTESIAN_POINT('',(3.91848455392433,0.552026825957499,6.09983432550923));
#164753=CARTESIAN_POINT('Origin',(-0.122092729018598,0.411147120165791,
-0.14691242890606));
#164754=CARTESIAN_POINT('Origin',(4.90675131577093,0.30001629144851,8.00672439438912));
#164755=CARTESIAN_POINT('Ctrl Pts',(3.860364389,0.551266351,6.350419771));
#164756=CARTESIAN_POINT('Ctrl Pts',(4.206290037,0.615380951,6.14013460900001));
#164757=CARTESIAN_POINT('Ctrl Pts',(4.527326934,0.680609079,5.893518076));
#164758=CARTESIAN_POINT('Ctrl Pts',(4.53054628336893,0.681263184913293,
5.89104501203975));
#164759=CARTESIAN_POINT('Ctrl Pts',(4.53376563273785,0.681917290826586,
5.88857194807951));
#164760=CARTESIAN_POINT('Ctrl Pts',(3.9145430984241,0.551266351,6.10236341471059));
#164761=CARTESIAN_POINT('Ctrl Pts',(4.24695640248066,0.615380951,5.88912698187087));
#164762=CARTESIAN_POINT('Ctrl Pts',(4.5542403313273,0.680609079,5.6410443994992));
#164763=CARTESIAN_POINT('Ctrl Pts',(4.55732176630146,0.681263184913293,
5.63855663403529));
#164764=CARTESIAN_POINT('Ctrl Pts',(4.56040320127563,0.681917290826586,
5.63606886857137));
#164765=CARTESIAN_POINT('Origin',(-0.136085561345225,0.803453460267691,
-0.136130227890238));
#164766=CARTESIAN_POINT('Ctrl Pts',(4.80055718210444,0.681884070047877,
5.67317903306963));
#164767=CARTESIAN_POINT('Ctrl Pts',(4.80363489255222,0.681246574523938,
5.67056898153481));
#164768=CARTESIAN_POINT('Ctrl Pts',(4.806712603,0.680609079,5.66795893));
#164769=CARTESIAN_POINT('Ctrl Pts',(4.811632272,0.679590053,5.663786806));
#164770=CARTESIAN_POINT('Ctrl Pts',(4.81654469,0.678571429,5.659606147));
#164771=CARTESIAN_POINT('Ctrl Pts',(5.120721229,0.615498301,5.40074009600001));
#164772=CARTESIAN_POINT('Ctrl Pts',(5.395400115,0.551245526,5.110763357));
#164773=CARTESIAN_POINT('Ctrl Pts',(4.5481140040602,0.681884070047877,5.64599158717324));
#164774=CARTESIAN_POINT('Ctrl Pts',(4.5511771000301,0.681246574523938,5.64351862808662));
#164775=CARTESIAN_POINT('Ctrl Pts',(4.554240196,0.680609079,5.641045669));
#164776=CARTESIAN_POINT('Ctrl Pts',(4.559136504,0.679590053,5.637092685));
#164777=CARTESIAN_POINT('Ctrl Pts',(4.564025943,0.678571429,5.633131207));
#164778=CARTESIAN_POINT('Ctrl Pts',(4.866779581,0.615498301,5.387836821));
#164779=CARTESIAN_POINT('Ctrl Pts',(5.141498385,0.551245526,5.111506076));
#164780=CARTESIAN_POINT('',(5.13815663269613,0.552026825934544,5.11486523958666));
#164781=CARTESIAN_POINT('Origin',(-0.150820139731521,0.41114713854277,-0.117231435818382));
#164782=CARTESIAN_POINT('Origin',(6.51225232756528,0.300122489565501,6.76356590004443));
#164783=CARTESIAN_POINT('Ctrl Pts',(5.135263749,0.551266351,5.372086254));
#164784=CARTESIAN_POINT('Ctrl Pts',(5.427896753,0.615380951,5.092353653));
#164785=CARTESIAN_POINT('Ctrl Pts',(5.688412722,0.680609079,4.782489435));
#164786=CARTESIAN_POINT('Ctrl Pts',(5.69102516913063,0.681263184913293,
4.7793821249556));
#164787=CARTESIAN_POINT('Ctrl Pts',(5.69363761626127,0.681917290826586,
4.77627481491121));
#164788=CARTESIAN_POINT('Ctrl Pts',(5.134851007,0.551266351,5.118183773));
#164789=CARTESIAN_POINT('Ctrl Pts',(5.413653213,0.615380951,4.838473655));
#164790=CARTESIAN_POINT('Ctrl Pts',(5.660422662,0.680609079,4.530134136));
#164791=CARTESIAN_POINT('Ctrl Pts',(5.66289725939779,0.681263184913293,
4.52704211559617));
#164792=CARTESIAN_POINT('Ctrl Pts',(5.66537185679557,0.681917290826586,
4.52395009519234));
#164793=CARTESIAN_POINT('Origin',(-0.162167589274738,0.803452522456232,
-0.103693095701407));
#164794=CARTESIAN_POINT('Ctrl Pts',(5.90788861795456,0.681884070047877,
4.50856537016347));
#164795=CARTESIAN_POINT('Ctrl Pts',(5.91033328897728,0.681246574523938,
4.50535472308173));
#164796=CARTESIAN_POINT('Ctrl Pts',(5.91277796,0.680609079,4.502144076));
#164797=CARTESIAN_POINT('Ctrl Pts',(5.916685726,0.679590053,4.49701191));
#164798=CARTESIAN_POINT('Ctrl Pts',(5.920584577,0.678571429,4.491872968));
#164799=CARTESIAN_POINT('Ctrl Pts',(6.162001088,0.615498301,4.173670097));
#164800=CARTESIAN_POINT('Ctrl Pts',(6.367921707,0.551245526,3.831425012));
#164801=CARTESIAN_POINT('Ctrl Pts',(5.65550292364228,0.681884070047877,
4.53628137163686));
#164802=CARTESIAN_POINT('Ctrl Pts',(5.65796279282114,0.681246574523938,
4.53320775381843));
#164803=CARTESIAN_POINT('Ctrl Pts',(5.660422662,0.680609079,4.530134136));
#164804=CARTESIAN_POINT('Ctrl Pts',(5.664354722,0.679590053,4.525221009));
#164805=CARTESIAN_POINT('Ctrl Pts',(5.668278248,0.678571429,4.520301063));
#164806=CARTESIAN_POINT('Ctrl Pts',(5.911222633,0.615498301,4.215658441));
#164807=CARTESIAN_POINT('Ctrl Pts',(6.120115721,0.551245526,3.886731733));
#164808=CARTESIAN_POINT('',(6.11757421807822,0.552026825940366,3.89073073953274));
#164809=CARTESIAN_POINT('Origin',(-0.172495070084803,0.411147101698712,
-0.0820685574945201));
#164810=CARTESIAN_POINT('Origin',(7.81397171485883,0.300138470944808,5.20550314261985));
#164811=CARTESIAN_POINT('Ctrl Pts',(6.170043883,0.551266351,4.142559954));
#164812=CARTESIAN_POINT('Ctrl Pts',(6.39570105,0.615380951,3.8064599));
#164813=CARTESIAN_POINT('Ctrl Pts',(6.583514653,0.680609079,3.447836903));
#164814=CARTESIAN_POINT('Ctrl Pts',(6.58539804275969,0.681263184913293,
3.44424064123114));
#164815=CARTESIAN_POINT('Ctrl Pts',(6.58728143251939,0.681917290826587,
3.44064437946229));
#164816=CARTESIAN_POINT('Ctrl Pts',(6.11505898654828,0.551266351,3.89468105272049));
#164817=CARTESIAN_POINT('Ctrl Pts',(6.32721347665985,0.615380951,3.56157618377961));
#164818=CARTESIAN_POINT('Ctrl Pts',(6.50192964480889,0.680609079,3.2073973571239));
#164819=CARTESIAN_POINT('Ctrl Pts',(6.50368169384414,0.681263184913293,
3.20384566137573));
#164820=CARTESIAN_POINT('Ctrl Pts',(6.5054337428794,0.681917290826587,3.20029396562756));
#164821=CARTESIAN_POINT('Origin',(-0.180667349183379,0.803453434661462,
-0.0664075156033789));
#164822=CARTESIAN_POINT('Ctrl Pts',(6.73897374700992,0.681884070047882,
3.13313619990097));
#164823=CARTESIAN_POINT('Ctrl Pts',(6.74067106900496,0.681246574523941,
3.12947508395048));
#164824=CARTESIAN_POINT('Ctrl Pts',(6.742368391,0.680609079,3.125813968));
#164825=CARTESIAN_POINT('Ctrl Pts',(6.745081532,0.679590053000001,3.119961735));
#164826=CARTESIAN_POINT('Ctrl Pts',(6.747784509,0.678571429,3.114104801));
#164827=CARTESIAN_POINT('Ctrl Pts',(6.915152625,0.615498301,2.751443923));
#164828=CARTESIAN_POINT('Ctrl Pts',(7.042686358,0.551245526,2.372933492));
#164829=CARTESIAN_POINT('Ctrl Pts',(6.49844681077687,0.681884070047882,
3.21445968164217));
#164830=CARTESIAN_POINT('Ctrl Pts',(6.50018843288844,0.681246574523941,
3.21092912382109));
#164831=CARTESIAN_POINT('Ctrl Pts',(6.501930055,0.680609079,3.207398566));
#164832=CARTESIAN_POINT('Ctrl Pts',(6.504714009,0.679590053000001,3.201755028));
#164833=CARTESIAN_POINT('Ctrl Pts',(6.507488162,0.678571429,3.196106666));
#164834=CARTESIAN_POINT('Ctrl Pts',(6.679263483,0.615498301,2.846360558));
#164835=CARTESIAN_POINT('Ctrl Pts',(6.81256324800001,0.551245526,2.480218134));
#164836=CARTESIAN_POINT('',(6.81094083240474,0.552026825957956,2.48466999354874));
#164837=CARTESIAN_POINT('Origin',(-0.186104521948789,0.411147115358488,
-0.0430684921105004));
#164838=CARTESIAN_POINT('Origin',(8.7514997255839,0.300018450747821,3.4045703757469));
#164839=CARTESIAN_POINT('Ctrl Pts',(6.916319623,0.551266351,2.719332154));
#164840=CARTESIAN_POINT('Ctrl Pts',(7.064449474,0.615380951,2.342580312));
#164841=CARTESIAN_POINT('Ctrl Pts',(7.170778755,0.680609079,1.951967349));
#164842=CARTESIAN_POINT('Ctrl Pts',(7.17184502217018,0.681263184913293,
1.94805029271246));
#164843=CARTESIAN_POINT('Ctrl Pts',(7.17291128934035,0.681917290826587,
1.94413323642491));
#164844=CARTESIAN_POINT('Ctrl Pts',(6.80933360604283,0.551266351,2.48906865116737));
#164845=CARTESIAN_POINT('Ctrl Pts',(6.94492034197236,0.615380951,2.11814464547145));
#164846=CARTESIAN_POINT('Ctrl Pts',(7.03941376445819,0.680609079,1.73468751145306));
#164847=CARTESIAN_POINT('Ctrl Pts',(7.0403613419575,0.681263184913293,1.73084221362609));
#164848=CARTESIAN_POINT('Ctrl Pts',(7.04130891945682,0.681917290826587,
1.72699691579912));
#164849=CARTESIAN_POINT('Origin',(-0.190719082213691,0.803453445641696,
-0.0260168029193106));
#164850=CARTESIAN_POINT('Ctrl Pts',(7.25495195577507,0.681884070047882,
1.61120506410122));
#164851=CARTESIAN_POINT('Ctrl Pts',(7.25582256288753,0.681246574523941,
1.60726466905061));
#164852=CARTESIAN_POINT('Ctrl Pts',(7.25669317,0.680609079,1.603324274));
#164853=CARTESIAN_POINT('Ctrl Pts',(7.258084821,0.679590053000001,1.597025618));
#164854=CARTESIAN_POINT('Ctrl Pts',(7.259465537,0.678571429,1.590724555));
#164855=CARTESIAN_POINT('Ctrl Pts',(7.344959311,0.615498301,1.200563289));
#164856=CARTESIAN_POINT('Ctrl Pts',(7.388142822,0.551245526,0.803486239));
#164857=CARTESIAN_POINT('Ctrl Pts',(7.03753054804688,0.681884070047882,
1.74233342918306));
#164858=CARTESIAN_POINT('Ctrl Pts',(7.03847248652344,0.681246574523941,
1.73851101659153));
#164859=CARTESIAN_POINT('Ctrl Pts',(7.039414425,0.680609079,1.734688604));
#164860=CARTESIAN_POINT('Ctrl Pts',(7.040920098,0.679590053000001,1.728578541));
#164861=CARTESIAN_POINT('Ctrl Pts',(7.042415162,0.678571429,1.722465874));
#164862=CARTESIAN_POINT('Ctrl Pts',(7.134989397,0.615498301,1.343970018));
#164863=CARTESIAN_POINT('Ctrl Pts',(7.186462889,0.551245526,0.957732292));
#164864=CARTESIAN_POINT('',(7.18583542279277,0.552026825978395,0.962428841414932));
#164865=CARTESIAN_POINT('Origin',(-0.191012030134711,0.411147106807098,
-0.00205461113786623));
#164866=CARTESIAN_POINT('Origin',(9.27850705784563,0.300053135916551,1.44360164381105));
#164867=CARTESIAN_POINT('Ctrl Pts',(7.339195944,0.551266351,1.168951406));
#164868=CARTESIAN_POINT('Ctrl Pts',(7.402872092,0.615380951,0.769164273));
#164869=CARTESIAN_POINT('Ctrl Pts',(7.422745213,0.680609079,0.364825971));
#164870=CARTESIAN_POINT('Ctrl Pts',(7.42294450012291,0.681263184913293,
0.360771277382102));
#164871=CARTESIAN_POINT('Ctrl Pts',(7.42314378724581,0.681917290826587,
0.356716583764203));
#164872=CARTESIAN_POINT('Ctrl Pts',(7.18521135359354,0.551266351,0.967070166715704));
#164873=CARTESIAN_POINT('Ctrl Pts',(7.23789045028809,0.615380951,0.575671017899855));
#164874=CARTESIAN_POINT('Ctrl Pts',(7.24774271989205,0.680609079,0.18086560584187));
#164875=CARTESIAN_POINT('Ctrl Pts',(7.24784151818667,0.681263184913293,
0.176906507787927));
#164876=CARTESIAN_POINT('Ctrl Pts',(7.24794031648128,0.681917290826587,
0.172947409733983));
#164877=CARTESIAN_POINT('Origin',(-0.191852911351374,0.803453428315243,
0.0155904250026355));
#164878=CARTESIAN_POINT('Ctrl Pts',(7.43169667121216,0.681884070047882,
0.0139357695080207));
#164879=CARTESIAN_POINT('Ctrl Pts',(7.43169985610608,0.681246574523941,
0.00990034375401035));
#164880=CARTESIAN_POINT('Ctrl Pts',(7.431703041,0.680609079,0.005864918));
#164881=CARTESIAN_POINT('Ctrl Pts',(7.431708132,0.679590053000001,-0.000585643));
#164882=CARTESIAN_POINT('Ctrl Pts',(7.431702024,0.678571429,-0.007036203));
#164883=CARTESIAN_POINT('Ctrl Pts',(7.431323862,0.615498301,-0.40645435));
#164884=CARTESIAN_POINT('Ctrl Pts',(7.38813793800001,0.551245526,-0.803531138000001));
#164885=CARTESIAN_POINT('Ctrl Pts',(7.24754717756366,0.681884070047882,
0.1887376018885));
#164886=CARTESIAN_POINT('Ctrl Pts',(7.24764538878184,0.681246574523941,
0.18480206644425));
#164887=CARTESIAN_POINT('Ctrl Pts',(7.2477436,0.680609079,0.180866531));
#164888=CARTESIAN_POINT('Ctrl Pts',(7.247900589,0.679590053000001,0.174575643));
#164889=CARTESIAN_POINT('Ctrl Pts',(7.248046656,0.678571429,0.168284491));
#164890=CARTESIAN_POINT('Ctrl Pts',(7.257091136,0.615498301,-0.221263065));
#164891=CARTESIAN_POINT('Ctrl Pts',(7.224331513,0.551245526,-0.609536047));
#164892=CARTESIAN_POINT('Ctrl Pts',(7.24570568262718,0.681884070047882,
0.190485620212305));
#164893=CARTESIAN_POINT('Ctrl Pts',(7.24580484410859,0.681246574523941,
0.186551083671152));
#164894=CARTESIAN_POINT('Ctrl Pts',(7.24590400559,0.680609079,0.18261654713));
#164895=CARTESIAN_POINT('Ctrl Pts',(7.24606251356999,0.679590053000001,
0.17632725586));
#164896=CARTESIAN_POINT('Ctrl Pts',(7.24621010232,0.678571429,0.17003769794));
#164897=CARTESIAN_POINT('Ctrl Pts',(7.25534880874,0.615498301,-0.21941115215));
#164898=CARTESIAN_POINT('Ctrl Pts',(7.22269344875001,0.551245526,-0.60759609609));
#164899=CARTESIAN_POINT('',(7.22472833507074,0.552026826383927,-0.604814410547277));
#164900=CARTESIAN_POINT('Origin',(-0.186987466365719,0.41114500527251,0.0390556790372377));
#164901=CARTESIAN_POINT('Ctrl Pts',(7.28652936256475,0.562053380502287,
-0.610421555679701));
#164902=CARTESIAN_POINT('Ctrl Pts',(7.26592120359517,0.558751695429002,
-0.60856673103941));
#164903=CARTESIAN_POINT('Ctrl Pts',(7.24532065958405,0.555410033641427,
-0.60669792256753));
#164904=CARTESIAN_POINT('Ctrl Pts',(7.22472833612555,0.552026824884503,
-0.604814404498353));
#164905=CARTESIAN_POINT('Ctrl Pts',(7.418899619,0.551266351,-0.436088211));
#164906=CARTESIAN_POINT('Ctrl Pts',(7.395144639,0.615380951,-0.840217033));
#164907=CARTESIAN_POINT('Ctrl Pts',(7.327632355,0.680609079,-1.239374263));
#164908=CARTESIAN_POINT('Ctrl Pts',(7.32695534363177,0.681263184913293,
-1.24337700096723));
#164909=CARTESIAN_POINT('Ctrl Pts',(7.32627833226354,0.681917290826587,
-1.24737973893445));
#164910=CARTESIAN_POINT('Ctrl Pts',(7.225117579,0.551266351,-0.600146619));
#164911=CARTESIAN_POINT('Ctrl Pts',(7.19242586500001,0.615380951,-0.993719575));
#164912=CARTESIAN_POINT('Ctrl Pts',(7.11717634000001,0.680609079,-1.381412661));
#164913=CARTESIAN_POINT('Ctrl Pts',(7.11642173978711,0.681263184913293,
-1.38530043683952));
#164914=CARTESIAN_POINT('Ctrl Pts',(7.11566713957423,0.681917290826587,
-1.38918821267904));
#164915=CARTESIAN_POINT('Origin',(-0.184016267475409,0.803452540152115,
0.056468539661578));
#164916=CARTESIAN_POINT('Ctrl Pts',(7.26094351293389,0.681884070047882,
-1.58398514730385));
#164917=CARTESIAN_POINT('Ctrl Pts',(7.26007912546694,0.681246574523941,
-1.58792691115192));
#164918=CARTESIAN_POINT('Ctrl Pts',(7.259214738,0.680609079,-1.591868675));
#164919=CARTESIAN_POINT('Ctrl Pts',(7.257833029,0.679590053000001,-1.598169519));
#164920=CARTESIAN_POINT('Ctrl Pts',(7.256440385,0.678571429,-1.604467956));
#164921=CARTESIAN_POINT('Ctrl Pts',(7.17020797,0.615498301,-1.994466635));
#164922=CARTESIAN_POINT('Ctrl Pts',(7.04267193700001,0.551245526,-2.372976291));
#164923=CARTESIAN_POINT('Ctrl Pts',(7.11867655828793,0.681884070047882,
-1.373683387019));
#164924=CARTESIAN_POINT('Ctrl Pts',(7.11792644914396,0.681246574523941,
-1.3775480240095));
#164925=CARTESIAN_POINT('Ctrl Pts',(7.11717634,0.680609079,-1.381412661));
#164926=CARTESIAN_POINT('Ctrl Pts',(7.115977303,0.679590053000001,-1.387590219));
#164927=CARTESIAN_POINT('Ctrl Pts',(7.114767544,0.678571429,-1.393765687));
#164928=CARTESIAN_POINT('Ctrl Pts',(7.03985936,0.615498301,-1.776150134));
#164929=CARTESIAN_POINT('Ctrl Pts',(6.92439842400001,0.551245526,-2.148303159));
#164930=CARTESIAN_POINT('',(6.9258009809809,0.552026825996016,-2.14377722029232));
#164931=CARTESIAN_POINT('Origin',(-0.174220359436987,0.411147148048371,
0.0783391005764139));
#164932=CARTESIAN_POINT('Origin',(9.02742321671478,0.300018637696928,-2.58584182573121));
#164933=CARTESIAN_POINT('Ctrl Pts',(7.151703794,0.551266351,-2.020736828));
#164934=CARTESIAN_POINT('Ctrl Pts',(7.04162844100001,0.615380951,-2.410310724));
#164935=CARTESIAN_POINT('Ctrl Pts',(6.889887551,0.680609079,-2.785622735));
#164936=CARTESIAN_POINT('Ctrl Pts',(6.8883658974361,0.681263184913293,-2.78938635375241));
#164937=CARTESIAN_POINT('Ctrl Pts',(6.88684424387221,0.681917290826587,
-2.79314997250481));
#164938=CARTESIAN_POINT('Ctrl Pts',(6.92718343146799,0.551266351,-2.13930282854591));
#164939=CARTESIAN_POINT('Ctrl Pts',(6.81064944691794,0.615380951,-2.5166464539081));
#164940=CARTESIAN_POINT('Ctrl Pts',(6.65381663525581,0.680609079,-2.87909900209931));
#164941=CARTESIAN_POINT('Ctrl Pts',(6.65224392003843,0.681263184913293,
-2.88273366650452));
#164942=CARTESIAN_POINT('Ctrl Pts',(6.65067120482106,0.681917290826587,
-2.88636833090973));
#164943=CARTESIAN_POINT('Origin',(-0.167571881686693,0.803452753912076,
0.0947052645359447));
#164944=CARTESIAN_POINT('Ctrl Pts',(6.7506767050316,0.681884070047882,-3.10784067502777));
#164945=CARTESIAN_POINT('Ctrl Pts',(6.7489851635158,0.681246574523941,-3.11150446601388));
#164946=CARTESIAN_POINT('Ctrl Pts',(6.747293622,0.680609079,-3.115168257));
#164947=CARTESIAN_POINT('Ctrl Pts',(6.744589721,0.679590053000001,-3.121024766));
#164948=CARTESIAN_POINT('Ctrl Pts',(6.741875659,0.678571429,-3.126876571));
#164949=CARTESIAN_POINT('Ctrl Pts',(6.573821121,0.615498301,-3.489219877));
#164950=CARTESIAN_POINT('Ctrl Pts',(6.367898423,0.551245526,-3.831463711));
#164951=CARTESIAN_POINT('Ctrl Pts',(6.65694453501887,0.681884070047882,
-2.87187246525371));
#164952=CARTESIAN_POINT('Ctrl Pts',(6.65538118000943,0.681246574523941,
-2.87548549812686));
#164953=CARTESIAN_POINT('Ctrl Pts',(6.653817825,0.680609079,-2.879098531));
#164954=CARTESIAN_POINT('Ctrl Pts',(6.651318828,0.679590053000001,-2.884873904));
#164955=CARTESIAN_POINT('Ctrl Pts',(6.64880981,0.678571429,-2.890644931));
#164956=CARTESIAN_POINT('Ctrl Pts',(6.49345158400001,0.615498301,-3.247986396));
#164957=CARTESIAN_POINT('Ctrl Pts',(6.300688161,0.551245526,-3.586618002));
#164958=CARTESIAN_POINT('',(6.3030308701282,0.552026825948882,-3.58249938561785));
#164959=CARTESIAN_POINT('Origin',(-0.15330670644422,0.411147129612742,0.113959870939336));
#164960=CARTESIAN_POINT('Origin',(8.26029530834744,0.300041800905005,-4.46592127356874));
#164961=CARTESIAN_POINT('Ctrl Pts',(6.550102248,0.551266351,-3.510898037));
#164962=CARTESIAN_POINT('Ctrl Pts',(6.358853524,0.615380951,-3.867700964));
#164963=CARTESIAN_POINT('Ctrl Pts',(6.129979263,0.680609079,-4.201618583));
#164964=CARTESIAN_POINT('Ctrl Pts',(6.1276841180662,0.681263184913293,-4.20496709990272));
#164965=CARTESIAN_POINT('Ctrl Pts',(6.12538897313239,0.681917290826587,
-4.20831561680543));
#164966=CARTESIAN_POINT('Ctrl Pts',(6.30534286154812,0.551266351,-3.57842678930755));
#164967=CARTESIAN_POINT('Ctrl Pts',(6.11041565201059,0.615380951,-3.92189696811787));
#164968=CARTESIAN_POINT('Ctrl Pts',(5.87933291988112,0.680609079,-4.24216115831215));
#164969=CARTESIAN_POINT('Ctrl Pts',(5.87701562845822,0.681263184913293,
-4.24537275899801));
#164970=CARTESIAN_POINT('Ctrl Pts',(5.87469833703533,0.681917290826587,
-4.24858435968387));
#164971=CARTESIAN_POINT('Origin',(-0.143295177047,0.803452728353365,0.128514024721328));
#164972=CARTESIAN_POINT('Ctrl Pts',(5.92475575618306,0.681884070047882,
-4.48637703227967));
#164973=CARTESIAN_POINT('Ctrl Pts',(5.92231615559153,0.681246574523941,
-4.48959153363984));
#164974=CARTESIAN_POINT('Ctrl Pts',(5.91987655500001,0.680609079,-4.492806035));
#164975=CARTESIAN_POINT('Ctrl Pts',(5.915976894,0.679590053000001,-4.497944362));
#164976=CARTESIAN_POINT('Ctrl Pts',(5.912068319,0.678571429,-4.503075913));
#164977=CARTESIAN_POINT('Ctrl Pts',(5.670049703,0.615498301,-4.820821076));
#164978=CARTESIAN_POINT('Ctrl Pts',(5.395369056,0.551245526,-5.11079614500001));
#164979=CARTESIAN_POINT('Ctrl Pts',(5.88394118241646,0.681884070047882,
-4.23577597926324));
#164980=CARTESIAN_POINT('Ctrl Pts',(5.88163768270823,0.681246574523941,
-4.23896846663162));
#164981=CARTESIAN_POINT('Ctrl Pts',(5.879334183,0.680609079,-4.242160954));
#164982=CARTESIAN_POINT('Ctrl Pts',(5.875652077,0.679590053000001,-4.247264092));
#164983=CARTESIAN_POINT('Ctrl Pts',(5.871961118,0.678571429,-4.25236083));
#164984=CARTESIAN_POINT('Ctrl Pts',(5.643417229,0.615498301,-4.567950425));
#164985=CARTESIAN_POINT('Ctrl Pts',(5.382364723,0.551245526,-4.857226574));
#164986=CARTESIAN_POINT('',(5.38553804102176,0.552026825913963,-4.85370786181476));
#164987=CARTESIAN_POINT('Origin',(-0.125224422707866,0.411147099587523,
0.144251912085741));
#164988=CARTESIAN_POINT('Origin',(7.1061891438417,0.300134040132493,-6.13650682902755));
#164989=CARTESIAN_POINT('Ctrl Pts',(5.642225201,0.551266351,-4.836893556));
#164990=CARTESIAN_POINT('Ctrl Pts',(5.378745684,0.615380951,-5.144241806));
#164991=CARTESIAN_POINT('Ctrl Pts',(5.083439958,0.680609079,-5.42115141600001));
#164992=CARTESIAN_POINT('Ctrl Pts',(5.08047864012183,0.681263184913293,
-5.42392825812168));
#164993=CARTESIAN_POINT('Ctrl Pts',(5.07751732224366,0.681917290826586,
-5.42670510024335));
#164994=CARTESIAN_POINT('Ctrl Pts',(5.388672745,0.551266351,-4.850227423));
#164995=CARTESIAN_POINT('Ctrl Pts',(5.124466893,0.615380951,-5.143763941));
#164996=CARTESIAN_POINT('Ctrl Pts',(4.829939409,0.680609079,-5.406864646));
#164997=CARTESIAN_POINT('Ctrl Pts',(4.82698589531167,0.681263184913293,
-5.40950301279373));
#164998=CARTESIAN_POINT('Ctrl Pts',(4.82403238162335,0.681917290826586,
-5.41214137958745));
#164999=CARTESIAN_POINT('Origin',(-0.112320525602429,0.80345250370582,0.156315845870442));
#165000=CARTESIAN_POINT('Ctrl Pts',(4.82179981207758,0.681884070047881,
-5.65513538147594));
#165001=CARTESIAN_POINT('Ctrl Pts',(4.81872622553879,0.681246574523941,
-5.65775028823797));
#165002=CARTESIAN_POINT('Ctrl Pts',(4.815652639,0.680609079,-5.660365195));
#165003=CARTESIAN_POINT('Ctrl Pts',(4.810739562,0.679590053000001,-5.66454508000001));
#165004=CARTESIAN_POINT('Ctrl Pts',(4.805819236,0.678571429,-5.668716429));
#165005=CARTESIAN_POINT('Ctrl Pts',(4.501153063,0.615498301,-5.927006039));
#165006=CARTESIAN_POINT('Ctrl Pts',(4.170558228,0.551245526,-6.15115343300001));
#165007=CARTESIAN_POINT('Ctrl Pts',(4.8358112798721,0.681884070047881,-5.40161931776974));
#165008=CARTESIAN_POINT('Ctrl Pts',(4.83287534443605,0.681246574523941,
-5.40424198188487));
#165009=CARTESIAN_POINT('Ctrl Pts',(4.829939409,0.680609079,-5.406864646));
#165010=CARTESIAN_POINT('Ctrl Pts',(4.825246365,0.679590053000001,-5.411056931));
#165011=CARTESIAN_POINT('Ctrl Pts',(4.82054605,0.678571429,-5.415241063));
#165012=CARTESIAN_POINT('Ctrl Pts',(4.529502956,0.615498301,-5.674322168));
#165013=CARTESIAN_POINT('Ctrl Pts',(4.212367892,0.551245526,-5.90071663));
#165014=CARTESIAN_POINT('',(4.21622343872244,0.552026825912812,-5.8979623527564));
#165015=CARTESIAN_POINT('Origin',(-0.0912870167708651,0.411147072761699,
0.167799146015306));
#165016=CARTESIAN_POINT('Origin',(5.62149350149955,0.300042050105536,-7.521392327659));
#165017=CARTESIAN_POINT('Ctrl Pts',(4.470523974,0.551266351,-5.936721307));
#165018=CARTESIAN_POINT('Ctrl Pts',(4.147133673,0.615380951,-6.180243619));
#165019=CARTESIAN_POINT('Ctrl Pts',(3.799204651,0.680609079,-6.387197234));
#165020=CARTESIAN_POINT('Ctrl Pts',(3.79571562812483,0.681263184913293,
-6.38927255928527));
#165021=CARTESIAN_POINT('Ctrl Pts',(3.79222660524966,0.681917290826586,
-6.39134788457053));
#165022=CARTESIAN_POINT('Ctrl Pts',(4.22003178354831,0.551266351,-5.8952369439236));
#165023=CARTESIAN_POINT('Ctrl Pts',(3.8989012549373,0.615380951,-6.12511422415422));
#165024=CARTESIAN_POINT('Ctrl Pts',(3.55470080472887,0.680609079,-6.31874901102887));
#165025=CARTESIAN_POINT('Ctrl Pts',(3.55124917187135,0.681263184913293,
-6.3206907754639));
#165026=CARTESIAN_POINT('Ctrl Pts',(3.54779753901383,0.681917290826586,
-6.32263253989893));
#165027=CARTESIAN_POINT('Origin',(-0.0760896690513591,0.803452726218141,
0.176804437617541));
#165028=CARTESIAN_POINT('Ctrl Pts',(3.49338187026732,0.681884070047882,
-6.55946588747028));
#165029=CARTESIAN_POINT('Ctrl Pts',(3.48981801463366,0.681246574523941,
-6.56135892873514));
#165030=CARTESIAN_POINT('Ctrl Pts',(3.486254159,0.680609079,-6.56325197));
#165031=CARTESIAN_POINT('Ctrl Pts',(3.480557395,0.679590053000001,-6.566277965));
#165032=CARTESIAN_POINT('Ctrl Pts',(3.474855387,0.678571429,-6.569294066));
#165033=CARTESIAN_POINT('Ctrl Pts',(3.121787509,0.615498301,-6.756050787));
#165034=CARTESIAN_POINT('Ctrl Pts',(2.750736733,0.551245526,-6.903889622));
#165035=CARTESIAN_POINT('Ctrl Pts',(3.56156421782437,0.681884070047882,
-6.31488893800863));
#165036=CARTESIAN_POINT('Ctrl Pts',(3.55813312741219,0.681246574523941,
-6.31681914700431));
#165037=CARTESIAN_POINT('Ctrl Pts',(3.554702037,0.680609079,-6.318749356));
#165038=CARTESIAN_POINT('Ctrl Pts',(3.549217496,0.679590053000001,-6.321834763));
#165039=CARTESIAN_POINT('Ctrl Pts',(3.543727607,0.678571429,-6.324910643));
#165040=CARTESIAN_POINT('Ctrl Pts',(3.20379416,0.615498301,-6.515368914));
#165041=CARTESIAN_POINT('Ctrl Pts',(2.84540542,0.551245526,-6.668295734));
#165042=CARTESIAN_POINT('Ctrl Pts',(3.56224604129995,0.681884070047882,
-6.31244316851402));
#165043=CARTESIAN_POINT('Ctrl Pts',(3.55881627853997,0.681246574523941,
-6.31437374918701));
#165044=CARTESIAN_POINT('Ctrl Pts',(3.55538651578,0.680609079,-6.31630432986));
#165045=CARTESIAN_POINT('Ctrl Pts',(3.54990409701,0.679590053000001,-6.31939033098));
#165046=CARTESIAN_POINT('Ctrl Pts',(3.5444163292,0.678571429,-6.32246680877));
#165047=CARTESIAN_POINT('Ctrl Pts',(3.20461422650999,0.615498301,-6.51296209527));
#165048=CARTESIAN_POINT('Ctrl Pts',(2.84635210687,0.551245526,-6.66593979512));
#165049=CARTESIAN_POINT('',(2.84976291824466,0.552026826190771,-6.66643467634339));
#165050=CARTESIAN_POINT('Origin',(-0.0530804187079026,0.411144977216728,
0.183499851431562));
#165051=CARTESIAN_POINT('Ctrl Pts',(2.87375705931618,0.56205338059825,-6.72366306341953));
#165052=CARTESIAN_POINT('Ctrl Pts',(2.86574278438241,0.558751695403869,
-6.70458669100326));
#165053=CARTESIAN_POINT('Ctrl Pts',(2.85774443038173,0.555410033604048,
-6.68551049651921));
#165054=CARTESIAN_POINT('Ctrl Pts',(2.84976292439803,0.552026824750786,
-6.66643467502883));
#165055=CARTESIAN_POINT('Ctrl Pts',(3.089786015,0.551266351,-6.758954569));
#165056=CARTESIAN_POINT('Ctrl Pts',(2.721606301,0.615380951,-6.927264109));
#165057=CARTESIAN_POINT('Ctrl Pts',(2.337322756,0.680609079,-7.054584809));
#165058=CARTESIAN_POINT('Ctrl Pts',(2.33346917094593,0.681263184913293,
-7.05586157755535));
#165059=CARTESIAN_POINT('Ctrl Pts',(2.32961558589186,0.681917290826586,
-7.0571383461107));
#165060=CARTESIAN_POINT('Ctrl Pts',(2.854069293,0.551266351,-6.664592146));
#165061=CARTESIAN_POINT('Ctrl Pts',(2.491029771,0.615380951,-6.82006151700001));
#165062=CARTESIAN_POINT('Ctrl Pts',(2.113250748,0.680609079,-6.93517637));
#165063=CARTESIAN_POINT('Ctrl Pts',(2.10946239011761,0.681263184913293,
-6.93633073864991));
#165064=CARTESIAN_POINT('Ctrl Pts',(2.10567403223522,0.681917290826586,
-6.93748510729981));
#165065=CARTESIAN_POINT('Origin',(-0.0363040560098285,0.803453434253933,
0.189031072590716));
#165066=CARTESIAN_POINT('Ctrl Pts',(2.00161727379074,0.681884070047882,
-7.15708305927178));
#165067=CARTESIAN_POINT('Ctrl Pts',(1.99772979139537,0.681246574523941,
-7.15816571863589));
#165068=CARTESIAN_POINT('Ctrl Pts',(1.993842309,0.680609079,-7.159248378));
#165069=CARTESIAN_POINT('Ctrl Pts',(1.987628233,0.679590053000001,-7.160978991));
#165070=CARTESIAN_POINT('Ctrl Pts',(1.981411162,0.678571429,-7.162698814));
#165071=CARTESIAN_POINT('Ctrl Pts',(1.59645064,0.615498301,-7.269190109));
#165072=CARTESIAN_POINT('Ctrl Pts',(1.202293846,0.551245526,-7.33380760600001));
#165073=CARTESIAN_POINT('Ctrl Pts',(2.12078237088003,0.681884070047882,
-6.93288137335172));
#165074=CARTESIAN_POINT('Ctrl Pts',(2.11701655944001,0.681246574523941,
-6.93402887167586));
#165075=CARTESIAN_POINT('Ctrl Pts',(2.113250748,0.680609079,-6.93517637));
#165076=CARTESIAN_POINT('Ctrl Pts',(2.107231161,0.679590053000001,-6.937010627));
#165077=CARTESIAN_POINT('Ctrl Pts',(2.1012084,0.678571429,-6.938834431));
#165078=CARTESIAN_POINT('Ctrl Pts',(1.728279509,0.615498301,-7.05176425));
#165079=CARTESIAN_POINT('Ctrl Pts',(1.345394953,0.551245526,-7.124072741));
#165080=CARTESIAN_POINT('',(1.35005064349767,0.552026825956876,-7.1231919291517));
#165081=CARTESIAN_POINT('Origin',(-0.0123928583365629,0.411147082466218,
0.190621017475019));
#165082=CARTESIAN_POINT('Origin',(1.94357642212787,0.300127903713799,-9.18589156190818));
#165083=CARTESIAN_POINT('Ctrl Pts',(1.564573096,0.551266351,-7.265146627));
#165084=CARTESIAN_POINT('Ctrl Pts',(1.168819643,0.615380951,-7.350373428));
#165085=CARTESIAN_POINT('Ctrl Pts',(0.766150247,0.680609079,-7.392107838));
#165086=CARTESIAN_POINT('Ctrl Pts',(0.762112289126585,0.681263184913293,
-7.39252634954104));
#165087=CARTESIAN_POINT('Ctrl Pts',(0.758074331253171,0.681917290826587,
-7.39294486108209));
#165088=CARTESIAN_POINT('Ctrl Pts',(1.35465137544855,0.551266351,-7.1223174988109));
#165089=CARTESIAN_POINT('Ctrl Pts',(0.966678236570384,0.615380951,-7.19610925931197));
#165090=CARTESIAN_POINT('Ctrl Pts',(0.572985231706459,0.680609079,-7.22732141540281));
#165091=CARTESIAN_POINT('Ctrl Pts',(0.56903728884194,0.681263184913293,
-7.22763441006465));
#165092=CARTESIAN_POINT('Ctrl Pts',(0.56508934597742,0.681917290826587,
-7.22794740472649));
#165093=CARTESIAN_POINT('Origin',(0.0051808062341413,0.803453412729377,
0.192415877054507));
#165094=CARTESIAN_POINT('Ctrl Pts',(0.416259277961287,0.681884070047882,
-7.42004298029424));
#165095=CARTESIAN_POINT('Ctrl Pts',(0.412229942980644,0.681246574523941,
-7.42026463414712));
#165096=CARTESIAN_POINT('Ctrl Pts',(0.408200608,0.680609079,-7.420486288));
#165097=CARTESIAN_POINT('Ctrl Pts',(0.401759783,0.679590053000001,-7.420840598));
#165098=CARTESIAN_POINT('Ctrl Pts',(0.395318353,0.678571429,-7.421183725));
#165099=CARTESIAN_POINT('Ctrl Pts',(-0.003534487,0.615498301,-7.442430181));
#165100=CARTESIAN_POINT('Ctrl Pts',(-0.402366966,0.551245526,-7.420804897));
#165101=CARTESIAN_POINT('Ctrl Pts',(0.580835096616944,0.681884070047882,
-7.22669998041423));
#165102=CARTESIAN_POINT('Ctrl Pts',(0.576910649808472,0.681246574523941,
-7.22701111220711));
#165103=CARTESIAN_POINT('Ctrl Pts',(0.572986203,0.680609079,-7.227322244));
#165104=CARTESIAN_POINT('Ctrl Pts',(0.56671304,0.679590053000001,-7.227819583));
#165105=CARTESIAN_POINT('Ctrl Pts',(0.560439023,0.678571429,-7.228306033));
#165106=CARTESIAN_POINT('Ctrl Pts',(0.17195243,0.615498301,-7.258426928));
#165107=CARTESIAN_POINT('Ctrl Pts',(-0.217524687,0.551245526,-7.246736025));
#165108=CARTESIAN_POINT('',(-0.212788494622047,0.552026825910877,-7.24687664144778));
#165109=CARTESIAN_POINT('Origin',(0.0288747599038717,0.411147101591151,
0.188828232147965));
#165110=CARTESIAN_POINT('Origin',(-0.0764596409031881,0.29994988413586,
-9.39079447355658));
#165111=CARTESIAN_POINT('Ctrl Pts',(-0.033797522,0.551266351,-7.431628504));
#165112=CARTESIAN_POINT('Ctrl Pts',(-0.438619722,0.615380951,-7.429787455));
#165113=CARTESIAN_POINT('Ctrl Pts',(-0.840846596,0.680609079,-7.38398412));
#165114=CARTESIAN_POINT('Ctrl Pts',(-0.8448801162747,0.681263184913293,
-7.38352480538849));
#165115=CARTESIAN_POINT('Ctrl Pts',(-0.848913636549401,0.681917290826586,
-7.38306549077698));
#165116=CARTESIAN_POINT('Ctrl Pts',(-0.208106472,0.551266351,-7.247012605));
#165117=CARTESIAN_POINT('Ctrl Pts',(-0.602872113,0.615380951,-7.23567644600001));
#165118=CARTESIAN_POINT('Ctrl Pts',(-0.994070541,0.680609079,-7.181526562));
#165119=CARTESIAN_POINT('Ctrl Pts',(-0.997993468314819,0.681263184913293,
-7.1809835484196));
#165120=CARTESIAN_POINT('Ctrl Pts',(-1.00191639562964,0.681917290826586,
-7.18044053483919));
#165121=CARTESIAN_POINT('Origin',(0.0464232560277618,0.803452544100388,
0.186803320626479));
#165122=CARTESIAN_POINT('Ctrl Pts',(-1.18856253854604,0.681884070047882,
-7.33604993996607));
#165123=CARTESIAN_POINT('Ctrl Pts',(-1.19254531877302,0.681246574523941,
-7.33540022348304));
#165124=CARTESIAN_POINT('Ctrl Pts',(-1.196528099,0.680609079,-7.334750507));
#165125=CARTESIAN_POINT('Ctrl Pts',(-1.202894507,0.679590053000001,-7.333711946));
#165126=CARTESIAN_POINT('Ctrl Pts',(-1.209259103,0.678571429,-7.332662334));
#165127=CARTESIAN_POINT('Ctrl Pts',(-1.603354344,0.615498301,-7.267670489));
#165128=CARTESIAN_POINT('Ctrl Pts',(-1.988213545,0.551245526,-7.160813598));
#165129=CARTESIAN_POINT('Ctrl Pts',(-0.986271382025895,0.681884070047882,
-7.18260612530439));
#165130=CARTESIAN_POINT('Ctrl Pts',(-0.990170961512947,0.681246574523941,
-7.18206634365219));
#165131=CARTESIAN_POINT('Ctrl Pts',(-0.994070541000001,0.680609079,-7.18152656200001));
#165132=CARTESIAN_POINT('Ctrl Pts',(-1.000303954,0.679590053000001,-7.18066373));
#165133=CARTESIAN_POINT('Ctrl Pts',(-1.00653586,0.678571429,-7.179790078));
#165134=CARTESIAN_POINT('Ctrl Pts',(-1.392414954,0.615498301,-7.125693629));
#165135=CARTESIAN_POINT('Ctrl Pts',(-1.770273114,0.551245526,-7.030549986));
#165136=CARTESIAN_POINT('Ctrl Pts',(-0.984248470460693,0.681884070047882,
-7.18107168715778));
#165137=CARTESIAN_POINT('Ctrl Pts',(-0.988147217940346,0.681246574523941,
-7.18053300485388));
#165138=CARTESIAN_POINT('Ctrl Pts',(-0.99204596542,0.680609079,-7.17999432255));
#165139=CARTESIAN_POINT('Ctrl Pts',(-0.998278048469998,0.679590053000001,
-7.17913324784));
#165140=CARTESIAN_POINT('Ctrl Pts',(-1.00450862757,0.678571429,-7.17826135544));
#165141=CARTESIAN_POINT('Ctrl Pts',(-1.3903055601,0.615498301,-7.1242738604));
#165142=CARTESIAN_POINT('Ctrl Pts',(-1.76809370969,0.551245526,-7.02924734988));
#165143=CARTESIAN_POINT('',(-1.76567787734294,0.55202682618642,-7.03170545575127));
#165144=CARTESIAN_POINT('Origin',(0.0687923889553491,0.411145011062635,
0.178205687137017));
#165145=CARTESIAN_POINT('Ctrl Pts',(-1.78120945030309,0.562053380603981,
-7.09178521393521));
#165146=CARTESIAN_POINT('Ctrl Pts',(-1.77604503026779,0.558751695424193,
-7.07174861365702));
#165147=CARTESIAN_POINT('Ctrl Pts',(-1.77086804335904,0.555410033626249,
-7.0517217898627));
#165148=CARTESIAN_POINT('Ctrl Pts',(-1.7656778697302,0.552026824831871,
-7.03170545921814));
#165149=CARTESIAN_POINT('Ctrl Pts',(-1.630587806,0.551266351,-7.250615691));
#165150=CARTESIAN_POINT('Ctrl Pts',(-2.025549717,0.615380951,-7.16179287900001));
#165151=CARTESIAN_POINT('Ctrl Pts',(-2.408526387,0.680609079,-7.030593512));
#165152=CARTESIAN_POINT('Ctrl Pts',(-2.41236686674672,0.681263184913293,
-7.02927784827629));
#165153=CARTESIAN_POINT('Ctrl Pts',(-2.41620734649343,0.681917290826587,
-7.02796218455258));
#165154=CARTESIAN_POINT('Ctrl Pts',(-1.761134548,0.551266351,-7.032844738));
#165155=CARTESIAN_POINT('Ctrl Pts',(-2.144233849,0.615380951,-6.936910668));
#165156=CARTESIAN_POINT('Ctrl Pts',(-2.51464565,0.680609079,-6.79993068));
#165157=CARTESIAN_POINT('Ctrl Pts',(-2.51836012957832,0.681263184913293,
-6.79855704836437));
#165158=CARTESIAN_POINT('Ctrl Pts',(-2.52207460915663,0.681917290826587,
-6.79718341672875));
#165159=CARTESIAN_POINT('Origin',(0.0854953302183697,0.803453457522902,
0.172456584285718));
#165160=CARTESIAN_POINT('Ctrl Pts',(-2.73780849035282,0.681884070047882,
-6.90903135754418));
#165161=CARTESIAN_POINT('Ctrl Pts',(-2.74155848617641,0.681246574523941,
-6.90754065077208));
#165162=CARTESIAN_POINT('Ctrl Pts',(-2.745308482,0.680609079,-6.906049944));
#165163=CARTESIAN_POINT('Ctrl Pts',(-2.751302788,0.679590053000001,-6.903667074));
#165164=CARTESIAN_POINT('Ctrl Pts',(-2.757292947,0.678571429,-6.901273802));
#165165=CARTESIAN_POINT('Ctrl Pts',(-3.128203135,0.615498301,-6.753082602));
#165166=CARTESIAN_POINT('Ctrl Pts',(-3.481093468,0.551245526,-6.565990615));
#165167=CARTESIAN_POINT('Ctrl Pts',(-2.50726090509375,0.681884070047882,
-6.80266159234725));
#165168=CARTESIAN_POINT('Ctrl Pts',(-2.51095327754687,0.681246574523941,
-6.80129613617363));
#165169=CARTESIAN_POINT('Ctrl Pts',(-2.51464565,0.680609079,-6.79993068000001));
#165170=CARTESIAN_POINT('Ctrl Pts',(-2.520547846,0.679590053000001,-6.797748021));
#165171=CARTESIAN_POINT('Ctrl Pts',(-2.526446244,0.678571429,-6.795555119));
#165172=CARTESIAN_POINT('Ctrl Pts',(-2.891674563,0.615498301,-6.659770816));
#165173=CARTESIAN_POINT('Ctrl Pts',(-3.240245538,0.551245526,-6.485623243));
#165174=CARTESIAN_POINT('',(-3.23600612945469,0.552026825943996,-6.48773953932139));
#165175=CARTESIAN_POINT('Origin',(0.10549294900999,0.411147121408226,0.159251690106229));
#165176=CARTESIAN_POINT('Origin',(-4.01239744936829,0.29999615904035,-8.49054704910549));
#165177=CARTESIAN_POINT('Ctrl Pts',(-3.151133616,0.551266351,-6.730572147));
#165178=CARTESIAN_POINT('Ctrl Pts',(-3.517767258,0.615380951,-6.558920827));
#165179=CARTESIAN_POINT('Ctrl Pts',(-3.86358616,0.680609079,-6.348460165));
#165180=CARTESIAN_POINT('Ctrl Pts',(-3.86705402264856,0.681263184913293,
-6.34634967114174));
#165181=CARTESIAN_POINT('Ctrl Pts',(-3.87052188529712,0.681917290826587,
-6.34423917728348));
#165182=CARTESIAN_POINT('Ctrl Pts',(-3.231813931,0.551266351,-6.489828867));
#165183=CARTESIAN_POINT('Ctrl Pts',(-3.585333593,0.615380951,-6.313782657));
#165184=CARTESIAN_POINT('Ctrl Pts',(-3.917638724,0.680609079,-6.100377597));
#165185=CARTESIAN_POINT('Ctrl Pts',(-3.92097107091642,0.681263184913293,
-6.09823757679779));
#165186=CARTESIAN_POINT('Ctrl Pts',(-3.92430341783284,0.681917290826586,
-6.09609755659558));
#165187=CARTESIAN_POINT('Origin',(0.120569400091427,0.8034525034028,0.15004570042049));
#165188=CARTESIAN_POINT('Ctrl Pts',(-4.15903756282769,0.681884070047881,
-6.15895414672883));
#165189=CARTESIAN_POINT('Ctrl Pts',(-4.16237942741384,0.681246574523941,
-6.15669215386441));
#165190=CARTESIAN_POINT('Ctrl Pts',(-4.165721292,0.680609079,-6.154430161));
#165191=CARTESIAN_POINT('Ctrl Pts',(-4.171063207,0.679590053000001,-6.150814403));
#165192=CARTESIAN_POINT('Ctrl Pts',(-4.176398838,0.678571429,-6.147189377));
#165193=CARTESIAN_POINT('Ctrl Pts',(-4.506780624,0.615498301,-5.922728079));
#165194=CARTESIAN_POINT('Ctrl Pts',(-4.811201331,0.551245526,-5.664149207));
#165195=CARTESIAN_POINT('Ctrl Pts',(-3.91101369546929,0.681884070047881,
-6.10463216359984));
#165196=CARTESIAN_POINT('Ctrl Pts',(-3.91432620973464,0.681246574523941,
-6.10250488029992));
#165197=CARTESIAN_POINT('Ctrl Pts',(-3.917638724,0.680609079,-6.100377597));
#165198=CARTESIAN_POINT('Ctrl Pts',(-3.922933723,0.679590053000001,-6.09697717));
#165199=CARTESIAN_POINT('Ctrl Pts',(-3.928222811,0.678571429,-6.093567555));
#165200=CARTESIAN_POINT('Ctrl Pts',(-4.255722683,0.615498301,-5.882444522));
#165201=CARTESIAN_POINT('Ctrl Pts',(-4.558707681,0.551245526,-5.637435967));
#165202=CARTESIAN_POINT('Ctrl Pts',(-3.9085334567957,0.681884070047881,
-6.10408894376855));
#165203=CARTESIAN_POINT('Ctrl Pts',(-3.91184567755785,0.681246574523941,
-6.10196300756427));
#165204=CARTESIAN_POINT('Ctrl Pts',(-3.91515789832,0.680609079,-6.09983707136001));
#165205=CARTESIAN_POINT('Ctrl Pts',(-3.92045242816,0.679590053000001,-6.09643879767));
#165206=CARTESIAN_POINT('Ctrl Pts',(-3.92574105073,0.678571429,-6.09303133678));
#165207=CARTESIAN_POINT('Ctrl Pts',(-4.25321210359,0.615498301,-5.88204168643001));
#165208=CARTESIAN_POINT('Ctrl Pts',(-4.55618274449999,0.551245526,-5.6371688346));
#165209=CARTESIAN_POINT('',(-4.55502232513917,0.552026826178051,-5.64041413373297));
#165210=CARTESIAN_POINT('Origin',(0.137260940792053,0.411144919528123,0.132849950390427));
#165211=CARTESIAN_POINT('Ctrl Pts',(-4.59434523690511,0.562053380745924,
-5.68841950546675));
#165212=CARTESIAN_POINT('Ctrl Pts',(-4.58124498540839,0.558751695407189,
-5.67240326384358));
#165213=CARTESIAN_POINT('Ctrl Pts',(-4.56813743426761,0.555410033596466,
-5.65640117123746));
#165214=CARTESIAN_POINT('Ctrl Pts',(-4.55502232113666,0.552026824779272,
-5.64041413851911));
#165215=CARTESIAN_POINT('Ctrl Pts',(-4.52433592,0.551266351,-5.89581453));
#165216=CARTESIAN_POINT('Ctrl Pts',(-4.845497912,0.615380951,-5.649360927));
#165217=CARTESIAN_POINT('Ctrl Pts',(-5.13798893900001,0.680609079,-5.369479877));
#165218=CARTESIAN_POINT('Ctrl Pts',(-5.1409220311523,0.681263184913293,
-5.36667323735792));
#165219=CARTESIAN_POINT('Ctrl Pts',(-5.1438551233046,0.681917290826586,
-5.36386659771584));
#165220=CARTESIAN_POINT('Ctrl Pts',(-4.551377285,0.551266351,-5.643355811));
#165221=CARTESIAN_POINT('Ctrl Pts',(-4.858787124,0.615380951,-5.395429187));
#165222=CARTESIAN_POINT('Ctrl Pts',(-5.137447365,0.680609079,-5.115577638));
#165223=CARTESIAN_POINT('Ctrl Pts',(-5.14024176240226,0.681263184913293,
-5.11277129419315));
#165224=CARTESIAN_POINT('Ctrl Pts',(-5.14303615980453,0.681917290826586,
-5.10996495038631));
#165225=CARTESIAN_POINT('Origin',(0.150005998797879,0.803453479443192,0.120618687140587));
#165226=CARTESIAN_POINT('Ctrl Pts',(-5.3857946597887,0.681884070047877,
-5.12089108640163));
#165227=CARTESIAN_POINT('Ctrl Pts',(-5.38857213189434,0.681246574523938,
-5.11796357520081));
#165228=CARTESIAN_POINT('Ctrl Pts',(-5.39134960400001,0.680609079,-5.115036064));
#165229=CARTESIAN_POINT('Ctrl Pts',(-5.395789347,0.679590053,-5.11035648600001));
#165230=CARTESIAN_POINT('Ctrl Pts',(-5.40022096,0.678571429,-5.105669209));
#165231=CARTESIAN_POINT('Ctrl Pts',(-5.67462606,0.615498301,-4.815433373));
#165232=CARTESIAN_POINT('Ctrl Pts',(-5.916342766,0.551245526,-4.497458479));
#165233=CARTESIAN_POINT('Ctrl Pts',(-5.13189183273128,0.681884070047877,
-5.12115692153225));
#165234=CARTESIAN_POINT('Ctrl Pts',(-5.13466959886564,0.681246574523938,
-5.11836727976612));
#165235=CARTESIAN_POINT('Ctrl Pts',(-5.137447365,0.680609079,-5.115577638));
#165236=CARTESIAN_POINT('Ctrl Pts',(-5.141887578,0.679590053,-5.111118442));
#165237=CARTESIAN_POINT('Ctrl Pts',(-5.146320044,0.678571429,-5.106651545));
#165238=CARTESIAN_POINT('Ctrl Pts',(-5.42077794,0.615498301,-4.830061659));
#165239=CARTESIAN_POINT('Ctrl Pts',(-5.66400972,0.551245526,-4.525648449));
#165240=CARTESIAN_POINT('',(-5.6610507458468,0.552026825822157,-4.52934923041454));
#165241=CARTESIAN_POINT('Origin',(0.162610771491941,0.411147080989508,0.100237490144345));
#165242=CARTESIAN_POINT('Origin',(-7.20657778905468,0.300004052182154,-6.02097698757969));
#165243=CARTESIAN_POINT('Ctrl Pts',(-5.685985305,0.551266351,-4.785375178));
#165244=CARTESIAN_POINT('Ctrl Pts',(-5.946658468,0.615380951,-4.475643188));
#165245=CARTESIAN_POINT('Ctrl Pts',(-6.172145066,0.680609079,-4.139428677));
#165246=CARTESIAN_POINT('Ctrl Pts',(-6.17440623954035,0.681263184913293,
-4.13605712692608));
#165247=CARTESIAN_POINT('Ctrl Pts',(-6.1766674130807,0.681917290826586,
-4.13268557685216));
#165248=CARTESIAN_POINT('Ctrl Pts',(-5.65812315589465,0.551266351,-4.53300444094894));
#165249=CARTESIAN_POINT('Ctrl Pts',(-5.9050489587658,0.615380951,-4.22479018258088));
#165250=CARTESIAN_POINT('Ctrl Pts',(-6.11703440087497,0.680609079,-3.89157770767668));
#165251=CARTESIAN_POINT('Ctrl Pts',(-6.11916018518716,0.681263184913293,
-3.88823626193999));
#165252=CARTESIAN_POINT('Ctrl Pts',(-6.12128596949935,0.681917290826586,
-3.8848948162033));
#165253=CARTESIAN_POINT('Origin',(0.172428499853304,0.803453447950604,0.0855519229008006));
#165254=CARTESIAN_POINT('Ctrl Pts',(-6.36071798545744,0.681884070047877,
-3.84338084831586));
#165255=CARTESIAN_POINT('Ctrl Pts',(-6.36280119322872,0.681246574523938,
-3.83992470665794));
#165256=CARTESIAN_POINT('Ctrl Pts',(-6.364884401,0.680609079,-3.836468565));
#165257=CARTESIAN_POINT('Ctrl Pts',(-6.368214374,0.679590053,-3.83094398));
#165258=CARTESIAN_POINT('Ctrl Pts',(-6.371534752,0.678571429,-3.825413623));
#165259=CARTESIAN_POINT('Ctrl Pts',(-6.577132288,0.615498301,-3.482974354));
#165260=CARTESIAN_POINT('Ctrl Pts',(-6.744842588,0.551245526,-3.12047159));
#165261=CARTESIAN_POINT('Ctrl Pts',(-6.11280841197592,0.681884070047877,
-3.89822207217764));
#165262=CARTESIAN_POINT('Ctrl Pts',(-6.11492154498796,0.681246574523938,
-3.89490051308882));
#165263=CARTESIAN_POINT('Ctrl Pts',(-6.117034678,0.680609079,-3.891578954));
#165264=CARTESIAN_POINT('Ctrl Pts',(-6.120412486,0.679590053,-3.886269497));
#165265=CARTESIAN_POINT('Ctrl Pts',(-6.123781072,0.678571429,-3.880954185));
#165266=CARTESIAN_POINT('Ctrl Pts',(-6.332363645,0.615498301,-3.551830482));
#165267=CARTESIAN_POINT('Ctrl Pts',(-6.50446896,0.551245526,-3.202246641));
#165268=CARTESIAN_POINT('',(-6.5023747244165,0.552026825926503,-3.2064969894312));
#165269=CARTESIAN_POINT('Origin',(0.180357310691638,0.411147121182753,0.0629375996474091));
#165270=CARTESIAN_POINT('Origin',(-8.33121035929084,0.300112759031273,-4.33028420864262));
#165271=CARTESIAN_POINT('Ctrl Pts',(-6.581764337,0.551266351,-3.451177002));
#165272=CARTESIAN_POINT('Ctrl Pts',(-6.769759885,0.615380951,-3.092649349));
#165273=CARTESIAN_POINT('Ctrl Pts',(-6.917698549,0.680609079,-2.715822393));
#165274=CARTESIAN_POINT('Ctrl Pts',(-6.91918207394382,0.681263184913293,
-2.71204358241988));
#165275=CARTESIAN_POINT('Ctrl Pts',(-6.92066559888766,0.681917290826586,
-2.70826477183976));
#165276=CARTESIAN_POINT('Ctrl Pts',(-6.50030134042989,0.551266351,-3.21069608698621));
#165277=CARTESIAN_POINT('Ctrl Pts',(-6.675197199408,0.615380951,-2.85660595835115));
#165278=CARTESIAN_POINT('Ctrl Pts',(-6.81059570720614,0.680609079,-2.48561320275527));
#165279=CARTESIAN_POINT('Ctrl Pts',(-6.81195347980084,0.681263184913293,
-2.48189289737989));
#165280=CARTESIAN_POINT('Ctrl Pts',(-6.81331125239553,0.681917290826586,
-2.47817259200452));
#165281=CARTESIAN_POINT('Origin',(0.186785362021775,0.803452743019938,0.0464835788768353));
#165282=CARTESIAN_POINT('Ctrl Pts',(-7.03822120603974,0.681884070047877,
-2.38615839511332));
#165283=CARTESIAN_POINT('Ctrl Pts',(-7.03951274151987,0.681246574523938,
-2.38233522805666));
#165284=CARTESIAN_POINT('Ctrl Pts',(-7.040804277,0.680609079,-2.378512061));
#165285=CARTESIAN_POINT('Ctrl Pts',(-7.042868775,0.679590053,-2.372400792));
#165286=CARTESIAN_POINT('Ctrl Pts',(-7.044922661,0.678571429,-2.366285948));
#165287=CARTESIAN_POINT('Ctrl Pts',(-7.17209912,0.615498301,-1.987655326));
#165288=CARTESIAN_POINT('Ctrl Pts',(-7.257961068,0.551245526,-1.597574918));
#165289=CARTESIAN_POINT('Ctrl Pts',(-6.80789686203716,0.681884070047877,
-2.49301069013488));
#165290=CARTESIAN_POINT('Ctrl Pts',(-6.80924655451858,0.681246574523938,
-2.48931252656744));
#165291=CARTESIAN_POINT('Ctrl Pts',(-6.810596247,0.680609079,-2.485614363));
#165292=CARTESIAN_POINT('Ctrl Pts',(-6.81275370800001,0.679590053,-2.47970291));
#165293=CARTESIAN_POINT('Ctrl Pts',(-6.814900903,0.678571429,-2.47378772));
#165294=CARTESIAN_POINT('Ctrl Pts',(-6.947855064,0.615498301,-2.107519659));
#165295=CARTESIAN_POINT('Ctrl Pts',(-7.04078646,0.551245526,-1.729111338));
#165296=CARTESIAN_POINT('Ctrl Pts',(-6.80559361859714,0.681884070047877,
-2.49407921308509));
#165297=CARTESIAN_POINT('Ctrl Pts',(-6.80694389264857,0.681246574523938,
-2.49038229955254));
#165298=CARTESIAN_POINT('Ctrl Pts',(-6.80829416669999,0.680609079,-2.48668538602));
#165299=CARTESIAN_POINT('Ctrl Pts',(-6.81045255733,0.679590053,-2.48077593118));
#165300=CARTESIAN_POINT('Ctrl Pts',(-6.81260068542,0.678571429,-2.47486273772));
#165301=CARTESIAN_POINT('Ctrl Pts',(-6.94561262344,0.615498301,-2.10871830233));
#165302=CARTESIAN_POINT('Ctrl Pts',(-7.03861471392,0.551245526,-1.7304267022));
#165303=CARTESIAN_POINT('',(-7.03965488398797,0.552026826194493,-1.73371251862539));
#165304=CARTESIAN_POINT('Origin',(0.189669970752134,0.411144947754553,0.0226941808511896));
#165305=CARTESIAN_POINT('Ctrl Pts',(-7.10001119453425,0.562053380786607,
-1.74813204994719));
#165306=CARTESIAN_POINT('Ctrl Pts',(-7.07988955854266,0.55875169543278,
-1.74330956532491));
#165307=CARTESIAN_POINT('Ctrl Pts',(-7.05977067420358,0.555410033642667,
-1.73850276224255));
#165308=CARTESIAN_POINT('Ctrl Pts',(-7.0396548836752,0.552026824799611,
-1.7337125249341));
#165309=CARTESIAN_POINT('Ctrl Pts',(-7.169787384,0.551266351,-1.955605624));
#165310=CARTESIAN_POINT('Ctrl Pts',(-7.276314852,0.615380951,-1.565046663));
#165311=CARTESIAN_POINT('Ctrl Pts',(-7.339788137,0.680609079,-1.165227272));
#165312=CARTESIAN_POINT('Ctrl Pts',(-7.34042464539488,0.681263184913293,
-1.16121789390008));
#165313=CARTESIAN_POINT('Ctrl Pts',(-7.34106115378977,0.681917290826586,
-1.15720851580015));
#165314=CARTESIAN_POINT('Ctrl Pts',(-7.03853332,0.551266351,-1.738260252));
#165315=CARTESIAN_POINT('Ctrl Pts',(-7.13322136,0.615380951,-1.354851078));
#165316=CARTESIAN_POINT('Ctrl Pts',(-7.185701905,0.680609079,-0.963425207));
#165317=CARTESIAN_POINT('Ctrl Pts',(-7.18622817849381,0.681263184913293,
-0.959499998892894));
#165318=CARTESIAN_POINT('Ctrl Pts',(-7.18675445198762,0.681917290826586,
-0.955574790785788));
#165319=CARTESIAN_POINT('Origin',(0.192414180828946,0.803453416295806,0.00524397244476754));
#165320=CARTESIAN_POINT('Ctrl Pts',(-7.38662502560974,0.681884070047877,
-0.817361827008927));
#165321=CARTESIAN_POINT('Ctrl Pts',(-7.38706449780487,0.681246574523938,
-0.813350401504463));
#165322=CARTESIAN_POINT('Ctrl Pts',(-7.38750397,0.680609079,-0.809338976000001));
#165323=CARTESIAN_POINT('Ctrl Pts',(-7.388206459,0.679590053,-0.802926779));
#165324=CARTESIAN_POINT('Ctrl Pts',(-7.388897816,0.678571429,-0.796513372));
#165325=CARTESIAN_POINT('Ctrl Pts',(-7.431706569,0.615498301,-0.399395744));
#165326=CARTESIAN_POINT('Ctrl Pts',(-7.431705355,0.551245526,2.2582E-5));
#165327=CARTESIAN_POINT('Ctrl Pts',(-7.18465562199158,0.681884070047877,
-0.971228900272081));
#165328=CARTESIAN_POINT('Ctrl Pts',(-7.18517876349579,0.681246574523938,
-0.967327053636041));
#165329=CARTESIAN_POINT('Ctrl Pts',(-7.185701905,0.680609079,-0.963425207));
#165330=CARTESIAN_POINT('Ctrl Pts',(-7.186538138,0.679590053,-0.95718817));
#165331=CARTESIAN_POINT('Ctrl Pts',(-7.187363542,0.678571429,-0.95094969));
#165332=CARTESIAN_POINT('Ctrl Pts',(-7.238472502,0.615498301,-0.564663559));
#165333=CARTESIAN_POINT('Ctrl Pts',(-7.247884611,0.551245526,-0.175124711));
#165334=CARTESIAN_POINT('Ctrl Pts',(-7.1826359279554,0.681884070047877,
-0.972767571004713));
#165335=CARTESIAN_POINT('Ctrl Pts',(-7.1831599061527,0.681246574523938,
-0.968866820157356));
#165336=CARTESIAN_POINT('Ctrl Pts',(-7.18368388435,0.680609079,-0.96496606931));
#165337=CARTESIAN_POINT('Ctrl Pts',(-7.18452145479,0.679590053,-0.95873078391));
#165338=CARTESIAN_POINT('Ctrl Pts',(-7.18534819926,0.678571429,-0.95249405318));
#165339=CARTESIAN_POINT('Ctrl Pts',(-7.23654016133,0.615498301,-0.56631623715));
#165340=CARTESIAN_POINT('Ctrl Pts',(-7.24604640356,0.551245526,-0.17687618393));
#165341=CARTESIAN_POINT('',(-7.24776860903089,0.552026825761896,-0.179861574595068));
#165342=CARTESIAN_POINT('Origin',(0.19011403374817,0.411144969445827,-0.0186098427601895));
#165343=CARTESIAN_POINT('Ctrl Pts',(-7.30981359466473,0.56205338065316,
-0.180969162687403));
#165344=CARTESIAN_POINT('Ctrl Pts',(-7.28912569973217,0.558751695414249,
-0.180584981340033));
#165345=CARTESIAN_POINT('Ctrl Pts',(-7.26844386309386,0.555410033612152,
-0.180215524115213));
#165346=CARTESIAN_POINT('Ctrl Pts',(-7.24776860924737,0.552026824727703,
-0.1798615806622));
#165347=CARTESIAN_POINT('Ctrl Pts',(-7.422559141,0.551266351,-0.368592301));
#165348=CARTESIAN_POINT('Ctrl Pts',(-7.442637425,0.615380951,0.035735865));
#165349=CARTESIAN_POINT('Ctrl Pts',(-7.418677388,0.680609079,0.439852581));
#165350=CARTESIAN_POINT('Ctrl Pts',(-7.41843711739337,0.681263184913293,
0.44390505255945));
#165351=CARTESIAN_POINT('Ctrl Pts',(-7.41819684678672,0.681917290826586,
0.4479575241189));
#165352=CARTESIAN_POINT('Ctrl Pts',(-7.247650894,0.551266351,-0.184544087));
#165353=CARTESIAN_POINT('Ctrl Pts',(-7.257703542,0.615380951,0.210256324));
#165354=CARTESIAN_POINT('Ctrl Pts',(-7.224812129,0.680609079,0.603812641));
#165355=CARTESIAN_POINT('Ctrl Pts',(-7.22448229479504,0.681263184913293,
0.607759213162297));
#165356=CARTESIAN_POINT('Ctrl Pts',(-7.22415246059009,0.681917290826586,
0.611705785324594));
#165357=CARTESIAN_POINT('Origin',(0.189042798006385,0.803453447834286,-0.0362419934487183));
#165358=CARTESIAN_POINT('Ctrl Pts',(-7.38963847013693,0.681884070047877,
0.789653671435307));
#165359=CARTESIAN_POINT('Ctrl Pts',(-7.38920532956846,0.681246574523939,
0.793665785717654));
#165360=CARTESIAN_POINT('Ctrl Pts',(-7.388772189,0.680609079,0.797677900000001));
#165361=CARTESIAN_POINT('Ctrl Pts',(-7.388079821,0.679590053,0.804091198));
#165362=CARTESIAN_POINT('Ctrl Pts',(-7.387376321,0.678571429,0.810503285));
#165363=CARTESIAN_POINT('Ctrl Pts',(-7.343815678,0.615498301,1.207539139));
#165364=CARTESIAN_POINT('Ctrl Pts',(-7.257951359,0.551245526,1.597619026));
#165365=CARTESIAN_POINT('Ctrl Pts',(-7.22546787182032,0.681884070047877,
0.595966473717341));
#165366=CARTESIAN_POINT('Ctrl Pts',(-7.22514000041016,0.681246574523939,
0.599889557358671));
#165367=CARTESIAN_POINT('Ctrl Pts',(-7.224812129,0.680609079,0.603812641));
#165368=CARTESIAN_POINT('Ctrl Pts',(-7.224288032,0.679590053,0.610083625));
#165369=CARTESIAN_POINT('Ctrl Pts',(-7.22375305,0.678571429,0.616353689));
#165370=CARTESIAN_POINT('Ctrl Pts',(-7.190627011,0.615498301,1.004595582));
#165371=CARTESIAN_POINT('Ctrl Pts',(-7.116079733,0.551245526,1.387050553));
#165372=CARTESIAN_POINT('',(-7.11698472798904,0.552026825929822,1.38239950192524));
#165373=CARTESIAN_POINT('Origin',(0.181669495499602,0.411147110446777,-0.0590434112763613));
#165374=CARTESIAN_POINT('Origin',(-9.25290503811619,0.3001208526991,1.5945150383709));
#165375=CARTESIAN_POINT('Ctrl Pts',(-7.328260282,0.551266351,1.235655988));
#165376=CARTESIAN_POINT('Ctrl Pts',(-7.260950543,0.615380951,1.634847424));
#165377=CARTESIAN_POINT('Ctrl Pts',(-7.150677531,0.680609079,2.024365416));
#165378=CARTESIAN_POINT('Ctrl Pts',(-7.14957171620143,0.681263184913293,
2.02827149194781));
#165379=CARTESIAN_POINT('Ctrl Pts',(-7.14846590140285,0.681917290826586,
2.03217756789561));
#165380=CARTESIAN_POINT('Ctrl Pts',(-7.117876367,0.551266351,1.377801155));
#165381=CARTESIAN_POINT('Ctrl Pts',(-7.042823572,0.615380951,1.765532373));
#165382=CARTESIAN_POINT('Ctrl Pts',(-6.926098167,0.680609079,2.14281688));
#165383=CARTESIAN_POINT('Ctrl Pts',(-6.92492764777796,0.681263184913293,
2.14660027888924));
#165384=CARTESIAN_POINT('Ctrl Pts',(-6.92375712855592,0.681917290826586,
2.15038367777849));
#165385=CARTESIAN_POINT('Origin',(0.176832129022559,0.803453450864247,-0.076033285388003));
#165386=CARTESIAN_POINT('Ctrl Pts',(-7.04712062926672,0.681884070047877,
2.35974584228104));
#165387=CARTESIAN_POINT('Ctrl Pts',(-7.04583513013336,0.681246574523938,
2.36357104314052));
#165388=CARTESIAN_POINT('Ctrl Pts',(-7.044549631,0.680609079,2.367396244));
#165389=CARTESIAN_POINT('Ctrl Pts',(-7.042494782,0.679590053,2.373510764));
#165390=CARTESIAN_POINT('Ctrl Pts',(-7.04042932,0.678571429,2.379621708));
#165391=CARTESIAN_POINT('Ctrl Pts',(-6.912536128,0.615498301,2.758010834));
#165392=CARTESIAN_POINT('Ctrl Pts',(-6.744823625,0.551245526,3.120512579));
#165393=CARTESIAN_POINT('Ctrl Pts',(-6.92842527283416,0.681884070047877,
2.13529511646555));
#165394=CARTESIAN_POINT('Ctrl Pts',(-6.92726171991709,0.681246574523938,
2.13905599823278));
#165395=CARTESIAN_POINT('Ctrl Pts',(-6.926098167,0.680609079,2.14281688));
#165396=CARTESIAN_POINT('Ctrl Pts',(-6.924238247,0.679590053,2.148828587));
#165397=CARTESIAN_POINT('Ctrl Pts',(-6.922367894,0.678571429,2.154837056));
#165398=CARTESIAN_POINT('Ctrl Pts',(-6.806555793,0.615498301,2.52688095));
#165399=CARTESIAN_POINT('Ctrl Pts',(-6.651534875,0.551245526,2.884368874));
#165400=CARTESIAN_POINT('',(-6.65341855000146,0.552026825966217,2.88002111040086));
#165401=CARTESIAN_POINT('Origin',(0.164729494829702,0.41114705736095,-0.0967165698653411));
#165402=CARTESIAN_POINT('Origin',(-8.69290291336178,0.300210269161947,3.54603265013523));
#165403=CARTESIAN_POINT('Ctrl Pts',(-6.891300118,0.551266351,2.782126377));
#165404=CARTESIAN_POINT('Ctrl Pts',(-6.739749684,0.615380951,3.157515334));
#165405=CARTESIAN_POINT('Ctrl Pts',(-6.548319939,0.680609079,3.514221174));
#165406=CARTESIAN_POINT('Ctrl Pts',(-6.54640028666558,0.681263184913293,
3.51779821057002));
#165407=CARTESIAN_POINT('Ctrl Pts',(-6.54448063433117,0.681917290826586,
3.52137524714005));
#165408=CARTESIAN_POINT('Ctrl Pts',(-6.6552766650606,0.551266351,2.87572241568554));
#165409=CARTESIAN_POINT('Ctrl Pts',(-6.49862778642101,0.615380951,3.23825449702954));
#165410=CARTESIAN_POINT('Ctrl Pts',(-6.30352632195629,0.680609079,3.58162572297104));
#165411=CARTESIAN_POINT('Ctrl Pts',(-6.30156984971784,0.681263184913293,
3.58506904038991));
#165412=CARTESIAN_POINT('Ctrl Pts',(-6.29961337747937,0.681917290826586,
3.58851235780879));
#165413=CARTESIAN_POINT('Origin',(0.156352826938365,0.803453443858178,-0.112269264913561));
#165414=CARTESIAN_POINT('Ctrl Pts',(-6.37508726444698,0.6818840700478,3.81949892020932));
#165415=CARTESIAN_POINT('Ctrl Pts',(-6.37300951372349,0.6812465745239,3.82295834560466));
#165416=CARTESIAN_POINT('Ctrl Pts',(-6.370931763,0.680609079,3.826417771));
#165417=CARTESIAN_POINT('Ctrl Pts',(-6.367610513,0.679590053,3.831947605));
#165418=CARTESIAN_POINT('Ctrl Pts',(-6.364279669,0.678571429,3.837471665));
#165419=CARTESIAN_POINT('Ctrl Pts',(-6.158034072,0.615498301,4.179521008));
#165420=CARTESIAN_POINT('Ctrl Pts',(-5.916315434,0.551245526,4.497494433));
#165421=CARTESIAN_POINT('Ctrl Pts',(-6.30741720870518,0.6818840700478,3.57477973384528));
#165422=CARTESIAN_POINT('Ctrl Pts',(-6.30547238085259,0.6812465745239,3.57820255892264));
#165423=CARTESIAN_POINT('Ctrl Pts',(-6.303527553,0.680609079,3.581625384));
#165424=CARTESIAN_POINT('Ctrl Pts',(-6.300418778,0.679590053,3.587096713));
#165425=CARTESIAN_POINT('Ctrl Pts',(-6.297300509,0.678571429,3.592562637));
#165426=CARTESIAN_POINT('Ctrl Pts',(-6.104217591,0.615498301,3.931012172));
#165427=CARTESIAN_POINT('Ctrl Pts',(-5.875971639,0.551245526,4.246817313));
#165428=CARTESIAN_POINT('',(-5.87874591598725,0.55202682617333,4.24297613144422));
#165429=CARTESIAN_POINT('Origin',(0.140086964193408,0.41114707159739,-0.129867334927797));
#165430=CARTESIAN_POINT('Origin',(-7.72986673852935,0.299963142155406,5.33334906303783));
#165431=CARTESIAN_POINT('Ctrl Pts',(-6.132110419,0.551266351,4.198507628));
#165432=CARTESIAN_POINT('Ctrl Pts',(-5.903405621,0.615380951,4.532541337));
#165433=CARTESIAN_POINT('Ctrl Pts',(-5.63977018500001,0.680609079,4.839755856));
#165434=CARTESIAN_POINT('Ctrl Pts',(-5.63712645593819,0.681263184913293,
4.84283659493409));
#165435=CARTESIAN_POINT('Ctrl Pts',(-5.63448272687637,0.681917290826586,
4.84591733386818));
#165436=CARTESIAN_POINT('Ctrl Pts',(-5.88148467891931,0.551266351,4.23917737896369));
#165437=CARTESIAN_POINT('Ctrl Pts',(-5.65056448275435,0.615380951,4.55955878216005));
#165438=CARTESIAN_POINT('Ctrl Pts',(-5.38620971812914,0.680609079,4.85296113255075));
#165439=CARTESIAN_POINT('Ctrl Pts',(-5.38355877565923,0.681263184913293,
4.85590336342949));
#165440=CARTESIAN_POINT('Ctrl Pts',(-5.38090783318931,0.681917290826586,
4.85884559430824));
#165441=CARTESIAN_POINT('Origin',(0.128560471524454,0.803452719747683,-0.143253674220777));
#165442=CARTESIAN_POINT('Ctrl Pts',(-5.40496190144401,0.68188407004776,
5.10065647404584));
#165443=CARTESIAN_POINT('Ctrl Pts',(-5.402189053722,0.68124657452388,5.10358836502292));
#165444=CARTESIAN_POINT('Ctrl Pts',(-5.399416206,0.680609079,5.106520256));
#165445=CARTESIAN_POINT('Ctrl Pts',(-5.394983855,0.679590053,5.111206835));
#165446=CARTESIAN_POINT('Ctrl Pts',(-5.390543374,0.678571429,5.115885712));
#165447=CARTESIAN_POINT('Ctrl Pts',(-5.115589186,0.615498301,5.405601425));
#165448=CARTESIAN_POINT('Ctrl Pts',(-4.811166908,0.551245526,5.664178446));
#165449=CARTESIAN_POINT('Ctrl Pts',(-5.39148132667926,0.68188407004776,
4.84711162513958));
#165450=CARTESIAN_POINT('Ctrl Pts',(-5.38884616133964,0.68124657452388,
4.8500363455698));
#165451=CARTESIAN_POINT('Ctrl Pts',(-5.386210996,0.680609079,4.852961066));
#165452=CARTESIAN_POINT('Ctrl Pts',(-5.381998728,0.679590053,4.857636183));
#165453=CARTESIAN_POINT('Ctrl Pts',(-5.377778351,0.678571429,4.862303981));
#165454=CARTESIAN_POINT('Ctrl Pts',(-5.116452959,0.615498301,5.15133363500001));
#165455=CARTESIAN_POINT('Ctrl Pts',(-4.825654501,0.551245526,5.410689294));
#165456=CARTESIAN_POINT('',(-4.82918965659591,0.552026825962079,5.4075343052009));
#165457=CARTESIAN_POINT('Origin',(0.108894174443853,0.411147075198583,-0.156945658187523));
#165458=CARTESIAN_POINT('Origin',(-6.40110697697016,0.300136499740306,6.86890405535685));
#165459=CARTESIAN_POINT('Ctrl Pts',(-5.086190052,0.551266351,5.418571329));
#165460=CARTESIAN_POINT('Ctrl Pts',(-4.791024871,0.615380951,5.695630744));
#165461=CARTESIAN_POINT('Ctrl Pts',(-4.467511046,0.680609079,5.938988933));
#165462=CARTESIAN_POINT('Ctrl Pts',(-4.46426685806371,0.681263184913293,
5.94142932237425));
#165463=CARTESIAN_POINT('Ctrl Pts',(-4.46102267012741,0.681917290826586,
5.94386971174849));
#165464=CARTESIAN_POINT('Ctrl Pts',(-4.83268101123186,0.551266351,5.40441311780555));
#165465=CARTESIAN_POINT('Ctrl Pts',(-4.53828706911003,0.615380951,5.66766316636527));
#165466=CARTESIAN_POINT('Ctrl Pts',(-4.21703993950809,0.680609079,5.89737747275712));
#165467=CARTESIAN_POINT('Ctrl Pts',(-4.21381848193228,0.681263184913293,
5.89968104164352));
#165468=CARTESIAN_POINT('Ctrl Pts',(-4.21059702435648,0.681917290826586,
5.90198461052992));
#165469=CARTESIAN_POINT('Origin',(0.0947614322425405,0.803453435370911,
-0.167543794197096));
#165470=CARTESIAN_POINT('Ctrl Pts',(-4.18210652789464,0.681884070047697,
6.14331299852755));
#165471=CARTESIAN_POINT('Ctrl Pts',(-4.17876823794732,0.681246574523849,
6.14558026326377));
#165472=CARTESIAN_POINT('Ctrl Pts',(-4.175429948,0.680609079,6.14784752800001));
#165473=CARTESIAN_POINT('Ctrl Pts',(-4.170093747,0.679590053,6.151471713));
#165474=CARTESIAN_POINT('Ctrl Pts',(-4.164751262,0.678571429,6.155086629));
#165475=CARTESIAN_POINT('Ctrl Pts',(-3.833945036,0.615498301,6.378921927));
#165476=CARTESIAN_POINT('Ctrl Pts',(-3.481053566,0.551245526,6.56601177));
#165477=CARTESIAN_POINT('Ctrl Pts',(-4.22344576855952,0.681884070047697,
5.8927979621922));
#165478=CARTESIAN_POINT('Ctrl Pts',(-4.22024348377976,0.681246574523849,
5.8950878220961));
#165479=CARTESIAN_POINT('Ctrl Pts',(-4.217041199,0.680609079,5.897377682));
#165480=CARTESIAN_POINT('Ctrl Pts',(-4.2119224,0.679590053,5.901037985));
#165481=CARTESIAN_POINT('Ctrl Pts',(-4.206797255,0.678571429,5.904689396));
#165482=CARTESIAN_POINT('Ctrl Pts',(-3.889448673,0.615498301,6.130784462));
#165483=CARTESIAN_POINT('Ctrl Pts',(-3.549695121,0.551245526,6.321563458));
#165484=CARTESIAN_POINT('',(-3.55382585594571,0.552026825906715,6.31924218473728));
#165485=CARTESIAN_POINT('Origin',(0.0726095802536447,0.411147127799279,
-0.176685306794135));
#165486=CARTESIAN_POINT('Origin',(-4.77447887405374,0.300179931536728,8.08381453320419));
#165487=CARTESIAN_POINT('Ctrl Pts',(-3.802445091,0.551266351,6.385268657));
#165488=CARTESIAN_POINT('Ctrl Pts',(-3.454621124,0.615380951,6.592398788));
#165489=CARTESIAN_POINT('Ctrl Pts',(-3.086356055,0.680609079,6.76052148800001));
#165490=CARTESIAN_POINT('Ctrl Pts',(-3.08266310279245,0.681263184913293,
6.76220741791399));
#165491=CARTESIAN_POINT('Ctrl Pts',(-3.0789701505849,0.681917290826586,
6.76389334782798));
#165492=CARTESIAN_POINT('Ctrl Pts',(-3.55790654742961,0.551266351,6.31694450745764));
#165493=CARTESIAN_POINT('Ctrl Pts',(-3.21380439414336,0.615380951,6.5107539204794));
#165494=CARTESIAN_POINT('Ctrl Pts',(-2.85068605802178,0.680609079,6.66603899693022));
#165495=CARTESIAN_POINT('Ctrl Pts',(-2.84704471711311,0.681263184913293,
6.66759619150052));
#165496=CARTESIAN_POINT('Ctrl Pts',(-2.84340337620444,0.681917290826586,
6.66915338607082));
#165497=CARTESIAN_POINT('Origin',(0.0565289924188023,0.80345341474124,-0.183997606089015));
#165498=CARTESIAN_POINT('Ctrl Pts',(-2.76370050292562,0.681884070047611,
6.89871503673943));
#165499=CARTESIAN_POINT('Ctrl Pts',(-2.75995286496281,0.681246574523805,
6.90021166036972));
#165500=CARTESIAN_POINT('Ctrl Pts',(-2.756205227,0.680609079,6.901708284));
#165501=CARTESIAN_POINT('Ctrl Pts',(-2.75021469,0.679590053,6.90410061200001));
#165502=CARTESIAN_POINT('Ctrl Pts',(-2.744220009,0.678571429,6.906482536));
#165503=CARTESIAN_POINT('Ctrl Pts',(-2.373029877,0.615498301,7.053971129));
#165504=CARTESIAN_POINT('Ctrl Pts',(-1.988170027,0.551245526,7.16082568100001));
#165505=CARTESIAN_POINT('Ctrl Pts',(-2.85792658132566,0.681884070047611,
6.66294361747932));
#165506=CARTESIAN_POINT('Ctrl Pts',(-2.85430691216284,0.681246574523805,
6.66449154473966));
#165507=CARTESIAN_POINT('Ctrl Pts',(-2.850687243,0.680609079,6.666039472));
#165508=CARTESIAN_POINT('Ctrl Pts',(-2.844901262,0.679590053,6.668513808));
#165509=CARTESIAN_POINT('Ctrl Pts',(-2.839110994,0.678571429,6.670978097));
#165510=CARTESIAN_POINT('Ctrl Pts',(-2.48057809,0.615498301,6.823566622));
#165511=CARTESIAN_POINT('Ctrl Pts',(-2.107755942,0.551245526,6.93684834));
#165512=CARTESIAN_POINT('',(-2.11228911074674,0.552026825786492,6.93546932179441));
#165513=CARTESIAN_POINT('Origin',(0.0329298365003622,0.41114712983725,-0.188163271897352));
#165514=CARTESIAN_POINT('Origin',(-2.92612069033567,0.299941709146899,8.92383548076064));
#165515=CARTESIAN_POINT('Ctrl Pts',(-2.340902024,0.551266351,7.053397919));
#165516=CARTESIAN_POINT('Ctrl Pts',(-1.956683132,0.615380951,7.180913592));
#165517=CARTESIAN_POINT('Ctrl Pts',(-1.560886485,0.680609079,7.265939572));
#165518=CARTESIAN_POINT('Ctrl Pts',(-1.55691744686872,0.681263184913293,
7.2667922102407));
#165519=CARTESIAN_POINT('Ctrl Pts',(-1.55294840873743,0.681917290826586,
7.26764484848138));
#165520=CARTESIAN_POINT('Ctrl Pts',(-2.11676832528776,0.551266351,6.93410259070982));
#165521=CARTESIAN_POINT('Ctrl Pts',(-1.73904779404177,0.615380951,7.04940905517114));
#165522=CARTESIAN_POINT('Ctrl Pts',(-1.35103726228651,0.680609079,7.12300394455444));
#165523=CARTESIAN_POINT('Ctrl Pts',(-1.3471463031095,0.681263184913293,
7.12374195212587));
#165524=CARTESIAN_POINT('Ctrl Pts',(-1.34325534393248,0.681917290826586,
7.12447995969728));
#165525=CARTESIAN_POINT('Origin',(0.0156526904332333,0.803452733533447,
-0.191844834767033));
#165526=CARTESIAN_POINT('Ctrl Pts',(-1.21606691399939,0.68188407004749,
7.33154082511757));
#165527=CARTESIAN_POINT('Ctrl Pts',(-1.21208516349969,0.681246574523745,
7.3321968275588));
#165528=CARTESIAN_POINT('Ctrl Pts',(-1.208103413,0.680609079000001,7.33285283000001));
#165529=CARTESIAN_POINT('Ctrl Pts',(-1.201738651,0.679590053,7.333901439));
#165530=CARTESIAN_POINT('Ctrl Pts',(-1.195372079,0.678571429,7.334938996));
#165531=CARTESIAN_POINT('Ctrl Pts',(-0.801154479,0.615498301,7.399184481));
#165532=CARTESIAN_POINT('Ctrl Pts',(-0.402321868,0.551245526,7.420807342));
#165533=CARTESIAN_POINT('Ctrl Pts',(-1.3587739249797,0.68188407004749,7.12153743297978));
#165534=CARTESIAN_POINT('Ctrl Pts',(-1.35490612248985,0.681246574523745,
7.12227104898989));
#165535=CARTESIAN_POINT('Ctrl Pts',(-1.35103832,0.680609079000001,7.123004665));
#165536=CARTESIAN_POINT('Ctrl Pts',(-1.344855702,0.679590053,7.124177338));
#165537=CARTESIAN_POINT('Ctrl Pts',(-1.338671059,0.678571429,7.125339276));
#165538=CARTESIAN_POINT('Ctrl Pts',(-0.955718432,0.615498301,7.19728639));
#165539=CARTESIAN_POINT('Ctrl Pts',(-0.567260438,0.551245526,7.227773903));
#165540=CARTESIAN_POINT('',(-0.571984069400262,0.552026825956257,7.22740162306855));
#165541=CARTESIAN_POINT('Origin',(-0.00828956117031529,0.41114712676337,
-0.190843312368436));
#165542=CARTESIAN_POINT('Origin',(-0.939094529349745,0.30008162841821,9.34267857849552));
#165543=CARTESIAN_POINT('Ctrl Pts',(-0.780723137064731,0.551266351,7.40094088412655));
#165544=CARTESIAN_POINT('Ctrl Pts',(-0.377572579286645,0.615380951,7.44346912117974));
#165545=CARTESIAN_POINT('Ctrl Pts',(0.0278120868452411,0.680609079,7.4419541167355));
#165546=CARTESIAN_POINT('Ctrl Pts',(0.0318772733745123,0.681263184913293,
7.44193892431167));
#165547=CARTESIAN_POINT('Ctrl Pts',(0.0359424599037835,0.681917290826586,
7.44192373188786));
#165548=CARTESIAN_POINT('Ctrl Pts',(-0.769900980000001,0.551266351,7.391718134));
#165549=CARTESIAN_POINT('Ctrl Pts',(-0.367252812,0.615380951,7.433656857));
#165550=CARTESIAN_POINT('Ctrl Pts',(0.037568402,0.680609079,7.431610398));
#165551=CARTESIAN_POINT('Ctrl Pts',(0.0416279382464465,0.681263184913293,
7.43158987616418));
#165552=CARTESIAN_POINT('Ctrl Pts',(0.0456874744928931,0.681917290826586,
7.43156935432838));
#165553=CARTESIAN_POINT('Ctrl Pts',(-0.576653346,0.551266351,7.227030574));
#165554=CARTESIAN_POINT('Ctrl Pts',(-0.182976184,0.615380951,7.258442542));
#165555=CARTESIAN_POINT('Ctrl Pts',(0.211783654,0.680609079,7.246906077));
#165556=CARTESIAN_POINT('Ctrl Pts',(0.215742295038516,0.681263184913293,
7.24679038963925));
#165557=CARTESIAN_POINT('Ctrl Pts',(0.219700936077032,0.681917290826586,
7.24667470227851));
#165558=CARTESIAN_POINT('Origin',(-0.0259542276886779,0.80345272965562,
-0.190724450753197));
#165559=CARTESIAN_POINT('Origin',(-7.084,3.7,7.084));
#165560=CARTESIAN_POINT('Ctrl Pts',(0.207089507,0.681369595,7.247041737));
#165561=CARTESIAN_POINT('Ctrl Pts',(0.215726884,0.679970133,7.246794918));
#165562=CARTESIAN_POINT('Ctrl Pts',(0.224363648,0.678571429,7.24652751));
#165563=CARTESIAN_POINT('Ctrl Pts',(0.611454754,0.615882895,7.234542573));
#165564=CARTESIAN_POINT('Ctrl Pts',(0.995066308,0.552026826,7.181388657));
#165565=CARTESIAN_POINT('Ctrl Pts',(0.056367661,0.681369595,7.406630948));
#165566=CARTESIAN_POINT('Ctrl Pts',(0.065195244,0.679970133,7.406563766));
#165567=CARTESIAN_POINT('Ctrl Pts',(0.074022642,0.678571429,7.406475542));
#165568=CARTESIAN_POINT('Ctrl Pts',(0.469657766,0.615882895,7.402521441));
#165569=CARTESIAN_POINT('Ctrl Pts',(0.86262025,0.552026826,7.356442456));
#165570=CARTESIAN_POINT('Ctrl Pts',(0.21765174455862,0.655900535668849,
7.40270156512545));
#165571=CARTESIAN_POINT('Ctrl Pts',(0.217001547613326,0.658682906707741,
7.38460695266366));
#165572=CARTESIAN_POINT('Ctrl Pts',(0.216340972118041,0.661493949096189,
7.36651709356107));
#165573=CARTESIAN_POINT('Ctrl Pts',(0.215669566035234,0.664334613017224,
7.34843231566661));
#165574=CARTESIAN_POINT('Ctrl Pts',(0.215041027322259,0.666993908621838,
7.33150219943251));
#165575=CARTESIAN_POINT('Ctrl Pts',(0.214402995011337,0.669679171588032,
7.31457648975586));
#165576=CARTESIAN_POINT('Ctrl Pts',(0.213755072783103,0.672391218148102,
7.29765547471631));
#165577=CARTESIAN_POINT('Ctrl Pts',(0.213107143282986,0.67510329514652,
7.28073426976565));
#165578=CARTESIAN_POINT('Ctrl Pts',(0.212445088585071,0.677841475225338,
7.26381776537258));
#165579=CARTESIAN_POINT('Ctrl Pts',(0.211783655068483,0.680609081981435,
7.24690609670463));
#165580=CARTESIAN_POINT('',(0.972815229604965,0.552026824384635,7.21079786933495));
#165581=CARTESIAN_POINT('Ctrl Pts',(0.627711922,0.499686101,7.275310889));
#165582=CARTESIAN_POINT('Ctrl Pts',(0.739025144,0.51775868,7.265706814));
#165583=CARTESIAN_POINT('Ctrl Pts',(0.849992445,0.535714286,7.252701816));
#165584=CARTESIAN_POINT('Ctrl Pts',(0.900321661,0.54385805,7.2468034));
#165585=CARTESIAN_POINT('Ctrl Pts',(0.950564171,0.552026826,7.240207079));
#165586=CARTESIAN_POINT('Ctrl Pts',(0.67478522,0.499686101,7.218529276));
#165587=CARTESIAN_POINT('Ctrl Pts',(0.785229676,0.51775868,7.208204972));
#165588=CARTESIAN_POINT('Ctrl Pts',(0.895306583,0.535714286,7.194506663));
#165589=CARTESIAN_POINT('Ctrl Pts',(0.945231961,0.54385805,7.188293795));
#165590=CARTESIAN_POINT('Ctrl Pts',(0.995066308,0.552026826,7.181388657));
#165591=CARTESIAN_POINT('Ctrl Pts',(0.99506630855658,0.552026826281282,
7.18138865673239));
#165592=CARTESIAN_POINT('Ctrl Pts',(0.961819032715832,0.546576979789078,
7.18599546025834));
#165593=CARTESIAN_POINT('Ctrl Pts',(0.928564162759112,0.541139220286484,
7.19036798743331));
#165594=CARTESIAN_POINT('Ctrl Pts',(0.895306583168572,0.535714286026804,
7.19450666298286));
#165595=CARTESIAN_POINT('Ctrl Pts',(0.822683552237206,0.523868108970865,
7.20354409641407));
#165596=CARTESIAN_POINT('Ctrl Pts',(0.749799676836557,0.511960760930993,
7.21149710151007));
#165597=CARTESIAN_POINT('Ctrl Pts',(0.676703532269255,0.49999999974866,
7.21834969580106));
#165598=CARTESIAN_POINT('Ctrl Pts',(0.67478522,0.499686101,7.218529276));
#165599=CARTESIAN_POINT('Ctrl Pts',(0.785229676,0.51775868,7.208204972));
#165600=CARTESIAN_POINT('Ctrl Pts',(0.895306583,0.535714286,7.194506663));
#165601=CARTESIAN_POINT('Ctrl Pts',(0.946186392,0.544013736,7.188175023));
#165602=CARTESIAN_POINT('Ctrl Pts',(0.99697156,0.552339147,7.181124404));
#165603=CARTESIAN_POINT('Ctrl Pts',(0.723670697,0.499686101,7.259056491));
#165604=CARTESIAN_POINT('Ctrl Pts',(0.834735225,0.51775868,7.247984233));
#165605=CARTESIAN_POINT('Ctrl Pts',(0.945409031,0.535714286,7.233519349));
#165606=CARTESIAN_POINT('Ctrl Pts',(0.996564739,0.544013736,7.226833383));
#165607=CARTESIAN_POINT('Ctrl Pts',(1.047620768,0.552339147,7.21942457099999));
#165608=CARTESIAN_POINT('Ctrl Pts',(0.99506631450015,0.552026827255544,
7.18138865590884));
#165609=CARTESIAN_POINT('Ctrl Pts',(0.99574332826213,0.551172308319168,
7.186567436955));
#165610=CARTESIAN_POINT('Ctrl Pts',(0.996419516854235,0.550320534977845,
7.19174677410628));
#165611=CARTESIAN_POINT('Ctrl Pts',(0.997094885402565,0.549471478062853,
7.19692666267777));
#165612=CARTESIAN_POINT('Ctrl Pts',(0.997721871981064,0.548683245783752,
7.2017354750225));
#165613=CARTESIAN_POINT('Ctrl Pts',(0.998348151970431,0.547897354469737,
7.20654476390293));
#165614=CARTESIAN_POINT('Ctrl Pts',(0.998973732569637,0.547113782422352,
7.21135452094716));
#165615=CARTESIAN_POINT('Ctrl Pts',(0.999599313800958,0.546330209583209,
7.21616428285138));
#165616=CARTESIAN_POINT('Ctrl Pts',(1.00022419579762,0.545548955818075,
7.22097451413375));
#165617=CARTESIAN_POINT('Ctrl Pts',(1.0008483868275,0.54476999986866,7.2257852066657));
#165618=CARTESIAN_POINT('Ctrl Pts',(0.993197311,0.55233793,7.181647381));
#165619=CARTESIAN_POINT('Ctrl Pts',(1.151022227,0.526068113,7.159820734));
#165620=CARTESIAN_POINT('Ctrl Pts',(1.307735906,0.49968693,7.131081741));
#165621=CARTESIAN_POINT('Ctrl Pts',(0.95487053,0.55233793,7.232276452));
#165622=CARTESIAN_POINT('Ctrl Pts',(1.113808078,0.526068113,7.21129208));
#165623=CARTESIAN_POINT('Ctrl Pts',(1.271670316,0.49968693,7.18334567));
#165624=CARTESIAN_POINT('Origin',(-0.049945526223899,0.410743194127898,
-0.190657471942941));
#165625=CARTESIAN_POINT('Ctrl Pts',(1.05073165838991,0.552548454735263,
7.22635066464236));
#165626=CARTESIAN_POINT('Ctrl Pts',(1.05230819469495,0.552287640367632,
7.22612072932118));
#165627=CARTESIAN_POINT('Ctrl Pts',(1.053884731,0.552026826,7.225890794));
#165628=CARTESIAN_POINT('Ctrl Pts',(1.211741222,0.525911829,7.202867675));
#165629=CARTESIAN_POINT('Ctrl Pts',(1.368441669,0.49968693,7.172972758));
#165630=CARTESIAN_POINT('Ctrl Pts',(0.991923006675841,0.552548454735263,
7.18181555581264));
#165631=CARTESIAN_POINT('Ctrl Pts',(0.993489831971372,0.552287640367632,
7.18159845552429));
#165632=CARTESIAN_POINT('Ctrl Pts',(0.995056657266902,0.552026826,7.18138135523595));
#165633=CARTESIAN_POINT('Ctrl Pts',(1.15194079775301,0.525911829,7.15964339106533));
#165634=CARTESIAN_POINT('Ctrl Pts',(1.30772594559837,0.49968693,7.13107486765992));
#165635=CARTESIAN_POINT('',(1.08259319807141,0.552026824387391,7.24761168748306));
#165636=CARTESIAN_POINT('Ctrl Pts',(0.987286864787933,0.550751630586317,
7.18246659083401));
#165637=CARTESIAN_POINT('Ctrl Pts',(0.991176586393967,0.551389228293159,
7.18192762391701));
#165638=CARTESIAN_POINT('Ctrl Pts',(0.995066308,0.552026826000001,7.181388657));
#165639=CARTESIAN_POINT('Ctrl Pts',(1.386277161,0.61615356,7.127181768));
#165640=CARTESIAN_POINT('Ctrl Pts',(1.769284534,0.681389364,7.030798834));
#165641=CARTESIAN_POINT('Ctrl Pts',(1.16219718885009,0.550751630586317,
7.31510228082505));
#165642=CARTESIAN_POINT('Ctrl Pts',(1.16615864842505,0.551389228293159,
7.31446849791252));
#165643=CARTESIAN_POINT('Ctrl Pts',(1.170120108,0.552026826000001,7.313834715));
#165644=CARTESIAN_POINT('Ctrl Pts',(1.568546046,0.61615356,7.250091656));
#165645=CARTESIAN_POINT('Ctrl Pts',(1.957689904,0.681389364,7.14344521600001));
#165646=CARTESIAN_POINT('Ctrl Pts',(1.76470286480055,0.680609082082805,
7.03195023316344));
#165647=CARTESIAN_POINT('Ctrl Pts',(1.76927629608276,0.677652752738448,
7.04944087630682));
#165648=CARTESIAN_POINT('Ctrl Pts',(1.77385099516534,0.67472989691538,7.06693689689647));
#165649=CARTESIAN_POINT('Ctrl Pts',(1.77841126959504,0.671836782554415,
7.08444156064863));
#165650=CARTESIAN_POINT('Ctrl Pts',(1.78268038335609,0.669128385390798,
7.10082860095926));
#165651=CARTESIAN_POINT('Ctrl Pts',(1.78694087127159,0.666446714500865,
7.11722232948892));
#165652=CARTESIAN_POINT('Ctrl Pts',(1.79119305702725,0.663790956144513,
7.13362238136369));
#165653=CARTESIAN_POINT('Ctrl Pts',(1.79544528843677,0.661135169274451,
7.15002260931861));
#165654=CARTESIAN_POINT('Ctrl Pts',(1.79968922868348,0.658505288583656,
7.16642920443237));
#165655=CARTESIAN_POINT('Ctrl Pts',(1.80392518236685,0.655900535538507,
7.18284182470367));
#165656=CARTESIAN_POINT('Ctrl Pts',(1.760147622,0.681369595,7.033091806));
#165657=CARTESIAN_POINT('Ctrl Pts',(1.768530003,0.679970133,7.030993976));
#165658=CARTESIAN_POINT('Ctrl Pts',(1.776907359,0.678571429,7.028876172));
#165659=CARTESIAN_POINT('Ctrl Pts',(2.152372083,0.615882895,6.933958291));
#165660=CARTESIAN_POINT('Ctrl Pts',(2.515588492,0.552026826,6.799581939));
#165661=CARTESIAN_POINT('Ctrl Pts',(1.647256531,0.681369595,7.22135065100001));
#165662=CARTESIAN_POINT('Ctrl Pts',(1.655863289,0.679970133,7.219387371));
#165663=CARTESIAN_POINT('Ctrl Pts',(1.664465341,0.678571429,7.21740358));
#165664=CARTESIAN_POINT('Ctrl Pts',(2.050000721,0.615882895,7.12849206600001));
#165665=CARTESIAN_POINT('Ctrl Pts',(2.423870341,0.552026826,6.999015065));
#165666=CARTESIAN_POINT('',(2.50017974262328,0.552026824384634,6.83308690443088));
#165667=CARTESIAN_POINT('Ctrl Pts',(2.177013151,0.499686101,6.970278656));
#165668=CARTESIAN_POINT('Ctrl Pts',(2.283659339,0.51775868,6.936970065));
#165669=CARTESIAN_POINT('Ctrl Pts',(2.389236596,0.535714286,6.900414428));
#165670=CARTESIAN_POINT('Ctrl Pts',(2.437121158,0.54385805,6.88383462));
#165671=CARTESIAN_POINT('Ctrl Pts',(2.484771012,0.552026826,6.866591863));
#165672=CARTESIAN_POINT('Ctrl Pts',(2.210779533,0.499686101,6.904705197));
#165673=CARTESIAN_POINT('Ctrl Pts',(2.316422439,0.51775868,6.870879977));
#165674=CARTESIAN_POINT('Ctrl Pts',(2.420981077,0.535714286,6.833838645));
#165675=CARTESIAN_POINT('Ctrl Pts',(2.468403645,0.54385805,6.81703855));
#165676=CARTESIAN_POINT('Ctrl Pts',(2.515588492,0.552026826,6.799581939));
#165677=CARTESIAN_POINT('Ctrl Pts',(2.51558848994905,0.552026825797967,
6.79958193941116));
#165678=CARTESIAN_POINT('Ctrl Pts',(2.48410884342391,0.546576979474308,
6.81122821934968));
#165679=CARTESIAN_POINT('Ctrl Pts',(2.4525714186327,0.541139220132675,6.82264733293808));
#165680=CARTESIAN_POINT('Ctrl Pts',(2.42098107697934,0.535714285996453,
6.83383864500732));
#165681=CARTESIAN_POINT('Ctrl Pts',(2.35199871315026,0.52386810886986,6.85827659379462));
#165682=CARTESIAN_POINT('Ctrl Pts',(2.28252848394537,0.511960760922405,
6.88171154060857));
#165683=CARTESIAN_POINT('Ctrl Pts',(2.21261439168748,0.499999999735721,
6.90411743489196));
#165684=CARTESIAN_POINT('Ctrl Pts',(2.210779533,0.499686101,6.904705197));
#165685=CARTESIAN_POINT('Ctrl Pts',(2.316422439,0.51775868,6.870879977));
#165686=CARTESIAN_POINT('Ctrl Pts',(2.420981077,0.535714286,6.833838645));
#165687=CARTESIAN_POINT('Ctrl Pts',(2.469310228,0.544013736,6.81671738));
#165688=CARTESIAN_POINT('Ctrl Pts',(2.517392394,0.552339147,6.798914291));
#165689=CARTESIAN_POINT('Ctrl Pts',(2.267234248,0.499686101,6.933775975));
#165690=CARTESIAN_POINT('Ctrl Pts',(2.373321941,0.51775868,6.89908699));
#165691=CARTESIAN_POINT('Ctrl Pts',(2.478298732,0.535714286,6.861168691));
#165692=CARTESIAN_POINT('Ctrl Pts',(2.526821163,0.544013736,6.843642074));
#165693=CARTESIAN_POINT('Ctrl Pts',(2.575090855,0.552339147,6.825430939));
#165694=CARTESIAN_POINT('Ctrl Pts',(2.51558849795866,0.552026827184613,
6.79958193644791));
#165695=CARTESIAN_POINT('Ctrl Pts',(2.51736296788845,0.551172308216822,
6.80449410254021));
#165696=CARTESIAN_POINT('Ctrl Pts',(2.51913675196281,0.550320534899973,
6.80940698905447));
#165697=CARTESIAN_POINT('Ctrl Pts',(2.52090985370924,0.54947147800732,6.81432059038011));
#165698=CARTESIAN_POINT('Ctrl Pts',(2.52255593423229,0.548683245737638,
6.81888219179778));
#165699=CARTESIAN_POINT('Ctrl Pts',(2.5242014271309,0.547897354431265,6.82344441050407));
#165700=CARTESIAN_POINT('Ctrl Pts',(2.52584633764004,0.5471137823873,6.82800723679375));
#165701=CARTESIAN_POINT('Ctrl Pts',(2.52749124979859,0.546330209557625,
6.83257006765872));
#165702=CARTESIAN_POINT('Ctrl Pts',(2.52913557998059,0.545548955797864,
6.83713350725973));
#165703=CARTESIAN_POINT('Ctrl Pts',(2.53077933509621,0.544770000008302,
6.84169754538297));
#165704=CARTESIAN_POINT('Ctrl Pts',(2.513818808,0.55233793,6.800236393));
#165705=CARTESIAN_POINT('Ctrl Pts',(2.663261782,0.526068113,6.744992349));
#165706=CARTESIAN_POINT('Ctrl Pts',(2.810133548,0.49968693,6.68323645));
#165707=CARTESIAN_POINT('Ctrl Pts',(2.48727184,0.55233793,6.85792091));
#165708=CARTESIAN_POINT('Ctrl Pts',(2.637982497,0.526068113,6.803260266));
#165709=CARTESIAN_POINT('Ctrl Pts',(2.786146352,0.49968693,6.742031513));
#165710=CARTESIAN_POINT('Origin',(-0.0897638160116732,0.410742936752906,
-0.175463805149405));
#165711=CARTESIAN_POINT('Ctrl Pts',(2.57961791904852,0.552548454735263,
6.83152635453666));
#165712=CARTESIAN_POINT('Ctrl Pts',(2.58110816752426,0.552287640367631,
6.83096288626833));
#165713=CARTESIAN_POINT('Ctrl Pts',(2.582598416,0.552026826,6.830399418));
#165714=CARTESIAN_POINT('Ctrl Pts',(2.731815021,0.525911829,6.773980087));
#165715=CARTESIAN_POINT('Ctrl Pts',(2.878425375,0.49968693,6.711098133));
#165716=CARTESIAN_POINT('Ctrl Pts',(2.51261044996927,0.552548454735263,
6.80067457404514));
#165717=CARTESIAN_POINT('Ctrl Pts',(2.51409397361356,0.552287640367631,
6.80012572831319));
#165718=CARTESIAN_POINT('Ctrl Pts',(2.51557749725783,0.552026826,6.79957688258125));
#165719=CARTESIAN_POINT('Ctrl Pts',(2.66412075379542,0.525911829,6.74462168677177));
#165720=CARTESIAN_POINT('Ctrl Pts',(2.8101223429279,0.49968693,6.68323187855741));
#165721=CARTESIAN_POINT('',(2.61530504560632,0.552026824384634,6.84544101758886));
#165722=CARTESIAN_POINT('Ctrl Pts',(2.50822148649275,0.550751630586317,
6.80230648424818));
#165723=CARTESIAN_POINT('Ctrl Pts',(2.51190440631477,0.551389228293159,
6.80094394353719));
#165724=CARTESIAN_POINT('Ctrl Pts',(2.51558732613678,0.552026826,6.79958140282619));
#165725=CARTESIAN_POINT('Ctrl Pts',(2.88599897792836,0.61615356,6.66254313433735));
#165726=CARTESIAN_POINT('Ctrl Pts',(3.23933234779194,0.681389364000001,
6.48607838264556));
#165727=CARTESIAN_POINT('Ctrl Pts',(2.70755642147094,0.550751630586317,
6.89424121325815));
#165728=CARTESIAN_POINT('Ctrl Pts',(2.71128901973547,0.551389228293159,
6.89277065112907));
#165729=CARTESIAN_POINT('Ctrl Pts',(2.715021618,0.552026826,6.891300089));
#165730=CARTESIAN_POINT('Ctrl Pts',(3.090429706,0.61615356,6.74339750800001));
#165731=CARTESIAN_POINT('Ctrl Pts',(3.447549765,0.681389364000001,6.555589976));
#165732=CARTESIAN_POINT('Ctrl Pts',(3.23510652986855,0.680609082082805,
6.48818819349658));
#165733=CARTESIAN_POINT('Ctrl Pts',(3.24333300793022,0.677652752623469,
6.50428676221162));
#165734=CARTESIAN_POINT('Ctrl Pts',(3.25156188047759,0.674729896811195,
6.52039031048621));
#165735=CARTESIAN_POINT('Ctrl Pts',(3.25977852354583,0.671836782445325,
6.53650540076861));
#165736=CARTESIAN_POINT('Ctrl Pts',(3.26747055705726,0.669128385297014,
6.55159158784801));
#165737=CARTESIAN_POINT('Ctrl Pts',(3.27515560416031,0.666446714422628,
6.5666861610813));
#165738=CARTESIAN_POINT('Ctrl Pts',(3.28283390253543,0.663790956081852,
6.5817886945425));
#165739=CARTESIAN_POINT('Ctrl Pts',(3.29051228334905,0.661135169227366,
6.59689139015297));
#165740=CARTESIAN_POINT('Ctrl Pts',(3.29818393559334,0.658505288552175,
6.61200208641671));
#165741=CARTESIAN_POINT('Ctrl Pts',(3.30584908284948,0.655900535589578,
6.62712038403327));
#165742=CARTESIAN_POINT('Ctrl Pts',(3.23090319,0.681369595,6.490282319));
#165743=CARTESIAN_POINT('Ctrl Pts',(3.238638624,0.679970133,6.486431571));
#165744=CARTESIAN_POINT('Ctrl Pts',(3.246364857,0.678571429,6.482562396));
#165745=CARTESIAN_POINT('Ctrl Pts',(3.592646886,0.615882895,6.30914982500001));
#165746=CARTESIAN_POINT('Ctrl Pts',(3.918484554,0.552026826,6.099834326));
#165747=CARTESIAN_POINT('Ctrl Pts',(3.161121518,0.681369595,6.698408024));
#165748=CARTESIAN_POINT('Ctrl Pts',(3.169105006,0.679970133,6.694640446));
#165749=CARTESIAN_POINT('Ctrl Pts',(3.177079491,0.678571429,6.690853848));
#165750=CARTESIAN_POINT('Ctrl Pts',(3.534487921,0.615882895,6.52114232600001));
#165751=CARTESIAN_POINT('Ctrl Pts',(3.871782949,0.552026826,6.314321508));
#165752=CARTESIAN_POINT('',(3.91063862958003,0.552026824384634,6.13586838986638));
#165753=CARTESIAN_POINT('Ctrl Pts',(3.624519664,0.499686101,6.339323939));
#165754=CARTESIAN_POINT('Ctrl Pts',(3.721512162,0.51775868,6.283868307));
#165755=CARTESIAN_POINT('Ctrl Pts',(3.816762699,0.535714286,6.225471331));
#165756=CARTESIAN_POINT('Ctrl Pts',(3.859963578,0.54385805,6.198985384));
#165757=CARTESIAN_POINT('Ctrl Pts',(3.902792722,0.552026826,6.171902443));
#165758=CARTESIAN_POINT('Ctrl Pts',(3.643400252,0.499686101,6.268024777));
#165759=CARTESIAN_POINT('Ctrl Pts',(3.739301863,0.51775868,6.21228027));
#165760=CARTESIAN_POINT('Ctrl Pts',(3.833453187,0.535714286,6.153627927));
#165761=CARTESIAN_POINT('Ctrl Pts',(3.876155517,0.54385805,6.127026159));
#165762=CARTESIAN_POINT('Ctrl Pts',(3.918484554,0.552026826,6.099834326));
#165763=CARTESIAN_POINT('Ctrl Pts',(3.91848455377917,0.552026826341472,
6.09983432539862));
#165764=CARTESIAN_POINT('Ctrl Pts',(3.8902444900359,0.546576979835352,6.11797551583042));
#165765=CARTESIAN_POINT('Ctrl Pts',(3.86189916403442,0.541139220312496,
6.13590727149343));
#165766=CARTESIAN_POINT('Ctrl Pts',(3.83345318706314,0.535714285972514,
6.15362792713793));
#165767=CARTESIAN_POINT('Ctrl Pts',(3.77133702917716,0.52386810879776,6.19232369985583));
#165768=CARTESIAN_POINT('Ctrl Pts',(3.7085287958654,0.511960760930835,6.23014479602785));
#165769=CARTESIAN_POINT('Ctrl Pts',(3.64506586129707,0.499999999748424,
6.26705631602722));
#165770=CARTESIAN_POINT('Ctrl Pts',(3.643400252,0.499686101,6.268024777));
#165771=CARTESIAN_POINT('Ctrl Pts',(3.739301863,0.51775868,6.21228027));
#165772=CARTESIAN_POINT('Ctrl Pts',(3.833453187,0.535714286,6.153627927));
#165773=CARTESIAN_POINT('Ctrl Pts',(3.876971864,0.544013736,6.126517609));
#165774=CARTESIAN_POINT('Ctrl Pts',(3.920102756,0.552339147,6.098794502));
#165775=CARTESIAN_POINT('Ctrl Pts',(3.704784445,0.499686101,6.284279802));
#165776=CARTESIAN_POINT('Ctrl Pts',(3.80093476,0.51775868,6.227596108));
#165777=CARTESIAN_POINT('Ctrl Pts',(3.895305939,0.535714286,6.16799741));
#165778=CARTESIAN_POINT('Ctrl Pts',(3.938926237,0.544013736,6.140449667));
#165779=CARTESIAN_POINT('Ctrl Pts',(3.982152555,0.552339147,6.112287742));
#165780=CARTESIAN_POINT('Ctrl Pts',(3.91848455882013,0.552026827314291,
6.09983432216034));
#165781=CARTESIAN_POINT('Ctrl Pts',(3.92127351299936,0.551172308244916,
6.10425018632747));
#165782=CARTESIAN_POINT('Ctrl Pts',(3.92406195243446,0.550320534932904,
6.10866690107976));
#165783=CARTESIAN_POINT('Ctrl Pts',(3.92684987915185,0.549471478043595,
6.11308446061508));
#165784=CARTESIAN_POINT('Ctrl Pts',(3.92943808477059,0.548683245771267,
6.11718555564713));
#165785=CARTESIAN_POINT('Ctrl Pts',(3.93202584919722,0.547897354461127,
6.12128737986063));
#165786=CARTESIAN_POINT('Ctrl Pts',(3.93461317544761,0.547113782415644,
6.12538992263642));
#165787=CARTESIAN_POINT('Ctrl Pts',(3.93720050431235,0.546330209578404,
6.1294924695576));
#165788=CARTESIAN_POINT('Ctrl Pts',(3.93978739565186,0.545548955813255,
6.13359573607793));
#165789=CARTESIAN_POINT('Ctrl Pts',(3.94237385365378,0.544769999912963,
6.13769971114459));
#165790=CARTESIAN_POINT('Ctrl Pts',(3.916896932,0.55233793,6.100853909));
#165791=CARTESIAN_POINT('Ctrl Pts',(4.050970176,0.526068113,6.014775618));
#165792=CARTESIAN_POINT('Ctrl Pts',(4.181132469,0.49968693,5.922890449));
#165793=CARTESIAN_POINT('Ctrl Pts',(3.903371084,0.55233793,6.162896608));
#165794=CARTESIAN_POINT('Ctrl Pts',(4.038807786,0.526068113,6.077115563));
#165795=CARTESIAN_POINT('Ctrl Pts',(4.170345281,0.49968693,5.985467455));
#165796=CARTESIAN_POINT('Origin',(-0.125384577725371,0.410742960799487,
-0.152064775049904));
#165797=CARTESIAN_POINT('Ctrl Pts',(3.98788411345982,0.552548454735263,
6.11726746511525));
#165798=CARTESIAN_POINT('Ctrl Pts',(3.98921839172991,0.552287640367631,
6.11639681105762));
#165799=CARTESIAN_POINT('Ctrl Pts',(3.99055267,0.552026826,6.115526157));
#165800=CARTESIAN_POINT('Ctrl Pts',(4.124152185,0.525911829,6.02834872));
#165801=CARTESIAN_POINT('Ctrl Pts',(4.253817109,0.49968693,5.935420018));
#165802=CARTESIAN_POINT('Ctrl Pts',(3.91581102107496,0.552548454735263,
6.10154160681932));
#165803=CARTESIAN_POINT('Ctrl Pts',(3.91714187514867,0.552287640367631,
6.10068667906915));
#165804=CARTESIAN_POINT('Ctrl Pts',(3.91847272922237,0.552026826,6.09983175131896));
#165805=CARTESIAN_POINT('Ctrl Pts',(4.05172938397585,0.525911829,6.01422896864239));
#165806=CARTESIAN_POINT('Ctrl Pts',(4.18112054306447,0.49968693,5.92288839317594));
#165807=CARTESIAN_POINT('',(4.02572813609744,0.552026824384634,6.12318513352432));
#165808=CARTESIAN_POINT('Ctrl Pts',(3.91187548180337,0.550751630586318,
6.10407886133619));
#165809=CARTESIAN_POINT('Ctrl Pts',(3.91517939102832,0.551389228293159,
6.10195645717512));
#165810=CARTESIAN_POINT('Ctrl Pts',(3.91848330025327,0.552026826,6.09983405301406));
#165811=CARTESIAN_POINT('Ctrl Pts',(4.25077575638218,0.61615356,5.88637210731273));
#165812=CARTESIAN_POINT('Ctrl Pts',(4.55791368301831,0.681389364000001,
5.63807677382268));
#165813=CARTESIAN_POINT('Ctrl Pts',(4.12631332540522,0.550751630586317,
6.15101308899582));
#165814=CARTESIAN_POINT('Ctrl Pts',(4.12964253020261,0.551389228293159,
6.14877450949791));
#165815=CARTESIAN_POINT('Ctrl Pts',(4.132971735,0.552026826,6.14653593));
#165816=CARTESIAN_POINT('Ctrl Pts',(4.467808307,0.61615356,5.921389587));
#165817=CARTESIAN_POINT('Ctrl Pts',(4.77620603,0.681389364000001,5.661202634));
#165818=CARTESIAN_POINT('Ctrl Pts',(4.55424020909657,0.680609082247605,
5.6410456839352));
#165819=CARTESIAN_POINT('Ctrl Pts',(4.56573507336456,0.677652752657951,
5.65499942765426));
#165820=CARTESIAN_POINT('Ctrl Pts',(4.57723334628363,0.674729896804321,
5.66895751963912));
#165821=CARTESIAN_POINT('Ctrl Pts',(4.58872215690221,0.671836782415114,
5.682929512709));
#165822=CARTESIAN_POINT('Ctrl Pts',(4.599477439182,0.669128385266211,5.69600943320442));
#165823=CARTESIAN_POINT('Ctrl Pts',(4.6102277011599,0.666446714392474,5.7090990456675));
#165824=CARTESIAN_POINT('Ctrl Pts',(4.62097308339939,0.663790956053537,
5.72219788303472));
#165825=CARTESIAN_POINT('Ctrl Pts',(4.63171858100736,0.661135169200881,
5.73529686103845));
#165826=CARTESIAN_POINT('Ctrl Pts',(4.64245922725447,0.658505288528707,
5.74840509909306));
#165827=CARTESIAN_POINT('Ctrl Pts',(4.65319515451439,0.655900535591315,
5.76152215973136));
#165828=CARTESIAN_POINT('Ctrl Pts',(4.550585316,0.681369595,5.643994444));
#165829=CARTESIAN_POINT('Ctrl Pts',(4.557312103,0.679970133,5.638570835));
#165830=CARTESIAN_POINT('Ctrl Pts',(4.564025943,0.678571429,5.633131207));
#165831=CARTESIAN_POINT('Ctrl Pts',(4.864933514,0.615882895,5.389332525));
#165832=CARTESIAN_POINT('Ctrl Pts',(5.138156632,0.552026826,5.11486524));
#165833=CARTESIAN_POINT('Ctrl Pts',(4.52717597500001,0.681369595,5.862255283));
#165834=CARTESIAN_POINT('Ctrl Pts',(4.534162896,0.679970133,5.856859574));
#165835=CARTESIAN_POINT('Ctrl Pts',(4.541136935,0.678571429,5.851447226));
#165836=CARTESIAN_POINT('Ctrl Pts',(4.853706394,0.615882895,5.608871218));
#165837=CARTESIAN_POINT('Ctrl Pts',(5.138655289,0.552026826,5.334377295));
#165838=CARTESIAN_POINT('',(5.13824039993051,0.552026824384634,5.15174348905096));
#165839=CARTESIAN_POINT('Ctrl Pts',(4.902547666,0.499686101,5.41194948));
#165840=CARTESIAN_POINT('Ctrl Pts',(4.985351212,0.51775868,5.33693985));
#165841=CARTESIAN_POINT('Ctrl Pts',(5.065821221,0.535714286,5.259432113));
#165842=CARTESIAN_POINT('Ctrl Pts',(5.102318391,0.54385805,5.224278481));
#165843=CARTESIAN_POINT('Ctrl Pts',(5.138324182,0.552026826,5.188621724));
#165844=CARTESIAN_POINT('Ctrl Pts',(4.905659624,0.499686101,5.338258485));
#165845=CARTESIAN_POINT('Ctrl Pts',(4.987335687,0.51775868,5.263201242));
#165846=CARTESIAN_POINT('Ctrl Pts',(5.066677286,0.535714286,5.185680407));
#165847=CARTESIAN_POINT('Ctrl Pts',(5.102662666,0.54385805,5.150520834));
#165848=CARTESIAN_POINT('Ctrl Pts',(5.138156632,0.552026826,5.11486524));
#165849=CARTESIAN_POINT('Ctrl Pts',(5.13815663264052,0.552026826325034,
5.11486523962076));
#165850=CARTESIAN_POINT('Ctrl Pts',(5.11447662501153,0.546576979803649,
5.13865307809982));
#165851=CARTESIAN_POINT('Ctrl Pts',(5.09064879432901,0.541139220286672,
5.1622590064672));
#165852=CARTESIAN_POINT('Ctrl Pts',(5.06667728595784,0.535714285990458,
5.1856804070412));
#165853=CARTESIAN_POINT('Ctrl Pts',(5.01433181580309,0.523868108829625,
5.23682463158345));
#165854=CARTESIAN_POINT('Ctrl Pts',(4.96112242201154,0.511960760879927,
5.28726340536358));
#165855=CARTESIAN_POINT('Ctrl Pts',(4.90707810144185,0.499999999671717,
5.3369546096604));
#165856=CARTESIAN_POINT('Ctrl Pts',(4.905659624,0.499686101,5.338258485));
#165857=CARTESIAN_POINT('Ctrl Pts',(4.987335687,0.51775868,5.263201242));
#165858=CARTESIAN_POINT('Ctrl Pts',(5.066677286,0.535714286,5.185680407));
#165859=CARTESIAN_POINT('Ctrl Pts',(5.103350603,0.544013736,5.149848684));
#165860=CARTESIAN_POINT('Ctrl Pts',(5.139513471,0.552339147,5.113501861));
#165861=CARTESIAN_POINT('Ctrl Pts',(4.969103039,0.499686101,5.340937689));
#165862=CARTESIAN_POINT('Ctrl Pts',(5.050820094,0.51775868,5.264909753));
#165863=CARTESIAN_POINT('Ctrl Pts',(5.130172969,0.535714286,5.186417426));
#165864=CARTESIAN_POINT('Ctrl Pts',(5.166851499,0.544013736,5.15013665899999));
#165865=CARTESIAN_POINT('Ctrl Pts',(5.203013228,0.552339147,5.113340763));
#165866=CARTESIAN_POINT('Ctrl Pts',(5.13815663689923,0.552026827305158,
5.11486523534265));
#165867=CARTESIAN_POINT('Ctrl Pts',(5.14182966686511,0.551172308293672,
5.11857831599279));
#165868=CARTESIAN_POINT('Ctrl Pts',(5.14550237726308,0.550320534953802,
5.12229233838852));
#165869=CARTESIAN_POINT('Ctrl Pts',(5.14917476853448,0.549471478040705,
5.12600729603646));
#165870=CARTESIAN_POINT('Ctrl Pts',(5.15258407752835,0.548683245753838,
5.12945612204244));
#165871=CARTESIAN_POINT('Ctrl Pts',(5.15599311239802,0.547897354432532,
5.13290575502544));
#165872=CARTESIAN_POINT('Ctrl Pts',(5.15940187380592,0.547113782378707,
5.13635618396623));
#165873=CARTESIAN_POINT('Ctrl Pts',(5.16281063865819,0.546330209533124,
5.1398066163935));
#165874=CARTESIAN_POINT('Ctrl Pts',(5.16621913090739,0.545548955762417,
5.1432578456512));
#165875=CARTESIAN_POINT('Ctrl Pts',(5.16962735214875,0.544769999814018,
5.14670986024279));
#165876=CARTESIAN_POINT('Ctrl Pts',(5.136825309,0.552337930000001,5.116202277));
#165877=CARTESIAN_POINT('Ctrl Pts',(5.249259707,0.526068113,5.00331466500001));
#165878=CARTESIAN_POINT('Ctrl Pts',(5.356626283,0.49968693,4.885596675));
#165879=CARTESIAN_POINT('Ctrl Pts',(5.136953033,0.552337930000001,5.17970211));
#165880=CARTESIAN_POINT('Ctrl Pts',(5.250782913,0.526068113,5.06681169));
#165881=CARTESIAN_POINT('Ctrl Pts',(5.359543499,0.49968693,4.949029591));
#165882=CARTESIAN_POINT('Origin',(-0.15514246281081,0.410743046427657,-0.121555536364255));
#165883=CARTESIAN_POINT('Ctrl Pts',(5.20968127961232,0.552548454735263,
5.11697194808294));
#165884=CARTESIAN_POINT('Ctrl Pts',(5.21079719830616,0.552287640367631,
5.11583481904148));
#165885=CARTESIAN_POINT('Ctrl Pts',(5.211913117,0.552026826,5.11469769000001));
#165886=CARTESIAN_POINT('Ctrl Pts',(5.323648577,0.525911829,5.000838466));
#165887=CARTESIAN_POINT('Ctrl Pts',(5.430305083,0.49968693,4.88220826));
#165888=CARTESIAN_POINT('Ctrl Pts',(5.13591261979726,0.552548454735263,
5.11710733610618));
#165889=CARTESIAN_POINT('Ctrl Pts',(5.13702857506005,0.552287640367631,
5.11598630179857));
#165890=CARTESIAN_POINT('Ctrl Pts',(5.13814453032285,0.552026826,5.11486526749095));
#165891=CARTESIAN_POINT('Ctrl Pts',(5.24988365192353,0.525911829,5.00261758786351));
#165892=CARTESIAN_POINT('Ctrl Pts',(5.35661419406909,0.49968693,4.88559723095795));
#165893=CARTESIAN_POINT('',(5.24791265298529,0.552026824385518,5.11461591869753));
#165894=CARTESIAN_POINT('Ctrl Pts',(5.13261580896174,0.550751630586318,
5.12043129408337));
#165895=CARTESIAN_POINT('Ctrl Pts',(5.13538622048087,0.551389228293159,
5.11764826704169));
#165896=CARTESIAN_POINT('Ctrl Pts',(5.138156632,0.552026826,5.11486524));
#165897=CARTESIAN_POINT('Ctrl Pts',(5.416792268,0.61615356,4.834960791));
#165898=CARTESIAN_POINT('Ctrl Pts',(5.663373315,0.681389364000001,4.526444819));
#165899=CARTESIAN_POINT('Ctrl Pts',(5.35212840517261,0.550751630586318,
5.12017042975023));
#165900=CARTESIAN_POINT('Ctrl Pts',(5.3548985465863,0.551389228293159,5.11726850637512));
#165901=CARTESIAN_POINT('Ctrl Pts',(5.357668688,0.552026826,5.11436658300001));
#165902=CARTESIAN_POINT('Ctrl Pts',(5.636277158,0.61615356,4.822504071));
#165903=CARTESIAN_POINT('Ctrl Pts',(5.88153221,0.681389364000001,4.50210375));
#165904=CARTESIAN_POINT('Ctrl Pts',(5.66042267728532,0.680609082247605,
4.53013414795068));
#165905=CARTESIAN_POINT('Ctrl Pts',(5.67464844079711,0.677652752733401,
4.54129060488698));
#165906=CARTESIAN_POINT('Ctrl Pts',(5.68887846756112,0.67472989689917,4.55245057562457));
#165907=CARTESIAN_POINT('Ctrl Pts',(5.70310224161805,0.6718367825388,4.56362615650412));
#165908=CARTESIAN_POINT('Ctrl Pts',(5.71641786775797,0.669128385382844,
4.57408820801682));
#165909=CARTESIAN_POINT('Ctrl Pts',(5.72973067445805,0.666446714501235,
4.58456080411605));
#165910=CARTESIAN_POINT('Ctrl Pts',(5.74304069858956,0.663790956153864,
4.59504345844241));
#165911=CARTESIAN_POINT('Ctrl Pts',(5.75635086562497,0.661135169292779,
4.60552622531643));
#165912=CARTESIAN_POINT('Ctrl Pts',(5.76965828536143,0.658505288611614,
4.61601907864229));
#165913=CARTESIAN_POINT('Ctrl Pts',(5.7829629925841,0.65590053576872,4.62652156291335));
#165914=CARTESIAN_POINT('Ctrl Pts',(5.65748713,0.681369595,4.533799662));
#165915=CARTESIAN_POINT('Ctrl Pts',(5.662890733,0.679970133,4.527056793));
#165916=CARTESIAN_POINT('Ctrl Pts',(5.668278248,0.678571429,4.520301063));
#165917=CARTESIAN_POINT('Ctrl Pts',(5.90974125700001,0.615882895,4.217516027));
#165918=CARTESIAN_POINT('Ctrl Pts',(6.11757421800001,0.552026826,3.89073074));
#165919=CARTESIAN_POINT('Ctrl Pts',(5.68154471500001,0.681369595,4.75199));
#165920=CARTESIAN_POINT('Ctrl Pts',(5.68720836800001,0.679970133,4.745218458));
#165921=CARTESIAN_POINT('Ctrl Pts',(5.692855864,0.678571429,4.738433436));
#165922=CARTESIAN_POINT('Ctrl Pts',(5.945970951,0.615882895,4.434335525));
#165923=CARTESIAN_POINT('Ctrl Pts',(6.16524982,0.552026826,4.105003528));
#165924=CARTESIAN_POINT('',(6.12558376061154,0.552026824384634,3.92672878840585));
#165925=CARTESIAN_POINT('Ctrl Pts',(5.951337988,0.499686101,4.231518279));
#165926=CARTESIAN_POINT('Ctrl Pts',(6.01608078,0.51775868,4.140462018));
#165927=CARTESIAN_POINT('Ctrl Pts',(6.078007573,0.535714286,4.047467695));
#165928=CARTESIAN_POINT('Ctrl Pts',(6.106094468,0.54385805,4.005290123));
#165929=CARTESIAN_POINT('Ctrl Pts',(6.133593314,0.552026826,3.96272682));
#165930=CARTESIAN_POINT('Ctrl Pts',(5.93853580499999,0.499686101,4.158881159));
#165931=CARTESIAN_POINT('Ctrl Pts',(6.002167238,0.51775868,4.068020773));
#165932=CARTESIAN_POINT('Ctrl Pts',(6.062989186,0.535714286,3.975256234));
#165933=CARTESIAN_POINT('Ctrl Pts',(6.090574979,0.54385805,3.93318288));
#165934=CARTESIAN_POINT('Ctrl Pts',(6.117574218,0.552026826,3.89073074));
#165935=CARTESIAN_POINT('Ctrl Pts',(6.11757421803917,0.552026826,3.89073074017603));
#165936=CARTESIAN_POINT('Ctrl Pts',(6.08891330648077,0.543355301187097,
3.93579560734626));
#165937=CARTESIAN_POINT('Ctrl Pts',(6.0597797826872,0.534726107642318,3.98050483233341));
#165938=CARTESIAN_POINT('Ctrl Pts',(6.00046156891768,0.517398613547625,
4.06937582139407));
#165939=CARTESIAN_POINT('Ctrl Pts',(5.97029013381289,0.508707842303121,
4.11351354118986));
#165940=CARTESIAN_POINT('Ctrl Pts',(5.93963516527631,0.499998391797793,
4.15731092236549));
#165941=CARTESIAN_POINT('Ctrl Pts',(5.93853580499999,0.499686101,4.158881159));
#165942=CARTESIAN_POINT('Ctrl Pts',(6.002167238,0.51775868,4.068020773));
#165943=CARTESIAN_POINT('Ctrl Pts',(6.062989186,0.535714286,3.975256234));
#165944=CARTESIAN_POINT('Ctrl Pts',(6.091102341,0.544013736,3.932378558));
#165945=CARTESIAN_POINT('Ctrl Pts',(6.118606248,0.552339147,3.889107555));
#165946=CARTESIAN_POINT('Ctrl Pts',(6.001071897,0.499686101,4.147859266));
#165947=CARTESIAN_POINT('Ctrl Pts',(6.064534695,0.51775868,4.05604207));
#165948=CARTESIAN_POINT('Ctrl Pts',(6.125158813,0.535714286,3.962326327));
#165949=CARTESIAN_POINT('Ctrl Pts',(6.153180527,0.544013736,3.919008985));
#165950=CARTESIAN_POINT('Ctrl Pts',(6.180586785,0.552339147,3.875299654));
#165951=CARTESIAN_POINT('Ctrl Pts',(6.11757422061379,0.552026827147516,
3.89073073448356));
#165952=CARTESIAN_POINT('Ctrl Pts',(6.12195958097685,0.551172308249902,
3.89356741198595));
#165953=CARTESIAN_POINT('Ctrl Pts',(6.12634483044024,0.550320534923268,
3.89640507858448));
#165954=CARTESIAN_POINT('Ctrl Pts',(6.13072996930273,0.549471478017472,
3.8992437271493));
#165955=CARTESIAN_POINT('Ctrl Pts',(6.13480096609976,0.548683245751088,
3.90187902093991));
#165956=CARTESIAN_POINT('Ctrl Pts',(6.13887186866908,0.54789735444499,3.9045151617502));
#165957=CARTESIAN_POINT('Ctrl Pts',(6.14294267528982,0.547113782401498,
3.90715213868288));
#165958=CARTESIAN_POINT('Ctrl Pts',(6.14701348601668,0.546330209567639,
3.90978911827541));
#165959=CARTESIAN_POINT('Ctrl Pts',(6.15108420182122,0.545548955803886,
3.91242693465806));
#165960=CARTESIAN_POINT('Ctrl Pts',(6.15515482213107,0.544770000002306,
3.91506557553979));
#165961=CARTESIAN_POINT('Ctrl Pts',(6.116561444,0.55233793,3.892322713));
#165962=CARTESIAN_POINT('Ctrl Pts',(6.202099688,0.526068113,3.757904278));
#165963=CARTESIAN_POINT('Ctrl Pts',(6.281650205,0.49968693,3.619857829));
#165964=CARTESIAN_POINT('Ctrl Pts',(6.130336769,0.55233793,3.954310498));
#165965=CARTESIAN_POINT('Ctrl Pts',(6.217237265,0.526068113,3.819589334));
#165966=CARTESIAN_POINT('Ctrl Pts',(6.29813542,0.49968693,3.681180604));
#165967=CARTESIAN_POINT('Origin',(-0.177646919336792,0.410743002151109,
-0.085363016941063));
#165968=CARTESIAN_POINT('Ctrl Pts',(6.18787953798209,0.552548454735263,
3.87741250926571));
#165969=CARTESIAN_POINT('Ctrl Pts',(6.18872491799105,0.552287640367631,
3.87606207613285));
#165970=CARTESIAN_POINT('Ctrl Pts',(6.189570298,0.552026826,3.874711643));
#165971=CARTESIAN_POINT('Ctrl Pts',(6.274217078,0.525911829,3.739494563));
#165972=CARTESIAN_POINT('Ctrl Pts',(6.352878027,0.49968693,3.60070987));
#165973=CARTESIAN_POINT('Ctrl Pts',(6.11586465391192,0.552548454735263,
3.89340281343582));
#165974=CARTESIAN_POINT('Ctrl Pts',(6.11671352951712,0.552287640367631,
3.89206809089803));
#165975=CARTESIAN_POINT('Ctrl Pts',(6.11756240512232,0.552026826,3.89073336836023));
#165976=CARTESIAN_POINT('Ctrl Pts',(6.20255919454128,0.525911829,3.7570893694238));
#165977=CARTESIAN_POINT('Ctrl Pts',(6.28163851817553,0.49968693,3.61986097073352));
#165978=CARTESIAN_POINT('',(6.22471060719365,0.552026824384635,3.86689294754188));
#165979=CARTESIAN_POINT('Ctrl Pts',(6.1133582207917,0.550751630586317,3.89735805329302));
#165980=CARTESIAN_POINT('Ctrl Pts',(6.11546559322124,0.551389228293159,
3.89404453597009));
#165981=CARTESIAN_POINT('Ctrl Pts',(6.1175729656508,0.552026826,3.89073101864715));
#165982=CARTESIAN_POINT('Ctrl Pts',(6.32952308683028,0.61615356,3.5574722228697));
#165983=CARTESIAN_POINT('Ctrl Pts',(6.50401741433089,0.681389364000001,
3.20316161303959));
#165984=CARTESIAN_POINT('Ctrl Pts',(6.32768390839934,0.550751630586317,
3.8499142910946));
#165985=CARTESIAN_POINT('Ctrl Pts',(6.32976545769968,0.551389228293159,
3.8464847145473));
#165986=CARTESIAN_POINT('Ctrl Pts',(6.331847007,0.552026826,3.843055138));
#165987=CARTESIAN_POINT('Ctrl Pts',(6.541199953,0.61615356,3.498123623));
#165988=CARTESIAN_POINT('Ctrl Pts',(6.71184448,0.681389364000001,3.132491498));
#165989=CARTESIAN_POINT('Ctrl Pts',(6.50193007241179,0.680609082082812,
3.20739857430726));
#165990=CARTESIAN_POINT('Ctrl Pts',(6.51822155404743,0.677652752690646,
3.21523608098733));
#165991=CARTESIAN_POINT('Ctrl Pts',(6.53451795468387,0.674729896901062,
3.22307610241689));
#165992=CARTESIAN_POINT('Ctrl Pts',(6.55081160437425,0.6718367825332,3.23093271345657));
#165993=CARTESIAN_POINT('Ctrl Pts',(6.56606495036792,0.669128385379044,
3.23828770198298));
#165994=CARTESIAN_POINT('Ctrl Pts',(6.58131780961128,0.666446714497193,
3.24565359466854));
#165995=CARTESIAN_POINT('Ctrl Pts',(6.59657011356126,0.663790956148093,
3.25302990859755));
#165996=CARTESIAN_POINT('Ctrl Pts',(6.61182258126854,0.66113516928528,3.26040630172281));
#165997=CARTESIAN_POINT('Ctrl Pts',(6.62707453419494,0.6585052886009,3.26779313607438));
#165998=CARTESIAN_POINT('Ctrl Pts',(6.64232590877187,0.655900535624813,
3.27518995864757));
#165999=CARTESIAN_POINT('Ctrl Pts',(6.499851134,0.681369595,3.211609446));
#166000=CARTESIAN_POINT('Ctrl Pts',(6.503678886,0.679970133000001,3.203862607));
#166001=CARTESIAN_POINT('Ctrl Pts',(6.507488162,0.678571429,3.196106666));
#166002=CARTESIAN_POINT('Ctrl Pts',(6.678216068,0.615882895,2.848493166));
#166003=CARTESIAN_POINT('Ctrl Pts',(6.81094083199999,0.552026826,2.484669994));
#166004=CARTESIAN_POINT('Ctrl Pts',(6.570250739,0.681369595,3.419526946));
#166005=CARTESIAN_POINT('Ctrl Pts',(6.574326298,0.679970133000001,3.411696201));
#166006=CARTESIAN_POINT('Ctrl Pts',(6.578383179,0.678571429,3.403855764));
#166007=CARTESIAN_POINT('Ctrl Pts',(6.76020851400001,0.615882895,3.052455232));
#166008=CARTESIAN_POINT('Ctrl Pts',(6.903564121,0.552026826,2.683684359));
#166009=CARTESIAN_POINT('',(6.82650163254454,0.552026824384641,2.51810461336765));
#166010=CARTESIAN_POINT('Ctrl Pts',(6.72185036,0.499686101,2.853225986));
#166011=CARTESIAN_POINT('Ctrl Pts',(6.76550509700001,0.51775868,2.750380783));
#166012=CARTESIAN_POINT('Ctrl Pts',(6.805993045,0.535714286,2.646248186));
#166013=CARTESIAN_POINT('Ctrl Pts',(6.824356353,0.54385805,2.59901885));
#166014=CARTESIAN_POINT('Ctrl Pts',(6.84206244,0.552026826,2.551539214));
#166015=CARTESIAN_POINT('Ctrl Pts',(6.693732651,0.499686101,2.785039173));
#166016=CARTESIAN_POINT('Ctrl Pts',(6.73634412,0.51775868,2.682624175));
#166017=CARTESIAN_POINT('Ctrl Pts',(6.775802451,0.535714286,2.578953498));
#166018=CARTESIAN_POINT('Ctrl Pts',(6.793698776,0.54385805,2.531933665));
#166019=CARTESIAN_POINT('Ctrl Pts',(6.81094083200001,0.552026826,2.484669994));
#166020=CARTESIAN_POINT('Ctrl Pts',(6.81094083261732,0.552026826308274,
2.48466999368684));
#166021=CARTESIAN_POINT('Ctrl Pts',(6.79943769339592,0.54657697978499,2.51620222876931));
#166022=CARTESIAN_POINT('Ctrl Pts',(6.78772401181845,0.541139220273715,
2.54763143566997));
#166023=CARTESIAN_POINT('Ctrl Pts',(6.77580245095149,0.535714285977923,
2.57895349812747));
#166024=CARTESIAN_POINT('Ctrl Pts',(6.74976989147918,0.5238681087781,2.64735003178684));
#166025=CARTESIAN_POINT('Ctrl Pts',(6.72265704507204,0.511960760856659,
2.71546906758587));
#166026=CARTESIAN_POINT('Ctrl Pts',(6.69447254313508,0.49999999963666,2.78326020476335));
#166027=CARTESIAN_POINT('Ctrl Pts',(6.693732651,0.499686101,2.785039173));
#166028=CARTESIAN_POINT('Ctrl Pts',(6.73634412,0.51775868,2.682624175));
#166029=CARTESIAN_POINT('Ctrl Pts',(6.775802451,0.535714286,2.578953498));
#166030=CARTESIAN_POINT('Ctrl Pts',(6.794040902,0.544013736,2.531034781));
#166031=CARTESIAN_POINT('Ctrl Pts',(6.811599798,0.552339147,2.482862903));
#166032=CARTESIAN_POINT('Ctrl Pts',(6.752437304,0.499686101,2.760831554));
#166033=CARTESIAN_POINT('Ctrl Pts',(6.794678393,0.51775868,2.657518367));
#166034=CARTESIAN_POINT('Ctrl Pts',(6.833739039,0.535714286,2.552961253));
#166035=CARTESIAN_POINT('Ctrl Pts',(6.851793672,0.544013736,2.504632806));
#166036=CARTESIAN_POINT('Ctrl Pts',(6.86916297300001,0.552339147,2.45605384));
#166037=CARTESIAN_POINT('Ctrl Pts',(6.81094083475798,0.552026827322456,
2.48466998781889));
#166038=CARTESIAN_POINT('Ctrl Pts',(6.81583346809674,0.551172308262818,
2.48649762393515));
#166039=CARTESIAN_POINT('Ctrl Pts',(6.82072620731759,0.550320534934142,
2.48832624838348));
#166040=CARTESIAN_POINT('Ctrl Pts',(6.82561904961501,0.549471478028082,
2.49015585562438));
#166041=CARTESIAN_POINT('Ctrl Pts',(6.8301613790905,0.548683245754012,2.49185439369157));
#166042=CARTESIAN_POINT('Ctrl Pts',(6.83470379862338,0.547897354441908,
2.49355377923814));
#166043=CARTESIAN_POINT('Ctrl Pts',(6.83924630418656,0.547113782394639,
2.49525400198954));
#166044=CARTESIAN_POINT('Ctrl Pts',(6.84378881433968,0.546330209555615,
2.49695422645892));
#166045=CARTESIAN_POINT('Ctrl Pts',(6.84833141166887,0.545548955788871,
2.49865528856461));
#166046=CARTESIAN_POINT('Ctrl Pts',(6.8528740929523,0.544769999918643,2.50035717676483));
#166047=CARTESIAN_POINT('Ctrl Pts',(6.810293963,0.55233793,2.486442465));
#166048=CARTESIAN_POINT('Ctrl Pts',(6.864936381,0.526068113,2.336778465));
#166049=CARTESIAN_POINT('Ctrl Pts',(6.912951145,0.49968693,2.184858455));
#166050=CARTESIAN_POINT('Ctrl Pts',(6.83707277,0.55233793,2.544019722));
#166051=CARTESIAN_POINT('Ctrl Pts',(6.892980514,0.526068113,2.393767227));
#166052=CARTESIAN_POINT('Ctrl Pts',(6.942233529,0.49968693,2.241203703));
#166053=CARTESIAN_POINT('Origin',(-0.191842828234754,0.410743194362546,
-0.045178034189591));
#166054=CARTESIAN_POINT('Ctrl Pts',(6.87673942742404,0.552548454735263,
2.45654957195124));
#166055=CARTESIAN_POINT('Ctrl Pts',(6.87727473971202,0.552287640367631,
2.45504897947562));
#166056=CARTESIAN_POINT('Ctrl Pts',(6.877810052,0.552026826,2.453548387));
#166057=CARTESIAN_POINT('Ctrl Pts',(6.93141016200001,0.525911829,2.303296051));
#166058=CARTESIAN_POINT('Ctrl Pts',(6.978397455,0.49968693,2.150846288));
#166059=CARTESIAN_POINT('Ctrl Pts',(6.80984565338549,0.552548454735263,
2.48764710157255));
#166060=CARTESIAN_POINT('Ctrl Pts',(6.81038775686044,0.552287640367631,
2.48616110094776));
#166061=CARTESIAN_POINT('Ctrl Pts',(6.8109298603354,0.552026826,2.48467510032297));
#166062=CARTESIAN_POINT('Ctrl Pts',(6.86520996288786,0.525911828999999,
2.33588382700963));
#166063=CARTESIAN_POINT('Ctrl Pts',(6.91294040680142,0.49968693,2.18486403559581));
#166064=CARTESIAN_POINT('',(6.91044801115398,0.552026824384643,2.43835835948284));
#166065=CARTESIAN_POINT('Ctrl Pts',(6.80824807877956,0.550751630586317,
2.49204867921741));
#166066=CARTESIAN_POINT('Ctrl Pts',(6.80959387373918,0.551389228293159,
2.48835960731475));
#166067=CARTESIAN_POINT('Ctrl Pts',(6.81093966869881,0.552026826,2.48467053541208));
#166068=CARTESIAN_POINT('Ctrl Pts',(6.94629372419259,0.61615356,2.11364013478368));
#166069=CARTESIAN_POINT('Ctrl Pts',(7.04054216339582,0.681389364000001,
1.73010198757639));
#166070=CARTESIAN_POINT('Ctrl Pts',(7.00736394446831,0.550751630586317,
2.39964043902942));
#166071=CARTESIAN_POINT('Ctrl Pts',(7.00865957073415,0.551389228293159,
2.39584357251471));
#166072=CARTESIAN_POINT('Ctrl Pts',(7.009955197,0.552026826,2.392046706));
#166073=CARTESIAN_POINT('Ctrl Pts',(7.140263509,0.61615356,2.010174804));
#166074=CARTESIAN_POINT('Ctrl Pts',(7.228318362,0.681389364000001,1.616407425));
#166075=CARTESIAN_POINT('Ctrl Pts',(7.03941444436854,0.680609082247612,
1.73468860817335));
#166076=CARTESIAN_POINT('Ctrl Pts',(7.05700987218025,0.67765275265413,1.73884069106667));
#166077=CARTESIAN_POINT('Ctrl Pts',(7.07461064485539,0.674729896832154,
1.74299417296873));
#166078=CARTESIAN_POINT('Ctrl Pts',(7.09221229723318,0.671836782470486,
1.74716444778147));
#166079=CARTESIAN_POINT('Ctrl Pts',(7.10869013358932,0.669128385327537,
1.7510684622711));
#166080=CARTESIAN_POINT('Ctrl Pts',(7.12516983864625,0.6664467144582,1.75498323062767));
#166081=CARTESIAN_POINT('Ctrl Pts',(7.14165124165079,0.663790956122426,
1.75890829596002));
#166082=CARTESIAN_POINT('Ctrl Pts',(7.15813282160895,0.661135169272935,
1.76283340343409));
#166083=CARTESIAN_POINT('Ctrl Pts',(7.17461614337578,0.658505288602688,
1.76676881869064));
#166084=CARTESIAN_POINT('Ctrl Pts',(7.19110104737666,0.655900535702375,
1.77071411332688));
#166085=CARTESIAN_POINT('Ctrl Pts',(7.038289323,0.681369595,1.739247943));
#166086=CARTESIAN_POINT('Ctrl Pts',(7.040362243,0.679970133000001,1.730859367));
#166087=CARTESIAN_POINT('Ctrl Pts',(7.042415162,0.678571429,1.722465874));
#166088=CARTESIAN_POINT('Ctrl Pts',(7.134424917,0.615882895,1.346277931));
#166089=CARTESIAN_POINT('Ctrl Pts',(7.185835423,0.552026826,0.962428841999999));
#166090=CARTESIAN_POINT('Ctrl Pts',(7.15173914100001,0.681369595,1.927170612));
#166091=CARTESIAN_POINT('Ctrl Pts',(7.154036037,0.679970133000001,1.918646822));
#166092=CARTESIAN_POINT('Ctrl Pts',(7.156312608,0.678571429,1.91011758));
#166093=CARTESIAN_POINT('Ctrl Pts',(7.258346241,0.615882895,1.527845525));
#166094=CARTESIAN_POINT('Ctrl Pts',(7.319075436,0.552026826,1.136879092));
#166095=CARTESIAN_POINT('',(7.20821987513909,0.552026824384642,0.991736666391452));
#166096=CARTESIAN_POINT('Ctrl Pts',(7.178056481,0.499686101,1.341520017));
#166097=CARTESIAN_POINT('Ctrl Pts',(7.198581915,0.51775868,1.2316948));
#166098=CARTESIAN_POINT('Ctrl Pts',(7.215737847,0.535714286,1.121293053));
#166099=CARTESIAN_POINT('Ctrl Pts',(7.22351891999999,0.54385805,1.071220344));
#166100=CARTESIAN_POINT('Ctrl Pts',(7.23060433,0.552026826,1.021044471));
#166101=CARTESIAN_POINT('Ctrl Pts',(7.135937999,0.499686101,1.28097185));
#166102=CARTESIAN_POINT('Ctrl Pts',(7.155537038,0.51775868,1.171791051));
#166103=CARTESIAN_POINT('Ctrl Pts',(7.171786724,0.535714286,1.062061763));
#166104=CARTESIAN_POINT('Ctrl Pts',(7.179156768,0.54385805,1.012294047));
#166105=CARTESIAN_POINT('Ctrl Pts',(7.185835423,0.552026826,0.962428842));
#166106=CARTESIAN_POINT('Ctrl Pts',(7.18583542290858,0.552026826224196,
0.962428841470711));
#166107=CARTESIAN_POINT('Ctrl Pts',(7.18137971978687,0.546576979749282,
0.995696704485362));
#166108=CARTESIAN_POINT('Ctrl Pts',(7.17669624816509,0.541139220265819,
1.02890920921096));
#166109=CARTESIAN_POINT('Ctrl Pts',(7.17178672409763,0.535714286068517,
1.06206176255485));
#166110=CARTESIAN_POINT('Ctrl Pts',(7.16106602474232,0.523868109155108,
1.13445545159152));
#166111=CARTESIAN_POINT('Ctrl Pts',(7.14923064057945,0.511960761034125,
1.20681036385961));
#166112=CARTESIAN_POINT('Ctrl Pts',(7.13627816756703,0.499999999904053,
1.27907541649017));
#166113=CARTESIAN_POINT('Ctrl Pts',(7.135937999,0.499686101,1.28097185));
#166114=CARTESIAN_POINT('Ctrl Pts',(7.155537038,0.51775868,1.171791051));
#166115=CARTESIAN_POINT('Ctrl Pts',(7.171786724,0.535714286,1.062061763));
#166116=CARTESIAN_POINT('Ctrl Pts',(7.179297663,0.544013736,1.01134263));
#166117=CARTESIAN_POINT('Ctrl Pts',(7.186090511,0.552339147,0.960522341));
#166118=CARTESIAN_POINT('Ctrl Pts',(7.188066246,0.499686101,1.244710427));
#166119=CARTESIAN_POINT('Ctrl Pts',(7.20711048100001,0.51775868,1.13473206));
#166120=CARTESIAN_POINT('Ctrl Pts',(7.222781222,0.535714286,1.024222548));
#166121=CARTESIAN_POINT('Ctrl Pts',(7.230024561,0.544013736,0.973142781));
#166122=CARTESIAN_POINT('Ctrl Pts',(7.236544735,0.552339147,0.921965678));
#166123=CARTESIAN_POINT('Ctrl Pts',(7.18583542372051,0.55202682721728,0.962428835408557));
#166124=CARTESIAN_POINT('Ctrl Pts',(7.19100655813224,0.551172308295944,
0.963161969826103));
#166125=CARTESIAN_POINT('Ctrl Pts',(7.1961780079224,0.550320534986493,0.96389604776062));
#166126=CARTESIAN_POINT('Ctrl Pts',(7.20134976964962,0.549471478100325,
0.964631063358087));
#166127=CARTESIAN_POINT('Ctrl Pts',(7.20615103750445,0.548683245820979,
0.96531342402106));
#166128=CARTESIAN_POINT('Ctrl Pts',(7.21095257549354,0.547897354504228,
0.965996592995543));
#166129=CARTESIAN_POINT('Ctrl Pts',(7.21575437747613,0.547113782451772,
0.966680561105015));
#166130=CARTESIAN_POINT('Ctrl Pts',(7.22055618431066,0.546330209607562,
0.967364529905598));
#166131=CARTESIAN_POINT('Ctrl Pts',(7.2253582563504,0.545548955835064,0.968049298016219));
#166132=CARTESIAN_POINT('Ctrl Pts',(7.23016058789743,0.544769999904026,
0.968734855199174));
#166133=CARTESIAN_POINT('Ctrl Pts',(7.185584706,0.55233793,0.96429893));
#166134=CARTESIAN_POINT('Ctrl Pts',(7.206776278,0.526068113,0.806387487));
#166135=CARTESIAN_POINT('Ctrl Pts',(7.221010173,0.49968693,0.647697528000001));
#166136=CARTESIAN_POINT('Ctrl Pts',(7.22411484800001,0.55233793,1.014773411));
#166137=CARTESIAN_POINT('Ctrl Pts',(7.246415654,0.526068113,0.856015224000001));
#166138=CARTESIAN_POINT('Ctrl Pts',(7.261720514,0.49968693,0.696430608));
#166139=CARTESIAN_POINT('Origin',(-0.19707097630675,0.410743212774269,-0.00288142655035101));
#166140=CARTESIAN_POINT('Ctrl Pts',(7.24405062408982,0.552548454735263,
0.920821105528827));
#166141=CARTESIAN_POINT('Ctrl Pts',(7.24425083804491,0.552287640367631,
0.919240519764414));
#166142=CARTESIAN_POINT('Ctrl Pts',(7.244451052,0.552026826,0.917659933999999));
#166143=CARTESIAN_POINT('Ctrl Pts',(7.26449821,0.525911829,0.759397976));
#166144=CARTESIAN_POINT('Ctrl Pts',(7.277614774,0.49968693,0.600411524));
#166145=CARTESIAN_POINT('Ctrl Pts',(7.18540583920389,0.552548454735263,
0.965571777466926));
#166146=CARTESIAN_POINT('Ctrl Pts',(7.18561582239313,0.552287640367631,
0.964003982485016));
#166147=CARTESIAN_POINT('Ctrl Pts',(7.18582580558238,0.552026826,0.962436187503104));
#166148=CARTESIAN_POINT('Ctrl Pts',(7.20685114405198,0.525911829,0.805454953604712));
#166149=CARTESIAN_POINT('Ctrl Pts',(7.22100088554379,0.49968693,0.647705286498134));
#166150=CARTESIAN_POINT('',(7.27306054677073,0.552026824384643,0.895808845480426));
#166151=CARTESIAN_POINT('Ctrl Pts',(7.18479182409675,0.550751630586318,
0.970213879985565));
#166152=CARTESIAN_POINT('Ctrl Pts',(7.18531311370807,0.551389228293159,
0.966321750393941));
#166153=CARTESIAN_POINT('Ctrl Pts',(7.18583440331938,0.552026826,0.962429620802318));
#166154=CARTESIAN_POINT('Ctrl Pts',(7.23826338774514,0.61615356,0.570976583350089));
#166155=CARTESIAN_POINT('Ctrl Pts',(7.24785898595394,0.681389364,0.17614471596048));
#166156=CARTESIAN_POINT('Ctrl Pts',(7.3593874306487,0.550751630586318,0.837162067481765));
#166157=CARTESIAN_POINT('Ctrl Pts',(7.35983655182435,0.551389228293159,
0.833175448240883));
#166158=CARTESIAN_POINT('Ctrl Pts',(7.360285673,0.552026826,0.829188829000001));
#166159=CARTESIAN_POINT('Ctrl Pts',(7.405456278,0.61615356,0.428232444));
#166160=CARTESIAN_POINT('Ctrl Pts',(7.406804111,0.681389364,0.024741937));
#166161=CARTESIAN_POINT('Ctrl Pts',(7.24774362022223,0.680609082082813,
0.180866530342211));
#166162=CARTESIAN_POINT('Ctrl Pts',(7.26582025148185,0.677652752743715,
0.181139042606722));
#166163=CARTESIAN_POINT('Ctrl Pts',(7.28390240363902,0.674729896880472,
0.181411772860856));
#166164=CARTESIAN_POINT('Ctrl Pts',(7.30198902492249,0.671836782520085,
0.181700714026023));
#166165=CARTESIAN_POINT('Ctrl Pts',(7.31892086638184,0.669128385362535,
0.181971207111659));
#166166=CARTESIAN_POINT('Ctrl Pts',(7.33585684461614,0.666446714477168,
0.182251800924234));
#166167=CARTESIAN_POINT('Ctrl Pts',(7.35279669464631,0.663790956124307,
0.182542085962166));
#166168=CARTESIAN_POINT('Ctrl Pts',(7.36973672655222,0.661135169257735,
0.182832374116761));
#166169=CARTESIAN_POINT('Ctrl Pts',(7.38668067541274,0.65850528856935,0.183132354621936));
#166170=CARTESIAN_POINT('Ctrl Pts',(7.40362829346862,0.655900535690581,
0.183441643835477));
#166171=CARTESIAN_POINT('Ctrl Pts',(7.247624926,0.681369595,0.185561138));
#166172=CARTESIAN_POINT('Ctrl Pts',(7.247846087,0.679970133000001,0.176923066));
#166173=CARTESIAN_POINT('Ctrl Pts',(7.248046656,0.678571429,0.168284491));
#166174=CARTESIAN_POINT('Ctrl Pts',(7.257035987,0.615882895,-0.218887764));
#166175=CARTESIAN_POINT('Ctrl Pts',(7.224728336,0.552026826,-0.604814414));
#166176=CARTESIAN_POINT('Ctrl Pts',(7.398820169,0.681369595,0.344701923));
#166177=CARTESIAN_POINT('Ctrl Pts',(7.399231002,0.679970133000001,0.335883649));
#166178=CARTESIAN_POINT('Ctrl Pts',(7.399620813,0.678571429,0.327064421));
#166179=CARTESIAN_POINT('Ctrl Pts',(7.417091764,0.615882895,-0.068204541));
#166180=CARTESIAN_POINT('Ctrl Pts',(7.39235491900001,0.552026826,-0.463085377));
#166181=CARTESIAN_POINT('',(7.25288976829728,0.552026824384642,-0.58100378604725));
#166182=CARTESIAN_POINT('Ctrl Pts',(7.298624658,0.499686101,-0.232913937));
#166183=CARTESIAN_POINT('Ctrl Pts',(7.295061043,0.51775868,-0.344583863));
#166184=CARTESIAN_POINT('Ctrl Pts',(7.288082768,0.535714286,-0.456092497));
#166185=CARTESIAN_POINT('Ctrl Pts',(7.28491777100001,0.54385805,-0.506667235));
#166186=CARTESIAN_POINT('Ctrl Pts',(7.281051199,0.552026826,-0.557193178));
#166187=CARTESIAN_POINT('Ctrl Pts',(7.244474816,0.499686101,-0.282992293));
#166188=CARTESIAN_POINT('Ctrl Pts',(7.240144997,0.51775868,-0.393833719));
#166189=CARTESIAN_POINT('Ctrl Pts',(7.23242622,0.535714286,-0.5044908));
#166190=CARTESIAN_POINT('Ctrl Pts',(7.22892537,0.54385805,-0.554679316));
#166191=CARTESIAN_POINT('Ctrl Pts',(7.224728336,0.552026826,-0.604814414));
#166192=CARTESIAN_POINT('Ctrl Pts',(7.22472833621218,0.552026825690736,
-0.604814410755777));
#166193=CARTESIAN_POINT('Ctrl Pts',(7.22752841142424,0.54657697938733,-0.571366488107131));
#166194=CARTESIAN_POINT('Ctrl Pts',(7.23009414317034,0.541139220081692,
-0.537923666472421));
#166195=CARTESIAN_POINT('Ctrl Pts',(7.23242622016378,0.535714285974483,
-0.504490800018465));
#166196=CARTESIAN_POINT('Ctrl Pts',(7.23751866907381,0.523868108761501,
-0.431484999794813));
#166197=CARTESIAN_POINT('Ctrl Pts',(7.24151415645778,0.51196076084533,-0.358277448234718));
#166198=CARTESIAN_POINT('Ctrl Pts',(7.24439935455547,0.499999999619591,
-0.284917513379212));
#166199=CARTESIAN_POINT('Ctrl Pts',(7.244474816,0.499686101,-0.282992293));
#166200=CARTESIAN_POINT('Ctrl Pts',(7.240144997,0.51775868,-0.393833719));
#166201=CARTESIAN_POINT('Ctrl Pts',(7.23242622,0.535714286,-0.5044908));
#166202=CARTESIAN_POINT('Ctrl Pts',(7.228858443,0.544013736,-0.555638777));
#166203=CARTESIAN_POINT('Ctrl Pts',(7.224567619,0.552339147,-0.606731178));
#166204=CARTESIAN_POINT('Ctrl Pts',(7.287589201,0.499686101,-0.329611976));
#166205=CARTESIAN_POINT('Ctrl Pts',(7.282546094,0.51775868,-0.441113058));
#166206=CARTESIAN_POINT('Ctrl Pts',(7.274094183,0.535714286,-0.552407665));
#166207=CARTESIAN_POINT('Ctrl Pts',(7.270187536,0.544013736,-0.603850319));
#166208=CARTESIAN_POINT('Ctrl Pts',(7.265553708,0.552339147,-0.655232575));
#166209=CARTESIAN_POINT('Ctrl Pts',(7.22472833538008,0.552026827310272,
-0.604814420695526));
#166210=CARTESIAN_POINT('Ctrl Pts',(7.22993617385133,0.551172308278917,
-0.605210067129426));
#166211=CARTESIAN_POINT('Ctrl Pts',(7.2351445231257,0.550320534943619,-0.605604860412332));
#166212=CARTESIAN_POINT('Ctrl Pts',(7.24035337861515,0.549471478034166,
-0.605998805004023));
#166213=CARTESIAN_POINT('Ctrl Pts',(7.24518908277755,0.548683245755601,
-0.606364528243161));
#166214=CARTESIAN_POINT('Ctrl Pts',(7.25002522452255,0.547897354441788,
-0.606729520133145));
#166215=CARTESIAN_POINT('Ctrl Pts',(7.25486179588049,0.547113782394678,
-0.607093788313525));
#166216=CARTESIAN_POINT('Ctrl Pts',(7.25969837212551,0.546330209555811,
-0.607458056861978));
#166217=CARTESIAN_POINT('Ctrl Pts',(7.26453537920458,0.545548955791126,
-0.607821601790319));
#166218=CARTESIAN_POINT('Ctrl Pts',(7.26937280931071,0.544769999981471,
-0.608184432575306));
#166219=CARTESIAN_POINT('Ctrl Pts',(7.224885495,0.55233793,-0.60293415));
#166220=CARTESIAN_POINT('Ctrl Pts',(7.211635327,0.526068113,-0.761709274));
#166221=CARTESIAN_POINT('Ctrl Pts',(7.19142279,0.49968693,-0.919749016));
#166222=CARTESIAN_POINT('Ctrl Pts',(7.273365344,0.55233793,-0.561922576));
#166223=CARTESIAN_POINT('Ctrl Pts',(7.261016453,0.526068113,-0.721763100000001));
#166224=CARTESIAN_POINT('Ctrl Pts',(7.241657518,0.49968693,-0.880906808));
#166225=CARTESIAN_POINT('Origin',(-0.193082213202791,0.410742918316382,
0.0395503751822959));
#166226=CARTESIAN_POINT('Ctrl Pts',(7.2726380643031,0.552548454735263,-0.657963931735703));
#166227=CARTESIAN_POINT('Ctrl Pts',(7.27249381815155,0.552287640367631,
-0.659550604367851));
#166228=CARTESIAN_POINT('Ctrl Pts',(7.272349572,0.552026826,-0.661137277));
#166229=CARTESIAN_POINT('Ctrl Pts',(7.257906396,0.525911829,-0.820008705));
#166230=CARTESIAN_POINT('Ctrl Pts',(7.236538914,0.49968693,-0.978097815));
#166231=CARTESIAN_POINT('Ctrl Pts',(7.22498443381837,0.552548454735263,
-0.601652610755724));
#166232=CARTESIAN_POINT('Ctrl Pts',(7.22485247814092,0.552287640367631,
-0.603228891742362));
#166233=CARTESIAN_POINT('Ctrl Pts',(7.22472052246348,0.552026826,-0.604805172728999));
#166234=CARTESIAN_POINT('Ctrl Pts',(7.21150797534791,0.525911829,-0.762636099034893));
#166235=CARTESIAN_POINT('Ctrl Pts',(7.19141538749405,0.49968693,-0.919739442320051));
#166236=CARTESIAN_POINT('',(7.29559285494497,0.552026824384643,-0.688627695488655));
#166237=CARTESIAN_POINT('Ctrl Pts',(7.22538351839981,0.550751630586317,
-0.596988021858047));
#166238=CARTESIAN_POINT('Ctrl Pts',(7.2250559271999,0.551389228293159,-0.600901217929023));
#166239=CARTESIAN_POINT('Ctrl Pts',(7.224728336,0.552026826,-0.604814414));
#166240=CARTESIAN_POINT('Ctrl Pts',(7.191780674,0.61615356,-0.998386224));
#166241=CARTESIAN_POINT('Ctrl Pts',(7.116274695,0.681389364000001,-1.38604995));
#166242=CARTESIAN_POINT('Ctrl Pts',(7.36729414063743,0.550751630586317,
-0.764461072856926));
#166243=CARTESIAN_POINT('Ctrl Pts',(7.36687575631872,0.551389228293159,
-0.768451034928463));
#166244=CARTESIAN_POINT('Ctrl Pts',(7.366457372,0.552026826,-0.772440997));
#166245=CARTESIAN_POINT('Ctrl Pts',(7.32437814300001,0.61615356,-1.173733589));
#166246=CARTESIAN_POINT('Ctrl Pts',(7.238955932,0.681389364000001,-1.568080456));
#166247=CARTESIAN_POINT('Ctrl Pts',(7.11717635924934,0.680609082247611,
-1.38141266504748));
#166248=CARTESIAN_POINT('Ctrl Pts',(7.13488895149141,0.677652752755135,
-1.38503246517533));
#166249=CARTESIAN_POINT('Ctrl Pts',(7.15260698192933,0.674729896880673,
-1.38865323946184));
#166250=CARTESIAN_POINT('Ctrl Pts',(7.17033286187557,0.67183678251324,-1.39225914256789));
#166251=CARTESIAN_POINT('Ctrl Pts',(7.18692699430104,0.669128385351528,
-1.39563481891437));
#166252=CARTESIAN_POINT('Ctrl Pts',(7.20352733814618,0.666446714464127,
-1.39900151995733));
#166253=CARTESIAN_POINT('Ctrl Pts',(7.22013354659556,0.663790956110893,
-1.40235958866437));
#166254=CARTESIAN_POINT('Ctrl Pts',(7.23673993333856,0.661135169243937,
-1.40571769342553));
#166255=CARTESIAN_POINT('Ctrl Pts',(7.25335222903067,0.658505288556828,
-1.40906717445963));
#166256=CARTESIAN_POINT('Ctrl Pts',(7.26997010890117,0.655900535569512,
-1.41240835399411));
#166257=CARTESIAN_POINT('Ctrl Pts',(7.118069642,0.681369595,-1.376802299));
#166258=CARTESIAN_POINT('Ctrl Pts',(7.116428702,0.679970133000001,-1.385285961));
#166259=CARTESIAN_POINT('Ctrl Pts',(7.114767544,0.678571429,-1.393765687));
#166260=CARTESIAN_POINT('Ctrl Pts',(7.040316119,0.615882895,-1.77381851));
#166261=CARTESIAN_POINT('Ctrl Pts',(6.925800981,0.552026826,-2.14377722));
#166262=CARTESIAN_POINT('Ctrl Pts',(7.299940589,0.681369595,-1.253884645));
#166263=CARTESIAN_POINT('Ctrl Pts',(7.298446148,0.679970133000001,-1.262585069));
#166264=CARTESIAN_POINT('Ctrl Pts',(7.296930973,0.678571429,-1.271281907));
#166265=CARTESIAN_POINT('Ctrl Pts',(7.22902232,0.615882895,-1.661065438));
#166266=CARTESIAN_POINT('Ctrl Pts',(7.119976101,0.552026826,-2.04139649));
#166267=CARTESIAN_POINT('',(6.95842259591819,0.552026824384643,-2.12657714645134));
#166268=CARTESIAN_POINT('Ctrl Pts',(7.077917257,0.499686101,-1.796457094));
#166269=CARTESIAN_POINT('Ctrl Pts',(7.050431225,0.51775868,-1.904750168));
#166270=CARTESIAN_POINT('Ctrl Pts',(7.019645038,0.535714286,-2.012151669));
#166271=CARTESIAN_POINT('Ctrl Pts',(7.005681963,0.54385805,-2.060863616));
#166272=CARTESIAN_POINT('Ctrl Pts',(6.99104420499999,0.552026826,-2.109377092));
#166273=CARTESIAN_POINT('Ctrl Pts',(7.014268043,0.499686101,-1.833724031));
#166274=CARTESIAN_POINT('Ctrl Pts',(6.986211822,0.51775868,-1.941043263));
#166275=CARTESIAN_POINT('Ctrl Pts',(6.954885505,0.535714286,-2.047453934));
#166276=CARTESIAN_POINT('Ctrl Pts',(6.940677455,0.54385805,-2.095716491));
#166277=CARTESIAN_POINT('Ctrl Pts',(6.925800981,0.552026826,-2.14377722));
#166278=CARTESIAN_POINT('Ctrl Pts',(6.92580098083625,0.55202682637027,-2.14377722018393));
#166279=CARTESIAN_POINT('Ctrl Pts',(6.93572590766086,0.546576979840938,
-2.11171322393334));
#166280=CARTESIAN_POINT('Ctrl Pts',(6.94542087273066,0.541139220308697,
-2.07960383231208));
#166281=CARTESIAN_POINT('Ctrl Pts',(6.95488550522624,0.53571428595539,-2.04745393400787));
#166282=CARTESIAN_POINT('Ctrl Pts',(6.97555298415123,0.523868108737258,
-1.97724969495729));
#166283=CARTESIAN_POINT('Ctrl Pts',(6.99519251853477,0.511960760918926,
-1.9066126073206));
#166284=CARTESIAN_POINT('Ctrl Pts',(7.01378048014667,0.499999999730479,
-1.83558801947582));
#166285=CARTESIAN_POINT('Ctrl Pts',(7.014268043,0.499686101,-1.833724031));
#166286=CARTESIAN_POINT('Ctrl Pts',(6.986211822,0.51775868,-1.941043263));
#166287=CARTESIAN_POINT('Ctrl Pts',(6.954885505,0.535714286,-2.047453934));
#166288=CARTESIAN_POINT('Ctrl Pts',(6.94040583800001,0.544013736,-2.096639133));
#166289=CARTESIAN_POINT('Ctrl Pts',(6.925231974,0.552339147,-2.145614621));
#166290=CARTESIAN_POINT('Ctrl Pts',(7.04635258300001,0.499686101,-1.88852209));
#166291=CARTESIAN_POINT('Ctrl Pts',(7.017457945,0.51775868,-1.99633222));
#166292=CARTESIAN_POINT('Ctrl Pts',(6.985278584,0.535714286,-2.103207909));
#166293=CARTESIAN_POINT('Ctrl Pts',(6.970404623,0.544013736,-2.152608049));
#166294=CARTESIAN_POINT('Ctrl Pts',(6.954833465,0.552339147,-2.20179288));
#166295=CARTESIAN_POINT('Ctrl Pts',(6.92580097903057,0.552026827361778,
-2.14377722601744));
#166296=CARTESIAN_POINT('Ctrl Pts',(6.93080200909239,0.551172308314244,
-2.14528315383995));
#166297=CARTESIAN_POINT('Ctrl Pts',(6.9358037212145,0.550320534985776,-2.14678835817033));
#166298=CARTESIAN_POINT('Ctrl Pts',(6.94080611015387,0.549471478079757,
-2.14829284249159));
#166299=CARTESIAN_POINT('Ctrl Pts',(6.94545013861374,0.548683245800462,
-2.14968954876334));
#166300=CARTESIAN_POINT('Ctrl Pts',(6.95009475163883,0.547897354483067,
-2.15108563486804));
#166301=CARTESIAN_POINT('Ctrl Pts',(6.95473993980467,0.547113782430111,
-2.15248110655001));
#166302=CARTESIAN_POINT('Ctrl Pts',(6.9593851326642,0.546330209585403,-2.15387657964202));
#166303=CARTESIAN_POINT('Ctrl Pts',(6.96403090183774,0.545548955812596,
-2.1552714386612));
#166304=CARTESIAN_POINT('Ctrl Pts',(6.96867723771985,0.544769999946634,
-2.1566656908487));
#166305=CARTESIAN_POINT('Ctrl Pts',(6.926358667,0.55233793,-2.1419747));
#166306=CARTESIAN_POINT('Ctrl Pts',(6.879286323,0.526068113,-2.294189355));
#166307=CARTESIAN_POINT('Ctrl Pts',(6.825572471,0.49968693,-2.444189118));
#166308=CARTESIAN_POINT('Ctrl Pts',(6.982521361,0.55233793,-2.112343688));
#166309=CARTESIAN_POINT('Ctrl Pts',(6.936100192,0.526068113,-2.265792583));
#166310=CARTESIAN_POINT('Ctrl Pts',(6.882982665,0.49968693,-2.417054001));
#166311=CARTESIAN_POINT('Origin',(-0.180065547040584,0.41074306335028,0.0801325185607973));
#166312=CARTESIAN_POINT('Ctrl Pts',(6.96116503193409,0.552548454735263,
-2.20598330608988));
#166313=CARTESIAN_POINT('Ctrl Pts',(6.96068307046704,0.552287640367631,
-2.20750187454494));
#166314=CARTESIAN_POINT('Ctrl Pts',(6.96020110900001,0.552026826,-2.209020443));
#166315=CARTESIAN_POINT('Ctrl Pts',(6.911942946,0.525911829,-2.36107269));
#166316=CARTESIAN_POINT('Ctrl Pts',(6.857090538,0.49968693,-2.510872388));
#166317=CARTESIAN_POINT('Ctrl Pts',(6.92673078560947,0.552548454735263,
-2.14074439141193));
#166318=CARTESIAN_POINT('Ctrl Pts',(6.92626306117155,0.552287640367631,
-2.14225545325307));
#166319=CARTESIAN_POINT('Ctrl Pts',(6.92579533673362,0.552026826,-2.1437665150942));
#166320=CARTESIAN_POINT('Ctrl Pts',(6.87896270859259,0.525911829,-2.29506713478976));
#166321=CARTESIAN_POINT('Ctrl Pts',(6.82556729961327,0.49968693,-2.44417817681576));
#166322=CARTESIAN_POINT('',(6.97699134907502,0.552026824384643,-2.24086477042585));
#166323=CARTESIAN_POINT('Ctrl Pts',(6.92812268768848,0.550751630586317,
-2.13627351282754));
#166324=CARTESIAN_POINT('Ctrl Pts',(6.9269615345349,0.551389228293159,-2.14002479779588));
#166325=CARTESIAN_POINT('Ctrl Pts',(6.92580038138132,0.552026826,-2.14377608276421));
#166326=CARTESIAN_POINT('Ctrl Pts',(6.80901677533298,0.61615356,-2.52106359609959));
#166327=CARTESIAN_POINT('Ctrl Pts',(6.65193990646636,0.681389364000001,
-2.88343238035801));
#166328=CARTESIAN_POINT('Ctrl Pts',(7.03071436425428,0.550751630586317,
-2.33033886258751));
#166329=CARTESIAN_POINT('Ctrl Pts',(7.02944803762714,0.551389228293159,
-2.33414560129375));
#166330=CARTESIAN_POINT('Ctrl Pts',(7.028181711,0.552026826,-2.33795234));
#166331=CARTESIAN_POINT('Ctrl Pts',(6.900820226,0.61615356,-2.720817143));
#166332=CARTESIAN_POINT('Ctrl Pts',(6.73262222,0.681389364000001,-3.08758115));
#166333=CARTESIAN_POINT('Ctrl Pts',(6.65381784291963,0.680609082082813,
-2.87909853969064));
#166334=CARTESIAN_POINT('Ctrl Pts',(6.67033817410484,0.6776527527603,-2.88644139503094));
#166335=CARTESIAN_POINT('Ctrl Pts',(6.68686360748815,0.67472989688632,-2.89378637035385));
#166336=CARTESIAN_POINT('Ctrl Pts',(6.70339990372129,0.671836782516796,
-2.9011185095998));
#166337=CARTESIAN_POINT('Ctrl Pts',(6.71888040393973,0.669128385364379,
-2.90798251237273));
#166338=CARTESIAN_POINT('Ctrl Pts',(6.73436889977625,0.666446714484579,
-2.91483908496629));
#166339=CARTESIAN_POINT('Ctrl Pts',(6.74986497879715,0.663790956137697,
-2.92168848777209));
#166340=CARTESIAN_POINT('Ctrl Pts',(6.76536122419264,0.661135169277106,
-2.9285379641169));
#166341=CARTESIAN_POINT('Ctrl Pts',(6.78086509422994,0.658505288595116,
-2.93538028861438));
#166342=CARTESIAN_POINT('Ctrl Pts',(6.79637620244565,0.655900535687991,
-2.94221570577926));
#166343=CARTESIAN_POINT('Ctrl Pts',(6.655681333,0.681369595,-2.874787991));
#166344=CARTESIAN_POINT('Ctrl Pts',(6.652255021,0.679970133000001,-2.882720556));
#166345=CARTESIAN_POINT('Ctrl Pts',(6.64880981,0.678571429,-2.890644931));
#166346=CARTESIAN_POINT('Ctrl Pts',(6.494398894,0.615882895,-3.245807475));
#166347=CARTESIAN_POINT('Ctrl Pts',(6.30303087,0.552026826,-3.582499385));
#166348=CARTESIAN_POINT('Ctrl Pts',(6.859723901,0.681369595,-2.793840961));
#166349=CARTESIAN_POINT('Ctrl Pts',(6.856394065,0.679970133000001,-2.802016714));
#166350=CARTESIAN_POINT('Ctrl Pts',(6.853044751,0.678571429,-2.810184506));
#166351=CARTESIAN_POINT('Ctrl Pts',(6.702931827,0.615882895,-3.176256762));
#166352=CARTESIAN_POINT('Ctrl Pts',(6.51467511499999,0.552026826,-3.524254171));
#166353=CARTESIAN_POINT('',(6.33858731690264,0.552026824384642,-3.57271412280189));
#166354=CARTESIAN_POINT('Ctrl Pts',(6.526254313,0.499686101,-3.275999914));
#166355=CARTESIAN_POINT('Ctrl Pts',(6.476131079,0.51775868,-3.375852472));
#166356=CARTESIAN_POINT('Ctrl Pts',(6.422976508,0.535714286,-3.474124865));
#166357=CARTESIAN_POINT('Ctrl Pts',(6.39886825300001,0.54385805,-3.518696306));
#166358=CARTESIAN_POINT('Ctrl Pts',(6.374143754,0.552026826,-3.562928878));
#166359=CARTESIAN_POINT('Ctrl Pts',(6.45608189200001,0.499686101,-3.298712871));
#166360=CARTESIAN_POINT('Ctrl Pts',(6.405611147,0.51775868,-3.397491781));
#166361=CARTESIAN_POINT('Ctrl Pts',(6.352142073,0.535714286,-3.494680397));
#166362=CARTESIAN_POINT('Ctrl Pts',(6.327891176,0.54385805,-3.538760292));
#166363=CARTESIAN_POINT('Ctrl Pts',(6.30303087,0.552026826,-3.582499385));
#166364=CARTESIAN_POINT('Ctrl Pts',(6.30303087087216,0.552026826,-3.58249938475998));
#166365=CARTESIAN_POINT('Ctrl Pts',(6.32942119521346,0.543355306040699,
-3.53606838697893));
#166366=CARTESIAN_POINT('Ctrl Pts',(6.35527595402902,0.534726110167779,
-3.48938637654263));
#166367=CARTESIAN_POINT('Ctrl Pts',(6.40600783888725,0.517399146342283,
-3.39535297685708));
#166368=CARTESIAN_POINT('Ctrl Pts',(6.43086999537852,0.508708910289016,
-3.3480245948714));
#166369=CARTESIAN_POINT('Ctrl Pts',(6.45520502561422,0.499999999749251,
-3.30042846896563));
#166370=CARTESIAN_POINT('Ctrl Pts',(6.45608189200001,0.499686101,-3.298712871));
#166371=CARTESIAN_POINT('Ctrl Pts',(6.405611147,0.51775868,-3.397491781));
#166372=CARTESIAN_POINT('Ctrl Pts',(6.352142073,0.535714286,-3.494680397));
#166373=CARTESIAN_POINT('Ctrl Pts',(6.327427568,0.544013736,-3.539602974));
#166374=CARTESIAN_POINT('Ctrl Pts',(6.30208017899999,0.552339147,-3.58417151));
#166375=CARTESIAN_POINT('Ctrl Pts',(6.475636351,0.499686101,-3.35912701));
#166376=CARTESIAN_POINT('Ctrl Pts',(6.424241261,0.51775868,-3.458205105));
#166377=CARTESIAN_POINT('Ctrl Pts',(6.369839123,0.535714286,-3.555664489));
#166378=CARTESIAN_POINT('Ctrl Pts',(6.344693336,0.544013736,-3.600712219));
#166379=CARTESIAN_POINT('Ctrl Pts',(6.318912939,0.552339147,-3.645399798));
#166380=CARTESIAN_POINT('Ctrl Pts',(6.30303086689364,0.552026827262453,
-3.58249939102387));
#166381=CARTESIAN_POINT('Ctrl Pts',(6.30759124515631,0.551172308355064,
-3.58504518515021));
#166382=CARTESIAN_POINT('Ctrl Pts',(6.31215244552515,0.550320535040699,
-3.58759041886908));
#166383=CARTESIAN_POINT('Ctrl Pts',(6.31671446167628,0.549471478150372,
-3.59013509489443));
#166384=CARTESIAN_POINT('Ctrl Pts',(6.32094966483229,0.548683245863939,
-3.59249747581913));
#166385=CARTESIAN_POINT('Ctrl Pts',(6.32518557221104,0.547897354540814,
-3.59485937672857));
#166386=CARTESIAN_POINT('Ctrl Pts',(6.32942217337293,0.547113782483501,
-3.59722080120781));
#166387=CARTESIAN_POINT('Ctrl Pts',(6.33365877881568,0.546330209634431,
-3.59958222807314));
#166388=CARTESIAN_POINT('Ctrl Pts',(6.33789607911214,0.545548955858564,
-3.60194317910222));
#166389=CARTESIAN_POINT('Ctrl Pts',(6.34213406360472,0.544769999909168,
-3.60430365896608));
#166390=CARTESIAN_POINT('Ctrl Pts',(6.303963006,0.55233793,-3.580858894));
#166391=CARTESIAN_POINT('Ctrl Pts',(6.22526953600001,0.526068113,-3.719395692));
#166392=CARTESIAN_POINT('Ctrl Pts',(6.140565969,0.49968693,-3.854341653));
#166393=CARTESIAN_POINT('Ctrl Pts',(6.365182439,0.55233793,-3.563993958));
#166394=CARTESIAN_POINT('Ctrl Pts',(6.286859595,0.526068113,-3.703876123));
#166395=CARTESIAN_POINT('Ctrl Pts',(6.202467193,0.49968693,-3.840182435));
#166396=CARTESIAN_POINT('Origin',(-0.1586294734711,0.410743067797852,0.116967770955398));
#166397=CARTESIAN_POINT('Ctrl Pts',(6.3241956596213,0.552548454735263,-3.65085335360889));
#166398=CARTESIAN_POINT('Ctrl Pts',(6.32339851881064,0.552287640367631,
-3.65223281130445));
#166399=CARTESIAN_POINT('Ctrl Pts',(6.322601378,0.552026826,-3.653612269));
#166400=CARTESIAN_POINT('Ctrl Pts',(6.242784725,0.525911829,-3.79173554));
#166401=CARTESIAN_POINT('Ctrl Pts',(6.157012229,0.49968693,-3.926241358));
#166402=CARTESIAN_POINT('Ctrl Pts',(6.30459090479817,0.552548454735263,
-3.57973734278873));
#166403=CARTESIAN_POINT('Ctrl Pts',(6.3038092818689,0.552287640367631,-3.58111252991794));
#166404=CARTESIAN_POINT('Ctrl Pts',(6.30302765893962,0.552026826,-3.58248771704715));
#166405=CARTESIAN_POINT('Ctrl Pts',(6.22476479083738,0.525911829,-3.72018338189855));
#166406=CARTESIAN_POINT('Ctrl Pts',(6.14056327055529,0.49968693,-3.85432985594832));
#166407=CARTESIAN_POINT('',(6.33215348256128,0.552026824384643,-3.68832149831073));
#166408=CARTESIAN_POINT('Ctrl Pts',(6.30691137181769,0.550751630586317,
-3.57567020898544));
#166409=CARTESIAN_POINT('Ctrl Pts',(6.3049709503943,0.551389228293159,-3.5790841773981));
#166410=CARTESIAN_POINT('Ctrl Pts',(6.30303052897091,0.552026826,-3.58249814581076));
#166411=CARTESIAN_POINT('Ctrl Pts',(6.10787159547656,0.61615356,-3.92585986423298));
#166412=CARTESIAN_POINT('Ctrl Pts',(5.87656852060082,0.681389364,-4.24598978409819));
#166413=CARTESIAN_POINT('Ctrl Pts',(6.36538619882949,0.550751630586317,
-3.78725259602702));
#166414=CARTESIAN_POINT('Ctrl Pts',(6.36333114191475,0.551389228293159,
-3.79069811251351));
#166415=CARTESIAN_POINT('Ctrl Pts',(6.361276085,0.552026826,-3.794143629));
#166416=CARTESIAN_POINT('Ctrl Pts',(6.154587625,0.61615356,-4.140678312));
#166417=CARTESIAN_POINT('Ctrl Pts',(5.911478575,0.681389364000001,-4.462709981));
#166418=CARTESIAN_POINT('Ctrl Pts',(5.87933419858893,0.680609082082812,
-4.24216096607059));
#166419=CARTESIAN_POINT('Ctrl Pts',(5.89388979747093,0.677652752742843,
-4.2528835319381));
#166420=CARTESIAN_POINT('Ctrl Pts',(5.90844992258692,0.674729896907878,
-4.26360926566706));
#166421=CARTESIAN_POINT('Ctrl Pts',(5.92302341609071,0.671836782544818,
-4.27432479842803));
#166422=CARTESIAN_POINT('Ctrl Pts',(5.93666643311042,0.669128385379447,
-4.28435617462449));
#166423=CARTESIAN_POINT('Ctrl Pts',(5.95031885609289,0.666446714488034,
-4.29438201316498));
#166424=CARTESIAN_POINT('Ctrl Pts',(5.96398022626894,0.663790956130785,
-4.30440247969411));
#166425=CARTESIAN_POINT('Ctrl Pts',(5.97764174312116,0.661135169259816,
-4.31442305380862));
#166426=CARTESIAN_POINT('Ctrl Pts',(5.99131224379848,0.658505288568692,
-4.3244382823449));
#166427=CARTESIAN_POINT('Ctrl Pts',(6.00499129856053,0.655900535637417,
-4.33444832106312));
#166428=CARTESIAN_POINT('Ctrl Pts',(5.882080762,0.681369595,-4.238351791));
#166429=CARTESIAN_POINT('Ctrl Pts',(5.87702928800001,0.679970133000001,
-4.245362341));
#166430=CARTESIAN_POINT('Ctrl Pts',(5.871961118,0.678571429,-4.25236083));
#166431=CARTESIAN_POINT('Ctrl Pts',(5.64481079600001,0.615882895,-4.566026089));
#166432=CARTESIAN_POINT('Ctrl Pts',(5.38553804100001,0.552026826,-4.853707861));
#166433=CARTESIAN_POINT('Ctrl Pts',(6.098754147,0.681369595,-4.203160378));
#166434=CARTESIAN_POINT('Ctrl Pts',(6.093744616,0.679970133000001,-4.21042917));
#166435=CARTESIAN_POINT('Ctrl Pts',(6.088717772,0.678571429,-4.217686));
#166436=CARTESIAN_POINT('Ctrl Pts',(5.863419691,0.615882895,-4.542929849));
#166437=CARTESIAN_POINT('Ctrl Pts',(5.60475516,0.552026826,-4.842321644));
#166438=CARTESIAN_POINT('',(5.42236674015786,0.552026824384643,-4.85179495805918));
#166439=CARTESIAN_POINT('Ctrl Pts',(5.66943097000001,0.499686101,-4.60236062));
#166440=CARTESIAN_POINT('Ctrl Pts',(5.599014242,0.51775868,-4.68910366600001));
#166441=CARTESIAN_POINT('Ctrl Pts',(5.525976735,0.535714286,-4.773651843));
#166442=CARTESIAN_POINT('Ctrl Pts',(5.492850576,0.54385805,-4.811998667));
#166443=CARTESIAN_POINT('Ctrl Pts',(5.459195426,0.552026826,-4.84988207));
#166444=CARTESIAN_POINT('Ctrl Pts',(5.596016527,0.499686101,-4.609457563));
#166445=CARTESIAN_POINT('Ctrl Pts',(5.52549121500001,0.51775868,-4.695077359));
#166446=CARTESIAN_POINT('Ctrl Pts',(5.452379538,0.535714286,-4.77849949));
#166447=CARTESIAN_POINT('Ctrl Pts',(5.419219739,0.54385805,-4.81633559500001));
#166448=CARTESIAN_POINT('Ctrl Pts',(5.385538041,0.552026826,-4.853707861));
#166449=CARTESIAN_POINT('Ctrl Pts',(5.38553804122079,0.552026826358493,
-4.85370786189697));
#166450=CARTESIAN_POINT('Ctrl Pts',(5.40800898309041,0.546576979810991,
-4.82877473554052));
#166451=CARTESIAN_POINT('Ctrl Pts',(5.4302902785008,0.541139220283038,-4.80370385122636));
#166452=CARTESIAN_POINT('Ctrl Pts',(5.45237953827665,0.535714285934403,
-4.77849948984032));
#166453=CARTESIAN_POINT('Ctrl Pts',(5.50061482983329,0.523868108611029,
-4.72346189596191));
#166454=CARTESIAN_POINT('Ctrl Pts',(5.54809893182974,0.511960760799632,
-4.66759983813293));
#166455=CARTESIAN_POINT('Ctrl Pts',(5.5947913592018,0.499999999550736,-4.61094454995047));
#166456=CARTESIAN_POINT('Ctrl Pts',(5.596016527,0.499686101,-4.609457563));
#166457=CARTESIAN_POINT('Ctrl Pts',(5.52549121500001,0.51775868,-4.695077359));
#166458=CARTESIAN_POINT('Ctrl Pts',(5.452379538,0.535714286,-4.77849949));
#166459=CARTESIAN_POINT('Ctrl Pts',(5.418585819,0.544013736,-4.817058913));
#166460=CARTESIAN_POINT('Ctrl Pts',(5.38425012,0.552339147,-4.855136522));
#166461=CARTESIAN_POINT('Ctrl Pts',(5.602126559,0.499686101,-4.672662884));
#166462=CARTESIAN_POINT('Ctrl Pts',(5.530634197,0.51775868,-4.758376164));
#166463=CARTESIAN_POINT('Ctrl Pts',(5.456553063,0.535714286,-4.84186215));
#166464=CARTESIAN_POINT('Ctrl Pts',(5.422311241,0.544013736,-4.880451088));
#166465=CARTESIAN_POINT('Ctrl Pts',(5.387527066,0.552339147,-4.918551872));
#166466=CARTESIAN_POINT('Ctrl Pts',(5.38553803705753,0.552026827368203,
-4.85370786651641));
#166467=CARTESIAN_POINT('Ctrl Pts',(5.38944452605589,0.551172308341726,
-4.85717448718889));
#166468=CARTESIAN_POINT('Ctrl Pts',(5.39335193808722,0.550320534996839,
-4.86064073811492));
#166469=CARTESIAN_POINT('Ctrl Pts',(5.39726026672052,0.549471478077806,
-4.86410661975057));
#166470=CARTESIAN_POINT('Ctrl Pts',(5.40088861101123,0.548683245788842,
-4.86732421300458));
#166471=CARTESIAN_POINT('Ctrl Pts',(5.40451774625319,0.547897354464642,
-4.87054148884905));
#166472=CARTESIAN_POINT('Ctrl Pts',(5.40814766147832,0.547113782407049,
-4.87375844854294));
#166473=CARTESIAN_POINT('Ctrl Pts',(5.41177758037128,0.546330209557698,
-4.8769754114874));
#166474=CARTESIAN_POINT('Ctrl Pts',(5.41540828016522,0.545548955782291,
-4.88019205909147));
#166475=CARTESIAN_POINT('Ctrl Pts',(5.41903974970139,0.54476999977346,-4.88340839344506));
#166476=CARTESIAN_POINT('Ctrl Pts',(5.386801042,0.55233793,-4.852306105));
#166477=CARTESIAN_POINT('Ctrl Pts',(5.280166064,0.526068113,-4.97068722));
#166478=CARTESIAN_POINT('Ctrl Pts',(5.168433427,0.49968693,-5.084269457));
#166479=CARTESIAN_POINT('Ctrl Pts',(5.450214661,0.55233793,-4.84899583));
#166480=CARTESIAN_POINT('Ctrl Pts',(5.343652431,0.526068113,-4.968770532));
#166481=CARTESIAN_POINT('Ctrl Pts',(5.231931248,0.49968693,-5.083748206));
#166482=CARTESIAN_POINT('Origin',(-0.129777259309849,0.410742903792786,
0.148334819574623));
#166483=CARTESIAN_POINT('Ctrl Pts',(5.39151392645153,0.552548454735263,
-4.92501355593251));
#166484=CARTESIAN_POINT('Ctrl Pts',(5.39043887972577,0.552287640367631,
-4.92618940096626));
#166485=CARTESIAN_POINT('Ctrl Pts',(5.389363833,0.552026826,-4.927365246));
#166486=CARTESIAN_POINT('Ctrl Pts',(5.281720829,0.525911829,-5.045101051));
#166487=CARTESIAN_POINT('Ctrl Pts',(5.16903887200001,0.49968693,-5.158023646));
#166488=CARTESIAN_POINT('Ctrl Pts',(5.38765536049434,0.552548454735263,
-4.85134575520336));
#166489=CARTESIAN_POINT('Ctrl Pts',(5.3865963868867,0.552287640367631,-4.8525207653942));
#166490=CARTESIAN_POINT('Ctrl Pts',(5.38553741327904,0.552026826,-4.85369577558505));
#166491=CARTESIAN_POINT('Ctrl Pts',(5.2795037892965,0.525911828999999,-4.97134798887189));
#166492=CARTESIAN_POINT('Ctrl Pts',(5.16843332766096,0.49968693,-5.08425735570182));
#166493=CARTESIAN_POINT('',(5.39123115681089,0.552026824384643,-4.96331641310191));
#166494=CARTESIAN_POINT('Ctrl Pts',(5.39079595785797,0.550751630586318,
-4.84787382396709));
#166495=CARTESIAN_POINT('Ctrl Pts',(5.38816699942899,0.551389228293159,
-4.85079084248355));
#166496=CARTESIAN_POINT('Ctrl Pts',(5.38553804100001,0.552026826,-4.853707861));
#166497=CARTESIAN_POINT('Ctrl Pts',(5.121129126,0.61615356,-5.147088575));
#166498=CARTESIAN_POINT('Ctrl Pts',(4.826415248,0.681389364,-5.41001070799999));
#166499=CARTESIAN_POINT('Ctrl Pts',(5.40241964904355,0.550751630586318,
-5.06707860853673));
#166500=CARTESIAN_POINT('Ctrl Pts',(5.39967195402178,0.551389228293159,
-5.07000179426836));
#166501=CARTESIAN_POINT('Ctrl Pts',(5.396924259,0.552026826,-5.07292498));
#166502=CARTESIAN_POINT('Ctrl Pts',(5.120573347,0.61615356,-5.366925965));
#166503=CARTESIAN_POINT('Ctrl Pts',(4.813920762,0.681389364,-5.62916745300001));
#166504=CARTESIAN_POINT('Ctrl Pts',(4.82993942163327,0.680609082082812,
-5.4068646610752));
#166505=CARTESIAN_POINT('Ctrl Pts',(4.84184968410275,0.677652752784265,
-5.42046556271524));
#166506=CARTESIAN_POINT('Ctrl Pts',(4.85376368616349,0.674729896895564,
-5.43407053107029));
#166507=CARTESIAN_POINT('Ctrl Pts',(4.86569293671695,0.671836782532443,
-5.44766841099454));
#166508=CARTESIAN_POINT('Ctrl Pts',(4.87686053821691,0.669128385374017,
-5.46039810457904));
#166509=CARTESIAN_POINT('Ctrl Pts',(4.88803851620062,0.66644671448801,-5.47312441198304));
#166510=CARTESIAN_POINT('Ctrl Pts',(4.89922638701745,0.663790956134898,
-5.48584739635545));
#166511=CARTESIAN_POINT('Ctrl Pts',(4.91041437795354,0.661135169268071,
-5.49857051732898));
#166512=CARTESIAN_POINT('Ctrl Pts',(4.92161229181551,0.65850528857982,-5.51129034896074));
#166513=CARTESIAN_POINT('Ctrl Pts',(4.93281967474729,0.655900535551958,
-5.52400695138184));
#166514=CARTESIAN_POINT('Ctrl Pts',(4.833440632,0.681369595,-5.403734972));
#166515=CARTESIAN_POINT('Ctrl Pts',(4.827000198,0.679970133000001,-5.409495702));
#166516=CARTESIAN_POINT('Ctrl Pts',(4.82054605,0.678571429,-5.415241063));
#166517=CARTESIAN_POINT('Ctrl Pts',(4.531277618,0.615882895,-5.672742398));
#166518=CARTESIAN_POINT('Ctrl Pts',(4.216223439,0.552026826,-5.897962352));
#166519=CARTESIAN_POINT('Ctrl Pts',(5.052613427,0.681369595,-5.415944688));
#166520=CARTESIAN_POINT('Ctrl Pts',(5.046158441,0.679970133000001,-5.421966639));
#166521=CARTESIAN_POINT('Ctrl Pts',(5.039689118,0.678571429,-5.427973185));
#166522=CARTESIAN_POINT('Ctrl Pts',(4.749740568,0.615882895,-5.697180586));
#166523=CARTESIAN_POINT('Ctrl Pts',(4.432763084,0.552026826,-5.933967539));
#166524=CARTESIAN_POINT('',(4.25260232110177,0.552026824384641,-5.90401125316438));
#166525=CARTESIAN_POINT('Ctrl Pts',(4.547511336,0.499686101,-5.713520057));
#166526=CARTESIAN_POINT('Ctrl Pts',(4.460093721,0.51775868,-5.783097584));
#166527=CARTESIAN_POINT('Ctrl Pts',(4.370588431,0.535714286,-5.849968167));
#166528=CARTESIAN_POINT('Ctrl Pts',(4.32999331,0.54385805,-5.880297318));
#166529=CARTESIAN_POINT('Ctrl Pts',(4.288981187,0.552026826,-5.910060166));
#166530=CARTESIAN_POINT('Ctrl Pts',(4.474287649,0.499686101,-5.704669143));
#166531=CARTESIAN_POINT('Ctrl Pts',(4.387005454,0.51775868,-5.773126338));
#166532=CARTESIAN_POINT('Ctrl Pts',(4.297669796,0.535714286,-5.838881257));
#166533=CARTESIAN_POINT('Ctrl Pts',(4.25715161,0.54385805,-5.868704398));
#166534=CARTESIAN_POINT('Ctrl Pts',(4.216223439,0.552026826,-5.897962352));
#166535=CARTESIAN_POINT('Ctrl Pts',(4.21622343978821,0.552026826,-5.89796235213106));
#166536=CARTESIAN_POINT('Ctrl Pts',(4.25967050727171,0.543355308490836,
-5.86690373837236));
#166537=CARTESIAN_POINT('Ctrl Pts',(4.30273690686368,0.534726114959304,
-5.83539243414648));
#166538=CARTESIAN_POINT('Ctrl Pts',(4.38826616643414,0.517398614624112,
-5.77134981348705));
#166539=CARTESIAN_POINT('Ctrl Pts',(4.43069788664702,0.50870945045658,-5.73883909642985));
#166540=CARTESIAN_POINT('Ctrl Pts',(4.47277146633137,0.499999999626732,
-5.70585799044219));
#166541=CARTESIAN_POINT('Ctrl Pts',(4.474287649,0.499686101,-5.704669143));
#166542=CARTESIAN_POINT('Ctrl Pts',(4.387005454,0.51775868,-5.773126338));
#166543=CARTESIAN_POINT('Ctrl Pts',(4.297669796,0.535714286,-5.838881257));
#166544=CARTESIAN_POINT('Ctrl Pts',(4.256377018,0.544013736,-5.869274531));
#166545=CARTESIAN_POINT('Ctrl Pts',(4.214658508,0.552339147,-5.899080747));
#166546=CARTESIAN_POINT('Ctrl Pts',(4.466667556,0.499686101,-5.767710235));
#166547=CARTESIAN_POINT('Ctrl Pts',(4.378420824,0.51775868,-5.836050841));
#166548=CARTESIAN_POINT('Ctrl Pts',(4.288124647,0.535714286,-5.901659717));
#166549=CARTESIAN_POINT('Ctrl Pts',(4.246387899,0.544013736,-5.931985488));
#166550=CARTESIAN_POINT('Ctrl Pts',(4.204226416,0.552339147,-5.961717928));
#166551=CARTESIAN_POINT('Ctrl Pts',(4.21622343369513,0.552026827225121,
-5.8979623562474));
#166552=CARTESIAN_POINT('Ctrl Pts',(4.21929336986428,0.551172308280893,
-5.90218770933082));
#166553=CARTESIAN_POINT('Ctrl Pts',(4.2223642873589,0.550320534952158,-5.90641289924824));
#166554=CARTESIAN_POINT('Ctrl Pts',(4.22543617940756,0.549471478050236,
-5.91063792555498));
#166555=CARTESIAN_POINT('Ctrl Pts',(4.22828800767696,0.548683245769649,
-5.91456028000939));
#166556=CARTESIAN_POINT('Ctrl Pts',(4.23114067663525,0.547897354454663,
-5.91848249450931));
#166557=CARTESIAN_POINT('Ctrl Pts',(4.23399417529381,0.547113782405765,
-5.92240456793084));
#166558=CARTESIAN_POINT('Ctrl Pts',(4.23684767683566,0.546330209565113,
-5.92632664531538));
#166559=CARTESIAN_POINT('Ctrl Pts',(4.23970200880008,0.545548955798003,
-5.93024858261012));
#166560=CARTESIAN_POINT('Ctrl Pts',(4.24255715914079,0.544769999937507,
-5.93417037982135));
#166561=CARTESIAN_POINT('Ctrl Pts',(4.217758247,0.55233793,-5.89686487600001));
#166562=CARTESIAN_POINT('Ctrl Pts',(4.088167896,0.526068113,-5.989554938));
#166563=CARTESIAN_POINT('Ctrl Pts',(3.954630682,0.49968693,-6.076462471));
#166564=CARTESIAN_POINT('Ctrl Pts',(4.280400903,0.55233793,-5.907264047));
#166565=CARTESIAN_POINT('Ctrl Pts',(4.150582018,0.526068113,-6.001330754));
#166566=CARTESIAN_POINT('Ctrl Pts',(4.016756013,0.49968693,-6.089603562));
#166567=CARTESIAN_POINT('Origin',(-0.0948546780510573,0.410743245677191,
0.172763753115606));
#166568=CARTESIAN_POINT('Ctrl Pts',(4.20673099430623,0.552548454735263,
-5.9688855986822));
#166569=CARTESIAN_POINT('Ctrl Pts',(4.20542830965312,0.552287640367631,
-5.9698028498411));
#166570=CARTESIAN_POINT('Ctrl Pts',(4.204125625,0.552026826,-5.970720101));
#166571=CARTESIAN_POINT('Ctrl Pts',(4.073689537,0.525911829,-6.062563244));
#166572=CARTESIAN_POINT('Ctrl Pts',(3.939367001,0.49968693,-6.148622482));
#166573=CARTESIAN_POINT('Ctrl Pts',(4.21879903966101,0.552548454735263,
-5.89611063196322));
#166574=CARTESIAN_POINT('Ctrl Pts',(4.21751223181639,0.552287640367631,
-5.89703052304883));
#166575=CARTESIAN_POINT('Ctrl Pts',(4.21622542397176,0.552026826,-5.89795041413444));
#166576=CARTESIAN_POINT('Ctrl Pts',(4.08737905976591,0.525911829,-5.99005788949816));
#166577=CARTESIAN_POINT('Ctrl Pts',(3.95463318641739,0.49968693,-6.07645063120944));
#166578=CARTESIAN_POINT('',(4.198220854242,0.552026824384649,-6.00623216873903));
#166579=CARTESIAN_POINT('Ctrl Pts',(4.22261278365116,0.550751630586318,
-5.89339374004824));
#166580=CARTESIAN_POINT('Ctrl Pts',(4.21941821673891,0.551389228293159,
-5.89567741205534));
#166581=CARTESIAN_POINT('Ctrl Pts',(4.21622364982665,0.552026826,-5.89796108406243));
#166582=CARTESIAN_POINT('Ctrl Pts',(3.89492835589839,0.61615356,-6.12764263054736));
#166583=CARTESIAN_POINT('Ctrl Pts',(3.55058430531378,0.681389364000001,
-6.3210630364675));
#166584=CARTESIAN_POINT('Ctrl Pts',(4.18684196093688,0.550751630586318,
-6.10997365687232));
#166585=CARTESIAN_POINT('Ctrl Pts',(4.18353010696844,0.551389228293159,
-6.11223782693617));
#166586=CARTESIAN_POINT('Ctrl Pts',(4.180218253,0.552026826,-6.114501997));
#166587=CARTESIAN_POINT('Ctrl Pts',(3.84712675,0.61615356,-6.342222125));
#166588=CARTESIAN_POINT('Ctrl Pts',(3.491269364,0.681389364000001,-6.532411311));
#166589=CARTESIAN_POINT('Ctrl Pts',(3.55470204599018,0.680609082082816,
-6.31874937382084));
#166590=CARTESIAN_POINT('Ctrl Pts',(3.5634100609705,0.677652752713562,-6.33459264818729));
#166591=CARTESIAN_POINT('Ctrl Pts',(3.5721208539121,0.674729896887179,-6.35044069837409));
#166592=CARTESIAN_POINT('Ctrl Pts',(3.5808480629607,0.671836782527383,-6.36628510364611));
#166593=CARTESIAN_POINT('Ctrl Pts',(3.58901806429499,0.669128385369925,
-6.38111788827318));
#166594=CARTESIAN_POINT('Ctrl Pts',(3.59719892743867,0.666446714485906,
-6.3959495965279));
#166595=CARTESIAN_POINT('Ctrl Pts',(3.60539016647564,0.663790956135505,
-6.41078018611097));
#166596=CARTESIAN_POINT('Ctrl Pts',(3.61358149345834,0.661135169271393,
-6.42561093492357));
#166597=CARTESIAN_POINT('Ctrl Pts',(3.62178321848122,0.658505288586583,
-6.44044060443574));
#166598=CARTESIAN_POINT('Ctrl Pts',(3.62999488593847,0.655900535633648,
-6.45526915564017));
#166599=CARTESIAN_POINT('Ctrl Pts',(3.558794191,0.681369595,-6.316445512));
#166600=CARTESIAN_POINT('Ctrl Pts',(3.551265944,0.679970133000001,-6.320687056));
#166601=CARTESIAN_POINT('Ctrl Pts',(3.543727607,0.678571429,-6.324910643));
#166602=CARTESIAN_POINT('Ctrl Pts',(3.205866935,0.615882895,-6.514207577));
#166603=CARTESIAN_POINT('Ctrl Pts',(2.849762915,0.552026826,-6.666434679));
#166604=CARTESIAN_POINT('Ctrl Pts',(3.770218119,0.681369595,-6.375485444));
#166605=CARTESIAN_POINT('Ctrl Pts',(3.762619505,0.679970133000001,-6.379978973));
#166606=CARTESIAN_POINT('Ctrl Pts',(3.755010202,0.678571429,-6.384454377));
#166607=CARTESIAN_POINT('Ctrl Pts',(3.413968854,0.615882895,-6.585037491));
#166608=CARTESIAN_POINT('Ctrl Pts',(3.053499932,0.552026826,-6.74814770699999));
#166609=CARTESIAN_POINT('',(2.88399094416683,0.552026824384642,-6.68016254454245));
#166610=CARTESIAN_POINT('Ctrl Pts',(3.212955126,0.499686101,-6.557521647));
#166611=CARTESIAN_POINT('Ctrl Pts',(3.112624175,0.51775868,-6.606680287));
#166612=CARTESIAN_POINT('Ctrl Pts',(3.01083627,0.535714286,-6.652746481));
#166613=CARTESIAN_POINT('Ctrl Pts',(2.964670369,0.54385805,-6.673639803));
#166614=CARTESIAN_POINT('Ctrl Pts',(2.918218955,0.552026826,-6.693890418));
#166615=CARTESIAN_POINT('Ctrl Pts',(3.143346053,0.499686101,-6.533136734));
#166616=CARTESIAN_POINT('Ctrl Pts',(3.043388194,0.51775868,-6.581230346));
#166617=CARTESIAN_POINT('Ctrl Pts',(2.94200579,0.535714286,-6.626243425));
#166618=CARTESIAN_POINT('Ctrl Pts',(2.896023804,0.54385805,-6.646659106));
#166619=CARTESIAN_POINT('Ctrl Pts',(2.849762915,0.552026826,-6.666434679));
#166620=CARTESIAN_POINT('Ctrl Pts',(2.84976291891813,0.552026825495856,
-6.6664346782059));
#166621=CARTESIAN_POINT('Ctrl Pts',(2.89887089484146,0.543355309227961,
-6.64544203478179));
#166622=CARTESIAN_POINT('Ctrl Pts',(2.94770444479558,0.534726112122594,
-6.62392544096408));
#166623=CARTESIAN_POINT('Ctrl Pts',(3.04500134496897,0.517398612370645,
-6.57976636581241));
#166624=CARTESIAN_POINT('Ctrl Pts',(3.09342989164506,0.508709445676462,
-6.55713728981927));
#166625=CARTESIAN_POINT('Ctrl Pts',(3.14160975114555,0.499999999561346,
-6.53397185222096));
#166626=CARTESIAN_POINT('Ctrl Pts',(3.143346053,0.499686101,-6.533136734));
#166627=CARTESIAN_POINT('Ctrl Pts',(3.043388194,0.51775868,-6.581230346));
#166628=CARTESIAN_POINT('Ctrl Pts',(2.94200579,0.535714286,-6.626243425));
#166629=CARTESIAN_POINT('Ctrl Pts',(2.895144759,0.544013736,-6.647049396));
#166630=CARTESIAN_POINT('Ctrl Pts',(2.84799415,0.552339147,-6.667190512));
#166631=CARTESIAN_POINT('Ctrl Pts',(3.122352143,0.499686101,-6.593065866));
#166632=CARTESIAN_POINT('Ctrl Pts',(3.02147736,0.51775868,-6.640838268));
#166633=CARTESIAN_POINT('Ctrl Pts',(2.919188289,0.535714286,-6.685502236));
#166634=CARTESIAN_POINT('Ctrl Pts',(2.871908178,0.544013736,-6.70614684));
#166635=CARTESIAN_POINT('Ctrl Pts',(2.824340811,0.552339147,-6.72612067900001));
#166636=CARTESIAN_POINT('Ctrl Pts',(2.84976290889703,0.55202682733598,-6.66643468166387));
#166637=CARTESIAN_POINT('Ctrl Pts',(2.85185274604644,0.551172308275351,
-6.67122119378965));
#166638=CARTESIAN_POINT('Ctrl Pts',(2.85394357611775,0.550320534936221,
-6.67600775770568));
#166639=CARTESIAN_POINT('Ctrl Pts',(2.85603539316663,0.549471478025613,
-6.68079437132065));
#166640=CARTESIAN_POINT('Ctrl Pts',(2.85797735687409,0.54868324575317,-6.68523808207772));
#166641=CARTESIAN_POINT('Ctrl Pts',(2.85992017173335,0.547897354447752,
-6.68968183686207));
#166642=CARTESIAN_POINT('Ctrl Pts',(2.86186382725496,0.547113782410433,
-6.6941256322136));
#166643=CARTESIAN_POINT('Ctrl Pts',(2.86380748474054,0.546330209581352,
-6.69856943205538));
#166644=CARTESIAN_POINT('Ctrl Pts',(2.86575198338132,0.545548955827773,
-6.70301327358507));
#166645=CARTESIAN_POINT('Ctrl Pts',(2.86769731172646,0.544769999923278,
-6.70745715414584));
#166646=CARTESIAN_POINT('Ctrl Pts',(2.851497765,0.55233793,-6.665692799));
#166647=CARTESIAN_POINT('Ctrl Pts',(2.705011541,0.526068113,-6.728357725));
#166648=CARTESIAN_POINT('Ctrl Pts',(2.555913802,0.49968693,-6.784526854));
#166649=CARTESIAN_POINT('Ctrl Pts',(2.910440355,0.55233793,-6.689315163));
#166650=CARTESIAN_POINT('Ctrl Pts',(2.763435003,0.526068113,-6.753275419));
#166651=CARTESIAN_POINT('Ctrl Pts',(2.613761731,0.49968693,-6.810715823));
#166652=CARTESIAN_POINT('Origin',(-0.0554976071978636,0.410743109954222,
0.189114824533242));
#166653=CARTESIAN_POINT('Ctrl Pts',(2.82524599699793,0.552548454735263,
-6.73365918371557));
#166654=CARTESIAN_POINT('Ctrl Pts',(2.82377658649897,0.552287640367631,
-6.73427495135779));
#166655=CARTESIAN_POINT('Ctrl Pts',(2.822307176,0.552026826,-6.734890719));
#166656=CARTESIAN_POINT('Ctrl Pts',(2.67517705,0.525911829,-6.796546717));
#166657=CARTESIAN_POINT('Ctrl Pts',(2.525494709,0.49968693,-6.851718563));
#166658=CARTESIAN_POINT('Ctrl Pts',(2.85267636463054,0.552548454735263,
-6.66517992915994));
#166659=CARTESIAN_POINT('Ctrl Pts',(2.85122189224375,0.552287640367631,
-6.66580168804706));
#166660=CARTESIAN_POINT('Ctrl Pts',(2.84976741985695,0.552026826,-6.66642344693418));
#166661=CARTESIAN_POINT('Ctrl Pts',(2.70413302723223,0.525911829,-6.72867934034711));
#166662=CARTESIAN_POINT('Ctrl Pts',(2.55591879307536,0.49968693,-6.7845158293819));
#166663=CARTESIAN_POINT('',(2.80890641028778,0.552026824384643,-6.76830318364549));
#166664=CARTESIAN_POINT('Ctrl Pts',(2.85698451967886,0.550751630586318,
-6.66334759239431));
#166665=CARTESIAN_POINT('Ctrl Pts',(2.85337371733943,0.551389228293159,
-6.66489113569716));
#166666=CARTESIAN_POINT('Ctrl Pts',(2.849762915,0.552026826,-6.666434679));
#166667=CARTESIAN_POINT('Ctrl Pts',(2.486604518,0.61615356,-6.821677381));
#166668=CARTESIAN_POINT('Ctrl Pts',(2.108731308,0.681389364000001,-6.93655190100001));
#166669=CARTESIAN_POINT('Ctrl Pts',(2.77549219559838,0.550751630586318,
-6.86717312735757));
#166670=CARTESIAN_POINT('Ctrl Pts',(2.77177104129919,0.551389228293159,
-6.86867241167878));
#166671=CARTESIAN_POINT('Ctrl Pts',(2.768049887,0.552026826,-6.87017169600001));
#166672=CARTESIAN_POINT('Ctrl Pts',(2.393792782,0.61615356,-7.020963027));
#166673=CARTESIAN_POINT('Ctrl Pts',(2.005370091,0.681389364000001,-7.130206877));
#166674=CARTESIAN_POINT('Ctrl Pts',(2.11325075290579,0.680609082082812,
-6.93517638941795));
#166675=CARTESIAN_POINT('Ctrl Pts',(2.11834934301391,0.6776527527642,-6.95252122234189));
#166676=CARTESIAN_POINT('Ctrl Pts',(2.12344962078689,0.674729896829384,
-6.96987131670069));
#166677=CARTESIAN_POINT('Ctrl Pts',(2.12856671375807,0.671836782472668,
-6.98722138055105));
#166678=CARTESIAN_POINT('Ctrl Pts',(2.13335709474363,0.669128385325786,
-7.00346369165135));
#166679=CARTESIAN_POINT('Ctrl Pts',(2.13815831498433,0.666446714451452,
-7.01970728651192));
#166680=CARTESIAN_POINT('Ctrl Pts',(2.14296990901684,0.663790956109898,
-7.03595201936503));
#166681=CARTESIAN_POINT('Ctrl Pts',(2.14778155470932,0.661135169254634,
-7.05219692663069));
#166682=CARTESIAN_POINT('Ctrl Pts',(2.15260358735908,0.658505288577833,
-7.06844301510056));
#166683=CARTESIAN_POINT('Ctrl Pts',(2.15743557081923,0.655900535694669,
-7.08469014864916));
#166684=CARTESIAN_POINT('Ctrl Pts',(2.117742488,0.681369595,-6.93380608));
#166685=CARTESIAN_POINT('Ctrl Pts',(2.10947844,0.679970133000001,-6.936330109));
#166686=CARTESIAN_POINT('Ctrl Pts',(2.1012084,0.678571429,-6.938834431));
#166687=CARTESIAN_POINT('Ctrl Pts',(1.730553477,0.615882895,-7.05107565));
#166688=CARTESIAN_POINT('Ctrl Pts',(1.350050644,0.552026826,-7.123191929));
#166689=CARTESIAN_POINT('Ctrl Pts',(2.311531602,0.681369595,-7.036915586));
#166690=CARTESIAN_POINT('Ctrl Pts',(2.303144664,0.679970133000001,-7.039670582));
#166691=CARTESIAN_POINT('Ctrl Pts',(2.294751182,0.678571429,-7.042405578));
#166692=CARTESIAN_POINT('Ctrl Pts',(1.918563751,0.615882895,-7.164985361));
#166693=CARTESIAN_POINT('Ctrl Pts',(1.531458517,0.552026826,-7.24679198800001));
#166694=CARTESIAN_POINT('',(1.38052735580328,0.552026824384641,-7.14395685910557));
#166695=CARTESIAN_POINT('Ctrl Pts',(1.728164706,0.499686101,-7.094900813));
#166696=CARTESIAN_POINT('Ctrl Pts',(1.619611782,0.51775868,-7.121341962));
#166697=CARTESIAN_POINT('Ctrl Pts',(1.510300752,0.535714286,-7.144449764));
#166698=CARTESIAN_POINT('Ctrl Pts',(1.460722737,0.54385805,-7.154930307));
#166699=CARTESIAN_POINT('Ctrl Pts',(1.411004048,0.552026826,-7.164721793));
#166700=CARTESIAN_POINT('Ctrl Pts',(1.665425089,0.499686101,-7.056122113));
#166701=CARTESIAN_POINT('Ctrl Pts',(1.557465485,0.51775868,-7.081603338));
#166702=CARTESIAN_POINT('Ctrl Pts',(1.448776863,0.535714286,-7.103769816));
#166703=CARTESIAN_POINT('Ctrl Pts',(1.399481142,0.54385805,-7.11382342199999));
#166704=CARTESIAN_POINT('Ctrl Pts',(1.350050644,0.552026826,-7.12319192899999));
#166705=CARTESIAN_POINT('Ctrl Pts',(1.35005064358211,0.55202682632986,-7.12319192927199));
#166706=CARTESIAN_POINT('Ctrl Pts',(1.38302848960185,0.546576979806139,
-7.11694167477289));
#166707=CARTESIAN_POINT('Ctrl Pts',(1.41593872707709,0.541139220287456,
-7.11046698299128));
#166708=CARTESIAN_POINT('Ctrl Pts',(1.44877686332883,0.53571428591939,-7.10376981614113));
#166709=CARTESIAN_POINT('Ctrl Pts',(1.52048397699588,0.523868108620023,
-7.08914552447919));
#166710=CARTESIAN_POINT('Ctrl Pts',(1.59209201781199,0.511960760913898,
-7.07341028179112));
#166711=CARTESIAN_POINT('Ctrl Pts',(1.66354985423408,0.499999999722903,
-7.05656445327241));
#166712=CARTESIAN_POINT('Ctrl Pts',(1.665425089,0.499686101,-7.056122113));
#166713=CARTESIAN_POINT('Ctrl Pts',(1.557465485,0.51775868,-7.081603338));
#166714=CARTESIAN_POINT('Ctrl Pts',(1.448776863,0.535714286,-7.103769816));
#166715=CARTESIAN_POINT('Ctrl Pts',(1.398538749,0.544013736,-7.114015618));
#166716=CARTESIAN_POINT('Ctrl Pts',(1.34816075,0.552339147,-7.12354985899999));
#166717=CARTESIAN_POINT('Ctrl Pts',(1.632039014,0.499686101,-7.110137064));
#166718=CARTESIAN_POINT('Ctrl Pts',(1.523252973,0.51775868,-7.13510747800001));
#166719=CARTESIAN_POINT('Ctrl Pts',(1.41375393,0.535714286,-7.1567381));
#166720=CARTESIAN_POINT('Ctrl Pts',(1.363141222,0.544013736,-7.166736219));
#166721=CARTESIAN_POINT('Ctrl Pts',(1.312392169,0.552339147,-7.176017503));
#166722=CARTESIAN_POINT('Ctrl Pts',(1.35005063742863,0.552026827346769,
-7.12319193043825));
#166723=CARTESIAN_POINT('Ctrl Pts',(1.35106265669364,0.551172308311127,
-7.12831578970783));
#166724=CARTESIAN_POINT('Ctrl Pts',(1.35207563461735,0.550320534970049,
-7.13343991304482));
#166725=CARTESIAN_POINT('Ctrl Pts',(1.35308956573833,0.549471478056719,
-7.13856429709401));
#166726=CARTESIAN_POINT('Ctrl Pts',(1.354030860992,0.548683245773404,-7.14332158117741));
#166727=CARTESIAN_POINT('Ctrl Pts',(1.35497297801486,0.547897354456482,
-7.1480790912348));
#166728=CARTESIAN_POINT('Ctrl Pts',(1.35591590731123,0.547113782407415,
-7.1528368216312));
#166729=CARTESIAN_POINT('Ctrl Pts',(1.35685883756039,0.546330209566589,
-7.15759455683505));
#166730=CARTESIAN_POINT('Ctrl Pts',(1.35780258032342,0.545548955800985,
-7.16235251357834));
#166731=CARTESIAN_POINT('Ctrl Pts',(1.35874712535521,0.544769999826398,
-7.16711068672649));
#166732=CARTESIAN_POINT('Ctrl Pts',(1.351904417,0.55233793,-7.122840336));
#166733=CARTESIAN_POINT('Ctrl Pts',(1.195371852,0.526068113,-7.152549982));
#166734=CARTESIAN_POINT('Ctrl Pts',(1.037685233,0.49968693,-7.175354302));
#166735=CARTESIAN_POINT('Ctrl Pts',(1.404390852,0.55233793,-7.158581336));
#166736=CARTESIAN_POINT('Ctrl Pts',(1.247072838,0.526068113,-7.189444432));
#166737=CARTESIAN_POINT('Ctrl Pts',(1.088550856,0.49968693,-7.213366582));
#166738=CARTESIAN_POINT('Origin',(-0.0135462466738689,0.410742949663908,
0.196625407235529));
#166739=CARTESIAN_POINT('Ctrl Pts',(1.31165563666942,0.552548454735263,
-7.18357434997127));
#166740=CARTESIAN_POINT('Ctrl Pts',(1.31008820833471,0.552287640367631,
-7.18385984148563));
#166741=CARTESIAN_POINT('Ctrl Pts',(1.30852078,0.552026826,-7.184145333));
#166742=CARTESIAN_POINT('Ctrl Pts',(1.151576258,0.525911829,-7.21273122));
#166743=CARTESIAN_POINT('Ctrl Pts',(0.99353309,0.49968693,-7.2344359));
#166744=CARTESIAN_POINT('Ctrl Pts',(1.35316571288421,0.552548454735263,
-7.12259282012464));
#166745=CARTESIAN_POINT('Ctrl Pts',(1.35161158546938,0.552287640367631,
-7.12288737406653));
#166746=CARTESIAN_POINT('Ctrl Pts',(1.35005745805455,0.552026826,-7.12318192800843));
#166747=CARTESIAN_POINT('Ctrl Pts',(1.19444473953571,0.525911829,-7.15267522386804));
#166748=CARTESIAN_POINT('Ctrl Pts',(1.03769247730763,0.49968693,-7.1753446081269));
#166749=CARTESIAN_POINT('',(1.28825062439923,0.552026824384644,-7.21389586373221));
#166750=CARTESIAN_POINT('Ctrl Pts',(1.35776776537411,0.550751630586317,
-7.12172838697859));
#166751=CARTESIAN_POINT('Ctrl Pts',(1.3539095659827,0.551389228293159,-7.12245962771548));
#166752=CARTESIAN_POINT('Ctrl Pts',(1.35005136659128,0.552026826,-7.12319086845238));
#166753=CARTESIAN_POINT('Ctrl Pts',(0.962010877365314,0.61615356,-7.19673580081601));
#166754=CARTESIAN_POINT('Ctrl Pts',(0.568277560521424,0.681389364000001,
-7.22769309322264));
#166755=CARTESIAN_POINT('Ctrl Pts',(1.23436350016688,0.550751630586317,
-7.30327121457896));
#166756=CARTESIAN_POINT('Ctrl Pts',(1.23040704258344,0.551389228293159,
-7.30393550828948));
#166757=CARTESIAN_POINT('Ctrl Pts',(1.226450585,0.552026826,-7.304599802));
#166758=CARTESIAN_POINT('Ctrl Pts',(0.828527725,0.61615356,-7.371411501));
#166759=CARTESIAN_POINT('Ctrl Pts',(0.425701942,0.681389364000001,-7.394601894));
#166760=CARTESIAN_POINT('Ctrl Pts',(0.572986203939546,0.680609082082812,
-7.22732226364026));
#166761=CARTESIAN_POINT('Ctrl Pts',(0.574236965657701,0.677652752658241,
-7.24535763046556));
#166762=CARTESIAN_POINT('Ctrl Pts',(0.575488243539233,0.674729896865504,
-7.2633984982882));
#166763=CARTESIAN_POINT('Ctrl Pts',(0.57675595093358,0.671836782506211,
-7.28144295100099));
#166764=CARTESIAN_POINT('Ctrl Pts',(0.577942718780051,0.669128385353143,
-7.29833531621256));
#166765=CARTESIAN_POINT('Ctrl Pts',(0.579139796495504,0.666446714472475,
-7.31523126529016));
#166766=CARTESIAN_POINT('Ctrl Pts',(0.580346760832762,0.663790956124645,
-7.33213055581337));
#166767=CARTESIAN_POINT('Ctrl Pts',(0.581553738128665,0.661135169263106,
-7.34903002777682));
#166768=CARTESIAN_POINT('Ctrl Pts',(0.582770605614792,0.658505288580088,
-7.36593288621745));
#166769=CARTESIAN_POINT('Ctrl Pts',(0.583996965696794,0.655900535579078,
-7.3828389043069));
#166770=CARTESIAN_POINT('Ctrl Pts',(0.5776675,0.681369595,-7.226949582));
#166771=CARTESIAN_POINT('Ctrl Pts',(0.56905407,0.679970133000001,-7.22763807400001));
#166772=CARTESIAN_POINT('Ctrl Pts',(0.560439023,0.678571429,-7.228306033));
#166773=CARTESIAN_POINT('Ctrl Pts',(0.174321262,0.615882895,-7.25824326300001));
#166774=CARTESIAN_POINT('Ctrl Pts',(-0.212788494,0.552026826,-7.246876641));
#166775=CARTESIAN_POINT('Ctrl Pts',(0.744760437,0.681369595,-7.36930737600001));
#166776=CARTESIAN_POINT('Ctrl Pts',(0.735977338,0.679970133000001,-7.37019501800001));
#166777=CARTESIAN_POINT('Ctrl Pts',(0.727192148,0.678571429,-7.371061721));
#166778=CARTESIAN_POINT('Ctrl Pts',(0.33344874,0.615882895,-7.409906479));
#166779=CARTESIAN_POINT('Ctrl Pts',(-0.062192196,0.552026826,-7.40658433));
#166780=CARTESIAN_POINT('',(-0.187488157518674,0.552026824384641,-7.27370769075728));
#166781=CARTESIAN_POINT('Ctrl Pts',(0.162567224,0.499686101,-7.300530302));
#166782=CARTESIAN_POINT('Ctrl Pts',(0.050868142,0.51775868,-7.30301760200001));
#166783=CARTESIAN_POINT('Ctrl Pts',(-0.060854751,0.535714286,-7.302086516));
#166784=CARTESIAN_POINT('Ctrl Pts',(-0.111526666,0.54385805,-7.301664223));
#166785=CARTESIAN_POINT('Ctrl Pts',(-0.162187841,0.552026826,-7.30053874));
#166786=CARTESIAN_POINT('Ctrl Pts',(0.1096307,0.499686101,-7.249171064));
#166787=CARTESIAN_POINT('Ctrl Pts',(-0.00128258,0.51775868,-7.250848428));
#166788=CARTESIAN_POINT('Ctrl Pts',(-0.112195259,0.535714286,-7.249131826));
#166789=CARTESIAN_POINT('Ctrl Pts',(-0.162499702,0.54385805,-7.248353261));
#166790=CARTESIAN_POINT('Ctrl Pts',(-0.212788494,0.552026826,-7.246876641));
#166791=CARTESIAN_POINT('Ctrl Pts',(-0.212788494593637,0.552026826142908,
-7.24687664176387));
#166792=CARTESIAN_POINT('Ctrl Pts',(-0.179238032192001,0.546576979665154,
-7.24786177688672));
#166793=CARTESIAN_POINT('Ctrl Pts',(-0.145705350411296,0.541139220209299,
-7.24861318818257));
#166794=CARTESIAN_POINT('Ctrl Pts',(-0.112195259273809,0.535714286044326,
-7.24913182599576));
#166795=CARTESIAN_POINT('Ctrl Pts',(-0.0390208298560378,0.523868109072172,
-7.2502643509093));
#166796=CARTESIAN_POINT('Ctrl Pts',(0.0342956684092109,0.511960761022386,
-7.25029060206938));
#166797=CARTESIAN_POINT('Ctrl Pts',(0.107704216070513,0.499999999886365,
-7.24919994256545));
#166798=CARTESIAN_POINT('Ctrl Pts',(0.1096307,0.499686101,-7.249171064));
#166799=CARTESIAN_POINT('Ctrl Pts',(-0.00128258,0.51775868,-7.250848428));
#166800=CARTESIAN_POINT('Ctrl Pts',(-0.112195259,0.535714286,-7.249131826));
#166801=CARTESIAN_POINT('Ctrl Pts',(-0.163461379,0.544013736,-7.248338377));
#166802=CARTESIAN_POINT('Ctrl Pts',(-0.214711149,0.552339147,-7.24681993199999));
#166803=CARTESIAN_POINT('Ctrl Pts',(0.0654135539999999,0.499686101,-7.29474615600001));
#166804=CARTESIAN_POINT('Ctrl Pts',(-0.0461970310000001,0.51775868,-7.29574699200001));
#166805=CARTESIAN_POINT('Ctrl Pts',(-0.157785991,0.535714286,-7.293332845));
#166806=CARTESIAN_POINT('Ctrl Pts',(-0.209364702,0.544013736,-7.292216977));
#166807=CARTESIAN_POINT('Ctrl Pts',(-0.260922472,0.552339147,-7.290371724));
#166808=CARTESIAN_POINT('Ctrl Pts',(-0.212788500831279,0.552026827156134,
-7.24687664158071));
#166809=CARTESIAN_POINT('Ctrl Pts',(-0.212901620729526,0.55117230828004,
-7.25209826172077));
#166810=CARTESIAN_POINT('Ctrl Pts',(-0.213013860674674,0.550320534954775,
-7.25732034620402));
#166811=CARTESIAN_POINT('Ctrl Pts',(-0.213125225767415,0.549471478053454,
-7.26254289021273));
#166812=CARTESIAN_POINT('Ctrl Pts',(-0.213228612902325,0.548683245778484,
-7.26739130230232));
#166813=CARTESIAN_POINT('Ctrl Pts',(-0.213331246070747,0.547897354466547,
-7.27224011173801));
#166814=CARTESIAN_POINT('Ctrl Pts',(-0.213433133333021,0.547113782419621,
-7.27708931097543));
#166815=CARTESIAN_POINT('Ctrl Pts',(-0.213535020698245,0.54633020958094,
-7.2819385151127));
#166816=CARTESIAN_POINT('Ctrl Pts',(-0.21363616218058,0.545548955814703,
-7.28678811027582));
#166817=CARTESIAN_POINT('Ctrl Pts',(-0.213736567463141,0.544769999955344,
-7.29163808927306));
#166818=CARTESIAN_POINT('Ctrl Pts',(-0.21090248,0.55233793,-7.246931774));
#166819=CARTESIAN_POINT('Ctrl Pts',(-0.370162096,0.526068113,-7.24229695100001));
#166820=CARTESIAN_POINT('Ctrl Pts',(-0.529064344,0.49968693,-7.230670157));
#166821=CARTESIAN_POINT('Ctrl Pts',(-0.167326407,0.55233793,-7.293120202));
#166822=CARTESIAN_POINT('Ctrl Pts',(-0.327601066,0.526068113,-7.289443013));
#166823=CARTESIAN_POINT('Ctrl Pts',(-0.487559448,0.49968693,-7.278728336));
#166824=CARTESIAN_POINT('Origin',(0.029039077562356,0.410742974322117,0.194940242366671));
#166825=CARTESIAN_POINT('Ctrl Pts',(-0.263266283044498,0.552548454735263,
-7.2975935627527));
#166826=CARTESIAN_POINT('Ctrl Pts',(-0.264858438022249,0.552287640367631,
-7.29753542887635));
#166827=CARTESIAN_POINT('Ctrl Pts',(-0.266450593,0.552026826,-7.297477295));
#166828=CARTESIAN_POINT('Ctrl Pts',(-0.425870961,0.525911829,-7.291656427));
#166829=CARTESIAN_POINT('Ctrl Pts',(-0.584885032,0.49968693,-7.278879055));
#166830=CARTESIAN_POINT('Ctrl Pts',(-0.209617462986227,0.552548454735263,
-7.2469611866814));
#166831=CARTESIAN_POINT('Ctrl Pts',(-0.21119857615827,0.552287640367631,
-7.24691476266089));
#166832=CARTESIAN_POINT('Ctrl Pts',(-0.212779689330313,0.552026826,-7.24686833864037));
#166833=CARTESIAN_POINT('Ctrl Pts',(-0.371094455957274,0.525911829,-7.24221996298682));
#166834=CARTESIAN_POINT('Ctrl Pts',(-0.529055185157377,0.49968693,-7.23066224707044));
#166835=CARTESIAN_POINT('',(-0.292642328452178,0.552026824384643,-7.32217479090157));
#166836=CARTESIAN_POINT('Ctrl Pts',(-0.204938109066285,0.550751630586317,
-7.24710715016635));
#166837=CARTESIAN_POINT('Ctrl Pts',(-0.208863301533143,0.551389228293159,
-7.24699189558317));
#166838=CARTESIAN_POINT('Ctrl Pts',(-0.212788494,0.552026826,-7.246876641));
#166839=CARTESIAN_POINT('Ctrl Pts',(-0.607566848,0.61615356,-7.23528484900001));
#166840=CARTESIAN_POINT('Ctrl Pts',(-0.998749843,0.681389364000001,-7.180877297));
#166841=CARTESIAN_POINT('Ctrl Pts',(-0.364482660369832,0.550751630586317,
-7.39787645705584));
#166842=CARTESIAN_POINT('Ctrl Pts',(-0.368489421684916,0.551389228293159,
-7.39767469852792));
#166843=CARTESIAN_POINT('Ctrl Pts',(-0.372496183,0.552026826,-7.39747294));
#166844=CARTESIAN_POINT('Ctrl Pts',(-0.775478368000001,0.61615356,-7.377180967));
#166845=CARTESIAN_POINT('Ctrl Pts',(-1.173871557,0.681389364000001,-7.313233544));
#166846=CARTESIAN_POINT('Ctrl Pts',(-0.994070543983947,0.680609082247612,
-7.18152658128588));
#166847=CARTESIAN_POINT('Ctrl Pts',(-0.996726094868221,0.677652752727981,
-7.19940916869543));
#166848=CARTESIAN_POINT('Ctrl Pts',(-0.999382324343535,0.674729896879857,
-7.21729723888549));
#166849=CARTESIAN_POINT('Ctrl Pts',(-1.00202327928226,0.671836782506551,
-7.23519234198709));
#166850=CARTESIAN_POINT('Ctrl Pts',(-1.00449561666871,0.669128385356906,
-7.25194489303733));
#166851=CARTESIAN_POINT('Ctrl Pts',(-1.00695865563338,0.666446714481601,
-7.26870316048478));
#166852=CARTESIAN_POINT('Ctrl Pts',(-1.00941275741744,0.663790956140528,
-7.28546681659049));
#166853=CARTESIAN_POINT('Ctrl Pts',(-1.01186688555012,0.661135169285732,
-7.3022306526803));
#166854=CARTESIAN_POINT('Ctrl Pts',(-1.01431208269765,0.65850528861085,
-7.31899992217427));
#166855=CARTESIAN_POINT('Ctrl Pts',(-1.01674868797125,0.655900535661223,
-7.33577431833995));
#166856=CARTESIAN_POINT('Ctrl Pts',(-0.989418577999999,0.681369595,-7.182168954));
#166857=CARTESIAN_POINT('Ctrl Pts',(-0.997978637,0.679970133000001,-7.180989716));
#166858=CARTESIAN_POINT('Ctrl Pts',(-1.00653586,0.678571429,-7.179790078));
#166859=CARTESIAN_POINT('Ctrl Pts',(-1.390062022,0.615882895,-7.126023487));
#166860=CARTESIAN_POINT('Ctrl Pts',(-1.76567788,0.552026826,-7.031705456));
#166861=CARTESIAN_POINT('Ctrl Pts',(-0.856834899,0.681369595,-7.357118544));
#166862=CARTESIAN_POINT('Ctrl Pts',(-0.865603471,0.679970133000001,-7.356097326));
#166863=CARTESIAN_POINT('Ctrl Pts',(-0.874369584,0.678571429,-7.35505521));
#166864=CARTESIAN_POINT('Ctrl Pts',(-1.267257964,0.615882895,-7.30834860600001));
#166865=CARTESIAN_POINT('Ctrl Pts',(-1.652934871,0.552026826,-7.220053021));
#166866=CARTESIAN_POINT('',(-1.74673693330736,0.552026824384643,-7.06334803539695));
#166867=CARTESIAN_POINT('Ctrl Pts',(-1.41063172,0.499686101,-7.16479510800001));
#166868=CARTESIAN_POINT('Ctrl Pts',(-1.520254036,0.51775868,-7.143212256));
#166869=CARTESIAN_POINT('Ctrl Pts',(-1.629164754,0.535714286,-7.118285819));
#166870=CARTESIAN_POINT('Ctrl Pts',(-1.678561207,0.54385805,-7.106980434));
#166871=CARTESIAN_POINT('Ctrl Pts',(-1.727796006,0.552026826,-7.09499061));
#166872=CARTESIAN_POINT('Ctrl Pts',(-1.4512899,0.499686101,-7.103256832));
#166873=CARTESIAN_POINT('Ctrl Pts',(-1.559970672,0.51775868,-7.081051904));
#166874=CARTESIAN_POINT('Ctrl Pts',(-1.667921256,0.535714286,-7.055532488));
#166875=CARTESIAN_POINT('Ctrl Pts',(-1.71688224,0.54385805,-7.043958157));
#166876=CARTESIAN_POINT('Ctrl Pts',(-1.76567788,0.552026826,-7.031705456));
#166877=CARTESIAN_POINT('Ctrl Pts',(-1.76567787792048,0.552026825801985,
-7.03170545779501));
#166878=CARTESIAN_POINT('Ctrl Pts',(-1.71387913432024,0.543355306566488,
-7.04471224566189));
#166879=CARTESIAN_POINT('Ctrl Pts',(-1.66198181461837,0.534726112489088,
-7.05713583498964));
#166880=CARTESIAN_POINT('Ctrl Pts',(-1.55780050367311,0.517398614477502,
-7.08086267381247));
#166881=CARTESIAN_POINT('Ctrl Pts',(-1.50555235354915,0.508709450041202,
-7.09215552884824));
#166882=CARTESIAN_POINT('Ctrl Pts',(-1.45317754991343,0.499999999567749,
-7.10287089870231));
#166883=CARTESIAN_POINT('Ctrl Pts',(-1.4512899,0.499686101,-7.103256832));
#166884=CARTESIAN_POINT('Ctrl Pts',(-1.559970672,0.51775868,-7.081051904));
#166885=CARTESIAN_POINT('Ctrl Pts',(-1.667921256,0.535714286,-7.055532488));
#166886=CARTESIAN_POINT('Ctrl Pts',(-1.717818234,0.544013736,-7.043736889));
#166887=CARTESIAN_POINT('Ctrl Pts',(-1.767543392,0.552339147,-7.031236759));
#166888=CARTESIAN_POINT('Ctrl Pts',(-1.504270571,0.499686101,-7.138261025));
#166889=CARTESIAN_POINT('Ctrl Pts',(-1.613486912,0.51775868,-7.11524548600001));
#166890=CARTESIAN_POINT('Ctrl Pts',(-1.721948015,0.535714286,-7.088899452));
#166891=CARTESIAN_POINT('Ctrl Pts',(-1.772080965,0.544013736,-7.076721774));
#166892=CARTESIAN_POINT('Ctrl Pts',(-1.822036668,0.552339147,-7.06383626599999));
#166893=CARTESIAN_POINT('Ctrl Pts',(-1.76567788662873,0.552026827401467,
-7.03170545488938));
#166894=CARTESIAN_POINT('Ctrl Pts',(-1.76691085502878,0.551172308331837,
-7.03678067949942));
#166895=CARTESIAN_POINT('Ctrl Pts',(-1.76814306468081,0.550320534997803,
-7.04185654629875));
#166896=CARTESIAN_POINT('Ctrl Pts',(-1.7693745187319,0.549471478087945,
-7.04693304994408));
#166897=CARTESIAN_POINT('Ctrl Pts',(-1.77051775403243,0.548683245810301,
-7.0516458836592));
#166898=CARTESIAN_POINT('Ctrl Pts',(-1.77166033842302,0.547897354495996,
-7.05635926750844));
#166899=CARTESIAN_POINT('Ctrl Pts',(-1.77280227815134,0.547113782447071,
-7.0610731923917));
#166900=CARTESIAN_POINT('Ctrl Pts',(-1.77394421903353,0.546330209606392,
-7.0657871220381));
#166901=CARTESIAN_POINT('Ctrl Pts',(-1.77508551553932,0.545548955838506,
-7.07050159390896));
#166902=CARTESIAN_POINT('Ctrl Pts',(-1.77622617503589,0.544769999908563,
-7.07521659892975));
#166903=CARTESIAN_POINT('Ctrl Pts',(-1.763847811,0.55233793,-7.032164738));
#166904=CARTESIAN_POINT('Ctrl Pts',(-1.918387675,0.526068113,-6.99340216400001));
#166905=CARTESIAN_POINT('Ctrl Pts',(-2.07107546,0.49968693,-6.947887912));
#166906=CARTESIAN_POINT('Ctrl Pts',(-1.731219669,0.55233793,-7.086640874));
#166907=CARTESIAN_POINT('Ctrl Pts',(-1.886956709,0.526068113,-7.048595341));
#166908=CARTESIAN_POINT('Ctrl Pts',(-2.040872013,0.49968693,-7.003744844));
#166909=CARTESIAN_POINT('Origin',(0.0702668821091162,0.410743074016567,
0.18414131516602));
#166910=CARTESIAN_POINT('Ctrl Pts',(-1.82587816458829,0.552548454735263,
-7.07038541198959));
#166911=CARTESIAN_POINT('Ctrl Pts',(-1.82742059879414,0.552287640367631,
-7.0699863709948));
#166912=CARTESIAN_POINT('Ctrl Pts',(-1.828963033,0.552026826,-7.06958733));
#166913=CARTESIAN_POINT('Ctrl Pts',(-1.983404926,0.525911829,-7.029631884));
#166914=CARTESIAN_POINT('Ctrl Pts',(-2.135954579,0.49968693,-6.982969915));
#166915=CARTESIAN_POINT('Ctrl Pts',(-1.7625991607403,0.552548454735263,
-7.03246970296457));
#166916=CARTESIAN_POINT('Ctrl Pts',(-1.76413332856506,0.552287640367631,
-7.0320844717185));
#166917=CARTESIAN_POINT('Ctrl Pts',(-1.76566749638983,0.552026826,-7.03169924047245));
#166918=CARTESIAN_POINT('Ctrl Pts',(-1.91928168760564,0.525911829,-6.99312654631239));
#166919=CARTESIAN_POINT('Ctrl Pts',(-2.07106481485737,0.49968693,-6.94788215586565));
#166920=CARTESIAN_POINT('',(-1.85985165227342,0.552026824384643,-7.08807696305218));
#166921=CARTESIAN_POINT('Ctrl Pts',(-1.75806058539698,0.550751630586318,
-7.03361817669735));
#166922=CARTESIAN_POINT('Ctrl Pts',(-1.76186923269849,0.551389228293159,
-7.03266181634868));
#166923=CARTESIAN_POINT('Ctrl Pts',(-1.76567788,0.552026826,-7.031705456));
#166924=CARTESIAN_POINT('Ctrl Pts',(-2.148734641,0.61615356,-6.935518997));
#166925=CARTESIAN_POINT('Ctrl Pts',(-2.519075981,0.681389364000001,-6.798290683));
#166926=CARTESIAN_POINT('Ctrl Pts',(-1.94628601731659,0.550751630586318,
-7.14656521854563));
#166927=CARTESIAN_POINT('Ctrl Pts',(-1.9501557306583,0.551389228293159,
-7.14550684177282));
#166928=CARTESIAN_POINT('Ctrl Pts',(-1.954025444,0.552026826,-7.14444846500001));
#166929=CARTESIAN_POINT('Ctrl Pts',(-2.343223955,0.61615356,-7.038001649));
#166930=CARTESIAN_POINT('Ctrl Pts',(-2.718556127,0.681389364000001,-6.889906523));
#166931=CARTESIAN_POINT('Ctrl Pts',(-2.51464565778637,0.680609082082812,
-6.79993069840003));
#166932=CARTESIAN_POINT('Ctrl Pts',(-2.52108335059132,0.677652752711293,
-6.8168243355651));
#166933=CARTESIAN_POINT('Ctrl Pts',(-2.52752288517147,0.674729896859141,
-6.83372318185063));
#166934=CARTESIAN_POINT('Ctrl Pts',(-2.533949014258,0.671836782489221,-6.85063218017266));
#166935=CARTESIAN_POINT('Ctrl Pts',(-2.5399648530648,0.669128385339904,
-6.86646158647935));
#166936=CARTESIAN_POINT('Ctrl Pts',(-2.54597283970899,0.666446714463603,
-6.88229857441854));
#166937=CARTESIAN_POINT('Ctrl Pts',(-2.5519732565292,0.663790956120468,
-6.89814274625858));
#166938=CARTESIAN_POINT('Ctrl Pts',(-2.55797373777326,0.66113516926362,
-6.91398708821056));
#166939=CARTESIAN_POINT('Ctrl Pts',(-2.563966664863,0.658505288585621,-6.9298386564313));
#166940=CARTESIAN_POINT('Ctrl Pts',(-2.56995230272842,0.655900535691932,
-6.94569707849852));
#166941=CARTESIAN_POINT('Ctrl Pts',(-2.510240543,0.681369595,-6.801558087));
#166942=CARTESIAN_POINT('Ctrl Pts',(-2.518346971,0.679970133000001,-6.79856626));
#166943=CARTESIAN_POINT('Ctrl Pts',(-2.526446244,0.678571429,-6.795555119));
#166944=CARTESIAN_POINT('Ctrl Pts',(-2.88944755,0.615882895,-6.660598773));
#166945=CARTESIAN_POINT('Ctrl Pts',(-3.236006129,0.552026826,-6.487739539));
#166946=CARTESIAN_POINT('Ctrl Pts',(-2.418365587,0.681369595,-7.000919025));
#166947=CARTESIAN_POINT('Ctrl Pts',(-2.426709623,0.679970133000001,-6.998036699));
#166948=CARTESIAN_POINT('Ctrl Pts',(-2.435046765,0.678571429,-6.995134492));
#166949=CARTESIAN_POINT('Ctrl Pts',(-2.808709094,0.615882895,-6.865060475));
#166950=CARTESIAN_POINT('Ctrl Pts',(-3.166388148,0.552026826,-6.695920057));
#166951=CARTESIAN_POINT('',(-3.22431023054923,0.552026824384642,-6.52271407592455));
#166952=CARTESIAN_POINT('Ctrl Pts',(-2.917871093,0.499686101,-6.694042058));
#166953=CARTESIAN_POINT('Ctrl Pts',(-3.020290825,0.51775868,-6.649398243));
#166954=CARTESIAN_POINT('Ctrl Pts',(-3.121296823,0.535714286,-6.601641988));
#166955=CARTESIAN_POINT('Ctrl Pts',(-3.167108091,0.54385805,-6.579982139));
#166956=CARTESIAN_POINT('Ctrl Pts',(-3.21261435,0.552026826,-6.557688604));
#166957=CARTESIAN_POINT('Ctrl Pts',(-2.944349797,0.499686101,-6.625202206));
#166958=CARTESIAN_POINT('Ctrl Pts',(-3.04571627,0.51775868,-6.580153264));
#166959=CARTESIAN_POINT('Ctrl Pts',(-3.145657109,0.535714286,-6.532024292));
#166960=CARTESIAN_POINT('Ctrl Pts',(-3.190985273,0.54385805,-6.510195399));
#166961=CARTESIAN_POINT('Ctrl Pts',(-3.236006129,0.552026826,-6.487739539));
#166962=CARTESIAN_POINT('Ctrl Pts',(-3.2360061284921,0.552026826,-6.48773954051878));
#166963=CARTESIAN_POINT('Ctrl Pts',(-3.18821448041655,0.543355305714346,
-6.51157743867596));
#166964=CARTESIAN_POINT('Ctrl Pts',(-3.14020118219395,0.534726109198169,
-6.53486696721718));
#166965=CARTESIAN_POINT('Ctrl Pts',(-3.04355912310762,0.517399145757902,
-6.58043358288906));
#166966=CARTESIAN_POINT('Ctrl Pts',(-2.99495413992492,0.50870890930923,
-6.60269697061331));
#166967=CARTESIAN_POINT('Ctrl Pts',(-2.94611035073431,0.499999999616657,
-6.62441950656244));
#166968=CARTESIAN_POINT('Ctrl Pts',(-2.944349797,0.499686101,-6.625202206));
#166969=CARTESIAN_POINT('Ctrl Pts',(-3.04571627,0.51775868,-6.580153264));
#166970=CARTESIAN_POINT('Ctrl Pts',(-3.145657109,0.535714286,-6.532024292));
#166971=CARTESIAN_POINT('Ctrl Pts',(-3.191851818,0.544013736,-6.50977809300001));
#166972=CARTESIAN_POINT('Ctrl Pts',(-3.237727271,0.552339147,-6.48688077));
#166973=CARTESIAN_POINT('Ctrl Pts',(-3.003616676,0.499686101,-6.64799874200001));
#166974=CARTESIAN_POINT('Ctrl Pts',(-3.105331939,0.51775868,-6.602043008));
#166975=CARTESIAN_POINT('Ctrl Pts',(-3.205593663,0.535714286,-6.552997));
#166976=CARTESIAN_POINT('Ctrl Pts',(-3.251936692,0.544013736,-6.530326927));
#166977=CARTESIAN_POINT('Ctrl Pts',(-3.297954455,0.552339147,-6.507003675));
#166978=CARTESIAN_POINT('Ctrl Pts',(-3.23600613543338,0.552026827322425,
-6.4877395367674));
#166979=CARTESIAN_POINT('Ctrl Pts',(-3.23830130142427,0.551172308398161,
-6.49243105314736));
#166980=CARTESIAN_POINT('Ctrl Pts',(-3.24059586393105,0.550320535064447,
-6.49712336031143));
#166981=CARTESIAN_POINT('Ctrl Pts',(-3.24288982539976,0.549471478157348,
-6.50181645186762));
#166982=CARTESIAN_POINT('Ctrl Pts',(-3.24501945239908,0.548683245862265,
-6.50617334043121));
#166983=CARTESIAN_POINT('Ctrl Pts',(-3.24714856196406,0.547897354532626,
-6.51053090619626));
#166984=CARTESIAN_POINT('Ctrl Pts',(-3.24927715823825,0.547113782470724,
-6.51488913893324));
#166985=CARTESIAN_POINT('Ctrl Pts',(-3.25140575666327,0.546330209617065,
-6.51924737607399));
#166986=CARTESIAN_POINT('Ctrl Pts',(-3.25353384233262,0.545548955838543,
-6.52360628128781));
#166987=CARTESIAN_POINT('Ctrl Pts',(-3.25566142035481,0.544769999879411,
-6.52796584418262));
#166988=CARTESIAN_POINT('Ctrl Pts',(-3.234317579,0.55233793,-6.48858149400001));
#166989=CARTESIAN_POINT('Ctrl Pts',(-3.376911579,0.526068113,-6.417503665));
#166990=CARTESIAN_POINT('Ctrl Pts',(-3.51624539,0.49968693,-6.34023015));
#166991=CARTESIAN_POINT('Ctrl Pts',(-3.214163023,0.55233793,-6.548798094));
#166992=CARTESIAN_POINT('Ctrl Pts',(-3.358080353,0.526068113,-6.478163184));
#166993=CARTESIAN_POINT('Ctrl Pts',(-3.498755672,0.49968693,-6.401274026));
#166994=CARTESIAN_POINT('Origin',(0.108208885721304,0.410743218181082,0.164730669642488));
#166995=CARTESIAN_POINT('Ctrl Pts',(-3.30311401212512,0.552548454735263,
-6.5125738978046));
#166996=CARTESIAN_POINT('Ctrl Pts',(-3.30453460306256,0.552287640367631,
-6.5118526084023));
#166997=CARTESIAN_POINT('Ctrl Pts',(-3.305955194,0.552026826,-6.511131319));
#166998=CARTESIAN_POINT('Ctrl Pts',(-3.448197082,0.525911829,-6.438909567));
#166999=CARTESIAN_POINT('Ctrl Pts',(-3.587149265,0.49968693,-6.360544862));
#167000=CARTESIAN_POINT('Ctrl Pts',(-3.23316367901391,0.552548454735263,
-6.48914775193897));
#167001=CARTESIAN_POINT('Ctrl Pts',(-3.234579165521,0.552287640367631,-6.48844172645311));
#167002=CARTESIAN_POINT('Ctrl Pts',(-3.2359946520281,0.552026826,-6.48773570096726));
#167003=CARTESIAN_POINT('Ctrl Pts',(-3.37772544018258,0.525911829,-6.41704230469282));
#167004=CARTESIAN_POINT('Ctrl Pts',(-3.51623375636657,0.49968693,-6.34022681684067));
#167005=CARTESIAN_POINT('',(-3.34009637854947,0.552026824384643,-6.52254853458343));
#167006=CARTESIAN_POINT('Ctrl Pts',(-3.22897810090943,0.550751630586318,
-6.49124503453278));
#167007=CARTESIAN_POINT('Ctrl Pts',(-3.23249211495472,0.551389228293159,
-6.48949228676639));
#167008=CARTESIAN_POINT('Ctrl Pts',(-3.236006129,0.552026826,-6.487739539));
#167009=CARTESIAN_POINT('Ctrl Pts',(-3.589429991,0.61615356,-6.311455985));
#167010=CARTESIAN_POINT('Ctrl Pts',(-3.921612925,0.681389364,-6.09782355200001));
#167011=CARTESIAN_POINT('Ctrl Pts',(-3.43708320223719,0.550751630586318,
-6.56108853400832));
#167012=CARTESIAN_POINT('Ctrl Pts',(-3.44063492411859,0.551389228293159,
-6.55922302750416));
#167013=CARTESIAN_POINT('Ctrl Pts',(-3.444186646,0.552026826,-6.557357521));
#167014=CARTESIAN_POINT('Ctrl Pts',(-3.801402994,0.61615356,-6.369733196));
#167015=CARTESIAN_POINT('Ctrl Pts',(-4.136124034,0.681389364,-6.14441513));
#167016=CARTESIAN_POINT('Ctrl Pts',(-3.91763873527765,0.680609082082812,
-6.10037761323453));
#167017=CARTESIAN_POINT('Ctrl Pts',(-3.9275575515231,0.6776527527834,-6.11549237277444));
#167018=CARTESIAN_POINT('Ctrl Pts',(-3.9374792857128,0.67472989692545,-6.13061182384924));
#167019=CARTESIAN_POINT('Ctrl Pts',(-3.94739011022992,0.671836782553413,
-6.1457440713838));
#167020=CARTESIAN_POINT('Ctrl Pts',(-3.95666815648968,0.669128385393101,
-6.15991016749386));
#167021=CARTESIAN_POINT('Ctrl Pts',(-3.96594016399478,0.666446714505989,
-6.17408535596371));
#167022=CARTESIAN_POINT('Ctrl Pts',(-3.97520632298163,0.663790956152371,
-6.18826918766651));
#167023=CARTESIAN_POINT('Ctrl Pts',(-3.98447258145517,0.66113516928504,
-6.2024531716549));
#167024=CARTESIAN_POINT('Ctrl Pts',(-3.99373301582162,0.658505288596885,
-6.2166458368851));
#167025=CARTESIAN_POINT('Ctrl Pts',(-4.00298780534354,0.655900535589649,
-6.23084676214381));
#167026=CARTESIAN_POINT('Ctrl Pts',(-3.91368645,0.681369595,-6.102913924));
#167027=CARTESIAN_POINT('Ctrl Pts',(-3.9209602,0.679970133000001,-6.098249402));
#167028=CARTESIAN_POINT('Ctrl Pts',(-3.928222811,0.678571429,-6.093567555));
#167029=CARTESIAN_POINT('Ctrl Pts',(-4.253725723,0.615882895,-5.883731863));
#167030=CARTESIAN_POINT('Ctrl Pts',(-4.55502232900001,0.552026826,-5.640414132));
#167031=CARTESIAN_POINT('Ctrl Pts',(-3.866816188,0.681369595,-6.317364314));
#167032=CARTESIAN_POINT('Ctrl Pts',(-3.874345531,0.679970133000001,-6.312755654));
#167033=CARTESIAN_POINT('Ctrl Pts',(-3.881863866,0.678571429,-6.30812906));
#167034=CARTESIAN_POINT('Ctrl Pts',(-4.218828109,0.615882895,-6.100769745));
#167035=CARTESIAN_POINT('Ctrl Pts',(-4.531784635,0.552026826,-5.85869331300001));
#167036=CARTESIAN_POINT('',(-4.55111836570588,0.552026824383862,-5.67708525624827));
#167037=CARTESIAN_POINT('Ctrl Pts',(-4.288674056,0.499686101,-5.910283042));
#167038=CARTESIAN_POINT('Ctrl Pts',(-4.379102171,0.51775868,-5.844665759));
#167039=CARTESIAN_POINT('Ctrl Pts',(-4.467480522,0.535714286,-5.776312715));
#167040=CARTESIAN_POINT('Ctrl Pts',(-4.507564521,0.54385805,-5.745311193));
#167041=CARTESIAN_POINT('Ctrl Pts',(-4.547214418,0.552026826,-5.713756368));
#167042=CARTESIAN_POINT('Ctrl Pts',(-4.29973517,0.499686101,-5.837360488));
#167043=CARTESIAN_POINT('Ctrl Pts',(-4.38904756,0.51775868,-5.77157397));
#167044=CARTESIAN_POINT('Ctrl Pts',(-4.476305531,0.535714286,-5.703085901));
#167045=CARTESIAN_POINT('Ctrl Pts',(-4.51588138099999,0.54385805,-5.672023139));
#167046=CARTESIAN_POINT('Ctrl Pts',(-4.555022329,0.552026826,-5.640414132));
#167047=CARTESIAN_POINT('Ctrl Pts',(-4.55502232574641,0.552026825573623,
-5.64041413432871));
#167048=CARTESIAN_POINT('Ctrl Pts',(-4.5289092151985,0.546576979320718,
-5.66150226752041));
#167049=CARTESIAN_POINT('Ctrl Pts',(-4.50266881557143,0.541139220053964,
-5.68239357447142));
#167050=CARTESIAN_POINT('Ctrl Pts',(-4.47630553125182,0.535714286005299,
-5.70308590100704));
#167051=CARTESIAN_POINT('Ctrl Pts',(-4.41873725026094,0.523868108875745,
-5.74827077517669));
#167052=CARTESIAN_POINT('Ctrl Pts',(-4.36038638074774,0.511960760877559,
-5.79266092730607));
#167053=CARTESIAN_POINT('Ctrl Pts',(-4.30128630597295,0.499999999668149,
-5.8362176204432));
#167054=CARTESIAN_POINT('Ctrl Pts',(-4.29973517,0.499686101,-5.837360488));
#167055=CARTESIAN_POINT('Ctrl Pts',(-4.38904756,0.51775868,-5.77157397));
#167056=CARTESIAN_POINT('Ctrl Pts',(-4.476305531,0.535714286,-5.703085901));
#167057=CARTESIAN_POINT('Ctrl Pts',(-4.516637959,0.544013736,-5.671429308));
#167058=CARTESIAN_POINT('Ctrl Pts',(-4.556518621,0.552339147,-5.639205445));
#167059=CARTESIAN_POINT('Ctrl Pts',(-4.362517003,0.499686101,-5.84688342700001));
#167060=CARTESIAN_POINT('Ctrl Pts',(-4.451975096,0.51775868,-5.780136338));
#167061=CARTESIAN_POINT('Ctrl Pts',(-4.539349314,0.535714286,-5.710683691));
#167062=CARTESIAN_POINT('Ctrl Pts',(-4.579735474,0.544013736,-5.67858125));
#167063=CARTESIAN_POINT('Ctrl Pts',(-4.619663557,0.552339147,-5.645910824));
#167064=CARTESIAN_POINT('Ctrl Pts',(-4.55502233394114,0.552026827283876,
-5.6404141277109));
#167065=CARTESIAN_POINT('Ctrl Pts',(-4.55827237826771,0.551172308283001,
-5.64450256670423));
#167066=CARTESIAN_POINT('Ctrl Pts',(-4.56152200254063,0.550320534963249,
-5.64859190724774));
#167067=CARTESIAN_POINT('Ctrl Pts',(-4.56477120845016,0.549471478067904,
-5.65268214304781));
#167068=CARTESIAN_POINT('Ctrl Pts',(-4.56778764820871,0.548683245789709,
-5.65647936311718));
#167069=CARTESIAN_POINT('Ctrl Pts',(-4.57080372820987,0.547897354475107,
-5.66027735578707));
#167070=CARTESIAN_POINT('Ctrl Pts',(-4.57381945031748,0.547113782422384,
-5.66407611019601));
#167071=CARTESIAN_POINT('Ctrl Pts',(-4.57683517544067,0.546330209586128,
-5.66787486840351));
#167072=CARTESIAN_POINT('Ctrl Pts',(-4.57985054342965,0.545548955819245,
-5.67167438931052));
#167073=CARTESIAN_POINT('Ctrl Pts',(-4.58286555741887,0.544770000006238,
-5.67547466108768));
#167074=CARTESIAN_POINT('Ctrl Pts',(-4.553554251,0.55233793,-5.641599391));
#167075=CARTESIAN_POINT('Ctrl Pts',(-4.677534851,0.526068113,-5.541529827));
#167076=CARTESIAN_POINT('Ctrl Pts',(-4.796999593,0.49968693,-5.436110273));
#167077=CARTESIAN_POINT('Ctrl Pts',(-4.546815687,0.55233793,-5.704740794));
#167078=CARTESIAN_POINT('Ctrl Pts',(-4.672183892,0.526068113,-5.604819318));
#167079=CARTESIAN_POINT('Ctrl Pts',(-4.793041404,0.49968693,-5.49948675));
#167080=CARTESIAN_POINT('Origin',(0.141090736557263,0.410743122402995,0.137617013932505));
#167081=CARTESIAN_POINT('Ctrl Pts',(-4.62589992017682,0.552548454735263,
-5.65024166521514));
#167082=CARTESIAN_POINT('Ctrl Pts',(-4.62713224258841,0.552287640367631,
-5.64923185410757));
#167083=CARTESIAN_POINT('Ctrl Pts',(-4.628364565,0.552026826,-5.64822204299999));
#167084=CARTESIAN_POINT('Ctrl Pts',(-4.751755375,0.525911829,-5.547110995));
#167085=CARTESIAN_POINT('Ctrl Pts',(-4.870612837,0.49968693,-5.440707802));
#167086=CARTESIAN_POINT('Ctrl Pts',(-4.55254905799952,0.552548454735263,
-5.64240046442604));
#167087=CARTESIAN_POINT('Ctrl Pts',(-4.55377967661359,0.552287640367631,
-5.6414066576638));
#167088=CARTESIAN_POINT('Ctrl Pts',(-4.55501029522768,0.552026826,-5.64041285090157));
#167089=CARTESIAN_POINT('Ctrl Pts',(-4.67823050624091,0.525911829,-5.54090429679079));
#167090=CARTESIAN_POINT('Ctrl Pts',(-4.79698751476151,0.49968693,-5.43610951865134));
#167091=CARTESIAN_POINT('',(-4.66416191124399,0.552026824384635,-5.65203298540041));
#167092=CARTESIAN_POINT('Ctrl Pts',(-4.54891219022449,0.550751630586317,
-5.64534848929436));
#167093=CARTESIAN_POINT('Ctrl Pts',(-4.55196725961225,0.551389228293159,
-5.64288131064718));
#167094=CARTESIAN_POINT('Ctrl Pts',(-4.555022329,0.552026826,-5.640414132));
#167095=CARTESIAN_POINT('Ctrl Pts',(-4.862287584,0.61615356,-5.392276306));
#167096=CARTESIAN_POINT('Ctrl Pts',(-5.14077960699999,0.681389364000001,
-5.112228969));
#167097=CARTESIAN_POINT('Ctrl Pts',(-4.76716619730485,0.550751630586317,
-5.66882264040786));
#167098=CARTESIAN_POINT('Ctrl Pts',(-4.77023385315242,0.551389228293159,
-5.66623723320393));
#167099=CARTESIAN_POINT('Ctrl Pts',(-4.773301509,0.552026826,-5.663651826));
#167100=CARTESIAN_POINT('Ctrl Pts',(-5.081832654,0.61615356,-5.403623099));
#167101=CARTESIAN_POINT('Ctrl Pts',(-5.360291378,0.681389364000001,-5.11161771400001));
#167102=CARTESIAN_POINT('Ctrl Pts',(-5.137447379847,0.680609082082805,-5.11557765142985));
#167103=CARTESIAN_POINT('Ctrl Pts',(-5.15038352582319,0.677652752674818,
-5.12820678402029));
#167104=CARTESIAN_POINT('Ctrl Pts',(-5.16332353063032,0.674729896868104,
-5.14083987093191));
#167105=CARTESIAN_POINT('Ctrl Pts',(-5.17625563150039,0.67183678250658,
-5.15348780056847));
#167106=CARTESIAN_POINT('Ctrl Pts',(-5.18836205414182,0.669128385351123,
-5.16532819550953));
#167107=CARTESIAN_POINT('Ctrl Pts',(-5.20046453379357,0.666446714469152,
-5.17717876839636));
#167108=CARTESIAN_POINT('Ctrl Pts',(-5.21256315969722,0.663790956120692,
-5.18903903970536));
#167109=CARTESIAN_POINT('Ctrl Pts',(-5.22466191549854,0.661135169258514,
-5.20089943835291));
#167110=CARTESIAN_POINT('Ctrl Pts',(-5.23675684956298,0.658505288575528,
-5.21276956729518));
#167111=CARTESIAN_POINT('Ctrl Pts',(-5.24884804614103,0.655900535635267,
-5.2246489769404));
#167112=CARTESIAN_POINT('Ctrl Pts',(-5.134132729,0.681369595,-5.118904289));
#167113=CARTESIAN_POINT('Ctrl Pts',(-5.140233688,0.679970133,-5.11278518));
#167114=CARTESIAN_POINT('Ctrl Pts',(-5.146320044,0.678571429,-5.106651545));
#167115=CARTESIAN_POINT('Ctrl Pts',(-5.419104408,0.615882895,-4.831748191));
#167116=CARTESIAN_POINT('Ctrl Pts',(-5.661050747,0.552026826,-4.529349229));
#167117=CARTESIAN_POINT('Ctrl Pts',(-5.134458762,0.681369595,-5.338416669));
#167118=CARTESIAN_POINT('Ctrl Pts',(-5.140821347,0.679970133,-5.33229717100001));
#167119=CARTESIAN_POINT('Ctrl Pts',(-5.147169327,0.678571429,-5.326162524));
#167120=CARTESIAN_POINT('Ctrl Pts',(-5.43167941,0.615882895,-5.051213803));
#167121=CARTESIAN_POINT('Ctrl Pts',(-5.685279909,0.552026826,-4.747520581));
#167122=CARTESIAN_POINT('',(-5.66512126373428,0.552026824384634,-4.56600223927398));
#167123=CARTESIAN_POINT('Ctrl Pts',(-5.458943387,0.499686101,-4.85016575900001));
#167124=CARTESIAN_POINT('Ctrl Pts',(-5.533151567,0.51775868,-4.766643201));
#167125=CARTESIAN_POINT('Ctrl Pts',(-5.604769797,0.535714286,-4.680889479));
#167126=CARTESIAN_POINT('Ctrl Pts',(-5.637252244,0.54385805,-4.641995881));
#167127=CARTESIAN_POINT('Ctrl Pts',(-5.669191793,0.552026826,-4.602655234));
#167128=CARTESIAN_POINT('Ctrl Pts',(-5.454069705,0.499686101,-4.776570282));
#167129=CARTESIAN_POINT('Ctrl Pts',(-5.527151864,0.51775868,-4.69312229100001));
#167130=CARTESIAN_POINT('Ctrl Pts',(-5.597646882,0.535714286,-4.607477551));
#167131=CARTESIAN_POINT('Ctrl Pts',(-5.629619895,0.54385805,-4.568633382));
#167132=CARTESIAN_POINT('Ctrl Pts',(-5.661050747,0.552026826,-4.529349229));
#167133=CARTESIAN_POINT('Ctrl Pts',(-5.66105074078458,0.552026824384634,
-4.52934923676839));
#167134=CARTESIAN_POINT('Ctrl Pts',(-5.64008146987551,0.546576979226268,
-4.55555788184023));
#167135=CARTESIAN_POINT('Ctrl Pts',(-5.61894557098121,0.541139220351658,
-4.58160167019615));
#167136=CARTESIAN_POINT('Ctrl Pts',(-5.59764688197218,0.535714285992477,
-4.6074775510536));
#167137=CARTESIAN_POINT('Ctrl Pts',(-5.55113792654149,0.523868108732891,
-4.66398150703629));
#167138=CARTESIAN_POINT('Ctrl Pts',(-5.50369384036136,0.511960761028742,
-4.71987755304587));
#167139=CARTESIAN_POINT('Ctrl Pts',(-5.45533889445124,0.499999999895942,
-4.7751206845917));
#167140=CARTESIAN_POINT('Ctrl Pts',(-5.454069705,0.499686101,-4.776570282));
#167141=CARTESIAN_POINT('Ctrl Pts',(-5.527151864,0.51775868,-4.69312229100001));
#167142=CARTESIAN_POINT('Ctrl Pts',(-5.597646882,0.535714286,-4.607477551));
#167143=CARTESIAN_POINT('Ctrl Pts',(-5.630231128,0.544013736,-4.567890792));
#167144=CARTESIAN_POINT('Ctrl Pts',(-5.662252225,0.552339147,-4.527847142));
#167145=CARTESIAN_POINT('Ctrl Pts',(-5.517430884,0.499686101,-4.772374341));
#167146=CARTESIAN_POINT('Ctrl Pts',(-5.590448845,0.51775868,-4.68795691599999));
#167147=CARTESIAN_POINT('Ctrl Pts',(-5.660850037,0.535714286,-4.601345159));
#167148=CARTESIAN_POINT('Ctrl Pts',(-5.693390914,0.544013736,-4.561311425));
#167149=CARTESIAN_POINT('Ctrl Pts',(-5.725362325,0.552339147,-4.520821458));
#167150=CARTESIAN_POINT('Ctrl Pts',(-5.6610507513522,0.552026827290018,
-4.52934922382194));
#167151=CARTESIAN_POINT('Ctrl Pts',(-5.66510370465548,0.551172308350208,
-4.5326434135973));
#167152=CARTESIAN_POINT('Ctrl Pts',(-5.66915644181873,0.550320535011006,
-4.53593857447903));
#167153=CARTESIAN_POINT('Ctrl Pts',(-5.67320896285281,0.549471478098695,
-4.53923469962419));
#167154=CARTESIAN_POINT('Ctrl Pts',(-5.67697116994167,0.548683245808849,
-4.54229469740892));
#167155=CARTESIAN_POINT('Ctrl Pts',(-5.68073319176982,0.547897354484637,
-4.54535552706958));
#167156=CARTESIAN_POINT('Ctrl Pts',(-5.68449502780371,0.547113782428027,
-4.54841717758078));
#167157=CARTESIAN_POINT('Ctrl Pts',(-5.68825686763873,0.54633020957966,
-4.55147883118561));
#167158=CARTESIAN_POINT('Ctrl Pts',(-5.69201852262752,0.545548955806292,
-4.5545413064157));
#167159=CARTESIAN_POINT('Ctrl Pts',(-5.69577999340436,0.544769999894628,
-4.55760459146533));
#167160=CARTESIAN_POINT('Ctrl Pts',(-5.659871788,0.55233793,-4.53082237));
#167161=CARTESIAN_POINT('Ctrl Pts',(-5.759441792,0.526068113,-4.406440213));
#167162=CARTESIAN_POINT('Ctrl Pts',(-5.853451427,0.49968693,-4.277803922));
#167163=CARTESIAN_POINT('Ctrl Pts',(-5.666864302,0.55233793,-4.593936154));
#167164=CARTESIAN_POINT('Ctrl Pts',(-5.767821305,0.526068113,-4.469400329));
#167165=CARTESIAN_POINT('Ctrl Pts',(-5.863209847,0.49968693,-4.340549585));
#167166=CARTESIAN_POINT('Origin',(0.167376173419037,0.410743101075361,0.104069638273634));
#167167=CARTESIAN_POINT('Ctrl Pts',(-5.73238388827847,0.552548454735263,
-4.52371041336006));
#167168=CARTESIAN_POINT('Ctrl Pts',(-5.73337032013923,0.552287640367632,
-4.52245929818003));
#167169=CARTESIAN_POINT('Ctrl Pts',(-5.734356752,0.552026826,-4.521208183));
#167170=CARTESIAN_POINT('Ctrl Pts',(-5.833126867,0.525911829,-4.395935678));
#167171=CARTESIAN_POINT('Ctrl Pts',(-5.926331967,0.49968693,-4.266469291));
#167172=CARTESIAN_POINT('Ctrl Pts',(-5.65906230248553,0.552548454735263,
-4.53182080222694));
#167173=CARTESIAN_POINT('Ctrl Pts',(-5.6600505108422,0.552287640367632,
-4.5305856834911));
#167174=CARTESIAN_POINT('Ctrl Pts',(-5.66103871919887,0.552026826,-4.52935056475526));
#167175=CARTESIAN_POINT('Ctrl Pts',(-5.75998671237974,0.525911829,-4.40567976251412));
#167176=CARTESIAN_POINT('Ctrl Pts',(-5.85343946900773,0.49968693,-4.27780578174788));
#167177=CARTESIAN_POINT('',(-5.77013641680195,0.552026824384827,-4.51723465591715));
#167178=CARTESIAN_POINT('Ctrl Pts',(-5.65614292522696,0.550751630586318,
-4.53548186325545));
#167179=CARTESIAN_POINT('Ctrl Pts',(-5.65859619839297,0.551389228293159,
-4.53241561695019));
#167180=CARTESIAN_POINT('Ctrl Pts',(-5.66104947155899,0.552026826000001,
-4.52934937064493));
#167181=CARTESIAN_POINT('Ctrl Pts',(-5.9077887462752,0.61615356,-4.22095999112541));
#167182=CARTESIAN_POINT('Ctrl Pts',(-6.11956789649333,0.681389364,-3.88759252035654));
#167183=CARTESIAN_POINT('Ctrl Pts',(-5.87434179975964,0.550751630586318,
-4.51148890129795));
#167184=CARTESIAN_POINT('Ctrl Pts',(-5.87678194937982,0.551389228293159,
-4.50830448414898));
#167185=CARTESIAN_POINT('Ctrl Pts',(-5.879222099,0.552026826000001,-4.505120067));
#167186=CARTESIAN_POINT('Ctrl Pts',(-6.124641466,0.61615356,-4.184845591));
#167187=CARTESIAN_POINT('Ctrl Pts',(-6.333817454,0.681389364000001,-3.839806735));
#167188=CARTESIAN_POINT('Ctrl Pts',(-6.11703469536907,0.680609082247603,
-3.89157896392074));
#167189=CARTESIAN_POINT('Ctrl Pts',(-6.13238329170514,0.677652752674814,
-3.90113194489534));
#167190=CARTESIAN_POINT('Ctrl Pts',(-6.14773650636248,0.674729896768819,
-3.91068795923836));
#167191=CARTESIAN_POINT('Ctrl Pts',(-6.16308519293365,0.671836782400283,
-3.92026016792834));
#167192=CARTESIAN_POINT('Ctrl Pts',(-6.17745390895607,0.669128385262255,
-3.92922121796579));
#167193=CARTESIAN_POINT('Ctrl Pts',(-6.19182096212797,0.666446714395948,
-3.93819305562519));
#167194=CARTESIAN_POINT('Ctrl Pts',(-6.20618633652179,0.663790956061759,
-3.94717519340858));
#167195=CARTESIAN_POINT('Ctrl Pts',(-6.22055186515037,0.661135169213851,
-3.95615742762927));
#167196=CARTESIAN_POINT('Ctrl Pts',(-6.23491575311536,0.658505288543741,
-3.96514998621989));
#167197=CARTESIAN_POINT('Ctrl Pts',(-6.24927798598832,0.655900535655765,
-3.97415241251114));
#167198=CARTESIAN_POINT('Ctrl Pts',(-6.114512667,0.681369595,-3.895540379));
#167199=CARTESIAN_POINT('Ctrl Pts',(-6.119155562,0.679970133,-3.888252805));
#167200=CARTESIAN_POINT('Ctrl Pts',(-6.123781072,0.678571429,-3.880954185));
#167201=CARTESIAN_POINT('Ctrl Pts',(-6.331091794,0.615882895,-3.553837343));
#167202=CARTESIAN_POINT('Ctrl Pts',(-6.502374724,0.552026826,-3.20649699));
#167203=CARTESIAN_POINT('Ctrl Pts',(-6.162019751,0.681369595,-4.109850593));
#167204=CARTESIAN_POINT('Ctrl Pts',(-6.166918071,0.679970133,-4.102506398));
#167205=CARTESIAN_POINT('Ctrl Pts',(-6.171798871,0.678571429,-4.095150548));
#167206=CARTESIAN_POINT('Ctrl Pts',(-6.390551418,0.615882895,-3.765468718));
#167207=CARTESIAN_POINT('Ctrl Pts',(-6.572937813,0.552026826,-3.414359063));
#167208=CARTESIAN_POINT('',(-6.51422938855193,0.552026824384625,-3.24141803243923));
#167209=CARTESIAN_POINT('Ctrl Pts',(-6.373958593,0.499686101,-3.563260116));
#167210=CARTESIAN_POINT('Ctrl Pts',(-6.42847694499999,0.51775868,-3.465737703));
#167211=CARTESIAN_POINT('Ctrl Pts',(-6.479986266,0.535714286,-3.366593053));
#167212=CARTESIAN_POINT('Ctrl Pts',(-6.503348317,0.54385805,-3.321626));
#167213=CARTESIAN_POINT('Ctrl Pts',(-6.526084062,0.552026826000001,-3.276339057));
#167214=CARTESIAN_POINT('Ctrl Pts',(-6.353378002,0.499686101,-3.492432958));
#167215=CARTESIAN_POINT('Ctrl Pts',(-6.40681269,0.51775868,-3.395225431));
#167216=CARTESIAN_POINT('Ctrl Pts',(-6.457248486,0.535714286,-3.296428672));
#167217=CARTESIAN_POINT('Ctrl Pts',(-6.48012364,0.54385805,-3.251619405));
#167218=CARTESIAN_POINT('Ctrl Pts',(-6.502374724,0.552026826000001,-3.20649699));
#167219=CARTESIAN_POINT('Ctrl Pts',(-6.50237472430817,0.552026826188107,
-3.20649698942514));
#167220=CARTESIAN_POINT('Ctrl Pts',(-6.48752978291789,0.546576979715855,
-3.23660067292705));
#167221=CARTESIAN_POINT('Ctrl Pts',(-6.47248667262769,0.541139220244448,
-3.26657916856151));
#167222=CARTESIAN_POINT('Ctrl Pts',(-6.45724848592935,0.535714285974849,
-3.29642867213839));
#167223=CARTESIAN_POINT('Ctrl Pts',(-6.42397356473939,0.523868108816351,
-3.36160964736033));
#167224=CARTESIAN_POINT('Ctrl Pts',(-6.38965469195533,0.511960760953255,
-3.42639795188723));
#167225=CARTESIAN_POINT('Ctrl Pts',(-6.35430589758883,0.499999999782203,
-3.49074441377444));
#167226=CARTESIAN_POINT('Ctrl Pts',(-6.353378002,0.499686101,-3.492432958));
#167227=CARTESIAN_POINT('Ctrl Pts',(-6.40681269,0.51775868,-3.395225431));
#167228=CARTESIAN_POINT('Ctrl Pts',(-6.457248486,0.535714286,-3.296428672));
#167229=CARTESIAN_POINT('Ctrl Pts',(-6.48056094700001,0.544013736,-3.25076278));
#167230=CARTESIAN_POINT('Ctrl Pts',(-6.503225208,0.552339147,-3.204771738));
#167231=CARTESIAN_POINT('Ctrl Pts',(-6.414355829,0.499686101,-3.474714335));
#167232=CARTESIAN_POINT('Ctrl Pts',(-6.46751942,0.51775868,-3.376573839));
#167233=CARTESIAN_POINT('Ctrl Pts',(-6.517655703,0.535714286,-3.276852842));
#167234=CARTESIAN_POINT('Ctrl Pts',(-6.54082972400001,0.544013736,-3.230759748));
#167235=CARTESIAN_POINT('Ctrl Pts',(-6.563349515,0.552339147,-3.184343505));
#167236=CARTESIAN_POINT('Ctrl Pts',(-6.50237472702647,0.552026827186047,
-3.20649698391275));
#167237=CARTESIAN_POINT('Ctrl Pts',(-6.50704107826924,0.551172308290511,
-3.20884289203978));
#167238=CARTESIAN_POINT('Ctrl Pts',(-6.51170742690672,0.55032053497357,
-3.21118979521659));
#167239=CARTESIAN_POINT('Ctrl Pts',(-6.51637377175448,0.549471478080048,
-3.21353768657626));
#167240=CARTESIAN_POINT('Ctrl Pts',(-6.52070582963712,0.548683245806524,
-3.21571738002029));
#167241=CARTESIAN_POINT('Ctrl Pts',(-6.52503788541765,0.547897354495662,
-3.2178979257188));
#167242=CARTESIAN_POINT('Ctrl Pts',(-6.52936993621104,0.547113782448559,
-3.22007931301918));
#167243=CARTESIAN_POINT('Ctrl Pts',(-6.53370199137159,0.546330209611536,
-3.22226070251861));
#167244=CARTESIAN_POINT('Ctrl Pts',(-6.53803404263738,0.545548955845697,
-3.2244429341727));
#167245=CARTESIAN_POINT('Ctrl Pts',(-6.54236608770616,0.544769999912445,
-3.22662599655894));
#167246=CARTESIAN_POINT('Ctrl Pts',(-6.50154001000001,0.552337930000001,
-3.208189131));
#167247=CARTESIAN_POINT('Ctrl Pts',(-6.572043636,0.526068113,-3.065310352));
#167248=CARTESIAN_POINT('Ctrl Pts',(-6.636202377,0.49968693,-2.919472213));
#167249=CARTESIAN_POINT('Ctrl Pts',(-6.521936642,0.552337930000001,-3.268324166));
#167250=CARTESIAN_POINT('Ctrl Pts',(-6.593761804,0.526068113,-3.124997148));
#167251=CARTESIAN_POINT('Ctrl Pts',(-6.659221114,0.49968693,-2.978653146));
#167252=CARTESIAN_POINT('Origin',(0.185833727268683,0.410743087570367,0.0656550491000485));
#167253=CARTESIAN_POINT('Ctrl Pts',(-6.570827957299,0.552548454735263,-3.18565548897648));
#167254=CARTESIAN_POINT('Ctrl Pts',(-6.57152237414949,0.552287640367631,
-3.18422157048824));
#167255=CARTESIAN_POINT('Ctrl Pts',(-6.572216791,0.552026826,-3.182787652));
#167256=CARTESIAN_POINT('Ctrl Pts',(-6.64174783,0.525911829,-3.039211294));
#167257=CARTESIAN_POINT('Ctrl Pts',(-6.704942401,0.49968693,-2.892735418));
#167258=CARTESIAN_POINT('Ctrl Pts',(-6.50096408335731,0.552548454735263,
-3.20933823603486));
#167259=CARTESIAN_POINT('Ctrl Pts',(-6.50166367393037,0.552287640367631,
-3.2079195580993));
#167260=CARTESIAN_POINT('Ctrl Pts',(-6.50236326450344,0.552026826,-3.20650088016375));
#167261=CARTESIAN_POINT('Ctrl Pts',(-6.57241234148776,0.525911829,-3.06445053850729));
#167262=CARTESIAN_POINT('Ctrl Pts',(-6.63619109832366,0.49968693,-2.91947659990067));
#167263=CARTESIAN_POINT('',(-6.6063057566483,0.552026824384635,-3.17121545456552));
#167264=CARTESIAN_POINT('Ctrl Pts',(-6.4988999771904,0.550751630586317,
-3.2135412840469));
#167265=CARTESIAN_POINT('Ctrl Pts',(-6.500636741881,0.551389228293159,-3.2100193436641));
#167266=CARTESIAN_POINT('Ctrl Pts',(-6.50237350657161,0.552026826,-3.2064974032813));
#167267=CARTESIAN_POINT('Ctrl Pts',(-6.67704955408538,0.61615356,-2.85227634560151));
#167268=CARTESIAN_POINT('Ctrl Pts',(-6.81221327267021,0.681389364,-2.48117656408361));
#167269=CARTESIAN_POINT('Ctrl Pts',(-6.7068397085662,0.550751630586317,
-3.14320295556554));
#167270=CARTESIAN_POINT('Ctrl Pts',(-6.7085382532831,0.551389228293159,
-3.13956842828277));
#167271=CARTESIAN_POINT('Ctrl Pts',(-6.710236798,0.552026826,-3.135933901));
#167272=CARTESIAN_POINT('Ctrl Pts',(-6.88106885100001,0.61615356,-2.770389355));
#167273=CARTESIAN_POINT('Ctrl Pts',(-7.011181266,0.681389364000001,-2.388450661));
#167274=CARTESIAN_POINT('Ctrl Pts',(-6.81059626604927,0.680609082247605,
-2.48561436902554));
#167275=CARTESIAN_POINT('Ctrl Pts',(-6.82763962922413,0.67765275263127,
-2.49164451250911));
#167276=CARTESIAN_POINT('Ctrl Pts',(-6.84468815497496,0.674729896800113,
-2.49767662485867));
#167277=CARTESIAN_POINT('Ctrl Pts',(-6.86173573966136,0.671836782439133,
-2.50372552673111));
#167278=CARTESIAN_POINT('Ctrl Pts',(-6.87769488401706,0.669128385292337,
-2.50938822323339));
#167279=CARTESIAN_POINT('Ctrl Pts',(-6.89365472342022,0.666446714418226,
-2.51506181260851));
#167280=CARTESIAN_POINT('Ctrl Pts',(-6.90961513751775,0.663790956077136,
-2.52074582218071));
#167281=CARTESIAN_POINT('Ctrl Pts',(-6.92557572297528,0.661135169222328,
-2.52642989277963));
#167282=CARTESIAN_POINT('Ctrl Pts',(-6.94153692556273,0.658505288546222,
-2.53212439906121));
#167283=CARTESIAN_POINT('Ctrl Pts',(-6.95749863316843,0.655900535537742,
-2.53782889725405));
#167284=CARTESIAN_POINT('Ctrl Pts',(-6.808984789,0.681369595,-2.49002533));
#167285=CARTESIAN_POINT('Ctrl Pts',(-6.811952522,0.679970133,-2.48191005));
#167286=CARTESIAN_POINT('Ctrl Pts',(-6.814900903,0.678571429,-2.47378772));
#167287=CARTESIAN_POINT('Ctrl Pts',(-6.947044364,0.615882895,-2.109753011));
#167288=CARTESIAN_POINT('Ctrl Pts',(-7.039654886,0.552026826,-1.733712515));
#167289=CARTESIAN_POINT('Ctrl Pts',(-6.901451545,0.681369595,-2.689112472));
#167290=CARTESIAN_POINT('Ctrl Pts',(-6.90465656,0.679970133,-2.680886986));
#167291=CARTESIAN_POINT('Ctrl Pts',(-6.907841959,0.678571429,-2.672653884));
#167292=CARTESIAN_POINT('Ctrl Pts',(-7.050608345,0.615882895,-2.3036545));
#167293=CARTESIAN_POINT('Ctrl Pts',(-7.153252451,0.552026826,-1.92154591));
#167294=CARTESIAN_POINT('',(-7.0587393865776,0.552026824384634,-1.76526872068638));
#167295=CARTESIAN_POINT('Ctrl Pts',(-6.990934579,0.499686101,-2.10974039));
#167296=CARTESIAN_POINT('Ctrl Pts',(-7.023213887,0.51775868,-2.002778163));
#167297=CARTESIAN_POINT('Ctrl Pts',(-7.052205779,0.535714286,-1.894878478));
#167298=CARTESIAN_POINT('Ctrl Pts',(-7.065355051,0.54385805,-1.845940579));
#167299=CARTESIAN_POINT('Ctrl Pts',(-7.077823892,0.552026826,-1.796824907));
#167300=CARTESIAN_POINT('Ctrl Pts',(-6.955609405,0.499686101,-2.04499335));
#167301=CARTESIAN_POINT('Ctrl Pts',(-6.986898075,0.51775868,-1.938571603));
#167302=CARTESIAN_POINT('Ctrl Pts',(-7.014916327,0.535714286,-1.831242452));
#167303=CARTESIAN_POINT('Ctrl Pts',(-7.02762400500001,0.54385805,-1.782563319));
#167304=CARTESIAN_POINT('Ctrl Pts',(-7.039654886,0.552026826,-1.733712515));
#167305=CARTESIAN_POINT('Ctrl Pts',(-7.03965488562795,0.552026825462645,
-1.7337125189069));
#167306=CARTESIAN_POINT('Ctrl Pts',(-7.02688357095935,0.543355306279276,
-1.7855698223019));
#167307=CARTESIAN_POINT('Ctrl Pts',(-7.01355081405543,0.534726109137552,
-1.83724106183393));
#167308=CARTESIAN_POINT('Ctrl Pts',(-6.98571521390196,0.517399144305422,
-1.94039718220693));
#167309=CARTESIAN_POINT('Ctrl Pts',(-6.97121732082761,0.508708906297517,
-1.99185507680409));
#167310=CARTESIAN_POINT('Ctrl Pts',(-6.95615261946262,0.499999999579507,
-2.04314481407824));
#167311=CARTESIAN_POINT('Ctrl Pts',(-6.955609405,0.499686101,-2.04499335));
#167312=CARTESIAN_POINT('Ctrl Pts',(-6.986898075,0.51775868,-1.938571603));
#167313=CARTESIAN_POINT('Ctrl Pts',(-7.014916327,0.535714286,-1.831242452));
#167314=CARTESIAN_POINT('Ctrl Pts',(-7.02786694,0.544013736,-1.781632713));
#167315=CARTESIAN_POINT('Ctrl Pts',(-7.040114608,0.552339147,-1.73184477));
#167316=CARTESIAN_POINT('Ctrl Pts',(-7.011352625,0.499686101,-2.014580548));
#167317=CARTESIAN_POINT('Ctrl Pts',(-7.042175974,0.51775868,-1.907305922));
#167318=CARTESIAN_POINT('Ctrl Pts',(-7.069703033,0.535714286,-1.799138528));
#167319=CARTESIAN_POINT('Ctrl Pts',(-7.082426605,0.544013736,-1.749141335));
#167320=CARTESIAN_POINT('Ctrl Pts',(-7.09444177600001,0.552339147,-1.698969189));
#167321=CARTESIAN_POINT('Ctrl Pts',(-7.03965488779841,0.552026827256097,
-1.73371250846653));
#167322=CARTESIAN_POINT('Ctrl Pts',(-7.04471644281915,0.551172308291889,
-1.73500044361819));
#167323=CARTESIAN_POINT('Ctrl Pts',(-7.04977820962006,0.550320534980668,
-1.73628935044783));
#167324=CARTESIAN_POINT('Ctrl Pts',(-7.05484018515242,0.549471478091212,
-1.73757922316128));
#167325=CARTESIAN_POINT('Ctrl Pts',(-7.05953953160199,0.548683245818368,
-1.73877669215685));
#167326=CARTESIAN_POINT('Ctrl Pts',(-7.06423905921018,0.547897354506795,
-1.73997499392441));
#167327=CARTESIAN_POINT('Ctrl Pts',(-7.0689387628729,0.547113782458042,
-1.74117411869096));
#167328=CARTESIAN_POINT('Ctrl Pts',(-7.07363847126248,0.546330209621188,
-1.74237324466356));
#167329=CARTESIAN_POINT('Ctrl Pts',(-7.0783383568923,0.545548955854658,
-1.74357319394025));
#167330=CARTESIAN_POINT('Ctrl Pts',(-7.08303841523824,0.544770000053604,
-1.74477395507826));
#167331=CARTESIAN_POINT('Ctrl Pts',(-7.03920344700001,0.55233793,-1.735544534));
#167332=CARTESIAN_POINT('Ctrl Pts',(-7.077344024,0.526068113,-1.580849986));
#167333=CARTESIAN_POINT('Ctrl Pts',(-7.108651881,0.49968693,-1.424629229));
#167334=CARTESIAN_POINT('Ctrl Pts',(-7.072050472,0.55233793,-1.789888972));
#167335=CARTESIAN_POINT('Ctrl Pts',(-7.11138533,0.526068113,-1.634472573));
#167336=CARTESIAN_POINT('Ctrl Pts',(-7.143854603,0.49968693,-1.477478196));
#167337=CARTESIAN_POINT('Origin',(0.195602985683564,0.410743067885095,0.0241713514715394));
#167338=CARTESIAN_POINT('Ctrl Pts',(-7.10202741463771,0.552548454735263,
-1.69864285574175));
#167339=CARTESIAN_POINT('Ctrl Pts',(-7.10239734631885,0.552287640367631,
-1.69709318237088));
#167340=CARTESIAN_POINT('Ctrl Pts',(-7.102767278,0.552026826,-1.695543509));
#167341=CARTESIAN_POINT('Ctrl Pts',(-7.139808047,0.525911829,-1.540376768));
#167342=CARTESIAN_POINT('Ctrl Pts',(-7.17003718,0.49968693,-1.383740452));
#167343=CARTESIAN_POINT('Ctrl Pts',(-7.03888800934273,0.552548454735263,
-1.73679058026029));
#167344=CARTESIAN_POINT('Ctrl Pts',(-7.03926627005464,0.552287640367631,
-1.73525467894045));
#167345=CARTESIAN_POINT('Ctrl Pts',(-7.03964453076656,0.552026826,-1.73371877762062));
#167346=CARTESIAN_POINT('Ctrl Pts',(-7.07751927457942,0.525911829,-1.57993101384067));
#167347=CARTESIAN_POINT('Ctrl Pts',(-7.10864180914119,0.49968693,-1.42463593786997));
#167348=CARTESIAN_POINT('',(-7.13357158119885,0.552026824384635,-1.67691374278907));
#167349=CARTESIAN_POINT('Ctrl Pts',(-7.03777679268802,0.550751630586317,
-1.74133842106059));
#167350=CARTESIAN_POINT('Ctrl Pts',(-7.03871583934401,0.551389228293159,
-1.73752546803029));
#167351=CARTESIAN_POINT('Ctrl Pts',(-7.039654886,0.552026826,-1.733712515));
#167352=CARTESIAN_POINT('Ctrl Pts',(-7.134100011,0.61615356,-1.350222703));
#167353=CARTESIAN_POINT('Ctrl Pts',(-7.186328152,0.681389364000001,-0.958742768));
#167354=CARTESIAN_POINT('Ctrl Pts',(-7.22573324546068,0.550751630586317,
-1.62794433293448));
#167355=CARTESIAN_POINT('Ctrl Pts',(-7.22661076323034,0.551389228293159,
-1.62402964196724));
#167356=CARTESIAN_POINT('Ctrl Pts',(-7.22748828100001,0.552026826,-1.620114951));
#167357=CARTESIAN_POINT('Ctrl Pts',(-7.315745105,0.61615356,-1.226392791));
#167358=CARTESIAN_POINT('Ctrl Pts',(-7.360710034,0.681389364000001,-0.825413289));
#167359=CARTESIAN_POINT('Ctrl Pts',(-7.18570192502824,0.680609082247603,
-0.963425208969651));
#167360=CARTESIAN_POINT('Ctrl Pts',(-7.20364312653453,0.677652752724234,
-0.965650551686538));
#167361=CARTESIAN_POINT('Ctrl Pts',(-7.22158979302487,0.674729896867849,
-0.967876707642936));
#167362=CARTESIAN_POINT('Ctrl Pts',(-7.23953914972131,0.671836782501652,
-0.970119462776265));
#167363=CARTESIAN_POINT('Ctrl Pts',(-7.25634249050251,0.669128385346457,
-0.972219024305487));
#167364=CARTESIAN_POINT('Ctrl Pts',(-7.27314885172766,0.666446714465226,
-0.974329074620163));
#167365=CARTESIAN_POINT('Ctrl Pts',(-7.28995801424599,0.663790956117991,
-0.976449177968538));
#167366=CARTESIAN_POINT('Ctrl Pts',(-7.30676735723696,0.661135169257037,
-0.978569304079536));
#167367=CARTESIAN_POINT('Ctrl Pts',(-7.32357954629348,0.658505288575763,
-0.980699489225385));
#167368=CARTESIAN_POINT('Ctrl Pts',(-7.34039437668371,0.655900535573722,
-0.98283932438691));
#167369=CARTESIAN_POINT('Ctrl Pts',(-7.18507635,0.681369595,-0.968079464000001));
#167370=CARTESIAN_POINT('Ctrl Pts',(-7.186230154,0.679970133,-0.959515940000001));
#167371=CARTESIAN_POINT('Ctrl Pts',(-7.187363542,0.678571429,-0.95094969));
#167372=CARTESIAN_POINT('Ctrl Pts',(-7.238160861,0.615882895,-0.567018973000001));
#167373=CARTESIAN_POINT('Ctrl Pts',(-7.247768609,0.552026826,-0.17986157));
#167374=CARTESIAN_POINT('Ctrl Pts',(-7.318179135,0.681369595,-1.14263444));
#167375=CARTESIAN_POINT('Ctrl Pts',(-7.319540982,0.679970133,-1.133912278));
#167376=CARTESIAN_POINT('Ctrl Pts',(-7.320882034,0.678571429,-1.125186894));
#167377=CARTESIAN_POINT('Ctrl Pts',(-7.38098666200001,0.615882895,-0.734123958000001));
#167378=CARTESIAN_POINT('Ctrl Pts',(-7.399088954,0.552026826,-0.338883407));
#167379=CARTESIAN_POINT('',(-7.27319057621652,0.552026824384633,-0.206577405480668));
#167380=CARTESIAN_POINT('Ctrl Pts',(-7.281022233,0.499686101,-0.557571548));
#167381=CARTESIAN_POINT('Ctrl Pts',(-7.289553152,0.51775868,-0.446170941));
#167382=CARTESIAN_POINT('Ctrl Pts',(-7.294671987,0.535714286,-0.334561492));
#167383=CARTESIAN_POINT('Ctrl Pts',(-7.296993635,0.54385805,-0.283941029));
#167384=CARTESIAN_POINT('Ctrl Pts',(-7.298612544,0.552026826,-0.233293221));
#167385=CARTESIAN_POINT('Ctrl Pts',(-7.232604243,0.499686101,-0.501932126));
#167386=CARTESIAN_POINT('Ctrl Pts',(-7.240283871,0.51775868,-0.391272321));
#167387=CARTESIAN_POINT('Ctrl Pts',(-7.244574478,0.535714286,-0.28042937));
#167388=CARTESIAN_POINT('Ctrl Pts',(-7.246520483,0.54385805,-0.230156553));
#167389=CARTESIAN_POINT('Ctrl Pts',(-7.247768609,0.552026826,-0.17986157));
#167390=CARTESIAN_POINT('Ctrl Pts',(-7.24776860911075,0.552026825539334,
-0.179861574560902));
#167391=CARTESIAN_POINT('Ctrl Pts',(-7.24693591438939,0.546576979279491,
-0.213416164634367));
#167392=CARTESIAN_POINT('Ctrl Pts',(-7.24587080090455,0.541139220024475,
-0.246940346863208));
#167393=CARTESIAN_POINT('Ctrl Pts',(-7.24457447812535,0.535714285988153,
-0.280429369954506));
#167394=CARTESIAN_POINT('Ctrl Pts',(-7.24174375852935,0.52386810879308,
-0.35355779757423));
#167395=CARTESIAN_POINT('Ctrl Pts',(-7.23780069555822,0.511960760818452,
-0.426768191841702));
#167396=CARTESIAN_POINT('Ctrl Pts',(-7.23273737687419,0.499999999575121,
-0.500010032745376));
#167397=CARTESIAN_POINT('Ctrl Pts',(-7.232604243,0.499686101,-0.501932126));
#167398=CARTESIAN_POINT('Ctrl Pts',(-7.240283871,0.51775868,-0.391272321));
#167399=CARTESIAN_POINT('Ctrl Pts',(-7.244574478,0.535714286,-0.28042937));
#167400=CARTESIAN_POINT('Ctrl Pts',(-7.246557685,0.544013736,-0.22919548));
#167401=CARTESIAN_POINT('Ctrl Pts',(-7.247816073,0.552339147,-0.177938666));
#167402=CARTESIAN_POINT('Ctrl Pts',(-7.28050636400001,0.499686101,-0.460247214));
#167403=CARTESIAN_POINT('Ctrl Pts',(-7.287548207,0.51775868,-0.348854501));
#167404=CARTESIAN_POINT('Ctrl Pts',(-7.291178906,0.535714286,-0.237298496));
#167405=CARTESIAN_POINT('Ctrl Pts',(-7.292857089,0.544013736,-0.185735018));
#167406=CARTESIAN_POINT('Ctrl Pts',(-7.293805824,0.552339147,-0.134152962));
#167407=CARTESIAN_POINT('Ctrl Pts',(-7.24776860938908,0.552026827360936,
-0.179861563345339));
#167408=CARTESIAN_POINT('Ctrl Pts',(-7.25298869621631,0.551172308315565,
-0.180031302772311));
#167409=CARTESIAN_POINT('Ctrl Pts',(-7.25820919857855,0.550320534990502,
-0.180201945437676));
#167410=CARTESIAN_POINT('Ctrl Pts',(-7.26343011242881,0.549471478090142,
-0.180373486544556));
#167411=CARTESIAN_POINT('Ctrl Pts',(-7.26827701119779,0.548683245806835,
-0.180532738814102));
#167412=CARTESIAN_POINT('Ctrl Pts',(-7.27312426591151,0.547897354487421,
-0.180692765451291));
#167413=CARTESIAN_POINT('Ctrl Pts',(-7.27797186947297,0.547113782434519,
-0.180853558004141));
#167414=CARTESIAN_POINT('Ctrl Pts',(-7.28281947793267,0.546330209589859,
-0.181014350719461));
#167415=CARTESIAN_POINT('Ctrl Pts',(-7.28766743646369,0.545548955819146,
-0.18117590939348));
#167416=CARTESIAN_POINT('Ctrl Pts',(-7.29251573835091,0.544769999940509,
-0.181338224129734));
#167417=CARTESIAN_POINT('Ctrl Pts',(-7.247721555,0.55233793,-0.181747804));
#167418=CARTESIAN_POINT('Ctrl Pts',(-7.251715671,0.526068113,-0.022470832));
#167419=CARTESIAN_POINT('Ctrl Pts',(-7.248708723,0.49968693,0.136827835));
#167420=CARTESIAN_POINT('Ctrl Pts',(-7.291483082,0.55233793,-0.22776056));
#167421=CARTESIAN_POINT('Ctrl Pts',(-7.296488381,0.526068113,-0.067521878));
#167422=CARTESIAN_POINT('Ctrl Pts',(-7.294449391,0.49968693,0.092781992));
#167423=CARTESIAN_POINT('Origin',(0.196226715612283,0.410743175436658,-0.0184426066818074));
#167424=CARTESIAN_POINT('Ctrl Pts',(-7.30114396216113,0.552548454735263,
-0.132203570485142));
#167425=CARTESIAN_POINT('Ctrl Pts',(-7.30117211108057,0.552287640367631,
-0.130610603242571));
#167426=CARTESIAN_POINT('Ctrl Pts',(-7.30120026,0.552026826,-0.129017636));
#167427=CARTESIAN_POINT('Ctrl Pts',(-7.304018774,0.525911829,0.030484063));
#167428=CARTESIAN_POINT('Ctrl Pts',(-7.299868989,0.49968693,0.18995668));
#167429=CARTESIAN_POINT('Ctrl Pts',(-7.24768135452721,0.552548454735263,
-0.183032527619515));
#167430=CARTESIAN_POINT('Ctrl Pts',(-7.24772059833278,0.552287640367631,
-0.181451219949218));
#167431=CARTESIAN_POINT('Ctrl Pts',(-7.24775984213834,0.552026826,-0.179869912278921));
#167432=CARTESIAN_POINT('Ctrl Pts',(-7.25168927238334,0.525911829,-0.0215356707994777));
#167433=CARTESIAN_POINT('Ctrl Pts',(-7.24870032881853,0.49968693,0.13681911782159));
#167434=CARTESIAN_POINT('',(-7.32727952735701,0.552026824384635,-0.104201408054877));
#167435=CARTESIAN_POINT('Ctrl Pts',(-7.24757376884405,0.550751630586317,
-0.187712921172618));
#167436=CARTESIAN_POINT('Ctrl Pts',(-7.24767118892203,0.551389228293159,
-0.183787245586309));
#167437=CARTESIAN_POINT('Ctrl Pts',(-7.247768609,0.552026826,-0.17986157));
#167438=CARTESIAN_POINT('Ctrl Pts',(-7.257566686,0.61615356,0.214965374));
#167439=CARTESIAN_POINT('Ctrl Pts',(-7.224417148,0.681389364000001,0.608520231));
#167440=CARTESIAN_POINT('Ctrl Pts',(-7.40675952790616,0.550751630586317,
-0.0365648420981692));
#167441=CARTESIAN_POINT('Ctrl Pts',(-7.40677498695308,0.551389228293159,
-0.0325530340490846));
#167442=CARTESIAN_POINT('Ctrl Pts',(-7.406790446,0.552026826,-0.028541226));
#167443=CARTESIAN_POINT('Ctrl Pts',(-7.408345248,0.61615356,0.374948537));
#167444=CARTESIAN_POINT('Ctrl Pts',(-7.366060182,0.681389364000001,0.776219491));
#167445=CARTESIAN_POINT('Ctrl Pts',(-7.22481214824486,0.680609082247605,
0.603812642854019));
#167446=CARTESIAN_POINT('Ctrl Pts',(-7.24281227785518,0.677652752599059,
0.605496154954779));
#167447=CARTESIAN_POINT('Ctrl Pts',(-7.26081791900121,0.674729896792423,
0.607180048451818));
#167448=CARTESIAN_POINT('Ctrl Pts',(-7.27882975580833,0.671836782432773,
0.608848308897028));
#167449=CARTESIAN_POINT('Ctrl Pts',(-7.29569158745369,0.669128385294513,
0.610410055601098));
#167450=CARTESIAN_POINT('Ctrl Pts',(-7.31255862370623,0.666446714429166,
0.611962208038781));
#167451=CARTESIAN_POINT('Ctrl Pts',(-7.32943055686501,0.663790956096888,
0.613505144663944));
#167452=CARTESIAN_POINT('Ctrl Pts',(-7.34630267117038,0.661135169250888,
0.615048097854947));
#167453=CARTESIAN_POINT('Ctrl Pts',(-7.36317972739769,0.658505288583637,
0.616581838997317));
#167454=CARTESIAN_POINT('Ctrl Pts',(-7.38006143764124,0.655900535683362,
0.618106723046989));
#167455=CARTESIAN_POINT('Ctrl Pts',(-7.225201726,0.681369595,0.599132722));
#167456=CARTESIAN_POINT('Ctrl Pts',(-7.22448765,0.679970133000001,0.607744069));
#167457=CARTESIAN_POINT('Ctrl Pts',(-7.22375305,0.678571429,0.616353689));
#167458=CARTESIAN_POINT('Ctrl Pts',(-7.190829,0.615882895,1.002228242));
#167459=CARTESIAN_POINT('Ctrl Pts',(-7.116984728,0.552026826,1.382399502));
#167460=CARTESIAN_POINT('Ctrl Pts',(-7.392716802,0.681369595,0.457271909));
#167461=CARTESIAN_POINT('Ctrl Pts',(-7.39217180299999,0.679970133000001,
0.466082908));
#167462=CARTESIAN_POINT('Ctrl Pts',(-7.391605803,0.678571429,0.474892584));
#167463=CARTESIAN_POINT('Ctrl Pts',(-7.366238246,0.615882895,0.869733404));
#167464=CARTESIAN_POINT('Ctrl Pts',(-7.298952281,0.552026826,1.259624909));
#167465=CARTESIAN_POINT('',(-7.1475554583687,0.552026824384634,1.36177323919174));
#167466=CARTESIAN_POINT('Ctrl Pts',(-7.230657381,0.499686101,1.02066872));
#167467=CARTESIAN_POINT('Ctrl Pts',(-7.215041014,0.51775868,1.131298737));
#167468=CARTESIAN_POINT('Ctrl Pts',(-7.196047441,0.535714286,1.241399218));
#167469=CARTESIAN_POINT('Ctrl Pts',(-7.187432907,0.54385805,1.291335288));
#167470=CARTESIAN_POINT('Ctrl Pts',(-7.178126185,0.552026826,1.341146996));
#167471=CARTESIAN_POINT('Ctrl Pts',(-7.171410545,0.499686101,1.064598886));
#167472=CARTESIAN_POINT('Ctrl Pts',(-7.155122041,0.51775868,1.174322419));
#167473=CARTESIAN_POINT('Ctrl Pts',(-7.135484378,0.535714286,1.283496277));
#167474=CARTESIAN_POINT('Ctrl Pts',(-7.126577716,0.54385805,1.333012078));
#167475=CARTESIAN_POINT('Ctrl Pts',(-7.116984728,0.552026826,1.382399502));
#167476=CARTESIAN_POINT('Ctrl Pts',(-7.11698472856132,0.552026826,1.38239950162127));
#167477=CARTESIAN_POINT('Ctrl Pts',(-7.1271681177084,0.54335530340197,1.32997253191968));
#167478=CARTESIAN_POINT('Ctrl Pts',(-7.13676382120383,0.534726110048207,
1.27747872812076));
#167479=CARTESIAN_POINT('Ctrl Pts',(-7.15481559744862,0.517398614706748,
1.17216567942275));
#167480=CARTESIAN_POINT('Ctrl Pts',(-7.16326323260566,0.508709450442465,
1.11938277393001));
#167481=CARTESIAN_POINT('Ctrl Pts',(-7.17112737305294,0.499999999526768,
1.06650466127345));
#167482=CARTESIAN_POINT('Ctrl Pts',(-7.171410545,0.499686101,1.064598886));
#167483=CARTESIAN_POINT('Ctrl Pts',(-7.155122041,0.51775868,1.174322419));
#167484=CARTESIAN_POINT('Ctrl Pts',(-7.135484378,0.535714286,1.283496277));
#167485=CARTESIAN_POINT('Ctrl Pts',(-7.126407446,0.544013736,1.333958678));
#167486=CARTESIAN_POINT('Ctrl Pts',(-7.11661771399999,0.552339147,1.384287653));
#167487=CARTESIAN_POINT('Ctrl Pts',(-7.209231717,0.499686101,1.115606768));
#167488=CARTESIAN_POINT('Ctrl Pts',(-7.192162786,0.51775868,1.22590897));
#167489=CARTESIAN_POINT('Ctrl Pts',(-7.171727357,0.535714286,1.33563735));
#167490=CARTESIAN_POINT('Ctrl Pts',(-7.162281682,0.544013736,1.386356063));
#167491=CARTESIAN_POINT('Ctrl Pts',(-7.152119618,0.552339147,1.436936109));
#167492=CARTESIAN_POINT('Ctrl Pts',(-7.11698472626396,0.552026827255857,
1.38239950799491));
#167493=CARTESIAN_POINT('Ctrl Pts',(-7.1221192597115,0.551172308251233,
1.38335590228193));
#167494=CARTESIAN_POINT('Ctrl Pts',(-7.12725439282643,0.550320534923491,
1.38431150292089));
#167495=CARTESIAN_POINT('Ctrl Pts',(-7.13239012095014,0.549471478020002,
1.38526631456333));
#167496=CARTESIAN_POINT('Ctrl Pts',(-7.13715793640245,0.548683245752477,
1.38615272552458));
#167497=CARTESIAN_POINT('Ctrl Pts',(-7.14192626594669,0.547897354448274,
1.3870384567244));
#167498=CARTESIAN_POINT('Ctrl Pts',(-7.146695100838,0.547113782408566,1.38792351489902));
#167499=CARTESIAN_POINT('Ctrl Pts',(-7.15146394053894,0.546330209578583,
1.38880857396627));
#167500=CARTESIAN_POINT('Ctrl Pts',(-7.15623328679112,0.545548955820519,
1.38969296022934));
#167501=CARTESIAN_POINT('Ctrl Pts',(-7.16100313085534,0.544769999895332,
1.39057668139717));
#167502=CARTESIAN_POINT('Ctrl Pts',(-7.117344258,0.55233793,1.380547252));
#167503=CARTESIAN_POINT('Ctrl Pts',(-7.087005153,0.526068113,1.536959034));
#167504=CARTESIAN_POINT('Ctrl Pts',(-7.049824001,0.49968693,1.691886981));
#167505=CARTESIAN_POINT('Ctrl Pts',(-7.169974048,0.55233793,1.345017684));
#167506=CARTESIAN_POINT('Ctrl Pts',(-7.140415745,0.526068113,1.502586065));
#167507=CARTESIAN_POINT('Ctrl Pts',(-7.103963832,0.49968693,1.658703797));
#167508=CARTESIAN_POINT('Origin',(0.187673976996539,0.410743035001748,-0.0601943055948376));
#167509=CARTESIAN_POINT('Ctrl Pts',(-7.15886713411727,0.552548454735263,
1.44041740752365));
#167510=CARTESIAN_POINT('Ctrl Pts',(-7.15855218405863,0.552287640367631,
1.44197918326182));
#167511=CARTESIAN_POINT('Ctrl Pts',(-7.158237234,0.552026826,1.443540959));
#167512=CARTESIAN_POINT('Ctrl Pts',(-7.126701702,0.525911829,1.599919494));
#167513=CARTESIAN_POINT('Ctrl Pts',(-7.088367037,0.49968693,1.754771648));
#167514=CARTESIAN_POINT('Ctrl Pts',(-7.11758117562899,0.552548454735263,
1.37928392241786));
#167515=CARTESIAN_POINT('Ctrl Pts',(-7.11727956752418,0.552287640367631,
1.38083669626055));
#167516=CARTESIAN_POINT('Ctrl Pts',(-7.11697795941937,0.552026826,1.38238947010324));
#167517=CARTESIAN_POINT('Ctrl Pts',(-7.08677833957566,0.525911829,1.53786665723719));
#167518=CARTESIAN_POINT('Ctrl Pts',(-7.04981767698064,0.49968693,1.69187666308286));
#167519=CARTESIAN_POINT('',(-7.17837202652185,0.552026824384635,1.47338326864946));
#167520=CARTESIAN_POINT('Ctrl Pts',(-7.11848153267414,0.550751630586317,
1.37468876324479));
#167521=CARTESIAN_POINT('Ctrl Pts',(-7.11773277148763,0.551389228293159,
1.37854360076192));
#167522=CARTESIAN_POINT('Ctrl Pts',(-7.11698401030112,0.552026826,1.38239843827904));
#167523=CARTESIAN_POINT('Ctrl Pts',(-7.04167694924802,0.61615356,1.77010080518193));
#167524=CARTESIAN_POINT('Ctrl Pts',(-6.9246998300991,0.681389364000001,
2.14732836561089));
#167525=CARTESIAN_POINT('Ctrl Pts',(-7.24145396603117,0.550751630586317,
1.55652438013174));
#167526=CARTESIAN_POINT('Ctrl Pts',(-7.24060664351558,0.551389228293159,
1.56044571756587));
#167527=CARTESIAN_POINT('Ctrl Pts',(-7.239759321,0.552026826,1.564367055));
#167528=CARTESIAN_POINT('Ctrl Pts',(-7.15453940100001,0.61615356,1.958757687));
#167529=CARTESIAN_POINT('Ctrl Pts',(-7.026981543,0.681389364000001,2.341557111));
#167530=CARTESIAN_POINT('Ctrl Pts',(-6.92609818588287,0.680609082082805,
2.14281688694626));
#167531=CARTESIAN_POINT('Ctrl Pts',(-6.94331557651135,0.67765275266803,
2.14833053518668));
#167532=CARTESIAN_POINT('Ctrl Pts',(-6.96053826846024,0.674729896853169,
2.15384574070214));
#167533=CARTESIAN_POINT('Ctrl Pts',(-6.97777037186197,0.671836782485758,
2.15934701054552));
#167534=CARTESIAN_POINT('Ctrl Pts',(-6.99390225394025,0.669128385331562,
2.16449703978601));
#167535=CARTESIAN_POINT('Ctrl Pts',(-7.01004128142473,0.666446714452519,
2.16963881791848));
#167536=CARTESIAN_POINT('Ctrl Pts',(-7.02618707245249,0.663790956108138,
2.17477264840016));
#167537=CARTESIAN_POINT('Ctrl Pts',(-7.04233303683055,0.661135169250039,
2.17990653400152));
#167538=CARTESIAN_POINT('Ctrl Pts',(-7.05848580790602,0.658505288572285,
2.18503248530502));
#167539=CARTESIAN_POINT('Ctrl Pts',(-7.07464502826342,0.655900535710891,
2.19015078679768));
#167540=CARTESIAN_POINT('Ctrl Pts',(-6.9274847,0.681369595,2.138330128));
#167541=CARTESIAN_POINT('Ctrl Pts',(-6.924936134,0.679970133,2.146586641));
#167542=CARTESIAN_POINT('Ctrl Pts',(-6.922367894,0.678571429,2.154837056));
#167543=CARTESIAN_POINT('Ctrl Pts',(-6.807261968,0.615882895,2.524612378));
#167544=CARTESIAN_POINT('Ctrl Pts',(-6.65341854999999,0.552026826,2.88002111));
#167545=CARTESIAN_POINT('Ctrl Pts',(-7.12157924800001,0.681369595,2.035796731));
#167546=CARTESIAN_POINT('Ctrl Pts',(-7.119152886,0.679970133,2.044284575));
#167547=CARTESIAN_POINT('Ctrl Pts',(-7.116706299,0.678571429,2.052766612));
#167548=CARTESIAN_POINT('Ctrl Pts',(-7.007052717,0.615882895,2.432922999));
#167549=CARTESIAN_POINT('Ctrl Pts',(-6.857524711,0.552026826,2.799234563));
#167550=CARTESIAN_POINT('',(-6.68770859093351,0.55202682438463,2.86644888132274));
#167551=CARTESIAN_POINT('Ctrl Pts',(-6.842195025,0.499686101,2.551183652));
#167552=CARTESIAN_POINT('Ctrl Pts',(-6.803161577,0.51775868,2.655870144));
#167553=CARTESIAN_POINT('Ctrl Pts',(-6.760943714,0.535714286,2.759313481));
#167554=CARTESIAN_POINT('Ctrl Pts',(-6.741795804,0.54385805,2.806230203));
#167555=CARTESIAN_POINT('Ctrl Pts',(-6.721998624,0.552026826000001,2.852876671));
#167556=CARTESIAN_POINT('Ctrl Pts',(-6.774889661,0.499686101,2.581350438));
#167557=CARTESIAN_POINT('Ctrl Pts',(-6.735394657,0.51775868,2.685007149));
#167558=CARTESIAN_POINT('Ctrl Pts',(-6.692746959,0.535714286,2.787407065));
#167559=CARTESIAN_POINT('Ctrl Pts',(-6.673404096,0.54385805,2.833850545));
#167560=CARTESIAN_POINT('Ctrl Pts',(-6.65341855,0.552026826000001,2.88002111));
#167561=CARTESIAN_POINT('Ctrl Pts',(-6.65341855027456,0.552026826354219,
2.88002111045043));
#167562=CARTESIAN_POINT('Ctrl Pts',(-6.66675202404212,0.546576979816255,
2.84921814757175));
#167563=CARTESIAN_POINT('Ctrl Pts',(-6.67986179275827,0.541139220289782,
2.81834519245283));
#167564=CARTESIAN_POINT('Ctrl Pts',(-6.69274695885586,0.535714286060686,
2.78740706534609));
#167565=CARTESIAN_POINT('Ctrl Pts',(-6.72088369664735,0.523868109091399,
2.71984891517481));
#167566=CARTESIAN_POINT('Ctrl Pts',(-6.74804531683569,0.51196076095622,
2.65174931160051));
#167567=CARTESIAN_POINT('Ctrl Pts',(-6.77420342353812,0.499999999786669,
2.58315078520083));
#167568=CARTESIAN_POINT('Ctrl Pts',(-6.774889661,0.499686101,2.581350438));
#167569=CARTESIAN_POINT('Ctrl Pts',(-6.735394657,0.51775868,2.685007149));
#167570=CARTESIAN_POINT('Ctrl Pts',(-6.692746959,0.535714286,2.787407065));
#167571=CARTESIAN_POINT('Ctrl Pts',(-6.673034316,0.544013736,2.834738411));
#167572=CARTESIAN_POINT('Ctrl Pts',(-6.652654221,0.552339147,2.88178622));
#167573=CARTESIAN_POINT('Ctrl Pts',(-6.800861408,0.499686101,2.639296217));
#167574=CARTESIAN_POINT('Ctrl Pts',(-6.760479825,0.51775868,2.743350299));
#167575=CARTESIAN_POINT('Ctrl Pts',(-6.716933807,0.535714286,2.846120278));
#167576=CARTESIAN_POINT('Ctrl Pts',(-6.696805943,0.544013736,2.893622674));
#167577=CARTESIAN_POINT('Ctrl Pts',(-6.676008248,0.552339147,2.940835644));
#167578=CARTESIAN_POINT('Ctrl Pts',(-6.65341854774275,0.552026827389055,
2.8800211162994));
#167579=CARTESIAN_POINT('Ctrl Pts',(-6.65822744166486,0.551172308368387,
2.88205892227521));
#167580=CARTESIAN_POINT('Ctrl Pts',(-6.66303709220779,0.550320535046825,
2.88409608323122));
#167581=CARTESIAN_POINT('Ctrl Pts',(-6.66784749345554,0.549471478151479,
2.88613260155777));
#167582=CARTESIAN_POINT('Ctrl Pts',(-6.67231328794614,0.548683245858544,
2.88802322810935));
#167583=CARTESIAN_POINT('Ctrl Pts',(-6.67677973063417,0.547897354530828,
2.8899133013166));
#167584=CARTESIAN_POINT('Ctrl Pts',(-6.68124681152564,0.547113782469392,
2.89180282587923));
#167585=CARTESIAN_POINT('Ctrl Pts',(-6.68571389693085,0.5463302096162,2.89369235235111));
#167586=CARTESIAN_POINT('Ctrl Pts',(-6.69018162166811,0.545548955836741,
2.89558133065308));
#167587=CARTESIAN_POINT('Ctrl Pts',(-6.6946499753884,0.54476999999312,2.89746976725727));
#167588=CARTESIAN_POINT('Ctrl Pts',(-6.654167854,0.55233793,2.878289453));
#167589=CARTESIAN_POINT('Ctrl Pts',(-6.59091415000001,0.526068113,3.024522403));
#167590=CARTESIAN_POINT('Ctrl Pts',(-6.521297344,0.49968693,3.167835372));
#167591=CARTESIAN_POINT('Ctrl Pts',(-6.71320499500001,0.55233793,2.854904395));
#167592=CARTESIAN_POINT('Ctrl Pts',(-6.650465205,0.526068113,3.002434754));
#167593=CARTESIAN_POINT('Ctrl Pts',(-6.58130482,0.49968693,3.147066456));
#167594=CARTESIAN_POINT('Origin',(0.17034727884052,0.410743050246431,-0.0991318348672909));
#167595=CARTESIAN_POINT('Ctrl Pts',(-6.68184963465256,0.552548454735263,
2.94568606831802));
#167596=CARTESIAN_POINT('Ctrl Pts',(-6.68120631232628,0.552287640367631,
2.94714362565901));
#167597=CARTESIAN_POINT('Ctrl Pts',(-6.68056299,0.552026826,2.948601183));
#167598=CARTESIAN_POINT('Ctrl Pts',(-6.616147978,0.525911829,3.094544468));
#167599=CARTESIAN_POINT('Ctrl Pts',(-6.545420922,0.49968693,3.237535445));
#167600=CARTESIAN_POINT('Ctrl Pts',(-6.654670810517,0.552548454735263,2.87710658956354));
#167601=CARTESIAN_POINT('Ctrl Pts',(-6.65404245337249,0.552287640367631,
2.87855822358338));
#167602=CARTESIAN_POINT('Ctrl Pts',(-6.653414096228,0.552026826,2.88000985760322));
#167603=CARTESIAN_POINT('Ctrl Pts',(-6.59049752804749,0.525911829,3.02536004830619));
#167604=CARTESIAN_POINT('Ctrl Pts',(-6.52129338588128,0.49968693,3.16782393583724));
#167605=CARTESIAN_POINT('',(-6.69381182758831,0.552026824386152,2.98207418132302));
#167606=CARTESIAN_POINT('Ctrl Pts',(-6.65653794114433,0.550751630586317,
2.87281241291839));
#167607=CARTESIAN_POINT('Ctrl Pts',(-6.65497800947308,0.551389228293159,
2.87641616495792));
#167608=CARTESIAN_POINT('Ctrl Pts',(-6.65341807780182,0.552026826,2.88001991699745));
#167609=CARTESIAN_POINT('Ctrl Pts',(-6.49652710679142,0.61615356,3.24246922627415));
#167610=CARTESIAN_POINT('Ctrl Pts',(-6.30119207219073,0.681389364000001,
3.58573079276282));
#167611=CARTESIAN_POINT('Ctrl Pts',(-6.73754606545278,0.550751630586317,
3.07683225208979));
#167612=CARTESIAN_POINT('Ctrl Pts',(-6.7358755812264,0.551389228293159,
3.08047976154489));
#167613=CARTESIAN_POINT('Ctrl Pts',(-6.734205097,0.552026826,3.084127271));
#167614=CARTESIAN_POINT('Ctrl Pts',(-6.566195243,0.61615356,3.450977506));
#167615=CARTESIAN_POINT('Ctrl Pts',(-6.359329057,0.681389364000001,3.797406123));
#167616=CARTESIAN_POINT('Ctrl Pts',(-6.30352756992328,0.68060908208268,
3.58162539475483));
#167617=CARTESIAN_POINT('Ctrl Pts',(-6.31915715586046,0.677652752700977,
3.59071136724813));
#167618=CARTESIAN_POINT('Ctrl Pts',(-6.33479158467919,0.674729896894376,
3.59979999996222));
#167619=CARTESIAN_POINT('Ctrl Pts',(-6.35043820069918,0.671836782521917,
3.60887704594859));
#167620=CARTESIAN_POINT('Ctrl Pts',(-6.3650858243296,0.669128385358378,
3.61737454809949));
#167621=CARTESIAN_POINT('Ctrl Pts',(-6.37974220004862,0.666446714467875,
3.62586552810993));
#167622=CARTESIAN_POINT('Ctrl Pts',(-6.39440688968761,0.663790956110878,
3.63435020025209));
#167623=CARTESIAN_POINT('Ctrl Pts',(-6.40907173677491,0.661135169240174,
3.64283496349042));
#167624=CARTESIAN_POINT('Ctrl Pts',(-6.4237449370569,0.658505288548661,
3.65131344117807));
#167625=CARTESIAN_POINT('Ctrl Pts',(-6.43842607969659,0.655900535543649,
3.65978583507949));
#167626=CARTESIAN_POINT('Ctrl Pts',(-6.30584618800001,0.681369595,3.577541593));
#167627=CARTESIAN_POINT('Ctrl Pts',(-6.3015823,0.679970133,3.585057207));
#167628=CARTESIAN_POINT('Ctrl Pts',(-6.297300509,0.678571429,3.592562637));
#167629=CARTESIAN_POINT('Ctrl Pts',(-6.105394932,0.615882895,3.928948446));
#167630=CARTESIAN_POINT('Ctrl Pts',(-5.878745916,0.552026826,4.242976131));
#167631=CARTESIAN_POINT('Ctrl Pts',(-6.51744456300001,0.681369595,3.51912996));
#167632=CARTESIAN_POINT('Ctrl Pts',(-6.513250293,0.679970133,3.526897768));
#167633=CARTESIAN_POINT('Ctrl Pts',(-6.509037518,0.678571429,3.534655555));
#167634=CARTESIAN_POINT('Ctrl Pts',(-6.32022519000001,0.615882895,3.882351818));
#167635=CARTESIAN_POINT('Ctrl Pts',(-6.095446908,0.552026826,4.207955121));
#167636=CARTESIAN_POINT('',(-5.91515190281437,0.552026824384634,4.23709255888292));
#167637=CARTESIAN_POINT('Ctrl Pts',(-6.133799235,0.499686101,3.962408073));
#167638=CARTESIAN_POINT('Ctrl Pts',(-6.073173866,0.51775868,4.056256015));
#167639=CARTESIAN_POINT('Ctrl Pts',(-6.009705774,0.535714286,4.148205311));
#167640=CARTESIAN_POINT('Ctrl Pts',(-5.980919823,0.54385805,4.189908912));
#167641=CARTESIAN_POINT('Ctrl Pts',(-5.951557878,0.552026826,4.231209003));
#167642=CARTESIAN_POINT('Ctrl Pts',(-6.061582466,0.499686101,3.977400912));
#167643=CARTESIAN_POINT('Ctrl Pts',(-6.000727704,0.51775868,4.07014392800001));
#167644=CARTESIAN_POINT('Ctrl Pts',(-5.93706413,0.535714286,4.160981797));
#167645=CARTESIAN_POINT('Ctrl Pts',(-5.908189518,0.54385805,4.20218131));
#167646=CARTESIAN_POINT('Ctrl Pts',(-5.878745916,0.552026826,4.242976131));
#167647=CARTESIAN_POINT('Ctrl Pts',(-5.87874591253852,0.552026827331392,
4.24297613682539));
#167648=CARTESIAN_POINT('Ctrl Pts',(-5.90818951603908,0.543858051066734,
4.20218131293737));
#167649=CARTESIAN_POINT('Ctrl Pts',(-5.93706413,0.535714286,4.160981797));
#167650=CARTESIAN_POINT('Ctrl Pts',(-6.00017468145858,0.51791465388332,
4.07093300385634));
#167651=CARTESIAN_POINT('Ctrl Pts',(-6.06052525045423,0.499999999933982,
3.97901164806512));
#167652=CARTESIAN_POINT('Ctrl Pts',(-6.06052525045423,0.499999999933982,
3.97901164806512));
#167653=CARTESIAN_POINT('Ctrl Pts',(-6.00017468145858,0.51791465388332,
4.07093300385634));
#167654=CARTESIAN_POINT('Ctrl Pts',(-5.93706413,0.535714286,4.160981797));
#167655=CARTESIAN_POINT('Ctrl Pts',(-5.90818951603908,0.543858051066734,
4.20218131293737));
#167656=CARTESIAN_POINT('Ctrl Pts',(-5.87874591253852,0.552026827331392,
4.24297613682539));
#167657=CARTESIAN_POINT('Ctrl Pts',(-6.07333975208833,0.499999999933982,
4.0408184325369));
#167658=CARTESIAN_POINT('Ctrl Pts',(-6.01205174511351,0.51791465388332,
4.1329341489989));
#167659=CARTESIAN_POINT('Ctrl Pts',(-5.94799829402805,0.535714286,4.22314878315257));
#167660=CARTESIAN_POINT('Ctrl Pts',(-5.91869227907855,0.543858051066734,
4.26442417559135));
#167661=CARTESIAN_POINT('Ctrl Pts',(-5.88881626406081,0.552026827331392,
4.30528888183963));
#167662=CARTESIAN_POINT('Ctrl Pts',(-5.87874591253852,0.552026827331392,
4.24297613682539));
#167663=CARTESIAN_POINT('Ctrl Pts',(-5.88300430884132,0.551172308387581,
4.24600007043486));
#167664=CARTESIAN_POINT('Ctrl Pts',(-5.88726358305087,0.550320535056991,
4.24902353649116));
#167665=CARTESIAN_POINT('Ctrl Pts',(-5.89152372856485,0.549471478151584,
4.25204653631538));
#167666=CARTESIAN_POINT('Ctrl Pts',(-5.89547868642776,0.548683245854569,
4.25485297494176));
#167667=CARTESIAN_POINT('Ctrl Pts',(-5.89943439628991,0.547897354521786,
4.25765901249858));
#167668=CARTESIAN_POINT('Ctrl Pts',(-5.90339084739567,0.547113782454407,
4.26046465142468));
#167669=CARTESIAN_POINT('Ctrl Pts',(-5.90734730248218,0.546330209598645,
4.26327029317365));
#167670=CARTESIAN_POINT('Ctrl Pts',(-5.91130449981241,0.545548955815742,
4.2660755369981));
#167671=CARTESIAN_POINT('Ctrl Pts',(-5.91526242801923,0.544769999921413,
4.26888038644755));
#167672=CARTESIAN_POINT('Ctrl Pts',(-5.879849956,0.55233793,4.241446038));
#167673=CARTESIAN_POINT('Ctrl Pts',(-5.78663932800001,0.526068113,4.370662467));
#167674=CARTESIAN_POINT('Ctrl Pts',(-5.687842072,0.49968693,4.495659303));
#167675=CARTESIAN_POINT('Ctrl Pts',(-5.942533939,0.55233793,4.23129895));
#167676=CARTESIAN_POINT('Ctrl Pts',(-5.849546304,0.526068113,4.361892931));
#167677=CARTESIAN_POINT('Ctrl Pts',(-5.750911309,0.49968693,4.488275785));
#167678=CARTESIAN_POINT('Origin',(0.145053107207914,0.41074311058109,-0.133432913130858));
#167679=CARTESIAN_POINT('Ctrl Pts',(-5.8923962720813,0.552548454735263,
4.31321772265892));
#167680=CARTESIAN_POINT('Ctrl Pts',(-5.89145465854065,0.552287640367631,
4.31450290782946));
#167681=CARTESIAN_POINT('Ctrl Pts',(-5.890513045,0.552026826,4.315788093));
#167682=CARTESIAN_POINT('Ctrl Pts',(-5.796230529,0.525911829,4.444471981));
#167683=CARTESIAN_POINT('Ctrl Pts',(-5.696418198,0.49968693,4.568915682));
#167684=CARTESIAN_POINT('Ctrl Pts',(-5.88059543510538,0.552548454735263,
4.24039894946615));
#167685=CARTESIAN_POINT('Ctrl Pts',(-5.87966971019993,0.552287640367631,
4.24168156687897));
#167686=CARTESIAN_POINT('Ctrl Pts',(-5.87874398529449,0.552026826,4.24296418429179));
#167687=CARTESIAN_POINT('Ctrl Pts',(-5.78605237728176,0.525911829,4.37139096611371));
#167688=CARTESIAN_POINT('Ctrl Pts',(-5.68784066486205,0.49968693,4.49564728337354));
#167689=CARTESIAN_POINT('',(-5.89625642747112,0.552026824384635,4.35132661890885));
#167690=CARTESIAN_POINT('Ctrl Pts',(-5.88334203389657,0.550751630586317,
4.23660654365286));
#167691=CARTESIAN_POINT('Ctrl Pts',(-5.88104387239856,0.551389228293159,
4.23979070277515));
#167692=CARTESIAN_POINT('Ctrl Pts',(-5.87874571090055,0.552026826,4.24297486189745));
#167693=CARTESIAN_POINT('Ctrl Pts',(-5.64760687603574,0.61615356,4.56322338672453));
#167694=CARTESIAN_POINT('Ctrl Pts',(-5.38304757597552,0.681389364000001,
4.8564684301278));
#167695=CARTESIAN_POINT('Ctrl Pts',(-5.91859799888374,0.550751630586317,
4.45327086703888));
#167696=CARTESIAN_POINT('Ctrl Pts',(-5.91618246294187,0.551389228293159,
4.45647399501944));
#167697=CARTESIAN_POINT('Ctrl Pts',(-5.913766927,0.552026826,4.459677123));
#167698=CARTESIAN_POINT('Ctrl Pts',(-5.670823094,0.61615356,4.781833451));
#167699=CARTESIAN_POINT('Ctrl Pts',(-5.394321411,0.681389364000001,5.07569264400001));
#167700=CARTESIAN_POINT('Ctrl Pts',(-5.3862110102017,0.680609082082614,
4.85296107987893));
#167701=CARTESIAN_POINT('Ctrl Pts',(-5.39952197013657,0.677652752615266,
4.86519452629108));
#167702=CARTESIAN_POINT('Ctrl Pts',(-5.41283708726114,0.674729896815345,
4.87743161198875));
#167703=CARTESIAN_POINT('Ctrl Pts',(-5.42616659749073,0.671836782445242,
4.88966000170458));
#167704=CARTESIAN_POINT('Ctrl Pts',(-5.43864505594036,0.669128385299696,
4.90110764309173));
#167705=CARTESIAN_POINT('Ctrl Pts',(-5.45113346393363,0.666446714428098,
4.91255079625585));
#167706=CARTESIAN_POINT('Ctrl Pts',(-5.46363134748315,0.663790956090451,
4.92398957626689));
#167707=CARTESIAN_POINT('Ctrl Pts',(-5.47612936521697,0.661135169239089,
4.93542847909109));
#167708=CARTESIAN_POINT('Ctrl Pts',(-5.4886368920659,0.658505288567361,
4.94686303900093));
#167709=CARTESIAN_POINT('Ctrl Pts',(-5.50115348400725,0.655900535618631,
4.95829336454301));
#167710=CARTESIAN_POINT('Ctrl Pts',(-5.38935331700001,0.681369595,4.84947119));
#167711=CARTESIAN_POINT('Ctrl Pts',(-5.383573482,0.679970133,4.855894483));
#167712=CARTESIAN_POINT('Ctrl Pts',(-5.377778351,0.678571429,4.862303981));
#167713=CARTESIAN_POINT('Ctrl Pts',(-5.118046414,0.615882895,5.149571251));
#167714=CARTESIAN_POINT('Ctrl Pts',(-4.829189657,0.552026826,5.407534305));
#167715=CARTESIAN_POINT('Ctrl Pts',(-5.608561414,0.681369595,4.837912584));
#167716=CARTESIAN_POINT('Ctrl Pts',(-5.602795355,0.679970133,4.844597141));
#167717=CARTESIAN_POINT('Ctrl Pts',(-5.597013377,0.678571429,4.851267933));
#167718=CARTESIAN_POINT('Ctrl Pts',(-5.33787095800001,0.615882895,5.150246182));
#167719=CARTESIAN_POINT('Ctrl Pts',(-5.048352782,0.552026826,5.419916374));
#167720=CARTESIAN_POINT('',(-4.86600928592336,0.552026824384634,5.40961449782261));
#167721=CARTESIAN_POINT('Ctrl Pts',(-5.13859381,0.499686101,5.188354696));
#167722=CARTESIAN_POINT('Ctrl Pts',(-5.059211294,0.51775868,5.266975863));
#167723=CARTESIAN_POINT('Ctrl Pts',(-4.977460671,0.535714286,5.343131672));
#167724=CARTESIAN_POINT('Ctrl Pts',(-4.940382678,0.54385805,5.377672137));
#167725=CARTESIAN_POINT('Ctrl Pts',(-4.9028289,0.552026826,5.41169470400001));
#167726=CARTESIAN_POINT('Ctrl Pts',(-5.064842411,0.499686101,5.18747254));
#167727=CARTESIAN_POINT('Ctrl Pts',(-4.985473393,0.51775868,5.264965301));
#167728=CARTESIAN_POINT('Ctrl Pts',(-4.903770781,0.535714286,5.339993645));
#167729=CARTESIAN_POINT('Ctrl Pts',(-4.866714564,0.54385805,5.374022748));
#167730=CARTESIAN_POINT('Ctrl Pts',(-4.829189657,0.552026826,5.40753430500001));
#167731=CARTESIAN_POINT('Ctrl Pts',(-4.82918965683727,0.552026826325504,
5.40753430538259));
#167732=CARTESIAN_POINT('Ctrl Pts',(-4.85422461787804,0.546576979803602,
5.38517687395041));
#167733=CARTESIAN_POINT('Ctrl Pts',(-4.87908593870346,0.54113922028644,
5.36266198795457));
#167734=CARTESIAN_POINT('Ctrl Pts',(-4.90377078115005,0.535714285967023,
5.33999364486221));
#167735=CARTESIAN_POINT('Ctrl Pts',(-4.95767392528447,0.523868108781526,
5.29049383644694));
#167736=CARTESIAN_POINT('Ctrl Pts',(-5.01091942444511,0.511960760933383,
5.24009317944469));
#167737=CARTESIAN_POINT('Ctrl Pts',(-5.06346365273142,0.49999999975226,
5.18881834708339));
#167738=CARTESIAN_POINT('Ctrl Pts',(-5.064842411,0.499686101,5.18747254));
#167739=CARTESIAN_POINT('Ctrl Pts',(-4.985473393,0.51775868,5.264965301));
#167740=CARTESIAN_POINT('Ctrl Pts',(-4.903770781,0.535714286,5.339993645));
#167741=CARTESIAN_POINT('Ctrl Pts',(-4.866006155,0.544013736,5.374673287));
#167742=CARTESIAN_POINT('Ctrl Pts',(-4.82775482,0.552339147,5.408815342));
#167743=CARTESIAN_POINT('Ctrl Pts',(-5.064082929,0.499686101,5.250967958));
#167744=CARTESIAN_POINT('Ctrl Pts',(-4.983742422,0.51775868,5.328449099));
#167745=CARTESIAN_POINT('Ctrl Pts',(-4.901069133,0.535714286,5.403436108));
#167746=CARTESIAN_POINT('Ctrl Pts',(-4.862855839,0.544013736,5.438096644));
#167747=CARTESIAN_POINT('Ctrl Pts',(-4.824156151,0.552339147,5.472213249));
#167748=CARTESIAN_POINT('Ctrl Pts',(-4.82918965212967,0.5520268273503,5.4075343095867));
#167749=CARTESIAN_POINT('Ctrl Pts',(-4.8326984334768,0.551172308320109,
5.41140297452869));
#167750=CARTESIAN_POINT('Ctrl Pts',(-4.83620817239363,0.550320534982899,
5.41527137164601));
#167751=CARTESIAN_POINT('Ctrl Pts',(-4.83971886247769,0.549471478073663,
5.41913950073001));
#167752=CARTESIAN_POINT('Ctrl Pts',(-4.84297805423243,0.548683245785531,
5.42273052531918));
#167753=CARTESIAN_POINT('Ctrl Pts',(-4.84623806662961,0.547897354464017,
5.42632131986788));
#167754=CARTESIAN_POINT('Ctrl Pts',(-4.84949888862985,0.547113782411179,
5.42991188444141));
#167755=CARTESIAN_POINT('Ctrl Pts',(-4.85275971392499,0.546330209566579,
5.43350245264303));
#167756=CARTESIAN_POINT('Ctrl Pts',(-4.85602134964807,0.545548955798043,
5.43709279177419));
#167757=CARTESIAN_POINT('Ctrl Pts',(-4.85928378415849,0.544769999867977,
5.44068290297567));
#167758=CARTESIAN_POINT('Ctrl Pts',(-4.83059681,0.55233793,5.40627732));
#167759=CARTESIAN_POINT('Ctrl Pts',(-4.71178768100001,0.526068113,5.512435211));
#167760=CARTESIAN_POINT('Ctrl Pts',(-4.588429626,0.49968693,5.613271201));
#167761=CARTESIAN_POINT('Ctrl Pts',(-4.893996599,0.55233793,5.40984266800001));
#167762=CARTESIAN_POINT('Ctrl Pts',(-4.775109118,0.526068113,5.517393842));
#167763=CARTESIAN_POINT('Ctrl Pts',(-4.651611577,0.49968693,5.619618328));
#167764=CARTESIAN_POINT('Origin',(0.112978642611034,0.410742823000216,-0.161496613303563));
#167765=CARTESIAN_POINT('Ctrl Pts',(-4.82742100891798,0.552548454735263,
5.47906810964861));
#167766=CARTESIAN_POINT('Ctrl Pts',(-4.82622513295899,0.552287640367631,
5.48012082882431));
#167767=CARTESIAN_POINT('Ctrl Pts',(-4.825029257,0.552026826,5.481173548));
#167768=CARTESIAN_POINT('Ctrl Pts',(-4.705287782,0.525911829,5.586580924));
#167769=CARTESIAN_POINT('Ctrl Pts',(-4.581057291,0.49968693,5.68665850000001));
#167770=CARTESIAN_POINT('Ctrl Pts',(-4.83154995323541,0.552548454735263,
5.40541496848023));
#167771=CARTESIAN_POINT('Ctrl Pts',(-4.830370146429,0.552287640367631,5.40646859551687));
#167772=CARTESIAN_POINT('Ctrl Pts',(-4.82919033962259,0.552026826,5.4075222225535));
#167773=CARTESIAN_POINT('Ctrl Pts',(-4.71105784757507,0.525911829,5.51302050146606));
#167774=CARTESIAN_POINT('Ctrl Pts',(-4.58843083562465,0.49968693,5.61325915989151));
#167775=CARTESIAN_POINT('',(-4.82299863007088,0.552026824384634,5.51711586088163));
#167776=CARTESIAN_POINT('Ctrl Pts',(-4.83504759308386,0.550751630586317,
5.40230166699065));
#167777=CARTESIAN_POINT('Ctrl Pts',(-4.83211866123137,0.551389228293159,
5.40491734544072));
#167778=CARTESIAN_POINT('Ctrl Pts',(-4.82918972937888,0.552026826,5.4075330238908));
#167779=CARTESIAN_POINT('Ctrl Pts',(-4.53461082516816,0.61615356,5.67060629783368));
#167780=CARTESIAN_POINT('Ctrl Pts',(-4.21319775811611,0.681389364,5.90012300633437));
#167781=CARTESIAN_POINT('Ctrl Pts',(-4.82290286777508,0.550751630586317,
5.62147948639974));
#167782=CARTESIAN_POINT('Ctrl Pts',(-4.81985522788754,0.551389228293159,
5.62408845819987));
#167783=CARTESIAN_POINT('Ctrl Pts',(-4.816807588,0.552026826,5.62669743));
#167784=CARTESIAN_POINT('Ctrl Pts',(-4.510289559,0.61615356,5.889096179));
#167785=CARTESIAN_POINT('Ctrl Pts',(-4.177081292,0.681389364000001,6.116645419));
#167786=CARTESIAN_POINT('Ctrl Pts',(-4.21704120998561,0.680609082247451,
5.89737769848892));
#167787=CARTESIAN_POINT('Ctrl Pts',(-4.22741113718361,0.677652752732438,
5.91218659723743));
#167788=CARTESIAN_POINT('Ctrl Pts',(-4.2377843429517,0.674729896861193,
5.92699994298084));
#167789=CARTESIAN_POINT('Ctrl Pts',(-4.24817347433186,0.671836782492805,
5.94180789041485));
#167790=CARTESIAN_POINT('Ctrl Pts',(-4.25789928888653,0.669128385341709,
5.95567039204358));
#167791=CARTESIAN_POINT('Ctrl Pts',(-4.26763578519879,0.666446714464492,
5.96953064924376));
#167792=CARTESIAN_POINT('Ctrl Pts',(-4.27738247562702,0.663790956121092,
5.9833886725012));
#167793=CARTESIAN_POINT('Ctrl Pts',(-4.28712927070118,0.661135169263983,
5.99724684454615));
#167794=CARTESIAN_POINT('Ctrl Pts',(-4.29688628616516,0.658505288586374,
6.01110281939429));
#167795=CARTESIAN_POINT('Ctrl Pts',(-4.30665306547384,0.655900535733099,
6.02495660721441));
#167796=CARTESIAN_POINT('Ctrl Pts',(-4.220860275,0.681369595,5.89464490299999));
#167797=CARTESIAN_POINT('Ctrl Pts',(-4.213834751,0.679970133,5.89967553000001));
#167798=CARTESIAN_POINT('Ctrl Pts',(-4.206797255,0.678571429,5.904689396));
#167799=CARTESIAN_POINT('Ctrl Pts',(-3.891383734,0.615882895,6.129405827));
#167800=CARTESIAN_POINT('Ctrl Pts',(-3.553825856,0.552026826,6.319242184));
#167801=CARTESIAN_POINT('Ctrl Pts',(-4.437428167,0.681369595,5.930479793));
#167802=CARTESIAN_POINT('Ctrl Pts',(-4.430359933,0.679970133,5.935768535));
#167803=CARTESIAN_POINT('Ctrl Pts',(-4.423279112,0.678571429,5.941040415));
#167804=CARTESIAN_POINT('Ctrl Pts',(-4.105923812,0.615882895,6.177320758));
#167805=CARTESIAN_POINT('Ctrl Pts',(-3.765203291,0.552026826,6.378448361));
#167806=CARTESIAN_POINT('',(-3.58933748268525,0.552026824384634,6.32918887507452));
#167807=CARTESIAN_POINT('Ctrl Pts',(-3.903113449,0.499686101,6.17169962));
#167808=CARTESIAN_POINT('Ctrl Pts',(-3.808685626,0.51775868,6.231417774));
#167809=CARTESIAN_POINT('Ctrl Pts',(-3.712475039,0.535714286,6.288219134));
#167810=CARTESIAN_POINT('Ctrl Pts',(-3.668838729,0.54385805,6.31398139));
#167811=CARTESIAN_POINT('Ctrl Pts',(-3.624849092,0.552026826,6.339135576));
#167812=CARTESIAN_POINT('Ctrl Pts',(-3.831275955,0.499686101,6.154983717));
#167813=CARTESIAN_POINT('Ctrl Pts',(-3.737103887,0.51775868,6.213602748));
#167814=CARTESIAN_POINT('Ctrl Pts',(-3.641182561,0.535714286,6.269313324));
#167815=CARTESIAN_POINT('Ctrl Pts',(-3.597677446,0.54385805,6.294580855));
#167816=CARTESIAN_POINT('Ctrl Pts',(-3.553825856,0.552026826,6.319242184));
#167817=CARTESIAN_POINT('Ctrl Pts',(-3.55382585773626,0.552026826,6.31924218448633));
#167818=CARTESIAN_POINT('Ctrl Pts',(-3.60037628942064,0.543355303658993,
6.29306307716329));
#167819=CARTESIAN_POINT('Ctrl Pts',(-3.64659721603784,0.534726107585227,
6.26639278095636));
#167820=CARTESIAN_POINT('Ctrl Pts',(-3.73854930035679,0.517398611874174,
6.21197293578532));
#167821=CARTESIAN_POINT('Ctrl Pts',(-3.78424732666389,0.508709444526294,
6.184240463273));
#167822=CARTESIAN_POINT('Ctrl Pts',(-3.8296401228719,0.499999999696683,
6.15600166741686));
#167823=CARTESIAN_POINT('Ctrl Pts',(-3.831275955,0.499686101,6.154983717));
#167824=CARTESIAN_POINT('Ctrl Pts',(-3.737103887,0.51775868,6.213602748));
#167825=CARTESIAN_POINT('Ctrl Pts',(-3.641182561,0.535714286,6.269313324));
#167826=CARTESIAN_POINT('Ctrl Pts',(-3.596845753,0.544013736,6.295063898));
#167827=CARTESIAN_POINT('Ctrl Pts',(-3.55214918,0.552339147,6.320184824));
#167828=CARTESIAN_POINT('Ctrl Pts',(-3.816884591,0.499686101,6.216831382));
#167829=CARTESIAN_POINT('Ctrl Pts',(-3.721766245,0.51775868,6.275230223));
#167830=CARTESIAN_POINT('Ctrl Pts',(-3.624905821,0.535714286,6.330691763));
#167831=CARTESIAN_POINT('Ctrl Pts',(-3.580134942,0.544013736,6.356327227));
#167832=CARTESIAN_POINT('Ctrl Pts',(-3.53500597,0.552339147,6.381326915));
#167833=CARTESIAN_POINT('Ctrl Pts',(-3.55382585052444,0.552026827376882,
6.31924218800207));
#167834=CARTESIAN_POINT('Ctrl Pts',(-3.55642095025658,0.551172308303609,
6.32377468954546));
#167835=CARTESIAN_POINT('Ctrl Pts',(-3.55901704240399,0.550320534962719,
6.32830713585479));
#167836=CARTESIAN_POINT('Ctrl Pts',(-3.56161412108933,0.549471478046711,
6.33283952487593));
#167837=CARTESIAN_POINT('Ctrl Pts',(-3.56402515059284,0.548683245758558,
6.33704722320754));
#167838=CARTESIAN_POINT('Ctrl Pts',(-3.56643703099503,0.54789735443435,
6.34125487329571));
#167839=CARTESIAN_POINT('Ctrl Pts',(-3.56884975150297,0.547113782376603,
6.34546247282981));
#167840=CARTESIAN_POINT('Ctrl Pts',(-3.57126247444884,0.546330209527098,
6.34967007661546));
#167841=CARTESIAN_POINT('Ctrl Pts',(-3.57367603811166,0.545548955751532,
6.35387763090795));
#167842=CARTESIAN_POINT('Ctrl Pts',(-3.57609043026655,0.544769999930891,
6.35808513457863));
#167843=CARTESIAN_POINT('Ctrl Pts',(-3.555470326,0.55233793,6.318317083));
#167844=CARTESIAN_POINT('Ctrl Pts',(-3.41661808,0.526068113,6.39645261100001));
#167845=CARTESIAN_POINT('Ctrl Pts',(-3.27446731,0.49968693,6.468412776));
#167846=CARTESIAN_POINT('Ctrl Pts',(-3.616621419,0.55233793,6.335428156));
#167847=CARTESIAN_POINT('Ctrl Pts',(-3.477393138,0.526068113,6.414907549));
#167848=CARTESIAN_POINT('Ctrl Pts',(-3.334807658,0.49968693,6.488193762));
#167849=CARTESIAN_POINT('Origin',(0.075619904091393,0.410742926312177,-0.182007274607002));
#167850=CARTESIAN_POINT('Ctrl Pts',(-3.53672090509896,0.552548454735263,
6.38872336160058));
#167851=CARTESIAN_POINT('Ctrl Pts',(-3.53532668454948,0.552287640367631,
6.38949439080029));
#167852=CARTESIAN_POINT('Ctrl Pts',(-3.533932464,0.552026826,6.39026542));
#167853=CARTESIAN_POINT('Ctrl Pts',(-3.394331008,0.525911829,6.467467552));
#167854=CARTESIAN_POINT('Ctrl Pts',(-3.251491236,0.49968693,6.538499487));
#167855=CARTESIAN_POINT('Ctrl Pts',(-3.55658656450835,0.552548454735263,
6.31767979036095));
#167856=CARTESIAN_POINT('Ctrl Pts',(-3.55520784226221,0.552287640367631,
6.31845516059789));
#167857=CARTESIAN_POINT('Ctrl Pts',(-3.55382912001605,0.552026826,6.31923053083484));
#167858=CARTESIAN_POINT('Ctrl Pts',(-3.41577948859051,0.525911829,6.39686732514053));
#167859=CARTESIAN_POINT('Ctrl Pts',(-3.27447107980831,0.49968693,6.46840127649554));
#167860=CARTESIAN_POINT('',(-3.52422277681663,0.552026824384635,6.42493089616388));
#167861=CARTESIAN_POINT('Ctrl Pts',(-3.56067169923797,0.550751630586317,
6.31539116543644));
#167862=CARTESIAN_POINT('Ctrl Pts',(-3.55724895063607,0.551389228293159,
6.31731605701395));
#167863=CARTESIAN_POINT('Ctrl Pts',(-3.55382620203417,0.552026826,6.31924094859146));
#167864=CARTESIAN_POINT('Ctrl Pts',(-3.20958141133387,0.61615356,6.51283795944189));
#167865=CARTESIAN_POINT('Ctrl Pts',(-2.8463434961876,0.681389364000001,
6.66789438649148));
#167866=CARTESIAN_POINT('Ctrl Pts',(-3.5016941591658,0.550751630586317,
6.52683397198676));
#167867=CARTESIAN_POINT('Ctrl Pts',(-3.4981569195829,0.551389228293159,
6.52872679499338));
#167868=CARTESIAN_POINT('Ctrl Pts',(-3.49461968,0.552026826,6.530619618));
#167869=CARTESIAN_POINT('Ctrl Pts',(-3.138859897,0.61615356,6.720991315));
#167870=CARTESIAN_POINT('Ctrl Pts',(-2.764525494,0.681389364000001,6.871590653));
#167871=CARTESIAN_POINT('Ctrl Pts',(-2.85068725011335,0.680609082082589,
6.66603949042971));
#167872=CARTESIAN_POINT('Ctrl Pts',(-2.85763125915416,0.677652752703801,
6.68273139310465));
#167873=CARTESIAN_POINT('Ctrl Pts',(-2.8645775133876,0.67472989686154,6.69942834382325));
#167874=CARTESIAN_POINT('Ctrl Pts',(-2.87154048165055,0.6718367824759,6.71612344585627));
#167875=CARTESIAN_POINT('Ctrl Pts',(-2.8780588839478,0.669128385317478,
6.73175261251841));
#167876=CARTESIAN_POINT('Ctrl Pts',(-2.8845882007636,0.66644671443324,6.74738188348409));
#167877=CARTESIAN_POINT('Ctrl Pts',(-2.89112795360198,0.66379095608324,
6.76301116416583));
#167878=CARTESIAN_POINT('Ctrl Pts',(-2.89766777665485,0.661135169219524,
6.77864061265232));
#167879=CARTESIAN_POINT('Ctrl Pts',(-2.90421805349058,0.658505288535728,
6.79427011238982));
#167880=CARTESIAN_POINT('Ctrl Pts',(-2.91077833515283,0.655900535563285,
6.80989957534335));
#167881=CARTESIAN_POINT('Ctrl Pts',(-2.855004498,0.681369595,6.664191573));
#167882=CARTESIAN_POINT('Ctrl Pts',(-2.84706179,0.679970133,6.667594306));
#167883=CARTESIAN_POINT('Ctrl Pts',(-2.839110994,0.678571429,6.670978097));
#167884=CARTESIAN_POINT('Ctrl Pts',(-2.482764276,0.615882895,6.8226362));
#167885=CARTESIAN_POINT('Ctrl Pts',(-2.112289109,0.552026826,6.935469322));
#167886=CARTESIAN_POINT('Ctrl Pts',(-3.058805711,0.681369595,6.745744357));
#167887=CARTESIAN_POINT('Ctrl Pts',(-3.050765805,0.679970133,6.749389991));
#167888=CARTESIAN_POINT('Ctrl Pts',(-3.042717231,0.678571429,6.753016449));
#167889=CARTESIAN_POINT('Ctrl Pts',(-2.681988233,0.615882895,6.915550681));
#167890=CARTESIAN_POINT('Ctrl Pts',(-2.305997078,0.552026826,7.038731191));
#167891=CARTESIAN_POINT('',(-2.14483224854103,0.552026824384634,6.95281741505674));
#167892=CARTESIAN_POINT('Ctrl Pts',(-2.485127842,0.499686101,6.866462729));
#167893=CARTESIAN_POINT('Ctrl Pts',(-2.380070051,0.51775868,6.904485514));
#167894=CARTESIAN_POINT('Ctrl Pts',(-2.2738982,0.535714286,6.939276459));
#167895=CARTESIAN_POINT('Ctrl Pts',(-2.22574396,0.54385805,6.95505589100001));
#167896=CARTESIAN_POINT('Ctrl Pts',(-2.177375369,0.552026826,6.970165514));
#167897=CARTESIAN_POINT('Ctrl Pts',(-2.418563293,0.499686101,6.834694697));
#167898=CARTESIAN_POINT('Ctrl Pts',(-2.313991557,0.51775868,6.871699036));
#167899=CARTESIAN_POINT('Ctrl Pts',(-2.208336691,0.535714286,6.905486881));
#167900=CARTESIAN_POINT('Ctrl Pts',(-2.16041693,0.54385805,6.920811357));
#167901=CARTESIAN_POINT('Ctrl Pts',(-2.112289109,0.552026826,6.93546932199999));
#167902=CARTESIAN_POINT('Ctrl Pts',(-2.11228911851721,0.552026824384636,
6.9354693191014));
#167903=CARTESIAN_POINT('Ctrl Pts',(-2.14439786744358,0.546576979114217,
6.92569017451321));
#167904=CARTESIAN_POINT('Ctrl Pts',(-2.17641514314413,0.541139220240677,
6.91569521643116));
#167905=CARTESIAN_POINT('Ctrl Pts',(-2.20833669128259,0.535714285951975,
6.90548688090963));
#167906=CARTESIAN_POINT('Ctrl Pts',(-2.27804228996729,0.523868108739421,
6.88319541385762));
#167907=CARTESIAN_POINT('Ctrl Pts',(-2.34752928232983,0.511960760974455,
6.85981022134622));
#167908=CARTESIAN_POINT('Ctrl Pts',(-2.41674687579387,0.499999999814145,
6.83533719297713));
#167909=CARTESIAN_POINT('Ctrl Pts',(-2.418563293,0.499686101,6.834694697));
#167910=CARTESIAN_POINT('Ctrl Pts',(-2.313991557,0.51775868,6.871699036));
#167911=CARTESIAN_POINT('Ctrl Pts',(-2.208336691,0.535714286,6.905486881));
#167912=CARTESIAN_POINT('Ctrl Pts',(-2.159500841,0.544013736,6.921104317));
#167913=CARTESIAN_POINT('Ctrl Pts',(-2.110448992,0.552339147,6.936029488));
#167914=CARTESIAN_POINT('Ctrl Pts',(-2.391212971,0.499686101,6.89200268));
#167915=CARTESIAN_POINT('Ctrl Pts',(-2.285764415,0.51775868,6.928588556));
#167916=CARTESIAN_POINT('Ctrl Pts',(-2.179245942,0.535714286,6.961931308));
#167917=CARTESIAN_POINT('Ctrl Pts',(-2.130010915,0.544013736,6.977343013));
#167918=CARTESIAN_POINT('Ctrl Pts',(-2.080562839,0.552339147,6.99205682800001));
#167919=CARTESIAN_POINT('Ctrl Pts',(-2.11228910270316,0.55202682722255,
6.93546932462214));
#167920=CARTESIAN_POINT('Ctrl Pts',(-2.11384917561811,0.551172308325923,
6.94045372896119));
#167921=CARTESIAN_POINT('Ctrl Pts',(-2.11541023070314,0.550320534981382,
6.9454382922976));
#167922=CARTESIAN_POINT('Ctrl Pts',(-2.11697226156282,0.549471478060439,
6.95042301176581));
#167923=CARTESIAN_POINT('Ctrl Pts',(-2.11842239183661,0.548683245780907,
6.95505063647782));
#167924=CARTESIAN_POINT('Ctrl Pts',(-2.11987336347447,0.547897354464024,
6.95967839699587));
#167925=CARTESIAN_POINT('Ctrl Pts',(-2.12132516643249,0.547113782412266,
6.96430628874322));
#167926=CARTESIAN_POINT('Ctrl Pts',(-2.12277697085747,0.546330209568754,
6.96893418516678));
#167927=CARTESIAN_POINT('Ctrl Pts',(-2.12422960697141,0.545548955797813,
6.97356221398711));
#167928=CARTESIAN_POINT('Ctrl Pts',(-2.12568306337267,0.544769999930616,
6.97819037138624));
#167929=CARTESIAN_POINT('Ctrl Pts',(-2.114094,0.55233793,6.934919362));
#167930=CARTESIAN_POINT('Ctrl Pts',(-1.961691214,0.526068113,6.981378996));
#167931=CARTESIAN_POINT('Ctrl Pts',(-1.807394542,0.49968693,7.021098559));
#167932=CARTESIAN_POINT('Ctrl Pts',(-2.17013704,0.55233793,6.964776065));
#167933=CARTESIAN_POINT('Ctrl Pts',(-2.017078119,0.526068113,7.012467309));
#167934=CARTESIAN_POINT('Ctrl Pts',(-1.862071839,0.49968693,7.053388468));
#167935=CARTESIAN_POINT('Origin',(0.0347259231310537,0.410742962889062,
-0.194008600247233));
#167936=CARTESIAN_POINT('Ctrl Pts',(-2.0806476628918,0.552548454735263,
6.99964900947168));
#167937=CARTESIAN_POINT('Ctrl Pts',(-2.0791202899459,0.552287640367631,
7.00010229623584));
#167938=CARTESIAN_POINT('Ctrl Pts',(-2.077592917,0.552026826,7.000555583));
#167939=CARTESIAN_POINT('Ctrl Pts',(-1.924659088,0.525911829,7.045942586));
#167940=CARTESIAN_POINT('Ctrl Pts',(-1.769889065,0.49968693,7.084607504));
#167941=CARTESIAN_POINT('Ctrl Pts',(-2.11532114214784,0.552548454735263,
6.93453692693789));
#167942=CARTESIAN_POINT('Ctrl Pts',(-2.11380797197949,0.552287640367631,
6.93499778492344));
#167943=CARTESIAN_POINT('Ctrl Pts',(-2.11229480181114,0.552026826,6.935458642909));
#167944=CARTESIAN_POINT('Ctrl Pts',(-1.96078307810616,0.525911829,6.98160374227399));
#167945=CARTESIAN_POINT('Ctrl Pts',(-1.80740069574729,0.49968693,7.02108813870865));
#167946=CARTESIAN_POINT('',(-2.06065818415013,0.552026824384635,7.03232330417225));
#167947=CARTESIAN_POINT('Ctrl Pts',(-2.11980275666774,0.550751630586317,
6.93317998964714));
#167948=CARTESIAN_POINT('Ctrl Pts',(-2.11604623522881,0.551389228293159,
6.93432408856375));
#167949=CARTESIAN_POINT('Ctrl Pts',(-2.11228971378988,0.552026826,6.93546818748035));
#167950=CARTESIAN_POINT('Ctrl Pts',(-1.73447553959357,0.61615356,7.05053655442669));
#167951=CARTESIAN_POINT('Ctrl Pts',(-1.34639737645262,0.681389364000001,
7.12388243289172));
#167952=CARTESIAN_POINT('Ctrl Pts',(-2.01675012375466,0.550751630586317,
7.12700095619441));
#167953=CARTESIAN_POINT('Ctrl Pts',(-2.01288868187733,0.551389228293159,
7.12808912409721));
#167954=CARTESIAN_POINT('Ctrl Pts',(-2.00902724,0.552026826,7.129177292));
#167955=CARTESIAN_POINT('Ctrl Pts',(-1.620660636,0.61615356,7.238620367));
#167956=CARTESIAN_POINT('Ctrl Pts',(-1.222703557,0.681389364000001,7.30522794400001));
#167957=CARTESIAN_POINT('Ctrl Pts',(-1.35103832261866,0.680609082082491,
7.12300468506535));
#167958=CARTESIAN_POINT('Ctrl Pts',(-1.35423171894373,0.677652752598905,
7.14079909641027));
#167959=CARTESIAN_POINT('Ctrl Pts',(-1.35742622271479,0.674729896796178,
7.15859892100758));
#167960=CARTESIAN_POINT('Ctrl Pts',(-1.36063744721483,0.671836782439989,
7.1764005331519));
#167961=CARTESIAN_POINT('Ctrl Pts',(-1.36364364406078,0.669128385299764,
7.19306556242043));
#167962=CARTESIAN_POINT('Ctrl Pts',(-1.36666047782784,0.666446714432678,
7.20973303985256));
#167963=CARTESIAN_POINT('Ctrl Pts',(-1.36968750153995,0.663790956098867,
7.22640277020986));
#167964=CARTESIAN_POINT('Ctrl Pts',(-1.3727145577519,0.661135169251343,
7.24307267954276));
#167965=CARTESIAN_POINT('Ctrl Pts',(-1.37575181232518,0.658505288582776,
7.25974488618265));
#167966=CARTESIAN_POINT('Ctrl Pts',(-1.37879884614972,0.655900535669628,
7.27641920769329));
#167967=CARTESIAN_POINT('Ctrl Pts',(-1.355651883,0.681369595,7.12212805100001));
#167968=CARTESIAN_POINT('Ctrl Pts',(-1.347163385,0.679970133,7.12374378300001));
#167969=CARTESIAN_POINT('Ctrl Pts',(-1.338671059,0.678571429,7.125339276));
#167970=CARTESIAN_POINT('Ctrl Pts',(-0.95805352,0.615882895,7.196847686));
#167971=CARTESIAN_POINT('Ctrl Pts',(-0.57198407,0.552026826,7.227401623));
#167972=CARTESIAN_POINT('Ctrl Pts',(-1.537156899,0.681369595,7.245585413));
#167973=CARTESIAN_POINT('Ctrl Pts',(-1.528521258,0.679970133,7.247417471));
#167974=CARTESIAN_POINT('Ctrl Pts',(-1.519881274,0.678571429,7.24922894));
#167975=CARTESIAN_POINT('Ctrl Pts',(-1.132645864,0.615882895,7.33041714));
#167976=CARTESIAN_POINT('Ctrl Pts',(-0.738965005000001,0.552026826,7.369890775));
#167977=CARTESIAN_POINT('',(-0.600037041950673,0.552026824384634,7.2513399406766));
#167978=CARTESIAN_POINT('Ctrl Pts',(-0.950940417999999,0.499686101,7.240157672));
#167979=CARTESIAN_POINT('Ctrl Pts',(-0.840165045,0.51775868,7.254707187));
#167980=CARTESIAN_POINT('Ctrl Pts',(-0.728996408,0.535714286,7.265860928));
#167981=CARTESIAN_POINT('Ctrl Pts',(-0.678575876,0.54385805,7.270919708));
#167982=CARTESIAN_POINT('Ctrl Pts',(-0.628089994,0.552026826,7.27527826));
#167983=CARTESIAN_POINT('Ctrl Pts',(-0.892761299,0.499686101,7.194822949));
#167984=CARTESIAN_POINT('Ctrl Pts',(-0.782679553,0.51775868,7.20848231500001));
#167985=CARTESIAN_POINT('Ctrl Pts',(-0.672231452,0.535714286,7.218767545));
#167986=CARTESIAN_POINT('Ctrl Pts',(-0.622137718,0.54385805,7.223432411));
#167987=CARTESIAN_POINT('Ctrl Pts',(-0.57198407,0.552026826,7.227401623));
#167988=CARTESIAN_POINT('Ctrl Pts',(-0.571984069433409,0.552026826253397,
7.22740162287586));
#167989=CARTESIAN_POINT('Ctrl Pts',(-0.605444369191663,0.546576979769284,
7.22475354004018));
#167990=CARTESIAN_POINT('Ctrl Pts',(-0.638861722984283,0.541139220276039,
7.22187502581563));
#167991=CARTESIAN_POINT('Ctrl Pts',(-0.672231451613071,0.535714286045145,
7.21876754515753));
#167992=CARTESIAN_POINT('Ctrl Pts',(-0.745099376405783,0.523868109062359,
7.21198188447546));
#167993=CARTESIAN_POINT('Ctrl Pts',(-0.817988928543338,0.511960760997416,
7.20408107381268));
#167994=CARTESIAN_POINT('Ctrl Pts',(-0.890849230764474,0.499999999848742,
7.19505994779791));
#167995=CARTESIAN_POINT('Ctrl Pts',(-0.892761299,0.499686101,7.194822949));
#167996=CARTESIAN_POINT('Ctrl Pts',(-0.782679553,0.51775868,7.20848231500001));
#167997=CARTESIAN_POINT('Ctrl Pts',(-0.672231452,0.535714286,7.218767545));
#167998=CARTESIAN_POINT('Ctrl Pts',(-0.621180069,0.544013736,7.22352159));
#167999=CARTESIAN_POINT('Ctrl Pts',(-0.570066555,0.552339147,7.227553121));
#168000=CARTESIAN_POINT('Ctrl Pts',(-0.853730891,0.499686101,7.244911592));
#168001=CARTESIAN_POINT('Ctrl Pts',(-0.742882782,0.51775868,7.257973788));
#168002=CARTESIAN_POINT('Ctrl Pts',(-0.631686945,0.535714286,7.267638682));
#168003=CARTESIAN_POINT('Ctrl Pts',(-0.580289944,0.544013736,7.27210599500001));
#168004=CARTESIAN_POINT('Ctrl Pts',(-0.528834902,0.552339147,7.275845934));
#168005=CARTESIAN_POINT('Ctrl Pts',(-0.57198406339264,0.552026827237287,
7.22740162335393));
#168006=CARTESIAN_POINT('Ctrl Pts',(-0.572436162740008,0.551172308319716,
7.23260486523954));
#168007=CARTESIAN_POINT('Ctrl Pts',(-0.572889187449938,0.550320535000218,
7.23780847285861));
#168008=CARTESIAN_POINT('Ctrl Pts',(-0.573343131559291,0.54947147810482,
7.24301244272147));
#168009=CARTESIAN_POINT('Ctrl Pts',(-0.573764556088678,0.548683245819846,
7.24784361137244));
#168010=CARTESIAN_POINT('Ctrl Pts',(-0.57418677311898,0.547897354498187,
7.25267509352273));
#168011=CARTESIAN_POINT('Ctrl Pts',(-0.574609773822212,0.547113782441845,
7.25750688254363));
#168012=CARTESIAN_POINT('Ctrl Pts',(-0.575032774952862,0.546330209593747,
7.26233867644677));
#168013=CARTESIAN_POINT('Ctrl Pts',(-0.57545655986563,0.545548955818372,
7.26717077843991));
#168014=CARTESIAN_POINT('Ctrl Pts',(-0.57588111869972,0.544769999874258,
7.27200318229781));
#168015=CARTESIAN_POINT('Ctrl Pts',(-0.573864989,0.55233793,7.227252519));
#168016=CARTESIAN_POINT('Ctrl Pts',(-0.415037848,0.526068113,7.239863859));
#168017=CARTESIAN_POINT('Ctrl Pts',(-0.255810014,0.49968693,7.24548557600001));
#168018=CARTESIAN_POINT('Ctrl Pts',(-0.622179465,0.55233793,7.268458786));
#168019=CARTESIAN_POINT('Ctrl Pts',(-0.462446769,0.526068113,7.282131892));
#168020=CARTESIAN_POINT('Ctrl Pts',(-0.30226761,0.49968693,7.288774568));
#168021=CARTESIAN_POINT('Origin',(-0.00779214677240493,0.410743181043314,
-0.196936069540853));
#168022=CARTESIAN_POINT('Ctrl Pts',(-0.527285648139283,0.552548454735263,
7.28327884871706));
#168023=CARTESIAN_POINT('Ctrl Pts',(-0.525696541069641,0.552287640367631,
7.28339319785853));
#168024=CARTESIAN_POINT('Ctrl Pts',(-0.524107434,0.552026826,7.283507547));
#168025=CARTESIAN_POINT('Ctrl Pts',(-0.364992249,0.525911829,7.294957175));
#168026=CARTESIAN_POINT('Ctrl Pts',(-0.205528848,0.49968693,7.299447149));
#168027=CARTESIAN_POINT('Ctrl Pts',(-0.575145653328268,0.552548454735263,
7.22714282424931));
#168028=CARTESIAN_POINT('Ctrl Pts',(-0.573568789395868,0.552287640367631,
7.22726762077373));
#168029=CARTESIAN_POINT('Ctrl Pts',(-0.571991925463469,0.552026826,7.22739241729816));
#168030=CARTESIAN_POINT('Ctrl Pts',(-0.414102629570901,0.525911829,7.23988812790829));
#168031=CARTESIAN_POINT('Ctrl Pts',(-0.255818263991973,0.49968693,7.24547672213723));
#168032=CARTESIAN_POINT('',(-0.500739504532394,0.552026824384634,7.31089209031286));
#168033=CARTESIAN_POINT('Ctrl Pts',(-0.5798133580548,0.550751630586317,
7.22678200501259));
#168034=CARTESIAN_POINT('Ctrl Pts',(-0.575898714027401,0.551389228293159,
7.2270918140063));
#168035=CARTESIAN_POINT('Ctrl Pts',(-0.57198407,0.552026826,7.227401623));
#168036=CARTESIAN_POINT('Ctrl Pts',(-0.178266631,0.61615356,7.25856083));
#168037=CARTESIAN_POINT('Ctrl Pts',(0.216505724,0.681389364000001,7.246766539));
#168038=CARTESIAN_POINT('Ctrl Pts',(-0.437505093897724,0.550751630586317,
7.39391729643459));
#168039=CARTESIAN_POINT('Ctrl Pts',(-0.433500006448862,0.551389228293159,
7.39414992771729));
#168040=CARTESIAN_POINT('Ctrl Pts',(-0.429494919,0.552026826,7.394382559));
#168041=CARTESIAN_POINT('Ctrl Pts',(-0.026681084,0.61615356,7.41777957600001));
#168042=CARTESIAN_POINT('Ctrl Pts',(0.37629064,0.681389364000001,7.397280897));
#168043=CARTESIAN_POINT('Origin',(-7.084,1.2,-7.084));
#168044=CARTESIAN_POINT('Origin',(-6.831,0.,6.831));
#170236=UNCERTAINTY_MEASURE_WITH_UNIT(LENGTH_MEASURE(0.01),#170251,
'DISTANCE_ACCURACY_VALUE',
'Maximum model space distance between geometric entities at asserted c
onnectivities');
#170242=UNCERTAINTY_MEASURE_WITH_UNIT(LENGTH_MEASURE(0.01),#170251,
'DISTANCE_ACCURACY_VALUE',
'Maximum model space distance between geometric entities at asserted c
onnectivities');
#170244=(
GEOMETRIC_REPRESENTATION_CONTEXT(3)
GLOBAL_UNCERTAINTY_ASSIGNED_CONTEXT((#170236))
GLOBAL_UNIT_ASSIGNED_CONTEXT((#170251,#170253,#170254))
REPRESENTATION_CONTEXT('','3D')
);
#170250=(
GEOMETRIC_REPRESENTATION_CONTEXT(3)
GLOBAL_UNCERTAINTY_ASSIGNED_CONTEXT((#170242))
GLOBAL_UNIT_ASSIGNED_CONTEXT((#170251,#170253,#170254))
REPRESENTATION_CONTEXT('','3D')
);
#170251=(
LENGTH_UNIT()
NAMED_UNIT(*)
SI_UNIT(.MILLI.,.METRE.)
);
#170253=(
NAMED_UNIT(*)
PLANE_ANGLE_UNIT()
SI_UNIT($,.RADIAN.)
);
#170254=(
NAMED_UNIT(*)
SI_UNIT($,.STERADIAN.)
SOLID_ANGLE_UNIT()
);
#170256=SHAPE_DEFINITION_REPRESENTATION(#170263,#170276);
#170263=PRODUCT_DEFINITION_SHAPE('',$,#170284);
#170276=SHAPE_REPRESENTATION('',(#71472),#170244);
#170282=PRODUCT_DEFINITION_CONTEXT('part definition',#170305,'design');
#170284=PRODUCT_DEFINITION('2026-11-14-09-55-10-334',
'Adjustable Thread',#170291,#170282);
#170291=PRODUCT_DEFINITION_FORMATION('',$,#170308);
#170305=APPLICATION_CONTEXT(
'Core Data for Automotive Mechanical Design Process');
#170306=PRODUCT_CONTEXT('part definition',#170305,'mechanical');
#170308=PRODUCT('2026-11-14-09-55-10-334','Adjustable Thread',$,(#170306));
#170315=PRESENTATION_STYLE_ASSIGNMENT((#170319));
#170319=SURFACE_STYLE_USAGE(.BOTH.,#170323);
#170323=SURFACE_SIDE_STYLE('',(#170327));
#170327=SURFACE_STYLE_FILL_AREA(#170331);
#170331=FILL_AREA_STYLE('Opaque(227,224,212)',(#170335));
#170335=FILL_AREA_STYLE_COLOUR('Opaque(227,224,212)',#170339);
#170339=COLOUR_RGB('Opaque(227,224,212)',0.890196078431372,0.87843137254902,
0.831372549019608);
ENDSEC;
END-ISO-10303-21;
